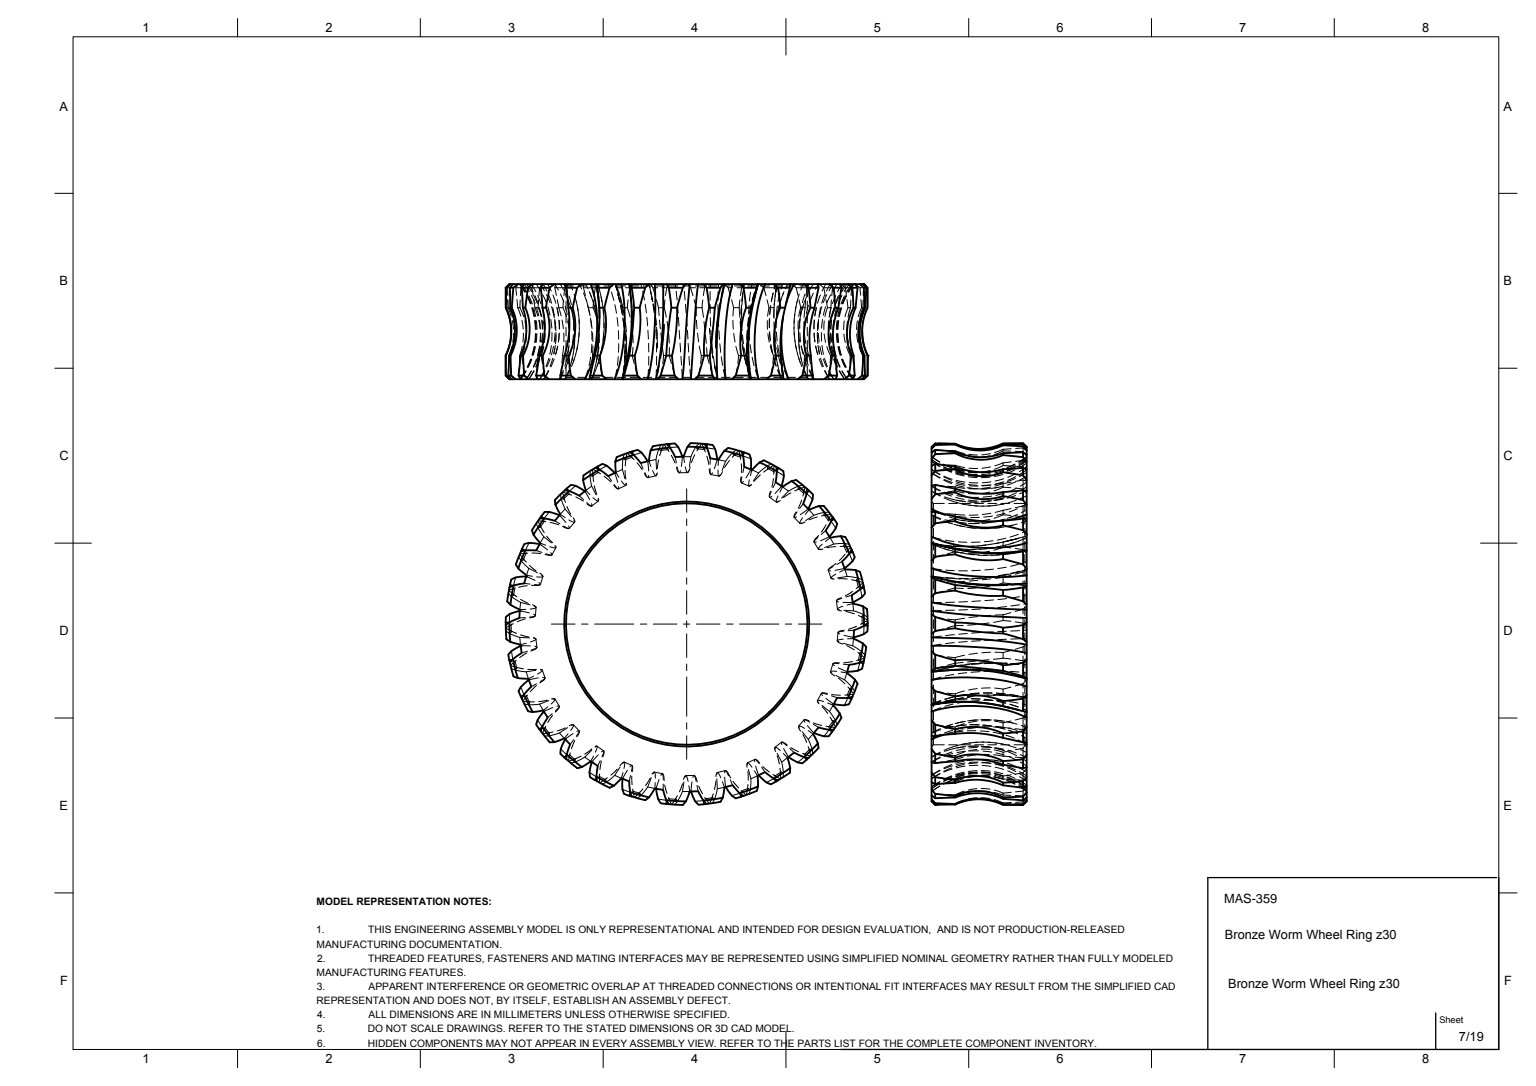
ISO-10303-21;
HEADER;
/* Generated by software containing ST-Developer
 * from STEP Tools, Inc. (www.steptools.com) 
 */

FILE_DESCRIPTION(
/* description */ (''),
/* implementation_level */ '2;1');

FILE_NAME(
/* name */ 'Bronze Worm Wheel Ring z30.step',
/* time_stamp */ '2026-10-15T14:25:16-07:00',
/* author */ (''),
/* organization */ (''),
/* preprocessor_version */ 'ST-DEVELOPER v20.2',
/* originating_system */ 'Autodesk Translation Framework v15.15.0.0',
/* authorisation */ '');

FILE_SCHEMA (('AUTOMOTIVE_DESIGN { 1 0 10303 214 3 1 1 }'));
ENDSEC;

DATA;
#10=MECHANICAL_DESIGN_GEOMETRIC_PRESENTATION_REPRESENTATION('',(#327),#86429);
#127=TOROIDAL_SURFACE('',#16553,6.3,1.5);
#128=TOROIDAL_SURFACE('',#16562,6.3,1.5);
#129=TOROIDAL_SURFACE('',#16571,6.3,1.5);
#130=TOROIDAL_SURFACE('',#16580,6.3,1.5);
#131=TOROIDAL_SURFACE('',#16589,6.3,1.5);
#132=TOROIDAL_SURFACE('',#16598,6.3,1.5);
#133=TOROIDAL_SURFACE('',#16607,6.3,1.5);
#134=TOROIDAL_SURFACE('',#16616,6.3,1.5);
#135=TOROIDAL_SURFACE('',#16625,6.3,1.5);
#136=TOROIDAL_SURFACE('',#16634,6.3,1.5);
#137=TOROIDAL_SURFACE('',#16643,6.3,1.5);
#138=TOROIDAL_SURFACE('',#16652,6.3,1.5);
#139=TOROIDAL_SURFACE('',#16661,6.3,1.5);
#140=TOROIDAL_SURFACE('',#16670,6.3,1.5);
#141=TOROIDAL_SURFACE('',#16679,6.3,1.5);
#142=TOROIDAL_SURFACE('',#16688,6.3,1.5);
#143=TOROIDAL_SURFACE('',#16697,6.3,1.5);
#144=TOROIDAL_SURFACE('',#16706,6.3,1.5);
#145=TOROIDAL_SURFACE('',#16715,6.3,1.5);
#146=TOROIDAL_SURFACE('',#16724,6.3,1.5);
#147=TOROIDAL_SURFACE('',#16733,6.3,1.5);
#148=TOROIDAL_SURFACE('',#16742,6.3,1.5);
#149=TOROIDAL_SURFACE('',#16751,6.3,1.5);
#150=TOROIDAL_SURFACE('',#16760,6.3,1.5);
#151=TOROIDAL_SURFACE('',#16769,6.3,1.5);
#152=TOROIDAL_SURFACE('',#16778,6.3,1.5);
#153=TOROIDAL_SURFACE('',#16787,6.3,1.5);
#154=TOROIDAL_SURFACE('',#16798,6.3,1.5);
#155=TOROIDAL_SURFACE('',#16811,6.3,1.5);
#156=TOROIDAL_SURFACE('',#16817,6.3,1.5);
#164=B_SPLINE_SURFACE_WITH_KNOTS('',3,3,((#29446,#29447,#29448,#29449,#29450,
#29451,#29452,#29453,#29454,#29455,#29456,#29457,#29458,#29459),(#29460,
#29461,#29462,#29463,#29464,#29465,#29466,#29467,#29468,#29469,#29470,#29471,
#29472,#29473),(#29474,#29475,#29476,#29477,#29478,#29479,#29480,#29481,
#29482,#29483,#29484,#29485,#29486,#29487),(#29488,#29489,#29490,#29491,
#29492,#29493,#29494,#29495,#29496,#29497,#29498,#29499,#29500,#29501),
(#29502,#29503,#29504,#29505,#29506,#29507,#29508,#29509,#29510,#29511,
#29512,#29513,#29514,#29515),(#29516,#29517,#29518,#29519,#29520,#29521,
#29522,#29523,#29524,#29525,#29526,#29527,#29528,#29529),(#29530,#29531,
#29532,#29533,#29534,#29535,#29536,#29537,#29538,#29539,#29540,#29541,#29542,
#29543),(#29544,#29545,#29546,#29547,#29548,#29549,#29550,#29551,#29552,
#29553,#29554,#29555,#29556,#29557),(#29558,#29559,#29560,#29561,#29562,
#29563,#29564,#29565,#29566,#29567,#29568,#29569,#29570,#29571),(#29572,
#29573,#29574,#29575,#29576,#29577,#29578,#29579,#29580,#29581,#29582,#29583,
#29584,#29585),(#29586,#29587,#29588,#29589,#29590,#29591,#29592,#29593,
#29594,#29595,#29596,#29597,#29598,#29599),(#29600,#29601,#29602,#29603,
#29604,#29605,#29606,#29607,#29608,#29609,#29610,#29611,#29612,#29613),
(#29614,#29615,#29616,#29617,#29618,#29619,#29620,#29621,#29622,#29623,
#29624,#29625,#29626,#29627),(#29628,#29629,#29630,#29631,#29632,#29633,
#29634,#29635,#29636,#29637,#29638,#29639,#29640,#29641),(#29642,#29643,
#29644,#29645,#29646,#29647,#29648,#29649,#29650,#29651,#29652,#29653,#29654,
#29655),(#29656,#29657,#29658,#29659,#29660,#29661,#29662,#29663,#29664,
#29665,#29666,#29667,#29668,#29669),(#29670,#29671,#29672,#29673,#29674,
#29675,#29676,#29677,#29678,#29679,#29680,#29681,#29682,#29683),(#29684,
#29685,#29686,#29687,#29688,#29689,#29690,#29691,#29692,#29693,#29694,#29695,
#29696,#29697),(#29698,#29699,#29700,#29701,#29702,#29703,#29704,#29705,
#29706,#29707,#29708,#29709,#29710,#29711),(#29712,#29713,#29714,#29715,
#29716,#29717,#29718,#29719,#29720,#29721,#29722,#29723,#29724,#29725),
(#29726,#29727,#29728,#29729,#29730,#29731,#29732,#29733,#29734,#29735,
#29736,#29737,#29738,#29739),(#29740,#29741,#29742,#29743,#29744,#29745,
#29746,#29747,#29748,#29749,#29750,#29751,#29752,#29753),(#29754,#29755,
#29756,#29757,#29758,#29759,#29760,#29761,#29762,#29763,#29764,#29765,#29766,
#29767),(#29768,#29769,#29770,#29771,#29772,#29773,#29774,#29775,#29776,
#29777,#29778,#29779,#29780,#29781),(#29782,#29783,#29784,#29785,#29786,
#29787,#29788,#29789,#29790,#29791,#29792,#29793,#29794,#29795),(#29796,
#29797,#29798,#29799,#29800,#29801,#29802,#29803,#29804,#29805,#29806,#29807,
#29808,#29809),(#29810,#29811,#29812,#29813,#29814,#29815,#29816,#29817,
#29818,#29819,#29820,#29821,#29822,#29823),(#29824,#29825,#29826,#29827,
#29828,#29829,#29830,#29831,#29832,#29833,#29834,#29835,#29836,#29837),
(#29838,#29839,#29840,#29841,#29842,#29843,#29844,#29845,#29846,#29847,
#29848,#29849,#29850,#29851),(#29852,#29853,#29854,#29855,#29856,#29857,
#29858,#29859,#29860,#29861,#29862,#29863,#29864,#29865),(#29866,#29867,
#29868,#29869,#29870,#29871,#29872,#29873,#29874,#29875,#29876,#29877,#29878,
#29879),(#29880,#29881,#29882,#29883,#29884,#29885,#29886,#29887,#29888,
#29889,#29890,#29891,#29892,#29893),(#29894,#29895,#29896,#29897,#29898,
#29899,#29900,#29901,#29902,#29903,#29904,#29905,#29906,#29907),(#29908,
#29909,#29910,#29911,#29912,#29913,#29914,#29915,#29916,#29917,#29918,#29919,
#29920,#29921)),.UNSPECIFIED.,.F.,.F.,.F.,(4,1,1,1,1,1,1,1,1,1,1,1,1,1,
1,1,1,1,1,1,1,1,1,1,1,1,1,1,1,1,1,4),(4,2,2,2,2,2,4),(0.0331549352864052,
0.102215297051662,0.171275658816919,0.172354726969501,0.173433795122083,
0.174512863274665,0.175591931427247,0.179908204037576,0.188540749258233,
0.19717329447889,0.205805839699547,0.223070930140861,0.240336020582176,
0.274866201464804,0.309396382347432,0.378456744112689,0.412986924995318,
0.447517105877946,0.482047286760574,0.516577467643203,0.551107648525831,
0.568372738967145,0.585637829408459,0.654698191173716,0.723758552938973,
0.79281891470423,0.827349095586858,0.861879276469487,0.896409457352115,
0.930939638234743,0.948204728676057,1.),(0.0377143719370964,0.167070624995476,
0.336553194126115,0.499999999999991,0.663446805873868,0.832929375004528,
0.962285628058762),.UNSPECIFIED.);
#165=B_SPLINE_SURFACE_WITH_KNOTS('',3,3,((#29982,#29983,#29984,#29985,#29986,
#29987,#29988,#29989,#29990,#29991,#29992,#29993,#29994,#29995),(#29996,
#29997,#29998,#29999,#30000,#30001,#30002,#30003,#30004,#30005,#30006,#30007,
#30008,#30009),(#30010,#30011,#30012,#30013,#30014,#30015,#30016,#30017,
#30018,#30019,#30020,#30021,#30022,#30023),(#30024,#30025,#30026,#30027,
#30028,#30029,#30030,#30031,#30032,#30033,#30034,#30035,#30036,#30037)),
 .UNSPECIFIED.,.F.,.F.,.F.,(4,4),(4,2,2,2,2,2,4),(0.,1.),(0.0377143719414207,
0.167070624995476,0.336553194126115,0.499999999999991,0.663446805873868,
0.832929375004528,0.962285628058582),.UNSPECIFIED.);
#166=B_SPLINE_SURFACE_WITH_KNOTS('',3,3,((#30052,#30053,#30054,#30055,#30056,
#30057,#30058,#30059,#30060,#30061,#30062,#30063,#30064,#30065),(#30066,
#30067,#30068,#30069,#30070,#30071,#30072,#30073,#30074,#30075,#30076,#30077,
#30078,#30079),(#30080,#30081,#30082,#30083,#30084,#30085,#30086,#30087,
#30088,#30089,#30090,#30091,#30092,#30093),(#30094,#30095,#30096,#30097,
#30098,#30099,#30100,#30101,#30102,#30103,#30104,#30105,#30106,#30107),
(#30108,#30109,#30110,#30111,#30112,#30113,#30114,#30115,#30116,#30117,
#30118,#30119,#30120,#30121),(#30122,#30123,#30124,#30125,#30126,#30127,
#30128,#30129,#30130,#30131,#30132,#30133,#30134,#30135),(#30136,#30137,
#30138,#30139,#30140,#30141,#30142,#30143,#30144,#30145,#30146,#30147,#30148,
#30149),(#30150,#30151,#30152,#30153,#30154,#30155,#30156,#30157,#30158,
#30159,#30160,#30161,#30162,#30163),(#30164,#30165,#30166,#30167,#30168,
#30169,#30170,#30171,#30172,#30173,#30174,#30175,#30176,#30177),(#30178,
#30179,#30180,#30181,#30182,#30183,#30184,#30185,#30186,#30187,#30188,#30189,
#30190,#30191),(#30192,#30193,#30194,#30195,#30196,#30197,#30198,#30199,
#30200,#30201,#30202,#30203,#30204,#30205),(#30206,#30207,#30208,#30209,
#30210,#30211,#30212,#30213,#30214,#30215,#30216,#30217,#30218,#30219),
(#30220,#30221,#30222,#30223,#30224,#30225,#30226,#30227,#30228,#30229,
#30230,#30231,#30232,#30233),(#30234,#30235,#30236,#30237,#30238,#30239,
#30240,#30241,#30242,#30243,#30244,#30245,#30246,#30247),(#30248,#30249,
#30250,#30251,#30252,#30253,#30254,#30255,#30256,#30257,#30258,#30259,#30260,
#30261),(#30262,#30263,#30264,#30265,#30266,#30267,#30268,#30269,#30270,
#30271,#30272,#30273,#30274,#30275),(#30276,#30277,#30278,#30279,#30280,
#30281,#30282,#30283,#30284,#30285,#30286,#30287,#30288,#30289),(#30290,
#30291,#30292,#30293,#30294,#30295,#30296,#30297,#30298,#30299,#30300,#30301,
#30302,#30303),(#30304,#30305,#30306,#30307,#30308,#30309,#30310,#30311,
#30312,#30313,#30314,#30315,#30316,#30317),(#30318,#30319,#30320,#30321,
#30322,#30323,#30324,#30325,#30326,#30327,#30328,#30329,#30330,#30331),
(#30332,#30333,#30334,#30335,#30336,#30337,#30338,#30339,#30340,#30341,
#30342,#30343,#30344,#30345),(#30346,#30347,#30348,#30349,#30350,#30351,
#30352,#30353,#30354,#30355,#30356,#30357,#30358,#30359),(#30360,#30361,
#30362,#30363,#30364,#30365,#30366,#30367,#30368,#30369,#30370,#30371,#30372,
#30373),(#30374,#30375,#30376,#30377,#30378,#30379,#30380,#30381,#30382,
#30383,#30384,#30385,#30386,#30387),(#30388,#30389,#30390,#30391,#30392,
#30393,#30394,#30395,#30396,#30397,#30398,#30399,#30400,#30401),(#30402,
#30403,#30404,#30405,#30406,#30407,#30408,#30409,#30410,#30411,#30412,#30413,
#30414,#30415),(#30416,#30417,#30418,#30419,#30420,#30421,#30422,#30423,
#30424,#30425,#30426,#30427,#30428,#30429),(#30430,#30431,#30432,#30433,
#30434,#30435,#30436,#30437,#30438,#30439,#30440,#30441,#30442,#30443),
(#30444,#30445,#30446,#30447,#30448,#30449,#30450,#30451,#30452,#30453,
#30454,#30455,#30456,#30457),(#30458,#30459,#30460,#30461,#30462,#30463,
#30464,#30465,#30466,#30467,#30468,#30469,#30470,#30471),(#30472,#30473,
#30474,#30475,#30476,#30477,#30478,#30479,#30480,#30481,#30482,#30483,#30484,
#30485),(#30486,#30487,#30488,#30489,#30490,#30491,#30492,#30493,#30494,
#30495,#30496,#30497,#30498,#30499),(#30500,#30501,#30502,#30503,#30504,
#30505,#30506,#30507,#30508,#30509,#30510,#30511,#30512,#30513),(#30514,
#30515,#30516,#30517,#30518,#30519,#30520,#30521,#30522,#30523,#30524,#30525,
#30526,#30527),(#30528,#30529,#30530,#30531,#30532,#30533,#30534,#30535,
#30536,#30537,#30538,#30539,#30540,#30541),(#30542,#30543,#30544,#30545,
#30546,#30547,#30548,#30549,#30550,#30551,#30552,#30553,#30554,#30555),
(#30556,#30557,#30558,#30559,#30560,#30561,#30562,#30563,#30564,#30565,
#30566,#30567,#30568,#30569)),.UNSPECIFIED.,.F.,.F.,.F.,(4,1,1,1,1,1,1,
1,1,1,1,1,1,1,1,1,1,1,1,1,1,1,1,1,1,1,1,1,1,1,1,1,1,1,4),(4,2,2,2,2,2,4),
(0.,0.0517952713240545,0.069060361765406,0.103590542648109,0.138120723530812,
0.146753268751488,0.155385813972164,0.189915994854866,0.276241447061624,
0.34530180882703,0.379831989709733,0.414362170592436,0.448892351475139,
0.46615744191649,0.483422532357842,0.552482894123248,0.587013075005951,
0.621543255888654,0.69060361765406,0.759663979419466,0.776929069860817,
0.794194160302169,0.802826705522845,0.81145925074352,0.815775523353858,
0.820091795964196,0.822249932269365,0.824408068574534,0.826566204879703,
0.827645273032287,0.82818480710858,0.828724341184872,0.897784702950278,
0.932314883832981,0.966845064715684),(0.037714371941,0.167070624995476,
0.336553194126115,0.499999999999991,0.663446805873868,0.832929375004528,
0.962285628058665),.UNSPECIFIED.);
#167=B_SPLINE_SURFACE_WITH_KNOTS('',3,3,((#30669,#30670,#30671,#30672,#30673,
#30674,#30675,#30676,#30677,#30678,#30679,#30680,#30681,#30682),(#30683,
#30684,#30685,#30686,#30687,#30688,#30689,#30690,#30691,#30692,#30693,#30694,
#30695,#30696),(#30697,#30698,#30699,#30700,#30701,#30702,#30703,#30704,
#30705,#30706,#30707,#30708,#30709,#30710),(#30711,#30712,#30713,#30714,
#30715,#30716,#30717,#30718,#30719,#30720,#30721,#30722,#30723,#30724),
(#30725,#30726,#30727,#30728,#30729,#30730,#30731,#30732,#30733,#30734,
#30735,#30736,#30737,#30738),(#30739,#30740,#30741,#30742,#30743,#30744,
#30745,#30746,#30747,#30748,#30749,#30750,#30751,#30752),(#30753,#30754,
#30755,#30756,#30757,#30758,#30759,#30760,#30761,#30762,#30763,#30764,#30765,
#30766),(#30767,#30768,#30769,#30770,#30771,#30772,#30773,#30774,#30775,
#30776,#30777,#30778,#30779,#30780),(#30781,#30782,#30783,#30784,#30785,
#30786,#30787,#30788,#30789,#30790,#30791,#30792,#30793,#30794),(#30795,
#30796,#30797,#30798,#30799,#30800,#30801,#30802,#30803,#30804,#30805,#30806,
#30807,#30808),(#30809,#30810,#30811,#30812,#30813,#30814,#30815,#30816,
#30817,#30818,#30819,#30820,#30821,#30822),(#30823,#30824,#30825,#30826,
#30827,#30828,#30829,#30830,#30831,#30832,#30833,#30834,#30835,#30836),
(#30837,#30838,#30839,#30840,#30841,#30842,#30843,#30844,#30845,#30846,
#30847,#30848,#30849,#30850),(#30851,#30852,#30853,#30854,#30855,#30856,
#30857,#30858,#30859,#30860,#30861,#30862,#30863,#30864),(#30865,#30866,
#30867,#30868,#30869,#30870,#30871,#30872,#30873,#30874,#30875,#30876,#30877,
#30878),(#30879,#30880,#30881,#30882,#30883,#30884,#30885,#30886,#30887,
#30888,#30889,#30890,#30891,#30892),(#30893,#30894,#30895,#30896,#30897,
#30898,#30899,#30900,#30901,#30902,#30903,#30904,#30905,#30906),(#30907,
#30908,#30909,#30910,#30911,#30912,#30913,#30914,#30915,#30916,#30917,#30918,
#30919,#30920),(#30921,#30922,#30923,#30924,#30925,#30926,#30927,#30928,
#30929,#30930,#30931,#30932,#30933,#30934),(#30935,#30936,#30937,#30938,
#30939,#30940,#30941,#30942,#30943,#30944,#30945,#30946,#30947,#30948),
(#30949,#30950,#30951,#30952,#30953,#30954,#30955,#30956,#30957,#30958,
#30959,#30960,#30961,#30962),(#30963,#30964,#30965,#30966,#30967,#30968,
#30969,#30970,#30971,#30972,#30973,#30974,#30975,#30976),(#30977,#30978,
#30979,#30980,#30981,#30982,#30983,#30984,#30985,#30986,#30987,#30988,#30989,
#30990),(#30991,#30992,#30993,#30994,#30995,#30996,#30997,#30998,#30999,
#31000,#31001,#31002,#31003,#31004),(#31005,#31006,#31007,#31008,#31009,
#31010,#31011,#31012,#31013,#31014,#31015,#31016,#31017,#31018),(#31019,
#31020,#31021,#31022,#31023,#31024,#31025,#31026,#31027,#31028,#31029,#31030,
#31031,#31032),(#31033,#31034,#31035,#31036,#31037,#31038,#31039,#31040,
#31041,#31042,#31043,#31044,#31045,#31046),(#31047,#31048,#31049,#31050,
#31051,#31052,#31053,#31054,#31055,#31056,#31057,#31058,#31059,#31060),
(#31061,#31062,#31063,#31064,#31065,#31066,#31067,#31068,#31069,#31070,
#31071,#31072,#31073,#31074),(#31075,#31076,#31077,#31078,#31079,#31080,
#31081,#31082,#31083,#31084,#31085,#31086,#31087,#31088),(#31089,#31090,
#31091,#31092,#31093,#31094,#31095,#31096,#31097,#31098,#31099,#31100,#31101,
#31102),(#31103,#31104,#31105,#31106,#31107,#31108,#31109,#31110,#31111,
#31112,#31113,#31114,#31115,#31116),(#31117,#31118,#31119,#31120,#31121,
#31122,#31123,#31124,#31125,#31126,#31127,#31128,#31129,#31130),(#31131,
#31132,#31133,#31134,#31135,#31136,#31137,#31138,#31139,#31140,#31141,#31142,
#31143,#31144),(#31145,#31146,#31147,#31148,#31149,#31150,#31151,#31152,
#31153,#31154,#31155,#31156,#31157,#31158),(#31159,#31160,#31161,#31162,
#31163,#31164,#31165,#31166,#31167,#31168,#31169,#31170,#31171,#31172)),
 .UNSPECIFIED.,.F.,.F.,.F.,(4,1,1,1,1,1,1,1,1,1,1,1,1,1,1,1,1,1,1,1,1,1,
1,1,1,1,1,1,1,1,1,1,1,4),(4,2,2,2,2,2,4),(0.033154935286399,0.0676851161690276,
0.102215297051656,0.171275658816913,0.172354726969496,0.173433795122078,
0.17451286327466,0.175591931427242,0.179908204037571,0.188540749258228,
0.197173294478885,0.205805839699542,0.223070930140856,0.240336020582171,
0.274866201464799,0.309396382347428,0.378456744112685,0.412986924995314,
0.447517105877942,0.482047286760571,0.5165774676432,0.551107648525828,0.568372738967142,
0.585637829408457,0.654698191173714,0.706493462497657,0.723758552938971,
0.792818914704228,0.827349095586857,0.861879276469486,0.896409457352114,
0.930939638234743,0.948204728676057,1.),(0.0377143719407808,0.167070624995476,
0.336553194126115,0.499999999999991,0.663446805873868,0.832929375004528,
0.962285628059334),.UNSPECIFIED.);
#168=B_SPLINE_SURFACE_WITH_KNOTS('',3,3,((#31237,#31238,#31239,#31240,#31241,
#31242,#31243,#31244,#31245,#31246,#31247,#31248,#31249,#31250),(#31251,
#31252,#31253,#31254,#31255,#31256,#31257,#31258,#31259,#31260,#31261,#31262,
#31263,#31264),(#31265,#31266,#31267,#31268,#31269,#31270,#31271,#31272,
#31273,#31274,#31275,#31276,#31277,#31278),(#31279,#31280,#31281,#31282,
#31283,#31284,#31285,#31286,#31287,#31288,#31289,#31290,#31291,#31292)),
 .UNSPECIFIED.,.F.,.F.,.F.,(4,4),(4,2,2,2,2,2,4),(0.,1.),(0.0377143719414207,
0.167070624995476,0.336553194126115,0.499999999999991,0.663446805873868,
0.832929375004528,0.962285628058582),.UNSPECIFIED.);
#169=B_SPLINE_SURFACE_WITH_KNOTS('',3,3,((#31307,#31308,#31309,#31310,#31311,
#31312,#31313,#31314,#31315,#31316,#31317,#31318,#31319,#31320),(#31321,
#31322,#31323,#31324,#31325,#31326,#31327,#31328,#31329,#31330,#31331,#31332,
#31333,#31334),(#31335,#31336,#31337,#31338,#31339,#31340,#31341,#31342,
#31343,#31344,#31345,#31346,#31347,#31348),(#31349,#31350,#31351,#31352,
#31353,#31354,#31355,#31356,#31357,#31358,#31359,#31360,#31361,#31362),
(#31363,#31364,#31365,#31366,#31367,#31368,#31369,#31370,#31371,#31372,
#31373,#31374,#31375,#31376),(#31377,#31378,#31379,#31380,#31381,#31382,
#31383,#31384,#31385,#31386,#31387,#31388,#31389,#31390),(#31391,#31392,
#31393,#31394,#31395,#31396,#31397,#31398,#31399,#31400,#31401,#31402,#31403,
#31404),(#31405,#31406,#31407,#31408,#31409,#31410,#31411,#31412,#31413,
#31414,#31415,#31416,#31417,#31418),(#31419,#31420,#31421,#31422,#31423,
#31424,#31425,#31426,#31427,#31428,#31429,#31430,#31431,#31432),(#31433,
#31434,#31435,#31436,#31437,#31438,#31439,#31440,#31441,#31442,#31443,#31444,
#31445,#31446),(#31447,#31448,#31449,#31450,#31451,#31452,#31453,#31454,
#31455,#31456,#31457,#31458,#31459,#31460),(#31461,#31462,#31463,#31464,
#31465,#31466,#31467,#31468,#31469,#31470,#31471,#31472,#31473,#31474),
(#31475,#31476,#31477,#31478,#31479,#31480,#31481,#31482,#31483,#31484,
#31485,#31486,#31487,#31488),(#31489,#31490,#31491,#31492,#31493,#31494,
#31495,#31496,#31497,#31498,#31499,#31500,#31501,#31502),(#31503,#31504,
#31505,#31506,#31507,#31508,#31509,#31510,#31511,#31512,#31513,#31514,#31515,
#31516),(#31517,#31518,#31519,#31520,#31521,#31522,#31523,#31524,#31525,
#31526,#31527,#31528,#31529,#31530),(#31531,#31532,#31533,#31534,#31535,
#31536,#31537,#31538,#31539,#31540,#31541,#31542,#31543,#31544),(#31545,
#31546,#31547,#31548,#31549,#31550,#31551,#31552,#31553,#31554,#31555,#31556,
#31557,#31558),(#31559,#31560,#31561,#31562,#31563,#31564,#31565,#31566,
#31567,#31568,#31569,#31570,#31571,#31572),(#31573,#31574,#31575,#31576,
#31577,#31578,#31579,#31580,#31581,#31582,#31583,#31584,#31585,#31586),
(#31587,#31588,#31589,#31590,#31591,#31592,#31593,#31594,#31595,#31596,
#31597,#31598,#31599,#31600),(#31601,#31602,#31603,#31604,#31605,#31606,
#31607,#31608,#31609,#31610,#31611,#31612,#31613,#31614),(#31615,#31616,
#31617,#31618,#31619,#31620,#31621,#31622,#31623,#31624,#31625,#31626,#31627,
#31628),(#31629,#31630,#31631,#31632,#31633,#31634,#31635,#31636,#31637,
#31638,#31639,#31640,#31641,#31642),(#31643,#31644,#31645,#31646,#31647,
#31648,#31649,#31650,#31651,#31652,#31653,#31654,#31655,#31656),(#31657,
#31658,#31659,#31660,#31661,#31662,#31663,#31664,#31665,#31666,#31667,#31668,
#31669,#31670),(#31671,#31672,#31673,#31674,#31675,#31676,#31677,#31678,
#31679,#31680,#31681,#31682,#31683,#31684),(#31685,#31686,#31687,#31688,
#31689,#31690,#31691,#31692,#31693,#31694,#31695,#31696,#31697,#31698),
(#31699,#31700,#31701,#31702,#31703,#31704,#31705,#31706,#31707,#31708,
#31709,#31710,#31711,#31712),(#31713,#31714,#31715,#31716,#31717,#31718,
#31719,#31720,#31721,#31722,#31723,#31724,#31725,#31726),(#31727,#31728,
#31729,#31730,#31731,#31732,#31733,#31734,#31735,#31736,#31737,#31738,#31739,
#31740),(#31741,#31742,#31743,#31744,#31745,#31746,#31747,#31748,#31749,
#31750,#31751,#31752,#31753,#31754),(#31755,#31756,#31757,#31758,#31759,
#31760,#31761,#31762,#31763,#31764,#31765,#31766,#31767,#31768),(#31769,
#31770,#31771,#31772,#31773,#31774,#31775,#31776,#31777,#31778,#31779,#31780,
#31781,#31782),(#31783,#31784,#31785,#31786,#31787,#31788,#31789,#31790,
#31791,#31792,#31793,#31794,#31795,#31796),(#31797,#31798,#31799,#31800,
#31801,#31802,#31803,#31804,#31805,#31806,#31807,#31808,#31809,#31810),
(#31811,#31812,#31813,#31814,#31815,#31816,#31817,#31818,#31819,#31820,
#31821,#31822,#31823,#31824),(#31825,#31826,#31827,#31828,#31829,#31830,
#31831,#31832,#31833,#31834,#31835,#31836,#31837,#31838),(#31839,#31840,
#31841,#31842,#31843,#31844,#31845,#31846,#31847,#31848,#31849,#31850,#31851,
#31852),(#31853,#31854,#31855,#31856,#31857,#31858,#31859,#31860,#31861,
#31862,#31863,#31864,#31865,#31866),(#31867,#31868,#31869,#31870,#31871,
#31872,#31873,#31874,#31875,#31876,#31877,#31878,#31879,#31880)),
 .UNSPECIFIED.,.F.,.F.,.F.,(4,1,1,1,1,1,1,1,1,1,1,1,1,1,1,1,1,1,1,1,1,1,
1,1,1,1,1,1,1,1,1,1,1,1,1,1,1,1,4),(4,2,2,2,2,2,4),(0.,0.0517952713240545,
0.069060361765406,0.103590542648109,0.138120723530812,0.155385813972164,
0.172650904413515,0.207181085296218,0.276241447061624,0.34530180882703,
0.379831989709733,0.414362170592436,0.448892351475139,0.483422532357842,
0.552482894123248,0.5697479845646,0.621543255888654,0.638808346330006,0.69060361765406,
0.707868708095412,0.716501253316088,0.725133798536763,0.759663979419467,
0.768296524640142,0.776929069860818,0.79419416030217,0.802826705522845,
0.811459250743521,0.820091795964197,0.824408068574535,0.825487136727119,
0.826566204879704,0.827645273032288,0.82818480710858,0.828454574146726,
0.828724341184873,0.897784702950279,0.932314883832982,0.966845064715685),
(0.0377143719412118,0.167070624995476,0.336553194126115,0.499999999999991,
0.663446805873868,0.832929375004528,0.962285628060063),.UNSPECIFIED.);
#170=B_SPLINE_SURFACE_WITH_KNOTS('',3,3,((#31940,#31941,#31942,#31943,#31944,
#31945,#31946,#31947,#31948,#31949,#31950,#31951,#31952,#31953),(#31954,
#31955,#31956,#31957,#31958,#31959,#31960,#31961,#31962,#31963,#31964,#31965,
#31966,#31967),(#31968,#31969,#31970,#31971,#31972,#31973,#31974,#31975,
#31976,#31977,#31978,#31979,#31980,#31981),(#31982,#31983,#31984,#31985,
#31986,#31987,#31988,#31989,#31990,#31991,#31992,#31993,#31994,#31995),
(#31996,#31997,#31998,#31999,#32000,#32001,#32002,#32003,#32004,#32005,
#32006,#32007,#32008,#32009),(#32010,#32011,#32012,#32013,#32014,#32015,
#32016,#32017,#32018,#32019,#32020,#32021,#32022,#32023),(#32024,#32025,
#32026,#32027,#32028,#32029,#32030,#32031,#32032,#32033,#32034,#32035,#32036,
#32037),(#32038,#32039,#32040,#32041,#32042,#32043,#32044,#32045,#32046,
#32047,#32048,#32049,#32050,#32051),(#32052,#32053,#32054,#32055,#32056,
#32057,#32058,#32059,#32060,#32061,#32062,#32063,#32064,#32065),(#32066,
#32067,#32068,#32069,#32070,#32071,#32072,#32073,#32074,#32075,#32076,#32077,
#32078,#32079),(#32080,#32081,#32082,#32083,#32084,#32085,#32086,#32087,
#32088,#32089,#32090,#32091,#32092,#32093),(#32094,#32095,#32096,#32097,
#32098,#32099,#32100,#32101,#32102,#32103,#32104,#32105,#32106,#32107),
(#32108,#32109,#32110,#32111,#32112,#32113,#32114,#32115,#32116,#32117,
#32118,#32119,#32120,#32121),(#32122,#32123,#32124,#32125,#32126,#32127,
#32128,#32129,#32130,#32131,#32132,#32133,#32134,#32135),(#32136,#32137,
#32138,#32139,#32140,#32141,#32142,#32143,#32144,#32145,#32146,#32147,#32148,
#32149),(#32150,#32151,#32152,#32153,#32154,#32155,#32156,#32157,#32158,
#32159,#32160,#32161,#32162,#32163),(#32164,#32165,#32166,#32167,#32168,
#32169,#32170,#32171,#32172,#32173,#32174,#32175,#32176,#32177),(#32178,
#32179,#32180,#32181,#32182,#32183,#32184,#32185,#32186,#32187,#32188,#32189,
#32190,#32191),(#32192,#32193,#32194,#32195,#32196,#32197,#32198,#32199,
#32200,#32201,#32202,#32203,#32204,#32205),(#32206,#32207,#32208,#32209,
#32210,#32211,#32212,#32213,#32214,#32215,#32216,#32217,#32218,#32219),
(#32220,#32221,#32222,#32223,#32224,#32225,#32226,#32227,#32228,#32229,
#32230,#32231,#32232,#32233),(#32234,#32235,#32236,#32237,#32238,#32239,
#32240,#32241,#32242,#32243,#32244,#32245,#32246,#32247),(#32248,#32249,
#32250,#32251,#32252,#32253,#32254,#32255,#32256,#32257,#32258,#32259,#32260,
#32261),(#32262,#32263,#32264,#32265,#32266,#32267,#32268,#32269,#32270,
#32271,#32272,#32273,#32274,#32275),(#32276,#32277,#32278,#32279,#32280,
#32281,#32282,#32283,#32284,#32285,#32286,#32287,#32288,#32289),(#32290,
#32291,#32292,#32293,#32294,#32295,#32296,#32297,#32298,#32299,#32300,#32301,
#32302,#32303),(#32304,#32305,#32306,#32307,#32308,#32309,#32310,#32311,
#32312,#32313,#32314,#32315,#32316,#32317),(#32318,#32319,#32320,#32321,
#32322,#32323,#32324,#32325,#32326,#32327,#32328,#32329,#32330,#32331),
(#32332,#32333,#32334,#32335,#32336,#32337,#32338,#32339,#32340,#32341,
#32342,#32343,#32344,#32345),(#32346,#32347,#32348,#32349,#32350,#32351,
#32352,#32353,#32354,#32355,#32356,#32357,#32358,#32359),(#32360,#32361,
#32362,#32363,#32364,#32365,#32366,#32367,#32368,#32369,#32370,#32371,#32372,
#32373),(#32374,#32375,#32376,#32377,#32378,#32379,#32380,#32381,#32382,
#32383,#32384,#32385,#32386,#32387),(#32388,#32389,#32390,#32391,#32392,
#32393,#32394,#32395,#32396,#32397,#32398,#32399,#32400,#32401),(#32402,
#32403,#32404,#32405,#32406,#32407,#32408,#32409,#32410,#32411,#32412,#32413,
#32414,#32415),(#32416,#32417,#32418,#32419,#32420,#32421,#32422,#32423,
#32424,#32425,#32426,#32427,#32428,#32429),(#32430,#32431,#32432,#32433,
#32434,#32435,#32436,#32437,#32438,#32439,#32440,#32441,#32442,#32443),
(#32444,#32445,#32446,#32447,#32448,#32449,#32450,#32451,#32452,#32453,
#32454,#32455,#32456,#32457)),.UNSPECIFIED.,.F.,.F.,.F.,(4,1,1,1,1,1,1,
1,1,1,1,1,1,1,1,1,1,1,1,1,1,1,1,1,1,1,1,1,1,1,1,1,1,1,4),(4,2,2,2,2,2,4),
(0.0331549352864065,0.0676851161690348,0.102215297051663,0.17127565881692,
0.171815192893211,0.172354726969502,0.172894261045793,0.173433795122084,
0.175591931427248,0.179908204037577,0.184224476647905,0.188540749258234,
0.205805839699548,0.223070930140862,0.240336020582177,0.274866201464805,
0.309396382347433,0.37845674411269,0.412986924995318,0.447517105877947,
0.482047286760575,0.516577467643203,0.551107648525831,0.568372738967146,
0.58563782940846,0.654698191173717,0.706493462497659,0.723758552938973,
0.79281891470423,0.827349095586858,0.861879276469487,0.896409457352115,
0.930939638234743,0.948204728676057,1.),(0.0377143719413302,0.167070624995476,
0.336553194126115,0.499999999999991,0.663446805873868,0.832929375004528,
0.962285628059334),.UNSPECIFIED.);
#171=B_SPLINE_SURFACE_WITH_KNOTS('',3,3,((#32522,#32523,#32524,#32525,#32526,
#32527,#32528,#32529,#32530,#32531,#32532,#32533,#32534,#32535),(#32536,
#32537,#32538,#32539,#32540,#32541,#32542,#32543,#32544,#32545,#32546,#32547,
#32548,#32549),(#32550,#32551,#32552,#32553,#32554,#32555,#32556,#32557,
#32558,#32559,#32560,#32561,#32562,#32563),(#32564,#32565,#32566,#32567,
#32568,#32569,#32570,#32571,#32572,#32573,#32574,#32575,#32576,#32577)),
 .UNSPECIFIED.,.F.,.F.,.F.,(4,4),(4,2,2,2,2,2,4),(0.,1.),(0.0377143719414212,
0.167070624995476,0.336553194126115,0.499999999999991,0.663446805873868,
0.832929375004528,0.962285628058582),.UNSPECIFIED.);
#172=B_SPLINE_SURFACE_WITH_KNOTS('',3,3,((#32592,#32593,#32594,#32595,#32596,
#32597,#32598,#32599,#32600,#32601,#32602,#32603,#32604,#32605),(#32606,
#32607,#32608,#32609,#32610,#32611,#32612,#32613,#32614,#32615,#32616,#32617,
#32618,#32619),(#32620,#32621,#32622,#32623,#32624,#32625,#32626,#32627,
#32628,#32629,#32630,#32631,#32632,#32633),(#32634,#32635,#32636,#32637,
#32638,#32639,#32640,#32641,#32642,#32643,#32644,#32645,#32646,#32647),
(#32648,#32649,#32650,#32651,#32652,#32653,#32654,#32655,#32656,#32657,
#32658,#32659,#32660,#32661),(#32662,#32663,#32664,#32665,#32666,#32667,
#32668,#32669,#32670,#32671,#32672,#32673,#32674,#32675),(#32676,#32677,
#32678,#32679,#32680,#32681,#32682,#32683,#32684,#32685,#32686,#32687,#32688,
#32689),(#32690,#32691,#32692,#32693,#32694,#32695,#32696,#32697,#32698,
#32699,#32700,#32701,#32702,#32703),(#32704,#32705,#32706,#32707,#32708,
#32709,#32710,#32711,#32712,#32713,#32714,#32715,#32716,#32717),(#32718,
#32719,#32720,#32721,#32722,#32723,#32724,#32725,#32726,#32727,#32728,#32729,
#32730,#32731),(#32732,#32733,#32734,#32735,#32736,#32737,#32738,#32739,
#32740,#32741,#32742,#32743,#32744,#32745),(#32746,#32747,#32748,#32749,
#32750,#32751,#32752,#32753,#32754,#32755,#32756,#32757,#32758,#32759),
(#32760,#32761,#32762,#32763,#32764,#32765,#32766,#32767,#32768,#32769,
#32770,#32771,#32772,#32773),(#32774,#32775,#32776,#32777,#32778,#32779,
#32780,#32781,#32782,#32783,#32784,#32785,#32786,#32787),(#32788,#32789,
#32790,#32791,#32792,#32793,#32794,#32795,#32796,#32797,#32798,#32799,#32800,
#32801),(#32802,#32803,#32804,#32805,#32806,#32807,#32808,#32809,#32810,
#32811,#32812,#32813,#32814,#32815),(#32816,#32817,#32818,#32819,#32820,
#32821,#32822,#32823,#32824,#32825,#32826,#32827,#32828,#32829),(#32830,
#32831,#32832,#32833,#32834,#32835,#32836,#32837,#32838,#32839,#32840,#32841,
#32842,#32843),(#32844,#32845,#32846,#32847,#32848,#32849,#32850,#32851,
#32852,#32853,#32854,#32855,#32856,#32857),(#32858,#32859,#32860,#32861,
#32862,#32863,#32864,#32865,#32866,#32867,#32868,#32869,#32870,#32871),
(#32872,#32873,#32874,#32875,#32876,#32877,#32878,#32879,#32880,#32881,
#32882,#32883,#32884,#32885),(#32886,#32887,#32888,#32889,#32890,#32891,
#32892,#32893,#32894,#32895,#32896,#32897,#32898,#32899),(#32900,#32901,
#32902,#32903,#32904,#32905,#32906,#32907,#32908,#32909,#32910,#32911,#32912,
#32913),(#32914,#32915,#32916,#32917,#32918,#32919,#32920,#32921,#32922,
#32923,#32924,#32925,#32926,#32927),(#32928,#32929,#32930,#32931,#32932,
#32933,#32934,#32935,#32936,#32937,#32938,#32939,#32940,#32941),(#32942,
#32943,#32944,#32945,#32946,#32947,#32948,#32949,#32950,#32951,#32952,#32953,
#32954,#32955),(#32956,#32957,#32958,#32959,#32960,#32961,#32962,#32963,
#32964,#32965,#32966,#32967,#32968,#32969),(#32970,#32971,#32972,#32973,
#32974,#32975,#32976,#32977,#32978,#32979,#32980,#32981,#32982,#32983),
(#32984,#32985,#32986,#32987,#32988,#32989,#32990,#32991,#32992,#32993,
#32994,#32995,#32996,#32997),(#32998,#32999,#33000,#33001,#33002,#33003,
#33004,#33005,#33006,#33007,#33008,#33009,#33010,#33011),(#33012,#33013,
#33014,#33015,#33016,#33017,#33018,#33019,#33020,#33021,#33022,#33023,#33024,
#33025),(#33026,#33027,#33028,#33029,#33030,#33031,#33032,#33033,#33034,
#33035,#33036,#33037,#33038,#33039),(#33040,#33041,#33042,#33043,#33044,
#33045,#33046,#33047,#33048,#33049,#33050,#33051,#33052,#33053),(#33054,
#33055,#33056,#33057,#33058,#33059,#33060,#33061,#33062,#33063,#33064,#33065,
#33066,#33067),(#33068,#33069,#33070,#33071,#33072,#33073,#33074,#33075,
#33076,#33077,#33078,#33079,#33080,#33081),(#33082,#33083,#33084,#33085,
#33086,#33087,#33088,#33089,#33090,#33091,#33092,#33093,#33094,#33095),
(#33096,#33097,#33098,#33099,#33100,#33101,#33102,#33103,#33104,#33105,
#33106,#33107,#33108,#33109),(#33110,#33111,#33112,#33113,#33114,#33115,
#33116,#33117,#33118,#33119,#33120,#33121,#33122,#33123),(#33124,#33125,
#33126,#33127,#33128,#33129,#33130,#33131,#33132,#33133,#33134,#33135,#33136,
#33137),(#33138,#33139,#33140,#33141,#33142,#33143,#33144,#33145,#33146,
#33147,#33148,#33149,#33150,#33151),(#33152,#33153,#33154,#33155,#33156,
#33157,#33158,#33159,#33160,#33161,#33162,#33163,#33164,#33165),(#33166,
#33167,#33168,#33169,#33170,#33171,#33172,#33173,#33174,#33175,#33176,#33177,
#33178,#33179),(#33180,#33181,#33182,#33183,#33184,#33185,#33186,#33187,
#33188,#33189,#33190,#33191,#33192,#33193),(#33194,#33195,#33196,#33197,
#33198,#33199,#33200,#33201,#33202,#33203,#33204,#33205,#33206,#33207),
(#33208,#33209,#33210,#33211,#33212,#33213,#33214,#33215,#33216,#33217,
#33218,#33219,#33220,#33221),(#33222,#33223,#33224,#33225,#33226,#33227,
#33228,#33229,#33230,#33231,#33232,#33233,#33234,#33235),(#33236,#33237,
#33238,#33239,#33240,#33241,#33242,#33243,#33244,#33245,#33246,#33247,#33248,
#33249)),.UNSPECIFIED.,.F.,.F.,.F.,(4,1,1,1,1,1,1,1,1,1,1,1,1,1,1,1,1,1,
1,1,1,1,1,1,1,1,1,1,1,1,1,1,1,1,1,1,1,1,1,1,1,1,1,1,4),(4,2,2,2,2,2,4),
(0.,0.0517952713240546,0.0690603617654062,0.103590542648109,0.138120723530812,
0.155385813972164,0.172650904413515,0.207181085296219,0.276241447061625,
0.345301808827031,0.379831989709734,0.414362170592437,0.422994715813113,
0.431627261033789,0.44889235147514,0.466157441916492,0.483422532357843,
0.552482894123249,0.621543255888656,0.656073436771359,0.690603617654062,
0.699236162874738,0.707868708095413,0.725133798536765,0.759663979419468,
0.77692906986082,0.785561615081495,0.789877887691833,0.794194160302171,
0.802826705522847,0.811459250743523,0.81577552335386,0.820091795964198,
0.824408068574536,0.826566204879705,0.827105738955997,0.82764527303229,
0.828184807108582,0.828454574146728,0.828589457665801,0.828724341184874,
0.880519612508929,0.89778470295028,0.932314883832983,0.966845064715687),
(0.0377143719413724,0.167070624995476,0.336553194126115,0.499999999999991,
0.663446805873868,0.832929375004528,0.96228562805881),.UNSPECIFIED.);
#173=B_SPLINE_SURFACE_WITH_KNOTS('',3,3,((#33305,#33306,#33307,#33308,#33309,
#33310,#33311,#33312,#33313,#33314,#33315,#33316,#33317,#33318),(#33319,
#33320,#33321,#33322,#33323,#33324,#33325,#33326,#33327,#33328,#33329,#33330,
#33331,#33332),(#33333,#33334,#33335,#33336,#33337,#33338,#33339,#33340,
#33341,#33342,#33343,#33344,#33345,#33346),(#33347,#33348,#33349,#33350,
#33351,#33352,#33353,#33354,#33355,#33356,#33357,#33358,#33359,#33360),
(#33361,#33362,#33363,#33364,#33365,#33366,#33367,#33368,#33369,#33370,
#33371,#33372,#33373,#33374),(#33375,#33376,#33377,#33378,#33379,#33380,
#33381,#33382,#33383,#33384,#33385,#33386,#33387,#33388),(#33389,#33390,
#33391,#33392,#33393,#33394,#33395,#33396,#33397,#33398,#33399,#33400,#33401,
#33402),(#33403,#33404,#33405,#33406,#33407,#33408,#33409,#33410,#33411,
#33412,#33413,#33414,#33415,#33416),(#33417,#33418,#33419,#33420,#33421,
#33422,#33423,#33424,#33425,#33426,#33427,#33428,#33429,#33430),(#33431,
#33432,#33433,#33434,#33435,#33436,#33437,#33438,#33439,#33440,#33441,#33442,
#33443,#33444),(#33445,#33446,#33447,#33448,#33449,#33450,#33451,#33452,
#33453,#33454,#33455,#33456,#33457,#33458),(#33459,#33460,#33461,#33462,
#33463,#33464,#33465,#33466,#33467,#33468,#33469,#33470,#33471,#33472),
(#33473,#33474,#33475,#33476,#33477,#33478,#33479,#33480,#33481,#33482,
#33483,#33484,#33485,#33486),(#33487,#33488,#33489,#33490,#33491,#33492,
#33493,#33494,#33495,#33496,#33497,#33498,#33499,#33500),(#33501,#33502,
#33503,#33504,#33505,#33506,#33507,#33508,#33509,#33510,#33511,#33512,#33513,
#33514),(#33515,#33516,#33517,#33518,#33519,#33520,#33521,#33522,#33523,
#33524,#33525,#33526,#33527,#33528),(#33529,#33530,#33531,#33532,#33533,
#33534,#33535,#33536,#33537,#33538,#33539,#33540,#33541,#33542),(#33543,
#33544,#33545,#33546,#33547,#33548,#33549,#33550,#33551,#33552,#33553,#33554,
#33555,#33556),(#33557,#33558,#33559,#33560,#33561,#33562,#33563,#33564,
#33565,#33566,#33567,#33568,#33569,#33570),(#33571,#33572,#33573,#33574,
#33575,#33576,#33577,#33578,#33579,#33580,#33581,#33582,#33583,#33584),
(#33585,#33586,#33587,#33588,#33589,#33590,#33591,#33592,#33593,#33594,
#33595,#33596,#33597,#33598),(#33599,#33600,#33601,#33602,#33603,#33604,
#33605,#33606,#33607,#33608,#33609,#33610,#33611,#33612),(#33613,#33614,
#33615,#33616,#33617,#33618,#33619,#33620,#33621,#33622,#33623,#33624,#33625,
#33626),(#33627,#33628,#33629,#33630,#33631,#33632,#33633,#33634,#33635,
#33636,#33637,#33638,#33639,#33640),(#33641,#33642,#33643,#33644,#33645,
#33646,#33647,#33648,#33649,#33650,#33651,#33652,#33653,#33654),(#33655,
#33656,#33657,#33658,#33659,#33660,#33661,#33662,#33663,#33664,#33665,#33666,
#33667,#33668),(#33669,#33670,#33671,#33672,#33673,#33674,#33675,#33676,
#33677,#33678,#33679,#33680,#33681,#33682),(#33683,#33684,#33685,#33686,
#33687,#33688,#33689,#33690,#33691,#33692,#33693,#33694,#33695,#33696),
(#33697,#33698,#33699,#33700,#33701,#33702,#33703,#33704,#33705,#33706,
#33707,#33708,#33709,#33710),(#33711,#33712,#33713,#33714,#33715,#33716,
#33717,#33718,#33719,#33720,#33721,#33722,#33723,#33724),(#33725,#33726,
#33727,#33728,#33729,#33730,#33731,#33732,#33733,#33734,#33735,#33736,#33737,
#33738),(#33739,#33740,#33741,#33742,#33743,#33744,#33745,#33746,#33747,
#33748,#33749,#33750,#33751,#33752),(#33753,#33754,#33755,#33756,#33757,
#33758,#33759,#33760,#33761,#33762,#33763,#33764,#33765,#33766),(#33767,
#33768,#33769,#33770,#33771,#33772,#33773,#33774,#33775,#33776,#33777,#33778,
#33779,#33780),(#33781,#33782,#33783,#33784,#33785,#33786,#33787,#33788,
#33789,#33790,#33791,#33792,#33793,#33794),(#33795,#33796,#33797,#33798,
#33799,#33800,#33801,#33802,#33803,#33804,#33805,#33806,#33807,#33808),
(#33809,#33810,#33811,#33812,#33813,#33814,#33815,#33816,#33817,#33818,
#33819,#33820,#33821,#33822),(#33823,#33824,#33825,#33826,#33827,#33828,
#33829,#33830,#33831,#33832,#33833,#33834,#33835,#33836),(#33837,#33838,
#33839,#33840,#33841,#33842,#33843,#33844,#33845,#33846,#33847,#33848,#33849,
#33850),(#33851,#33852,#33853,#33854,#33855,#33856,#33857,#33858,#33859,
#33860,#33861,#33862,#33863,#33864)),.UNSPECIFIED.,.F.,.F.,.F.,(4,1,1,1,
1,1,1,1,1,1,1,1,1,1,1,1,1,1,1,1,1,1,1,1,1,1,1,1,1,1,1,1,1,1,1,1,1,4),(4,
2,2,2,2,2,4),(0.0331549352864051,0.102215297051662,0.171275658816919,0.171545425855064,
0.17181519289321,0.172354726969501,0.173433795122083,0.174512863274665,
0.175591931427247,0.179908204037576,0.184224476647904,0.186382612953069,
0.188540749258233,0.19717329447889,0.205805839699547,0.214438384920204,
0.223070930140861,0.22738720275119,0.231703475361518,0.240336020582175,
0.309396382347432,0.343926563230061,0.378456744112689,0.447517105877946,
0.482047286760574,0.499312377201888,0.507944922422545,0.512261195032874,
0.516577467643203,0.585637829408459,0.723758552938973,0.79281891470423,
0.827349095586858,0.861879276469486,0.896409457352115,0.930939638234743,
0.948204728676057,1.),(0.0377143719413517,0.167070624995476,0.336553194126115,
0.499999999999991,0.663446805873868,0.832929375004528,0.96228562805941),
 .UNSPECIFIED.);
#174=B_SPLINE_SURFACE_WITH_KNOTS('',3,3,((#33923,#33924,#33925,#33926,#33927,
#33928,#33929,#33930,#33931,#33932,#33933,#33934,#33935,#33936),(#33937,
#33938,#33939,#33940,#33941,#33942,#33943,#33944,#33945,#33946,#33947,#33948,
#33949,#33950),(#33951,#33952,#33953,#33954,#33955,#33956,#33957,#33958,
#33959,#33960,#33961,#33962,#33963,#33964),(#33965,#33966,#33967,#33968,
#33969,#33970,#33971,#33972,#33973,#33974,#33975,#33976,#33977,#33978)),
 .UNSPECIFIED.,.F.,.F.,.F.,(4,4),(4,2,2,2,2,2,4),(0.,1.),(0.0377143719414209,
0.167070624995476,0.336553194126115,0.499999999999991,0.663446805873868,
0.832929375004528,0.962285628058582),.UNSPECIFIED.);
#175=B_SPLINE_SURFACE_WITH_KNOTS('',3,3,((#33993,#33994,#33995,#33996,#33997,
#33998,#33999,#34000,#34001,#34002,#34003,#34004,#34005,#34006),(#34007,
#34008,#34009,#34010,#34011,#34012,#34013,#34014,#34015,#34016,#34017,#34018,
#34019,#34020),(#34021,#34022,#34023,#34024,#34025,#34026,#34027,#34028,
#34029,#34030,#34031,#34032,#34033,#34034),(#34035,#34036,#34037,#34038,
#34039,#34040,#34041,#34042,#34043,#34044,#34045,#34046,#34047,#34048),
(#34049,#34050,#34051,#34052,#34053,#34054,#34055,#34056,#34057,#34058,
#34059,#34060,#34061,#34062),(#34063,#34064,#34065,#34066,#34067,#34068,
#34069,#34070,#34071,#34072,#34073,#34074,#34075,#34076),(#34077,#34078,
#34079,#34080,#34081,#34082,#34083,#34084,#34085,#34086,#34087,#34088,#34089,
#34090),(#34091,#34092,#34093,#34094,#34095,#34096,#34097,#34098,#34099,
#34100,#34101,#34102,#34103,#34104),(#34105,#34106,#34107,#34108,#34109,
#34110,#34111,#34112,#34113,#34114,#34115,#34116,#34117,#34118),(#34119,
#34120,#34121,#34122,#34123,#34124,#34125,#34126,#34127,#34128,#34129,#34130,
#34131,#34132),(#34133,#34134,#34135,#34136,#34137,#34138,#34139,#34140,
#34141,#34142,#34143,#34144,#34145,#34146),(#34147,#34148,#34149,#34150,
#34151,#34152,#34153,#34154,#34155,#34156,#34157,#34158,#34159,#34160),
(#34161,#34162,#34163,#34164,#34165,#34166,#34167,#34168,#34169,#34170,
#34171,#34172,#34173,#34174),(#34175,#34176,#34177,#34178,#34179,#34180,
#34181,#34182,#34183,#34184,#34185,#34186,#34187,#34188),(#34189,#34190,
#34191,#34192,#34193,#34194,#34195,#34196,#34197,#34198,#34199,#34200,#34201,
#34202),(#34203,#34204,#34205,#34206,#34207,#34208,#34209,#34210,#34211,
#34212,#34213,#34214,#34215,#34216),(#34217,#34218,#34219,#34220,#34221,
#34222,#34223,#34224,#34225,#34226,#34227,#34228,#34229,#34230),(#34231,
#34232,#34233,#34234,#34235,#34236,#34237,#34238,#34239,#34240,#34241,#34242,
#34243,#34244),(#34245,#34246,#34247,#34248,#34249,#34250,#34251,#34252,
#34253,#34254,#34255,#34256,#34257,#34258),(#34259,#34260,#34261,#34262,
#34263,#34264,#34265,#34266,#34267,#34268,#34269,#34270,#34271,#34272),
(#34273,#34274,#34275,#34276,#34277,#34278,#34279,#34280,#34281,#34282,
#34283,#34284,#34285,#34286),(#34287,#34288,#34289,#34290,#34291,#34292,
#34293,#34294,#34295,#34296,#34297,#34298,#34299,#34300),(#34301,#34302,
#34303,#34304,#34305,#34306,#34307,#34308,#34309,#34310,#34311,#34312,#34313,
#34314),(#34315,#34316,#34317,#34318,#34319,#34320,#34321,#34322,#34323,
#34324,#34325,#34326,#34327,#34328),(#34329,#34330,#34331,#34332,#34333,
#34334,#34335,#34336,#34337,#34338,#34339,#34340,#34341,#34342),(#34343,
#34344,#34345,#34346,#34347,#34348,#34349,#34350,#34351,#34352,#34353,#34354,
#34355,#34356),(#34357,#34358,#34359,#34360,#34361,#34362,#34363,#34364,
#34365,#34366,#34367,#34368,#34369,#34370),(#34371,#34372,#34373,#34374,
#34375,#34376,#34377,#34378,#34379,#34380,#34381,#34382,#34383,#34384),
(#34385,#34386,#34387,#34388,#34389,#34390,#34391,#34392,#34393,#34394,
#34395,#34396,#34397,#34398),(#34399,#34400,#34401,#34402,#34403,#34404,
#34405,#34406,#34407,#34408,#34409,#34410,#34411,#34412),(#34413,#34414,
#34415,#34416,#34417,#34418,#34419,#34420,#34421,#34422,#34423,#34424,#34425,
#34426),(#34427,#34428,#34429,#34430,#34431,#34432,#34433,#34434,#34435,
#34436,#34437,#34438,#34439,#34440)),.UNSPECIFIED.,.F.,.F.,.F.,(4,1,1,1,
1,1,1,1,1,1,1,1,1,1,1,1,1,1,1,1,1,1,1,1,1,1,1,1,1,4),(4,2,2,2,2,2,4),(0.,
0.0517952713240544,0.0690603617654059,0.103590542648109,0.138120723530812,
0.155385813972163,0.189915994854866,0.276241447061624,0.310771627944327,
0.345301808827029,0.379831989709732,0.397097080151084,0.40572962537176,
0.414362170592435,0.483422532357841,0.552482894123247,0.621543255888653,
0.64744089155068,0.690603617654059,0.725133798536762,0.759663979419465,
0.776929069860816,0.794194160302168,0.811459250743519,0.820091795964195,
0.824408068574533,0.826566204879702,0.828724341184871,0.897784702950277,
0.966845064715683),(0.0377143719413786,0.167070624995476,0.336553194126115,
0.499999999999991,0.663446805873868,0.832929375004528,0.96228562805878),
 .UNSPECIFIED.);
#176=B_SPLINE_SURFACE_WITH_KNOTS('',3,3,((#34496,#34497,#34498,#34499,#34500,
#34501,#34502,#34503,#34504,#34505,#34506,#34507,#34508,#34509),(#34510,
#34511,#34512,#34513,#34514,#34515,#34516,#34517,#34518,#34519,#34520,#34521,
#34522,#34523),(#34524,#34525,#34526,#34527,#34528,#34529,#34530,#34531,
#34532,#34533,#34534,#34535,#34536,#34537),(#34538,#34539,#34540,#34541,
#34542,#34543,#34544,#34545,#34546,#34547,#34548,#34549,#34550,#34551),
(#34552,#34553,#34554,#34555,#34556,#34557,#34558,#34559,#34560,#34561,
#34562,#34563,#34564,#34565),(#34566,#34567,#34568,#34569,#34570,#34571,
#34572,#34573,#34574,#34575,#34576,#34577,#34578,#34579),(#34580,#34581,
#34582,#34583,#34584,#34585,#34586,#34587,#34588,#34589,#34590,#34591,#34592,
#34593),(#34594,#34595,#34596,#34597,#34598,#34599,#34600,#34601,#34602,
#34603,#34604,#34605,#34606,#34607),(#34608,#34609,#34610,#34611,#34612,
#34613,#34614,#34615,#34616,#34617,#34618,#34619,#34620,#34621),(#34622,
#34623,#34624,#34625,#34626,#34627,#34628,#34629,#34630,#34631,#34632,#34633,
#34634,#34635),(#34636,#34637,#34638,#34639,#34640,#34641,#34642,#34643,
#34644,#34645,#34646,#34647,#34648,#34649),(#34650,#34651,#34652,#34653,
#34654,#34655,#34656,#34657,#34658,#34659,#34660,#34661,#34662,#34663),
(#34664,#34665,#34666,#34667,#34668,#34669,#34670,#34671,#34672,#34673,
#34674,#34675,#34676,#34677),(#34678,#34679,#34680,#34681,#34682,#34683,
#34684,#34685,#34686,#34687,#34688,#34689,#34690,#34691),(#34692,#34693,
#34694,#34695,#34696,#34697,#34698,#34699,#34700,#34701,#34702,#34703,#34704,
#34705),(#34706,#34707,#34708,#34709,#34710,#34711,#34712,#34713,#34714,
#34715,#34716,#34717,#34718,#34719),(#34720,#34721,#34722,#34723,#34724,
#34725,#34726,#34727,#34728,#34729,#34730,#34731,#34732,#34733),(#34734,
#34735,#34736,#34737,#34738,#34739,#34740,#34741,#34742,#34743,#34744,#34745,
#34746,#34747),(#34748,#34749,#34750,#34751,#34752,#34753,#34754,#34755,
#34756,#34757,#34758,#34759,#34760,#34761),(#34762,#34763,#34764,#34765,
#34766,#34767,#34768,#34769,#34770,#34771,#34772,#34773,#34774,#34775),
(#34776,#34777,#34778,#34779,#34780,#34781,#34782,#34783,#34784,#34785,
#34786,#34787,#34788,#34789),(#34790,#34791,#34792,#34793,#34794,#34795,
#34796,#34797,#34798,#34799,#34800,#34801,#34802,#34803),(#34804,#34805,
#34806,#34807,#34808,#34809,#34810,#34811,#34812,#34813,#34814,#34815,#34816,
#34817),(#34818,#34819,#34820,#34821,#34822,#34823,#34824,#34825,#34826,
#34827,#34828,#34829,#34830,#34831),(#34832,#34833,#34834,#34835,#34836,
#34837,#34838,#34839,#34840,#34841,#34842,#34843,#34844,#34845),(#34846,
#34847,#34848,#34849,#34850,#34851,#34852,#34853,#34854,#34855,#34856,#34857,
#34858,#34859),(#34860,#34861,#34862,#34863,#34864,#34865,#34866,#34867,
#34868,#34869,#34870,#34871,#34872,#34873),(#34874,#34875,#34876,#34877,
#34878,#34879,#34880,#34881,#34882,#34883,#34884,#34885,#34886,#34887),
(#34888,#34889,#34890,#34891,#34892,#34893,#34894,#34895,#34896,#34897,
#34898,#34899,#34900,#34901),(#34902,#34903,#34904,#34905,#34906,#34907,
#34908,#34909,#34910,#34911,#34912,#34913,#34914,#34915),(#34916,#34917,
#34918,#34919,#34920,#34921,#34922,#34923,#34924,#34925,#34926,#34927,#34928,
#34929),(#34930,#34931,#34932,#34933,#34934,#34935,#34936,#34937,#34938,
#34939,#34940,#34941,#34942,#34943),(#34944,#34945,#34946,#34947,#34948,
#34949,#34950,#34951,#34952,#34953,#34954,#34955,#34956,#34957),(#34958,
#34959,#34960,#34961,#34962,#34963,#34964,#34965,#34966,#34967,#34968,#34969,
#34970,#34971),(#34972,#34973,#34974,#34975,#34976,#34977,#34978,#34979,
#34980,#34981,#34982,#34983,#34984,#34985),(#34986,#34987,#34988,#34989,
#34990,#34991,#34992,#34993,#34994,#34995,#34996,#34997,#34998,#34999),
(#35000,#35001,#35002,#35003,#35004,#35005,#35006,#35007,#35008,#35009,
#35010,#35011,#35012,#35013),(#35014,#35015,#35016,#35017,#35018,#35019,
#35020,#35021,#35022,#35023,#35024,#35025,#35026,#35027),(#35028,#35029,
#35030,#35031,#35032,#35033,#35034,#35035,#35036,#35037,#35038,#35039,#35040,
#35041),(#35042,#35043,#35044,#35045,#35046,#35047,#35048,#35049,#35050,
#35051,#35052,#35053,#35054,#35055),(#35056,#35057,#35058,#35059,#35060,
#35061,#35062,#35063,#35064,#35065,#35066,#35067,#35068,#35069),(#35070,
#35071,#35072,#35073,#35074,#35075,#35076,#35077,#35078,#35079,#35080,#35081,
#35082,#35083),(#35084,#35085,#35086,#35087,#35088,#35089,#35090,#35091,
#35092,#35093,#35094,#35095,#35096,#35097),(#35098,#35099,#35100,#35101,
#35102,#35103,#35104,#35105,#35106,#35107,#35108,#35109,#35110,#35111),
(#35112,#35113,#35114,#35115,#35116,#35117,#35118,#35119,#35120,#35121,
#35122,#35123,#35124,#35125),(#35126,#35127,#35128,#35129,#35130,#35131,
#35132,#35133,#35134,#35135,#35136,#35137,#35138,#35139),(#35140,#35141,
#35142,#35143,#35144,#35145,#35146,#35147,#35148,#35149,#35150,#35151,#35152,
#35153)),.UNSPECIFIED.,.F.,.F.,.F.,(4,1,1,1,1,1,1,1,1,1,1,1,1,1,1,1,1,1,
1,1,1,1,1,1,1,1,1,1,1,1,1,1,1,1,1,1,1,1,1,1,1,1,1,1,4),(4,2,2,2,2,2,4),
(0.0331549352864063,0.0676851161690347,0.102215297051663,0.136745477934291,
0.17127565881692,0.171545425855065,0.171815192893211,0.172084959931356,
0.172354726969502,0.173433795122084,0.175591931427248,0.177750067732413,
0.179908204037577,0.184224476647905,0.188540749258234,0.205805839699548,
0.223070930140862,0.227387202751191,0.231703475361519,0.240336020582176,
0.274866201464805,0.292131291906119,0.309396382347433,0.343926563230061,
0.37845674411269,0.412986924995318,0.430252015436632,0.447517105877946,
0.516577467643203,0.551107648525831,0.58563782940846,0.620168010291088,
0.654698191173717,0.671963281615031,0.723758552938973,0.79281891470423,
0.827349095586858,0.844614186028172,0.853246731248829,0.861879276469487,
0.896409457352115,0.930939638234743,0.948204728676057,0.965469819117372,
1.),(0.0377143719413899,0.167070624995476,0.336553194126115,0.499999999999991,
0.663446805873868,0.832929375004528,0.96228562805941),.UNSPECIFIED.);
#177=B_SPLINE_SURFACE_WITH_KNOTS('',3,3,((#35212,#35213,#35214,#35215,#35216,
#35217,#35218,#35219,#35220,#35221,#35222,#35223,#35224,#35225),(#35226,
#35227,#35228,#35229,#35230,#35231,#35232,#35233,#35234,#35235,#35236,#35237,
#35238,#35239),(#35240,#35241,#35242,#35243,#35244,#35245,#35246,#35247,
#35248,#35249,#35250,#35251,#35252,#35253),(#35254,#35255,#35256,#35257,
#35258,#35259,#35260,#35261,#35262,#35263,#35264,#35265,#35266,#35267)),
 .UNSPECIFIED.,.F.,.F.,.F.,(4,4),(4,2,2,2,2,2,4),(0.,1.),(0.0377143719414212,
0.167070624995476,0.336553194126115,0.499999999999991,0.663446805873868,
0.832929375004528,0.962285628058582),.UNSPECIFIED.);
#178=B_SPLINE_SURFACE_WITH_KNOTS('',3,3,((#35282,#35283,#35284,#35285,#35286,
#35287,#35288,#35289,#35290,#35291,#35292,#35293,#35294,#35295),(#35296,
#35297,#35298,#35299,#35300,#35301,#35302,#35303,#35304,#35305,#35306,#35307,
#35308,#35309),(#35310,#35311,#35312,#35313,#35314,#35315,#35316,#35317,
#35318,#35319,#35320,#35321,#35322,#35323),(#35324,#35325,#35326,#35327,
#35328,#35329,#35330,#35331,#35332,#35333,#35334,#35335,#35336,#35337),
(#35338,#35339,#35340,#35341,#35342,#35343,#35344,#35345,#35346,#35347,
#35348,#35349,#35350,#35351),(#35352,#35353,#35354,#35355,#35356,#35357,
#35358,#35359,#35360,#35361,#35362,#35363,#35364,#35365),(#35366,#35367,
#35368,#35369,#35370,#35371,#35372,#35373,#35374,#35375,#35376,#35377,#35378,
#35379),(#35380,#35381,#35382,#35383,#35384,#35385,#35386,#35387,#35388,
#35389,#35390,#35391,#35392,#35393),(#35394,#35395,#35396,#35397,#35398,
#35399,#35400,#35401,#35402,#35403,#35404,#35405,#35406,#35407),(#35408,
#35409,#35410,#35411,#35412,#35413,#35414,#35415,#35416,#35417,#35418,#35419,
#35420,#35421),(#35422,#35423,#35424,#35425,#35426,#35427,#35428,#35429,
#35430,#35431,#35432,#35433,#35434,#35435),(#35436,#35437,#35438,#35439,
#35440,#35441,#35442,#35443,#35444,#35445,#35446,#35447,#35448,#35449),
(#35450,#35451,#35452,#35453,#35454,#35455,#35456,#35457,#35458,#35459,
#35460,#35461,#35462,#35463),(#35464,#35465,#35466,#35467,#35468,#35469,
#35470,#35471,#35472,#35473,#35474,#35475,#35476,#35477),(#35478,#35479,
#35480,#35481,#35482,#35483,#35484,#35485,#35486,#35487,#35488,#35489,#35490,
#35491),(#35492,#35493,#35494,#35495,#35496,#35497,#35498,#35499,#35500,
#35501,#35502,#35503,#35504,#35505),(#35506,#35507,#35508,#35509,#35510,
#35511,#35512,#35513,#35514,#35515,#35516,#35517,#35518,#35519),(#35520,
#35521,#35522,#35523,#35524,#35525,#35526,#35527,#35528,#35529,#35530,#35531,
#35532,#35533),(#35534,#35535,#35536,#35537,#35538,#35539,#35540,#35541,
#35542,#35543,#35544,#35545,#35546,#35547),(#35548,#35549,#35550,#35551,
#35552,#35553,#35554,#35555,#35556,#35557,#35558,#35559,#35560,#35561),
(#35562,#35563,#35564,#35565,#35566,#35567,#35568,#35569,#35570,#35571,
#35572,#35573,#35574,#35575),(#35576,#35577,#35578,#35579,#35580,#35581,
#35582,#35583,#35584,#35585,#35586,#35587,#35588,#35589),(#35590,#35591,
#35592,#35593,#35594,#35595,#35596,#35597,#35598,#35599,#35600,#35601,#35602,
#35603),(#35604,#35605,#35606,#35607,#35608,#35609,#35610,#35611,#35612,
#35613,#35614,#35615,#35616,#35617),(#35618,#35619,#35620,#35621,#35622,
#35623,#35624,#35625,#35626,#35627,#35628,#35629,#35630,#35631),(#35632,
#35633,#35634,#35635,#35636,#35637,#35638,#35639,#35640,#35641,#35642,#35643,
#35644,#35645),(#35646,#35647,#35648,#35649,#35650,#35651,#35652,#35653,
#35654,#35655,#35656,#35657,#35658,#35659),(#35660,#35661,#35662,#35663,
#35664,#35665,#35666,#35667,#35668,#35669,#35670,#35671,#35672,#35673),
(#35674,#35675,#35676,#35677,#35678,#35679,#35680,#35681,#35682,#35683,
#35684,#35685,#35686,#35687),(#35688,#35689,#35690,#35691,#35692,#35693,
#35694,#35695,#35696,#35697,#35698,#35699,#35700,#35701),(#35702,#35703,
#35704,#35705,#35706,#35707,#35708,#35709,#35710,#35711,#35712,#35713,#35714,
#35715),(#35716,#35717,#35718,#35719,#35720,#35721,#35722,#35723,#35724,
#35725,#35726,#35727,#35728,#35729)),.UNSPECIFIED.,.F.,.F.,.F.,(4,1,1,1,
1,1,1,1,1,1,1,1,1,1,1,1,1,1,1,1,1,1,1,1,1,1,1,1,1,4),(4,2,2,2,2,2,4),(0.,
0.0517952713240546,0.0690603617654061,0.103590542648109,0.138120723530812,
0.155385813972164,0.189915994854867,0.276241447061625,0.310771627944328,
0.345301808827031,0.379831989709734,0.397097080151085,0.405729625371761,
0.414362170592437,0.483422532357843,0.552482894123249,0.621543255888655,
0.647440891550682,0.690603617654061,0.725133798536764,0.759663979419467,
0.776929069860819,0.79419416030217,0.811459250743522,0.820091795964198,
0.824408068574536,0.826566204879705,0.828724341184873,0.89778470295028,
0.966845064715686),(0.0377143719408444,0.167070624995476,0.336553194126115,
0.499999999999991,0.663446805873868,0.832929375004528,0.962285628060942),
 .UNSPECIFIED.);
#179=B_SPLINE_SURFACE_WITH_KNOTS('',3,3,((#35785,#35786,#35787,#35788,#35789,
#35790,#35791,#35792,#35793,#35794,#35795,#35796,#35797,#35798),(#35799,
#35800,#35801,#35802,#35803,#35804,#35805,#35806,#35807,#35808,#35809,#35810,
#35811,#35812),(#35813,#35814,#35815,#35816,#35817,#35818,#35819,#35820,
#35821,#35822,#35823,#35824,#35825,#35826),(#35827,#35828,#35829,#35830,
#35831,#35832,#35833,#35834,#35835,#35836,#35837,#35838,#35839,#35840),
(#35841,#35842,#35843,#35844,#35845,#35846,#35847,#35848,#35849,#35850,
#35851,#35852,#35853,#35854),(#35855,#35856,#35857,#35858,#35859,#35860,
#35861,#35862,#35863,#35864,#35865,#35866,#35867,#35868),(#35869,#35870,
#35871,#35872,#35873,#35874,#35875,#35876,#35877,#35878,#35879,#35880,#35881,
#35882),(#35883,#35884,#35885,#35886,#35887,#35888,#35889,#35890,#35891,
#35892,#35893,#35894,#35895,#35896),(#35897,#35898,#35899,#35900,#35901,
#35902,#35903,#35904,#35905,#35906,#35907,#35908,#35909,#35910),(#35911,
#35912,#35913,#35914,#35915,#35916,#35917,#35918,#35919,#35920,#35921,#35922,
#35923,#35924),(#35925,#35926,#35927,#35928,#35929,#35930,#35931,#35932,
#35933,#35934,#35935,#35936,#35937,#35938),(#35939,#35940,#35941,#35942,
#35943,#35944,#35945,#35946,#35947,#35948,#35949,#35950,#35951,#35952),
(#35953,#35954,#35955,#35956,#35957,#35958,#35959,#35960,#35961,#35962,
#35963,#35964,#35965,#35966),(#35967,#35968,#35969,#35970,#35971,#35972,
#35973,#35974,#35975,#35976,#35977,#35978,#35979,#35980),(#35981,#35982,
#35983,#35984,#35985,#35986,#35987,#35988,#35989,#35990,#35991,#35992,#35993,
#35994),(#35995,#35996,#35997,#35998,#35999,#36000,#36001,#36002,#36003,
#36004,#36005,#36006,#36007,#36008),(#36009,#36010,#36011,#36012,#36013,
#36014,#36015,#36016,#36017,#36018,#36019,#36020,#36021,#36022),(#36023,
#36024,#36025,#36026,#36027,#36028,#36029,#36030,#36031,#36032,#36033,#36034,
#36035,#36036),(#36037,#36038,#36039,#36040,#36041,#36042,#36043,#36044,
#36045,#36046,#36047,#36048,#36049,#36050),(#36051,#36052,#36053,#36054,
#36055,#36056,#36057,#36058,#36059,#36060,#36061,#36062,#36063,#36064),
(#36065,#36066,#36067,#36068,#36069,#36070,#36071,#36072,#36073,#36074,
#36075,#36076,#36077,#36078),(#36079,#36080,#36081,#36082,#36083,#36084,
#36085,#36086,#36087,#36088,#36089,#36090,#36091,#36092),(#36093,#36094,
#36095,#36096,#36097,#36098,#36099,#36100,#36101,#36102,#36103,#36104,#36105,
#36106),(#36107,#36108,#36109,#36110,#36111,#36112,#36113,#36114,#36115,
#36116,#36117,#36118,#36119,#36120),(#36121,#36122,#36123,#36124,#36125,
#36126,#36127,#36128,#36129,#36130,#36131,#36132,#36133,#36134),(#36135,
#36136,#36137,#36138,#36139,#36140,#36141,#36142,#36143,#36144,#36145,#36146,
#36147,#36148),(#36149,#36150,#36151,#36152,#36153,#36154,#36155,#36156,
#36157,#36158,#36159,#36160,#36161,#36162),(#36163,#36164,#36165,#36166,
#36167,#36168,#36169,#36170,#36171,#36172,#36173,#36174,#36175,#36176),
(#36177,#36178,#36179,#36180,#36181,#36182,#36183,#36184,#36185,#36186,
#36187,#36188,#36189,#36190),(#36191,#36192,#36193,#36194,#36195,#36196,
#36197,#36198,#36199,#36200,#36201,#36202,#36203,#36204),(#36205,#36206,
#36207,#36208,#36209,#36210,#36211,#36212,#36213,#36214,#36215,#36216,#36217,
#36218),(#36219,#36220,#36221,#36222,#36223,#36224,#36225,#36226,#36227,
#36228,#36229,#36230,#36231,#36232),(#36233,#36234,#36235,#36236,#36237,
#36238,#36239,#36240,#36241,#36242,#36243,#36244,#36245,#36246),(#36247,
#36248,#36249,#36250,#36251,#36252,#36253,#36254,#36255,#36256,#36257,#36258,
#36259,#36260)),.UNSPECIFIED.,.F.,.F.,.F.,(4,1,1,1,1,1,1,1,1,1,1,1,1,1,
1,1,1,1,1,1,1,1,1,1,1,1,1,1,1,1,1,4),(4,2,2,2,2,2,4),(0.0331549352864075,
0.102215297051664,0.171275658816921,0.172354726969503,0.173433795122085,
0.174512863274667,0.175591931427249,0.179908204037578,0.188540749258235,
0.201489567089221,0.205805839699549,0.223070930140863,0.240336020582177,
0.274866201464806,0.309396382347434,0.378456744112691,0.412986924995319,
0.447517105877947,0.482047286760576,0.516577467643204,0.551107648525832,
0.568372738967146,0.58563782940846,0.654698191173717,0.723758552938974,
0.79281891470423,0.827349095586859,0.861879276469487,0.896409457352115,
0.930939638234743,0.948204728676058,1.),(0.0377143719407316,0.167070624995476,
0.336553194126115,0.499999999999991,0.663446805873868,0.832929375004528,
0.962285628058715),.UNSPECIFIED.);
#180=B_SPLINE_SURFACE_WITH_KNOTS('',3,3,((#36323,#36324,#36325,#36326,#36327,
#36328,#36329,#36330,#36331,#36332,#36333,#36334,#36335,#36336),(#36337,
#36338,#36339,#36340,#36341,#36342,#36343,#36344,#36345,#36346,#36347,#36348,
#36349,#36350),(#36351,#36352,#36353,#36354,#36355,#36356,#36357,#36358,
#36359,#36360,#36361,#36362,#36363,#36364),(#36365,#36366,#36367,#36368,
#36369,#36370,#36371,#36372,#36373,#36374,#36375,#36376,#36377,#36378)),
 .UNSPECIFIED.,.F.,.F.,.F.,(4,4),(4,2,2,2,2,2,4),(0.,1.),(0.0377143719414212,
0.167070624995476,0.336553194126115,0.499999999999991,0.663446805873868,
0.832929375004528,0.962285628058582),.UNSPECIFIED.);
#181=B_SPLINE_SURFACE_WITH_KNOTS('',3,3,((#36393,#36394,#36395,#36396,#36397,
#36398,#36399,#36400,#36401,#36402,#36403,#36404,#36405,#36406),(#36407,
#36408,#36409,#36410,#36411,#36412,#36413,#36414,#36415,#36416,#36417,#36418,
#36419,#36420),(#36421,#36422,#36423,#36424,#36425,#36426,#36427,#36428,
#36429,#36430,#36431,#36432,#36433,#36434),(#36435,#36436,#36437,#36438,
#36439,#36440,#36441,#36442,#36443,#36444,#36445,#36446,#36447,#36448),
(#36449,#36450,#36451,#36452,#36453,#36454,#36455,#36456,#36457,#36458,
#36459,#36460,#36461,#36462),(#36463,#36464,#36465,#36466,#36467,#36468,
#36469,#36470,#36471,#36472,#36473,#36474,#36475,#36476),(#36477,#36478,
#36479,#36480,#36481,#36482,#36483,#36484,#36485,#36486,#36487,#36488,#36489,
#36490),(#36491,#36492,#36493,#36494,#36495,#36496,#36497,#36498,#36499,
#36500,#36501,#36502,#36503,#36504),(#36505,#36506,#36507,#36508,#36509,
#36510,#36511,#36512,#36513,#36514,#36515,#36516,#36517,#36518),(#36519,
#36520,#36521,#36522,#36523,#36524,#36525,#36526,#36527,#36528,#36529,#36530,
#36531,#36532),(#36533,#36534,#36535,#36536,#36537,#36538,#36539,#36540,
#36541,#36542,#36543,#36544,#36545,#36546),(#36547,#36548,#36549,#36550,
#36551,#36552,#36553,#36554,#36555,#36556,#36557,#36558,#36559,#36560),
(#36561,#36562,#36563,#36564,#36565,#36566,#36567,#36568,#36569,#36570,
#36571,#36572,#36573,#36574),(#36575,#36576,#36577,#36578,#36579,#36580,
#36581,#36582,#36583,#36584,#36585,#36586,#36587,#36588),(#36589,#36590,
#36591,#36592,#36593,#36594,#36595,#36596,#36597,#36598,#36599,#36600,#36601,
#36602),(#36603,#36604,#36605,#36606,#36607,#36608,#36609,#36610,#36611,
#36612,#36613,#36614,#36615,#36616),(#36617,#36618,#36619,#36620,#36621,
#36622,#36623,#36624,#36625,#36626,#36627,#36628,#36629,#36630),(#36631,
#36632,#36633,#36634,#36635,#36636,#36637,#36638,#36639,#36640,#36641,#36642,
#36643,#36644),(#36645,#36646,#36647,#36648,#36649,#36650,#36651,#36652,
#36653,#36654,#36655,#36656,#36657,#36658),(#36659,#36660,#36661,#36662,
#36663,#36664,#36665,#36666,#36667,#36668,#36669,#36670,#36671,#36672),
(#36673,#36674,#36675,#36676,#36677,#36678,#36679,#36680,#36681,#36682,
#36683,#36684,#36685,#36686),(#36687,#36688,#36689,#36690,#36691,#36692,
#36693,#36694,#36695,#36696,#36697,#36698,#36699,#36700),(#36701,#36702,
#36703,#36704,#36705,#36706,#36707,#36708,#36709,#36710,#36711,#36712,#36713,
#36714),(#36715,#36716,#36717,#36718,#36719,#36720,#36721,#36722,#36723,
#36724,#36725,#36726,#36727,#36728),(#36729,#36730,#36731,#36732,#36733,
#36734,#36735,#36736,#36737,#36738,#36739,#36740,#36741,#36742),(#36743,
#36744,#36745,#36746,#36747,#36748,#36749,#36750,#36751,#36752,#36753,#36754,
#36755,#36756),(#36757,#36758,#36759,#36760,#36761,#36762,#36763,#36764,
#36765,#36766,#36767,#36768,#36769,#36770),(#36771,#36772,#36773,#36774,
#36775,#36776,#36777,#36778,#36779,#36780,#36781,#36782,#36783,#36784),
(#36785,#36786,#36787,#36788,#36789,#36790,#36791,#36792,#36793,#36794,
#36795,#36796,#36797,#36798),(#36799,#36800,#36801,#36802,#36803,#36804,
#36805,#36806,#36807,#36808,#36809,#36810,#36811,#36812),(#36813,#36814,
#36815,#36816,#36817,#36818,#36819,#36820,#36821,#36822,#36823,#36824,#36825,
#36826),(#36827,#36828,#36829,#36830,#36831,#36832,#36833,#36834,#36835,
#36836,#36837,#36838,#36839,#36840),(#36841,#36842,#36843,#36844,#36845,
#36846,#36847,#36848,#36849,#36850,#36851,#36852,#36853,#36854),(#36855,
#36856,#36857,#36858,#36859,#36860,#36861,#36862,#36863,#36864,#36865,#36866,
#36867,#36868),(#36869,#36870,#36871,#36872,#36873,#36874,#36875,#36876,
#36877,#36878,#36879,#36880,#36881,#36882),(#36883,#36884,#36885,#36886,
#36887,#36888,#36889,#36890,#36891,#36892,#36893,#36894,#36895,#36896),
(#36897,#36898,#36899,#36900,#36901,#36902,#36903,#36904,#36905,#36906,
#36907,#36908,#36909,#36910),(#36911,#36912,#36913,#36914,#36915,#36916,
#36917,#36918,#36919,#36920,#36921,#36922,#36923,#36924),(#36925,#36926,
#36927,#36928,#36929,#36930,#36931,#36932,#36933,#36934,#36935,#36936,#36937,
#36938),(#36939,#36940,#36941,#36942,#36943,#36944,#36945,#36946,#36947,
#36948,#36949,#36950,#36951,#36952),(#36953,#36954,#36955,#36956,#36957,
#36958,#36959,#36960,#36961,#36962,#36963,#36964,#36965,#36966),(#36967,
#36968,#36969,#36970,#36971,#36972,#36973,#36974,#36975,#36976,#36977,#36978,
#36979,#36980),(#36981,#36982,#36983,#36984,#36985,#36986,#36987,#36988,
#36989,#36990,#36991,#36992,#36993,#36994),(#36995,#36996,#36997,#36998,
#36999,#37000,#37001,#37002,#37003,#37004,#37005,#37006,#37007,#37008)),
 .UNSPECIFIED.,.F.,.F.,.F.,(4,1,1,1,1,1,1,1,1,1,1,1,1,1,1,1,1,1,1,1,1,1,
1,1,1,1,1,1,1,1,1,1,1,1,1,1,1,1,1,1,1,4),(4,2,2,2,2,2,4),(0.,0.0345301808827031,
0.0517952713240546,0.0690603617654061,0.103590542648109,0.138120723530812,
0.155385813972164,0.172650904413515,0.207181085296218,0.276241447061624,
0.345301808827031,0.379831989709734,0.414362170592437,0.44889235147514,
0.483422532357843,0.552482894123249,0.5697479845646,0.587013075005952,0.621543255888655,
0.656073436771358,0.690603617654061,0.725133798536764,0.759663979419467,
0.763980252029805,0.768296524640143,0.770454660945312,0.776929069860819,
0.79419416030217,0.811459250743522,0.813617387048691,0.815775523353859,
0.820091795964197,0.824408068574535,0.82548713672712,0.826566204879704,
0.827645273032289,0.828184807108581,0.828454574146727,0.828724341184873,
0.897784702950279,0.932314883832982,0.966845064715685),(0.0377143719397814,
0.167070624995476,0.336553194126115,0.499999999999991,0.663446805873868,
0.832929375004528,0.962285628059059),.UNSPECIFIED.);
#182=B_SPLINE_SURFACE_WITH_KNOTS('',3,3,((#37068,#37069,#37070,#37071,#37072,
#37073,#37074,#37075,#37076,#37077,#37078,#37079,#37080,#37081),(#37082,
#37083,#37084,#37085,#37086,#37087,#37088,#37089,#37090,#37091,#37092,#37093,
#37094,#37095),(#37096,#37097,#37098,#37099,#37100,#37101,#37102,#37103,
#37104,#37105,#37106,#37107,#37108,#37109),(#37110,#37111,#37112,#37113,
#37114,#37115,#37116,#37117,#37118,#37119,#37120,#37121,#37122,#37123),
(#37124,#37125,#37126,#37127,#37128,#37129,#37130,#37131,#37132,#37133,
#37134,#37135,#37136,#37137),(#37138,#37139,#37140,#37141,#37142,#37143,
#37144,#37145,#37146,#37147,#37148,#37149,#37150,#37151),(#37152,#37153,
#37154,#37155,#37156,#37157,#37158,#37159,#37160,#37161,#37162,#37163,#37164,
#37165),(#37166,#37167,#37168,#37169,#37170,#37171,#37172,#37173,#37174,
#37175,#37176,#37177,#37178,#37179),(#37180,#37181,#37182,#37183,#37184,
#37185,#37186,#37187,#37188,#37189,#37190,#37191,#37192,#37193),(#37194,
#37195,#37196,#37197,#37198,#37199,#37200,#37201,#37202,#37203,#37204,#37205,
#37206,#37207),(#37208,#37209,#37210,#37211,#37212,#37213,#37214,#37215,
#37216,#37217,#37218,#37219,#37220,#37221),(#37222,#37223,#37224,#37225,
#37226,#37227,#37228,#37229,#37230,#37231,#37232,#37233,#37234,#37235),
(#37236,#37237,#37238,#37239,#37240,#37241,#37242,#37243,#37244,#37245,
#37246,#37247,#37248,#37249),(#37250,#37251,#37252,#37253,#37254,#37255,
#37256,#37257,#37258,#37259,#37260,#37261,#37262,#37263),(#37264,#37265,
#37266,#37267,#37268,#37269,#37270,#37271,#37272,#37273,#37274,#37275,#37276,
#37277),(#37278,#37279,#37280,#37281,#37282,#37283,#37284,#37285,#37286,
#37287,#37288,#37289,#37290,#37291),(#37292,#37293,#37294,#37295,#37296,
#37297,#37298,#37299,#37300,#37301,#37302,#37303,#37304,#37305),(#37306,
#37307,#37308,#37309,#37310,#37311,#37312,#37313,#37314,#37315,#37316,#37317,
#37318,#37319),(#37320,#37321,#37322,#37323,#37324,#37325,#37326,#37327,
#37328,#37329,#37330,#37331,#37332,#37333),(#37334,#37335,#37336,#37337,
#37338,#37339,#37340,#37341,#37342,#37343,#37344,#37345,#37346,#37347),
(#37348,#37349,#37350,#37351,#37352,#37353,#37354,#37355,#37356,#37357,
#37358,#37359,#37360,#37361),(#37362,#37363,#37364,#37365,#37366,#37367,
#37368,#37369,#37370,#37371,#37372,#37373,#37374,#37375),(#37376,#37377,
#37378,#37379,#37380,#37381,#37382,#37383,#37384,#37385,#37386,#37387,#37388,
#37389),(#37390,#37391,#37392,#37393,#37394,#37395,#37396,#37397,#37398,
#37399,#37400,#37401,#37402,#37403),(#37404,#37405,#37406,#37407,#37408,
#37409,#37410,#37411,#37412,#37413,#37414,#37415,#37416,#37417),(#37418,
#37419,#37420,#37421,#37422,#37423,#37424,#37425,#37426,#37427,#37428,#37429,
#37430,#37431),(#37432,#37433,#37434,#37435,#37436,#37437,#37438,#37439,
#37440,#37441,#37442,#37443,#37444,#37445),(#37446,#37447,#37448,#37449,
#37450,#37451,#37452,#37453,#37454,#37455,#37456,#37457,#37458,#37459),
(#37460,#37461,#37462,#37463,#37464,#37465,#37466,#37467,#37468,#37469,
#37470,#37471,#37472,#37473),(#37474,#37475,#37476,#37477,#37478,#37479,
#37480,#37481,#37482,#37483,#37484,#37485,#37486,#37487),(#37488,#37489,
#37490,#37491,#37492,#37493,#37494,#37495,#37496,#37497,#37498,#37499,#37500,
#37501),(#37502,#37503,#37504,#37505,#37506,#37507,#37508,#37509,#37510,
#37511,#37512,#37513,#37514,#37515),(#37516,#37517,#37518,#37519,#37520,
#37521,#37522,#37523,#37524,#37525,#37526,#37527,#37528,#37529)),
 .UNSPECIFIED.,.F.,.F.,.F.,(4,1,1,1,1,1,1,1,1,1,1,1,1,1,1,1,1,1,1,1,1,1,
1,1,1,1,1,1,1,1,4),(4,2,2,2,2,2,4),(0.0331549352864083,0.102215297051665,
0.171275658816921,0.172354726969503,0.173433795122086,0.174512863274668,
0.17559193142725,0.179908204037578,0.188540749258235,0.20580583969955,0.223070930140864,
0.231703475361521,0.240336020582178,0.309396382347434,0.378456744112691,
0.412986924995319,0.447517105877948,0.482047286760576,0.516577467643204,
0.551107648525832,0.568372738967146,0.585637829408461,0.654698191173717,
0.723758552938974,0.79281891470423,0.827349095586859,0.861879276469487,
0.896409457352115,0.930939638234743,0.948204728676058,1.),(0.0377143719413654,
0.167070624995476,0.336553194126115,0.499999999999991,0.663446805873868,
0.832929375004528,0.962285628058767),.UNSPECIFIED.);
#183=B_SPLINE_SURFACE_WITH_KNOTS('',3,3,((#37588,#37589,#37590,#37591,#37592,
#37593,#37594,#37595,#37596,#37597,#37598,#37599,#37600,#37601),(#37602,
#37603,#37604,#37605,#37606,#37607,#37608,#37609,#37610,#37611,#37612,#37613,
#37614,#37615),(#37616,#37617,#37618,#37619,#37620,#37621,#37622,#37623,
#37624,#37625,#37626,#37627,#37628,#37629),(#37630,#37631,#37632,#37633,
#37634,#37635,#37636,#37637,#37638,#37639,#37640,#37641,#37642,#37643)),
 .UNSPECIFIED.,.F.,.F.,.F.,(4,4),(4,2,2,2,2,2,4),(0.,1.),(0.037714371941421,
0.167070624995476,0.336553194126115,0.499999999999991,0.663446805873868,
0.832929375004528,0.962285628058582),.UNSPECIFIED.);
#184=B_SPLINE_SURFACE_WITH_KNOTS('',3,3,((#37658,#37659,#37660,#37661,#37662,
#37663,#37664,#37665,#37666,#37667,#37668,#37669,#37670,#37671),(#37672,
#37673,#37674,#37675,#37676,#37677,#37678,#37679,#37680,#37681,#37682,#37683,
#37684,#37685),(#37686,#37687,#37688,#37689,#37690,#37691,#37692,#37693,
#37694,#37695,#37696,#37697,#37698,#37699),(#37700,#37701,#37702,#37703,
#37704,#37705,#37706,#37707,#37708,#37709,#37710,#37711,#37712,#37713),
(#37714,#37715,#37716,#37717,#37718,#37719,#37720,#37721,#37722,#37723,
#37724,#37725,#37726,#37727),(#37728,#37729,#37730,#37731,#37732,#37733,
#37734,#37735,#37736,#37737,#37738,#37739,#37740,#37741),(#37742,#37743,
#37744,#37745,#37746,#37747,#37748,#37749,#37750,#37751,#37752,#37753,#37754,
#37755),(#37756,#37757,#37758,#37759,#37760,#37761,#37762,#37763,#37764,
#37765,#37766,#37767,#37768,#37769),(#37770,#37771,#37772,#37773,#37774,
#37775,#37776,#37777,#37778,#37779,#37780,#37781,#37782,#37783),(#37784,
#37785,#37786,#37787,#37788,#37789,#37790,#37791,#37792,#37793,#37794,#37795,
#37796,#37797),(#37798,#37799,#37800,#37801,#37802,#37803,#37804,#37805,
#37806,#37807,#37808,#37809,#37810,#37811),(#37812,#37813,#37814,#37815,
#37816,#37817,#37818,#37819,#37820,#37821,#37822,#37823,#37824,#37825),
(#37826,#37827,#37828,#37829,#37830,#37831,#37832,#37833,#37834,#37835,
#37836,#37837,#37838,#37839),(#37840,#37841,#37842,#37843,#37844,#37845,
#37846,#37847,#37848,#37849,#37850,#37851,#37852,#37853),(#37854,#37855,
#37856,#37857,#37858,#37859,#37860,#37861,#37862,#37863,#37864,#37865,#37866,
#37867),(#37868,#37869,#37870,#37871,#37872,#37873,#37874,#37875,#37876,
#37877,#37878,#37879,#37880,#37881),(#37882,#37883,#37884,#37885,#37886,
#37887,#37888,#37889,#37890,#37891,#37892,#37893,#37894,#37895),(#37896,
#37897,#37898,#37899,#37900,#37901,#37902,#37903,#37904,#37905,#37906,#37907,
#37908,#37909),(#37910,#37911,#37912,#37913,#37914,#37915,#37916,#37917,
#37918,#37919,#37920,#37921,#37922,#37923),(#37924,#37925,#37926,#37927,
#37928,#37929,#37930,#37931,#37932,#37933,#37934,#37935,#37936,#37937),
(#37938,#37939,#37940,#37941,#37942,#37943,#37944,#37945,#37946,#37947,
#37948,#37949,#37950,#37951),(#37952,#37953,#37954,#37955,#37956,#37957,
#37958,#37959,#37960,#37961,#37962,#37963,#37964,#37965),(#37966,#37967,
#37968,#37969,#37970,#37971,#37972,#37973,#37974,#37975,#37976,#37977,#37978,
#37979),(#37980,#37981,#37982,#37983,#37984,#37985,#37986,#37987,#37988,
#37989,#37990,#37991,#37992,#37993),(#37994,#37995,#37996,#37997,#37998,
#37999,#38000,#38001,#38002,#38003,#38004,#38005,#38006,#38007),(#38008,
#38009,#38010,#38011,#38012,#38013,#38014,#38015,#38016,#38017,#38018,#38019,
#38020,#38021),(#38022,#38023,#38024,#38025,#38026,#38027,#38028,#38029,
#38030,#38031,#38032,#38033,#38034,#38035),(#38036,#38037,#38038,#38039,
#38040,#38041,#38042,#38043,#38044,#38045,#38046,#38047,#38048,#38049),
(#38050,#38051,#38052,#38053,#38054,#38055,#38056,#38057,#38058,#38059,
#38060,#38061,#38062,#38063),(#38064,#38065,#38066,#38067,#38068,#38069,
#38070,#38071,#38072,#38073,#38074,#38075,#38076,#38077),(#38078,#38079,
#38080,#38081,#38082,#38083,#38084,#38085,#38086,#38087,#38088,#38089,#38090,
#38091),(#38092,#38093,#38094,#38095,#38096,#38097,#38098,#38099,#38100,
#38101,#38102,#38103,#38104,#38105),(#38106,#38107,#38108,#38109,#38110,
#38111,#38112,#38113,#38114,#38115,#38116,#38117,#38118,#38119)),
 .UNSPECIFIED.,.F.,.F.,.F.,(4,1,1,1,1,1,1,1,1,1,1,1,1,1,1,1,1,1,1,1,1,1,
1,1,1,1,1,1,1,1,4),(4,2,2,2,2,2,4),(0.,0.0517952713240546,0.0690603617654061,
0.103590542648109,0.138120723530812,0.155385813972164,0.172650904413515,
0.207181085296218,0.276241447061625,0.414362170592437,0.422994715813113,
0.431627261033788,0.44889235147514,0.474789987137167,0.483422532357843,
0.552482894123249,0.604278165447304,0.621543255888655,0.690603617654061,
0.725133798536764,0.759663979419467,0.776929069860819,0.79419416030217,
0.811459250743522,0.820091795964198,0.824408068574536,0.826566204879705,
0.827645273032289,0.828724341184873,0.89778470295028,0.966845064715686),
(0.0377143719413095,0.167070624995476,0.336553194126115,0.499999999999991,
0.663446805873868,0.832929375004528,0.962285628059314),.UNSPECIFIED.);
#185=B_SPLINE_SURFACE_WITH_KNOTS('',3,3,((#38171,#38172,#38173,#38174,#38175,
#38176,#38177,#38178,#38179,#38180,#38181,#38182,#38183,#38184),(#38185,
#38186,#38187,#38188,#38189,#38190,#38191,#38192,#38193,#38194,#38195,#38196,
#38197,#38198),(#38199,#38200,#38201,#38202,#38203,#38204,#38205,#38206,
#38207,#38208,#38209,#38210,#38211,#38212),(#38213,#38214,#38215,#38216,
#38217,#38218,#38219,#38220,#38221,#38222,#38223,#38224,#38225,#38226),
(#38227,#38228,#38229,#38230,#38231,#38232,#38233,#38234,#38235,#38236,
#38237,#38238,#38239,#38240),(#38241,#38242,#38243,#38244,#38245,#38246,
#38247,#38248,#38249,#38250,#38251,#38252,#38253,#38254),(#38255,#38256,
#38257,#38258,#38259,#38260,#38261,#38262,#38263,#38264,#38265,#38266,#38267,
#38268),(#38269,#38270,#38271,#38272,#38273,#38274,#38275,#38276,#38277,
#38278,#38279,#38280,#38281,#38282),(#38283,#38284,#38285,#38286,#38287,
#38288,#38289,#38290,#38291,#38292,#38293,#38294,#38295,#38296),(#38297,
#38298,#38299,#38300,#38301,#38302,#38303,#38304,#38305,#38306,#38307,#38308,
#38309,#38310),(#38311,#38312,#38313,#38314,#38315,#38316,#38317,#38318,
#38319,#38320,#38321,#38322,#38323,#38324),(#38325,#38326,#38327,#38328,
#38329,#38330,#38331,#38332,#38333,#38334,#38335,#38336,#38337,#38338),
(#38339,#38340,#38341,#38342,#38343,#38344,#38345,#38346,#38347,#38348,
#38349,#38350,#38351,#38352),(#38353,#38354,#38355,#38356,#38357,#38358,
#38359,#38360,#38361,#38362,#38363,#38364,#38365,#38366),(#38367,#38368,
#38369,#38370,#38371,#38372,#38373,#38374,#38375,#38376,#38377,#38378,#38379,
#38380),(#38381,#38382,#38383,#38384,#38385,#38386,#38387,#38388,#38389,
#38390,#38391,#38392,#38393,#38394),(#38395,#38396,#38397,#38398,#38399,
#38400,#38401,#38402,#38403,#38404,#38405,#38406,#38407,#38408),(#38409,
#38410,#38411,#38412,#38413,#38414,#38415,#38416,#38417,#38418,#38419,#38420,
#38421,#38422),(#38423,#38424,#38425,#38426,#38427,#38428,#38429,#38430,
#38431,#38432,#38433,#38434,#38435,#38436),(#38437,#38438,#38439,#38440,
#38441,#38442,#38443,#38444,#38445,#38446,#38447,#38448,#38449,#38450),
(#38451,#38452,#38453,#38454,#38455,#38456,#38457,#38458,#38459,#38460,
#38461,#38462,#38463,#38464),(#38465,#38466,#38467,#38468,#38469,#38470,
#38471,#38472,#38473,#38474,#38475,#38476,#38477,#38478),(#38479,#38480,
#38481,#38482,#38483,#38484,#38485,#38486,#38487,#38488,#38489,#38490,#38491,
#38492),(#38493,#38494,#38495,#38496,#38497,#38498,#38499,#38500,#38501,
#38502,#38503,#38504,#38505,#38506),(#38507,#38508,#38509,#38510,#38511,
#38512,#38513,#38514,#38515,#38516,#38517,#38518,#38519,#38520),(#38521,
#38522,#38523,#38524,#38525,#38526,#38527,#38528,#38529,#38530,#38531,#38532,
#38533,#38534),(#38535,#38536,#38537,#38538,#38539,#38540,#38541,#38542,
#38543,#38544,#38545,#38546,#38547,#38548),(#38549,#38550,#38551,#38552,
#38553,#38554,#38555,#38556,#38557,#38558,#38559,#38560,#38561,#38562),
(#38563,#38564,#38565,#38566,#38567,#38568,#38569,#38570,#38571,#38572,
#38573,#38574,#38575,#38576)),.UNSPECIFIED.,.F.,.F.,.F.,(4,1,1,1,1,1,1,
1,1,1,1,1,1,1,1,1,1,1,1,1,1,1,1,1,1,1,4),(4,2,2,2,2,2,4),(0.0331549352864055,
0.102215297051662,0.171275658816919,0.173433795122083,0.175591931427247,
0.179908204037576,0.188540749258233,0.205805839699547,0.240336020582176,
0.274866201464804,0.309396382347432,0.378456744112689,0.412986924995318,
0.447517105877946,0.516577467643203,0.585637829408459,0.602902919849774,
0.620168010291088,0.654698191173716,0.689228372056345,0.723758552938973,
0.810084005145544,0.861879276469486,0.896409457352115,0.930939638234743,
0.948204728676057,1.),(0.0377143719413947,0.167070624995476,0.336553194126115,
0.499999999999991,0.663446805873868,0.832929375004528,0.962285628058718),
 .UNSPECIFIED.);
#186=B_SPLINE_SURFACE_WITH_KNOTS('',3,3,((#38633,#38634,#38635,#38636,#38637,
#38638,#38639,#38640,#38641,#38642,#38643,#38644,#38645,#38646),(#38647,
#38648,#38649,#38650,#38651,#38652,#38653,#38654,#38655,#38656,#38657,#38658,
#38659,#38660),(#38661,#38662,#38663,#38664,#38665,#38666,#38667,#38668,
#38669,#38670,#38671,#38672,#38673,#38674),(#38675,#38676,#38677,#38678,
#38679,#38680,#38681,#38682,#38683,#38684,#38685,#38686,#38687,#38688)),
 .UNSPECIFIED.,.F.,.F.,.F.,(4,4),(4,2,2,2,2,2,4),(0.,1.),(0.0377143719414212,
0.167070624995476,0.336553194126115,0.499999999999991,0.663446805873868,
0.832929375004528,0.962285628058582),.UNSPECIFIED.);
#187=B_SPLINE_SURFACE_WITH_KNOTS('',3,3,((#38703,#38704,#38705,#38706,#38707,
#38708,#38709,#38710,#38711,#38712,#38713,#38714,#38715,#38716),(#38717,
#38718,#38719,#38720,#38721,#38722,#38723,#38724,#38725,#38726,#38727,#38728,
#38729,#38730),(#38731,#38732,#38733,#38734,#38735,#38736,#38737,#38738,
#38739,#38740,#38741,#38742,#38743,#38744),(#38745,#38746,#38747,#38748,
#38749,#38750,#38751,#38752,#38753,#38754,#38755,#38756,#38757,#38758),
(#38759,#38760,#38761,#38762,#38763,#38764,#38765,#38766,#38767,#38768,
#38769,#38770,#38771,#38772),(#38773,#38774,#38775,#38776,#38777,#38778,
#38779,#38780,#38781,#38782,#38783,#38784,#38785,#38786),(#38787,#38788,
#38789,#38790,#38791,#38792,#38793,#38794,#38795,#38796,#38797,#38798,#38799,
#38800),(#38801,#38802,#38803,#38804,#38805,#38806,#38807,#38808,#38809,
#38810,#38811,#38812,#38813,#38814),(#38815,#38816,#38817,#38818,#38819,
#38820,#38821,#38822,#38823,#38824,#38825,#38826,#38827,#38828),(#38829,
#38830,#38831,#38832,#38833,#38834,#38835,#38836,#38837,#38838,#38839,#38840,
#38841,#38842),(#38843,#38844,#38845,#38846,#38847,#38848,#38849,#38850,
#38851,#38852,#38853,#38854,#38855,#38856),(#38857,#38858,#38859,#38860,
#38861,#38862,#38863,#38864,#38865,#38866,#38867,#38868,#38869,#38870),
(#38871,#38872,#38873,#38874,#38875,#38876,#38877,#38878,#38879,#38880,
#38881,#38882,#38883,#38884),(#38885,#38886,#38887,#38888,#38889,#38890,
#38891,#38892,#38893,#38894,#38895,#38896,#38897,#38898),(#38899,#38900,
#38901,#38902,#38903,#38904,#38905,#38906,#38907,#38908,#38909,#38910,#38911,
#38912),(#38913,#38914,#38915,#38916,#38917,#38918,#38919,#38920,#38921,
#38922,#38923,#38924,#38925,#38926),(#38927,#38928,#38929,#38930,#38931,
#38932,#38933,#38934,#38935,#38936,#38937,#38938,#38939,#38940),(#38941,
#38942,#38943,#38944,#38945,#38946,#38947,#38948,#38949,#38950,#38951,#38952,
#38953,#38954),(#38955,#38956,#38957,#38958,#38959,#38960,#38961,#38962,
#38963,#38964,#38965,#38966,#38967,#38968),(#38969,#38970,#38971,#38972,
#38973,#38974,#38975,#38976,#38977,#38978,#38979,#38980,#38981,#38982),
(#38983,#38984,#38985,#38986,#38987,#38988,#38989,#38990,#38991,#38992,
#38993,#38994,#38995,#38996),(#38997,#38998,#38999,#39000,#39001,#39002,
#39003,#39004,#39005,#39006,#39007,#39008,#39009,#39010),(#39011,#39012,
#39013,#39014,#39015,#39016,#39017,#39018,#39019,#39020,#39021,#39022,#39023,
#39024),(#39025,#39026,#39027,#39028,#39029,#39030,#39031,#39032,#39033,
#39034,#39035,#39036,#39037,#39038),(#39039,#39040,#39041,#39042,#39043,
#39044,#39045,#39046,#39047,#39048,#39049,#39050,#39051,#39052),(#39053,
#39054,#39055,#39056,#39057,#39058,#39059,#39060,#39061,#39062,#39063,#39064,
#39065,#39066),(#39067,#39068,#39069,#39070,#39071,#39072,#39073,#39074,
#39075,#39076,#39077,#39078,#39079,#39080),(#39081,#39082,#39083,#39084,
#39085,#39086,#39087,#39088,#39089,#39090,#39091,#39092,#39093,#39094),
(#39095,#39096,#39097,#39098,#39099,#39100,#39101,#39102,#39103,#39104,
#39105,#39106,#39107,#39108),(#39109,#39110,#39111,#39112,#39113,#39114,
#39115,#39116,#39117,#39118,#39119,#39120,#39121,#39122),(#39123,#39124,
#39125,#39126,#39127,#39128,#39129,#39130,#39131,#39132,#39133,#39134,#39135,
#39136),(#39137,#39138,#39139,#39140,#39141,#39142,#39143,#39144,#39145,
#39146,#39147,#39148,#39149,#39150),(#39151,#39152,#39153,#39154,#39155,
#39156,#39157,#39158,#39159,#39160,#39161,#39162,#39163,#39164),(#39165,
#39166,#39167,#39168,#39169,#39170,#39171,#39172,#39173,#39174,#39175,#39176,
#39177,#39178),(#39179,#39180,#39181,#39182,#39183,#39184,#39185,#39186,
#39187,#39188,#39189,#39190,#39191,#39192)),.UNSPECIFIED.,.F.,.F.,.F.,(4,
1,1,1,1,1,1,1,1,1,1,1,1,1,1,1,1,1,1,1,1,1,1,1,1,1,1,1,1,1,1,1,4),(4,2,2,
2,2,2,4),(0.,0.0517952713240544,0.0690603617654059,0.103590542648109,0.138120723530812,
0.155385813972163,0.172650904413515,0.207181085296218,0.276241447061624,
0.34530180882703,0.379831989709732,0.414362170592435,0.431627261033787,
0.448892351475138,0.46615744191649,0.483422532357841,0.552482894123247,
0.58701307500595,0.604278165447302,0.621543255888653,0.656073436771356,
0.690603617654059,0.759663979419465,0.776929069860816,0.794194160302168,
0.811459250743519,0.820091795964195,0.824408068574533,0.826566204879702,
0.827645273032286,0.828724341184871,0.897784702950277,0.966845064715683),
(0.0377143719406538,0.167070624995476,0.336553194126115,0.499999999999991,
0.663446805873868,0.832929375004528,0.96228562805863),.UNSPECIFIED.);
#188=B_SPLINE_SURFACE_WITH_KNOTS('',3,3,((#39248,#39249,#39250,#39251,#39252,
#39253,#39254,#39255,#39256,#39257,#39258,#39259,#39260,#39261),(#39262,
#39263,#39264,#39265,#39266,#39267,#39268,#39269,#39270,#39271,#39272,#39273,
#39274,#39275),(#39276,#39277,#39278,#39279,#39280,#39281,#39282,#39283,
#39284,#39285,#39286,#39287,#39288,#39289),(#39290,#39291,#39292,#39293,
#39294,#39295,#39296,#39297,#39298,#39299,#39300,#39301,#39302,#39303),
(#39304,#39305,#39306,#39307,#39308,#39309,#39310,#39311,#39312,#39313,
#39314,#39315,#39316,#39317),(#39318,#39319,#39320,#39321,#39322,#39323,
#39324,#39325,#39326,#39327,#39328,#39329,#39330,#39331),(#39332,#39333,
#39334,#39335,#39336,#39337,#39338,#39339,#39340,#39341,#39342,#39343,#39344,
#39345),(#39346,#39347,#39348,#39349,#39350,#39351,#39352,#39353,#39354,
#39355,#39356,#39357,#39358,#39359),(#39360,#39361,#39362,#39363,#39364,
#39365,#39366,#39367,#39368,#39369,#39370,#39371,#39372,#39373),(#39374,
#39375,#39376,#39377,#39378,#39379,#39380,#39381,#39382,#39383,#39384,#39385,
#39386,#39387),(#39388,#39389,#39390,#39391,#39392,#39393,#39394,#39395,
#39396,#39397,#39398,#39399,#39400,#39401),(#39402,#39403,#39404,#39405,
#39406,#39407,#39408,#39409,#39410,#39411,#39412,#39413,#39414,#39415),
(#39416,#39417,#39418,#39419,#39420,#39421,#39422,#39423,#39424,#39425,
#39426,#39427,#39428,#39429),(#39430,#39431,#39432,#39433,#39434,#39435,
#39436,#39437,#39438,#39439,#39440,#39441,#39442,#39443),(#39444,#39445,
#39446,#39447,#39448,#39449,#39450,#39451,#39452,#39453,#39454,#39455,#39456,
#39457),(#39458,#39459,#39460,#39461,#39462,#39463,#39464,#39465,#39466,
#39467,#39468,#39469,#39470,#39471),(#39472,#39473,#39474,#39475,#39476,
#39477,#39478,#39479,#39480,#39481,#39482,#39483,#39484,#39485),(#39486,
#39487,#39488,#39489,#39490,#39491,#39492,#39493,#39494,#39495,#39496,#39497,
#39498,#39499),(#39500,#39501,#39502,#39503,#39504,#39505,#39506,#39507,
#39508,#39509,#39510,#39511,#39512,#39513),(#39514,#39515,#39516,#39517,
#39518,#39519,#39520,#39521,#39522,#39523,#39524,#39525,#39526,#39527),
(#39528,#39529,#39530,#39531,#39532,#39533,#39534,#39535,#39536,#39537,
#39538,#39539,#39540,#39541),(#39542,#39543,#39544,#39545,#39546,#39547,
#39548,#39549,#39550,#39551,#39552,#39553,#39554,#39555),(#39556,#39557,
#39558,#39559,#39560,#39561,#39562,#39563,#39564,#39565,#39566,#39567,#39568,
#39569),(#39570,#39571,#39572,#39573,#39574,#39575,#39576,#39577,#39578,
#39579,#39580,#39581,#39582,#39583),(#39584,#39585,#39586,#39587,#39588,
#39589,#39590,#39591,#39592,#39593,#39594,#39595,#39596,#39597),(#39598,
#39599,#39600,#39601,#39602,#39603,#39604,#39605,#39606,#39607,#39608,#39609,
#39610,#39611),(#39612,#39613,#39614,#39615,#39616,#39617,#39618,#39619,
#39620,#39621,#39622,#39623,#39624,#39625),(#39626,#39627,#39628,#39629,
#39630,#39631,#39632,#39633,#39634,#39635,#39636,#39637,#39638,#39639),
(#39640,#39641,#39642,#39643,#39644,#39645,#39646,#39647,#39648,#39649,
#39650,#39651,#39652,#39653),(#39654,#39655,#39656,#39657,#39658,#39659,
#39660,#39661,#39662,#39663,#39664,#39665,#39666,#39667),(#39668,#39669,
#39670,#39671,#39672,#39673,#39674,#39675,#39676,#39677,#39678,#39679,#39680,
#39681),(#39682,#39683,#39684,#39685,#39686,#39687,#39688,#39689,#39690,
#39691,#39692,#39693,#39694,#39695),(#39696,#39697,#39698,#39699,#39700,
#39701,#39702,#39703,#39704,#39705,#39706,#39707,#39708,#39709),(#39710,
#39711,#39712,#39713,#39714,#39715,#39716,#39717,#39718,#39719,#39720,#39721,
#39722,#39723),(#39724,#39725,#39726,#39727,#39728,#39729,#39730,#39731,
#39732,#39733,#39734,#39735,#39736,#39737),(#39738,#39739,#39740,#39741,
#39742,#39743,#39744,#39745,#39746,#39747,#39748,#39749,#39750,#39751)),
 .UNSPECIFIED.,.F.,.F.,.F.,(4,1,1,1,1,1,1,1,1,1,1,1,1,1,1,1,1,1,1,1,1,1,
1,1,1,1,1,1,1,1,1,1,1,4),(4,2,2,2,2,2,4),(0.0331549352864097,0.102215297051666,
0.171275658816923,0.171815192893214,0.172354726969505,0.172894261045796,
0.173433795122087,0.175591931427251,0.177750067732415,0.178829135884997,
0.17990820403758,0.188540749258237,0.205805839699551,0.214438384920208,
0.223070930140865,0.231703475361522,0.240336020582179,0.274866201464807,
0.309396382347435,0.378456744112692,0.41298692499532,0.430252015436634,
0.447517105877948,0.516577467643205,0.585637829408461,0.671963281615032,
0.689228372056346,0.723758552938974,0.810084005145545,0.861879276469487,
0.896409457352115,0.930939638234744,0.948204728676058,1.),(0.0377143719409187,
0.167070624995476,0.336553194126115,0.499999999999991,0.663446805873868,
0.832929375004528,0.962285628058664),.UNSPECIFIED.);
#189=B_SPLINE_SURFACE_WITH_KNOTS('',3,3,((#39812,#39813,#39814,#39815,#39816,
#39817,#39818,#39819,#39820,#39821,#39822,#39823,#39824,#39825),(#39826,
#39827,#39828,#39829,#39830,#39831,#39832,#39833,#39834,#39835,#39836,#39837,
#39838,#39839),(#39840,#39841,#39842,#39843,#39844,#39845,#39846,#39847,
#39848,#39849,#39850,#39851,#39852,#39853),(#39854,#39855,#39856,#39857,
#39858,#39859,#39860,#39861,#39862,#39863,#39864,#39865,#39866,#39867)),
 .UNSPECIFIED.,.F.,.F.,.F.,(4,4),(4,2,2,2,2,2,4),(0.,1.),(0.0377143719414211,
0.167070624995476,0.336553194126115,0.499999999999991,0.663446805873868,
0.832929375004528,0.962285628058582),.UNSPECIFIED.);
#190=B_SPLINE_SURFACE_WITH_KNOTS('',3,3,((#39882,#39883,#39884,#39885,#39886,
#39887,#39888,#39889,#39890,#39891,#39892,#39893,#39894,#39895),(#39896,
#39897,#39898,#39899,#39900,#39901,#39902,#39903,#39904,#39905,#39906,#39907,
#39908,#39909),(#39910,#39911,#39912,#39913,#39914,#39915,#39916,#39917,
#39918,#39919,#39920,#39921,#39922,#39923),(#39924,#39925,#39926,#39927,
#39928,#39929,#39930,#39931,#39932,#39933,#39934,#39935,#39936,#39937),
(#39938,#39939,#39940,#39941,#39942,#39943,#39944,#39945,#39946,#39947,
#39948,#39949,#39950,#39951),(#39952,#39953,#39954,#39955,#39956,#39957,
#39958,#39959,#39960,#39961,#39962,#39963,#39964,#39965),(#39966,#39967,
#39968,#39969,#39970,#39971,#39972,#39973,#39974,#39975,#39976,#39977,#39978,
#39979),(#39980,#39981,#39982,#39983,#39984,#39985,#39986,#39987,#39988,
#39989,#39990,#39991,#39992,#39993),(#39994,#39995,#39996,#39997,#39998,
#39999,#40000,#40001,#40002,#40003,#40004,#40005,#40006,#40007),(#40008,
#40009,#40010,#40011,#40012,#40013,#40014,#40015,#40016,#40017,#40018,#40019,
#40020,#40021),(#40022,#40023,#40024,#40025,#40026,#40027,#40028,#40029,
#40030,#40031,#40032,#40033,#40034,#40035),(#40036,#40037,#40038,#40039,
#40040,#40041,#40042,#40043,#40044,#40045,#40046,#40047,#40048,#40049),
(#40050,#40051,#40052,#40053,#40054,#40055,#40056,#40057,#40058,#40059,
#40060,#40061,#40062,#40063),(#40064,#40065,#40066,#40067,#40068,#40069,
#40070,#40071,#40072,#40073,#40074,#40075,#40076,#40077),(#40078,#40079,
#40080,#40081,#40082,#40083,#40084,#40085,#40086,#40087,#40088,#40089,#40090,
#40091),(#40092,#40093,#40094,#40095,#40096,#40097,#40098,#40099,#40100,
#40101,#40102,#40103,#40104,#40105),(#40106,#40107,#40108,#40109,#40110,
#40111,#40112,#40113,#40114,#40115,#40116,#40117,#40118,#40119),(#40120,
#40121,#40122,#40123,#40124,#40125,#40126,#40127,#40128,#40129,#40130,#40131,
#40132,#40133),(#40134,#40135,#40136,#40137,#40138,#40139,#40140,#40141,
#40142,#40143,#40144,#40145,#40146,#40147),(#40148,#40149,#40150,#40151,
#40152,#40153,#40154,#40155,#40156,#40157,#40158,#40159,#40160,#40161),
(#40162,#40163,#40164,#40165,#40166,#40167,#40168,#40169,#40170,#40171,
#40172,#40173,#40174,#40175),(#40176,#40177,#40178,#40179,#40180,#40181,
#40182,#40183,#40184,#40185,#40186,#40187,#40188,#40189),(#40190,#40191,
#40192,#40193,#40194,#40195,#40196,#40197,#40198,#40199,#40200,#40201,#40202,
#40203),(#40204,#40205,#40206,#40207,#40208,#40209,#40210,#40211,#40212,
#40213,#40214,#40215,#40216,#40217),(#40218,#40219,#40220,#40221,#40222,
#40223,#40224,#40225,#40226,#40227,#40228,#40229,#40230,#40231),(#40232,
#40233,#40234,#40235,#40236,#40237,#40238,#40239,#40240,#40241,#40242,#40243,
#40244,#40245),(#40246,#40247,#40248,#40249,#40250,#40251,#40252,#40253,
#40254,#40255,#40256,#40257,#40258,#40259),(#40260,#40261,#40262,#40263,
#40264,#40265,#40266,#40267,#40268,#40269,#40270,#40271,#40272,#40273),
(#40274,#40275,#40276,#40277,#40278,#40279,#40280,#40281,#40282,#40283,
#40284,#40285,#40286,#40287),(#40288,#40289,#40290,#40291,#40292,#40293,
#40294,#40295,#40296,#40297,#40298,#40299,#40300,#40301),(#40302,#40303,
#40304,#40305,#40306,#40307,#40308,#40309,#40310,#40311,#40312,#40313,#40314,
#40315),(#40316,#40317,#40318,#40319,#40320,#40321,#40322,#40323,#40324,
#40325,#40326,#40327,#40328,#40329),(#40330,#40331,#40332,#40333,#40334,
#40335,#40336,#40337,#40338,#40339,#40340,#40341,#40342,#40343),(#40344,
#40345,#40346,#40347,#40348,#40349,#40350,#40351,#40352,#40353,#40354,#40355,
#40356,#40357),(#40358,#40359,#40360,#40361,#40362,#40363,#40364,#40365,
#40366,#40367,#40368,#40369,#40370,#40371),(#40372,#40373,#40374,#40375,
#40376,#40377,#40378,#40379,#40380,#40381,#40382,#40383,#40384,#40385),
(#40386,#40387,#40388,#40389,#40390,#40391,#40392,#40393,#40394,#40395,
#40396,#40397,#40398,#40399),(#40400,#40401,#40402,#40403,#40404,#40405,
#40406,#40407,#40408,#40409,#40410,#40411,#40412,#40413),(#40414,#40415,
#40416,#40417,#40418,#40419,#40420,#40421,#40422,#40423,#40424,#40425,#40426,
#40427),(#40428,#40429,#40430,#40431,#40432,#40433,#40434,#40435,#40436,
#40437,#40438,#40439,#40440,#40441)),.UNSPECIFIED.,.F.,.F.,.F.,(4,1,1,1,
1,1,1,1,1,1,1,1,1,1,1,1,1,1,1,1,1,1,1,1,1,1,1,1,1,1,1,1,1,1,1,1,1,4),(4,
2,2,2,2,2,4),(0.,0.0517952713240544,0.0690603617654059,0.0863254522067574,
0.103590542648109,0.138120723530812,0.155385813972163,0.189915994854866,
0.207181085296218,0.276241447061624,0.345301808827029,0.379831989709732,
0.414362170592435,0.448892351475138,0.500687622799193,0.552482894123247,
0.569747984564599,0.621543255888653,0.638808346330004,0.690603617654059,
0.725133798536762,0.742398888978113,0.759663979419465,0.776929069860816,
0.794194160302168,0.798510432912505,0.802826705522843,0.811459250743519,
0.820091795964195,0.822249932269364,0.824408068574533,0.826566204879702,
0.827645273032286,0.828184807108578,0.828724341184871,0.897784702950276,
0.932314883832979,0.966845064715682),(0.0377143719385139,0.167070624995476,
0.336553194126115,0.499999999999991,0.663446805873868,0.832929375004528,
0.962285628061),.UNSPECIFIED.);
#191=B_SPLINE_SURFACE_WITH_KNOTS('',3,3,((#40497,#40498,#40499,#40500,#40501,
#40502,#40503,#40504,#40505,#40506,#40507,#40508,#40509,#40510),(#40511,
#40512,#40513,#40514,#40515,#40516,#40517,#40518,#40519,#40520,#40521,#40522,
#40523,#40524),(#40525,#40526,#40527,#40528,#40529,#40530,#40531,#40532,
#40533,#40534,#40535,#40536,#40537,#40538),(#40539,#40540,#40541,#40542,
#40543,#40544,#40545,#40546,#40547,#40548,#40549,#40550,#40551,#40552),
(#40553,#40554,#40555,#40556,#40557,#40558,#40559,#40560,#40561,#40562,
#40563,#40564,#40565,#40566),(#40567,#40568,#40569,#40570,#40571,#40572,
#40573,#40574,#40575,#40576,#40577,#40578,#40579,#40580),(#40581,#40582,
#40583,#40584,#40585,#40586,#40587,#40588,#40589,#40590,#40591,#40592,#40593,
#40594),(#40595,#40596,#40597,#40598,#40599,#40600,#40601,#40602,#40603,
#40604,#40605,#40606,#40607,#40608),(#40609,#40610,#40611,#40612,#40613,
#40614,#40615,#40616,#40617,#40618,#40619,#40620,#40621,#40622),(#40623,
#40624,#40625,#40626,#40627,#40628,#40629,#40630,#40631,#40632,#40633,#40634,
#40635,#40636),(#40637,#40638,#40639,#40640,#40641,#40642,#40643,#40644,
#40645,#40646,#40647,#40648,#40649,#40650),(#40651,#40652,#40653,#40654,
#40655,#40656,#40657,#40658,#40659,#40660,#40661,#40662,#40663,#40664),
(#40665,#40666,#40667,#40668,#40669,#40670,#40671,#40672,#40673,#40674,
#40675,#40676,#40677,#40678),(#40679,#40680,#40681,#40682,#40683,#40684,
#40685,#40686,#40687,#40688,#40689,#40690,#40691,#40692),(#40693,#40694,
#40695,#40696,#40697,#40698,#40699,#40700,#40701,#40702,#40703,#40704,#40705,
#40706),(#40707,#40708,#40709,#40710,#40711,#40712,#40713,#40714,#40715,
#40716,#40717,#40718,#40719,#40720),(#40721,#40722,#40723,#40724,#40725,
#40726,#40727,#40728,#40729,#40730,#40731,#40732,#40733,#40734),(#40735,
#40736,#40737,#40738,#40739,#40740,#40741,#40742,#40743,#40744,#40745,#40746,
#40747,#40748),(#40749,#40750,#40751,#40752,#40753,#40754,#40755,#40756,
#40757,#40758,#40759,#40760,#40761,#40762),(#40763,#40764,#40765,#40766,
#40767,#40768,#40769,#40770,#40771,#40772,#40773,#40774,#40775,#40776),
(#40777,#40778,#40779,#40780,#40781,#40782,#40783,#40784,#40785,#40786,
#40787,#40788,#40789,#40790),(#40791,#40792,#40793,#40794,#40795,#40796,
#40797,#40798,#40799,#40800,#40801,#40802,#40803,#40804),(#40805,#40806,
#40807,#40808,#40809,#40810,#40811,#40812,#40813,#40814,#40815,#40816,#40817,
#40818),(#40819,#40820,#40821,#40822,#40823,#40824,#40825,#40826,#40827,
#40828,#40829,#40830,#40831,#40832),(#40833,#40834,#40835,#40836,#40837,
#40838,#40839,#40840,#40841,#40842,#40843,#40844,#40845,#40846),(#40847,
#40848,#40849,#40850,#40851,#40852,#40853,#40854,#40855,#40856,#40857,#40858,
#40859,#40860),(#40861,#40862,#40863,#40864,#40865,#40866,#40867,#40868,
#40869,#40870,#40871,#40872,#40873,#40874),(#40875,#40876,#40877,#40878,
#40879,#40880,#40881,#40882,#40883,#40884,#40885,#40886,#40887,#40888),
(#40889,#40890,#40891,#40892,#40893,#40894,#40895,#40896,#40897,#40898,
#40899,#40900,#40901,#40902)),.UNSPECIFIED.,.F.,.F.,.F.,(4,1,1,1,1,1,1,
1,1,1,1,1,1,1,1,1,1,1,1,1,1,1,1,1,1,1,4),(4,2,2,2,2,2,4),(0.0331549352864072,
0.102215297051664,0.17127565881692,0.173433795122085,0.175591931427249,
0.179908204037578,0.188540749258235,0.205805839699549,0.240336020582177,
0.274866201464805,0.309396382347434,0.37845674411269,0.412986924995319,
0.447517105877947,0.516577467643204,0.58563782940846,0.602902919849775,
0.620168010291089,0.654698191173717,0.689228372056345,0.723758552938974,
0.810084005145544,0.861879276469487,0.896409457352115,0.930939638234743,
0.948204728676058,1.),(0.0377143719409187,0.167070624995476,0.336553194126115,
0.499999999999991,0.663446805873868,0.832929375004528,0.962285628058774),
 .UNSPECIFIED.);
#192=B_SPLINE_SURFACE_WITH_KNOTS('',3,3,((#40959,#40960,#40961,#40962,#40963,
#40964,#40965,#40966,#40967,#40968,#40969,#40970,#40971,#40972),(#40973,
#40974,#40975,#40976,#40977,#40978,#40979,#40980,#40981,#40982,#40983,#40984,
#40985,#40986),(#40987,#40988,#40989,#40990,#40991,#40992,#40993,#40994,
#40995,#40996,#40997,#40998,#40999,#41000),(#41001,#41002,#41003,#41004,
#41005,#41006,#41007,#41008,#41009,#41010,#41011,#41012,#41013,#41014)),
 .UNSPECIFIED.,.F.,.F.,.F.,(4,4),(4,2,2,2,2,2,4),(0.,1.),(0.0377143719414211,
0.167070624995476,0.336553194126115,0.499999999999991,0.663446805873868,
0.832929375004528,0.962285628058582),.UNSPECIFIED.);
#193=B_SPLINE_SURFACE_WITH_KNOTS('',3,3,((#41029,#41030,#41031,#41032,#41033,
#41034,#41035,#41036,#41037,#41038,#41039,#41040,#41041,#41042),(#41043,
#41044,#41045,#41046,#41047,#41048,#41049,#41050,#41051,#41052,#41053,#41054,
#41055,#41056),(#41057,#41058,#41059,#41060,#41061,#41062,#41063,#41064,
#41065,#41066,#41067,#41068,#41069,#41070),(#41071,#41072,#41073,#41074,
#41075,#41076,#41077,#41078,#41079,#41080,#41081,#41082,#41083,#41084),
(#41085,#41086,#41087,#41088,#41089,#41090,#41091,#41092,#41093,#41094,
#41095,#41096,#41097,#41098),(#41099,#41100,#41101,#41102,#41103,#41104,
#41105,#41106,#41107,#41108,#41109,#41110,#41111,#41112),(#41113,#41114,
#41115,#41116,#41117,#41118,#41119,#41120,#41121,#41122,#41123,#41124,#41125,
#41126),(#41127,#41128,#41129,#41130,#41131,#41132,#41133,#41134,#41135,
#41136,#41137,#41138,#41139,#41140),(#41141,#41142,#41143,#41144,#41145,
#41146,#41147,#41148,#41149,#41150,#41151,#41152,#41153,#41154),(#41155,
#41156,#41157,#41158,#41159,#41160,#41161,#41162,#41163,#41164,#41165,#41166,
#41167,#41168),(#41169,#41170,#41171,#41172,#41173,#41174,#41175,#41176,
#41177,#41178,#41179,#41180,#41181,#41182),(#41183,#41184,#41185,#41186,
#41187,#41188,#41189,#41190,#41191,#41192,#41193,#41194,#41195,#41196),
(#41197,#41198,#41199,#41200,#41201,#41202,#41203,#41204,#41205,#41206,
#41207,#41208,#41209,#41210),(#41211,#41212,#41213,#41214,#41215,#41216,
#41217,#41218,#41219,#41220,#41221,#41222,#41223,#41224),(#41225,#41226,
#41227,#41228,#41229,#41230,#41231,#41232,#41233,#41234,#41235,#41236,#41237,
#41238),(#41239,#41240,#41241,#41242,#41243,#41244,#41245,#41246,#41247,
#41248,#41249,#41250,#41251,#41252),(#41253,#41254,#41255,#41256,#41257,
#41258,#41259,#41260,#41261,#41262,#41263,#41264,#41265,#41266),(#41267,
#41268,#41269,#41270,#41271,#41272,#41273,#41274,#41275,#41276,#41277,#41278,
#41279,#41280),(#41281,#41282,#41283,#41284,#41285,#41286,#41287,#41288,
#41289,#41290,#41291,#41292,#41293,#41294),(#41295,#41296,#41297,#41298,
#41299,#41300,#41301,#41302,#41303,#41304,#41305,#41306,#41307,#41308),
(#41309,#41310,#41311,#41312,#41313,#41314,#41315,#41316,#41317,#41318,
#41319,#41320,#41321,#41322),(#41323,#41324,#41325,#41326,#41327,#41328,
#41329,#41330,#41331,#41332,#41333,#41334,#41335,#41336),(#41337,#41338,
#41339,#41340,#41341,#41342,#41343,#41344,#41345,#41346,#41347,#41348,#41349,
#41350),(#41351,#41352,#41353,#41354,#41355,#41356,#41357,#41358,#41359,
#41360,#41361,#41362,#41363,#41364),(#41365,#41366,#41367,#41368,#41369,
#41370,#41371,#41372,#41373,#41374,#41375,#41376,#41377,#41378),(#41379,
#41380,#41381,#41382,#41383,#41384,#41385,#41386,#41387,#41388,#41389,#41390,
#41391,#41392),(#41393,#41394,#41395,#41396,#41397,#41398,#41399,#41400,
#41401,#41402,#41403,#41404,#41405,#41406),(#41407,#41408,#41409,#41410,
#41411,#41412,#41413,#41414,#41415,#41416,#41417,#41418,#41419,#41420),
(#41421,#41422,#41423,#41424,#41425,#41426,#41427,#41428,#41429,#41430,
#41431,#41432,#41433,#41434),(#41435,#41436,#41437,#41438,#41439,#41440,
#41441,#41442,#41443,#41444,#41445,#41446,#41447,#41448),(#41449,#41450,
#41451,#41452,#41453,#41454,#41455,#41456,#41457,#41458,#41459,#41460,#41461,
#41462),(#41463,#41464,#41465,#41466,#41467,#41468,#41469,#41470,#41471,
#41472,#41473,#41474,#41475,#41476),(#41477,#41478,#41479,#41480,#41481,
#41482,#41483,#41484,#41485,#41486,#41487,#41488,#41489,#41490),(#41491,
#41492,#41493,#41494,#41495,#41496,#41497,#41498,#41499,#41500,#41501,#41502,
#41503,#41504),(#41505,#41506,#41507,#41508,#41509,#41510,#41511,#41512,
#41513,#41514,#41515,#41516,#41517,#41518),(#41519,#41520,#41521,#41522,
#41523,#41524,#41525,#41526,#41527,#41528,#41529,#41530,#41531,#41532),
(#41533,#41534,#41535,#41536,#41537,#41538,#41539,#41540,#41541,#41542,
#41543,#41544,#41545,#41546)),.UNSPECIFIED.,.F.,.F.,.F.,(4,1,1,1,1,1,1,
1,1,1,1,1,1,1,1,1,1,1,1,1,1,1,1,1,1,1,1,1,1,1,1,1,1,1,4),(4,2,2,2,2,2,4),
(0.,0.034530180882703,0.0517952713240545,0.0690603617654059,0.103590542648109,
0.138120723530812,0.155385813972163,0.189915994854866,0.207181085296218,
0.276241447061624,0.34530180882703,0.379831989709733,0.414362170592436,
0.448892351475139,0.483422532357842,0.552482894123247,0.621543255888653,
0.656073436771356,0.690603617654059,0.725133798536762,0.759663979419465,
0.776929069860817,0.785561615081493,0.794194160302168,0.81145925074352,
0.815775523353858,0.820091795964196,0.824408068574533,0.826566204879702,
0.827645273032287,0.828724341184871,0.880519612508926,0.897784702950277,
0.93231488383298,0.966845064715683),(0.0377143719413868,0.167070624995476,
0.336553194126115,0.499999999999991,0.663446805873868,0.832929375004528,
0.962285628060268),.UNSPECIFIED.);
#194=B_SPLINE_SURFACE_WITH_KNOTS('',3,3,((#41598,#41599,#41600,#41601,#41602,
#41603,#41604,#41605,#41606,#41607,#41608,#41609,#41610,#41611),(#41612,
#41613,#41614,#41615,#41616,#41617,#41618,#41619,#41620,#41621,#41622,#41623,
#41624,#41625),(#41626,#41627,#41628,#41629,#41630,#41631,#41632,#41633,
#41634,#41635,#41636,#41637,#41638,#41639),(#41640,#41641,#41642,#41643,
#41644,#41645,#41646,#41647,#41648,#41649,#41650,#41651,#41652,#41653),
(#41654,#41655,#41656,#41657,#41658,#41659,#41660,#41661,#41662,#41663,
#41664,#41665,#41666,#41667),(#41668,#41669,#41670,#41671,#41672,#41673,
#41674,#41675,#41676,#41677,#41678,#41679,#41680,#41681),(#41682,#41683,
#41684,#41685,#41686,#41687,#41688,#41689,#41690,#41691,#41692,#41693,#41694,
#41695),(#41696,#41697,#41698,#41699,#41700,#41701,#41702,#41703,#41704,
#41705,#41706,#41707,#41708,#41709),(#41710,#41711,#41712,#41713,#41714,
#41715,#41716,#41717,#41718,#41719,#41720,#41721,#41722,#41723),(#41724,
#41725,#41726,#41727,#41728,#41729,#41730,#41731,#41732,#41733,#41734,#41735,
#41736,#41737),(#41738,#41739,#41740,#41741,#41742,#41743,#41744,#41745,
#41746,#41747,#41748,#41749,#41750,#41751),(#41752,#41753,#41754,#41755,
#41756,#41757,#41758,#41759,#41760,#41761,#41762,#41763,#41764,#41765),
(#41766,#41767,#41768,#41769,#41770,#41771,#41772,#41773,#41774,#41775,
#41776,#41777,#41778,#41779),(#41780,#41781,#41782,#41783,#41784,#41785,
#41786,#41787,#41788,#41789,#41790,#41791,#41792,#41793),(#41794,#41795,
#41796,#41797,#41798,#41799,#41800,#41801,#41802,#41803,#41804,#41805,#41806,
#41807),(#41808,#41809,#41810,#41811,#41812,#41813,#41814,#41815,#41816,
#41817,#41818,#41819,#41820,#41821),(#41822,#41823,#41824,#41825,#41826,
#41827,#41828,#41829,#41830,#41831,#41832,#41833,#41834,#41835),(#41836,
#41837,#41838,#41839,#41840,#41841,#41842,#41843,#41844,#41845,#41846,#41847,
#41848,#41849),(#41850,#41851,#41852,#41853,#41854,#41855,#41856,#41857,
#41858,#41859,#41860,#41861,#41862,#41863),(#41864,#41865,#41866,#41867,
#41868,#41869,#41870,#41871,#41872,#41873,#41874,#41875,#41876,#41877),
(#41878,#41879,#41880,#41881,#41882,#41883,#41884,#41885,#41886,#41887,
#41888,#41889,#41890,#41891),(#41892,#41893,#41894,#41895,#41896,#41897,
#41898,#41899,#41900,#41901,#41902,#41903,#41904,#41905),(#41906,#41907,
#41908,#41909,#41910,#41911,#41912,#41913,#41914,#41915,#41916,#41917,#41918,
#41919),(#41920,#41921,#41922,#41923,#41924,#41925,#41926,#41927,#41928,
#41929,#41930,#41931,#41932,#41933),(#41934,#41935,#41936,#41937,#41938,
#41939,#41940,#41941,#41942,#41943,#41944,#41945,#41946,#41947),(#41948,
#41949,#41950,#41951,#41952,#41953,#41954,#41955,#41956,#41957,#41958,#41959,
#41960,#41961),(#41962,#41963,#41964,#41965,#41966,#41967,#41968,#41969,
#41970,#41971,#41972,#41973,#41974,#41975),(#41976,#41977,#41978,#41979,
#41980,#41981,#41982,#41983,#41984,#41985,#41986,#41987,#41988,#41989),
(#41990,#41991,#41992,#41993,#41994,#41995,#41996,#41997,#41998,#41999,
#42000,#42001,#42002,#42003),(#42004,#42005,#42006,#42007,#42008,#42009,
#42010,#42011,#42012,#42013,#42014,#42015,#42016,#42017)),.UNSPECIFIED.,
 .F.,.F.,.F.,(4,1,1,1,1,1,1,1,1,1,1,1,1,1,1,1,1,1,1,1,1,1,1,1,1,1,1,4),
(4,2,2,2,2,2,4),(0.0331549352864093,0.102215297051666,0.171275658816922,
0.173433795122087,0.175591931427251,0.179908204037579,0.188540749258236,
0.20580583969955,0.214438384920208,0.223070930140865,0.240336020582179,
0.309396382347435,0.395721834554006,0.447517105877948,0.482047286760576,
0.49931237720189,0.516577467643205,0.551107648525833,0.585637829408461,
0.620168010291089,0.723758552938974,0.79281891470423,0.827349095586859,
0.861879276469487,0.896409457352115,0.930939638234743,0.948204728676058,
1.),(0.0377143719413723,0.167070624995476,0.336553194126115,0.499999999999991,
0.663446805873868,0.832929375004528,0.96228562805941),.UNSPECIFIED.);
#195=B_SPLINE_SURFACE_WITH_KNOTS('',3,3,((#42074,#42075,#42076,#42077,#42078,
#42079,#42080,#42081,#42082,#42083,#42084,#42085,#42086,#42087),(#42088,
#42089,#42090,#42091,#42092,#42093,#42094,#42095,#42096,#42097,#42098,#42099,
#42100,#42101),(#42102,#42103,#42104,#42105,#42106,#42107,#42108,#42109,
#42110,#42111,#42112,#42113,#42114,#42115),(#42116,#42117,#42118,#42119,
#42120,#42121,#42122,#42123,#42124,#42125,#42126,#42127,#42128,#42129)),
 .UNSPECIFIED.,.F.,.F.,.F.,(4,4),(4,2,2,2,2,2,4),(0.,1.),(0.0377143719414211,
0.167070624995476,0.336553194126115,0.499999999999991,0.663446805873868,
0.832929375004528,0.962285628058582),.UNSPECIFIED.);
#196=B_SPLINE_SURFACE_WITH_KNOTS('',3,3,((#42144,#42145,#42146,#42147,#42148,
#42149,#42150,#42151,#42152,#42153,#42154,#42155,#42156,#42157),(#42158,
#42159,#42160,#42161,#42162,#42163,#42164,#42165,#42166,#42167,#42168,#42169,
#42170,#42171),(#42172,#42173,#42174,#42175,#42176,#42177,#42178,#42179,
#42180,#42181,#42182,#42183,#42184,#42185),(#42186,#42187,#42188,#42189,
#42190,#42191,#42192,#42193,#42194,#42195,#42196,#42197,#42198,#42199),
(#42200,#42201,#42202,#42203,#42204,#42205,#42206,#42207,#42208,#42209,
#42210,#42211,#42212,#42213),(#42214,#42215,#42216,#42217,#42218,#42219,
#42220,#42221,#42222,#42223,#42224,#42225,#42226,#42227),(#42228,#42229,
#42230,#42231,#42232,#42233,#42234,#42235,#42236,#42237,#42238,#42239,#42240,
#42241),(#42242,#42243,#42244,#42245,#42246,#42247,#42248,#42249,#42250,
#42251,#42252,#42253,#42254,#42255),(#42256,#42257,#42258,#42259,#42260,
#42261,#42262,#42263,#42264,#42265,#42266,#42267,#42268,#42269),(#42270,
#42271,#42272,#42273,#42274,#42275,#42276,#42277,#42278,#42279,#42280,#42281,
#42282,#42283),(#42284,#42285,#42286,#42287,#42288,#42289,#42290,#42291,
#42292,#42293,#42294,#42295,#42296,#42297),(#42298,#42299,#42300,#42301,
#42302,#42303,#42304,#42305,#42306,#42307,#42308,#42309,#42310,#42311),
(#42312,#42313,#42314,#42315,#42316,#42317,#42318,#42319,#42320,#42321,
#42322,#42323,#42324,#42325),(#42326,#42327,#42328,#42329,#42330,#42331,
#42332,#42333,#42334,#42335,#42336,#42337,#42338,#42339),(#42340,#42341,
#42342,#42343,#42344,#42345,#42346,#42347,#42348,#42349,#42350,#42351,#42352,
#42353),(#42354,#42355,#42356,#42357,#42358,#42359,#42360,#42361,#42362,
#42363,#42364,#42365,#42366,#42367),(#42368,#42369,#42370,#42371,#42372,
#42373,#42374,#42375,#42376,#42377,#42378,#42379,#42380,#42381),(#42382,
#42383,#42384,#42385,#42386,#42387,#42388,#42389,#42390,#42391,#42392,#42393,
#42394,#42395),(#42396,#42397,#42398,#42399,#42400,#42401,#42402,#42403,
#42404,#42405,#42406,#42407,#42408,#42409),(#42410,#42411,#42412,#42413,
#42414,#42415,#42416,#42417,#42418,#42419,#42420,#42421,#42422,#42423),
(#42424,#42425,#42426,#42427,#42428,#42429,#42430,#42431,#42432,#42433,
#42434,#42435,#42436,#42437),(#42438,#42439,#42440,#42441,#42442,#42443,
#42444,#42445,#42446,#42447,#42448,#42449,#42450,#42451),(#42452,#42453,
#42454,#42455,#42456,#42457,#42458,#42459,#42460,#42461,#42462,#42463,#42464,
#42465),(#42466,#42467,#42468,#42469,#42470,#42471,#42472,#42473,#42474,
#42475,#42476,#42477,#42478,#42479),(#42480,#42481,#42482,#42483,#42484,
#42485,#42486,#42487,#42488,#42489,#42490,#42491,#42492,#42493),(#42494,
#42495,#42496,#42497,#42498,#42499,#42500,#42501,#42502,#42503,#42504,#42505,
#42506,#42507)),.UNSPECIFIED.,.F.,.F.,.F.,(4,1,1,1,1,1,1,1,1,1,1,1,1,1,
1,1,1,1,1,1,1,1,1,4),(4,2,2,2,2,2,4),(0.,0.0517952713240544,0.0690603617654059,
0.103590542648109,0.138120723530812,0.189915994854866,0.276241447061623,
0.310771627944326,0.414362170592435,0.431627261033787,0.483422532357841,
0.552482894123247,0.621543255888653,0.690603617654059,0.759663979419464,
0.776929069860816,0.794194160302167,0.811459250743519,0.820091795964194,
0.824408068574532,0.826566204879701,0.82872434118487,0.897784702950276,
0.966845064715682),(0.0377143719391271,0.167070624995476,0.336553194126115,
0.499999999999991,0.663446805873868,0.832929375004528,0.962285628058624),
 .UNSPECIFIED.);
#197=B_SPLINE_SURFACE_WITH_KNOTS('',3,3,((#42559,#42560,#42561,#42562,#42563,
#42564,#42565,#42566,#42567,#42568,#42569,#42570,#42571,#42572),(#42573,
#42574,#42575,#42576,#42577,#42578,#42579,#42580,#42581,#42582,#42583,#42584,
#42585,#42586),(#42587,#42588,#42589,#42590,#42591,#42592,#42593,#42594,
#42595,#42596,#42597,#42598,#42599,#42600),(#42601,#42602,#42603,#42604,
#42605,#42606,#42607,#42608,#42609,#42610,#42611,#42612,#42613,#42614),
(#42615,#42616,#42617,#42618,#42619,#42620,#42621,#42622,#42623,#42624,
#42625,#42626,#42627,#42628),(#42629,#42630,#42631,#42632,#42633,#42634,
#42635,#42636,#42637,#42638,#42639,#42640,#42641,#42642),(#42643,#42644,
#42645,#42646,#42647,#42648,#42649,#42650,#42651,#42652,#42653,#42654,#42655,
#42656),(#42657,#42658,#42659,#42660,#42661,#42662,#42663,#42664,#42665,
#42666,#42667,#42668,#42669,#42670),(#42671,#42672,#42673,#42674,#42675,
#42676,#42677,#42678,#42679,#42680,#42681,#42682,#42683,#42684),(#42685,
#42686,#42687,#42688,#42689,#42690,#42691,#42692,#42693,#42694,#42695,#42696,
#42697,#42698),(#42699,#42700,#42701,#42702,#42703,#42704,#42705,#42706,
#42707,#42708,#42709,#42710,#42711,#42712),(#42713,#42714,#42715,#42716,
#42717,#42718,#42719,#42720,#42721,#42722,#42723,#42724,#42725,#42726),
(#42727,#42728,#42729,#42730,#42731,#42732,#42733,#42734,#42735,#42736,
#42737,#42738,#42739,#42740),(#42741,#42742,#42743,#42744,#42745,#42746,
#42747,#42748,#42749,#42750,#42751,#42752,#42753,#42754),(#42755,#42756,
#42757,#42758,#42759,#42760,#42761,#42762,#42763,#42764,#42765,#42766,#42767,
#42768),(#42769,#42770,#42771,#42772,#42773,#42774,#42775,#42776,#42777,
#42778,#42779,#42780,#42781,#42782),(#42783,#42784,#42785,#42786,#42787,
#42788,#42789,#42790,#42791,#42792,#42793,#42794,#42795,#42796),(#42797,
#42798,#42799,#42800,#42801,#42802,#42803,#42804,#42805,#42806,#42807,#42808,
#42809,#42810),(#42811,#42812,#42813,#42814,#42815,#42816,#42817,#42818,
#42819,#42820,#42821,#42822,#42823,#42824),(#42825,#42826,#42827,#42828,
#42829,#42830,#42831,#42832,#42833,#42834,#42835,#42836,#42837,#42838),
(#42839,#42840,#42841,#42842,#42843,#42844,#42845,#42846,#42847,#42848,
#42849,#42850,#42851,#42852),(#42853,#42854,#42855,#42856,#42857,#42858,
#42859,#42860,#42861,#42862,#42863,#42864,#42865,#42866),(#42867,#42868,
#42869,#42870,#42871,#42872,#42873,#42874,#42875,#42876,#42877,#42878,#42879,
#42880),(#42881,#42882,#42883,#42884,#42885,#42886,#42887,#42888,#42889,
#42890,#42891,#42892,#42893,#42894),(#42895,#42896,#42897,#42898,#42899,
#42900,#42901,#42902,#42903,#42904,#42905,#42906,#42907,#42908),(#42909,
#42910,#42911,#42912,#42913,#42914,#42915,#42916,#42917,#42918,#42919,#42920,
#42921,#42922),(#42923,#42924,#42925,#42926,#42927,#42928,#42929,#42930,
#42931,#42932,#42933,#42934,#42935,#42936),(#42937,#42938,#42939,#42940,
#42941,#42942,#42943,#42944,#42945,#42946,#42947,#42948,#42949,#42950),
(#42951,#42952,#42953,#42954,#42955,#42956,#42957,#42958,#42959,#42960,
#42961,#42962,#42963,#42964),(#42965,#42966,#42967,#42968,#42969,#42970,
#42971,#42972,#42973,#42974,#42975,#42976,#42977,#42978)),.UNSPECIFIED.,
 .F.,.F.,.F.,(4,1,1,1,1,1,1,1,1,1,1,1,1,1,1,1,1,1,1,1,1,1,1,1,1,1,1,4),
(4,2,2,2,2,2,4),(0.0331549352864094,0.102215297051666,0.171275658816922,
0.173433795122087,0.175591931427251,0.179908204037579,0.188540749258236,
0.205805839699551,0.223070930140865,0.240336020582179,0.274866201464807,
0.309396382347435,0.378456744112692,0.41298692499532,0.447517105877948,
0.482047286760576,0.516577467643205,0.551107648525833,0.568372738967147,
0.585637829408461,0.689228372056346,0.723758552938974,0.810084005145545,
0.861879276469487,0.896409457352115,0.930939638234743,0.948204728676058,
1.),(0.0377143719413819,0.167070624995476,0.336553194126115,0.499999999999991,
0.663446805873868,0.832929375004528,0.962285628058676),.UNSPECIFIED.);
#198=B_SPLINE_SURFACE_WITH_KNOTS('',3,3,((#43039,#43040,#43041,#43042,#43043,
#43044,#43045,#43046,#43047,#43048,#43049,#43050,#43051,#43052),(#43053,
#43054,#43055,#43056,#43057,#43058,#43059,#43060,#43061,#43062,#43063,#43064,
#43065,#43066),(#43067,#43068,#43069,#43070,#43071,#43072,#43073,#43074,
#43075,#43076,#43077,#43078,#43079,#43080),(#43081,#43082,#43083,#43084,
#43085,#43086,#43087,#43088,#43089,#43090,#43091,#43092,#43093,#43094)),
 .UNSPECIFIED.,.F.,.F.,.F.,(4,4),(4,2,2,2,2,2,4),(0.,1.),(0.0377143719414212,
0.167070624995476,0.336553194126115,0.499999999999991,0.663446805873868,
0.832929375004528,0.962285628058582),.UNSPECIFIED.);
#199=B_SPLINE_SURFACE_WITH_KNOTS('',3,3,((#43109,#43110,#43111,#43112,#43113,
#43114,#43115,#43116,#43117,#43118,#43119,#43120,#43121,#43122),(#43123,
#43124,#43125,#43126,#43127,#43128,#43129,#43130,#43131,#43132,#43133,#43134,
#43135,#43136),(#43137,#43138,#43139,#43140,#43141,#43142,#43143,#43144,
#43145,#43146,#43147,#43148,#43149,#43150),(#43151,#43152,#43153,#43154,
#43155,#43156,#43157,#43158,#43159,#43160,#43161,#43162,#43163,#43164),
(#43165,#43166,#43167,#43168,#43169,#43170,#43171,#43172,#43173,#43174,
#43175,#43176,#43177,#43178),(#43179,#43180,#43181,#43182,#43183,#43184,
#43185,#43186,#43187,#43188,#43189,#43190,#43191,#43192),(#43193,#43194,
#43195,#43196,#43197,#43198,#43199,#43200,#43201,#43202,#43203,#43204,#43205,
#43206),(#43207,#43208,#43209,#43210,#43211,#43212,#43213,#43214,#43215,
#43216,#43217,#43218,#43219,#43220),(#43221,#43222,#43223,#43224,#43225,
#43226,#43227,#43228,#43229,#43230,#43231,#43232,#43233,#43234),(#43235,
#43236,#43237,#43238,#43239,#43240,#43241,#43242,#43243,#43244,#43245,#43246,
#43247,#43248),(#43249,#43250,#43251,#43252,#43253,#43254,#43255,#43256,
#43257,#43258,#43259,#43260,#43261,#43262),(#43263,#43264,#43265,#43266,
#43267,#43268,#43269,#43270,#43271,#43272,#43273,#43274,#43275,#43276),
(#43277,#43278,#43279,#43280,#43281,#43282,#43283,#43284,#43285,#43286,
#43287,#43288,#43289,#43290),(#43291,#43292,#43293,#43294,#43295,#43296,
#43297,#43298,#43299,#43300,#43301,#43302,#43303,#43304),(#43305,#43306,
#43307,#43308,#43309,#43310,#43311,#43312,#43313,#43314,#43315,#43316,#43317,
#43318),(#43319,#43320,#43321,#43322,#43323,#43324,#43325,#43326,#43327,
#43328,#43329,#43330,#43331,#43332),(#43333,#43334,#43335,#43336,#43337,
#43338,#43339,#43340,#43341,#43342,#43343,#43344,#43345,#43346),(#43347,
#43348,#43349,#43350,#43351,#43352,#43353,#43354,#43355,#43356,#43357,#43358,
#43359,#43360),(#43361,#43362,#43363,#43364,#43365,#43366,#43367,#43368,
#43369,#43370,#43371,#43372,#43373,#43374),(#43375,#43376,#43377,#43378,
#43379,#43380,#43381,#43382,#43383,#43384,#43385,#43386,#43387,#43388),
(#43389,#43390,#43391,#43392,#43393,#43394,#43395,#43396,#43397,#43398,
#43399,#43400,#43401,#43402),(#43403,#43404,#43405,#43406,#43407,#43408,
#43409,#43410,#43411,#43412,#43413,#43414,#43415,#43416),(#43417,#43418,
#43419,#43420,#43421,#43422,#43423,#43424,#43425,#43426,#43427,#43428,#43429,
#43430),(#43431,#43432,#43433,#43434,#43435,#43436,#43437,#43438,#43439,
#43440,#43441,#43442,#43443,#43444),(#43445,#43446,#43447,#43448,#43449,
#43450,#43451,#43452,#43453,#43454,#43455,#43456,#43457,#43458),(#43459,
#43460,#43461,#43462,#43463,#43464,#43465,#43466,#43467,#43468,#43469,#43470,
#43471,#43472),(#43473,#43474,#43475,#43476,#43477,#43478,#43479,#43480,
#43481,#43482,#43483,#43484,#43485,#43486),(#43487,#43488,#43489,#43490,
#43491,#43492,#43493,#43494,#43495,#43496,#43497,#43498,#43499,#43500),
(#43501,#43502,#43503,#43504,#43505,#43506,#43507,#43508,#43509,#43510,
#43511,#43512,#43513,#43514),(#43515,#43516,#43517,#43518,#43519,#43520,
#43521,#43522,#43523,#43524,#43525,#43526,#43527,#43528),(#43529,#43530,
#43531,#43532,#43533,#43534,#43535,#43536,#43537,#43538,#43539,#43540,#43541,
#43542)),.UNSPECIFIED.,.F.,.F.,.F.,(4,1,1,1,1,1,1,1,1,1,1,1,1,1,1,1,1,1,
1,1,1,1,1,1,1,1,1,1,4),(4,2,2,2,2,2,4),(0.,0.0517952713240544,0.0690603617654058,
0.103590542648109,0.138120723530812,0.155385813972163,0.189915994854866,
0.276241447061623,0.345301808827029,0.397097080151083,0.414362170592435,
0.448892351475138,0.552482894123247,0.621543255888652,0.690603617654058,
0.725133798536761,0.759663979419464,0.76829652464014,0.776929069860816,
0.794194160302167,0.811459250743518,0.815775523353856,0.820091795964194,
0.824408068574532,0.826566204879701,0.827645273032285,0.82872434118487,
0.897784702950276,0.966845064715681),(0.037714371940714,0.167070624995476,
0.336553194126115,0.499999999999991,0.663446805873868,0.832929375004528,
0.962285628059076),.UNSPECIFIED.);
#200=B_SPLINE_SURFACE_WITH_KNOTS('',3,3,((#43594,#43595,#43596,#43597,#43598,
#43599,#43600,#43601,#43602,#43603,#43604,#43605,#43606,#43607),(#43608,
#43609,#43610,#43611,#43612,#43613,#43614,#43615,#43616,#43617,#43618,#43619,
#43620,#43621),(#43622,#43623,#43624,#43625,#43626,#43627,#43628,#43629,
#43630,#43631,#43632,#43633,#43634,#43635),(#43636,#43637,#43638,#43639,
#43640,#43641,#43642,#43643,#43644,#43645,#43646,#43647,#43648,#43649),
(#43650,#43651,#43652,#43653,#43654,#43655,#43656,#43657,#43658,#43659,
#43660,#43661,#43662,#43663),(#43664,#43665,#43666,#43667,#43668,#43669,
#43670,#43671,#43672,#43673,#43674,#43675,#43676,#43677),(#43678,#43679,
#43680,#43681,#43682,#43683,#43684,#43685,#43686,#43687,#43688,#43689,#43690,
#43691),(#43692,#43693,#43694,#43695,#43696,#43697,#43698,#43699,#43700,
#43701,#43702,#43703,#43704,#43705),(#43706,#43707,#43708,#43709,#43710,
#43711,#43712,#43713,#43714,#43715,#43716,#43717,#43718,#43719),(#43720,
#43721,#43722,#43723,#43724,#43725,#43726,#43727,#43728,#43729,#43730,#43731,
#43732,#43733),(#43734,#43735,#43736,#43737,#43738,#43739,#43740,#43741,
#43742,#43743,#43744,#43745,#43746,#43747),(#43748,#43749,#43750,#43751,
#43752,#43753,#43754,#43755,#43756,#43757,#43758,#43759,#43760,#43761),
(#43762,#43763,#43764,#43765,#43766,#43767,#43768,#43769,#43770,#43771,
#43772,#43773,#43774,#43775),(#43776,#43777,#43778,#43779,#43780,#43781,
#43782,#43783,#43784,#43785,#43786,#43787,#43788,#43789),(#43790,#43791,
#43792,#43793,#43794,#43795,#43796,#43797,#43798,#43799,#43800,#43801,#43802,
#43803),(#43804,#43805,#43806,#43807,#43808,#43809,#43810,#43811,#43812,
#43813,#43814,#43815,#43816,#43817),(#43818,#43819,#43820,#43821,#43822,
#43823,#43824,#43825,#43826,#43827,#43828,#43829,#43830,#43831),(#43832,
#43833,#43834,#43835,#43836,#43837,#43838,#43839,#43840,#43841,#43842,#43843,
#43844,#43845),(#43846,#43847,#43848,#43849,#43850,#43851,#43852,#43853,
#43854,#43855,#43856,#43857,#43858,#43859),(#43860,#43861,#43862,#43863,
#43864,#43865,#43866,#43867,#43868,#43869,#43870,#43871,#43872,#43873),
(#43874,#43875,#43876,#43877,#43878,#43879,#43880,#43881,#43882,#43883,
#43884,#43885,#43886,#43887),(#43888,#43889,#43890,#43891,#43892,#43893,
#43894,#43895,#43896,#43897,#43898,#43899,#43900,#43901),(#43902,#43903,
#43904,#43905,#43906,#43907,#43908,#43909,#43910,#43911,#43912,#43913,#43914,
#43915),(#43916,#43917,#43918,#43919,#43920,#43921,#43922,#43923,#43924,
#43925,#43926,#43927,#43928,#43929),(#43930,#43931,#43932,#43933,#43934,
#43935,#43936,#43937,#43938,#43939,#43940,#43941,#43942,#43943),(#43944,
#43945,#43946,#43947,#43948,#43949,#43950,#43951,#43952,#43953,#43954,#43955,
#43956,#43957),(#43958,#43959,#43960,#43961,#43962,#43963,#43964,#43965,
#43966,#43967,#43968,#43969,#43970,#43971),(#43972,#43973,#43974,#43975,
#43976,#43977,#43978,#43979,#43980,#43981,#43982,#43983,#43984,#43985),
(#43986,#43987,#43988,#43989,#43990,#43991,#43992,#43993,#43994,#43995,
#43996,#43997,#43998,#43999),(#44000,#44001,#44002,#44003,#44004,#44005,
#44006,#44007,#44008,#44009,#44010,#44011,#44012,#44013),(#44014,#44015,
#44016,#44017,#44018,#44019,#44020,#44021,#44022,#44023,#44024,#44025,#44026,
#44027)),.UNSPECIFIED.,.F.,.F.,.F.,(4,1,1,1,1,1,1,1,1,1,1,1,1,1,1,1,1,1,
1,1,1,1,1,1,1,1,1,1,4),(4,2,2,2,2,2,4),(0.0331549352864062,0.102215297051663,
0.136745477934291,0.17127565881692,0.173433795122084,0.175591931427248,
0.179908204037577,0.188540749258234,0.197173294478891,0.205805839699548,
0.223070930140862,0.240336020582176,0.274866201464805,0.309396382347433,
0.37845674411269,0.412986924995318,0.430252015436632,0.447517105877946,
0.516577467643203,0.58563782940846,0.654698191173716,0.689228372056345,
0.723758552938973,0.827349095586858,0.861879276469486,0.896409457352115,
0.930939638234743,0.948204728676057,1.),(0.0377143719407421,0.167070624995476,
0.336553194126115,0.499999999999991,0.663446805873868,0.832929375004528,
0.962285628059324),.UNSPECIFIED.);
#201=B_SPLINE_SURFACE_WITH_KNOTS('',3,3,((#44088,#44089,#44090,#44091,#44092,
#44093,#44094,#44095,#44096,#44097,#44098,#44099,#44100,#44101),(#44102,
#44103,#44104,#44105,#44106,#44107,#44108,#44109,#44110,#44111,#44112,#44113,
#44114,#44115),(#44116,#44117,#44118,#44119,#44120,#44121,#44122,#44123,
#44124,#44125,#44126,#44127,#44128,#44129),(#44130,#44131,#44132,#44133,
#44134,#44135,#44136,#44137,#44138,#44139,#44140,#44141,#44142,#44143)),
 .UNSPECIFIED.,.F.,.F.,.F.,(4,4),(4,2,2,2,2,2,4),(0.,1.),(0.0377143719414212,
0.167070624995476,0.336553194126115,0.499999999999991,0.663446805873868,
0.832929375004528,0.962285628058582),.UNSPECIFIED.);
#202=B_SPLINE_SURFACE_WITH_KNOTS('',3,3,((#44158,#44159,#44160,#44161,#44162,
#44163,#44164,#44165,#44166,#44167,#44168,#44169,#44170,#44171),(#44172,
#44173,#44174,#44175,#44176,#44177,#44178,#44179,#44180,#44181,#44182,#44183,
#44184,#44185),(#44186,#44187,#44188,#44189,#44190,#44191,#44192,#44193,
#44194,#44195,#44196,#44197,#44198,#44199),(#44200,#44201,#44202,#44203,
#44204,#44205,#44206,#44207,#44208,#44209,#44210,#44211,#44212,#44213),
(#44214,#44215,#44216,#44217,#44218,#44219,#44220,#44221,#44222,#44223,
#44224,#44225,#44226,#44227),(#44228,#44229,#44230,#44231,#44232,#44233,
#44234,#44235,#44236,#44237,#44238,#44239,#44240,#44241),(#44242,#44243,
#44244,#44245,#44246,#44247,#44248,#44249,#44250,#44251,#44252,#44253,#44254,
#44255),(#44256,#44257,#44258,#44259,#44260,#44261,#44262,#44263,#44264,
#44265,#44266,#44267,#44268,#44269),(#44270,#44271,#44272,#44273,#44274,
#44275,#44276,#44277,#44278,#44279,#44280,#44281,#44282,#44283),(#44284,
#44285,#44286,#44287,#44288,#44289,#44290,#44291,#44292,#44293,#44294,#44295,
#44296,#44297),(#44298,#44299,#44300,#44301,#44302,#44303,#44304,#44305,
#44306,#44307,#44308,#44309,#44310,#44311),(#44312,#44313,#44314,#44315,
#44316,#44317,#44318,#44319,#44320,#44321,#44322,#44323,#44324,#44325),
(#44326,#44327,#44328,#44329,#44330,#44331,#44332,#44333,#44334,#44335,
#44336,#44337,#44338,#44339),(#44340,#44341,#44342,#44343,#44344,#44345,
#44346,#44347,#44348,#44349,#44350,#44351,#44352,#44353),(#44354,#44355,
#44356,#44357,#44358,#44359,#44360,#44361,#44362,#44363,#44364,#44365,#44366,
#44367),(#44368,#44369,#44370,#44371,#44372,#44373,#44374,#44375,#44376,
#44377,#44378,#44379,#44380,#44381),(#44382,#44383,#44384,#44385,#44386,
#44387,#44388,#44389,#44390,#44391,#44392,#44393,#44394,#44395),(#44396,
#44397,#44398,#44399,#44400,#44401,#44402,#44403,#44404,#44405,#44406,#44407,
#44408,#44409),(#44410,#44411,#44412,#44413,#44414,#44415,#44416,#44417,
#44418,#44419,#44420,#44421,#44422,#44423),(#44424,#44425,#44426,#44427,
#44428,#44429,#44430,#44431,#44432,#44433,#44434,#44435,#44436,#44437),
(#44438,#44439,#44440,#44441,#44442,#44443,#44444,#44445,#44446,#44447,
#44448,#44449,#44450,#44451),(#44452,#44453,#44454,#44455,#44456,#44457,
#44458,#44459,#44460,#44461,#44462,#44463,#44464,#44465),(#44466,#44467,
#44468,#44469,#44470,#44471,#44472,#44473,#44474,#44475,#44476,#44477,#44478,
#44479),(#44480,#44481,#44482,#44483,#44484,#44485,#44486,#44487,#44488,
#44489,#44490,#44491,#44492,#44493),(#44494,#44495,#44496,#44497,#44498,
#44499,#44500,#44501,#44502,#44503,#44504,#44505,#44506,#44507),(#44508,
#44509,#44510,#44511,#44512,#44513,#44514,#44515,#44516,#44517,#44518,#44519,
#44520,#44521),(#44522,#44523,#44524,#44525,#44526,#44527,#44528,#44529,
#44530,#44531,#44532,#44533,#44534,#44535),(#44536,#44537,#44538,#44539,
#44540,#44541,#44542,#44543,#44544,#44545,#44546,#44547,#44548,#44549),
(#44550,#44551,#44552,#44553,#44554,#44555,#44556,#44557,#44558,#44559,
#44560,#44561,#44562,#44563),(#44564,#44565,#44566,#44567,#44568,#44569,
#44570,#44571,#44572,#44573,#44574,#44575,#44576,#44577),(#44578,#44579,
#44580,#44581,#44582,#44583,#44584,#44585,#44586,#44587,#44588,#44589,#44590,
#44591),(#44592,#44593,#44594,#44595,#44596,#44597,#44598,#44599,#44600,
#44601,#44602,#44603,#44604,#44605),(#44606,#44607,#44608,#44609,#44610,
#44611,#44612,#44613,#44614,#44615,#44616,#44617,#44618,#44619),(#44620,
#44621,#44622,#44623,#44624,#44625,#44626,#44627,#44628,#44629,#44630,#44631,
#44632,#44633),(#44634,#44635,#44636,#44637,#44638,#44639,#44640,#44641,
#44642,#44643,#44644,#44645,#44646,#44647)),.UNSPECIFIED.,.F.,.F.,.F.,(4,
1,1,1,1,1,1,1,1,1,1,1,1,1,1,1,1,1,1,1,1,1,1,1,1,1,1,1,1,1,1,1,4),(4,2,2,
2,2,2,4),(0.,0.0517952713240545,0.069060361765406,0.0863254522067576,0.103590542648109,
0.138120723530812,0.155385813972164,0.189915994854867,0.207181085296218,
0.276241447061624,0.34530180882703,0.379831989709733,0.414362170592436,
0.448892351475139,0.483422532357842,0.517952713240545,0.552482894123248,
0.587013075005951,0.656073436771357,0.69060361765406,0.725133798536763,
0.759663979419467,0.785561615081494,0.79419416030217,0.811459250743521,
0.815775523353859,0.820091795964197,0.824408068574535,0.828724341184873,
0.880519612508927,0.897784702950279,0.932314883832982,0.966845064715685),
(0.0377143719406521,0.167070624995476,0.336553194126115,0.499999999999991,
0.663446805873868,0.832929375004528,0.962285628059093),.UNSPECIFIED.);
#203=B_SPLINE_SURFACE_WITH_KNOTS('',3,3,((#44699,#44700,#44701,#44702,#44703,
#44704,#44705,#44706,#44707,#44708,#44709,#44710,#44711,#44712),(#44713,
#44714,#44715,#44716,#44717,#44718,#44719,#44720,#44721,#44722,#44723,#44724,
#44725,#44726),(#44727,#44728,#44729,#44730,#44731,#44732,#44733,#44734,
#44735,#44736,#44737,#44738,#44739,#44740),(#44741,#44742,#44743,#44744,
#44745,#44746,#44747,#44748,#44749,#44750,#44751,#44752,#44753,#44754),
(#44755,#44756,#44757,#44758,#44759,#44760,#44761,#44762,#44763,#44764,
#44765,#44766,#44767,#44768),(#44769,#44770,#44771,#44772,#44773,#44774,
#44775,#44776,#44777,#44778,#44779,#44780,#44781,#44782),(#44783,#44784,
#44785,#44786,#44787,#44788,#44789,#44790,#44791,#44792,#44793,#44794,#44795,
#44796),(#44797,#44798,#44799,#44800,#44801,#44802,#44803,#44804,#44805,
#44806,#44807,#44808,#44809,#44810),(#44811,#44812,#44813,#44814,#44815,
#44816,#44817,#44818,#44819,#44820,#44821,#44822,#44823,#44824),(#44825,
#44826,#44827,#44828,#44829,#44830,#44831,#44832,#44833,#44834,#44835,#44836,
#44837,#44838),(#44839,#44840,#44841,#44842,#44843,#44844,#44845,#44846,
#44847,#44848,#44849,#44850,#44851,#44852),(#44853,#44854,#44855,#44856,
#44857,#44858,#44859,#44860,#44861,#44862,#44863,#44864,#44865,#44866),
(#44867,#44868,#44869,#44870,#44871,#44872,#44873,#44874,#44875,#44876,
#44877,#44878,#44879,#44880),(#44881,#44882,#44883,#44884,#44885,#44886,
#44887,#44888,#44889,#44890,#44891,#44892,#44893,#44894),(#44895,#44896,
#44897,#44898,#44899,#44900,#44901,#44902,#44903,#44904,#44905,#44906,#44907,
#44908),(#44909,#44910,#44911,#44912,#44913,#44914,#44915,#44916,#44917,
#44918,#44919,#44920,#44921,#44922),(#44923,#44924,#44925,#44926,#44927,
#44928,#44929,#44930,#44931,#44932,#44933,#44934,#44935,#44936),(#44937,
#44938,#44939,#44940,#44941,#44942,#44943,#44944,#44945,#44946,#44947,#44948,
#44949,#44950),(#44951,#44952,#44953,#44954,#44955,#44956,#44957,#44958,
#44959,#44960,#44961,#44962,#44963,#44964),(#44965,#44966,#44967,#44968,
#44969,#44970,#44971,#44972,#44973,#44974,#44975,#44976,#44977,#44978),
(#44979,#44980,#44981,#44982,#44983,#44984,#44985,#44986,#44987,#44988,
#44989,#44990,#44991,#44992),(#44993,#44994,#44995,#44996,#44997,#44998,
#44999,#45000,#45001,#45002,#45003,#45004,#45005,#45006),(#45007,#45008,
#45009,#45010,#45011,#45012,#45013,#45014,#45015,#45016,#45017,#45018,#45019,
#45020),(#45021,#45022,#45023,#45024,#45025,#45026,#45027,#45028,#45029,
#45030,#45031,#45032,#45033,#45034),(#45035,#45036,#45037,#45038,#45039,
#45040,#45041,#45042,#45043,#45044,#45045,#45046,#45047,#45048),(#45049,
#45050,#45051,#45052,#45053,#45054,#45055,#45056,#45057,#45058,#45059,#45060,
#45061,#45062),(#45063,#45064,#45065,#45066,#45067,#45068,#45069,#45070,
#45071,#45072,#45073,#45074,#45075,#45076),(#45077,#45078,#45079,#45080,
#45081,#45082,#45083,#45084,#45085,#45086,#45087,#45088,#45089,#45090)),
 .UNSPECIFIED.,.F.,.F.,.F.,(4,1,1,1,1,1,1,1,1,1,1,1,1,1,1,1,1,1,1,1,1,1,
1,1,1,4),(4,2,2,2,2,2,4),(0.0331549352864051,0.102215297051662,0.171275658816919,
0.175591931427247,0.179908204037576,0.188540749258233,0.205805839699547,
0.223070930140861,0.240336020582175,0.274866201464804,0.309396382347432,
0.378456744112689,0.412986924995317,0.430252015436631,0.447517105877946,
0.516577467643203,0.585637829408459,0.654698191173716,0.689228372056344,
0.723758552938973,0.827349095586858,0.861879276469486,0.896409457352115,
0.930939638234743,0.948204728676057,1.),(0.0377143719409181,0.167070624995476,
0.336553194126115,0.499999999999991,0.663446805873868,0.832929375004528,
0.962285628059611),.UNSPECIFIED.);
#204=B_SPLINE_SURFACE_WITH_KNOTS('',3,3,((#45149,#45150,#45151,#45152,#45153,
#45154,#45155,#45156,#45157,#45158,#45159,#45160,#45161,#45162),(#45163,
#45164,#45165,#45166,#45167,#45168,#45169,#45170,#45171,#45172,#45173,#45174,
#45175,#45176),(#45177,#45178,#45179,#45180,#45181,#45182,#45183,#45184,
#45185,#45186,#45187,#45188,#45189,#45190),(#45191,#45192,#45193,#45194,
#45195,#45196,#45197,#45198,#45199,#45200,#45201,#45202,#45203,#45204)),
 .UNSPECIFIED.,.F.,.F.,.F.,(4,4),(4,2,2,2,2,2,4),(0.,1.),(0.0377143719414212,
0.167070624995476,0.336553194126115,0.499999999999991,0.663446805873868,
0.832929375004528,0.962285628058582),.UNSPECIFIED.);
#205=B_SPLINE_SURFACE_WITH_KNOTS('',3,3,((#45219,#45220,#45221,#45222,#45223,
#45224,#45225,#45226,#45227,#45228,#45229,#45230,#45231,#45232),(#45233,
#45234,#45235,#45236,#45237,#45238,#45239,#45240,#45241,#45242,#45243,#45244,
#45245,#45246),(#45247,#45248,#45249,#45250,#45251,#45252,#45253,#45254,
#45255,#45256,#45257,#45258,#45259,#45260),(#45261,#45262,#45263,#45264,
#45265,#45266,#45267,#45268,#45269,#45270,#45271,#45272,#45273,#45274),
(#45275,#45276,#45277,#45278,#45279,#45280,#45281,#45282,#45283,#45284,
#45285,#45286,#45287,#45288),(#45289,#45290,#45291,#45292,#45293,#45294,
#45295,#45296,#45297,#45298,#45299,#45300,#45301,#45302),(#45303,#45304,
#45305,#45306,#45307,#45308,#45309,#45310,#45311,#45312,#45313,#45314,#45315,
#45316),(#45317,#45318,#45319,#45320,#45321,#45322,#45323,#45324,#45325,
#45326,#45327,#45328,#45329,#45330),(#45331,#45332,#45333,#45334,#45335,
#45336,#45337,#45338,#45339,#45340,#45341,#45342,#45343,#45344),(#45345,
#45346,#45347,#45348,#45349,#45350,#45351,#45352,#45353,#45354,#45355,#45356,
#45357,#45358),(#45359,#45360,#45361,#45362,#45363,#45364,#45365,#45366,
#45367,#45368,#45369,#45370,#45371,#45372),(#45373,#45374,#45375,#45376,
#45377,#45378,#45379,#45380,#45381,#45382,#45383,#45384,#45385,#45386),
(#45387,#45388,#45389,#45390,#45391,#45392,#45393,#45394,#45395,#45396,
#45397,#45398,#45399,#45400),(#45401,#45402,#45403,#45404,#45405,#45406,
#45407,#45408,#45409,#45410,#45411,#45412,#45413,#45414),(#45415,#45416,
#45417,#45418,#45419,#45420,#45421,#45422,#45423,#45424,#45425,#45426,#45427,
#45428),(#45429,#45430,#45431,#45432,#45433,#45434,#45435,#45436,#45437,
#45438,#45439,#45440,#45441,#45442),(#45443,#45444,#45445,#45446,#45447,
#45448,#45449,#45450,#45451,#45452,#45453,#45454,#45455,#45456),(#45457,
#45458,#45459,#45460,#45461,#45462,#45463,#45464,#45465,#45466,#45467,#45468,
#45469,#45470),(#45471,#45472,#45473,#45474,#45475,#45476,#45477,#45478,
#45479,#45480,#45481,#45482,#45483,#45484),(#45485,#45486,#45487,#45488,
#45489,#45490,#45491,#45492,#45493,#45494,#45495,#45496,#45497,#45498),
(#45499,#45500,#45501,#45502,#45503,#45504,#45505,#45506,#45507,#45508,
#45509,#45510,#45511,#45512),(#45513,#45514,#45515,#45516,#45517,#45518,
#45519,#45520,#45521,#45522,#45523,#45524,#45525,#45526),(#45527,#45528,
#45529,#45530,#45531,#45532,#45533,#45534,#45535,#45536,#45537,#45538,#45539,
#45540),(#45541,#45542,#45543,#45544,#45545,#45546,#45547,#45548,#45549,
#45550,#45551,#45552,#45553,#45554),(#45555,#45556,#45557,#45558,#45559,
#45560,#45561,#45562,#45563,#45564,#45565,#45566,#45567,#45568),(#45569,
#45570,#45571,#45572,#45573,#45574,#45575,#45576,#45577,#45578,#45579,#45580,
#45581,#45582)),.UNSPECIFIED.,.F.,.F.,.F.,(4,1,1,1,1,1,1,1,1,1,1,1,1,1,
1,1,1,1,1,1,1,1,1,4),(4,2,2,2,2,2,4),(0.,0.0517952713240545,0.0690603617654061,
0.103590542648109,0.138120723530812,0.155385813972164,0.276241447061624,
0.310771627944327,0.34530180882703,0.414362170592436,0.483422532357842,
0.535217803681897,0.552482894123248,0.621543255888655,0.656073436771358,
0.690603617654061,0.725133798536764,0.759663979419467,0.79419416030217,
0.811459250743521,0.820091795964197,0.828724341184873,0.897784702950279,
0.966845064715685),(0.037714371941385,0.167070624995476,0.336553194126115,
0.499999999999991,0.663446805873868,0.832929375004528,0.962285628060415),
 .UNSPECIFIED.);
#206=B_SPLINE_SURFACE_WITH_KNOTS('',3,3,((#45642,#45643,#45644,#45645,#45646,
#45647,#45648,#45649,#45650,#45651,#45652,#45653,#45654,#45655),(#45656,
#45657,#45658,#45659,#45660,#45661,#45662,#45663,#45664,#45665,#45666,#45667,
#45668,#45669),(#45670,#45671,#45672,#45673,#45674,#45675,#45676,#45677,
#45678,#45679,#45680,#45681,#45682,#45683),(#45684,#45685,#45686,#45687,
#45688,#45689,#45690,#45691,#45692,#45693,#45694,#45695,#45696,#45697),
(#45698,#45699,#45700,#45701,#45702,#45703,#45704,#45705,#45706,#45707,
#45708,#45709,#45710,#45711),(#45712,#45713,#45714,#45715,#45716,#45717,
#45718,#45719,#45720,#45721,#45722,#45723,#45724,#45725),(#45726,#45727,
#45728,#45729,#45730,#45731,#45732,#45733,#45734,#45735,#45736,#45737,#45738,
#45739),(#45740,#45741,#45742,#45743,#45744,#45745,#45746,#45747,#45748,
#45749,#45750,#45751,#45752,#45753),(#45754,#45755,#45756,#45757,#45758,
#45759,#45760,#45761,#45762,#45763,#45764,#45765,#45766,#45767),(#45768,
#45769,#45770,#45771,#45772,#45773,#45774,#45775,#45776,#45777,#45778,#45779,
#45780,#45781),(#45782,#45783,#45784,#45785,#45786,#45787,#45788,#45789,
#45790,#45791,#45792,#45793,#45794,#45795),(#45796,#45797,#45798,#45799,
#45800,#45801,#45802,#45803,#45804,#45805,#45806,#45807,#45808,#45809),
(#45810,#45811,#45812,#45813,#45814,#45815,#45816,#45817,#45818,#45819,
#45820,#45821,#45822,#45823),(#45824,#45825,#45826,#45827,#45828,#45829,
#45830,#45831,#45832,#45833,#45834,#45835,#45836,#45837),(#45838,#45839,
#45840,#45841,#45842,#45843,#45844,#45845,#45846,#45847,#45848,#45849,#45850,
#45851),(#45852,#45853,#45854,#45855,#45856,#45857,#45858,#45859,#45860,
#45861,#45862,#45863,#45864,#45865),(#45866,#45867,#45868,#45869,#45870,
#45871,#45872,#45873,#45874,#45875,#45876,#45877,#45878,#45879),(#45880,
#45881,#45882,#45883,#45884,#45885,#45886,#45887,#45888,#45889,#45890,#45891,
#45892,#45893),(#45894,#45895,#45896,#45897,#45898,#45899,#45900,#45901,
#45902,#45903,#45904,#45905,#45906,#45907),(#45908,#45909,#45910,#45911,
#45912,#45913,#45914,#45915,#45916,#45917,#45918,#45919,#45920,#45921),
(#45922,#45923,#45924,#45925,#45926,#45927,#45928,#45929,#45930,#45931,
#45932,#45933,#45934,#45935),(#45936,#45937,#45938,#45939,#45940,#45941,
#45942,#45943,#45944,#45945,#45946,#45947,#45948,#45949),(#45950,#45951,
#45952,#45953,#45954,#45955,#45956,#45957,#45958,#45959,#45960,#45961,#45962,
#45963),(#45964,#45965,#45966,#45967,#45968,#45969,#45970,#45971,#45972,
#45973,#45974,#45975,#45976,#45977),(#45978,#45979,#45980,#45981,#45982,
#45983,#45984,#45985,#45986,#45987,#45988,#45989,#45990,#45991),(#45992,
#45993,#45994,#45995,#45996,#45997,#45998,#45999,#46000,#46001,#46002,#46003,
#46004,#46005)),.UNSPECIFIED.,.F.,.F.,.F.,(4,1,1,1,1,1,1,1,1,1,1,1,1,1,
1,1,1,1,1,1,1,1,1,4),(4,2,2,2,2,2,4),(0.0331549352864075,0.102215297051664,
0.171275658816921,0.175591931427249,0.179908204037578,0.188540749258235,
0.205805839699549,0.223070930140863,0.240336020582177,0.309396382347434,
0.37845674411269,0.412986924995319,0.430252015436633,0.447517105877947,
0.58563782940846,0.620168010291089,0.671963281615031,0.723758552938974,
0.810084005145544,0.861879276469487,0.896409457352115,0.930939638234743,
0.948204728676058,1.),(0.0377143719412197,0.167070624995476,0.336553194126115,
0.499999999999991,0.663446805873868,0.832929375004528,0.962285628058676),
 .UNSPECIFIED.);
#207=B_SPLINE_SURFACE_WITH_KNOTS('',3,3,((#46064,#46065,#46066,#46067,#46068,
#46069,#46070,#46071,#46072,#46073,#46074,#46075,#46076,#46077),(#46078,
#46079,#46080,#46081,#46082,#46083,#46084,#46085,#46086,#46087,#46088,#46089,
#46090,#46091),(#46092,#46093,#46094,#46095,#46096,#46097,#46098,#46099,
#46100,#46101,#46102,#46103,#46104,#46105),(#46106,#46107,#46108,#46109,
#46110,#46111,#46112,#46113,#46114,#46115,#46116,#46117,#46118,#46119)),
 .UNSPECIFIED.,.F.,.F.,.F.,(4,4),(4,2,2,2,2,2,4),(0.,1.),(0.0377143719414212,
0.167070624995476,0.336553194126115,0.499999999999991,0.663446805873868,
0.832929375004528,0.962285628058582),.UNSPECIFIED.);
#208=B_SPLINE_SURFACE_WITH_KNOTS('',3,3,((#46134,#46135,#46136,#46137,#46138,
#46139,#46140,#46141,#46142,#46143,#46144,#46145,#46146,#46147),(#46148,
#46149,#46150,#46151,#46152,#46153,#46154,#46155,#46156,#46157,#46158,#46159,
#46160,#46161),(#46162,#46163,#46164,#46165,#46166,#46167,#46168,#46169,
#46170,#46171,#46172,#46173,#46174,#46175),(#46176,#46177,#46178,#46179,
#46180,#46181,#46182,#46183,#46184,#46185,#46186,#46187,#46188,#46189),
(#46190,#46191,#46192,#46193,#46194,#46195,#46196,#46197,#46198,#46199,
#46200,#46201,#46202,#46203),(#46204,#46205,#46206,#46207,#46208,#46209,
#46210,#46211,#46212,#46213,#46214,#46215,#46216,#46217),(#46218,#46219,
#46220,#46221,#46222,#46223,#46224,#46225,#46226,#46227,#46228,#46229,#46230,
#46231),(#46232,#46233,#46234,#46235,#46236,#46237,#46238,#46239,#46240,
#46241,#46242,#46243,#46244,#46245),(#46246,#46247,#46248,#46249,#46250,
#46251,#46252,#46253,#46254,#46255,#46256,#46257,#46258,#46259),(#46260,
#46261,#46262,#46263,#46264,#46265,#46266,#46267,#46268,#46269,#46270,#46271,
#46272,#46273),(#46274,#46275,#46276,#46277,#46278,#46279,#46280,#46281,
#46282,#46283,#46284,#46285,#46286,#46287),(#46288,#46289,#46290,#46291,
#46292,#46293,#46294,#46295,#46296,#46297,#46298,#46299,#46300,#46301),
(#46302,#46303,#46304,#46305,#46306,#46307,#46308,#46309,#46310,#46311,
#46312,#46313,#46314,#46315),(#46316,#46317,#46318,#46319,#46320,#46321,
#46322,#46323,#46324,#46325,#46326,#46327,#46328,#46329),(#46330,#46331,
#46332,#46333,#46334,#46335,#46336,#46337,#46338,#46339,#46340,#46341,#46342,
#46343),(#46344,#46345,#46346,#46347,#46348,#46349,#46350,#46351,#46352,
#46353,#46354,#46355,#46356,#46357),(#46358,#46359,#46360,#46361,#46362,
#46363,#46364,#46365,#46366,#46367,#46368,#46369,#46370,#46371),(#46372,
#46373,#46374,#46375,#46376,#46377,#46378,#46379,#46380,#46381,#46382,#46383,
#46384,#46385),(#46386,#46387,#46388,#46389,#46390,#46391,#46392,#46393,
#46394,#46395,#46396,#46397,#46398,#46399),(#46400,#46401,#46402,#46403,
#46404,#46405,#46406,#46407,#46408,#46409,#46410,#46411,#46412,#46413),
(#46414,#46415,#46416,#46417,#46418,#46419,#46420,#46421,#46422,#46423,
#46424,#46425,#46426,#46427),(#46428,#46429,#46430,#46431,#46432,#46433,
#46434,#46435,#46436,#46437,#46438,#46439,#46440,#46441),(#46442,#46443,
#46444,#46445,#46446,#46447,#46448,#46449,#46450,#46451,#46452,#46453,#46454,
#46455),(#46456,#46457,#46458,#46459,#46460,#46461,#46462,#46463,#46464,
#46465,#46466,#46467,#46468,#46469),(#46470,#46471,#46472,#46473,#46474,
#46475,#46476,#46477,#46478,#46479,#46480,#46481,#46482,#46483),(#46484,
#46485,#46486,#46487,#46488,#46489,#46490,#46491,#46492,#46493,#46494,#46495,
#46496,#46497),(#46498,#46499,#46500,#46501,#46502,#46503,#46504,#46505,
#46506,#46507,#46508,#46509,#46510,#46511)),.UNSPECIFIED.,.F.,.F.,.F.,(4,
1,1,1,1,1,1,1,1,1,1,1,1,1,1,1,1,1,1,1,1,1,1,1,4),(4,2,2,2,2,2,4),(0.,0.0517952713240545,
0.0690603617654059,0.103590542648109,0.138120723530812,0.155385813972163,
0.189915994854866,0.276241447061624,0.34530180882703,0.379831989709733,
0.414362170592436,0.448892351475139,0.552482894123247,0.621543255888653,
0.690603617654059,0.759663979419465,0.768296524640141,0.776929069860817,
0.794194160302168,0.81145925074352,0.820091795964196,0.828724341184871,
0.897784702950277,0.93231488383298,0.966845064715683),(0.0377143719404219,
0.167070624995476,0.336553194126115,0.499999999999991,0.663446805873868,
0.832929375004528,0.962285628059789),.UNSPECIFIED.);
#209=B_SPLINE_SURFACE_WITH_KNOTS('',3,3,((#46567,#46568,#46569,#46570,#46571,
#46572,#46573,#46574,#46575,#46576,#46577,#46578,#46579,#46580),(#46581,
#46582,#46583,#46584,#46585,#46586,#46587,#46588,#46589,#46590,#46591,#46592,
#46593,#46594),(#46595,#46596,#46597,#46598,#46599,#46600,#46601,#46602,
#46603,#46604,#46605,#46606,#46607,#46608),(#46609,#46610,#46611,#46612,
#46613,#46614,#46615,#46616,#46617,#46618,#46619,#46620,#46621,#46622),
(#46623,#46624,#46625,#46626,#46627,#46628,#46629,#46630,#46631,#46632,
#46633,#46634,#46635,#46636),(#46637,#46638,#46639,#46640,#46641,#46642,
#46643,#46644,#46645,#46646,#46647,#46648,#46649,#46650),(#46651,#46652,
#46653,#46654,#46655,#46656,#46657,#46658,#46659,#46660,#46661,#46662,#46663,
#46664),(#46665,#46666,#46667,#46668,#46669,#46670,#46671,#46672,#46673,
#46674,#46675,#46676,#46677,#46678),(#46679,#46680,#46681,#46682,#46683,
#46684,#46685,#46686,#46687,#46688,#46689,#46690,#46691,#46692),(#46693,
#46694,#46695,#46696,#46697,#46698,#46699,#46700,#46701,#46702,#46703,#46704,
#46705,#46706),(#46707,#46708,#46709,#46710,#46711,#46712,#46713,#46714,
#46715,#46716,#46717,#46718,#46719,#46720),(#46721,#46722,#46723,#46724,
#46725,#46726,#46727,#46728,#46729,#46730,#46731,#46732,#46733,#46734),
(#46735,#46736,#46737,#46738,#46739,#46740,#46741,#46742,#46743,#46744,
#46745,#46746,#46747,#46748),(#46749,#46750,#46751,#46752,#46753,#46754,
#46755,#46756,#46757,#46758,#46759,#46760,#46761,#46762),(#46763,#46764,
#46765,#46766,#46767,#46768,#46769,#46770,#46771,#46772,#46773,#46774,#46775,
#46776),(#46777,#46778,#46779,#46780,#46781,#46782,#46783,#46784,#46785,
#46786,#46787,#46788,#46789,#46790),(#46791,#46792,#46793,#46794,#46795,
#46796,#46797,#46798,#46799,#46800,#46801,#46802,#46803,#46804),(#46805,
#46806,#46807,#46808,#46809,#46810,#46811,#46812,#46813,#46814,#46815,#46816,
#46817,#46818),(#46819,#46820,#46821,#46822,#46823,#46824,#46825,#46826,
#46827,#46828,#46829,#46830,#46831,#46832),(#46833,#46834,#46835,#46836,
#46837,#46838,#46839,#46840,#46841,#46842,#46843,#46844,#46845,#46846),
(#46847,#46848,#46849,#46850,#46851,#46852,#46853,#46854,#46855,#46856,
#46857,#46858,#46859,#46860),(#46861,#46862,#46863,#46864,#46865,#46866,
#46867,#46868,#46869,#46870,#46871,#46872,#46873,#46874),(#46875,#46876,
#46877,#46878,#46879,#46880,#46881,#46882,#46883,#46884,#46885,#46886,#46887,
#46888),(#46889,#46890,#46891,#46892,#46893,#46894,#46895,#46896,#46897,
#46898,#46899,#46900,#46901,#46902),(#46903,#46904,#46905,#46906,#46907,
#46908,#46909,#46910,#46911,#46912,#46913,#46914,#46915,#46916),(#46917,
#46918,#46919,#46920,#46921,#46922,#46923,#46924,#46925,#46926,#46927,#46928,
#46929,#46930),(#46931,#46932,#46933,#46934,#46935,#46936,#46937,#46938,
#46939,#46940,#46941,#46942,#46943,#46944),(#46945,#46946,#46947,#46948,
#46949,#46950,#46951,#46952,#46953,#46954,#46955,#46956,#46957,#46958),
(#46959,#46960,#46961,#46962,#46963,#46964,#46965,#46966,#46967,#46968,
#46969,#46970,#46971,#46972),(#46973,#46974,#46975,#46976,#46977,#46978,
#46979,#46980,#46981,#46982,#46983,#46984,#46985,#46986),(#46987,#46988,
#46989,#46990,#46991,#46992,#46993,#46994,#46995,#46996,#46997,#46998,#46999,
#47000)),.UNSPECIFIED.,.F.,.F.,.F.,(4,1,1,1,1,1,1,1,1,1,1,1,1,1,1,1,1,1,
1,1,1,1,1,1,1,1,1,1,4),(4,2,2,2,2,2,4),(0.0331549352864085,0.0676851161690368,
0.102215297051665,0.119480387492979,0.171275658816922,0.179908204037579,
0.188540749258236,0.197173294478893,0.20580583969955,0.240336020582178,
0.274866201464806,0.309396382347435,0.378456744112691,0.412986924995319,
0.447517105877948,0.482047286760576,0.551107648525832,0.585637829408461,
0.620168010291089,0.654698191173717,0.723758552938974,0.810084005145544,
0.827349095586859,0.844614186028173,0.861879276469487,0.896409457352115,
0.930939638234743,0.948204728676058,1.),(0.0377143719401151,0.167070624995476,
0.336553194126115,0.499999999999991,0.663446805873868,0.832929375004528,
0.962285628058773),.UNSPECIFIED.);
#210=B_SPLINE_SURFACE_WITH_KNOTS('',3,3,((#47059,#47060,#47061,#47062,#47063,
#47064,#47065,#47066,#47067,#47068,#47069,#47070,#47071,#47072),(#47073,
#47074,#47075,#47076,#47077,#47078,#47079,#47080,#47081,#47082,#47083,#47084,
#47085,#47086),(#47087,#47088,#47089,#47090,#47091,#47092,#47093,#47094,
#47095,#47096,#47097,#47098,#47099,#47100),(#47101,#47102,#47103,#47104,
#47105,#47106,#47107,#47108,#47109,#47110,#47111,#47112,#47113,#47114)),
 .UNSPECIFIED.,.F.,.F.,.F.,(4,4),(4,2,2,2,2,2,4),(0.,1.),(0.0377143719414212,
0.167070624995476,0.336553194126115,0.499999999999991,0.663446805873868,
0.832929375004528,0.962285628058582),.UNSPECIFIED.);
#211=B_SPLINE_SURFACE_WITH_KNOTS('',3,3,((#47129,#47130,#47131,#47132,#47133,
#47134,#47135,#47136,#47137,#47138,#47139,#47140,#47141,#47142),(#47143,
#47144,#47145,#47146,#47147,#47148,#47149,#47150,#47151,#47152,#47153,#47154,
#47155,#47156),(#47157,#47158,#47159,#47160,#47161,#47162,#47163,#47164,
#47165,#47166,#47167,#47168,#47169,#47170),(#47171,#47172,#47173,#47174,
#47175,#47176,#47177,#47178,#47179,#47180,#47181,#47182,#47183,#47184),
(#47185,#47186,#47187,#47188,#47189,#47190,#47191,#47192,#47193,#47194,
#47195,#47196,#47197,#47198),(#47199,#47200,#47201,#47202,#47203,#47204,
#47205,#47206,#47207,#47208,#47209,#47210,#47211,#47212),(#47213,#47214,
#47215,#47216,#47217,#47218,#47219,#47220,#47221,#47222,#47223,#47224,#47225,
#47226),(#47227,#47228,#47229,#47230,#47231,#47232,#47233,#47234,#47235,
#47236,#47237,#47238,#47239,#47240),(#47241,#47242,#47243,#47244,#47245,
#47246,#47247,#47248,#47249,#47250,#47251,#47252,#47253,#47254),(#47255,
#47256,#47257,#47258,#47259,#47260,#47261,#47262,#47263,#47264,#47265,#47266,
#47267,#47268),(#47269,#47270,#47271,#47272,#47273,#47274,#47275,#47276,
#47277,#47278,#47279,#47280,#47281,#47282),(#47283,#47284,#47285,#47286,
#47287,#47288,#47289,#47290,#47291,#47292,#47293,#47294,#47295,#47296),
(#47297,#47298,#47299,#47300,#47301,#47302,#47303,#47304,#47305,#47306,
#47307,#47308,#47309,#47310),(#47311,#47312,#47313,#47314,#47315,#47316,
#47317,#47318,#47319,#47320,#47321,#47322,#47323,#47324),(#47325,#47326,
#47327,#47328,#47329,#47330,#47331,#47332,#47333,#47334,#47335,#47336,#47337,
#47338),(#47339,#47340,#47341,#47342,#47343,#47344,#47345,#47346,#47347,
#47348,#47349,#47350,#47351,#47352),(#47353,#47354,#47355,#47356,#47357,
#47358,#47359,#47360,#47361,#47362,#47363,#47364,#47365,#47366),(#47367,
#47368,#47369,#47370,#47371,#47372,#47373,#47374,#47375,#47376,#47377,#47378,
#47379,#47380),(#47381,#47382,#47383,#47384,#47385,#47386,#47387,#47388,
#47389,#47390,#47391,#47392,#47393,#47394),(#47395,#47396,#47397,#47398,
#47399,#47400,#47401,#47402,#47403,#47404,#47405,#47406,#47407,#47408),
(#47409,#47410,#47411,#47412,#47413,#47414,#47415,#47416,#47417,#47418,
#47419,#47420,#47421,#47422),(#47423,#47424,#47425,#47426,#47427,#47428,
#47429,#47430,#47431,#47432,#47433,#47434,#47435,#47436),(#47437,#47438,
#47439,#47440,#47441,#47442,#47443,#47444,#47445,#47446,#47447,#47448,#47449,
#47450),(#47451,#47452,#47453,#47454,#47455,#47456,#47457,#47458,#47459,
#47460,#47461,#47462,#47463,#47464),(#47465,#47466,#47467,#47468,#47469,
#47470,#47471,#47472,#47473,#47474,#47475,#47476,#47477,#47478),(#47479,
#47480,#47481,#47482,#47483,#47484,#47485,#47486,#47487,#47488,#47489,#47490,
#47491,#47492),(#47493,#47494,#47495,#47496,#47497,#47498,#47499,#47500,
#47501,#47502,#47503,#47504,#47505,#47506),(#47507,#47508,#47509,#47510,
#47511,#47512,#47513,#47514,#47515,#47516,#47517,#47518,#47519,#47520),
(#47521,#47522,#47523,#47524,#47525,#47526,#47527,#47528,#47529,#47530,
#47531,#47532,#47533,#47534)),.UNSPECIFIED.,.F.,.F.,.F.,(4,1,1,1,1,1,1,
1,1,1,1,1,1,1,1,1,1,1,1,1,1,1,1,1,1,1,4),(4,2,2,2,2,2,4),(0.,0.0517952713240544,
0.0690603617654059,0.103590542648109,0.138120723530812,0.172650904413515,
0.276241447061623,0.310771627944326,0.345301808827029,0.414362170592435,
0.483422532357841,0.552482894123247,0.569747984564598,0.58701307500595,
0.621543255888653,0.690603617654059,0.725133798536761,0.759663979419464,
0.776929069860816,0.794194160302167,0.811459250743519,0.820091795964194,
0.824408068574532,0.82872434118487,0.897784702950276,0.932314883832979,
0.966845064715682),(0.0377143719394609,0.167070624995476,0.336553194126115,
0.499999999999991,0.663446805873868,0.832929375004528,0.962285628058648),
 .UNSPECIFIED.);
#212=B_SPLINE_SURFACE_WITH_KNOTS('',3,3,((#47592,#47593,#47594,#47595,#47596,
#47597,#47598,#47599,#47600,#47601,#47602,#47603,#47604,#47605),(#47606,
#47607,#47608,#47609,#47610,#47611,#47612,#47613,#47614,#47615,#47616,#47617,
#47618,#47619),(#47620,#47621,#47622,#47623,#47624,#47625,#47626,#47627,
#47628,#47629,#47630,#47631,#47632,#47633),(#47634,#47635,#47636,#47637,
#47638,#47639,#47640,#47641,#47642,#47643,#47644,#47645,#47646,#47647),
(#47648,#47649,#47650,#47651,#47652,#47653,#47654,#47655,#47656,#47657,
#47658,#47659,#47660,#47661),(#47662,#47663,#47664,#47665,#47666,#47667,
#47668,#47669,#47670,#47671,#47672,#47673,#47674,#47675),(#47676,#47677,
#47678,#47679,#47680,#47681,#47682,#47683,#47684,#47685,#47686,#47687,#47688,
#47689),(#47690,#47691,#47692,#47693,#47694,#47695,#47696,#47697,#47698,
#47699,#47700,#47701,#47702,#47703),(#47704,#47705,#47706,#47707,#47708,
#47709,#47710,#47711,#47712,#47713,#47714,#47715,#47716,#47717),(#47718,
#47719,#47720,#47721,#47722,#47723,#47724,#47725,#47726,#47727,#47728,#47729,
#47730,#47731),(#47732,#47733,#47734,#47735,#47736,#47737,#47738,#47739,
#47740,#47741,#47742,#47743,#47744,#47745),(#47746,#47747,#47748,#47749,
#47750,#47751,#47752,#47753,#47754,#47755,#47756,#47757,#47758,#47759),
(#47760,#47761,#47762,#47763,#47764,#47765,#47766,#47767,#47768,#47769,
#47770,#47771,#47772,#47773),(#47774,#47775,#47776,#47777,#47778,#47779,
#47780,#47781,#47782,#47783,#47784,#47785,#47786,#47787),(#47788,#47789,
#47790,#47791,#47792,#47793,#47794,#47795,#47796,#47797,#47798,#47799,#47800,
#47801),(#47802,#47803,#47804,#47805,#47806,#47807,#47808,#47809,#47810,
#47811,#47812,#47813,#47814,#47815),(#47816,#47817,#47818,#47819,#47820,
#47821,#47822,#47823,#47824,#47825,#47826,#47827,#47828,#47829),(#47830,
#47831,#47832,#47833,#47834,#47835,#47836,#47837,#47838,#47839,#47840,#47841,
#47842,#47843),(#47844,#47845,#47846,#47847,#47848,#47849,#47850,#47851,
#47852,#47853,#47854,#47855,#47856,#47857),(#47858,#47859,#47860,#47861,
#47862,#47863,#47864,#47865,#47866,#47867,#47868,#47869,#47870,#47871),
(#47872,#47873,#47874,#47875,#47876,#47877,#47878,#47879,#47880,#47881,
#47882,#47883,#47884,#47885)),.UNSPECIFIED.,.F.,.F.,.F.,(4,1,1,1,1,1,1,
1,1,1,1,1,1,1,1,1,1,1,4),(4,2,2,2,2,2,4),(0.0331549352864064,0.102215297051663,
0.136745477934291,0.240336020582176,0.309396382347433,0.37845674411269,
0.447517105877946,0.551107648525831,0.58563782940846,0.620168010291088,
0.706493462497659,0.723758552938973,0.758288733821602,0.827349095586858,
0.861879276469487,0.896409457352115,0.930939638234743,0.948204728676057,
1.),(0.0377143719408274,0.167070624995476,0.336553194126115,0.499999999999991,
0.663446805873868,0.832929375004528,0.962285628058718),.UNSPECIFIED.);
#213=B_SPLINE_SURFACE_WITH_KNOTS('',3,3,((#47942,#47943,#47944,#47945,#47946,
#47947,#47948,#47949,#47950,#47951,#47952,#47953,#47954,#47955),(#47956,
#47957,#47958,#47959,#47960,#47961,#47962,#47963,#47964,#47965,#47966,#47967,
#47968,#47969),(#47970,#47971,#47972,#47973,#47974,#47975,#47976,#47977,
#47978,#47979,#47980,#47981,#47982,#47983),(#47984,#47985,#47986,#47987,
#47988,#47989,#47990,#47991,#47992,#47993,#47994,#47995,#47996,#47997)),
 .UNSPECIFIED.,.F.,.F.,.F.,(4,4),(4,2,2,2,2,2,4),(0.,1.),(0.0377143719414211,
0.167070624995476,0.336553194126115,0.499999999999991,0.663446805873868,
0.832929375004528,0.962285628058582),.UNSPECIFIED.);
#214=B_SPLINE_SURFACE_WITH_KNOTS('',3,3,((#48012,#48013,#48014,#48015,#48016,
#48017,#48018,#48019,#48020,#48021,#48022,#48023,#48024,#48025),(#48026,
#48027,#48028,#48029,#48030,#48031,#48032,#48033,#48034,#48035,#48036,#48037,
#48038,#48039),(#48040,#48041,#48042,#48043,#48044,#48045,#48046,#48047,
#48048,#48049,#48050,#48051,#48052,#48053),(#48054,#48055,#48056,#48057,
#48058,#48059,#48060,#48061,#48062,#48063,#48064,#48065,#48066,#48067),
(#48068,#48069,#48070,#48071,#48072,#48073,#48074,#48075,#48076,#48077,
#48078,#48079,#48080,#48081),(#48082,#48083,#48084,#48085,#48086,#48087,
#48088,#48089,#48090,#48091,#48092,#48093,#48094,#48095),(#48096,#48097,
#48098,#48099,#48100,#48101,#48102,#48103,#48104,#48105,#48106,#48107,#48108,
#48109),(#48110,#48111,#48112,#48113,#48114,#48115,#48116,#48117,#48118,
#48119,#48120,#48121,#48122,#48123),(#48124,#48125,#48126,#48127,#48128,
#48129,#48130,#48131,#48132,#48133,#48134,#48135,#48136,#48137),(#48138,
#48139,#48140,#48141,#48142,#48143,#48144,#48145,#48146,#48147,#48148,#48149,
#48150,#48151),(#48152,#48153,#48154,#48155,#48156,#48157,#48158,#48159,
#48160,#48161,#48162,#48163,#48164,#48165),(#48166,#48167,#48168,#48169,
#48170,#48171,#48172,#48173,#48174,#48175,#48176,#48177,#48178,#48179),
(#48180,#48181,#48182,#48183,#48184,#48185,#48186,#48187,#48188,#48189,
#48190,#48191,#48192,#48193),(#48194,#48195,#48196,#48197,#48198,#48199,
#48200,#48201,#48202,#48203,#48204,#48205,#48206,#48207),(#48208,#48209,
#48210,#48211,#48212,#48213,#48214,#48215,#48216,#48217,#48218,#48219,#48220,
#48221),(#48222,#48223,#48224,#48225,#48226,#48227,#48228,#48229,#48230,
#48231,#48232,#48233,#48234,#48235),(#48236,#48237,#48238,#48239,#48240,
#48241,#48242,#48243,#48244,#48245,#48246,#48247,#48248,#48249),(#48250,
#48251,#48252,#48253,#48254,#48255,#48256,#48257,#48258,#48259,#48260,#48261,
#48262,#48263),(#48264,#48265,#48266,#48267,#48268,#48269,#48270,#48271,
#48272,#48273,#48274,#48275,#48276,#48277),(#48278,#48279,#48280,#48281,
#48282,#48283,#48284,#48285,#48286,#48287,#48288,#48289,#48290,#48291),
(#48292,#48293,#48294,#48295,#48296,#48297,#48298,#48299,#48300,#48301,
#48302,#48303,#48304,#48305),(#48306,#48307,#48308,#48309,#48310,#48311,
#48312,#48313,#48314,#48315,#48316,#48317,#48318,#48319),(#48320,#48321,
#48322,#48323,#48324,#48325,#48326,#48327,#48328,#48329,#48330,#48331,#48332,
#48333),(#48334,#48335,#48336,#48337,#48338,#48339,#48340,#48341,#48342,
#48343,#48344,#48345,#48346,#48347),(#48348,#48349,#48350,#48351,#48352,
#48353,#48354,#48355,#48356,#48357,#48358,#48359,#48360,#48361),(#48362,
#48363,#48364,#48365,#48366,#48367,#48368,#48369,#48370,#48371,#48372,#48373,
#48374,#48375),(#48376,#48377,#48378,#48379,#48380,#48381,#48382,#48383,
#48384,#48385,#48386,#48387,#48388,#48389),(#48390,#48391,#48392,#48393,
#48394,#48395,#48396,#48397,#48398,#48399,#48400,#48401,#48402,#48403),
(#48404,#48405,#48406,#48407,#48408,#48409,#48410,#48411,#48412,#48413,
#48414,#48415,#48416,#48417),(#48418,#48419,#48420,#48421,#48422,#48423,
#48424,#48425,#48426,#48427,#48428,#48429,#48430,#48431),(#48432,#48433,
#48434,#48435,#48436,#48437,#48438,#48439,#48440,#48441,#48442,#48443,#48444,
#48445),(#48446,#48447,#48448,#48449,#48450,#48451,#48452,#48453,#48454,
#48455,#48456,#48457,#48458,#48459),(#48460,#48461,#48462,#48463,#48464,
#48465,#48466,#48467,#48468,#48469,#48470,#48471,#48472,#48473)),
 .UNSPECIFIED.,.F.,.F.,.F.,(4,1,1,1,1,1,1,1,1,1,1,1,1,1,1,1,1,1,1,1,1,1,
1,1,1,1,1,1,1,1,4),(4,2,2,2,2,2,4),(0.,0.0517952713240545,0.069060361765406,
0.103590542648109,0.138120723530812,0.172650904413515,0.207181085296218,
0.276241447061624,0.34530180882703,0.414362170592436,0.448892351475139,
0.517952713240545,0.552482894123248,0.587013075005951,0.621543255888654,
0.647440891550682,0.69060361765406,0.725133798536763,0.759663979419467,
0.776929069860818,0.79419416030217,0.811459250743521,0.815775523353859,
0.820091795964197,0.824408068574535,0.826566204879704,0.827645273032288,
0.828724341184873,0.897784702950279,0.932314883832982,0.966845064715685),
(0.0377143719414145,0.167070624995476,0.336553194126115,0.499999999999991,
0.663446805873868,0.832929375004528,0.962285628059096),.UNSPECIFIED.);
#215=B_SPLINE_SURFACE_WITH_KNOTS('',3,3,((#48533,#48534,#48535,#48536,#48537,
#48538,#48539,#48540,#48541,#48542,#48543,#48544,#48545,#48546),(#48547,
#48548,#48549,#48550,#48551,#48552,#48553,#48554,#48555,#48556,#48557,#48558,
#48559,#48560),(#48561,#48562,#48563,#48564,#48565,#48566,#48567,#48568,
#48569,#48570,#48571,#48572,#48573,#48574),(#48575,#48576,#48577,#48578,
#48579,#48580,#48581,#48582,#48583,#48584,#48585,#48586,#48587,#48588),
(#48589,#48590,#48591,#48592,#48593,#48594,#48595,#48596,#48597,#48598,
#48599,#48600,#48601,#48602),(#48603,#48604,#48605,#48606,#48607,#48608,
#48609,#48610,#48611,#48612,#48613,#48614,#48615,#48616),(#48617,#48618,
#48619,#48620,#48621,#48622,#48623,#48624,#48625,#48626,#48627,#48628,#48629,
#48630),(#48631,#48632,#48633,#48634,#48635,#48636,#48637,#48638,#48639,
#48640,#48641,#48642,#48643,#48644),(#48645,#48646,#48647,#48648,#48649,
#48650,#48651,#48652,#48653,#48654,#48655,#48656,#48657,#48658),(#48659,
#48660,#48661,#48662,#48663,#48664,#48665,#48666,#48667,#48668,#48669,#48670,
#48671,#48672),(#48673,#48674,#48675,#48676,#48677,#48678,#48679,#48680,
#48681,#48682,#48683,#48684,#48685,#48686),(#48687,#48688,#48689,#48690,
#48691,#48692,#48693,#48694,#48695,#48696,#48697,#48698,#48699,#48700),
(#48701,#48702,#48703,#48704,#48705,#48706,#48707,#48708,#48709,#48710,
#48711,#48712,#48713,#48714),(#48715,#48716,#48717,#48718,#48719,#48720,
#48721,#48722,#48723,#48724,#48725,#48726,#48727,#48728),(#48729,#48730,
#48731,#48732,#48733,#48734,#48735,#48736,#48737,#48738,#48739,#48740,#48741,
#48742),(#48743,#48744,#48745,#48746,#48747,#48748,#48749,#48750,#48751,
#48752,#48753,#48754,#48755,#48756),(#48757,#48758,#48759,#48760,#48761,
#48762,#48763,#48764,#48765,#48766,#48767,#48768,#48769,#48770),(#48771,
#48772,#48773,#48774,#48775,#48776,#48777,#48778,#48779,#48780,#48781,#48782,
#48783,#48784),(#48785,#48786,#48787,#48788,#48789,#48790,#48791,#48792,
#48793,#48794,#48795,#48796,#48797,#48798),(#48799,#48800,#48801,#48802,
#48803,#48804,#48805,#48806,#48807,#48808,#48809,#48810,#48811,#48812),
(#48813,#48814,#48815,#48816,#48817,#48818,#48819,#48820,#48821,#48822,
#48823,#48824,#48825,#48826),(#48827,#48828,#48829,#48830,#48831,#48832,
#48833,#48834,#48835,#48836,#48837,#48838,#48839,#48840),(#48841,#48842,
#48843,#48844,#48845,#48846,#48847,#48848,#48849,#48850,#48851,#48852,#48853,
#48854),(#48855,#48856,#48857,#48858,#48859,#48860,#48861,#48862,#48863,
#48864,#48865,#48866,#48867,#48868),(#48869,#48870,#48871,#48872,#48873,
#48874,#48875,#48876,#48877,#48878,#48879,#48880,#48881,#48882),(#48883,
#48884,#48885,#48886,#48887,#48888,#48889,#48890,#48891,#48892,#48893,#48894,
#48895,#48896),(#48897,#48898,#48899,#48900,#48901,#48902,#48903,#48904,
#48905,#48906,#48907,#48908,#48909,#48910),(#48911,#48912,#48913,#48914,
#48915,#48916,#48917,#48918,#48919,#48920,#48921,#48922,#48923,#48924),
(#48925,#48926,#48927,#48928,#48929,#48930,#48931,#48932,#48933,#48934,
#48935,#48936,#48937,#48938),(#48939,#48940,#48941,#48942,#48943,#48944,
#48945,#48946,#48947,#48948,#48949,#48950,#48951,#48952)),.UNSPECIFIED.,
 .F.,.F.,.F.,(4,1,1,1,1,1,1,1,1,1,1,1,1,1,1,1,1,1,1,1,1,1,1,1,1,1,1,4),
(4,2,2,2,2,2,4),(0.0331549352864089,0.102215297051665,0.171275658816922,
0.173433795122086,0.17559193142725,0.179908204037579,0.188540749258236,
0.20580583969955,0.223070930140864,0.240336020582178,0.274866201464807,
0.309396382347435,0.378456744112691,0.41298692499532,0.447517105877948,
0.482047286760576,0.516577467643204,0.551107648525833,0.568372738967147,
0.585637829408461,0.689228372056346,0.723758552938974,0.810084005145545,
0.861879276469487,0.896409457352115,0.930939638234743,0.948204728676058,
1.),(0.0377143719403939,0.167070624995476,0.336553194126115,0.499999999999991,
0.663446805873868,0.832929375004528,0.962285628059341),.UNSPECIFIED.);
#216=B_SPLINE_SURFACE_WITH_KNOTS('',3,3,((#49013,#49014,#49015,#49016,#49017,
#49018,#49019,#49020,#49021,#49022,#49023,#49024,#49025,#49026),(#49027,
#49028,#49029,#49030,#49031,#49032,#49033,#49034,#49035,#49036,#49037,#49038,
#49039,#49040),(#49041,#49042,#49043,#49044,#49045,#49046,#49047,#49048,
#49049,#49050,#49051,#49052,#49053,#49054),(#49055,#49056,#49057,#49058,
#49059,#49060,#49061,#49062,#49063,#49064,#49065,#49066,#49067,#49068)),
 .UNSPECIFIED.,.F.,.F.,.F.,(4,4),(4,2,2,2,2,2,4),(0.,1.),(0.0377143719414212,
0.167070624995476,0.336553194126115,0.499999999999991,0.663446805873868,
0.832929375004528,0.962285628058582),.UNSPECIFIED.);
#217=B_SPLINE_SURFACE_WITH_KNOTS('',3,3,((#49083,#49084,#49085,#49086,#49087,
#49088,#49089,#49090,#49091,#49092,#49093,#49094,#49095,#49096),(#49097,
#49098,#49099,#49100,#49101,#49102,#49103,#49104,#49105,#49106,#49107,#49108,
#49109,#49110),(#49111,#49112,#49113,#49114,#49115,#49116,#49117,#49118,
#49119,#49120,#49121,#49122,#49123,#49124),(#49125,#49126,#49127,#49128,
#49129,#49130,#49131,#49132,#49133,#49134,#49135,#49136,#49137,#49138),
(#49139,#49140,#49141,#49142,#49143,#49144,#49145,#49146,#49147,#49148,
#49149,#49150,#49151,#49152),(#49153,#49154,#49155,#49156,#49157,#49158,
#49159,#49160,#49161,#49162,#49163,#49164,#49165,#49166),(#49167,#49168,
#49169,#49170,#49171,#49172,#49173,#49174,#49175,#49176,#49177,#49178,#49179,
#49180),(#49181,#49182,#49183,#49184,#49185,#49186,#49187,#49188,#49189,
#49190,#49191,#49192,#49193,#49194),(#49195,#49196,#49197,#49198,#49199,
#49200,#49201,#49202,#49203,#49204,#49205,#49206,#49207,#49208),(#49209,
#49210,#49211,#49212,#49213,#49214,#49215,#49216,#49217,#49218,#49219,#49220,
#49221,#49222),(#49223,#49224,#49225,#49226,#49227,#49228,#49229,#49230,
#49231,#49232,#49233,#49234,#49235,#49236),(#49237,#49238,#49239,#49240,
#49241,#49242,#49243,#49244,#49245,#49246,#49247,#49248,#49249,#49250),
(#49251,#49252,#49253,#49254,#49255,#49256,#49257,#49258,#49259,#49260,
#49261,#49262,#49263,#49264),(#49265,#49266,#49267,#49268,#49269,#49270,
#49271,#49272,#49273,#49274,#49275,#49276,#49277,#49278),(#49279,#49280,
#49281,#49282,#49283,#49284,#49285,#49286,#49287,#49288,#49289,#49290,#49291,
#49292),(#49293,#49294,#49295,#49296,#49297,#49298,#49299,#49300,#49301,
#49302,#49303,#49304,#49305,#49306),(#49307,#49308,#49309,#49310,#49311,
#49312,#49313,#49314,#49315,#49316,#49317,#49318,#49319,#49320),(#49321,
#49322,#49323,#49324,#49325,#49326,#49327,#49328,#49329,#49330,#49331,#49332,
#49333,#49334),(#49335,#49336,#49337,#49338,#49339,#49340,#49341,#49342,
#49343,#49344,#49345,#49346,#49347,#49348),(#49349,#49350,#49351,#49352,
#49353,#49354,#49355,#49356,#49357,#49358,#49359,#49360,#49361,#49362),
(#49363,#49364,#49365,#49366,#49367,#49368,#49369,#49370,#49371,#49372,
#49373,#49374,#49375,#49376),(#49377,#49378,#49379,#49380,#49381,#49382,
#49383,#49384,#49385,#49386,#49387,#49388,#49389,#49390),(#49391,#49392,
#49393,#49394,#49395,#49396,#49397,#49398,#49399,#49400,#49401,#49402,#49403,
#49404),(#49405,#49406,#49407,#49408,#49409,#49410,#49411,#49412,#49413,
#49414,#49415,#49416,#49417,#49418),(#49419,#49420,#49421,#49422,#49423,
#49424,#49425,#49426,#49427,#49428,#49429,#49430,#49431,#49432),(#49433,
#49434,#49435,#49436,#49437,#49438,#49439,#49440,#49441,#49442,#49443,#49444,
#49445,#49446),(#49447,#49448,#49449,#49450,#49451,#49452,#49453,#49454,
#49455,#49456,#49457,#49458,#49459,#49460),(#49461,#49462,#49463,#49464,
#49465,#49466,#49467,#49468,#49469,#49470,#49471,#49472,#49473,#49474),
(#49475,#49476,#49477,#49478,#49479,#49480,#49481,#49482,#49483,#49484,
#49485,#49486,#49487,#49488),(#49489,#49490,#49491,#49492,#49493,#49494,
#49495,#49496,#49497,#49498,#49499,#49500,#49501,#49502),(#49503,#49504,
#49505,#49506,#49507,#49508,#49509,#49510,#49511,#49512,#49513,#49514,#49515,
#49516),(#49517,#49518,#49519,#49520,#49521,#49522,#49523,#49524,#49525,
#49526,#49527,#49528,#49529,#49530)),.UNSPECIFIED.,.F.,.F.,.F.,(4,1,1,1,
1,1,1,1,1,1,1,1,1,1,1,1,1,1,1,1,1,1,1,1,1,1,1,1,1,4),(4,2,2,2,2,2,4),(0.,
0.0517952713240545,0.069060361765406,0.103590542648109,0.138120723530812,
0.172650904413515,0.207181085296218,0.276241447061624,0.34530180882703,
0.414362170592436,0.483422532357842,0.552482894123248,0.561115439343924,
0.5697479845646,0.587013075005951,0.621543255888654,0.69060361765406,0.725133798536763,
0.759663979419466,0.776929069860818,0.794194160302169,0.811459250743521,
0.815775523353859,0.820091795964197,0.824408068574535,0.826566204879703,
0.827645273032288,0.828724341184872,0.897784702950278,0.966845064715684),
(0.037714371939343,0.167070624995476,0.336553194126115,0.499999999999991,
0.663446805873868,0.832929375004528,0.962285628058644),.UNSPECIFIED.);
#218=B_SPLINE_SURFACE_WITH_KNOTS('',3,3,((#49586,#49587,#49588,#49589,#49590,
#49591,#49592,#49593,#49594,#49595,#49596,#49597,#49598,#49599),(#49600,
#49601,#49602,#49603,#49604,#49605,#49606,#49607,#49608,#49609,#49610,#49611,
#49612,#49613),(#49614,#49615,#49616,#49617,#49618,#49619,#49620,#49621,
#49622,#49623,#49624,#49625,#49626,#49627),(#49628,#49629,#49630,#49631,
#49632,#49633,#49634,#49635,#49636,#49637,#49638,#49639,#49640,#49641),
(#49642,#49643,#49644,#49645,#49646,#49647,#49648,#49649,#49650,#49651,
#49652,#49653,#49654,#49655),(#49656,#49657,#49658,#49659,#49660,#49661,
#49662,#49663,#49664,#49665,#49666,#49667,#49668,#49669),(#49670,#49671,
#49672,#49673,#49674,#49675,#49676,#49677,#49678,#49679,#49680,#49681,#49682,
#49683),(#49684,#49685,#49686,#49687,#49688,#49689,#49690,#49691,#49692,
#49693,#49694,#49695,#49696,#49697),(#49698,#49699,#49700,#49701,#49702,
#49703,#49704,#49705,#49706,#49707,#49708,#49709,#49710,#49711),(#49712,
#49713,#49714,#49715,#49716,#49717,#49718,#49719,#49720,#49721,#49722,#49723,
#49724,#49725),(#49726,#49727,#49728,#49729,#49730,#49731,#49732,#49733,
#49734,#49735,#49736,#49737,#49738,#49739),(#49740,#49741,#49742,#49743,
#49744,#49745,#49746,#49747,#49748,#49749,#49750,#49751,#49752,#49753),
(#49754,#49755,#49756,#49757,#49758,#49759,#49760,#49761,#49762,#49763,
#49764,#49765,#49766,#49767),(#49768,#49769,#49770,#49771,#49772,#49773,
#49774,#49775,#49776,#49777,#49778,#49779,#49780,#49781),(#49782,#49783,
#49784,#49785,#49786,#49787,#49788,#49789,#49790,#49791,#49792,#49793,#49794,
#49795),(#49796,#49797,#49798,#49799,#49800,#49801,#49802,#49803,#49804,
#49805,#49806,#49807,#49808,#49809),(#49810,#49811,#49812,#49813,#49814,
#49815,#49816,#49817,#49818,#49819,#49820,#49821,#49822,#49823),(#49824,
#49825,#49826,#49827,#49828,#49829,#49830,#49831,#49832,#49833,#49834,#49835,
#49836,#49837),(#49838,#49839,#49840,#49841,#49842,#49843,#49844,#49845,
#49846,#49847,#49848,#49849,#49850,#49851),(#49852,#49853,#49854,#49855,
#49856,#49857,#49858,#49859,#49860,#49861,#49862,#49863,#49864,#49865),
(#49866,#49867,#49868,#49869,#49870,#49871,#49872,#49873,#49874,#49875,
#49876,#49877,#49878,#49879),(#49880,#49881,#49882,#49883,#49884,#49885,
#49886,#49887,#49888,#49889,#49890,#49891,#49892,#49893),(#49894,#49895,
#49896,#49897,#49898,#49899,#49900,#49901,#49902,#49903,#49904,#49905,#49906,
#49907),(#49908,#49909,#49910,#49911,#49912,#49913,#49914,#49915,#49916,
#49917,#49918,#49919,#49920,#49921),(#49922,#49923,#49924,#49925,#49926,
#49927,#49928,#49929,#49930,#49931,#49932,#49933,#49934,#49935),(#49936,
#49937,#49938,#49939,#49940,#49941,#49942,#49943,#49944,#49945,#49946,#49947,
#49948,#49949),(#49950,#49951,#49952,#49953,#49954,#49955,#49956,#49957,
#49958,#49959,#49960,#49961,#49962,#49963),(#49964,#49965,#49966,#49967,
#49968,#49969,#49970,#49971,#49972,#49973,#49974,#49975,#49976,#49977),
(#49978,#49979,#49980,#49981,#49982,#49983,#49984,#49985,#49986,#49987,
#49988,#49989,#49990,#49991),(#49992,#49993,#49994,#49995,#49996,#49997,
#49998,#49999,#50000,#50001,#50002,#50003,#50004,#50005)),.UNSPECIFIED.,
 .F.,.F.,.F.,(4,1,1,1,1,1,1,1,1,1,1,1,1,1,1,1,1,1,1,1,1,1,1,1,1,1,1,4),
(4,2,2,2,2,2,4),(0.0331549352864079,0.102215297051665,0.171275658816921,
0.173433795122085,0.17559193142725,0.179908204037578,0.188540749258235,
0.205805839699549,0.240336020582178,0.309396382347434,0.378456744112691,
0.412986924995319,0.430252015436633,0.43888456065729,0.443200833267619,
0.447517105877947,0.516577467643204,0.585637829408461,0.620168010291089,
0.723758552938974,0.79281891470423,0.827349095586858,0.861879276469487,
0.896409457352115,0.913674547793429,0.930939638234743,0.948204728676058,
1.00005376760518),(0.0377143719409181,0.167070624995476,0.336553194126115,
0.499999999999991,0.663446805873868,0.832929375004528,0.962339395663765),
 .UNSPECIFIED.);
#219=B_SPLINE_SURFACE_WITH_KNOTS('',3,3,((#50068,#50069,#50070,#50071,#50072,
#50073,#50074,#50075,#50076,#50077,#50078,#50079,#50080,#50081),(#50082,
#50083,#50084,#50085,#50086,#50087,#50088,#50089,#50090,#50091,#50092,#50093,
#50094,#50095),(#50096,#50097,#50098,#50099,#50100,#50101,#50102,#50103,
#50104,#50105,#50106,#50107,#50108,#50109),(#50110,#50111,#50112,#50113,
#50114,#50115,#50116,#50117,#50118,#50119,#50120,#50121,#50122,#50123)),
 .UNSPECIFIED.,.F.,.F.,.F.,(4,4),(4,2,2,2,2,2,4),(0.,1.),(0.0377143719414212,
0.167070624995476,0.336553194126115,0.499999999999991,0.663446805873868,
0.832929375004528,0.962285628058582),.UNSPECIFIED.);
#220=B_SPLINE_SURFACE_WITH_KNOTS('',3,3,((#50138,#50139,#50140,#50141,#50142,
#50143,#50144,#50145,#50146,#50147,#50148,#50149,#50150,#50151),(#50152,
#50153,#50154,#50155,#50156,#50157,#50158,#50159,#50160,#50161,#50162,#50163,
#50164,#50165),(#50166,#50167,#50168,#50169,#50170,#50171,#50172,#50173,
#50174,#50175,#50176,#50177,#50178,#50179),(#50180,#50181,#50182,#50183,
#50184,#50185,#50186,#50187,#50188,#50189,#50190,#50191,#50192,#50193),
(#50194,#50195,#50196,#50197,#50198,#50199,#50200,#50201,#50202,#50203,
#50204,#50205,#50206,#50207),(#50208,#50209,#50210,#50211,#50212,#50213,
#50214,#50215,#50216,#50217,#50218,#50219,#50220,#50221),(#50222,#50223,
#50224,#50225,#50226,#50227,#50228,#50229,#50230,#50231,#50232,#50233,#50234,
#50235),(#50236,#50237,#50238,#50239,#50240,#50241,#50242,#50243,#50244,
#50245,#50246,#50247,#50248,#50249),(#50250,#50251,#50252,#50253,#50254,
#50255,#50256,#50257,#50258,#50259,#50260,#50261,#50262,#50263),(#50264,
#50265,#50266,#50267,#50268,#50269,#50270,#50271,#50272,#50273,#50274,#50275,
#50276,#50277),(#50278,#50279,#50280,#50281,#50282,#50283,#50284,#50285,
#50286,#50287,#50288,#50289,#50290,#50291),(#50292,#50293,#50294,#50295,
#50296,#50297,#50298,#50299,#50300,#50301,#50302,#50303,#50304,#50305),
(#50306,#50307,#50308,#50309,#50310,#50311,#50312,#50313,#50314,#50315,
#50316,#50317,#50318,#50319),(#50320,#50321,#50322,#50323,#50324,#50325,
#50326,#50327,#50328,#50329,#50330,#50331,#50332,#50333),(#50334,#50335,
#50336,#50337,#50338,#50339,#50340,#50341,#50342,#50343,#50344,#50345,#50346,
#50347),(#50348,#50349,#50350,#50351,#50352,#50353,#50354,#50355,#50356,
#50357,#50358,#50359,#50360,#50361),(#50362,#50363,#50364,#50365,#50366,
#50367,#50368,#50369,#50370,#50371,#50372,#50373,#50374,#50375),(#50376,
#50377,#50378,#50379,#50380,#50381,#50382,#50383,#50384,#50385,#50386,#50387,
#50388,#50389),(#50390,#50391,#50392,#50393,#50394,#50395,#50396,#50397,
#50398,#50399,#50400,#50401,#50402,#50403),(#50404,#50405,#50406,#50407,
#50408,#50409,#50410,#50411,#50412,#50413,#50414,#50415,#50416,#50417),
(#50418,#50419,#50420,#50421,#50422,#50423,#50424,#50425,#50426,#50427,
#50428,#50429,#50430,#50431),(#50432,#50433,#50434,#50435,#50436,#50437,
#50438,#50439,#50440,#50441,#50442,#50443,#50444,#50445),(#50446,#50447,
#50448,#50449,#50450,#50451,#50452,#50453,#50454,#50455,#50456,#50457,#50458,
#50459),(#50460,#50461,#50462,#50463,#50464,#50465,#50466,#50467,#50468,
#50469,#50470,#50471,#50472,#50473),(#50474,#50475,#50476,#50477,#50478,
#50479,#50480,#50481,#50482,#50483,#50484,#50485,#50486,#50487),(#50488,
#50489,#50490,#50491,#50492,#50493,#50494,#50495,#50496,#50497,#50498,#50499,
#50500,#50501)),.UNSPECIFIED.,.F.,.F.,.F.,(4,1,1,1,1,1,1,1,1,1,1,1,1,1,
1,1,1,1,1,1,1,1,1,4),(4,2,2,2,2,2,4),(0.,0.0517952713240544,0.0690603617654059,
0.103590542648109,0.138120723530812,0.189915994854866,0.276241447061624,
0.310771627944327,0.414362170592435,0.431627261033787,0.483422532357841,
0.552482894123247,0.621543255888653,0.690603617654059,0.759663979419465,
0.776929069860816,0.794194160302168,0.811459250743519,0.820091795964195,
0.824408068574533,0.826566204879702,0.828724341184871,0.897784702950277,
0.966845064715683),(0.0377143719411898,0.167070624995476,0.336553194126115,
0.499999999999991,0.663446805873868,0.832929375004528,0.962285628059115),
 .UNSPECIFIED.);
#221=B_SPLINE_SURFACE_WITH_KNOTS('',3,3,((#50553,#50554,#50555,#50556,#50557,
#50558,#50559,#50560,#50561,#50562,#50563,#50564,#50565,#50566),(#50567,
#50568,#50569,#50570,#50571,#50572,#50573,#50574,#50575,#50576,#50577,#50578,
#50579,#50580),(#50581,#50582,#50583,#50584,#50585,#50586,#50587,#50588,
#50589,#50590,#50591,#50592,#50593,#50594),(#50595,#50596,#50597,#50598,
#50599,#50600,#50601,#50602,#50603,#50604,#50605,#50606,#50607,#50608),
(#50609,#50610,#50611,#50612,#50613,#50614,#50615,#50616,#50617,#50618,
#50619,#50620,#50621,#50622),(#50623,#50624,#50625,#50626,#50627,#50628,
#50629,#50630,#50631,#50632,#50633,#50634,#50635,#50636),(#50637,#50638,
#50639,#50640,#50641,#50642,#50643,#50644,#50645,#50646,#50647,#50648,#50649,
#50650),(#50651,#50652,#50653,#50654,#50655,#50656,#50657,#50658,#50659,
#50660,#50661,#50662,#50663,#50664),(#50665,#50666,#50667,#50668,#50669,
#50670,#50671,#50672,#50673,#50674,#50675,#50676,#50677,#50678),(#50679,
#50680,#50681,#50682,#50683,#50684,#50685,#50686,#50687,#50688,#50689,#50690,
#50691,#50692),(#50693,#50694,#50695,#50696,#50697,#50698,#50699,#50700,
#50701,#50702,#50703,#50704,#50705,#50706),(#50707,#50708,#50709,#50710,
#50711,#50712,#50713,#50714,#50715,#50716,#50717,#50718,#50719,#50720),
(#50721,#50722,#50723,#50724,#50725,#50726,#50727,#50728,#50729,#50730,
#50731,#50732,#50733,#50734),(#50735,#50736,#50737,#50738,#50739,#50740,
#50741,#50742,#50743,#50744,#50745,#50746,#50747,#50748),(#50749,#50750,
#50751,#50752,#50753,#50754,#50755,#50756,#50757,#50758,#50759,#50760,#50761,
#50762),(#50763,#50764,#50765,#50766,#50767,#50768,#50769,#50770,#50771,
#50772,#50773,#50774,#50775,#50776),(#50777,#50778,#50779,#50780,#50781,
#50782,#50783,#50784,#50785,#50786,#50787,#50788,#50789,#50790),(#50791,
#50792,#50793,#50794,#50795,#50796,#50797,#50798,#50799,#50800,#50801,#50802,
#50803,#50804),(#50805,#50806,#50807,#50808,#50809,#50810,#50811,#50812,
#50813,#50814,#50815,#50816,#50817,#50818),(#50819,#50820,#50821,#50822,
#50823,#50824,#50825,#50826,#50827,#50828,#50829,#50830,#50831,#50832),
(#50833,#50834,#50835,#50836,#50837,#50838,#50839,#50840,#50841,#50842,
#50843,#50844,#50845,#50846),(#50847,#50848,#50849,#50850,#50851,#50852,
#50853,#50854,#50855,#50856,#50857,#50858,#50859,#50860),(#50861,#50862,
#50863,#50864,#50865,#50866,#50867,#50868,#50869,#50870,#50871,#50872,#50873,
#50874),(#50875,#50876,#50877,#50878,#50879,#50880,#50881,#50882,#50883,
#50884,#50885,#50886,#50887,#50888),(#50889,#50890,#50891,#50892,#50893,
#50894,#50895,#50896,#50897,#50898,#50899,#50900,#50901,#50902),(#50903,
#50904,#50905,#50906,#50907,#50908,#50909,#50910,#50911,#50912,#50913,#50914,
#50915,#50916),(#50917,#50918,#50919,#50920,#50921,#50922,#50923,#50924,
#50925,#50926,#50927,#50928,#50929,#50930),(#50931,#50932,#50933,#50934,
#50935,#50936,#50937,#50938,#50939,#50940,#50941,#50942,#50943,#50944)),
 .UNSPECIFIED.,.F.,.F.,.F.,(4,1,1,1,1,1,1,1,1,1,1,1,1,1,1,1,1,1,1,1,1,1,
1,1,1,4),(4,2,2,2,2,2,4),(0.0331549352864085,0.102215297051665,0.171275658816922,
0.17559193142725,0.179908204037579,0.188540749258236,0.20580583969955,0.240336020582178,
0.274866201464806,0.309396382347435,0.378456744112691,0.412986924995319,
0.447517105877948,0.482047286760576,0.516577467643204,0.551107648525832,
0.585637829408461,0.654698191173717,0.723758552938974,0.810084005145544,
0.827349095586859,0.861879276469487,0.896409457352115,0.930939638234743,
0.948204728676058,1.),(0.0377143719408683,0.167070624995476,0.336553194126115,
0.499999999999991,0.663446805873868,0.832929375004528,0.962285628059217),
 .UNSPECIFIED.);
#222=B_SPLINE_SURFACE_WITH_KNOTS('',3,3,((#51003,#51004,#51005,#51006,#51007,
#51008,#51009,#51010,#51011,#51012,#51013,#51014,#51015,#51016),(#51017,
#51018,#51019,#51020,#51021,#51022,#51023,#51024,#51025,#51026,#51027,#51028,
#51029,#51030),(#51031,#51032,#51033,#51034,#51035,#51036,#51037,#51038,
#51039,#51040,#51041,#51042,#51043,#51044),(#51045,#51046,#51047,#51048,
#51049,#51050,#51051,#51052,#51053,#51054,#51055,#51056,#51057,#51058)),
 .UNSPECIFIED.,.F.,.F.,.F.,(4,4),(4,2,2,2,2,2,4),(0.,1.),(0.0377143719414212,
0.167070624995476,0.336553194126115,0.499999999999991,0.663446805873868,
0.832929375004528,0.962285628058582),.UNSPECIFIED.);
#223=B_SPLINE_SURFACE_WITH_KNOTS('',3,3,((#51073,#51074,#51075,#51076,#51077,
#51078,#51079,#51080,#51081,#51082,#51083,#51084,#51085,#51086),(#51087,
#51088,#51089,#51090,#51091,#51092,#51093,#51094,#51095,#51096,#51097,#51098,
#51099,#51100),(#51101,#51102,#51103,#51104,#51105,#51106,#51107,#51108,
#51109,#51110,#51111,#51112,#51113,#51114),(#51115,#51116,#51117,#51118,
#51119,#51120,#51121,#51122,#51123,#51124,#51125,#51126,#51127,#51128),
(#51129,#51130,#51131,#51132,#51133,#51134,#51135,#51136,#51137,#51138,
#51139,#51140,#51141,#51142),(#51143,#51144,#51145,#51146,#51147,#51148,
#51149,#51150,#51151,#51152,#51153,#51154,#51155,#51156),(#51157,#51158,
#51159,#51160,#51161,#51162,#51163,#51164,#51165,#51166,#51167,#51168,#51169,
#51170),(#51171,#51172,#51173,#51174,#51175,#51176,#51177,#51178,#51179,
#51180,#51181,#51182,#51183,#51184),(#51185,#51186,#51187,#51188,#51189,
#51190,#51191,#51192,#51193,#51194,#51195,#51196,#51197,#51198),(#51199,
#51200,#51201,#51202,#51203,#51204,#51205,#51206,#51207,#51208,#51209,#51210,
#51211,#51212),(#51213,#51214,#51215,#51216,#51217,#51218,#51219,#51220,
#51221,#51222,#51223,#51224,#51225,#51226),(#51227,#51228,#51229,#51230,
#51231,#51232,#51233,#51234,#51235,#51236,#51237,#51238,#51239,#51240),
(#51241,#51242,#51243,#51244,#51245,#51246,#51247,#51248,#51249,#51250,
#51251,#51252,#51253,#51254),(#51255,#51256,#51257,#51258,#51259,#51260,
#51261,#51262,#51263,#51264,#51265,#51266,#51267,#51268),(#51269,#51270,
#51271,#51272,#51273,#51274,#51275,#51276,#51277,#51278,#51279,#51280,#51281,
#51282),(#51283,#51284,#51285,#51286,#51287,#51288,#51289,#51290,#51291,
#51292,#51293,#51294,#51295,#51296),(#51297,#51298,#51299,#51300,#51301,
#51302,#51303,#51304,#51305,#51306,#51307,#51308,#51309,#51310),(#51311,
#51312,#51313,#51314,#51315,#51316,#51317,#51318,#51319,#51320,#51321,#51322,
#51323,#51324),(#51325,#51326,#51327,#51328,#51329,#51330,#51331,#51332,
#51333,#51334,#51335,#51336,#51337,#51338),(#51339,#51340,#51341,#51342,
#51343,#51344,#51345,#51346,#51347,#51348,#51349,#51350,#51351,#51352),
(#51353,#51354,#51355,#51356,#51357,#51358,#51359,#51360,#51361,#51362,
#51363,#51364,#51365,#51366),(#51367,#51368,#51369,#51370,#51371,#51372,
#51373,#51374,#51375,#51376,#51377,#51378,#51379,#51380),(#51381,#51382,
#51383,#51384,#51385,#51386,#51387,#51388,#51389,#51390,#51391,#51392,#51393,
#51394),(#51395,#51396,#51397,#51398,#51399,#51400,#51401,#51402,#51403,
#51404,#51405,#51406,#51407,#51408),(#51409,#51410,#51411,#51412,#51413,
#51414,#51415,#51416,#51417,#51418,#51419,#51420,#51421,#51422),(#51423,
#51424,#51425,#51426,#51427,#51428,#51429,#51430,#51431,#51432,#51433,#51434,
#51435,#51436),(#51437,#51438,#51439,#51440,#51441,#51442,#51443,#51444,
#51445,#51446,#51447,#51448,#51449,#51450)),.UNSPECIFIED.,.F.,.F.,.F.,(4,
1,1,1,1,1,1,1,1,1,1,1,1,1,1,1,1,1,1,1,1,1,1,1,4),(4,2,2,2,2,2,4),(0.,0.0517952713240545,
0.069060361765406,0.103590542648109,0.138120723530812,0.172650904413515,
0.207181085296218,0.276241447061624,0.414362170592436,0.431627261033787,
0.483422532357842,0.552482894123248,0.621543255888654,0.69060361765406,
0.759663979419466,0.776929069860817,0.785561615081493,0.794194160302168,
0.81145925074352,0.820091795964196,0.824408068574534,0.826566204879703,
0.828724341184871,0.897784702950277,0.966845064715684),(0.037714371941379,
0.167070624995476,0.336553194126115,0.499999999999991,0.663446805873868,
0.832929375004528,0.962285628059256),.UNSPECIFIED.);
#224=B_SPLINE_SURFACE_WITH_KNOTS('',3,3,((#51502,#51503,#51504,#51505,#51506,
#51507,#51508,#51509,#51510,#51511,#51512,#51513,#51514,#51515),(#51516,
#51517,#51518,#51519,#51520,#51521,#51522,#51523,#51524,#51525,#51526,#51527,
#51528,#51529),(#51530,#51531,#51532,#51533,#51534,#51535,#51536,#51537,
#51538,#51539,#51540,#51541,#51542,#51543),(#51544,#51545,#51546,#51547,
#51548,#51549,#51550,#51551,#51552,#51553,#51554,#51555,#51556,#51557),
(#51558,#51559,#51560,#51561,#51562,#51563,#51564,#51565,#51566,#51567,
#51568,#51569,#51570,#51571),(#51572,#51573,#51574,#51575,#51576,#51577,
#51578,#51579,#51580,#51581,#51582,#51583,#51584,#51585),(#51586,#51587,
#51588,#51589,#51590,#51591,#51592,#51593,#51594,#51595,#51596,#51597,#51598,
#51599),(#51600,#51601,#51602,#51603,#51604,#51605,#51606,#51607,#51608,
#51609,#51610,#51611,#51612,#51613),(#51614,#51615,#51616,#51617,#51618,
#51619,#51620,#51621,#51622,#51623,#51624,#51625,#51626,#51627),(#51628,
#51629,#51630,#51631,#51632,#51633,#51634,#51635,#51636,#51637,#51638,#51639,
#51640,#51641),(#51642,#51643,#51644,#51645,#51646,#51647,#51648,#51649,
#51650,#51651,#51652,#51653,#51654,#51655),(#51656,#51657,#51658,#51659,
#51660,#51661,#51662,#51663,#51664,#51665,#51666,#51667,#51668,#51669),
(#51670,#51671,#51672,#51673,#51674,#51675,#51676,#51677,#51678,#51679,
#51680,#51681,#51682,#51683),(#51684,#51685,#51686,#51687,#51688,#51689,
#51690,#51691,#51692,#51693,#51694,#51695,#51696,#51697),(#51698,#51699,
#51700,#51701,#51702,#51703,#51704,#51705,#51706,#51707,#51708,#51709,#51710,
#51711),(#51712,#51713,#51714,#51715,#51716,#51717,#51718,#51719,#51720,
#51721,#51722,#51723,#51724,#51725),(#51726,#51727,#51728,#51729,#51730,
#51731,#51732,#51733,#51734,#51735,#51736,#51737,#51738,#51739),(#51740,
#51741,#51742,#51743,#51744,#51745,#51746,#51747,#51748,#51749,#51750,#51751,
#51752,#51753),(#51754,#51755,#51756,#51757,#51758,#51759,#51760,#51761,
#51762,#51763,#51764,#51765,#51766,#51767),(#51768,#51769,#51770,#51771,
#51772,#51773,#51774,#51775,#51776,#51777,#51778,#51779,#51780,#51781),
(#51782,#51783,#51784,#51785,#51786,#51787,#51788,#51789,#51790,#51791,
#51792,#51793,#51794,#51795),(#51796,#51797,#51798,#51799,#51800,#51801,
#51802,#51803,#51804,#51805,#51806,#51807,#51808,#51809),(#51810,#51811,
#51812,#51813,#51814,#51815,#51816,#51817,#51818,#51819,#51820,#51821,#51822,
#51823),(#51824,#51825,#51826,#51827,#51828,#51829,#51830,#51831,#51832,
#51833,#51834,#51835,#51836,#51837),(#51838,#51839,#51840,#51841,#51842,
#51843,#51844,#51845,#51846,#51847,#51848,#51849,#51850,#51851),(#51852,
#51853,#51854,#51855,#51856,#51857,#51858,#51859,#51860,#51861,#51862,#51863,
#51864,#51865),(#51866,#51867,#51868,#51869,#51870,#51871,#51872,#51873,
#51874,#51875,#51876,#51877,#51878,#51879),(#51880,#51881,#51882,#51883,
#51884,#51885,#51886,#51887,#51888,#51889,#51890,#51891,#51892,#51893),
(#51894,#51895,#51896,#51897,#51898,#51899,#51900,#51901,#51902,#51903,
#51904,#51905,#51906,#51907),(#51908,#51909,#51910,#51911,#51912,#51913,
#51914,#51915,#51916,#51917,#51918,#51919,#51920,#51921),(#51922,#51923,
#51924,#51925,#51926,#51927,#51928,#51929,#51930,#51931,#51932,#51933,#51934,
#51935),(#51936,#51937,#51938,#51939,#51940,#51941,#51942,#51943,#51944,
#51945,#51946,#51947,#51948,#51949),(#51950,#51951,#51952,#51953,#51954,
#51955,#51956,#51957,#51958,#51959,#51960,#51961,#51962,#51963)),
 .UNSPECIFIED.,.F.,.F.,.F.,(4,1,1,1,1,1,1,1,1,1,1,1,1,1,1,1,1,1,1,1,1,1,
1,1,1,1,1,1,1,1,4),(4,2,2,2,2,2,4),(0.0331549352864046,0.102215297051661,
0.171275658816918,0.1723547269695,0.173433795122083,0.174512863274665,0.175591931427247,
0.179908204037575,0.188540749258232,0.19717329447889,0.201489567089218,
0.205805839699547,0.223070930140861,0.240336020582175,0.274866201464803,
0.309396382347432,0.378456744112689,0.412986924995317,0.430252015436631,
0.447517105877945,0.516577467643202,0.585637829408459,0.654698191173716,
0.689228372056344,0.723758552938973,0.810084005145544,0.861879276469486,
0.896409457352115,0.930939638234743,0.948204728676057,1.),(0.0377143719409187,
0.167070624995476,0.336553194126115,0.499999999999991,0.663446805873868,
0.832929375004528,0.962285628058616),.UNSPECIFIED.);
#225=B_SPLINE_SURFACE_WITH_KNOTS('',3,3,((#52024,#52025,#52026,#52027,#52028,
#52029,#52030,#52031,#52032,#52033,#52034,#52035,#52036,#52037),(#52038,
#52039,#52040,#52041,#52042,#52043,#52044,#52045,#52046,#52047,#52048,#52049,
#52050,#52051),(#52052,#52053,#52054,#52055,#52056,#52057,#52058,#52059,
#52060,#52061,#52062,#52063,#52064,#52065),(#52066,#52067,#52068,#52069,
#52070,#52071,#52072,#52073,#52074,#52075,#52076,#52077,#52078,#52079)),
 .UNSPECIFIED.,.F.,.F.,.F.,(4,4),(4,2,2,2,2,2,4),(0.,1.),(0.0377143719414211,
0.167070624995476,0.336553194126115,0.499999999999991,0.663446805873868,
0.832929375004528,0.962285628058582),.UNSPECIFIED.);
#226=B_SPLINE_SURFACE_WITH_KNOTS('',3,3,((#52094,#52095,#52096,#52097,#52098,
#52099,#52100,#52101,#52102,#52103,#52104,#52105,#52106,#52107),(#52108,
#52109,#52110,#52111,#52112,#52113,#52114,#52115,#52116,#52117,#52118,#52119,
#52120,#52121),(#52122,#52123,#52124,#52125,#52126,#52127,#52128,#52129,
#52130,#52131,#52132,#52133,#52134,#52135),(#52136,#52137,#52138,#52139,
#52140,#52141,#52142,#52143,#52144,#52145,#52146,#52147,#52148,#52149),
(#52150,#52151,#52152,#52153,#52154,#52155,#52156,#52157,#52158,#52159,
#52160,#52161,#52162,#52163),(#52164,#52165,#52166,#52167,#52168,#52169,
#52170,#52171,#52172,#52173,#52174,#52175,#52176,#52177),(#52178,#52179,
#52180,#52181,#52182,#52183,#52184,#52185,#52186,#52187,#52188,#52189,#52190,
#52191),(#52192,#52193,#52194,#52195,#52196,#52197,#52198,#52199,#52200,
#52201,#52202,#52203,#52204,#52205),(#52206,#52207,#52208,#52209,#52210,
#52211,#52212,#52213,#52214,#52215,#52216,#52217,#52218,#52219),(#52220,
#52221,#52222,#52223,#52224,#52225,#52226,#52227,#52228,#52229,#52230,#52231,
#52232,#52233),(#52234,#52235,#52236,#52237,#52238,#52239,#52240,#52241,
#52242,#52243,#52244,#52245,#52246,#52247),(#52248,#52249,#52250,#52251,
#52252,#52253,#52254,#52255,#52256,#52257,#52258,#52259,#52260,#52261),
(#52262,#52263,#52264,#52265,#52266,#52267,#52268,#52269,#52270,#52271,
#52272,#52273,#52274,#52275),(#52276,#52277,#52278,#52279,#52280,#52281,
#52282,#52283,#52284,#52285,#52286,#52287,#52288,#52289),(#52290,#52291,
#52292,#52293,#52294,#52295,#52296,#52297,#52298,#52299,#52300,#52301,#52302,
#52303),(#52304,#52305,#52306,#52307,#52308,#52309,#52310,#52311,#52312,
#52313,#52314,#52315,#52316,#52317),(#52318,#52319,#52320,#52321,#52322,
#52323,#52324,#52325,#52326,#52327,#52328,#52329,#52330,#52331),(#52332,
#52333,#52334,#52335,#52336,#52337,#52338,#52339,#52340,#52341,#52342,#52343,
#52344,#52345),(#52346,#52347,#52348,#52349,#52350,#52351,#52352,#52353,
#52354,#52355,#52356,#52357,#52358,#52359),(#52360,#52361,#52362,#52363,
#52364,#52365,#52366,#52367,#52368,#52369,#52370,#52371,#52372,#52373),
(#52374,#52375,#52376,#52377,#52378,#52379,#52380,#52381,#52382,#52383,
#52384,#52385,#52386,#52387),(#52388,#52389,#52390,#52391,#52392,#52393,
#52394,#52395,#52396,#52397,#52398,#52399,#52400,#52401),(#52402,#52403,
#52404,#52405,#52406,#52407,#52408,#52409,#52410,#52411,#52412,#52413,#52414,
#52415),(#52416,#52417,#52418,#52419,#52420,#52421,#52422,#52423,#52424,
#52425,#52426,#52427,#52428,#52429),(#52430,#52431,#52432,#52433,#52434,
#52435,#52436,#52437,#52438,#52439,#52440,#52441,#52442,#52443),(#52444,
#52445,#52446,#52447,#52448,#52449,#52450,#52451,#52452,#52453,#52454,#52455,
#52456,#52457),(#52458,#52459,#52460,#52461,#52462,#52463,#52464,#52465,
#52466,#52467,#52468,#52469,#52470,#52471),(#52472,#52473,#52474,#52475,
#52476,#52477,#52478,#52479,#52480,#52481,#52482,#52483,#52484,#52485),
(#52486,#52487,#52488,#52489,#52490,#52491,#52492,#52493,#52494,#52495,
#52496,#52497,#52498,#52499),(#52500,#52501,#52502,#52503,#52504,#52505,
#52506,#52507,#52508,#52509,#52510,#52511,#52512,#52513),(#52514,#52515,
#52516,#52517,#52518,#52519,#52520,#52521,#52522,#52523,#52524,#52525,#52526,
#52527),(#52528,#52529,#52530,#52531,#52532,#52533,#52534,#52535,#52536,
#52537,#52538,#52539,#52540,#52541),(#52542,#52543,#52544,#52545,#52546,
#52547,#52548,#52549,#52550,#52551,#52552,#52553,#52554,#52555),(#52556,
#52557,#52558,#52559,#52560,#52561,#52562,#52563,#52564,#52565,#52566,#52567,
#52568,#52569),(#52570,#52571,#52572,#52573,#52574,#52575,#52576,#52577,
#52578,#52579,#52580,#52581,#52582,#52583),(#52584,#52585,#52586,#52587,
#52588,#52589,#52590,#52591,#52592,#52593,#52594,#52595,#52596,#52597),
(#52598,#52599,#52600,#52601,#52602,#52603,#52604,#52605,#52606,#52607,
#52608,#52609,#52610,#52611),(#52612,#52613,#52614,#52615,#52616,#52617,
#52618,#52619,#52620,#52621,#52622,#52623,#52624,#52625),(#52626,#52627,
#52628,#52629,#52630,#52631,#52632,#52633,#52634,#52635,#52636,#52637,#52638,
#52639),(#52640,#52641,#52642,#52643,#52644,#52645,#52646,#52647,#52648,
#52649,#52650,#52651,#52652,#52653),(#52654,#52655,#52656,#52657,#52658,
#52659,#52660,#52661,#52662,#52663,#52664,#52665,#52666,#52667)),
 .UNSPECIFIED.,.F.,.F.,.F.,(4,1,1,1,1,1,1,1,1,1,1,1,1,1,1,1,1,1,1,1,1,1,
1,1,1,1,1,1,1,1,1,1,1,1,1,1,1,1,4),(4,2,2,2,2,2,4),(0.,0.0517952713240546,
0.0690603617654062,0.103590542648109,0.138120723530812,0.172650904413515,
0.207181085296219,0.276241447061625,0.310771627944328,0.345301808827031,
0.414362170592437,0.422994715813113,0.431627261033789,0.44889235147514,
0.483422532357843,0.552482894123249,0.587013075005953,0.595645620226628,
0.621543255888656,0.656073436771359,0.690603617654062,0.725133798536765,
0.759663979419468,0.763980252029806,0.768296524640144,0.77692906986082,
0.794194160302171,0.802826705522847,0.811459250743523,0.820091795964198,
0.824408068574536,0.825487136727121,0.826566204879705,0.82764527303229,
0.828184807108582,0.828454574146728,0.828724341184874,0.89778470295028,
0.966845064715687),(0.0377143719402601,0.167070624995476,0.336553194126115,
0.499999999999991,0.663446805873868,0.832929375004528,0.962285628059988),
 .UNSPECIFIED.);
#227=B_SPLINE_SURFACE_WITH_KNOTS('',3,3,((#52721,#52722,#52723,#52724,#52725,
#52726,#52727,#52728,#52729,#52730,#52731,#52732,#52733,#52734),(#52735,
#52736,#52737,#52738,#52739,#52740,#52741,#52742,#52743,#52744,#52745,#52746,
#52747,#52748),(#52749,#52750,#52751,#52752,#52753,#52754,#52755,#52756,
#52757,#52758,#52759,#52760,#52761,#52762),(#52763,#52764,#52765,#52766,
#52767,#52768,#52769,#52770,#52771,#52772,#52773,#52774,#52775,#52776),
(#52777,#52778,#52779,#52780,#52781,#52782,#52783,#52784,#52785,#52786,
#52787,#52788,#52789,#52790),(#52791,#52792,#52793,#52794,#52795,#52796,
#52797,#52798,#52799,#52800,#52801,#52802,#52803,#52804),(#52805,#52806,
#52807,#52808,#52809,#52810,#52811,#52812,#52813,#52814,#52815,#52816,#52817,
#52818),(#52819,#52820,#52821,#52822,#52823,#52824,#52825,#52826,#52827,
#52828,#52829,#52830,#52831,#52832),(#52833,#52834,#52835,#52836,#52837,
#52838,#52839,#52840,#52841,#52842,#52843,#52844,#52845,#52846),(#52847,
#52848,#52849,#52850,#52851,#52852,#52853,#52854,#52855,#52856,#52857,#52858,
#52859,#52860),(#52861,#52862,#52863,#52864,#52865,#52866,#52867,#52868,
#52869,#52870,#52871,#52872,#52873,#52874),(#52875,#52876,#52877,#52878,
#52879,#52880,#52881,#52882,#52883,#52884,#52885,#52886,#52887,#52888),
(#52889,#52890,#52891,#52892,#52893,#52894,#52895,#52896,#52897,#52898,
#52899,#52900,#52901,#52902),(#52903,#52904,#52905,#52906,#52907,#52908,
#52909,#52910,#52911,#52912,#52913,#52914,#52915,#52916),(#52917,#52918,
#52919,#52920,#52921,#52922,#52923,#52924,#52925,#52926,#52927,#52928,#52929,
#52930),(#52931,#52932,#52933,#52934,#52935,#52936,#52937,#52938,#52939,
#52940,#52941,#52942,#52943,#52944),(#52945,#52946,#52947,#52948,#52949,
#52950,#52951,#52952,#52953,#52954,#52955,#52956,#52957,#52958),(#52959,
#52960,#52961,#52962,#52963,#52964,#52965,#52966,#52967,#52968,#52969,#52970,
#52971,#52972),(#52973,#52974,#52975,#52976,#52977,#52978,#52979,#52980,
#52981,#52982,#52983,#52984,#52985,#52986),(#52987,#52988,#52989,#52990,
#52991,#52992,#52993,#52994,#52995,#52996,#52997,#52998,#52999,#53000),
(#53001,#53002,#53003,#53004,#53005,#53006,#53007,#53008,#53009,#53010,
#53011,#53012,#53013,#53014),(#53015,#53016,#53017,#53018,#53019,#53020,
#53021,#53022,#53023,#53024,#53025,#53026,#53027,#53028),(#53029,#53030,
#53031,#53032,#53033,#53034,#53035,#53036,#53037,#53038,#53039,#53040,#53041,
#53042),(#53043,#53044,#53045,#53046,#53047,#53048,#53049,#53050,#53051,
#53052,#53053,#53054,#53055,#53056),(#53057,#53058,#53059,#53060,#53061,
#53062,#53063,#53064,#53065,#53066,#53067,#53068,#53069,#53070),(#53071,
#53072,#53073,#53074,#53075,#53076,#53077,#53078,#53079,#53080,#53081,#53082,
#53083,#53084),(#53085,#53086,#53087,#53088,#53089,#53090,#53091,#53092,
#53093,#53094,#53095,#53096,#53097,#53098),(#53099,#53100,#53101,#53102,
#53103,#53104,#53105,#53106,#53107,#53108,#53109,#53110,#53111,#53112),
(#53113,#53114,#53115,#53116,#53117,#53118,#53119,#53120,#53121,#53122,
#53123,#53124,#53125,#53126)),.UNSPECIFIED.,.F.,.F.,.F.,(4,1,1,1,1,1,1,
1,1,1,1,1,1,1,1,1,1,1,1,1,1,1,1,1,1,1,4),(4,2,2,2,2,2,4),(0.0331549352864105,
0.102215297051667,0.171275658816923,0.173433795122088,0.175591931427252,
0.17990820403758,0.188540749258237,0.205805839699551,0.24033602058218,0.274866201464808,
0.309396382347436,0.378456744112692,0.412986924995321,0.447517105877949,
0.516577467643205,0.585637829408462,0.602902919849776,0.62016801029109,
0.654698191173718,0.689228372056346,0.723758552938975,0.810084005145545,
0.861879276469487,0.896409457352116,0.930939638234744,0.948204728676058,
1.),(0.0377143719413902,0.167070624995476,0.336553194126115,0.499999999999991,
0.663446805873868,0.832929375004528,0.962285628058762),.UNSPECIFIED.);
#228=B_SPLINE_SURFACE_WITH_KNOTS('',3,3,((#53183,#53184,#53185,#53186,#53187,
#53188,#53189,#53190,#53191,#53192,#53193,#53194,#53195,#53196),(#53197,
#53198,#53199,#53200,#53201,#53202,#53203,#53204,#53205,#53206,#53207,#53208,
#53209,#53210),(#53211,#53212,#53213,#53214,#53215,#53216,#53217,#53218,
#53219,#53220,#53221,#53222,#53223,#53224),(#53225,#53226,#53227,#53228,
#53229,#53230,#53231,#53232,#53233,#53234,#53235,#53236,#53237,#53238)),
 .UNSPECIFIED.,.F.,.F.,.F.,(4,4),(4,2,2,2,2,2,4),(0.,1.),(0.0377143719414212,
0.167070624995476,0.336553194126115,0.499999999999991,0.663446805873868,
0.832929375004528,0.962285628058582),.UNSPECIFIED.);
#229=B_SPLINE_SURFACE_WITH_KNOTS('',3,3,((#53253,#53254,#53255,#53256,#53257,
#53258,#53259,#53260,#53261,#53262,#53263,#53264,#53265,#53266),(#53267,
#53268,#53269,#53270,#53271,#53272,#53273,#53274,#53275,#53276,#53277,#53278,
#53279,#53280),(#53281,#53282,#53283,#53284,#53285,#53286,#53287,#53288,
#53289,#53290,#53291,#53292,#53293,#53294),(#53295,#53296,#53297,#53298,
#53299,#53300,#53301,#53302,#53303,#53304,#53305,#53306,#53307,#53308),
(#53309,#53310,#53311,#53312,#53313,#53314,#53315,#53316,#53317,#53318,
#53319,#53320,#53321,#53322),(#53323,#53324,#53325,#53326,#53327,#53328,
#53329,#53330,#53331,#53332,#53333,#53334,#53335,#53336),(#53337,#53338,
#53339,#53340,#53341,#53342,#53343,#53344,#53345,#53346,#53347,#53348,#53349,
#53350),(#53351,#53352,#53353,#53354,#53355,#53356,#53357,#53358,#53359,
#53360,#53361,#53362,#53363,#53364),(#53365,#53366,#53367,#53368,#53369,
#53370,#53371,#53372,#53373,#53374,#53375,#53376,#53377,#53378),(#53379,
#53380,#53381,#53382,#53383,#53384,#53385,#53386,#53387,#53388,#53389,#53390,
#53391,#53392),(#53393,#53394,#53395,#53396,#53397,#53398,#53399,#53400,
#53401,#53402,#53403,#53404,#53405,#53406),(#53407,#53408,#53409,#53410,
#53411,#53412,#53413,#53414,#53415,#53416,#53417,#53418,#53419,#53420),
(#53421,#53422,#53423,#53424,#53425,#53426,#53427,#53428,#53429,#53430,
#53431,#53432,#53433,#53434),(#53435,#53436,#53437,#53438,#53439,#53440,
#53441,#53442,#53443,#53444,#53445,#53446,#53447,#53448),(#53449,#53450,
#53451,#53452,#53453,#53454,#53455,#53456,#53457,#53458,#53459,#53460,#53461,
#53462),(#53463,#53464,#53465,#53466,#53467,#53468,#53469,#53470,#53471,
#53472,#53473,#53474,#53475,#53476),(#53477,#53478,#53479,#53480,#53481,
#53482,#53483,#53484,#53485,#53486,#53487,#53488,#53489,#53490),(#53491,
#53492,#53493,#53494,#53495,#53496,#53497,#53498,#53499,#53500,#53501,#53502,
#53503,#53504),(#53505,#53506,#53507,#53508,#53509,#53510,#53511,#53512,
#53513,#53514,#53515,#53516,#53517,#53518),(#53519,#53520,#53521,#53522,
#53523,#53524,#53525,#53526,#53527,#53528,#53529,#53530,#53531,#53532),
(#53533,#53534,#53535,#53536,#53537,#53538,#53539,#53540,#53541,#53542,
#53543,#53544,#53545,#53546),(#53547,#53548,#53549,#53550,#53551,#53552,
#53553,#53554,#53555,#53556,#53557,#53558,#53559,#53560),(#53561,#53562,
#53563,#53564,#53565,#53566,#53567,#53568,#53569,#53570,#53571,#53572,#53573,
#53574),(#53575,#53576,#53577,#53578,#53579,#53580,#53581,#53582,#53583,
#53584,#53585,#53586,#53587,#53588),(#53589,#53590,#53591,#53592,#53593,
#53594,#53595,#53596,#53597,#53598,#53599,#53600,#53601,#53602),(#53603,
#53604,#53605,#53606,#53607,#53608,#53609,#53610,#53611,#53612,#53613,#53614,
#53615,#53616),(#53617,#53618,#53619,#53620,#53621,#53622,#53623,#53624,
#53625,#53626,#53627,#53628,#53629,#53630),(#53631,#53632,#53633,#53634,
#53635,#53636,#53637,#53638,#53639,#53640,#53641,#53642,#53643,#53644),
(#53645,#53646,#53647,#53648,#53649,#53650,#53651,#53652,#53653,#53654,
#53655,#53656,#53657,#53658),(#53659,#53660,#53661,#53662,#53663,#53664,
#53665,#53666,#53667,#53668,#53669,#53670,#53671,#53672),(#53673,#53674,
#53675,#53676,#53677,#53678,#53679,#53680,#53681,#53682,#53683,#53684,#53685,
#53686),(#53687,#53688,#53689,#53690,#53691,#53692,#53693,#53694,#53695,
#53696,#53697,#53698,#53699,#53700),(#53701,#53702,#53703,#53704,#53705,
#53706,#53707,#53708,#53709,#53710,#53711,#53712,#53713,#53714)),
 .UNSPECIFIED.,.F.,.F.,.F.,(4,1,1,1,1,1,1,1,1,1,1,1,1,1,1,1,1,1,1,1,1,1,
1,1,1,1,1,1,1,1,4),(4,2,2,2,2,2,4),(0.,0.0517952713240545,0.069060361765406,
0.103590542648109,0.138120723530812,0.172650904413515,0.207181085296218,
0.276241447061624,0.310771627944327,0.414362170592436,0.483422532357842,
0.500687622799194,0.517952713240545,0.552482894123248,0.621543255888654,
0.69060361765406,0.759663979419466,0.776929069860818,0.785561615081493,
0.789877887691831,0.794194160302169,0.802826705522845,0.811459250743521,
0.820091795964196,0.824408068574534,0.826566204879703,0.827645273032288,
0.82818480710858,0.828724341184872,0.897784702950278,0.966845064715684),
(0.0377143719414203,0.167070624995476,0.336553194126115,0.499999999999991,
0.663446805873868,0.832929375004528,0.962285628060272),.UNSPECIFIED.);
#230=B_SPLINE_SURFACE_WITH_KNOTS('',3,3,((#53766,#53767,#53768,#53769,#53770,
#53771,#53772,#53773,#53774,#53775,#53776,#53777,#53778,#53779),(#53780,
#53781,#53782,#53783,#53784,#53785,#53786,#53787,#53788,#53789,#53790,#53791,
#53792,#53793),(#53794,#53795,#53796,#53797,#53798,#53799,#53800,#53801,
#53802,#53803,#53804,#53805,#53806,#53807),(#53808,#53809,#53810,#53811,
#53812,#53813,#53814,#53815,#53816,#53817,#53818,#53819,#53820,#53821),
(#53822,#53823,#53824,#53825,#53826,#53827,#53828,#53829,#53830,#53831,
#53832,#53833,#53834,#53835),(#53836,#53837,#53838,#53839,#53840,#53841,
#53842,#53843,#53844,#53845,#53846,#53847,#53848,#53849),(#53850,#53851,
#53852,#53853,#53854,#53855,#53856,#53857,#53858,#53859,#53860,#53861,#53862,
#53863),(#53864,#53865,#53866,#53867,#53868,#53869,#53870,#53871,#53872,
#53873,#53874,#53875,#53876,#53877),(#53878,#53879,#53880,#53881,#53882,
#53883,#53884,#53885,#53886,#53887,#53888,#53889,#53890,#53891),(#53892,
#53893,#53894,#53895,#53896,#53897,#53898,#53899,#53900,#53901,#53902,#53903,
#53904,#53905),(#53906,#53907,#53908,#53909,#53910,#53911,#53912,#53913,
#53914,#53915,#53916,#53917,#53918,#53919),(#53920,#53921,#53922,#53923,
#53924,#53925,#53926,#53927,#53928,#53929,#53930,#53931,#53932,#53933),
(#53934,#53935,#53936,#53937,#53938,#53939,#53940,#53941,#53942,#53943,
#53944,#53945,#53946,#53947),(#53948,#53949,#53950,#53951,#53952,#53953,
#53954,#53955,#53956,#53957,#53958,#53959,#53960,#53961),(#53962,#53963,
#53964,#53965,#53966,#53967,#53968,#53969,#53970,#53971,#53972,#53973,#53974,
#53975),(#53976,#53977,#53978,#53979,#53980,#53981,#53982,#53983,#53984,
#53985,#53986,#53987,#53988,#53989),(#53990,#53991,#53992,#53993,#53994,
#53995,#53996,#53997,#53998,#53999,#54000,#54001,#54002,#54003),(#54004,
#54005,#54006,#54007,#54008,#54009,#54010,#54011,#54012,#54013,#54014,#54015,
#54016,#54017),(#54018,#54019,#54020,#54021,#54022,#54023,#54024,#54025,
#54026,#54027,#54028,#54029,#54030,#54031),(#54032,#54033,#54034,#54035,
#54036,#54037,#54038,#54039,#54040,#54041,#54042,#54043,#54044,#54045),
(#54046,#54047,#54048,#54049,#54050,#54051,#54052,#54053,#54054,#54055,
#54056,#54057,#54058,#54059),(#54060,#54061,#54062,#54063,#54064,#54065,
#54066,#54067,#54068,#54069,#54070,#54071,#54072,#54073),(#54074,#54075,
#54076,#54077,#54078,#54079,#54080,#54081,#54082,#54083,#54084,#54085,#54086,
#54087),(#54088,#54089,#54090,#54091,#54092,#54093,#54094,#54095,#54096,
#54097,#54098,#54099,#54100,#54101),(#54102,#54103,#54104,#54105,#54106,
#54107,#54108,#54109,#54110,#54111,#54112,#54113,#54114,#54115),(#54116,
#54117,#54118,#54119,#54120,#54121,#54122,#54123,#54124,#54125,#54126,#54127,
#54128,#54129),(#54130,#54131,#54132,#54133,#54134,#54135,#54136,#54137,
#54138,#54139,#54140,#54141,#54142,#54143),(#54144,#54145,#54146,#54147,
#54148,#54149,#54150,#54151,#54152,#54153,#54154,#54155,#54156,#54157),
(#54158,#54159,#54160,#54161,#54162,#54163,#54164,#54165,#54166,#54167,
#54168,#54169,#54170,#54171),(#54172,#54173,#54174,#54175,#54176,#54177,
#54178,#54179,#54180,#54181,#54182,#54183,#54184,#54185),(#54186,#54187,
#54188,#54189,#54190,#54191,#54192,#54193,#54194,#54195,#54196,#54197,#54198,
#54199)),.UNSPECIFIED.,.F.,.F.,.F.,(4,1,1,1,1,1,1,1,1,1,1,1,1,1,1,1,1,1,
1,1,1,1,1,1,1,1,1,1,4),(4,2,2,2,2,2,4),(0.0331549352864077,0.102215297051664,
0.171275658816921,0.173433795122085,0.175591931427249,0.179908204037578,
0.188540749258235,0.205805839699549,0.223070930140863,0.240336020582177,
0.309396382347434,0.378456744112691,0.447517105877947,0.516577467643204,
0.551107648525832,0.58563782940846,0.594270374629118,0.602902919849775,
0.620168010291089,0.654698191173717,0.689228372056345,0.723758552938974,
0.810084005145544,0.844614186028173,0.861879276469487,0.896409457352115,
0.930939638234743,0.948204728676058,1.),(0.0377143719414061,0.167070624995476,
0.336553194126115,0.499999999999991,0.663446805873868,0.832929375004528,
0.962285628058718),.UNSPECIFIED.);
#231=B_SPLINE_SURFACE_WITH_KNOTS('',3,3,((#54256,#54257,#54258,#54259,#54260,
#54261,#54262,#54263,#54264,#54265,#54266,#54267,#54268,#54269),(#54270,
#54271,#54272,#54273,#54274,#54275,#54276,#54277,#54278,#54279,#54280,#54281,
#54282,#54283),(#54284,#54285,#54286,#54287,#54288,#54289,#54290,#54291,
#54292,#54293,#54294,#54295,#54296,#54297),(#54298,#54299,#54300,#54301,
#54302,#54303,#54304,#54305,#54306,#54307,#54308,#54309,#54310,#54311)),
 .UNSPECIFIED.,.F.,.F.,.F.,(4,4),(4,2,2,2,2,2,4),(0.,1.),(0.0377143719414212,
0.167070624995476,0.336553194126115,0.499999999999991,0.663446805873868,
0.832929375004528,0.962285628058582),.UNSPECIFIED.);
#232=B_SPLINE_SURFACE_WITH_KNOTS('',3,3,((#54326,#54327,#54328,#54329,#54330,
#54331,#54332,#54333,#54334,#54335,#54336,#54337,#54338,#54339),(#54340,
#54341,#54342,#54343,#54344,#54345,#54346,#54347,#54348,#54349,#54350,#54351,
#54352,#54353),(#54354,#54355,#54356,#54357,#54358,#54359,#54360,#54361,
#54362,#54363,#54364,#54365,#54366,#54367),(#54368,#54369,#54370,#54371,
#54372,#54373,#54374,#54375,#54376,#54377,#54378,#54379,#54380,#54381),
(#54382,#54383,#54384,#54385,#54386,#54387,#54388,#54389,#54390,#54391,
#54392,#54393,#54394,#54395),(#54396,#54397,#54398,#54399,#54400,#54401,
#54402,#54403,#54404,#54405,#54406,#54407,#54408,#54409),(#54410,#54411,
#54412,#54413,#54414,#54415,#54416,#54417,#54418,#54419,#54420,#54421,#54422,
#54423),(#54424,#54425,#54426,#54427,#54428,#54429,#54430,#54431,#54432,
#54433,#54434,#54435,#54436,#54437),(#54438,#54439,#54440,#54441,#54442,
#54443,#54444,#54445,#54446,#54447,#54448,#54449,#54450,#54451),(#54452,
#54453,#54454,#54455,#54456,#54457,#54458,#54459,#54460,#54461,#54462,#54463,
#54464,#54465),(#54466,#54467,#54468,#54469,#54470,#54471,#54472,#54473,
#54474,#54475,#54476,#54477,#54478,#54479),(#54480,#54481,#54482,#54483,
#54484,#54485,#54486,#54487,#54488,#54489,#54490,#54491,#54492,#54493),
(#54494,#54495,#54496,#54497,#54498,#54499,#54500,#54501,#54502,#54503,
#54504,#54505,#54506,#54507),(#54508,#54509,#54510,#54511,#54512,#54513,
#54514,#54515,#54516,#54517,#54518,#54519,#54520,#54521),(#54522,#54523,
#54524,#54525,#54526,#54527,#54528,#54529,#54530,#54531,#54532,#54533,#54534,
#54535),(#54536,#54537,#54538,#54539,#54540,#54541,#54542,#54543,#54544,
#54545,#54546,#54547,#54548,#54549),(#54550,#54551,#54552,#54553,#54554,
#54555,#54556,#54557,#54558,#54559,#54560,#54561,#54562,#54563),(#54564,
#54565,#54566,#54567,#54568,#54569,#54570,#54571,#54572,#54573,#54574,#54575,
#54576,#54577),(#54578,#54579,#54580,#54581,#54582,#54583,#54584,#54585,
#54586,#54587,#54588,#54589,#54590,#54591),(#54592,#54593,#54594,#54595,
#54596,#54597,#54598,#54599,#54600,#54601,#54602,#54603,#54604,#54605),
(#54606,#54607,#54608,#54609,#54610,#54611,#54612,#54613,#54614,#54615,
#54616,#54617,#54618,#54619),(#54620,#54621,#54622,#54623,#54624,#54625,
#54626,#54627,#54628,#54629,#54630,#54631,#54632,#54633),(#54634,#54635,
#54636,#54637,#54638,#54639,#54640,#54641,#54642,#54643,#54644,#54645,#54646,
#54647),(#54648,#54649,#54650,#54651,#54652,#54653,#54654,#54655,#54656,
#54657,#54658,#54659,#54660,#54661),(#54662,#54663,#54664,#54665,#54666,
#54667,#54668,#54669,#54670,#54671,#54672,#54673,#54674,#54675),(#54676,
#54677,#54678,#54679,#54680,#54681,#54682,#54683,#54684,#54685,#54686,#54687,
#54688,#54689),(#54690,#54691,#54692,#54693,#54694,#54695,#54696,#54697,
#54698,#54699,#54700,#54701,#54702,#54703),(#54704,#54705,#54706,#54707,
#54708,#54709,#54710,#54711,#54712,#54713,#54714,#54715,#54716,#54717),
(#54718,#54719,#54720,#54721,#54722,#54723,#54724,#54725,#54726,#54727,
#54728,#54729,#54730,#54731),(#54732,#54733,#54734,#54735,#54736,#54737,
#54738,#54739,#54740,#54741,#54742,#54743,#54744,#54745),(#54746,#54747,
#54748,#54749,#54750,#54751,#54752,#54753,#54754,#54755,#54756,#54757,#54758,
#54759)),.UNSPECIFIED.,.F.,.F.,.F.,(4,1,1,1,1,1,1,1,1,1,1,1,1,1,1,1,1,1,
1,1,1,1,1,1,1,1,1,1,4),(4,2,2,2,2,2,4),(0.,0.0517952713240543,0.0690603617654058,
0.103590542648109,0.138120723530812,0.155385813972163,0.189915994854866,
0.276241447061623,0.345301808827029,0.414362170592435,0.431627261033786,
0.448892351475138,0.48342253235784,0.517952713240543,0.552482894123246,
0.587013075005949,0.621543255888652,0.690603617654058,0.699236162874733,
0.725133798536761,0.759663979419464,0.794194160302166,0.811459250743518,
0.820091795964194,0.824408068574531,0.8265662048797,0.828724341184869,0.897784702950275,
0.966845064715681),(0.0377143719405064,0.167070624995476,0.336553194126115,
0.499999999999991,0.663446805873868,0.832929375004528,0.962285628058607),
 .UNSPECIFIED.);
#233=B_SPLINE_SURFACE_WITH_KNOTS('',3,3,((#54817,#54818,#54819,#54820,#54821,
#54822,#54823,#54824,#54825,#54826,#54827,#54828,#54829,#54830),(#54831,
#54832,#54833,#54834,#54835,#54836,#54837,#54838,#54839,#54840,#54841,#54842,
#54843,#54844),(#54845,#54846,#54847,#54848,#54849,#54850,#54851,#54852,
#54853,#54854,#54855,#54856,#54857,#54858),(#54859,#54860,#54861,#54862,
#54863,#54864,#54865,#54866,#54867,#54868,#54869,#54870,#54871,#54872),
(#54873,#54874,#54875,#54876,#54877,#54878,#54879,#54880,#54881,#54882,
#54883,#54884,#54885,#54886),(#54887,#54888,#54889,#54890,#54891,#54892,
#54893,#54894,#54895,#54896,#54897,#54898,#54899,#54900),(#54901,#54902,
#54903,#54904,#54905,#54906,#54907,#54908,#54909,#54910,#54911,#54912,#54913,
#54914),(#54915,#54916,#54917,#54918,#54919,#54920,#54921,#54922,#54923,
#54924,#54925,#54926,#54927,#54928),(#54929,#54930,#54931,#54932,#54933,
#54934,#54935,#54936,#54937,#54938,#54939,#54940,#54941,#54942),(#54943,
#54944,#54945,#54946,#54947,#54948,#54949,#54950,#54951,#54952,#54953,#54954,
#54955,#54956),(#54957,#54958,#54959,#54960,#54961,#54962,#54963,#54964,
#54965,#54966,#54967,#54968,#54969,#54970),(#54971,#54972,#54973,#54974,
#54975,#54976,#54977,#54978,#54979,#54980,#54981,#54982,#54983,#54984),
(#54985,#54986,#54987,#54988,#54989,#54990,#54991,#54992,#54993,#54994,
#54995,#54996,#54997,#54998),(#54999,#55000,#55001,#55002,#55003,#55004,
#55005,#55006,#55007,#55008,#55009,#55010,#55011,#55012),(#55013,#55014,
#55015,#55016,#55017,#55018,#55019,#55020,#55021,#55022,#55023,#55024,#55025,
#55026),(#55027,#55028,#55029,#55030,#55031,#55032,#55033,#55034,#55035,
#55036,#55037,#55038,#55039,#55040),(#55041,#55042,#55043,#55044,#55045,
#55046,#55047,#55048,#55049,#55050,#55051,#55052,#55053,#55054),(#55055,
#55056,#55057,#55058,#55059,#55060,#55061,#55062,#55063,#55064,#55065,#55066,
#55067,#55068),(#55069,#55070,#55071,#55072,#55073,#55074,#55075,#55076,
#55077,#55078,#55079,#55080,#55081,#55082),(#55083,#55084,#55085,#55086,
#55087,#55088,#55089,#55090,#55091,#55092,#55093,#55094,#55095,#55096),
(#55097,#55098,#55099,#55100,#55101,#55102,#55103,#55104,#55105,#55106,
#55107,#55108,#55109,#55110),(#55111,#55112,#55113,#55114,#55115,#55116,
#55117,#55118,#55119,#55120,#55121,#55122,#55123,#55124),(#55125,#55126,
#55127,#55128,#55129,#55130,#55131,#55132,#55133,#55134,#55135,#55136,#55137,
#55138),(#55139,#55140,#55141,#55142,#55143,#55144,#55145,#55146,#55147,
#55148,#55149,#55150,#55151,#55152),(#55153,#55154,#55155,#55156,#55157,
#55158,#55159,#55160,#55161,#55162,#55163,#55164,#55165,#55166),(#55167,
#55168,#55169,#55170,#55171,#55172,#55173,#55174,#55175,#55176,#55177,#55178,
#55179,#55180),(#55181,#55182,#55183,#55184,#55185,#55186,#55187,#55188,
#55189,#55190,#55191,#55192,#55193,#55194),(#55195,#55196,#55197,#55198,
#55199,#55200,#55201,#55202,#55203,#55204,#55205,#55206,#55207,#55208),
(#55209,#55210,#55211,#55212,#55213,#55214,#55215,#55216,#55217,#55218,
#55219,#55220,#55221,#55222),(#55223,#55224,#55225,#55226,#55227,#55228,
#55229,#55230,#55231,#55232,#55233,#55234,#55235,#55236),(#55237,#55238,
#55239,#55240,#55241,#55242,#55243,#55244,#55245,#55246,#55247,#55248,#55249,
#55250),(#55251,#55252,#55253,#55254,#55255,#55256,#55257,#55258,#55259,
#55260,#55261,#55262,#55263,#55264),(#55265,#55266,#55267,#55268,#55269,
#55270,#55271,#55272,#55273,#55274,#55275,#55276,#55277,#55278)),
 .UNSPECIFIED.,.F.,.F.,.F.,(4,1,1,1,1,1,1,1,1,1,1,1,1,1,1,1,1,1,1,1,1,1,
1,1,1,1,1,1,1,1,4),(4,2,2,2,2,2,4),(0.0331549352864095,0.102215297051666,
0.171275658816922,0.172354726969505,0.173433795122087,0.175591931427251,
0.179908204037579,0.188540749258237,0.205805839699551,0.223070930140865,
0.240336020582179,0.274866201464807,0.309396382347435,0.378456744112692,
0.395721834554006,0.447517105877948,0.516577467643205,0.525210012863862,
0.551107648525833,0.568372738967147,0.577005284187804,0.585637829408461,
0.723758552938974,0.79281891470423,0.827349095586859,0.844614186028173,
0.861879276469487,0.896409457352115,0.930939638234743,0.948204728676058,
1.),(0.0377143719411004,0.167070624995476,0.336553194126115,0.499999999999991,
0.663446805873868,0.832929375004528,0.962285628058762),.UNSPECIFIED.);
#234=B_SPLINE_SURFACE_WITH_KNOTS('',3,3,((#55335,#55336,#55337,#55338,#55339,
#55340,#55341,#55342,#55343,#55344,#55345,#55346,#55347,#55348),(#55349,
#55350,#55351,#55352,#55353,#55354,#55355,#55356,#55357,#55358,#55359,#55360,
#55361,#55362),(#55363,#55364,#55365,#55366,#55367,#55368,#55369,#55370,
#55371,#55372,#55373,#55374,#55375,#55376),(#55377,#55378,#55379,#55380,
#55381,#55382,#55383,#55384,#55385,#55386,#55387,#55388,#55389,#55390)),
 .UNSPECIFIED.,.F.,.F.,.F.,(4,4),(4,2,2,2,2,2,4),(0.,1.),(0.0377143719414212,
0.167070624995476,0.336553194126115,0.499999999999991,0.663446805873868,
0.832929375004528,0.962285628058582),.UNSPECIFIED.);
#235=B_SPLINE_SURFACE_WITH_KNOTS('',3,3,((#55405,#55406,#55407,#55408,#55409,
#55410,#55411,#55412,#55413,#55414,#55415,#55416,#55417,#55418),(#55419,
#55420,#55421,#55422,#55423,#55424,#55425,#55426,#55427,#55428,#55429,#55430,
#55431,#55432),(#55433,#55434,#55435,#55436,#55437,#55438,#55439,#55440,
#55441,#55442,#55443,#55444,#55445,#55446),(#55447,#55448,#55449,#55450,
#55451,#55452,#55453,#55454,#55455,#55456,#55457,#55458,#55459,#55460),
(#55461,#55462,#55463,#55464,#55465,#55466,#55467,#55468,#55469,#55470,
#55471,#55472,#55473,#55474),(#55475,#55476,#55477,#55478,#55479,#55480,
#55481,#55482,#55483,#55484,#55485,#55486,#55487,#55488),(#55489,#55490,
#55491,#55492,#55493,#55494,#55495,#55496,#55497,#55498,#55499,#55500,#55501,
#55502),(#55503,#55504,#55505,#55506,#55507,#55508,#55509,#55510,#55511,
#55512,#55513,#55514,#55515,#55516),(#55517,#55518,#55519,#55520,#55521,
#55522,#55523,#55524,#55525,#55526,#55527,#55528,#55529,#55530),(#55531,
#55532,#55533,#55534,#55535,#55536,#55537,#55538,#55539,#55540,#55541,#55542,
#55543,#55544),(#55545,#55546,#55547,#55548,#55549,#55550,#55551,#55552,
#55553,#55554,#55555,#55556,#55557,#55558),(#55559,#55560,#55561,#55562,
#55563,#55564,#55565,#55566,#55567,#55568,#55569,#55570,#55571,#55572),
(#55573,#55574,#55575,#55576,#55577,#55578,#55579,#55580,#55581,#55582,
#55583,#55584,#55585,#55586),(#55587,#55588,#55589,#55590,#55591,#55592,
#55593,#55594,#55595,#55596,#55597,#55598,#55599,#55600),(#55601,#55602,
#55603,#55604,#55605,#55606,#55607,#55608,#55609,#55610,#55611,#55612,#55613,
#55614),(#55615,#55616,#55617,#55618,#55619,#55620,#55621,#55622,#55623,
#55624,#55625,#55626,#55627,#55628),(#55629,#55630,#55631,#55632,#55633,
#55634,#55635,#55636,#55637,#55638,#55639,#55640,#55641,#55642),(#55643,
#55644,#55645,#55646,#55647,#55648,#55649,#55650,#55651,#55652,#55653,#55654,
#55655,#55656),(#55657,#55658,#55659,#55660,#55661,#55662,#55663,#55664,
#55665,#55666,#55667,#55668,#55669,#55670),(#55671,#55672,#55673,#55674,
#55675,#55676,#55677,#55678,#55679,#55680,#55681,#55682,#55683,#55684),
(#55685,#55686,#55687,#55688,#55689,#55690,#55691,#55692,#55693,#55694,
#55695,#55696,#55697,#55698),(#55699,#55700,#55701,#55702,#55703,#55704,
#55705,#55706,#55707,#55708,#55709,#55710,#55711,#55712),(#55713,#55714,
#55715,#55716,#55717,#55718,#55719,#55720,#55721,#55722,#55723,#55724,#55725,
#55726),(#55727,#55728,#55729,#55730,#55731,#55732,#55733,#55734,#55735,
#55736,#55737,#55738,#55739,#55740),(#55741,#55742,#55743,#55744,#55745,
#55746,#55747,#55748,#55749,#55750,#55751,#55752,#55753,#55754),(#55755,
#55756,#55757,#55758,#55759,#55760,#55761,#55762,#55763,#55764,#55765,#55766,
#55767,#55768),(#55769,#55770,#55771,#55772,#55773,#55774,#55775,#55776,
#55777,#55778,#55779,#55780,#55781,#55782),(#55783,#55784,#55785,#55786,
#55787,#55788,#55789,#55790,#55791,#55792,#55793,#55794,#55795,#55796),
(#55797,#55798,#55799,#55800,#55801,#55802,#55803,#55804,#55805,#55806,
#55807,#55808,#55809,#55810),(#55811,#55812,#55813,#55814,#55815,#55816,
#55817,#55818,#55819,#55820,#55821,#55822,#55823,#55824),(#55825,#55826,
#55827,#55828,#55829,#55830,#55831,#55832,#55833,#55834,#55835,#55836,#55837,
#55838)),.UNSPECIFIED.,.F.,.F.,.F.,(4,1,1,1,1,1,1,1,1,1,1,1,1,1,1,1,1,1,
1,1,1,1,1,1,1,1,1,1,4),(4,2,2,2,2,2,4),(0.,0.0517952713240543,0.0690603617654058,
0.103590542648109,0.138120723530812,0.155385813972163,0.189915994854866,
0.276241447061623,0.345301808827029,0.414362170592435,0.431627261033786,
0.448892351475138,0.48342253235784,0.517952713240543,0.552482894123246,
0.587013075005949,0.621543255888652,0.690603617654058,0.699236162874733,
0.725133798536761,0.759663979419464,0.794194160302166,0.811459250743518,
0.820091795964194,0.824408068574531,0.8265662048797,0.828724341184869,0.897784702950275,
0.966845064715681),(0.0377143719395592,0.167070624995476,0.336553194126115,
0.499999999999991,0.663446805873868,0.832929375004528,0.962285628060022),
 .UNSPECIFIED.);
#236=B_SPLINE_SURFACE_WITH_KNOTS('',3,3,((#55896,#55897,#55898,#55899,#55900,
#55901,#55902,#55903,#55904,#55905,#55906,#55907,#55908,#55909),(#55910,
#55911,#55912,#55913,#55914,#55915,#55916,#55917,#55918,#55919,#55920,#55921,
#55922,#55923),(#55924,#55925,#55926,#55927,#55928,#55929,#55930,#55931,
#55932,#55933,#55934,#55935,#55936,#55937),(#55938,#55939,#55940,#55941,
#55942,#55943,#55944,#55945,#55946,#55947,#55948,#55949,#55950,#55951),
(#55952,#55953,#55954,#55955,#55956,#55957,#55958,#55959,#55960,#55961,
#55962,#55963,#55964,#55965),(#55966,#55967,#55968,#55969,#55970,#55971,
#55972,#55973,#55974,#55975,#55976,#55977,#55978,#55979),(#55980,#55981,
#55982,#55983,#55984,#55985,#55986,#55987,#55988,#55989,#55990,#55991,#55992,
#55993),(#55994,#55995,#55996,#55997,#55998,#55999,#56000,#56001,#56002,
#56003,#56004,#56005,#56006,#56007),(#56008,#56009,#56010,#56011,#56012,
#56013,#56014,#56015,#56016,#56017,#56018,#56019,#56020,#56021),(#56022,
#56023,#56024,#56025,#56026,#56027,#56028,#56029,#56030,#56031,#56032,#56033,
#56034,#56035),(#56036,#56037,#56038,#56039,#56040,#56041,#56042,#56043,
#56044,#56045,#56046,#56047,#56048,#56049),(#56050,#56051,#56052,#56053,
#56054,#56055,#56056,#56057,#56058,#56059,#56060,#56061,#56062,#56063),
(#56064,#56065,#56066,#56067,#56068,#56069,#56070,#56071,#56072,#56073,
#56074,#56075,#56076,#56077),(#56078,#56079,#56080,#56081,#56082,#56083,
#56084,#56085,#56086,#56087,#56088,#56089,#56090,#56091),(#56092,#56093,
#56094,#56095,#56096,#56097,#56098,#56099,#56100,#56101,#56102,#56103,#56104,
#56105),(#56106,#56107,#56108,#56109,#56110,#56111,#56112,#56113,#56114,
#56115,#56116,#56117,#56118,#56119),(#56120,#56121,#56122,#56123,#56124,
#56125,#56126,#56127,#56128,#56129,#56130,#56131,#56132,#56133),(#56134,
#56135,#56136,#56137,#56138,#56139,#56140,#56141,#56142,#56143,#56144,#56145,
#56146,#56147),(#56148,#56149,#56150,#56151,#56152,#56153,#56154,#56155,
#56156,#56157,#56158,#56159,#56160,#56161),(#56162,#56163,#56164,#56165,
#56166,#56167,#56168,#56169,#56170,#56171,#56172,#56173,#56174,#56175),
(#56176,#56177,#56178,#56179,#56180,#56181,#56182,#56183,#56184,#56185,
#56186,#56187,#56188,#56189),(#56190,#56191,#56192,#56193,#56194,#56195,
#56196,#56197,#56198,#56199,#56200,#56201,#56202,#56203),(#56204,#56205,
#56206,#56207,#56208,#56209,#56210,#56211,#56212,#56213,#56214,#56215,#56216,
#56217),(#56218,#56219,#56220,#56221,#56222,#56223,#56224,#56225,#56226,
#56227,#56228,#56229,#56230,#56231),(#56232,#56233,#56234,#56235,#56236,
#56237,#56238,#56239,#56240,#56241,#56242,#56243,#56244,#56245),(#56246,
#56247,#56248,#56249,#56250,#56251,#56252,#56253,#56254,#56255,#56256,#56257,
#56258,#56259),(#56260,#56261,#56262,#56263,#56264,#56265,#56266,#56267,
#56268,#56269,#56270,#56271,#56272,#56273),(#56274,#56275,#56276,#56277,
#56278,#56279,#56280,#56281,#56282,#56283,#56284,#56285,#56286,#56287),
(#56288,#56289,#56290,#56291,#56292,#56293,#56294,#56295,#56296,#56297,
#56298,#56299,#56300,#56301),(#56302,#56303,#56304,#56305,#56306,#56307,
#56308,#56309,#56310,#56311,#56312,#56313,#56314,#56315),(#56316,#56317,
#56318,#56319,#56320,#56321,#56322,#56323,#56324,#56325,#56326,#56327,#56328,
#56329),(#56330,#56331,#56332,#56333,#56334,#56335,#56336,#56337,#56338,
#56339,#56340,#56341,#56342,#56343),(#56344,#56345,#56346,#56347,#56348,
#56349,#56350,#56351,#56352,#56353,#56354,#56355,#56356,#56357),(#56358,
#56359,#56360,#56361,#56362,#56363,#56364,#56365,#56366,#56367,#56368,#56369,
#56370,#56371),(#56372,#56373,#56374,#56375,#56376,#56377,#56378,#56379,
#56380,#56381,#56382,#56383,#56384,#56385),(#56386,#56387,#56388,#56389,
#56390,#56391,#56392,#56393,#56394,#56395,#56396,#56397,#56398,#56399),
(#56400,#56401,#56402,#56403,#56404,#56405,#56406,#56407,#56408,#56409,
#56410,#56411,#56412,#56413),(#56414,#56415,#56416,#56417,#56418,#56419,
#56420,#56421,#56422,#56423,#56424,#56425,#56426,#56427),(#56428,#56429,
#56430,#56431,#56432,#56433,#56434,#56435,#56436,#56437,#56438,#56439,#56440,
#56441),(#56442,#56443,#56444,#56445,#56446,#56447,#56448,#56449,#56450,
#56451,#56452,#56453,#56454,#56455),(#56456,#56457,#56458,#56459,#56460,
#56461,#56462,#56463,#56464,#56465,#56466,#56467,#56468,#56469),(#56470,
#56471,#56472,#56473,#56474,#56475,#56476,#56477,#56478,#56479,#56480,#56481,
#56482,#56483),(#56484,#56485,#56486,#56487,#56488,#56489,#56490,#56491,
#56492,#56493,#56494,#56495,#56496,#56497)),.UNSPECIFIED.,.F.,.F.,.F.,(4,
1,1,1,1,1,1,1,1,1,1,1,1,1,1,1,1,1,1,1,1,1,1,1,1,1,1,1,1,1,1,1,1,1,1,1,1,
1,1,1,4),(4,2,2,2,2,2,4),(0.0331549352864066,0.067685116169035,0.102215297051663,
0.136745477934292,0.17127565881692,0.171815192893211,0.172354726969502,
0.173433795122084,0.175591931427249,0.179908204037577,0.184224476647906,
0.188540749258234,0.205805839699548,0.214438384920205,0.240336020582177,
0.274866201464805,0.309396382347433,0.37845674411269,0.412986924995318,
0.430252015436632,0.43888456065729,0.443200833267618,0.445358969572782,
0.446438037725365,0.447517105877947,0.482047286760575,0.516577467643203,
0.551107648525832,0.58563782940846,0.620168010291088,0.654698191173717,
0.689228372056345,0.723758552938973,0.79281891470423,0.827349095586858,
0.844614186028173,0.861879276469487,0.896409457352115,0.930939638234743,
0.948204728676058,1.),(0.0377143719407316,0.167070624995476,0.336553194126115,
0.499999999999991,0.663446805873868,0.832929375004528,0.962285628060079),
 .UNSPECIFIED.);
#237=B_SPLINE_SURFACE_WITH_KNOTS('',3,3,((#56560,#56561,#56562,#56563,#56564,
#56565,#56566,#56567,#56568,#56569,#56570,#56571,#56572,#56573),(#56574,
#56575,#56576,#56577,#56578,#56579,#56580,#56581,#56582,#56583,#56584,#56585,
#56586,#56587),(#56588,#56589,#56590,#56591,#56592,#56593,#56594,#56595,
#56596,#56597,#56598,#56599,#56600,#56601),(#56602,#56603,#56604,#56605,
#56606,#56607,#56608,#56609,#56610,#56611,#56612,#56613,#56614,#56615)),
 .UNSPECIFIED.,.F.,.F.,.F.,(4,4),(4,2,2,2,2,2,4),(0.,1.),(0.0377143719414212,
0.167070624995476,0.336553194126115,0.499999999999991,0.663446805873868,
0.832929375004528,0.962285628058582),.UNSPECIFIED.);
#238=B_SPLINE_SURFACE_WITH_KNOTS('',3,3,((#56630,#56631,#56632,#56633,#56634,
#56635,#56636,#56637,#56638,#56639,#56640,#56641,#56642,#56643),(#56644,
#56645,#56646,#56647,#56648,#56649,#56650,#56651,#56652,#56653,#56654,#56655,
#56656,#56657),(#56658,#56659,#56660,#56661,#56662,#56663,#56664,#56665,
#56666,#56667,#56668,#56669,#56670,#56671),(#56672,#56673,#56674,#56675,
#56676,#56677,#56678,#56679,#56680,#56681,#56682,#56683,#56684,#56685),
(#56686,#56687,#56688,#56689,#56690,#56691,#56692,#56693,#56694,#56695,
#56696,#56697,#56698,#56699),(#56700,#56701,#56702,#56703,#56704,#56705,
#56706,#56707,#56708,#56709,#56710,#56711,#56712,#56713),(#56714,#56715,
#56716,#56717,#56718,#56719,#56720,#56721,#56722,#56723,#56724,#56725,#56726,
#56727),(#56728,#56729,#56730,#56731,#56732,#56733,#56734,#56735,#56736,
#56737,#56738,#56739,#56740,#56741),(#56742,#56743,#56744,#56745,#56746,
#56747,#56748,#56749,#56750,#56751,#56752,#56753,#56754,#56755),(#56756,
#56757,#56758,#56759,#56760,#56761,#56762,#56763,#56764,#56765,#56766,#56767,
#56768,#56769),(#56770,#56771,#56772,#56773,#56774,#56775,#56776,#56777,
#56778,#56779,#56780,#56781,#56782,#56783),(#56784,#56785,#56786,#56787,
#56788,#56789,#56790,#56791,#56792,#56793,#56794,#56795,#56796,#56797),
(#56798,#56799,#56800,#56801,#56802,#56803,#56804,#56805,#56806,#56807,
#56808,#56809,#56810,#56811),(#56812,#56813,#56814,#56815,#56816,#56817,
#56818,#56819,#56820,#56821,#56822,#56823,#56824,#56825),(#56826,#56827,
#56828,#56829,#56830,#56831,#56832,#56833,#56834,#56835,#56836,#56837,#56838,
#56839),(#56840,#56841,#56842,#56843,#56844,#56845,#56846,#56847,#56848,
#56849,#56850,#56851,#56852,#56853),(#56854,#56855,#56856,#56857,#56858,
#56859,#56860,#56861,#56862,#56863,#56864,#56865,#56866,#56867),(#56868,
#56869,#56870,#56871,#56872,#56873,#56874,#56875,#56876,#56877,#56878,#56879,
#56880,#56881),(#56882,#56883,#56884,#56885,#56886,#56887,#56888,#56889,
#56890,#56891,#56892,#56893,#56894,#56895),(#56896,#56897,#56898,#56899,
#56900,#56901,#56902,#56903,#56904,#56905,#56906,#56907,#56908,#56909),
(#56910,#56911,#56912,#56913,#56914,#56915,#56916,#56917,#56918,#56919,
#56920,#56921,#56922,#56923),(#56924,#56925,#56926,#56927,#56928,#56929,
#56930,#56931,#56932,#56933,#56934,#56935,#56936,#56937),(#56938,#56939,
#56940,#56941,#56942,#56943,#56944,#56945,#56946,#56947,#56948,#56949,#56950,
#56951),(#56952,#56953,#56954,#56955,#56956,#56957,#56958,#56959,#56960,
#56961,#56962,#56963,#56964,#56965),(#56966,#56967,#56968,#56969,#56970,
#56971,#56972,#56973,#56974,#56975,#56976,#56977,#56978,#56979),(#56980,
#56981,#56982,#56983,#56984,#56985,#56986,#56987,#56988,#56989,#56990,#56991,
#56992,#56993),(#56994,#56995,#56996,#56997,#56998,#56999,#57000,#57001,
#57002,#57003,#57004,#57005,#57006,#57007),(#57008,#57009,#57010,#57011,
#57012,#57013,#57014,#57015,#57016,#57017,#57018,#57019,#57020,#57021),
(#57022,#57023,#57024,#57025,#57026,#57027,#57028,#57029,#57030,#57031,
#57032,#57033,#57034,#57035),(#57036,#57037,#57038,#57039,#57040,#57041,
#57042,#57043,#57044,#57045,#57046,#57047,#57048,#57049),(#57050,#57051,
#57052,#57053,#57054,#57055,#57056,#57057,#57058,#57059,#57060,#57061,#57062,
#57063),(#57064,#57065,#57066,#57067,#57068,#57069,#57070,#57071,#57072,
#57073,#57074,#57075,#57076,#57077),(#57078,#57079,#57080,#57081,#57082,
#57083,#57084,#57085,#57086,#57087,#57088,#57089,#57090,#57091),(#57092,
#57093,#57094,#57095,#57096,#57097,#57098,#57099,#57100,#57101,#57102,#57103,
#57104,#57105),(#57106,#57107,#57108,#57109,#57110,#57111,#57112,#57113,
#57114,#57115,#57116,#57117,#57118,#57119),(#57120,#57121,#57122,#57123,
#57124,#57125,#57126,#57127,#57128,#57129,#57130,#57131,#57132,#57133),
(#57134,#57135,#57136,#57137,#57138,#57139,#57140,#57141,#57142,#57143,
#57144,#57145,#57146,#57147),(#57148,#57149,#57150,#57151,#57152,#57153,
#57154,#57155,#57156,#57157,#57158,#57159,#57160,#57161),(#57162,#57163,
#57164,#57165,#57166,#57167,#57168,#57169,#57170,#57171,#57172,#57173,#57174,
#57175),(#57176,#57177,#57178,#57179,#57180,#57181,#57182,#57183,#57184,
#57185,#57186,#57187,#57188,#57189)),.UNSPECIFIED.,.F.,.F.,.F.,(4,1,1,1,
1,1,1,1,1,1,1,1,1,1,1,1,1,1,1,1,1,1,1,1,1,1,1,1,1,1,1,1,1,1,1,1,1,4),(4,
2,2,2,2,2,4),(0.,0.0517952713240546,0.0690603617654061,0.103590542648109,
0.138120723530812,0.172650904413515,0.207181085296218,0.276241447061624,
0.414362170592437,0.483422532357843,0.48773880496818,0.492055077578518,
0.500687622799194,0.517952713240546,0.552482894123249,0.621543255888655,
0.638808346330006,0.690603617654061,0.759663979419467,0.768296524640143,
0.772612797250481,0.776929069860818,0.785561615081494,0.79419416030217,
0.802826705522846,0.811459250743522,0.81361738704869,0.815775523353859,
0.820091795964197,0.824408068574535,0.82548713672712,0.826566204879704,
0.827645273032289,0.828184807108581,0.828454574146727,0.828724341184873,
0.897784702950279,0.966845064715685),(0.0377143719407368,0.167070624995476,
0.336553194126115,0.499999999999991,0.663446805873868,0.832929375004528,
0.96228562805882),.UNSPECIFIED.);
#239=B_SPLINE_SURFACE_WITH_KNOTS('',3,3,((#57243,#57244,#57245,#57246,#57247,
#57248,#57249,#57250,#57251,#57252,#57253,#57254,#57255,#57256),(#57257,
#57258,#57259,#57260,#57261,#57262,#57263,#57264,#57265,#57266,#57267,#57268,
#57269,#57270),(#57271,#57272,#57273,#57274,#57275,#57276,#57277,#57278,
#57279,#57280,#57281,#57282,#57283,#57284),(#57285,#57286,#57287,#57288,
#57289,#57290,#57291,#57292,#57293,#57294,#57295,#57296,#57297,#57298),
(#57299,#57300,#57301,#57302,#57303,#57304,#57305,#57306,#57307,#57308,
#57309,#57310,#57311,#57312),(#57313,#57314,#57315,#57316,#57317,#57318,
#57319,#57320,#57321,#57322,#57323,#57324,#57325,#57326),(#57327,#57328,
#57329,#57330,#57331,#57332,#57333,#57334,#57335,#57336,#57337,#57338,#57339,
#57340),(#57341,#57342,#57343,#57344,#57345,#57346,#57347,#57348,#57349,
#57350,#57351,#57352,#57353,#57354),(#57355,#57356,#57357,#57358,#57359,
#57360,#57361,#57362,#57363,#57364,#57365,#57366,#57367,#57368),(#57369,
#57370,#57371,#57372,#57373,#57374,#57375,#57376,#57377,#57378,#57379,#57380,
#57381,#57382),(#57383,#57384,#57385,#57386,#57387,#57388,#57389,#57390,
#57391,#57392,#57393,#57394,#57395,#57396),(#57397,#57398,#57399,#57400,
#57401,#57402,#57403,#57404,#57405,#57406,#57407,#57408,#57409,#57410),
(#57411,#57412,#57413,#57414,#57415,#57416,#57417,#57418,#57419,#57420,
#57421,#57422,#57423,#57424),(#57425,#57426,#57427,#57428,#57429,#57430,
#57431,#57432,#57433,#57434,#57435,#57436,#57437,#57438),(#57439,#57440,
#57441,#57442,#57443,#57444,#57445,#57446,#57447,#57448,#57449,#57450,#57451,
#57452),(#57453,#57454,#57455,#57456,#57457,#57458,#57459,#57460,#57461,
#57462,#57463,#57464,#57465,#57466),(#57467,#57468,#57469,#57470,#57471,
#57472,#57473,#57474,#57475,#57476,#57477,#57478,#57479,#57480),(#57481,
#57482,#57483,#57484,#57485,#57486,#57487,#57488,#57489,#57490,#57491,#57492,
#57493,#57494),(#57495,#57496,#57497,#57498,#57499,#57500,#57501,#57502,
#57503,#57504,#57505,#57506,#57507,#57508),(#57509,#57510,#57511,#57512,
#57513,#57514,#57515,#57516,#57517,#57518,#57519,#57520,#57521,#57522),
(#57523,#57524,#57525,#57526,#57527,#57528,#57529,#57530,#57531,#57532,
#57533,#57534,#57535,#57536),(#57537,#57538,#57539,#57540,#57541,#57542,
#57543,#57544,#57545,#57546,#57547,#57548,#57549,#57550),(#57551,#57552,
#57553,#57554,#57555,#57556,#57557,#57558,#57559,#57560,#57561,#57562,#57563,
#57564),(#57565,#57566,#57567,#57568,#57569,#57570,#57571,#57572,#57573,
#57574,#57575,#57576,#57577,#57578),(#57579,#57580,#57581,#57582,#57583,
#57584,#57585,#57586,#57587,#57588,#57589,#57590,#57591,#57592),(#57593,
#57594,#57595,#57596,#57597,#57598,#57599,#57600,#57601,#57602,#57603,#57604,
#57605,#57606),(#57607,#57608,#57609,#57610,#57611,#57612,#57613,#57614,
#57615,#57616,#57617,#57618,#57619,#57620),(#57621,#57622,#57623,#57624,
#57625,#57626,#57627,#57628,#57629,#57630,#57631,#57632,#57633,#57634),
(#57635,#57636,#57637,#57638,#57639,#57640,#57641,#57642,#57643,#57644,
#57645,#57646,#57647,#57648),(#57649,#57650,#57651,#57652,#57653,#57654,
#57655,#57656,#57657,#57658,#57659,#57660,#57661,#57662),(#57663,#57664,
#57665,#57666,#57667,#57668,#57669,#57670,#57671,#57672,#57673,#57674,#57675,
#57676),(#57677,#57678,#57679,#57680,#57681,#57682,#57683,#57684,#57685,
#57686,#57687,#57688,#57689,#57690),(#57691,#57692,#57693,#57694,#57695,
#57696,#57697,#57698,#57699,#57700,#57701,#57702,#57703,#57704),(#57705,
#57706,#57707,#57708,#57709,#57710,#57711,#57712,#57713,#57714,#57715,#57716,
#57717,#57718),(#57719,#57720,#57721,#57722,#57723,#57724,#57725,#57726,
#57727,#57728,#57729,#57730,#57731,#57732),(#57733,#57734,#57735,#57736,
#57737,#57738,#57739,#57740,#57741,#57742,#57743,#57744,#57745,#57746)),
 .UNSPECIFIED.,.F.,.F.,.F.,(4,1,1,1,1,1,1,1,1,1,1,1,1,1,1,1,1,1,1,1,1,1,
1,1,1,1,1,1,1,1,1,1,1,4),(4,2,2,2,2,2,4),(0.0331549352864083,0.0676851161690366,
0.102215297051665,0.171275658816921,0.172354726969504,0.173433795122086,
0.174512863274668,0.17559193142725,0.179908204037579,0.188540749258236,
0.197173294478893,0.20580583969955,0.223070930140864,0.240336020582178,
0.274866201464806,0.309396382347435,0.378456744112691,0.412986924995319,
0.447517105877948,0.482047286760576,0.516577467643204,0.551107648525832,
0.568372738967147,0.585637829408461,0.654698191173717,0.70649346249766,
0.723758552938974,0.79281891470423,0.827349095586859,0.861879276469487,
0.896409457352115,0.930939638234743,0.948204728676058,1.),(0.037714371941404,
0.167070624995476,0.336553194126115,0.499999999999991,0.663446805873868,
0.832929375004528,0.962285628059334),.UNSPECIFIED.);
#240=B_SPLINE_SURFACE_WITH_KNOTS('',3,3,((#57811,#57812,#57813,#57814,#57815,
#57816,#57817,#57818,#57819,#57820,#57821,#57822,#57823,#57824),(#57825,
#57826,#57827,#57828,#57829,#57830,#57831,#57832,#57833,#57834,#57835,#57836,
#57837,#57838),(#57839,#57840,#57841,#57842,#57843,#57844,#57845,#57846,
#57847,#57848,#57849,#57850,#57851,#57852),(#57853,#57854,#57855,#57856,
#57857,#57858,#57859,#57860,#57861,#57862,#57863,#57864,#57865,#57866)),
 .UNSPECIFIED.,.F.,.F.,.F.,(4,4),(4,2,2,2,2,2,4),(0.,1.),(0.0377143719414212,
0.167070624995476,0.336553194126115,0.499999999999991,0.663446805873868,
0.832929375004528,0.962285628058582),.UNSPECIFIED.);
#241=B_SPLINE_SURFACE_WITH_KNOTS('',3,3,((#57881,#57882,#57883,#57884,#57885,
#57886,#57887,#57888,#57889,#57890,#57891,#57892,#57893,#57894),(#57895,
#57896,#57897,#57898,#57899,#57900,#57901,#57902,#57903,#57904,#57905,#57906,
#57907,#57908),(#57909,#57910,#57911,#57912,#57913,#57914,#57915,#57916,
#57917,#57918,#57919,#57920,#57921,#57922),(#57923,#57924,#57925,#57926,
#57927,#57928,#57929,#57930,#57931,#57932,#57933,#57934,#57935,#57936),
(#57937,#57938,#57939,#57940,#57941,#57942,#57943,#57944,#57945,#57946,
#57947,#57948,#57949,#57950),(#57951,#57952,#57953,#57954,#57955,#57956,
#57957,#57958,#57959,#57960,#57961,#57962,#57963,#57964),(#57965,#57966,
#57967,#57968,#57969,#57970,#57971,#57972,#57973,#57974,#57975,#57976,#57977,
#57978),(#57979,#57980,#57981,#57982,#57983,#57984,#57985,#57986,#57987,
#57988,#57989,#57990,#57991,#57992),(#57993,#57994,#57995,#57996,#57997,
#57998,#57999,#58000,#58001,#58002,#58003,#58004,#58005,#58006),(#58007,
#58008,#58009,#58010,#58011,#58012,#58013,#58014,#58015,#58016,#58017,#58018,
#58019,#58020),(#58021,#58022,#58023,#58024,#58025,#58026,#58027,#58028,
#58029,#58030,#58031,#58032,#58033,#58034),(#58035,#58036,#58037,#58038,
#58039,#58040,#58041,#58042,#58043,#58044,#58045,#58046,#58047,#58048),
(#58049,#58050,#58051,#58052,#58053,#58054,#58055,#58056,#58057,#58058,
#58059,#58060,#58061,#58062),(#58063,#58064,#58065,#58066,#58067,#58068,
#58069,#58070,#58071,#58072,#58073,#58074,#58075,#58076),(#58077,#58078,
#58079,#58080,#58081,#58082,#58083,#58084,#58085,#58086,#58087,#58088,#58089,
#58090),(#58091,#58092,#58093,#58094,#58095,#58096,#58097,#58098,#58099,
#58100,#58101,#58102,#58103,#58104),(#58105,#58106,#58107,#58108,#58109,
#58110,#58111,#58112,#58113,#58114,#58115,#58116,#58117,#58118),(#58119,
#58120,#58121,#58122,#58123,#58124,#58125,#58126,#58127,#58128,#58129,#58130,
#58131,#58132),(#58133,#58134,#58135,#58136,#58137,#58138,#58139,#58140,
#58141,#58142,#58143,#58144,#58145,#58146),(#58147,#58148,#58149,#58150,
#58151,#58152,#58153,#58154,#58155,#58156,#58157,#58158,#58159,#58160),
(#58161,#58162,#58163,#58164,#58165,#58166,#58167,#58168,#58169,#58170,
#58171,#58172,#58173,#58174),(#58175,#58176,#58177,#58178,#58179,#58180,
#58181,#58182,#58183,#58184,#58185,#58186,#58187,#58188),(#58189,#58190,
#58191,#58192,#58193,#58194,#58195,#58196,#58197,#58198,#58199,#58200,#58201,
#58202),(#58203,#58204,#58205,#58206,#58207,#58208,#58209,#58210,#58211,
#58212,#58213,#58214,#58215,#58216),(#58217,#58218,#58219,#58220,#58221,
#58222,#58223,#58224,#58225,#58226,#58227,#58228,#58229,#58230),(#58231,
#58232,#58233,#58234,#58235,#58236,#58237,#58238,#58239,#58240,#58241,#58242,
#58243,#58244)),.UNSPECIFIED.,.F.,.F.,.F.,(4,1,1,1,1,1,1,1,1,1,1,1,1,1,
1,1,1,1,1,1,1,1,1,4),(4,2,2,2,2,2,4),(0.,0.0517952713240544,0.0690603617654058,
0.103590542648109,0.138120723530812,0.189915994854866,0.24171126617892,
0.276241447061623,0.310771627944326,0.345301808827029,0.379831989709732,
0.414362170592435,0.448892351475138,0.483422532357841,0.552482894123247,
0.587013075005949,0.690603617654058,0.759663979419464,0.76829652464014,
0.776929069860816,0.794194160302167,0.863254522067573,0.897784702950276,
0.966845064715682),(0.0377143719413297,0.167070624995476,0.336553194126115,
0.499999999999991,0.663446805873868,0.832929375004528,0.962285628058621),
 .UNSPECIFIED.);
#242=B_SPLINE_SURFACE_WITH_KNOTS('',3,3,((#58300,#58301,#58302,#58303,#58304,
#58305,#58306,#58307,#58308,#58309,#58310,#58311,#58312,#58313),(#58314,
#58315,#58316,#58317,#58318,#58319,#58320,#58321,#58322,#58323,#58324,#58325,
#58326,#58327),(#58328,#58329,#58330,#58331,#58332,#58333,#58334,#58335,
#58336,#58337,#58338,#58339,#58340,#58341),(#58342,#58343,#58344,#58345,
#58346,#58347,#58348,#58349,#58350,#58351,#58352,#58353,#58354,#58355),
(#58356,#58357,#58358,#58359,#58360,#58361,#58362,#58363,#58364,#58365,
#58366,#58367,#58368,#58369),(#58370,#58371,#58372,#58373,#58374,#58375,
#58376,#58377,#58378,#58379,#58380,#58381,#58382,#58383),(#58384,#58385,
#58386,#58387,#58388,#58389,#58390,#58391,#58392,#58393,#58394,#58395,#58396,
#58397),(#58398,#58399,#58400,#58401,#58402,#58403,#58404,#58405,#58406,
#58407,#58408,#58409,#58410,#58411),(#58412,#58413,#58414,#58415,#58416,
#58417,#58418,#58419,#58420,#58421,#58422,#58423,#58424,#58425),(#58426,
#58427,#58428,#58429,#58430,#58431,#58432,#58433,#58434,#58435,#58436,#58437,
#58438,#58439),(#58440,#58441,#58442,#58443,#58444,#58445,#58446,#58447,
#58448,#58449,#58450,#58451,#58452,#58453),(#58454,#58455,#58456,#58457,
#58458,#58459,#58460,#58461,#58462,#58463,#58464,#58465,#58466,#58467),
(#58468,#58469,#58470,#58471,#58472,#58473,#58474,#58475,#58476,#58477,
#58478,#58479,#58480,#58481),(#58482,#58483,#58484,#58485,#58486,#58487,
#58488,#58489,#58490,#58491,#58492,#58493,#58494,#58495),(#58496,#58497,
#58498,#58499,#58500,#58501,#58502,#58503,#58504,#58505,#58506,#58507,#58508,
#58509),(#58510,#58511,#58512,#58513,#58514,#58515,#58516,#58517,#58518,
#58519,#58520,#58521,#58522,#58523),(#58524,#58525,#58526,#58527,#58528,
#58529,#58530,#58531,#58532,#58533,#58534,#58535,#58536,#58537),(#58538,
#58539,#58540,#58541,#58542,#58543,#58544,#58545,#58546,#58547,#58548,#58549,
#58550,#58551),(#58552,#58553,#58554,#58555,#58556,#58557,#58558,#58559,
#58560,#58561,#58562,#58563,#58564,#58565),(#58566,#58567,#58568,#58569,
#58570,#58571,#58572,#58573,#58574,#58575,#58576,#58577,#58578,#58579),
(#58580,#58581,#58582,#58583,#58584,#58585,#58586,#58587,#58588,#58589,
#58590,#58591,#58592,#58593),(#58594,#58595,#58596,#58597,#58598,#58599,
#58600,#58601,#58602,#58603,#58604,#58605,#58606,#58607),(#58608,#58609,
#58610,#58611,#58612,#58613,#58614,#58615,#58616,#58617,#58618,#58619,#58620,
#58621),(#58622,#58623,#58624,#58625,#58626,#58627,#58628,#58629,#58630,
#58631,#58632,#58633,#58634,#58635),(#58636,#58637,#58638,#58639,#58640,
#58641,#58642,#58643,#58644,#58645,#58646,#58647,#58648,#58649),(#58650,
#58651,#58652,#58653,#58654,#58655,#58656,#58657,#58658,#58659,#58660,#58661,
#58662,#58663),(#58664,#58665,#58666,#58667,#58668,#58669,#58670,#58671,
#58672,#58673,#58674,#58675,#58676,#58677),(#58678,#58679,#58680,#58681,
#58682,#58683,#58684,#58685,#58686,#58687,#58688,#58689,#58690,#58691),
(#58692,#58693,#58694,#58695,#58696,#58697,#58698,#58699,#58700,#58701,
#58702,#58703,#58704,#58705),(#58706,#58707,#58708,#58709,#58710,#58711,
#58712,#58713,#58714,#58715,#58716,#58717,#58718,#58719),(#58720,#58721,
#58722,#58723,#58724,#58725,#58726,#58727,#58728,#58729,#58730,#58731,#58732,
#58733),(#58734,#58735,#58736,#58737,#58738,#58739,#58740,#58741,#58742,
#58743,#58744,#58745,#58746,#58747),(#58748,#58749,#58750,#58751,#58752,
#58753,#58754,#58755,#58756,#58757,#58758,#58759,#58760,#58761),(#58762,
#58763,#58764,#58765,#58766,#58767,#58768,#58769,#58770,#58771,#58772,#58773,
#58774,#58775),(#58776,#58777,#58778,#58779,#58780,#58781,#58782,#58783,
#58784,#58785,#58786,#58787,#58788,#58789),(#58790,#58791,#58792,#58793,
#58794,#58795,#58796,#58797,#58798,#58799,#58800,#58801,#58802,#58803)),
 .UNSPECIFIED.,.F.,.F.,.F.,(4,1,1,1,1,1,1,1,1,1,1,1,1,1,1,1,1,1,1,1,1,1,
1,1,1,1,1,1,1,1,1,1,1,4),(4,2,2,2,2,2,4),(0.0331549352864083,0.0676851161690366,
0.102215297051665,0.171275658816921,0.172354726969504,0.173433795122086,
0.174512863274668,0.17559193142725,0.179908204037578,0.188540749258236,
0.197173294478893,0.20580583969955,0.223070930140864,0.240336020582178,
0.274866201464806,0.309396382347434,0.378456744112691,0.412986924995319,
0.447517105877948,0.482047286760576,0.516577467643204,0.551107648525832,
0.568372738967146,0.585637829408461,0.654698191173717,0.70649346249766,
0.723758552938974,0.79281891470423,0.827349095586859,0.861879276469487,
0.896409457352115,0.930939638234743,0.948204728676058,1.),(0.0377143719412435,
0.167070624995476,0.336553194126115,0.499999999999991,0.663446805873868,
0.832929375004528,0.962285628059578),.UNSPECIFIED.);
#243=B_SPLINE_SURFACE_WITH_KNOTS('',3,3,((#58868,#58869,#58870,#58871,#58872,
#58873,#58874,#58875,#58876,#58877,#58878,#58879,#58880,#58881),(#58882,
#58883,#58884,#58885,#58886,#58887,#58888,#58889,#58890,#58891,#58892,#58893,
#58894,#58895),(#58896,#58897,#58898,#58899,#58900,#58901,#58902,#58903,
#58904,#58905,#58906,#58907,#58908,#58909),(#58910,#58911,#58912,#58913,
#58914,#58915,#58916,#58917,#58918,#58919,#58920,#58921,#58922,#58923)),
 .UNSPECIFIED.,.F.,.F.,.F.,(4,4),(4,2,2,2,2,2,4),(0.,1.),(0.037714371941421,
0.167070624995476,0.336553194126115,0.499999999999991,0.663446805873868,
0.832929375004528,0.962285628058582),.UNSPECIFIED.);
#244=B_SPLINE_SURFACE_WITH_KNOTS('',3,3,((#58938,#58939,#58940,#58941,#58942,
#58943,#58944,#58945,#58946,#58947,#58948,#58949,#58950,#58951),(#58952,
#58953,#58954,#58955,#58956,#58957,#58958,#58959,#58960,#58961,#58962,#58963,
#58964,#58965),(#58966,#58967,#58968,#58969,#58970,#58971,#58972,#58973,
#58974,#58975,#58976,#58977,#58978,#58979),(#58980,#58981,#58982,#58983,
#58984,#58985,#58986,#58987,#58988,#58989,#58990,#58991,#58992,#58993),
(#58994,#58995,#58996,#58997,#58998,#58999,#59000,#59001,#59002,#59003,
#59004,#59005,#59006,#59007),(#59008,#59009,#59010,#59011,#59012,#59013,
#59014,#59015,#59016,#59017,#59018,#59019,#59020,#59021),(#59022,#59023,
#59024,#59025,#59026,#59027,#59028,#59029,#59030,#59031,#59032,#59033,#59034,
#59035),(#59036,#59037,#59038,#59039,#59040,#59041,#59042,#59043,#59044,
#59045,#59046,#59047,#59048,#59049),(#59050,#59051,#59052,#59053,#59054,
#59055,#59056,#59057,#59058,#59059,#59060,#59061,#59062,#59063),(#59064,
#59065,#59066,#59067,#59068,#59069,#59070,#59071,#59072,#59073,#59074,#59075,
#59076,#59077),(#59078,#59079,#59080,#59081,#59082,#59083,#59084,#59085,
#59086,#59087,#59088,#59089,#59090,#59091),(#59092,#59093,#59094,#59095,
#59096,#59097,#59098,#59099,#59100,#59101,#59102,#59103,#59104,#59105),
(#59106,#59107,#59108,#59109,#59110,#59111,#59112,#59113,#59114,#59115,
#59116,#59117,#59118,#59119),(#59120,#59121,#59122,#59123,#59124,#59125,
#59126,#59127,#59128,#59129,#59130,#59131,#59132,#59133),(#59134,#59135,
#59136,#59137,#59138,#59139,#59140,#59141,#59142,#59143,#59144,#59145,#59146,
#59147),(#59148,#59149,#59150,#59151,#59152,#59153,#59154,#59155,#59156,
#59157,#59158,#59159,#59160,#59161),(#59162,#59163,#59164,#59165,#59166,
#59167,#59168,#59169,#59170,#59171,#59172,#59173,#59174,#59175),(#59176,
#59177,#59178,#59179,#59180,#59181,#59182,#59183,#59184,#59185,#59186,#59187,
#59188,#59189),(#59190,#59191,#59192,#59193,#59194,#59195,#59196,#59197,
#59198,#59199,#59200,#59201,#59202,#59203),(#59204,#59205,#59206,#59207,
#59208,#59209,#59210,#59211,#59212,#59213,#59214,#59215,#59216,#59217),
(#59218,#59219,#59220,#59221,#59222,#59223,#59224,#59225,#59226,#59227,
#59228,#59229,#59230,#59231),(#59232,#59233,#59234,#59235,#59236,#59237,
#59238,#59239,#59240,#59241,#59242,#59243,#59244,#59245),(#59246,#59247,
#59248,#59249,#59250,#59251,#59252,#59253,#59254,#59255,#59256,#59257,#59258,
#59259),(#59260,#59261,#59262,#59263,#59264,#59265,#59266,#59267,#59268,
#59269,#59270,#59271,#59272,#59273),(#59274,#59275,#59276,#59277,#59278,
#59279,#59280,#59281,#59282,#59283,#59284,#59285,#59286,#59287),(#59288,
#59289,#59290,#59291,#59292,#59293,#59294,#59295,#59296,#59297,#59298,#59299,
#59300,#59301),(#59302,#59303,#59304,#59305,#59306,#59307,#59308,#59309,
#59310,#59311,#59312,#59313,#59314,#59315),(#59316,#59317,#59318,#59319,
#59320,#59321,#59322,#59323,#59324,#59325,#59326,#59327,#59328,#59329),
(#59330,#59331,#59332,#59333,#59334,#59335,#59336,#59337,#59338,#59339,
#59340,#59341,#59342,#59343),(#59344,#59345,#59346,#59347,#59348,#59349,
#59350,#59351,#59352,#59353,#59354,#59355,#59356,#59357),(#59358,#59359,
#59360,#59361,#59362,#59363,#59364,#59365,#59366,#59367,#59368,#59369,#59370,
#59371),(#59372,#59373,#59374,#59375,#59376,#59377,#59378,#59379,#59380,
#59381,#59382,#59383,#59384,#59385),(#59386,#59387,#59388,#59389,#59390,
#59391,#59392,#59393,#59394,#59395,#59396,#59397,#59398,#59399),(#59400,
#59401,#59402,#59403,#59404,#59405,#59406,#59407,#59408,#59409,#59410,#59411,
#59412,#59413),(#59414,#59415,#59416,#59417,#59418,#59419,#59420,#59421,
#59422,#59423,#59424,#59425,#59426,#59427),(#59428,#59429,#59430,#59431,
#59432,#59433,#59434,#59435,#59436,#59437,#59438,#59439,#59440,#59441),
(#59442,#59443,#59444,#59445,#59446,#59447,#59448,#59449,#59450,#59451,
#59452,#59453,#59454,#59455),(#59456,#59457,#59458,#59459,#59460,#59461,
#59462,#59463,#59464,#59465,#59466,#59467,#59468,#59469),(#59470,#59471,
#59472,#59473,#59474,#59475,#59476,#59477,#59478,#59479,#59480,#59481,#59482,
#59483),(#59484,#59485,#59486,#59487,#59488,#59489,#59490,#59491,#59492,
#59493,#59494,#59495,#59496,#59497),(#59498,#59499,#59500,#59501,#59502,
#59503,#59504,#59505,#59506,#59507,#59508,#59509,#59510,#59511),(#59512,
#59513,#59514,#59515,#59516,#59517,#59518,#59519,#59520,#59521,#59522,#59523,
#59524,#59525),(#59526,#59527,#59528,#59529,#59530,#59531,#59532,#59533,
#59534,#59535,#59536,#59537,#59538,#59539),(#59540,#59541,#59542,#59543,
#59544,#59545,#59546,#59547,#59548,#59549,#59550,#59551,#59552,#59553),
(#59554,#59555,#59556,#59557,#59558,#59559,#59560,#59561,#59562,#59563,
#59564,#59565,#59566,#59567),(#59568,#59569,#59570,#59571,#59572,#59573,
#59574,#59575,#59576,#59577,#59578,#59579,#59580,#59581),(#59582,#59583,
#59584,#59585,#59586,#59587,#59588,#59589,#59590,#59591,#59592,#59593,#59594,
#59595)),.UNSPECIFIED.,.F.,.F.,.F.,(4,1,1,1,1,1,1,1,1,1,1,1,1,1,1,1,1,1,
1,1,1,1,1,1,1,1,1,1,1,1,1,1,1,1,1,1,1,1,1,1,1,1,1,1,4),(4,2,2,2,2,2,4),
(0.,0.0517952713240546,0.0690603617654062,0.103590542648109,0.138120723530812,
0.155385813972164,0.172650904413515,0.207181085296219,0.276241447061625,
0.345301808827031,0.379831989709734,0.414362170592437,0.422994715813113,
0.431627261033789,0.44889235147514,0.466157441916492,0.483422532357843,
0.55248289412325,0.621543255888656,0.656073436771359,0.690603617654062,
0.699236162874738,0.707868708095414,0.725133798536765,0.759663979419468,
0.763980252029806,0.768296524640144,0.77692906986082,0.785561615081495,
0.794194160302171,0.802826705522847,0.811459250743523,0.820091795964199,
0.822249932269367,0.823329000421952,0.824408068574537,0.826566204879705,
0.82764527303229,0.827915040070436,0.828184807108582,0.828454574146728,
0.828724341184874,0.897784702950281,0.932314883832984,0.966845064715687),
(0.0377143719413837,0.167070624995476,0.336553194126115,0.499999999999991,
0.663446805873868,0.832929375004528,0.962285628058658),.UNSPECIFIED.);
#245=B_SPLINE_SURFACE_WITH_KNOTS('',3,3,((#59653,#59654,#59655,#59656,#59657,
#59658,#59659,#59660,#59661,#59662,#59663,#59664,#59665,#59666),(#59667,
#59668,#59669,#59670,#59671,#59672,#59673,#59674,#59675,#59676,#59677,#59678,
#59679,#59680),(#59681,#59682,#59683,#59684,#59685,#59686,#59687,#59688,
#59689,#59690,#59691,#59692,#59693,#59694),(#59695,#59696,#59697,#59698,
#59699,#59700,#59701,#59702,#59703,#59704,#59705,#59706,#59707,#59708),
(#59709,#59710,#59711,#59712,#59713,#59714,#59715,#59716,#59717,#59718,
#59719,#59720,#59721,#59722),(#59723,#59724,#59725,#59726,#59727,#59728,
#59729,#59730,#59731,#59732,#59733,#59734,#59735,#59736),(#59737,#59738,
#59739,#59740,#59741,#59742,#59743,#59744,#59745,#59746,#59747,#59748,#59749,
#59750),(#59751,#59752,#59753,#59754,#59755,#59756,#59757,#59758,#59759,
#59760,#59761,#59762,#59763,#59764),(#59765,#59766,#59767,#59768,#59769,
#59770,#59771,#59772,#59773,#59774,#59775,#59776,#59777,#59778),(#59779,
#59780,#59781,#59782,#59783,#59784,#59785,#59786,#59787,#59788,#59789,#59790,
#59791,#59792),(#59793,#59794,#59795,#59796,#59797,#59798,#59799,#59800,
#59801,#59802,#59803,#59804,#59805,#59806),(#59807,#59808,#59809,#59810,
#59811,#59812,#59813,#59814,#59815,#59816,#59817,#59818,#59819,#59820),
(#59821,#59822,#59823,#59824,#59825,#59826,#59827,#59828,#59829,#59830,
#59831,#59832,#59833,#59834),(#59835,#59836,#59837,#59838,#59839,#59840,
#59841,#59842,#59843,#59844,#59845,#59846,#59847,#59848),(#59849,#59850,
#59851,#59852,#59853,#59854,#59855,#59856,#59857,#59858,#59859,#59860,#59861,
#59862),(#59863,#59864,#59865,#59866,#59867,#59868,#59869,#59870,#59871,
#59872,#59873,#59874,#59875,#59876),(#59877,#59878,#59879,#59880,#59881,
#59882,#59883,#59884,#59885,#59886,#59887,#59888,#59889,#59890),(#59891,
#59892,#59893,#59894,#59895,#59896,#59897,#59898,#59899,#59900,#59901,#59902,
#59903,#59904),(#59905,#59906,#59907,#59908,#59909,#59910,#59911,#59912,
#59913,#59914,#59915,#59916,#59917,#59918),(#59919,#59920,#59921,#59922,
#59923,#59924,#59925,#59926,#59927,#59928,#59929,#59930,#59931,#59932),
(#59933,#59934,#59935,#59936,#59937,#59938,#59939,#59940,#59941,#59942,
#59943,#59944,#59945,#59946),(#59947,#59948,#59949,#59950,#59951,#59952,
#59953,#59954,#59955,#59956,#59957,#59958,#59959,#59960),(#59961,#59962,
#59963,#59964,#59965,#59966,#59967,#59968,#59969,#59970,#59971,#59972,#59973,
#59974),(#59975,#59976,#59977,#59978,#59979,#59980,#59981,#59982,#59983,
#59984,#59985,#59986,#59987,#59988),(#59989,#59990,#59991,#59992,#59993,
#59994,#59995,#59996,#59997,#59998,#59999,#60000,#60001,#60002),(#60003,
#60004,#60005,#60006,#60007,#60008,#60009,#60010,#60011,#60012,#60013,#60014,
#60015,#60016),(#60017,#60018,#60019,#60020,#60021,#60022,#60023,#60024,
#60025,#60026,#60027,#60028,#60029,#60030),(#60031,#60032,#60033,#60034,
#60035,#60036,#60037,#60038,#60039,#60040,#60041,#60042,#60043,#60044),
(#60045,#60046,#60047,#60048,#60049,#60050,#60051,#60052,#60053,#60054,
#60055,#60056,#60057,#60058),(#60059,#60060,#60061,#60062,#60063,#60064,
#60065,#60066,#60067,#60068,#60069,#60070,#60071,#60072),(#60073,#60074,
#60075,#60076,#60077,#60078,#60079,#60080,#60081,#60082,#60083,#60084,#60085,
#60086),(#60087,#60088,#60089,#60090,#60091,#60092,#60093,#60094,#60095,
#60096,#60097,#60098,#60099,#60100),(#60101,#60102,#60103,#60104,#60105,
#60106,#60107,#60108,#60109,#60110,#60111,#60112,#60113,#60114),(#60115,
#60116,#60117,#60118,#60119,#60120,#60121,#60122,#60123,#60124,#60125,#60126,
#60127,#60128),(#60129,#60130,#60131,#60132,#60133,#60134,#60135,#60136,
#60137,#60138,#60139,#60140,#60141,#60142),(#60143,#60144,#60145,#60146,
#60147,#60148,#60149,#60150,#60151,#60152,#60153,#60154,#60155,#60156),
(#60157,#60158,#60159,#60160,#60161,#60162,#60163,#60164,#60165,#60166,
#60167,#60168,#60169,#60170),(#60171,#60172,#60173,#60174,#60175,#60176,
#60177,#60178,#60179,#60180,#60181,#60182,#60183,#60184),(#60185,#60186,
#60187,#60188,#60189,#60190,#60191,#60192,#60193,#60194,#60195,#60196,#60197,
#60198),(#60199,#60200,#60201,#60202,#60203,#60204,#60205,#60206,#60207,
#60208,#60209,#60210,#60211,#60212)),.UNSPECIFIED.,.F.,.F.,.F.,(4,1,1,1,
1,1,1,1,1,1,1,1,1,1,1,1,1,1,1,1,1,1,1,1,1,1,1,1,1,1,1,1,1,1,1,1,1,4),(4,
2,2,2,2,2,4),(0.0331549352864082,0.102215297051665,0.171275658816921,0.171815192893212,
0.172354726969503,0.172894261045795,0.173433795122086,0.17559193142725,
0.179908204037578,0.182066340342743,0.184224476647907,0.188540749258235,
0.197173294478893,0.201489567089221,0.20580583969955,0.214438384920207,
0.223070930140864,0.227387202751192,0.231703475361521,0.240336020582178,
0.309396382347434,0.361191653671377,0.378456744112691,0.447517105877948,
0.482047286760576,0.49931237720189,0.507944922422547,0.512261195032876,
0.516577467643204,0.585637829408461,0.723758552938974,0.79281891470423,
0.827349095586859,0.861879276469487,0.896409457352115,0.930939638234743,
0.948204728676058,1.),(0.0377143719407819,0.167070624995476,0.336553194126115,
0.499999999999991,0.663446805873868,0.832929375004528,0.962285628058724),
 .UNSPECIFIED.);
#246=B_SPLINE_SURFACE_WITH_KNOTS('',3,3,((#60271,#60272,#60273,#60274,#60275,
#60276,#60277,#60278,#60279,#60280,#60281,#60282,#60283,#60284),(#60285,
#60286,#60287,#60288,#60289,#60290,#60291,#60292,#60293,#60294,#60295,#60296,
#60297,#60298),(#60299,#60300,#60301,#60302,#60303,#60304,#60305,#60306,
#60307,#60308,#60309,#60310,#60311,#60312),(#60313,#60314,#60315,#60316,
#60317,#60318,#60319,#60320,#60321,#60322,#60323,#60324,#60325,#60326)),
 .UNSPECIFIED.,.F.,.F.,.F.,(4,4),(4,2,2,2,2,2,4),(0.,1.),(0.0377143719414212,
0.167070624995476,0.336553194126115,0.499999999999991,0.663446805873868,
0.832929375004528,0.962285628058582),.UNSPECIFIED.);
#247=B_SPLINE_SURFACE_WITH_KNOTS('',3,3,((#60341,#60342,#60343,#60344,#60345,
#60346,#60347,#60348,#60349,#60350,#60351,#60352,#60353,#60354),(#60355,
#60356,#60357,#60358,#60359,#60360,#60361,#60362,#60363,#60364,#60365,#60366,
#60367,#60368),(#60369,#60370,#60371,#60372,#60373,#60374,#60375,#60376,
#60377,#60378,#60379,#60380,#60381,#60382),(#60383,#60384,#60385,#60386,
#60387,#60388,#60389,#60390,#60391,#60392,#60393,#60394,#60395,#60396),
(#60397,#60398,#60399,#60400,#60401,#60402,#60403,#60404,#60405,#60406,
#60407,#60408,#60409,#60410),(#60411,#60412,#60413,#60414,#60415,#60416,
#60417,#60418,#60419,#60420,#60421,#60422,#60423,#60424),(#60425,#60426,
#60427,#60428,#60429,#60430,#60431,#60432,#60433,#60434,#60435,#60436,#60437,
#60438),(#60439,#60440,#60441,#60442,#60443,#60444,#60445,#60446,#60447,
#60448,#60449,#60450,#60451,#60452),(#60453,#60454,#60455,#60456,#60457,
#60458,#60459,#60460,#60461,#60462,#60463,#60464,#60465,#60466),(#60467,
#60468,#60469,#60470,#60471,#60472,#60473,#60474,#60475,#60476,#60477,#60478,
#60479,#60480),(#60481,#60482,#60483,#60484,#60485,#60486,#60487,#60488,
#60489,#60490,#60491,#60492,#60493,#60494),(#60495,#60496,#60497,#60498,
#60499,#60500,#60501,#60502,#60503,#60504,#60505,#60506,#60507,#60508),
(#60509,#60510,#60511,#60512,#60513,#60514,#60515,#60516,#60517,#60518,
#60519,#60520,#60521,#60522),(#60523,#60524,#60525,#60526,#60527,#60528,
#60529,#60530,#60531,#60532,#60533,#60534,#60535,#60536),(#60537,#60538,
#60539,#60540,#60541,#60542,#60543,#60544,#60545,#60546,#60547,#60548,#60549,
#60550),(#60551,#60552,#60553,#60554,#60555,#60556,#60557,#60558,#60559,
#60560,#60561,#60562,#60563,#60564),(#60565,#60566,#60567,#60568,#60569,
#60570,#60571,#60572,#60573,#60574,#60575,#60576,#60577,#60578),(#60579,
#60580,#60581,#60582,#60583,#60584,#60585,#60586,#60587,#60588,#60589,#60590,
#60591,#60592),(#60593,#60594,#60595,#60596,#60597,#60598,#60599,#60600,
#60601,#60602,#60603,#60604,#60605,#60606),(#60607,#60608,#60609,#60610,
#60611,#60612,#60613,#60614,#60615,#60616,#60617,#60618,#60619,#60620),
(#60621,#60622,#60623,#60624,#60625,#60626,#60627,#60628,#60629,#60630,
#60631,#60632,#60633,#60634),(#60635,#60636,#60637,#60638,#60639,#60640,
#60641,#60642,#60643,#60644,#60645,#60646,#60647,#60648),(#60649,#60650,
#60651,#60652,#60653,#60654,#60655,#60656,#60657,#60658,#60659,#60660,#60661,
#60662),(#60663,#60664,#60665,#60666,#60667,#60668,#60669,#60670,#60671,
#60672,#60673,#60674,#60675,#60676),(#60677,#60678,#60679,#60680,#60681,
#60682,#60683,#60684,#60685,#60686,#60687,#60688,#60689,#60690),(#60691,
#60692,#60693,#60694,#60695,#60696,#60697,#60698,#60699,#60700,#60701,#60702,
#60703,#60704)),.UNSPECIFIED.,.F.,.F.,.F.,(4,1,1,1,1,1,1,1,1,1,1,1,1,1,
1,1,1,1,1,1,1,1,1,4),(4,2,2,2,2,2,4),(0.,0.0517952713240545,0.069060361765406,
0.103590542648109,0.138120723530812,0.189915994854866,0.241711266178921,
0.276241447061624,0.310771627944327,0.34530180882703,0.362566899268381,
0.379831989709733,0.414362170592436,0.552482894123248,0.587013075005951,
0.621543255888654,0.69060361765406,0.759663979419466,0.768296524640142,
0.776929069860817,0.794194160302169,0.863254522067575,0.897784702950278,
0.966845064715684),(0.0377143719414028,0.167070624995476,0.336553194126115,
0.499999999999991,0.663446805873868,0.832929375004528,0.962285628059076),
 .UNSPECIFIED.);
#248=B_SPLINE_SURFACE_WITH_KNOTS('',3,3,((#60773,#60774,#60775,#60776,#60777,
#60778,#60779,#60780,#60781,#60782,#60783,#60784,#60785,#60786),(#60787,
#60788,#60789,#60790,#60791,#60792,#60793,#60794,#60795,#60796,#60797,#60798,
#60799,#60800),(#60801,#60802,#60803,#60804,#60805,#60806,#60807,#60808,
#60809,#60810,#60811,#60812,#60813,#60814),(#60815,#60816,#60817,#60818,
#60819,#60820,#60821,#60822,#60823,#60824,#60825,#60826,#60827,#60828),
(#60829,#60830,#60831,#60832,#60833,#60834,#60835,#60836,#60837,#60838,
#60839,#60840,#60841,#60842),(#60843,#60844,#60845,#60846,#60847,#60848,
#60849,#60850,#60851,#60852,#60853,#60854,#60855,#60856),(#60857,#60858,
#60859,#60860,#60861,#60862,#60863,#60864,#60865,#60866,#60867,#60868,#60869,
#60870),(#60871,#60872,#60873,#60874,#60875,#60876,#60877,#60878,#60879,
#60880,#60881,#60882,#60883,#60884),(#60885,#60886,#60887,#60888,#60889,
#60890,#60891,#60892,#60893,#60894,#60895,#60896,#60897,#60898),(#60899,
#60900,#60901,#60902,#60903,#60904,#60905,#60906,#60907,#60908,#60909,#60910,
#60911,#60912),(#60913,#60914,#60915,#60916,#60917,#60918,#60919,#60920,
#60921,#60922,#60923,#60924,#60925,#60926),(#60927,#60928,#60929,#60930,
#60931,#60932,#60933,#60934,#60935,#60936,#60937,#60938,#60939,#60940),
(#60941,#60942,#60943,#60944,#60945,#60946,#60947,#60948,#60949,#60950,
#60951,#60952,#60953,#60954),(#60955,#60956,#60957,#60958,#60959,#60960,
#60961,#60962,#60963,#60964,#60965,#60966,#60967,#60968),(#60969,#60970,
#60971,#60972,#60973,#60974,#60975,#60976,#60977,#60978,#60979,#60980,#60981,
#60982),(#60983,#60984,#60985,#60986,#60987,#60988,#60989,#60990,#60991,
#60992,#60993,#60994,#60995,#60996),(#60997,#60998,#60999,#61000,#61001,
#61002,#61003,#61004,#61005,#61006,#61007,#61008,#61009,#61010),(#61011,
#61012,#61013,#61014,#61015,#61016,#61017,#61018,#61019,#61020,#61021,#61022,
#61023,#61024),(#61025,#61026,#61027,#61028,#61029,#61030,#61031,#61032,
#61033,#61034,#61035,#61036,#61037,#61038),(#61039,#61040,#61041,#61042,
#61043,#61044,#61045,#61046,#61047,#61048,#61049,#61050,#61051,#61052),
(#61053,#61054,#61055,#61056,#61057,#61058,#61059,#61060,#61061,#61062,
#61063,#61064,#61065,#61066),(#61067,#61068,#61069,#61070,#61071,#61072,
#61073,#61074,#61075,#61076,#61077,#61078,#61079,#61080),(#61081,#61082,
#61083,#61084,#61085,#61086,#61087,#61088,#61089,#61090,#61091,#61092,#61093,
#61094),(#61095,#61096,#61097,#61098,#61099,#61100,#61101,#61102,#61103,
#61104,#61105,#61106,#61107,#61108),(#61109,#61110,#61111,#61112,#61113,
#61114,#61115,#61116,#61117,#61118,#61119,#61120,#61121,#61122),(#61123,
#61124,#61125,#61126,#61127,#61128,#61129,#61130,#61131,#61132,#61133,#61134,
#61135,#61136),(#61137,#61138,#61139,#61140,#61141,#61142,#61143,#61144,
#61145,#61146,#61147,#61148,#61149,#61150),(#61151,#61152,#61153,#61154,
#61155,#61156,#61157,#61158,#61159,#61160,#61161,#61162,#61163,#61164),
(#61165,#61166,#61167,#61168,#61169,#61170,#61171,#61172,#61173,#61174,
#61175,#61176,#61177,#61178),(#61179,#61180,#61181,#61182,#61183,#61184,
#61185,#61186,#61187,#61188,#61189,#61190,#61191,#61192),(#61193,#61194,
#61195,#61196,#61197,#61198,#61199,#61200,#61201,#61202,#61203,#61204,#61205,
#61206),(#61207,#61208,#61209,#61210,#61211,#61212,#61213,#61214,#61215,
#61216,#61217,#61218,#61219,#61220),(#61221,#61222,#61223,#61224,#61225,
#61226,#61227,#61228,#61229,#61230,#61231,#61232,#61233,#61234),(#61235,
#61236,#61237,#61238,#61239,#61240,#61241,#61242,#61243,#61244,#61245,#61246,
#61247,#61248),(#61249,#61250,#61251,#61252,#61253,#61254,#61255,#61256,
#61257,#61258,#61259,#61260,#61261,#61262),(#61263,#61264,#61265,#61266,
#61267,#61268,#61269,#61270,#61271,#61272,#61273,#61274,#61275,#61276)),
 .UNSPECIFIED.,.F.,.F.,.F.,(4,1,1,1,1,1,1,1,1,1,1,1,1,1,1,1,1,1,1,1,1,1,
1,1,1,1,1,1,1,1,1,1,1,4),(4,2,2,2,2,2,4),(0.0331549352864088,0.102215297051665,
0.171275658816922,0.171815192893213,0.172354726969504,0.172894261045795,
0.173433795122086,0.17559193142725,0.179908204037579,0.182066340342743,
0.188540749258236,0.197173294478893,0.20580583969955,0.214438384920207,
0.223070930140864,0.240336020582178,0.274866201464807,0.292131291906121,
0.309396382347435,0.378456744112691,0.41298692499532,0.430252015436634,
0.447517105877948,0.516577467643204,0.585637829408461,0.654698191173717,
0.689228372056346,0.723758552938974,0.810084005145544,0.861879276469487,
0.896409457352115,0.930939638234743,0.948204728676058,1.),(0.0377143719413782,
0.167070624995476,0.336553194126115,0.499999999999991,0.663446805873868,
0.832929375004528,0.962285628059578),.UNSPECIFIED.);
#249=B_SPLINE_SURFACE_WITH_KNOTS('',3,3,((#61328,#61329,#61330,#61331,#61332,
#61333,#61334,#61335,#61336,#61337,#61338,#61339,#61340,#61341),(#61342,
#61343,#61344,#61345,#61346,#61347,#61348,#61349,#61350,#61351,#61352,#61353,
#61354,#61355),(#61356,#61357,#61358,#61359,#61360,#61361,#61362,#61363,
#61364,#61365,#61366,#61367,#61368,#61369),(#61370,#61371,#61372,#61373,
#61374,#61375,#61376,#61377,#61378,#61379,#61380,#61381,#61382,#61383)),
 .UNSPECIFIED.,.F.,.F.,.F.,(4,4),(4,2,2,2,2,2,4),(0.,1.),(0.037714371941421,
0.167070624995476,0.336553194126115,0.499999999999991,0.663446805873868,
0.832929375004528,0.962285628058582),.UNSPECIFIED.);
#250=B_SPLINE_SURFACE_WITH_KNOTS('',3,3,((#61398,#61399,#61400,#61401,#61402,
#61403,#61404,#61405,#61406,#61407,#61408,#61409,#61410,#61411),(#61412,
#61413,#61414,#61415,#61416,#61417,#61418,#61419,#61420,#61421,#61422,#61423,
#61424,#61425),(#61426,#61427,#61428,#61429,#61430,#61431,#61432,#61433,
#61434,#61435,#61436,#61437,#61438,#61439),(#61440,#61441,#61442,#61443,
#61444,#61445,#61446,#61447,#61448,#61449,#61450,#61451,#61452,#61453),
(#61454,#61455,#61456,#61457,#61458,#61459,#61460,#61461,#61462,#61463,
#61464,#61465,#61466,#61467),(#61468,#61469,#61470,#61471,#61472,#61473,
#61474,#61475,#61476,#61477,#61478,#61479,#61480,#61481),(#61482,#61483,
#61484,#61485,#61486,#61487,#61488,#61489,#61490,#61491,#61492,#61493,#61494,
#61495),(#61496,#61497,#61498,#61499,#61500,#61501,#61502,#61503,#61504,
#61505,#61506,#61507,#61508,#61509),(#61510,#61511,#61512,#61513,#61514,
#61515,#61516,#61517,#61518,#61519,#61520,#61521,#61522,#61523),(#61524,
#61525,#61526,#61527,#61528,#61529,#61530,#61531,#61532,#61533,#61534,#61535,
#61536,#61537),(#61538,#61539,#61540,#61541,#61542,#61543,#61544,#61545,
#61546,#61547,#61548,#61549,#61550,#61551),(#61552,#61553,#61554,#61555,
#61556,#61557,#61558,#61559,#61560,#61561,#61562,#61563,#61564,#61565),
(#61566,#61567,#61568,#61569,#61570,#61571,#61572,#61573,#61574,#61575,
#61576,#61577,#61578,#61579),(#61580,#61581,#61582,#61583,#61584,#61585,
#61586,#61587,#61588,#61589,#61590,#61591,#61592,#61593),(#61594,#61595,
#61596,#61597,#61598,#61599,#61600,#61601,#61602,#61603,#61604,#61605,#61606,
#61607),(#61608,#61609,#61610,#61611,#61612,#61613,#61614,#61615,#61616,
#61617,#61618,#61619,#61620,#61621),(#61622,#61623,#61624,#61625,#61626,
#61627,#61628,#61629,#61630,#61631,#61632,#61633,#61634,#61635),(#61636,
#61637,#61638,#61639,#61640,#61641,#61642,#61643,#61644,#61645,#61646,#61647,
#61648,#61649),(#61650,#61651,#61652,#61653,#61654,#61655,#61656,#61657,
#61658,#61659,#61660,#61661,#61662,#61663),(#61664,#61665,#61666,#61667,
#61668,#61669,#61670,#61671,#61672,#61673,#61674,#61675,#61676,#61677),
(#61678,#61679,#61680,#61681,#61682,#61683,#61684,#61685,#61686,#61687,
#61688,#61689,#61690,#61691),(#61692,#61693,#61694,#61695,#61696,#61697,
#61698,#61699,#61700,#61701,#61702,#61703,#61704,#61705),(#61706,#61707,
#61708,#61709,#61710,#61711,#61712,#61713,#61714,#61715,#61716,#61717,#61718,
#61719),(#61720,#61721,#61722,#61723,#61724,#61725,#61726,#61727,#61728,
#61729,#61730,#61731,#61732,#61733),(#61734,#61735,#61736,#61737,#61738,
#61739,#61740,#61741,#61742,#61743,#61744,#61745,#61746,#61747),(#61748,
#61749,#61750,#61751,#61752,#61753,#61754,#61755,#61756,#61757,#61758,#61759,
#61760,#61761),(#61762,#61763,#61764,#61765,#61766,#61767,#61768,#61769,
#61770,#61771,#61772,#61773,#61774,#61775),(#61776,#61777,#61778,#61779,
#61780,#61781,#61782,#61783,#61784,#61785,#61786,#61787,#61788,#61789),
(#61790,#61791,#61792,#61793,#61794,#61795,#61796,#61797,#61798,#61799,
#61800,#61801,#61802,#61803),(#61804,#61805,#61806,#61807,#61808,#61809,
#61810,#61811,#61812,#61813,#61814,#61815,#61816,#61817),(#61818,#61819,
#61820,#61821,#61822,#61823,#61824,#61825,#61826,#61827,#61828,#61829,#61830,
#61831),(#61832,#61833,#61834,#61835,#61836,#61837,#61838,#61839,#61840,
#61841,#61842,#61843,#61844,#61845),(#61846,#61847,#61848,#61849,#61850,
#61851,#61852,#61853,#61854,#61855,#61856,#61857,#61858,#61859),(#61860,
#61861,#61862,#61863,#61864,#61865,#61866,#61867,#61868,#61869,#61870,#61871,
#61872,#61873),(#61874,#61875,#61876,#61877,#61878,#61879,#61880,#61881,
#61882,#61883,#61884,#61885,#61886,#61887),(#61888,#61889,#61890,#61891,
#61892,#61893,#61894,#61895,#61896,#61897,#61898,#61899,#61900,#61901),
(#61902,#61903,#61904,#61905,#61906,#61907,#61908,#61909,#61910,#61911,
#61912,#61913,#61914,#61915),(#61916,#61917,#61918,#61919,#61920,#61921,
#61922,#61923,#61924,#61925,#61926,#61927,#61928,#61929),(#61930,#61931,
#61932,#61933,#61934,#61935,#61936,#61937,#61938,#61939,#61940,#61941,#61942,
#61943),(#61944,#61945,#61946,#61947,#61948,#61949,#61950,#61951,#61952,
#61953,#61954,#61955,#61956,#61957),(#61958,#61959,#61960,#61961,#61962,
#61963,#61964,#61965,#61966,#61967,#61968,#61969,#61970,#61971),(#61972,
#61973,#61974,#61975,#61976,#61977,#61978,#61979,#61980,#61981,#61982,#61983,
#61984,#61985),(#61986,#61987,#61988,#61989,#61990,#61991,#61992,#61993,
#61994,#61995,#61996,#61997,#61998,#61999),(#62000,#62001,#62002,#62003,
#62004,#62005,#62006,#62007,#62008,#62009,#62010,#62011,#62012,#62013),
(#62014,#62015,#62016,#62017,#62018,#62019,#62020,#62021,#62022,#62023,
#62024,#62025,#62026,#62027),(#62028,#62029,#62030,#62031,#62032,#62033,
#62034,#62035,#62036,#62037,#62038,#62039,#62040,#62041)),.UNSPECIFIED.,
 .F.,.F.,.F.,(4,1,1,1,1,1,1,1,1,1,1,1,1,1,1,1,1,1,1,1,1,1,1,1,1,1,1,1,1,
1,1,1,1,1,1,1,1,1,1,1,1,1,1,4),(4,2,2,2,2,2,4),(0.,0.034530180882703,0.0517952713240545,
0.069060361765406,0.103590542648109,0.138120723530812,0.146753268751488,
0.155385813972164,0.172650904413515,0.207181085296218,0.276241447061624,
0.310771627944327,0.34530180882703,0.379831989709733,0.414362170592436,
0.448892351475139,0.483422532357842,0.500687622799194,0.552482894123248,
0.5697479845646,0.621543255888654,0.656073436771357,0.69060361765406,0.707868708095412,
0.716501253316088,0.725133798536763,0.759663979419467,0.776929069860818,
0.785561615081494,0.79419416030217,0.802826705522845,0.811459250743521,
0.820091795964197,0.824408068574535,0.825487136727119,0.826566204879704,
0.827645273032288,0.82818480710858,0.828454574146726,0.828724341184873,
0.863254522067576,0.897784702950279,0.932314883832982,0.966845064715685),
(0.0377143719413179,0.167070624995476,0.336553194126115,0.499999999999991,
0.663446805873868,0.832929375004528,0.962285628060395),.UNSPECIFIED.);
#251=B_SPLINE_SURFACE_WITH_KNOTS('',3,3,((#62109,#62110,#62111,#62112,#62113,
#62114,#62115,#62116,#62117,#62118,#62119,#62120,#62121,#62122),(#62123,
#62124,#62125,#62126,#62127,#62128,#62129,#62130,#62131,#62132,#62133,#62134,
#62135,#62136),(#62137,#62138,#62139,#62140,#62141,#62142,#62143,#62144,
#62145,#62146,#62147,#62148,#62149,#62150),(#62151,#62152,#62153,#62154,
#62155,#62156,#62157,#62158,#62159,#62160,#62161,#62162,#62163,#62164),
(#62165,#62166,#62167,#62168,#62169,#62170,#62171,#62172,#62173,#62174,
#62175,#62176,#62177,#62178),(#62179,#62180,#62181,#62182,#62183,#62184,
#62185,#62186,#62187,#62188,#62189,#62190,#62191,#62192),(#62193,#62194,
#62195,#62196,#62197,#62198,#62199,#62200,#62201,#62202,#62203,#62204,#62205,
#62206),(#62207,#62208,#62209,#62210,#62211,#62212,#62213,#62214,#62215,
#62216,#62217,#62218,#62219,#62220),(#62221,#62222,#62223,#62224,#62225,
#62226,#62227,#62228,#62229,#62230,#62231,#62232,#62233,#62234),(#62235,
#62236,#62237,#62238,#62239,#62240,#62241,#62242,#62243,#62244,#62245,#62246,
#62247,#62248),(#62249,#62250,#62251,#62252,#62253,#62254,#62255,#62256,
#62257,#62258,#62259,#62260,#62261,#62262),(#62263,#62264,#62265,#62266,
#62267,#62268,#62269,#62270,#62271,#62272,#62273,#62274,#62275,#62276),
(#62277,#62278,#62279,#62280,#62281,#62282,#62283,#62284,#62285,#62286,
#62287,#62288,#62289,#62290),(#62291,#62292,#62293,#62294,#62295,#62296,
#62297,#62298,#62299,#62300,#62301,#62302,#62303,#62304),(#62305,#62306,
#62307,#62308,#62309,#62310,#62311,#62312,#62313,#62314,#62315,#62316,#62317,
#62318),(#62319,#62320,#62321,#62322,#62323,#62324,#62325,#62326,#62327,
#62328,#62329,#62330,#62331,#62332),(#62333,#62334,#62335,#62336,#62337,
#62338,#62339,#62340,#62341,#62342,#62343,#62344,#62345,#62346),(#62347,
#62348,#62349,#62350,#62351,#62352,#62353,#62354,#62355,#62356,#62357,#62358,
#62359,#62360),(#62361,#62362,#62363,#62364,#62365,#62366,#62367,#62368,
#62369,#62370,#62371,#62372,#62373,#62374),(#62375,#62376,#62377,#62378,
#62379,#62380,#62381,#62382,#62383,#62384,#62385,#62386,#62387,#62388),
(#62389,#62390,#62391,#62392,#62393,#62394,#62395,#62396,#62397,#62398,
#62399,#62400,#62401,#62402),(#62403,#62404,#62405,#62406,#62407,#62408,
#62409,#62410,#62411,#62412,#62413,#62414,#62415,#62416),(#62417,#62418,
#62419,#62420,#62421,#62422,#62423,#62424,#62425,#62426,#62427,#62428,#62429,
#62430),(#62431,#62432,#62433,#62434,#62435,#62436,#62437,#62438,#62439,
#62440,#62441,#62442,#62443,#62444),(#62445,#62446,#62447,#62448,#62449,
#62450,#62451,#62452,#62453,#62454,#62455,#62456,#62457,#62458),(#62459,
#62460,#62461,#62462,#62463,#62464,#62465,#62466,#62467,#62468,#62469,#62470,
#62471,#62472),(#62473,#62474,#62475,#62476,#62477,#62478,#62479,#62480,
#62481,#62482,#62483,#62484,#62485,#62486),(#62487,#62488,#62489,#62490,
#62491,#62492,#62493,#62494,#62495,#62496,#62497,#62498,#62499,#62500),
(#62501,#62502,#62503,#62504,#62505,#62506,#62507,#62508,#62509,#62510,
#62511,#62512,#62513,#62514),(#62515,#62516,#62517,#62518,#62519,#62520,
#62521,#62522,#62523,#62524,#62525,#62526,#62527,#62528)),.UNSPECIFIED.,
 .F.,.F.,.F.,(4,1,1,1,1,1,1,1,1,1,1,1,1,1,1,1,1,1,1,1,1,1,1,1,1,1,1,4),
(4,2,2,2,2,2,4),(0.0331549352864031,0.10221529705166,0.171275658816917,
0.173433795122081,0.175591931427245,0.179908204037574,0.188540749258231,
0.205805839699545,0.214438384920203,0.22307093014086,0.240336020582174,
0.309396382347431,0.395721834554002,0.447517105877945,0.482047286760573,
0.499312377201887,0.516577467643202,0.55110764852583,0.585637829408458,
0.620168010291087,0.723758552938972,0.792818914704229,0.827349095586858,
0.861879276469486,0.896409457352115,0.930939638234743,0.948204728676057,
1.),(0.0377143719413312,0.167070624995476,0.336553194126115,0.499999999999991,
0.663446805873868,0.832929375004528,0.962285628058676),.UNSPECIFIED.);
#252=B_SPLINE_SURFACE_WITH_KNOTS('',3,3,((#62573,#62574,#62575,#62576,#62577,
#62578,#62579,#62580,#62581,#62582,#62583,#62584,#62585,#62586),(#62587,
#62588,#62589,#62590,#62591,#62592,#62593,#62594,#62595,#62596,#62597,#62598,
#62599,#62600),(#62601,#62602,#62603,#62604,#62605,#62606,#62607,#62608,
#62609,#62610,#62611,#62612,#62613,#62614),(#62615,#62616,#62617,#62618,
#62619,#62620,#62621,#62622,#62623,#62624,#62625,#62626,#62627,#62628)),
 .UNSPECIFIED.,.F.,.F.,.F.,(4,4),(4,2,2,2,2,2,4),(0.,1.),(0.037714371941421,
0.167070624995476,0.336553194126115,0.499999999999991,0.663446805873868,
0.832929375004528,0.962285628058582),.UNSPECIFIED.);
#253=B_SPLINE_SURFACE_WITH_KNOTS('',3,3,((#62643,#62644,#62645,#62646,#62647,
#62648,#62649,#62650,#62651,#62652,#62653,#62654,#62655,#62656),(#62657,
#62658,#62659,#62660,#62661,#62662,#62663,#62664,#62665,#62666,#62667,#62668,
#62669,#62670),(#62671,#62672,#62673,#62674,#62675,#62676,#62677,#62678,
#62679,#62680,#62681,#62682,#62683,#62684),(#62685,#62686,#62687,#62688,
#62689,#62690,#62691,#62692,#62693,#62694,#62695,#62696,#62697,#62698),
(#62699,#62700,#62701,#62702,#62703,#62704,#62705,#62706,#62707,#62708,
#62709,#62710,#62711,#62712),(#62713,#62714,#62715,#62716,#62717,#62718,
#62719,#62720,#62721,#62722,#62723,#62724,#62725,#62726),(#62727,#62728,
#62729,#62730,#62731,#62732,#62733,#62734,#62735,#62736,#62737,#62738,#62739,
#62740),(#62741,#62742,#62743,#62744,#62745,#62746,#62747,#62748,#62749,
#62750,#62751,#62752,#62753,#62754),(#62755,#62756,#62757,#62758,#62759,
#62760,#62761,#62762,#62763,#62764,#62765,#62766,#62767,#62768),(#62769,
#62770,#62771,#62772,#62773,#62774,#62775,#62776,#62777,#62778,#62779,#62780,
#62781,#62782),(#62783,#62784,#62785,#62786,#62787,#62788,#62789,#62790,
#62791,#62792,#62793,#62794,#62795,#62796),(#62797,#62798,#62799,#62800,
#62801,#62802,#62803,#62804,#62805,#62806,#62807,#62808,#62809,#62810),
(#62811,#62812,#62813,#62814,#62815,#62816,#62817,#62818,#62819,#62820,
#62821,#62822,#62823,#62824),(#62825,#62826,#62827,#62828,#62829,#62830,
#62831,#62832,#62833,#62834,#62835,#62836,#62837,#62838),(#62839,#62840,
#62841,#62842,#62843,#62844,#62845,#62846,#62847,#62848,#62849,#62850,#62851,
#62852),(#62853,#62854,#62855,#62856,#62857,#62858,#62859,#62860,#62861,
#62862,#62863,#62864,#62865,#62866),(#62867,#62868,#62869,#62870,#62871,
#62872,#62873,#62874,#62875,#62876,#62877,#62878,#62879,#62880),(#62881,
#62882,#62883,#62884,#62885,#62886,#62887,#62888,#62889,#62890,#62891,#62892,
#62893,#62894),(#62895,#62896,#62897,#62898,#62899,#62900,#62901,#62902,
#62903,#62904,#62905,#62906,#62907,#62908),(#62909,#62910,#62911,#62912,
#62913,#62914,#62915,#62916,#62917,#62918,#62919,#62920,#62921,#62922),
(#62923,#62924,#62925,#62926,#62927,#62928,#62929,#62930,#62931,#62932,
#62933,#62934,#62935,#62936),(#62937,#62938,#62939,#62940,#62941,#62942,
#62943,#62944,#62945,#62946,#62947,#62948,#62949,#62950),(#62951,#62952,
#62953,#62954,#62955,#62956,#62957,#62958,#62959,#62960,#62961,#62962,#62963,
#62964),(#62965,#62966,#62967,#62968,#62969,#62970,#62971,#62972,#62973,
#62974,#62975,#62976,#62977,#62978),(#62979,#62980,#62981,#62982,#62983,
#62984,#62985,#62986,#62987,#62988,#62989,#62990,#62991,#62992),(#62993,
#62994,#62995,#62996,#62997,#62998,#62999,#63000,#63001,#63002,#63003,#63004,
#63005,#63006),(#63007,#63008,#63009,#63010,#63011,#63012,#63013,#63014,
#63015,#63016,#63017,#63018,#63019,#63020),(#63021,#63022,#63023,#63024,
#63025,#63026,#63027,#63028,#63029,#63030,#63031,#63032,#63033,#63034),
(#63035,#63036,#63037,#63038,#63039,#63040,#63041,#63042,#63043,#63044,
#63045,#63046,#63047,#63048),(#63049,#63050,#63051,#63052,#63053,#63054,
#63055,#63056,#63057,#63058,#63059,#63060,#63061,#63062),(#63063,#63064,
#63065,#63066,#63067,#63068,#63069,#63070,#63071,#63072,#63073,#63074,#63075,
#63076)),.UNSPECIFIED.,.F.,.F.,.F.,(4,1,1,1,1,1,1,1,1,1,1,1,1,1,1,1,1,1,
1,1,1,1,1,1,1,1,1,1,4),(4,2,2,2,2,2,4),(0.,0.0517952713240546,0.0690603617654061,
0.103590542648109,0.138120723530812,0.155385813972164,0.189915994854867,
0.276241447061624,0.34530180882703,0.414362170592436,0.431627261033788,
0.448892351475139,0.483422532357842,0.517952713240545,0.552482894123249,
0.587013075005952,0.621543255888655,0.690603617654061,0.699236162874737,
0.725133798536764,0.759663979419467,0.79419416030217,0.811459250743521,
0.820091795964197,0.824408068574535,0.826566204879704,0.828724341184873,
0.897784702950279,0.966845064715685),(0.0377143719404219,0.167070624995476,
0.336553194126115,0.499999999999991,0.663446805873868,0.832929375004528,
0.962285628061492),.UNSPECIFIED.);
#291=SHAPE_REPRESENTATION_RELATIONSHIP('SRR','None',#86506,#309);
#309=ADVANCED_BREP_SHAPE_REPRESENTATION('',(#345),#86415);
#327=STYLED_ITEM('',(#86605),#345);
#345=MANIFOLD_SOLID_BREP('Body1',#15617);
#418=B_SPLINE_CURVE_WITH_KNOTS('',3,(#26828,#26829,#26830,#26831,#26832,
#26833,#26834,#26835,#26836,#26837,#26838,#26839,#26840,#26841,#26842,#26843,
#26844,#26845,#26846),.UNSPECIFIED.,.F.,.F.,(4,1,1,1,1,1,1,1,1,1,1,1,1,
1,1,1,4),(0.,0.0325793930090435,0.0434391906787246,0.0651587860180869,0.0868783813574492,
0.0923082801922898,0.0977381790271304,0.119457774366493,0.173756762714898,
0.217195953393623,0.238915548732985,0.260635144072348,0.28235473941171,
0.293214537081391,0.304074334751072,0.347513525429797,0.350797960844041),
 .UNSPECIFIED.);
#419=B_SPLINE_CURVE_WITH_KNOTS('',3,(#26850,#26851,#26852,#26853,#26854,
#26855,#26856,#26857,#26858,#26859,#26860,#26861,#26862,#26863,#26864,#26865,
#26866,#26867,#26868),.UNSPECIFIED.,.F.,.F.,(4,1,1,1,1,1,1,1,1,1,1,1,1,
1,1,1,4),(0.351264129075342,0.354255847547048,0.372150346521233,0.390044845495419,
0.407939344469604,0.416886593956697,0.42583384344379,0.46162284139216,0.488464589853438,
0.497411839340531,0.533200837288902,0.551095336263087,0.568989835237273,
0.586884334211458,0.604778833185643,0.613726082672736,0.640567831134014),
 .UNSPECIFIED.);
#420=B_SPLINE_CURVE_WITH_KNOTS('',3,(#26872,#26873,#26874,#26875,#26876,
#26877,#26878,#26879,#26880,#26881,#26882,#26883,#26884,#26885,#26886,#26887,
#26888,#26889),.UNSPECIFIED.,.F.,.F.,(4,1,1,1,1,1,1,1,1,1,1,1,1,1,1,4),
(0.,0.0325793930343183,0.0434391907124244,0.0651587860686366,0.0868783814248488,
0.0977381791029549,0.108597976781061,0.130317572137273,0.173756762849698,
0.217195953562122,0.238915548918334,0.260635144274546,0.282354739630759,
0.304074334986971,0.347513525699395,0.350847233099761),.UNSPECIFIED.);
#421=B_SPLINE_CURVE_WITH_KNOTS('',3,(#26893,#26894,#26895,#26896,#26897,
#26898,#26899,#26900,#26901,#26902,#26903,#26904,#26905,#26906,#26907,#26908,
#26909,#26910,#26911),.UNSPECIFIED.,.F.,.F.,(4,1,1,1,1,1,1,1,1,1,1,1,1,
1,1,1,4),(0.351264249492161,0.354255847579901,0.372150346750411,0.39004484592092,
0.40793934509143,0.416886594676685,0.42583384426194,0.46162284260296,0.488464591358724,
0.497411840943979,0.533200839284999,0.551095338455509,0.568989837626019,
0.586884336796529,0.604778835967039,0.613726085552294,0.640567834308058),
 .UNSPECIFIED.);
#422=B_SPLINE_CURVE_WITH_KNOTS('',3,(#26915,#26916,#26917,#26918,#26919,
#26920,#26921,#26922,#26923,#26924,#26925,#26926,#26927,#26928,#26929,#26930,
#26931,#26932,#26933,#26934,#26935),.UNSPECIFIED.,.F.,.F.,(4,1,1,1,1,1,
1,1,1,1,1,1,1,1,1,1,1,1,4),(0.,0.0325793930168542,0.0434391906891389,0.0651587860337083,
0.0868783813782778,0.0977381790505625,0.108597976722847,0.130317572067417,
0.173756762756556,0.217195953445694,0.238915548790264,0.260635144134833,
0.266065042970976,0.271494941807118,0.282354739479403,0.293214537151688,
0.304074334823972,0.347513525513111,0.350819403961439),.UNSPECIFIED.);
#423=B_SPLINE_CURVE_WITH_KNOTS('',3,(#26939,#26940,#26941,#26942,#26943,
#26944,#26945,#26946,#26947,#26948,#26949,#26950,#26951,#26952,#26953,#26954,
#26955,#26956),.UNSPECIFIED.,.F.,.F.,(4,1,1,1,1,1,1,1,1,1,1,1,1,1,1,4),
(0.351261425313741,0.35425584743808,0.372150345761052,0.381097594922539,
0.385571219503282,0.387808031793653,0.390044844084025,0.425833840729969,
0.497411834021859,0.533200830667804,0.551095328990776,0.568989827313749,
0.586884325636721,0.604778823959693,0.61372607312118,0.640567820605638),
 .UNSPECIFIED.);
#424=B_SPLINE_CURVE_WITH_KNOTS('',3,(#26960,#26961,#26962,#26963,#26964,
#26965,#26966,#26967,#26968,#26969,#26970,#26971,#26972,#26973,#26974,#26975,
#26976,#26977,#26978),.UNSPECIFIED.,.F.,.F.,(4,1,1,1,1,1,1,1,1,1,1,1,1,
1,1,1,4),(0.,0.0325793930229512,0.0434391906972683,0.0651587860459025,0.0868783813945366,
0.0977381790688537,0.119457774417488,0.173756762789073,0.195476358137707,
0.217195953486341,0.238915548834976,0.249775346509293,0.255205245346451,
0.26063514418361,0.304074334880878,0.347513525578146,0.350819878802366),
 .UNSPECIFIED.);
#425=B_SPLINE_CURVE_WITH_KNOTS('',3,(#26982,#26983,#26984,#26985,#26986,
#26987,#26988,#26989,#26990,#26991,#26992,#26993,#26994,#26995,#26996,#26997,
#26998,#26999,#27000,#27001,#27002),.UNSPECIFIED.,.F.,.F.,(4,1,1,1,1,1,
1,1,1,1,1,1,1,1,1,1,1,1,4),(0.351261425313739,0.354255847492041,0.390044844782951,
0.407939343428406,0.42583384207386,0.443728340719315,0.46162283936477,0.470570088687497,
0.497411836655679,0.533200833946589,0.551095332592044,0.560042581914771,
0.564516206576135,0.568989831237498,0.586884329882953,0.604778828528408,
0.613726077851135,0.622673327173863,0.640567825819317),.UNSPECIFIED.);
#426=B_SPLINE_CURVE_WITH_KNOTS('',3,(#27006,#27007,#27008,#27009,#27010,
#27011,#27012,#27013,#27014,#27015,#27016,#27017,#27018,#27019,#27020,#27021,
#27022,#27023,#27024),.UNSPECIFIED.,.F.,.F.,(4,1,1,1,1,1,1,1,1,1,1,1,1,
1,1,1,4),(0.,0.032579393007947,0.0434391906772627,0.065158786015894,0.0868783813545254,
0.0977381790238411,0.119457774362472,0.173756762709051,0.195476358047682,
0.217195953386313,0.238915548724945,0.24977534639426,0.255205245228918,
0.260635144063576,0.304074334740839,0.347513525418102,0.350819155150611),
 .UNSPECIFIED.);
#427=B_SPLINE_CURVE_WITH_KNOTS('',3,(#27028,#27029,#27030,#27031,#27032,
#27033,#27034,#27035,#27036,#27037,#27038,#27039,#27040,#27041,#27042,#27043,
#27044,#27045),.UNSPECIFIED.,.F.,.F.,(4,1,1,1,1,1,1,1,1,1,1,1,1,1,1,4),
(0.351261425313739,0.35425584787858,0.372150348833954,0.390044849789328,
0.407939350744702,0.416886601222389,0.425833851700076,0.461622853610824,
0.497411855521572,0.53320085743232,0.551095358387694,0.568989859343068,
0.586884360298442,0.604778861253817,0.613726111731503,0.640567863164564),
 .UNSPECIFIED.);
#428=B_SPLINE_CURVE_WITH_KNOTS('',3,(#27049,#27050,#27051,#27052,#27053,
#27054,#27055,#27056,#27057,#27058,#27059,#27060,#27061,#27062,#27063,#27064,
#27065,#27066,#27067),.UNSPECIFIED.,.F.,.F.,(4,1,1,1,1,1,1,1,1,1,1,1,1,
1,1,1,4),(0.,0.0218558225633788,0.0327837338450682,0.0437116451267576,0.0655674676901365,
0.0874232902535153,0.0983512015352047,0.109279112816894,0.131134935380273,
0.174846580507031,0.218558225633788,0.240414048197167,0.262269870760546,
0.284125693323925,0.305981515887303,0.349693161014061,0.353045062814117),
 .UNSPECIFIED.);
#429=B_SPLINE_CURVE_WITH_KNOTS('',3,(#27071,#27072,#27073,#27074,#27075,
#27076,#27077,#27078,#27079,#27080,#27081,#27082,#27083,#27084,#27085,#27086,
#27087,#27088),.UNSPECIFIED.,.F.,.F.,(4,1,1,1,1,1,1,1,1,1,1,1,1,1,1,4),
(0.134726986384039,0.138033894591262,0.157795792183236,0.177557689775211,
0.197319587367185,0.207200536163172,0.21708148495916,0.256605280143108,
0.296129075327057,0.335652870511006,0.35541476810298,0.375176665694955,
0.394938563286929,0.414700460878903,0.424581409674891,0.454224256062852),
 .UNSPECIFIED.);
#430=B_SPLINE_CURVE_WITH_KNOTS('',3,(#27092,#27093,#27094,#27095,#27096,
#27097,#27098,#27099,#27100,#27101,#27102,#27103,#27104,#27105,#27106,#27107,
#27108,#27109,#27110),.UNSPECIFIED.,.F.,.F.,(4,1,1,1,1,1,1,1,1,1,1,1,1,
1,1,1,4),(0.,0.032572548443813,0.0434300645917507,0.065145096887626,0.0868601291835013,
0.097717645331439,0.108575161479377,0.130290193775252,0.173720258367003,
0.260580387550504,0.266009145624473,0.271437903698442,0.282295419846379,
0.298581694068286,0.304010452142255,0.347440516734005,0.350748646683325),
 .UNSPECIFIED.);
#431=B_SPLINE_CURVE_WITH_KNOTS('',3,(#27114,#27115,#27116,#27117,#27118,
#27119,#27120,#27121,#27122,#27123,#27124,#27125,#27126,#27127,#27128,#27129,
#27130),.UNSPECIFIED.,.F.,.F.,(4,1,1,1,1,1,1,1,1,1,1,1,1,1,4),(0.0574324344854207,
0.0593504322920632,0.0822759013466683,0.105201370401273,0.110932737664925,
0.116664104928576,0.128126839455878,0.139589573983181,0.151052308510483,
0.17970914482874,0.196903246619694,0.208365981146996,0.219828715674299,
0.22556008293795,0.242754184728904),.UNSPECIFIED.);
#432=B_SPLINE_CURVE_WITH_KNOTS('',3,(#27134,#27135,#27136,#27137,#27138,
#27139,#27140,#27141,#27142,#27143,#27144,#27145,#27146,#27147,#27148,#27149,
#27150,#27151,#27152,#27153),.UNSPECIFIED.,.F.,.F.,(4,1,1,1,1,1,1,1,1,1,
1,1,1,1,1,1,1,4),(0.,0.0325789546137133,0.0434386061516177,0.0651579092274265,
0.0868772123032354,0.0977368638411398,0.108596515379044,0.130315818454853,
0.173754424606471,0.217193030758089,0.238912333833897,0.260631636909706,
0.271491288447611,0.282350939985515,0.29321059152342,0.304070243061324,
0.347508849212942,0.350821898751245),.UNSPECIFIED.);
#433=B_SPLINE_CURVE_WITH_KNOTS('',3,(#27157,#27158,#27159,#27160,#27161,
#27162,#27163,#27164,#27165,#27166,#27167,#27168,#27169,#27170,#27171),
 .UNSPECIFIED.,.F.,.F.,(4,1,1,1,1,1,1,1,1,1,1,1,4),(0.351261425313739,0.354255847717629,
0.390044847704719,0.425833847691809,0.470570097675672,0.479517347672445,
0.49741184766599,0.542148097649853,0.568989847640171,0.586884347633716,
0.604778847627261,0.613726097624034,0.640567847614352),.UNSPECIFIED.);
#434=B_SPLINE_CURVE_WITH_KNOTS('',3,(#27175,#27176,#27177,#27178,#27179,
#27180,#27181,#27182,#27183,#27184,#27185,#27186,#27187,#27188,#27189,#27190,
#27191,#27192,#27193),.UNSPECIFIED.,.F.,.F.,(4,1,1,1,1,1,1,1,1,1,1,1,1,
1,1,1,4),(0.,0.0325793930141872,0.043439190685583,0.0542989883569787,0.0651587860283745,
0.086878381371166,0.0977381790425617,0.119457774385353,0.130317572056749,
0.173756762742332,0.217195953427915,0.238915548770706,0.260635144113498,
0.282354739456289,0.314934132470477,0.347513525484664,0.350848293700851),
 .UNSPECIFIED.);
#435=B_SPLINE_CURVE_WITH_KNOTS('',3,(#27197,#27198,#27199,#27200,#27201,
#27202,#27203,#27204,#27205,#27206,#27207,#27208,#27209,#27210,#27211,#27212,
#27213),.UNSPECIFIED.,.F.,.F.,(4,1,1,1,1,1,1,1,1,1,1,1,1,1,4),(0.351261530740907,
0.354255847382348,0.390044843362201,0.425833839342054,0.434781088337017,
0.44372833733198,0.461622835321907,0.479517333311833,0.49741183130176,0.542148076276576,
0.568989823261466,0.586884321251392,0.604778819241319,0.613726068236282,
0.640567815221172),.UNSPECIFIED.);
#436=B_SPLINE_CURVE_WITH_KNOTS('',3,(#27217,#27218,#27219,#27220,#27221,
#27222,#27223,#27224,#27225,#27226,#27227,#27228,#27229,#27230,#27231,#27232,
#27233,#27234,#27235),.UNSPECIFIED.,.F.,.F.,(4,1,1,1,1,1,1,1,1,1,1,1,1,
1,1,1,4),(0.,0.021719595347394,0.032579393021091,0.043439190694788,0.065158786042182,
0.0868783813895759,0.0977381790632729,0.119457774410667,0.130317572084364,
0.173756762779152,0.21719595347394,0.238915548821334,0.260635144168728,
0.282354739516122,0.304074334863516,0.347513525558304,0.350824050932044),
 .UNSPECIFIED.);
#437=B_SPLINE_CURVE_WITH_KNOTS('',3,(#27239,#27240,#27241,#27242,#27243,
#27244,#27245,#27246,#27247,#27248,#27249,#27250,#27251,#27252,#27253,#27254,
#27255,#27256),.UNSPECIFIED.,.F.,.F.,(4,1,1,1,1,1,1,1,1,1,1,1,1,1,1,4),
(0.351271479446867,0.354255847276431,0.3721503446334,0.381097593311884,
0.390044841990369,0.407939339347338,0.425833836704307,0.443728334061276,
0.497411826132183,0.533200820846121,0.55109531820309,0.568989815560059,
0.586884312917028,0.604778810273997,0.613726058952482,0.640567804987935),
 .UNSPECIFIED.);
#438=B_SPLINE_CURVE_WITH_KNOTS('',3,(#27260,#27261,#27262,#27263,#27264,
#27265,#27266,#27267,#27268,#27269,#27270,#27271,#27272,#27273,#27274),
 .UNSPECIFIED.,.F.,.F.,(4,1,1,1,1,1,1,1,1,1,1,1,4),(0.,0.0325793930123882,
0.0434391906831843,0.0651587860247764,0.0868783813663685,0.119457774378757,
0.173756762732737,0.195476358074329,0.260635144099105,0.271494941769902,
0.30407433478229,0.347513525465474,0.350791036601536),.UNSPECIFIED.);
#439=B_SPLINE_CURVE_WITH_KNOTS('',3,(#27278,#27279,#27280,#27281,#27282,
#27283,#27284,#27285,#27286,#27287,#27288,#27289,#27290,#27291,#27292,#27293,
#27294),.UNSPECIFIED.,.F.,.F.,(4,1,1,1,1,1,1,1,1,1,1,1,1,1,4),(0.351261728605554,
0.354255847725072,0.37215034776309,0.390044847801108,0.407939347839126,
0.416886597858135,0.425833847877144,0.479517347991197,0.497411848029215,
0.542148098124259,0.568989848181286,0.586884348219304,0.604778848257322,
0.613726098276331,0.640567848333357),.UNSPECIFIED.);
#440=B_SPLINE_CURVE_WITH_KNOTS('',3,(#27298,#27299,#27300,#27301,#27302,
#27303,#27304,#27305,#27306,#27307,#27308,#27309,#27310,#27311,#27312,#27313),
 .UNSPECIFIED.,.F.,.F.,(4,1,1,1,1,1,1,1,1,1,1,1,1,4),(0.,0.0325793930249551,
0.0434391906999401,0.0651587860499102,0.0868783813998803,0.0977381790748653,
0.119457774424835,0.173756762799761,0.217195953499701,0.249775346524656,
0.260635144199641,0.282354739549611,0.347513525599521,0.350789741290272),
 .UNSPECIFIED.);
#441=B_SPLINE_CURVE_WITH_KNOTS('',3,(#27317,#27318,#27319,#27320,#27321,
#27322,#27323,#27324,#27325,#27326,#27327,#27328,#27329,#27330,#27331),
 .UNSPECIFIED.,.F.,.F.,(4,1,1,1,1,1,1,1,1,1,1,1,4),(0.351261425313738,0.35425584759651,
0.390044846136022,0.425833844675534,0.461622843215046,0.479517342484802,
0.497411841754558,0.551095339563825,0.568989838833581,0.586884338103337,
0.604778837373093,0.613726087007971,0.640567835912605),.UNSPECIFIED.);
#442=B_SPLINE_CURVE_WITH_KNOTS('',3,(#27335,#27336,#27337,#27338,#27339,
#27340,#27341,#27342,#27343,#27344,#27345,#27346,#27347,#27348,#27349,#27350,
#27351,#27352,#27353,#27354),.UNSPECIFIED.,.F.,.F.,(4,1,1,1,1,1,1,1,1,1,
1,1,1,1,1,1,1,4),(0.,0.0325793930116233,0.0434391906821644,0.0542989883527054,
0.0651587860232465,0.0868783813643287,0.0977381790348698,0.119457774375952,
0.130317572046493,0.173756762728657,0.217195953410822,0.238915548751904,
0.260635144092986,0.282354739434068,0.30407433477515,0.325793930116233,
0.347513525457315,0.350813372103892),.UNSPECIFIED.);
#443=B_SPLINE_CURVE_WITH_KNOTS('',3,(#27358,#27359,#27360,#27361,#27362,
#27363,#27364,#27365,#27366,#27367,#27368,#27369,#27370,#27371,#27372),
 .UNSPECIFIED.,.F.,.F.,(4,1,1,1,1,1,1,1,1,1,1,1,4),(0.351261425313738,0.354255847421228,
0.390044843865796,0.425833840310363,0.461622836754931,0.479517334977215,
0.497411833199498,0.55109532786635,0.568989826088633,0.586884324310917,
0.604778822533201,0.613726071644343,0.640567818977768),.UNSPECIFIED.);
#444=B_SPLINE_CURVE_WITH_KNOTS('',3,(#27376,#27377,#27378,#27379,#27380,
#27381,#27382,#27383,#27384,#27385,#27386,#27387,#27388,#27389,#27390,#27391),
 .UNSPECIFIED.,.F.,.F.,(4,1,1,1,1,1,1,1,1,1,1,1,1,4),(0.,0.0325793097402814,
0.0434390796537085,0.0651586194805627,0.086878159307417,0.0977379292208441,
0.173756318614834,0.195475858441688,0.217195398268542,0.260634477922251,
0.304073557575959,0.336652867316241,0.347512637229668,0.350798526118062),
 .UNSPECIFIED.);
#445=B_SPLINE_CURVE_WITH_KNOTS('',3,(#27395,#27396,#27397,#27398,#27399,
#27400,#27401,#27402,#27403,#27404,#27405,#27406,#27407,#27408),
 .UNSPECIFIED.,.F.,.F.,(4,1,1,1,1,1,1,1,1,1,1,4),(0.0931972916890651,0.0981391683195413,
0.216268676323884,0.24580105332497,0.290099618826599,0.334398184328228,
0.408229126830942,0.452527692332571,0.482060069333657,0.511592446334743,
0.526358634835285,0.570657200336914),.UNSPECIFIED.);
#446=B_SPLINE_CURVE_WITH_KNOTS('',3,(#27412,#27413,#27414,#27415,#27416,
#27417,#27418,#27419,#27420,#27421,#27422,#27423,#27424,#27425,#27426,#27427),
 .UNSPECIFIED.,.F.,.F.,(4,1,1,1,1,1,1,1,1,1,1,1,1,4),(0.,0.0368941921573239,
0.0491922562097653,0.0737883843146479,0.0983845124195305,0.110682576471972,
0.135278704576854,0.196769024839061,0.245961281048826,0.270557409153709,
0.295153537258592,0.319749665363474,0.393538049678122,0.397251142174947),
 .UNSPECIFIED.);
#447=B_SPLINE_CURVE_WITH_KNOTS('',3,(#27431,#27432,#27433,#27434,#27435,
#27436,#27437,#27438,#27439,#27440,#27441,#27442,#27443,#27444,#27445,#27446,
#27447,#27448),.UNSPECIFIED.,.F.,.F.,(4,1,1,1,1,1,1,1,1,1,1,1,1,1,1,4),
(0.136741791121389,0.139904182663315,0.158819432388561,0.196649931839055,
0.215565181564302,0.234480431289549,0.253395681014796,0.291226180465289,
0.338514304778406,0.34797192964103,0.357429554503653,0.366887179366277,
0.385802429091524,0.404717678816771,0.414175303679394,0.442548178267264),
 .UNSPECIFIED.);
#448=B_SPLINE_CURVE_WITH_KNOTS('',3,(#27452,#27453,#27454,#27455,#27456,
#27457,#27458,#27459,#27460,#27461,#27462,#27463,#27464,#27465,#27466),
 .UNSPECIFIED.,.F.,.F.,(4,1,1,1,1,1,1,1,1,1,1,1,4),(0.,0.0325793930125535,
0.0434391906834047,0.0651587860251071,0.0868783813668094,0.108597976708512,
0.173756762733619,0.195476358075321,0.217195953417024,0.260635144100428,
0.304074334783833,0.347513525467238,0.350846174826461),.UNSPECIFIED.);
#449=B_SPLINE_CURVE_WITH_KNOTS('',3,(#27470,#27471,#27472,#27473,#27474,
#27475,#27476,#27477,#27478,#27479,#27480,#27481,#27482,#27483,#27484,#27485),
 .UNSPECIFIED.,.F.,.F.,(4,1,1,1,1,1,1,1,1,1,1,1,1,4),(0.351271301501517,
0.354255847707038,0.407939347497804,0.425833847428059,0.443728347358315,
0.488464597183953,0.497411847149081,0.515306347079336,0.551095346939847,
0.568989846870102,0.586884346800358,0.604778846730613,0.613726096695741,
0.640567846591124),.UNSPECIFIED.);
#450=B_SPLINE_CURVE_WITH_KNOTS('',3,(#27489,#27490,#27491,#27492,#27493,
#27494,#27495,#27496,#27497,#27498,#27499,#27500,#27501,#27502,#27503,#27504),
 .UNSPECIFIED.,.F.,.F.,(4,1,1,1,1,1,1,1,1,1,1,1,1,4),(0.,0.0325793930317906,
0.0434391907090541,0.0651587860635812,0.0868783814181082,0.108597976772635,
0.130317572127162,0.173756762836216,0.217195953545271,0.260635144254325,
0.282354739608852,0.325793930317906,0.347513525672433,0.350848293890421),
 .UNSPECIFIED.);
#451=B_SPLINE_CURVE_WITH_KNOTS('',3,(#27508,#27509,#27510,#27511,#27512,
#27513,#27514,#27515,#27516,#27517,#27518,#27519,#27520,#27521,#27522,#27523,
#27524),.UNSPECIFIED.,.F.,.F.,(4,1,1,1,1,1,1,1,1,1,1,1,1,1,4),(0.351261678797134,
0.35425584762492,0.372150347064446,0.390044846503972,0.407939345943498,
0.416886595663261,0.425833845383024,0.479517343701602,0.497411843141128,
0.542148091739942,0.568989840899231,0.586884340338757,0.604778839778283,
0.613726089498046,0.640567838657335),.UNSPECIFIED.);
#452=B_SPLINE_CURVE_WITH_KNOTS('',3,(#27528,#27529,#27530,#27531,#27532,
#27533,#27534,#27535,#27536,#27537,#27538,#27539,#27540,#27541,#27542),
 .UNSPECIFIED.,.F.,.F.,(4,1,1,1,1,1,1,1,1,1,1,1,4),(0.,0.0325793930157896,
0.0434391906877195,0.0651587860315793,0.086878381375439,0.108597976719299,
0.130317572063159,0.173756762750878,0.217195953438598,0.260635144126317,
0.304074334814037,0.347513525501756,0.350842474191291),.UNSPECIFIED.);
#453=B_SPLINE_CURVE_WITH_KNOTS('',3,(#27546,#27547,#27548,#27549,#27550,
#27551,#27552,#27553,#27554,#27555,#27556,#27557,#27558,#27559,#27560,#27561,
#27562,#27563,#27564,#27565,#27566,#27567,#27568,#27569,#27570,#27571,#27572,
#27573,#27574,#27575,#27576,#27577,#27578,#27579,#27580,#27581,#27582,#27583,
#27584,#27585),.UNSPECIFIED.,.F.,.F.,(4,3,3,3,3,3,3,3,3,3,3,3,3,4),(0.000100343318888589,
0.00211700710578998,0.0116301296248504,0.0176438447776065,0.0203218262442056,
0.0279911126768708,0.0341353720887311,0.0378914478697084,0.0416646752176139,
0.045727158280587,0.0481343714586611,0.0509000843805532,0.0542503351447326,
0.0813895718295443),.UNSPECIFIED.);
#454=B_SPLINE_CURVE_WITH_KNOTS('',3,(#27589,#27590,#27591,#27592,#27593,
#27594,#27595,#27596,#27597,#27598,#27599,#27600,#27601,#27602,#27603),
 .UNSPECIFIED.,.F.,.F.,(4,1,1,1,1,1,1,1,1,1,1,1,4),(0.,0.0325793930236318,
0.0434391906981757,0.0651587860472636,0.0868783813963514,0.119457774419983,
0.173756762792703,0.195476358141791,0.260635144189054,0.271494941863598,
0.30407433488723,0.347513525585406,0.350787783602951),.UNSPECIFIED.);
#455=B_SPLINE_CURVE_WITH_KNOTS('',3,(#27607,#27608,#27609,#27610,#27611,
#27612,#27613,#27614,#27615,#27616,#27617,#27618,#27619,#27620,#27621,#27622,
#27623),.UNSPECIFIED.,.F.,.F.,(4,1,1,1,1,1,1,1,1,1,1,1,1,1,4),(0.351273472241782,
0.354255847802748,0.372150348304963,0.390044848807178,0.407939349309393,
0.425833849811608,0.461622850816039,0.497411851820469,0.542148103076006,
0.551095353327114,0.568989853829329,0.586884354331544,0.604778854833759,
0.613726105084867,0.64056785583819),.UNSPECIFIED.);
#456=B_SPLINE_CURVE_WITH_KNOTS('',3,(#27627,#27628,#27629,#27630,#27631,
#27632,#27633,#27634,#27635,#27636,#27637,#27638,#27639,#27640,#27641),
 .UNSPECIFIED.,.F.,.F.,(4,1,1,1,1,1,1,1,1,1,1,1,4),(0.,0.032579393022239,
0.0434391906963187,0.065158786044478,0.0868783813926374,0.108597976740797,
0.130317572088956,0.173756762785275,0.260635144177912,0.271494941851992,
0.304074334874231,0.347513525570549,0.350823140362429),.UNSPECIFIED.);
#457=B_SPLINE_CURVE_WITH_KNOTS('',3,(#27645,#27646,#27647,#27648,#27649,
#27650,#27651,#27652,#27653,#27654,#27655,#27656,#27657,#27658,#27659),
 .UNSPECIFIED.,.F.,.F.,(4,1,1,1,1,1,1,1,1,1,1,1,4),(0.351261425313741,0.35425584764769,
0.390044846798899,0.425833845950108,0.461622845101317,0.479517344676922,
0.497411844252526,0.542148093191537,0.568989842554944,0.586884342130548,
0.604778841706153,0.613726091493955,0.640567840857362),.UNSPECIFIED.);
#458=B_SPLINE_CURVE_WITH_KNOTS('',3,(#27663,#27664,#27665,#27666,#27667,
#27668,#27669,#27670,#27671,#27672,#27673,#27674,#27675,#27676,#27677,#27678,
#27679,#27680,#27681),.UNSPECIFIED.,.F.,.F.,(4,1,1,1,1,1,1,1,1,1,1,1,1,
1,1,1,4),(0.,0.0327837338451708,0.0437116451268944,0.0655674676903416,0.0874232902537888,
0.109279112817236,0.131134935380683,0.174846580507578,0.196702403071025,
0.218558225634472,0.262269870761366,0.267733826402228,0.27319778204309,
0.284125693324814,0.305981515888261,0.349693161015155,0.35304098170316),
 .UNSPECIFIED.);
#459=B_SPLINE_CURVE_WITH_KNOTS('',3,(#27685,#27686,#27687,#27688,#27689,
#27690,#27691,#27692,#27693,#27694,#27695,#27696,#27697,#27698,#27699,#27700,
#27701),.UNSPECIFIED.,.F.,.F.,(4,1,1,1,1,1,1,1,1,1,1,1,1,1,4),(0.134727030764327,
0.138033894591211,0.177557689775802,0.217081484960394,0.226962433756542,
0.23684338255269,0.256605280144986,0.276367177737282,0.296129075329578,
0.345533819310318,0.375176665698762,0.394938563291058,0.414700460883354,
0.424581409679502,0.454224256067946),.UNSPECIFIED.);
#460=B_SPLINE_CURVE_WITH_KNOTS('',3,(#27705,#27706,#27707,#27708,#27709,
#27710,#27711,#27712),.UNSPECIFIED.,.F.,.F.,(4,2,2,4),(0.,0.0512135387342888,
0.087237825725378,0.157821777158906),.UNSPECIFIED.);
#461=B_SPLINE_CURVE_WITH_KNOTS('',3,(#27716,#27717,#27718,#27719,#27720,
#27721,#27722,#27723,#27724,#27725,#27726,#27727,#27728,#27729,#27730,#27731,
#27732,#27733,#27734,#27735),.UNSPECIFIED.,.F.,.F.,(4,1,1,1,1,1,1,1,1,1,
1,1,1,1,1,1,1,4),(0.0574322859850518,0.0593504322657392,0.0822759010057599,
0.0937386353757703,0.105201369745781,0.108067053338283,0.110932736930786,
0.116664104115791,0.128126838485801,0.139589572855812,0.151052307225822,
0.179709143150848,0.191171877520858,0.196903244705864,0.208365979075874,
0.219828713445884,0.22556008063089,0.242754182185905),.UNSPECIFIED.);
#462=B_SPLINE_CURVE_WITH_KNOTS('',3,(#27739,#27740,#27741,#27742,#27743,
#27744,#27745,#27746,#27747,#27748,#27749,#27750,#27751,#27752,#27753,#27754,
#27755,#27756),.UNSPECIFIED.,.F.,.F.,(4,1,1,1,1,1,1,1,1,1,1,1,1,1,1,4),
(0.,0.0325789545997274,0.0434386061329699,0.0651579091994548,0.0868772122659398,
0.0977368637991822,0.119456166865667,0.17375442453188,0.217193030664849,
0.260631636797819,0.271491288331062,0.282350939864304,0.304070242930789,
0.325789545997274,0.347508849063759,0.350802705344221),.UNSPECIFIED.);
#463=B_SPLINE_CURVE_WITH_KNOTS('',3,(#27760,#27761,#27762,#27763,#27764,
#27765,#27766,#27767,#27768,#27769,#27770,#27771,#27772,#27773,#27774,#27775,
#27776,#27777,#27778),.UNSPECIFIED.,.F.,.F.,(4,1,1,1,1,1,1,1,1,1,1,1,1,
1,1,1,4),(0.351274828846267,0.354255848623625,0.39004485943905,0.394518485790978,
0.407939364846763,0.416886617550619,0.421360243902547,0.425833870254475,
0.497411891885325,0.53320090270075,0.551095408108462,0.560042660812319,
0.568989913516175,0.586884418923887,0.6047789243316,0.613726177035456,0.640567935147025),
 .UNSPECIFIED.);
#464=B_SPLINE_CURVE_WITH_KNOTS('',3,(#27782,#27783,#27784,#27785,#27786,
#27787,#27788,#27789,#27790,#27791,#27792,#27793,#27794,#27795,#27796,#27797,
#27798,#27799),.UNSPECIFIED.,.F.,.F.,(4,1,1,1,1,1,1,1,1,1,1,1,1,1,1,4),
(0.,0.0325793930123313,0.0434391906831083,0.0651587860246625,0.0868783813662167,
0.0977381790369938,0.119457774378548,0.173756762732433,0.217195953415542,
0.26063514409865,0.271494941769427,0.282354739440204,0.304074334781758,
0.325793930123313,0.347513525464867,0.350806496344244),.UNSPECIFIED.);
#465=B_SPLINE_CURVE_WITH_KNOTS('',3,(#27803,#27804,#27805,#27806,#27807,
#27808,#27809,#27810,#27811,#27812,#27813,#27814,#27815,#27816,#27817,#27818,
#27819,#27820,#27821,#27822,#27823,#27824,#27825),.UNSPECIFIED.,.F.,.F.,
(4,2,2,1,1,1,1,1,1,1,1,1,1,1,1,1,1,1,4),(0.351271261271763,0.353137441377921,
0.354255847573797,0.372150346707808,0.390044845841819,0.407939344975829,
0.42583384410984,0.443728343243851,0.461622842377862,0.479517341511873,
0.497411840645883,0.533200838913905,0.551095338047916,0.560042587614921,
0.568989837181927,0.586884336315937,0.604778835449948,0.613726085016954,
0.64056783371797),.UNSPECIFIED.);
#466=B_SPLINE_CURVE_WITH_KNOTS('',3,(#27829,#27830,#27831,#27832,#27833,
#27834,#27835,#27836,#27837,#27838,#27839,#27840,#27841,#27842,#27843,#27844,
#27845,#27846),.UNSPECIFIED.,.F.,.F.,(4,1,1,1,1,1,1,1,1,1,1,1,1,1,1,4),
(0.,0.0325793930260695,0.0434391907014261,0.0651587860521391,0.0868783814028521,
0.108597976753565,0.130317572104278,0.173756762805704,0.260635144208556,
0.304074334909982,0.306789284328822,0.309504233747661,0.314934132585339,
0.325793930260696,0.347513525611409,0.350836093641256),.UNSPECIFIED.);
#467=B_SPLINE_CURVE_WITH_KNOTS('',3,(#27850,#27851,#27852,#27853,#27854,
#27855,#27856,#27857,#27858,#27859,#27860,#27861,#27862,#27863,#27864,#27865,
#27866,#27867,#27868),.UNSPECIFIED.,.F.,.F.,(4,1,1,1,1,1,1,1,1,1,1,1,1,
1,1,1,4),(0.351264100247147,0.354255847560549,0.372150346615404,0.390044845670259,
0.407939344725115,0.416886594252542,0.42583384377997,0.461622841889681,
0.488464590471964,0.497411839999392,0.533200838109102,0.551095337163958,
0.568989836218813,0.586884335273668,0.604778834328524,0.613726083855951,
0.640567832438234),.UNSPECIFIED.);
#468=B_SPLINE_CURVE_WITH_KNOTS('',3,(#27872,#27873,#27874,#27875,#27876,
#27877,#27878,#27879,#27880,#27881,#27882,#27883,#27884,#27885,#27886,#27887,
#27888,#27889),.UNSPECIFIED.,.F.,.F.,(4,1,1,1,1,1,1,1,1,1,1,1,1,1,1,4),
(0.,0.0325793930079354,0.0434391906772472,0.0651587860158707,0.0868783813544943,
0.11945777436243,0.152037167370365,0.173756762708989,0.195476358047612,
0.217195953386236,0.238915548724859,0.260635144063483,0.282354739402107,
0.30407433474073,0.347513525417977,0.350816322009827),.UNSPECIFIED.);
#469=B_SPLINE_CURVE_WITH_KNOTS('',3,(#27893,#27894,#27895,#27896,#27897,
#27898,#27899,#27900,#27901,#27902,#27903,#27904,#27905,#27906,#27907,#27908,
#27909,#27910,#27911),.UNSPECIFIED.,.F.,.F.,(4,1,1,1,1,1,1,1,1,1,1,1,1,
1,1,1,4),(0.351263876883672,0.354255847479606,0.372150346050742,0.390044844621878,
0.407939343193014,0.416886592478582,0.42583384176415,0.461622838906422,
0.488464586763126,0.497411836048694,0.533200833190966,0.551095331762102,
0.568989830333238,0.586884328904374,0.60477882747551,0.613726076761078,
0.640567824617782),.UNSPECIFIED.);
#470=B_SPLINE_CURVE_WITH_KNOTS('',3,(#27915,#27916,#27917,#27918,#27919,
#27920,#27921,#27922,#27923,#27924,#27925,#27926,#27927,#27928,#27929,#27930,
#27931,#27932,#27933,#27934,#27935),.UNSPECIFIED.,.F.,.F.,(4,1,1,1,1,1,
1,1,1,1,1,1,1,1,1,1,1,1,4),(0.,0.0325793930226444,0.0434391906968592,0.0651587860452888,
0.0868783813937184,0.0977381790679332,0.108597976742148,0.130317572090578,
0.173756762787437,0.217195953484296,0.238915548832726,0.260635144181155,
0.266065043018263,0.27149494185537,0.282354739529585,0.2932145372038,0.304074334878014,
0.347513525574874,0.350818340766546),.UNSPECIFIED.);
#471=B_SPLINE_CURVE_WITH_KNOTS('',3,(#27939,#27940,#27941,#27942,#27943,
#27944,#27945,#27946,#27947,#27948,#27949,#27950,#27951,#27952,#27953,#27954,
#27955,#27956),.UNSPECIFIED.,.F.,.F.,(4,1,1,1,1,1,1,1,1,1,1,1,1,1,1,4),
(0.351261425313741,0.354255848056333,0.372150350073952,0.381097601082762,
0.385571226587167,0.38780803933937,0.390044852091572,0.425833856126811,
0.49741186419729,0.533200868232529,0.551095370250149,0.568989872267768,
0.586884374285388,0.604778876303007,0.613726127311817,0.640567880338247),
 .UNSPECIFIED.);
#472=B_SPLINE_CURVE_WITH_KNOTS('',3,(#27960,#27961,#27962,#27963,#27964,
#27965,#27966,#27967,#27968,#27969,#27970,#27971,#27972,#27973,#27974,#27975,
#27976),.UNSPECIFIED.,.F.,.F.,(4,1,1,1,1,1,1,1,1,1,1,1,1,1,4),(0.,0.0325793930148059,
0.0434391906864078,0.0651587860296118,0.0868783813728157,0.119457774387622,
0.152037167402427,0.173756762745631,0.195476358088835,0.217195953432039,
0.228055751103641,0.238915548775243,0.260635144118447,0.347513525491263,
0.35080304454135),.UNSPECIFIED.);
#473=B_SPLINE_CURVE_WITH_KNOTS('',3,(#27980,#27981,#27982,#27983,#27984,
#27985,#27986,#27987,#27988,#27989,#27990,#27991,#27992,#27993,#27994),
 .UNSPECIFIED.,.F.,.F.,(4,1,1,1,1,1,1,1,1,1,1,1,4),(0.35126142531374,0.354255847892618,
0.390044849971179,0.42583385204974,0.4616228541283,0.479517355167581,0.497411856206861,
0.542148108805062,0.568989860363982,0.586884361403262,0.604778862442543,
0.613726112962183,0.640567864521103),.UNSPECIFIED.);
#474=B_SPLINE_CURVE_WITH_KNOTS('',3,(#27998,#27999,#28000,#28001,#28002,
#28003,#28004,#28005,#28006,#28007,#28008,#28009,#28010,#28011,#28012,#28013,
#28014,#28015,#28016,#28017,#28018,#28019),.UNSPECIFIED.,.F.,.F.,(4,1,1,
1,1,1,1,1,1,1,1,1,1,1,1,1,1,1,1,4),(0.,0.0217195398190078,0.0325793097285116,
0.0434390796380155,0.0651586194570233,0.086878159276031,0.092308044230783,
0.0977379291855349,0.108597699095039,0.130317238914047,0.173756318552062,
0.19547585837107,0.217195398190078,0.238914938009085,0.260634477828093,
0.282354017647101,0.304073557466109,0.314933327375612,0.347512637104124,
0.350829886386395),.UNSPECIFIED.);
#475=B_SPLINE_CURVE_WITH_KNOTS('',3,(#28023,#28024,#28025,#28026,#28027,
#28028,#28029,#28030,#28031,#28032,#28033,#28034,#28035,#28036,#28037,#28038,
#28039,#28040),.UNSPECIFIED.,.F.,.F.,(4,1,1,1,1,1,1,1,1,1,1,1,1,1,1,4),
(0.0932056818412186,0.0981391682442792,0.127671545353425,0.142437733907998,
0.15720392246257,0.186736299571716,0.216268676680861,0.245801053790007,
0.334398185117444,0.393462939335735,0.42299531644488,0.452527693554026,
0.482060070663172,0.511592447772317,0.52635863632689,0.570657201990608),
 .UNSPECIFIED.);
#476=B_SPLINE_CURVE_WITH_KNOTS('',3,(#28044,#28045,#28046,#28047,#28048,
#28049),.UNSPECIFIED.,.F.,.F.,(4,2,4),(0.,0.0601601681445252,0.0880292330372518),
 .UNSPECIFIED.);
#477=B_SPLINE_CURVE_WITH_KNOTS('',3,(#28053,#28054,#28055,#28056,#28057,
#28058,#28059,#28060,#28061,#28062,#28063,#28064,#28065,#28066,#28067,#28068,
#28069,#28070,#28071,#28072,#28073,#28074,#28075,#28076,#28077,#28078,#28079,
#28080,#28081,#28082,#28083,#28084,#28085,#28086,#28087,#28088,#28089,#28090,
#28091,#28092,#28093,#28094,#28095,#28096,#28097,#28098,#28099,#28100,#28101,
#28102,#28103,#28104,#28105,#28106,#28107,#28108,#28109,#28110),
 .UNSPECIFIED.,.F.,.F.,(4,3,3,3,3,3,3,3,3,3,3,3,3,3,3,3,3,3,3,4),(6.08712730435348E-5,
0.00275844945283138,0.0137381870738885,0.0225620476034396,0.0312714732191953,
0.0362576288629832,0.0423533777643801,0.0549063154363092,0.0674592531082383,
0.0925651284520965,0.142776879139813,0.255475301627304,0.367738092144255,
0.372730032656669,0.391490074030401,0.400744250952332,0.409965101196975,
0.421939848038402,0.429790402970525,0.485968151358161),.UNSPECIFIED.);
#478=B_SPLINE_CURVE_WITH_KNOTS('',3,(#28119,#28120,#28121,#28122,#28123,
#28124,#28125,#28126),.UNSPECIFIED.,.F.,.F.,(4,2,2,4),(6.11743783436508E-5,
0.191849769363527,0.239938446755784,0.283419085994991),.UNSPECIFIED.);
#479=B_SPLINE_CURVE_WITH_KNOTS('',3,(#28130,#28131,#28132,#28133,#28134,
#28135,#28136,#28137,#28138,#28139,#28140,#28141,#28142,#28143,#28144,#28145,
#28146,#28147),.UNSPECIFIED.,.F.,.F.,(4,1,1,1,1,1,1,1,1,1,1,1,1,1,1,4),
(0.,0.0325750462990963,0.0434333950654617,0.0651500925981926,0.0868667901309233,
0.108583487663654,0.130300185196385,0.173733580261847,0.217166975327308,
0.26060037039277,0.271458719159135,0.282317067925501,0.304033765458232,
0.325750462990963,0.347467160523693,0.350763145419038),.UNSPECIFIED.);
#480=B_SPLINE_CURVE_WITH_KNOTS('',3,(#28151,#28152,#28153,#28154,#28155,
#28156,#28157,#28158,#28159,#28160,#28161,#28162,#28163,#28164,#28165,#28166,
#28167,#28168),.UNSPECIFIED.,.F.,.F.,(4,1,1,1,1,1,1,1,1,1,1,1,1,1,1,4),
(0.0932058072533814,0.096518162942361,0.116363502645051,0.136208842347741,
0.156054182050431,0.165976851901776,0.175899521753121,0.215590201158501,
0.255280880563881,0.304894229820606,0.324739569523297,0.334662239374642,
0.354507579077332,0.374352918780022,0.384275588631367,0.414043598185402),
 .UNSPECIFIED.);
#481=B_SPLINE_CURVE_WITH_KNOTS('',3,(#28172,#28173,#28174,#28175,#28176,
#28177,#28178,#28179,#28180,#28181,#28182,#28183,#28184,#28185,#28186,#28187,
#28188,#28189),.UNSPECIFIED.,.F.,.F.,(4,1,1,1,1,1,1,1,1,1,1,1,1,1,1,4),
(0.,0.0325788513745152,0.0434384684993537,0.0651577027490305,0.0868769369987073,
0.108596171248384,0.130315405498061,0.173753873997415,0.238911576746445,
0.260630810996122,0.282350045245799,0.304069279495476,0.314928896620314,
0.325788513745152,0.347507747994829,0.350794257840603),.UNSPECIFIED.);
#482=B_SPLINE_CURVE_WITH_KNOTS('',3,(#28193,#28194,#28195,#28196,#28197,
#28198,#28199,#28200,#28201,#28202,#28203,#28204,#28205,#28206,#28207,#28208,
#28209,#28210,#28211,#28212,#28213,#28214,#28215,#28216,#28217,#28218,#28219,
#28220,#28221,#28222,#28223,#28224,#28225,#28226,#28227,#28228,#28229,#28230,
#28231,#28232,#28233,#28234,#28235,#28236,#28237,#28238,#28239,#28240,#28241,
#28242,#28243,#28244,#28245,#28246,#28247,#28248,#28249,#28250),
 .UNSPECIFIED.,.F.,.F.,(4,3,3,3,3,3,3,3,3,3,3,3,3,3,3,3,3,3,3,4),(2.64881849881361E-5,
0.00307223750536735,0.028642489643384,0.0367669288755048,0.0524286784203567,
0.0679644484217536,0.0833030784739446,0.0990034397740617,0.115012342116765,
0.132014384921338,0.171542385361576,0.19885726229201,0.214932531301613,
0.22333513626821,0.232015923980944,0.270309223346912,0.31550125331855,0.341731569313757,
0.371362864081148,0.439678803039698),.UNSPECIFIED.);
#483=B_SPLINE_CURVE_WITH_KNOTS('',3,(#28254,#28255,#28256,#28257,#28258,
#28259,#28260,#28261,#28262,#28263,#28264,#28265,#28266,#28267,#28268),
 .UNSPECIFIED.,.F.,.F.,(4,1,1,1,1,1,1,1,1,1,1,1,4),(0.,0.0325813112900846,
0.0434417483867794,0.0651626225801691,0.0868834967735589,0.119464808063643,
0.173766993547118,0.195487867740507,0.217208741933897,0.260650490320676,
0.304092238707456,0.347533987094235,0.350847240140668),.UNSPECIFIED.);
#484=B_SPLINE_CURVE_WITH_KNOTS('',3,(#28272,#28273,#28274,#28275,#28276,
#28277),.UNSPECIFIED.,.F.,.F.,(4,2,4),(8.14301014391022E-5,0.196579653373709,
0.311490292475107),.UNSPECIFIED.);
#485=B_SPLINE_CURVE_WITH_KNOTS('',3,(#28281,#28282,#28283,#28284,#28285,
#28286,#28287,#28288,#28289,#28290,#28291,#28292,#28293,#28294,#28295,#28296,
#28297,#28298),.UNSPECIFIED.,.F.,.F.,(4,1,1,1,1,1,1,1,1,1,1,1,1,1,1,4),
(0.,0.0325813113329355,0.0434417484439139,0.0651626226658709,0.0868834968878278,
0.108604371109785,0.130325245331742,0.173766993775656,0.260650490663484,
0.304092239107397,0.306807348385142,0.309522457662887,0.314952676218376,
0.325813113329354,0.347533987551311,0.350857049542678),.UNSPECIFIED.);
#486=B_SPLINE_CURVE_WITH_KNOTS('',3,(#28302,#28303,#28304,#28305,#28306,
#28307,#28308,#28309,#28310,#28311,#28312,#28313,#28314,#28315,#28316,#28317,
#28318,#28319,#28320,#28321,#28322,#28323,#28324,#28325,#28326,#28327,#28328,
#28329,#28330,#28331,#28332,#28333,#28334,#28335,#28336,#28337,#28338,#28339,
#28340,#28341,#28342,#28343,#28344,#28345,#28346,#28347,#28348,#28349,#28350,
#28351,#28352,#28353,#28354,#28355,#28356),.UNSPECIFIED.,.F.,.F.,(4,3,3,
3,3,3,3,3,3,3,3,3,3,3,3,3,3,3,4),(2.11964464360651E-5,0.00307933761122651,
0.0395949433846797,0.0486546450384591,0.0576974609832352,0.0668894095700696,
0.071471610540102,0.0760053733416042,0.0940997687264147,0.112217019766355,
0.148197822286634,0.184121554894769,0.202078226650051,0.211018420941679,
0.219896800832225,0.23983820976113,0.2677172728698,0.278184634008653,0.312492015504387),
 .UNSPECIFIED.);
#487=B_SPLINE_CURVE_WITH_KNOTS('',3,(#28360,#28361,#28362,#28363,#28364,
#28365,#28366,#28367,#28368,#28369,#28370,#28371,#28372,#28373,#28374,#28375,
#28376,#28377,#28378),.UNSPECIFIED.,.F.,.F.,(4,1,1,1,1,1,1,1,1,1,1,1,1,
1,1,1,4),(0.,0.0325813112891162,0.0434417483854882,0.0651626225782322,0.0868834967709763,
0.10860437096372,0.130325245156464,0.173766993541953,0.184627430638325,
0.217208741927441,0.260650490312929,0.271510927409301,0.282371364505673,
0.304092238698417,0.325813112891161,0.347533987083905,0.35082133726808),
 .UNSPECIFIED.);
#488=B_SPLINE_CURVE_WITH_KNOTS('',3,(#28382,#28383,#28384,#28385,#28386,
#28387),.UNSPECIFIED.,.F.,.F.,(4,2,4),(0.000173516420610335,0.167723093051734,
0.254522511958816),.UNSPECIFIED.);
#489=B_SPLINE_CURVE_WITH_KNOTS('',3,(#28391,#28392,#28393,#28394,#28395,
#28396,#28397,#28398,#28399,#28400,#28401,#28402,#28403,#28404,#28405,#28406,
#28407,#28408,#28409),.UNSPECIFIED.,.F.,.F.,(4,1,1,1,1,1,1,1,1,1,1,1,1,
1,1,1,4),(0.,0.0325813113093916,0.0434417484125221,0.0651626226187831,0.0868834968250442,
0.108604371031305,0.130325245237566,0.173766993650088,0.184627430753219,
0.21720874206261,0.260650490475133,0.271510927578263,0.282371364681394,
0.304092238887655,0.325813113093916,0.347533987300177,0.350820075515927),
 .UNSPECIFIED.);
#490=B_SPLINE_CURVE_WITH_KNOTS('',3,(#28413,#28414,#28415,#28416,#28417,
#28418),.UNSPECIFIED.,.F.,.F.,(4,2,4),(0.,0.264764622084999,0.482894632601792),
 .UNSPECIFIED.);
#491=B_SPLINE_CURVE_WITH_KNOTS('',3,(#28422,#28423,#28424,#28425,#28426,
#28427,#28428,#28429,#28430,#28431,#28432,#28433,#28434,#28435,#28436,#28437,
#28438,#28439,#28440,#28441,#28442,#28443,#28444),.UNSPECIFIED.,.F.,.F.,
(4,1,1,1,1,1,1,1,1,1,1,1,1,1,1,1,1,1,1,1,4),(0.,0.0325813113021046,0.0434417484028061,
0.0651626226042092,0.0868834968056123,0.0977439339063137,0.108604371007015,
0.130325245208418,0.173766993611225,0.195487867812628,0.217208742014031,
0.238929616215434,0.260650490416837,0.28237136461824,0.304092238819643,
0.325813113021046,0.347533987222449,0.348212764541243,0.348891541860037,
0.350249096497625,0.35080830738772),.UNSPECIFIED.);
#492=B_SPLINE_CURVE_WITH_KNOTS('',3,(#28448,#28449,#28450,#28451,#28452,
#28453,#28454,#28455,#28456,#28457,#28458,#28459,#28460,#28461,#28462,#28463,
#28464,#28465,#28466,#28467,#28468,#28469,#28470,#28471,#28472,#28473,#28474,
#28475,#28476,#28477,#28478,#28479,#28480,#28481,#28482,#28483,#28484,#28485,
#28486,#28487,#28488,#28489,#28490,#28491,#28492,#28493),.UNSPECIFIED.,
 .F.,.F.,(4,3,3,3,3,3,3,3,3,3,3,3,3,3,3,4),(2.29325682757538E-5,0.00307497248475355,
0.0214432536953726,0.0402954758924377,0.0593096938468517,0.0691626711428028,
0.0790635228724472,0.120294907072033,0.165515885024277,0.233611439622154,
0.268825942121262,0.290245409680214,0.354810754057985,0.445312525809899,
0.479839949490667,0.594280619733159),.UNSPECIFIED.);
#493=B_SPLINE_CURVE_WITH_KNOTS('',3,(#28497,#28498,#28499,#28500,#28501,
#28502,#28503,#28504,#28505,#28506,#28507,#28508,#28509,#28510,#28511,#28512,
#28513,#28514,#28515),.UNSPECIFIED.,.F.,.F.,(4,1,1,1,1,1,1,1,1,1,1,1,1,
1,1,1,4),(0.,0.0325811093290978,0.0434414791054637,0.0651622186581956,0.0868829582109275,
0.0977433279872934,0.108603697763659,0.130324437316391,0.173765916421855,
0.260648874632782,0.266079059520965,0.271509244409148,0.282369614185514,
0.298660168850063,0.304090353738246,0.34753183284371,0.35083845041488),
 .UNSPECIFIED.);
#494=B_SPLINE_CURVE_WITH_KNOTS('',3,(#28519,#28520,#28521,#28522,#28523,
#28524,#28525,#28526,#28527,#28528,#28529,#28530,#28531,#28532,#28533,#28534,
#28535,#28536),.UNSPECIFIED.,.F.,.F.,(4,1,1,1,1,1,1,1,1,1,1,1,1,1,1,4),
(0.134735529536501,0.138033894591027,0.157795792185277,0.177557689779527,
0.197319587373778,0.207200536170903,0.217081484968028,0.256605280156529,
0.29612907534503,0.345533819330656,0.365295716924906,0.375176665722032,
0.394938563316282,0.414700460910532,0.424581409707658,0.454224256099033),
 .UNSPECIFIED.);
#495=B_SPLINE_CURVE_WITH_KNOTS('',3,(#28540,#28541,#28542,#28543,#28544,
#28545,#28546,#28547,#28548,#28549,#28550,#28551,#28552,#28553,#28554,#28555,
#28556,#28557,#28558,#28559),.UNSPECIFIED.,.F.,.F.,(4,1,1,1,1,1,1,1,1,1,
1,1,1,1,1,1,1,4),(0.,0.0325779980296814,0.0434373307062418,0.0651559960593628,
0.0868746614124837,0.0977339940890442,0.119452659442165,0.173749322824967,
0.195467988178088,0.217186653531209,0.23890531888433,0.249764651560891,
0.255194317899171,0.260623984237451,0.282342649590572,0.304061314943693,
0.347498645649935,0.350792283140098),.UNSPECIFIED.);
#496=B_SPLINE_CURVE_WITH_KNOTS('',3,(#28563,#28564,#28565,#28566,#28567,
#28568,#28569,#28570,#28571,#28572,#28573,#28574,#28575,#28576,#28577,#28578,
#28579),.UNSPECIFIED.,.F.,.F.,(4,1,1,1,1,1,1,1,1,1,1,1,1,1,4),(0.0574322859849621,
0.0593504322721664,0.0708131666834375,0.0765445338890731,0.0822759010947087,
0.105201369917251,0.139589573151064,0.151052307562335,0.173977776384878,
0.185440510796149,0.19690324520742,0.208365979618691,0.219828714029962,
0.225560081235598,0.242754182852504),.UNSPECIFIED.);
#497=B_SPLINE_CURVE_WITH_KNOTS('',3,(#28583,#28584,#28585,#28586,#28587,
#28588,#28589,#28590,#28591,#28592,#28593,#28594,#28595,#28596,#28597,#28598,
#28599),.UNSPECIFIED.,.F.,.F.,(4,1,1,1,1,1,1,1,1,1,1,1,1,1,4),(0.,0.0325780266935636,
0.0434373689247514,0.0651560533871272,0.086874737849503,0.119452764543067,
0.173749475699006,0.195468160161382,0.217186844623757,0.238905529086133,
0.249764871317321,0.260624213548509,0.30406158247326,0.347498951398012,
0.35078480449443),.UNSPECIFIED.);
#498=B_SPLINE_CURVE_WITH_KNOTS('',3,(#28603,#28604,#28605,#28606,#28607,
#28608,#28609,#28610),.UNSPECIFIED.,.F.,.F.,(4,2,2,4),(0.000125698572975419,
0.227792182462144,0.286179225344766,0.357965061381181),.UNSPECIFIED.);
#499=B_SPLINE_CURVE_WITH_KNOTS('',3,(#28614,#28615,#28616,#28617,#28618,
#28619,#28620,#28621,#28622,#28623,#28624,#28625,#28626,#28627,#28628),
 .UNSPECIFIED.,.F.,.F.,(4,1,1,1,1,1,1,1,1,1,1,1,4),(0.,0.032581311307726,
0.0434417484103013,0.065162622615452,0.0868834968206025,0.119464808128328,
0.173766993641205,0.195487867846356,0.217208742051506,0.260650490461807,
0.304092238872109,0.34753398728241,0.350846347076693),.UNSPECIFIED.);
#500=B_SPLINE_CURVE_WITH_KNOTS('',3,(#28632,#28633,#28634,#28635,#28636,
#28637),.UNSPECIFIED.,.F.,.F.,(4,2,4),(6.30123959129944E-5,0.28662538597019,
0.558744736279564),.UNSPECIFIED.);
#501=B_SPLINE_CURVE_WITH_KNOTS('',3,(#28641,#28642,#28643,#28644,#28645,
#28646,#28647,#28648,#28649,#28650,#28651,#28652,#28653,#28654,#28655,#28656,
#28657),.UNSPECIFIED.,.F.,.F.,(4,1,1,1,1,1,1,1,1,1,1,1,1,1,4),(0.,0.0325813112990995,
0.0434417483987993,0.065162622598199,0.0868834967975986,0.108604370996998,
0.119464808096698,0.173766993595197,0.217208741993997,0.260650490392796,
0.282371364592195,0.304092238791595,0.325813112990995,0.347533987190394,
0.350818585035077),.UNSPECIFIED.);
#502=B_SPLINE_CURVE_WITH_KNOTS('',3,(#28661,#28662,#28663,#28664,#28665,
#28666),.UNSPECIFIED.,.F.,.F.,(4,2,4),(8.10097431310763E-5,0.0939376681945024,
0.135055213019345),.UNSPECIFIED.);
#503=B_SPLINE_CURVE_WITH_KNOTS('',3,(#28670,#28671,#28672,#28673,#28674,
#28675,#28676,#28677,#28678,#28679,#28680,#28681,#28682,#28683,#28684,#28685,
#28686),.UNSPECIFIED.,.F.,.F.,(4,1,1,1,1,1,1,1,1,1,1,1,2,4),(0.,0.0325813113113254,
0.0434417484151006,0.0543021855188758,0.0651626226226509,0.0868834968302012,
0.108604371037751,0.130325245245302,0.173766993660402,0.238929616283053,
0.260650490490603,0.304092238905704,0.347533987320804,0.350868951891457),
 .UNSPECIFIED.);
#504=B_SPLINE_CURVE_WITH_KNOTS('',3,(#28690,#28691,#28692,#28693,#28694,
#28695),.UNSPECIFIED.,.F.,.F.,(4,2,4),(9.94409432394449E-5,0.227746038346159,
0.389493151962301),.UNSPECIFIED.);
#505=B_SPLINE_CURVE_WITH_KNOTS('',3,(#28699,#28700,#28701,#28702,#28703,
#28704,#28705,#28706,#28707,#28708,#28709,#28710,#28711,#28712,#28713,#28714,
#28715),.UNSPECIFIED.,.F.,.F.,(4,1,1,1,1,1,1,1,1,1,1,1,1,1,4),(0.,0.0325813113011869,
0.0434417484015825,0.0651626226023737,0.0868834968031649,0.119464808104352,
0.17376699360633,0.195487867807121,0.260650490409495,0.27151092750989,0.282371364610286,
0.304092238811077,0.325813113011869,0.34753398721266,0.350822431972601),
 .UNSPECIFIED.);
#506=B_SPLINE_CURVE_WITH_KNOTS('',3,(#28719,#28720,#28721,#28722,#28723,
#28724),.UNSPECIFIED.,.F.,.F.,(4,2,4),(5.13423395914222E-5,0.227662696235558,
0.386226851134491),.UNSPECIFIED.);
#507=B_SPLINE_CURVE_WITH_KNOTS('',3,(#28728,#28729,#28730,#28731,#28732,
#28733,#28734,#28735,#28736,#28737,#28738,#28739,#28740,#28741,#28742,#28743),
 .UNSPECIFIED.,.F.,.F.,(4,1,1,1,1,1,1,1,1,1,1,1,1,4),(0.,0.0325813113000667,
0.0434417484000888,0.0651626226001333,0.0868834968001777,0.108604371000222,
0.152046119400311,0.173766993600355,0.184627430700377,0.238929616200488,
0.260650490400533,0.282371364600577,0.347533987200711,0.35081085871336),
 .UNSPECIFIED.);
#508=B_SPLINE_CURVE_WITH_KNOTS('',3,(#28747,#28748,#28749,#28750,#28751,
#28752,#28753,#28754,#28755,#28756,#28757,#28758,#28759,#28760,#28761,#28762,
#28763,#28764,#28765,#28766,#28767,#28768,#28769,#28770,#28771,#28772,#28773,
#28774,#28775,#28776,#28777,#28778,#28779,#28780,#28781,#28782,#28783),
 .UNSPECIFIED.,.F.,.F.,(4,3,3,3,3,3,3,3,3,3,3,3,4),(0.000120425573379091,
0.00317624209811181,0.034923100327543,0.0622117780158951,0.0875829757712474,
0.0998257630783663,0.112050473037524,0.149386931156097,0.162459268273195,
0.176536957109724,0.194439588055033,0.206018741387147,0.264230255678867),
 .UNSPECIFIED.);
#509=B_SPLINE_CURVE_WITH_KNOTS('',3,(#28787,#28788,#28789,#28790,#28791,
#28792,#28793,#28794,#28795,#28796,#28797,#28798,#28799,#28800,#28801,#28802,
#28803,#28804),.UNSPECIFIED.,.F.,.F.,(4,1,1,1,1,1,1,1,1,1,1,1,1,1,1,4),
(0.,0.0325751931318221,0.0434335908424294,0.0651503862636442,0.0868671816848588,
0.0977255793954661,0.108583977106074,0.119442374816681,0.173734363369718,
0.217167954212147,0.238884749633362,0.260601545054576,0.282318340475791,
0.325751931318221,0.347468726739435,0.350792906271863),.UNSPECIFIED.);
#510=B_SPLINE_CURVE_WITH_KNOTS('',3,(#28808,#28809,#28810,#28811,#28812,
#28813,#28814,#28815,#28816,#28817),.UNSPECIFIED.,.F.,.F.,(4,2,2,2,4),(2.68015753038539E-5,
0.146332244518046,0.219070648592723,0.270822325009499,0.340813208551893),
 .UNSPECIFIED.);
#511=B_SPLINE_CURVE_WITH_KNOTS('',3,(#28821,#28822,#28823,#28824,#28825,
#28826,#28827,#28828,#28829,#28830,#28831,#28832,#28833,#28834),
 .UNSPECIFIED.,.F.,.F.,(4,1,1,1,1,1,1,1,1,1,1,4),(0.,0.0325788513687624,
0.0434384684916831,0.0651577027375248,0.0868769369833663,0.119455788352129,
0.173753873966733,0.206332725335495,0.238911576704257,0.260630810950099,
0.347507747933465,0.35083610433132),.UNSPECIFIED.);
#512=B_SPLINE_CURVE_WITH_KNOTS('',3,(#28838,#28839,#28840,#28841,#28842,
#28843),.UNSPECIFIED.,.F.,.F.,(4,2,4),(4.81243928056727E-5,0.094951878313684,
0.175392450319733),.UNSPECIFIED.);
#513=B_SPLINE_CURVE_WITH_KNOTS('',3,(#28847,#28848,#28849,#28850,#28851,
#28852,#28853,#28854,#28855,#28856,#28857,#28858,#28859,#28860,#28861),
 .UNSPECIFIED.,.F.,.F.,(4,1,1,1,1,1,1,1,1,1,1,1,4),(0.,0.0325813112935661,
0.0434417483914214,0.0651626225871322,0.0868834967828429,0.108604370978554,
0.173766993565686,0.195487867761397,0.217208741957107,0.260650490348529,
0.30409223873995,0.347533987131372,0.350868951700208),.UNSPECIFIED.);
#514=B_SPLINE_CURVE_WITH_KNOTS('',3,(#28865,#28866,#28867,#28868,#28869,
#28870,#28871,#28872,#28873,#28874,#28875,#28876,#28877,#28878,#28879,#28880,
#28881,#28882,#28883,#28884,#28885,#28886,#28887,#28888,#28889,#28890,#28891,
#28892,#28893,#28894,#28895,#28896,#28897,#28898,#28899,#28900,#28901,#28902,
#28903,#28904,#28905,#28906,#28907,#28908,#28909,#28910,#28911,#28912,#28913,
#28914,#28915,#28916),.UNSPECIFIED.,.F.,.F.,(4,3,3,3,3,3,3,3,3,3,3,3,3,
3,3,3,3,4),(2.08975011247579E-5,0.00308607105095766,0.0215396517126696,
0.0405802381433016,0.0599061205553268,0.0800477842295079,0.100708814480148,
0.122385505337789,0.169065775168934,0.2240388208304,0.240016854106345,0.276817460735969,
0.299181834597421,0.36391927474236,0.406482599347405,0.447325093929158,
0.482679027142275,0.593863693098499),.UNSPECIFIED.);
#515=B_SPLINE_CURVE_WITH_KNOTS('',3,(#28920,#28921,#28922,#28923,#28924,
#28925,#28926,#28927,#28928,#28929,#28930,#28931,#28932,#28933,#28934),
 .UNSPECIFIED.,.F.,.F.,(4,1,1,1,1,1,1,1,1,1,1,1,4),(0.,0.0325813113014245,
0.0434417484018993,0.065162622602849,0.0868834968037986,0.108604371004748,
0.173766993607597,0.195487867808547,0.217208742009496,0.260650490411396,
0.304092238813295,0.347533987215194,0.350868415382151),.UNSPECIFIED.);
#516=B_SPLINE_CURVE_WITH_KNOTS('',3,(#28938,#28939,#28940,#28941,#28942,
#28943,#28944,#28945,#28946,#28947,#28948,#28949,#28950,#28951,#28952,#28953,
#28954,#28955,#28956,#28957,#28958,#28959,#28960,#28961,#28962,#28963,#28964,
#28965,#28966,#28967,#28968,#28969,#28970,#28971,#28972,#28973,#28974,#28975,
#28976,#28977),.UNSPECIFIED.,.F.,.F.,(4,3,3,3,3,3,3,3,3,3,3,3,3,4),(1.8132500310452E-5,
0.00304106400815239,0.0495323610481579,0.0633408111336385,0.0700209626369159,
0.0898911299380531,0.116220295863278,0.151110195365111,0.166467059445078,
0.17462226984871,0.194444744111124,0.224081832239665,0.235151757120569,
0.271406539154298),.UNSPECIFIED.);
#517=B_SPLINE_CURVE_WITH_KNOTS('',3,(#28981,#28982,#28983,#28984,#28985,
#28986,#28987,#28988,#28989,#28990,#28991,#28992,#28993,#28994,#28995,#28996,
#28997),.UNSPECIFIED.,.F.,.F.,(4,1,1,1,1,1,1,1,1,1,1,1,1,1,4),(0.,0.0325813113088777,
0.0434417484118369,0.0651626226177552,0.0868834968236736,0.119464808132551,
0.173766993647347,0.195487867853266,0.260650490471021,0.27151092757398,
0.282371364676939,0.304092238882858,0.325813113088776,0.347533987294695,
0.350822723223362),.UNSPECIFIED.);
#518=B_SPLINE_CURVE_WITH_KNOTS('',3,(#29001,#29002,#29003,#29004,#29005,
#29006),.UNSPECIFIED.,.F.,.F.,(4,2,4),(7.69577465685739E-5,0.0940098568691888,
0.135160714322205),.UNSPECIFIED.);
#519=B_SPLINE_CURVE_WITH_KNOTS('',3,(#29010,#29011,#29012,#29013,#29014,
#29015,#29016,#29017,#29018,#29019,#29020,#29021,#29022,#29023,#29024,#29025,
#29026,#29027),.UNSPECIFIED.,.F.,.F.,(4,1,1,1,1,1,1,1,1,1,1,1,1,1,1,4),
(0.,0.0325813113041659,0.0434417484055545,0.0651626226083318,0.086883496811109,
0.108604371013886,0.130325245216663,0.173766993622218,0.23892961623055,
0.260650490433327,0.282371364636104,0.304092238838881,0.31495267594027,
0.325813113041659,0.347533987244436,0.350814109544273),.UNSPECIFIED.);
#520=B_SPLINE_CURVE_WITH_KNOTS('',3,(#29031,#29032,#29033,#29034,#29035,
#29036,#29037,#29038),.UNSPECIFIED.,.F.,.F.,(4,2,2,4),(3.31139120221695E-5,
0.227629525449843,0.255364348773956,0.28456350304073),.UNSPECIFIED.);
#521=B_SPLINE_CURVE_WITH_KNOTS('',3,(#29042,#29043,#29044,#29045,#29046,
#29047,#29048,#29049,#29050,#29051,#29052,#29053,#29054,#29055,#29056,#29057,
#29058),.UNSPECIFIED.,.F.,.F.,(4,1,1,1,1,1,1,1,1,1,1,1,1,1,4),(0.,0.0325813112927442,
0.0434417483903256,0.0651626225854883,0.0868834967806511,0.119464808073395,
0.173766993561302,0.195487867756465,0.217208741951628,0.23892961614679,
0.249790053244372,0.260650490341953,0.304092238732279,0.347533987122604,
0.350819280994235),.UNSPECIFIED.);
#522=B_SPLINE_CURVE_WITH_KNOTS('',3,(#29062,#29063,#29064,#29065,#29066,
#29067,#29068,#29069),.UNSPECIFIED.,.F.,.F.,(4,2,2,4),(8.75783588774737E-5,
0.227723333688707,0.267086083002731,0.303951261502786),.UNSPECIFIED.);
#523=B_SPLINE_CURVE_WITH_KNOTS('',3,(#29073,#29074,#29075,#29076,#29077,
#29078,#29079,#29080,#29081,#29082,#29083,#29084,#29085,#29086,#29087),
 .UNSPECIFIED.,.F.,.F.,(4,1,1,1,1,1,1,1,1,1,1,1,4),(0.,0.0325811092953062,
0.0434414790604082,0.0651622185906124,0.0868829581208164,0.119464067416123,
0.173765916241633,0.195486655771837,0.206347025536939,0.260648874362449,
0.304090353422858,0.347531832483266,0.350844600598755),.UNSPECIFIED.);
#524=B_SPLINE_CURVE_WITH_KNOTS('',3,(#29091,#29092,#29093,#29094,#29095,
#29096,#29097,#29098),.UNSPECIFIED.,.F.,.F.,(4,2,2,4),(2.27200726371039E-5,
0.231955136446205,0.488819014410125,1.2898502229429),.UNSPECIFIED.);
#525=B_SPLINE_CURVE_WITH_KNOTS('',3,(#29102,#29103,#29104,#29105,#29106,
#29107,#29108,#29109,#29110,#29111,#29112,#29113,#29114,#29115,#29116,#29117,
#29118),.UNSPECIFIED.,.F.,.F.,(4,1,1,1,1,1,1,1,1,1,1,1,1,1,4),(0.,0.0325779980334532,
0.043437330711271,0.0651559960669065,0.0868746614225421,0.119452659455995,
0.173749322845084,0.19546798820072,0.217186653556355,0.238905318911991,
0.249764651589808,0.260623984267626,0.304061314978897,0.347498645690168,
0.350781901481053),.UNSPECIFIED.);
#526=B_SPLINE_CURVE_WITH_KNOTS('',3,(#29122,#29123,#29124,#29125,#29126,
#29127,#29128,#29129,#29130,#29131,#29132,#29133,#29134,#29135,#29136,#29137,
#29138,#29139,#29140,#29141,#29142,#29143,#29144,#29145,#29146,#29147,#29148,
#29149,#29150,#29151,#29152,#29153,#29154,#29155,#29156,#29157,#29158,#29159,
#29160,#29161,#29162,#29163,#29164,#29165,#29166,#29167,#29168,#29169,#29170),
 .UNSPECIFIED.,.F.,.F.,(4,3,3,3,3,3,3,3,3,3,3,3,3,3,3,3,4),(1.37553095906785E-6,
0.00304386864164244,0.0381582824207633,0.0424078913534377,0.0550000496558162,
0.0634874491076403,0.0677090991850859,0.0718883344512816,0.139202166901755,
0.175799272796621,0.200576190294692,0.220626076332347,0.243429823456619,
0.289644318509875,0.337908382119408,0.363805344557365,0.456456048950493),
 .UNSPECIFIED.);
#527=B_SPLINE_CURVE_WITH_KNOTS('',3,(#29174,#29175,#29176,#29177,#29178,
#29179,#29180,#29181,#29182,#29183,#29184,#29185,#29186,#29187,#29188,#29189,
#29190,#29191),.UNSPECIFIED.,.F.,.F.,(4,1,1,1,1,1,1,1,1,1,1,1,1,1,1,4),
(0.,0.0325780266754328,0.043437368900577,0.0651560533508656,0.0868747378011541,
0.108593422251443,0.130312106701731,0.173749475602308,0.217186844502885,
0.260624213403462,0.271483555628607,0.282342897853751,0.304061582304039,
0.325780266754328,0.347498951204616,0.350807062835108),.UNSPECIFIED.);
#528=B_SPLINE_CURVE_WITH_KNOTS('',3,(#29195,#29196,#29197,#29198,#29199,
#29200,#29201,#29202,#29203,#29204,#29205,#29206,#29207,#29208,#29209,#29210,
#29211,#29212,#29213,#29214,#29215,#29216,#29217,#29218,#29219,#29220,#29221,
#29222,#29223,#29224,#29225,#29226,#29227,#29228,#29229,#29230,#29231,#29232,
#29233,#29234,#29235,#29236,#29237,#29238,#29239,#29240,#29241,#29242,#29243),
 .UNSPECIFIED.,.F.,.F.,(4,3,3,3,3,3,3,3,3,3,3,3,3,3,3,3,4),(0.,0.00302406508941641,
0.0395522621603711,0.057705333245643,0.0759815108224394,0.0940426303547463,
0.112199213405293,0.148158415042036,0.184110455163659,0.202070811707743,
0.211010109764078,0.219889141985247,0.237220260655798,0.25240704224699,
0.259630849810946,0.267667276481433,0.284994839229281),.UNSPECIFIED.);
#529=B_SPLINE_CURVE_WITH_KNOTS('',3,(#29247,#29248,#29249,#29250,#29251,
#29252,#29253,#29254,#29255,#29256,#29257,#29258,#29259,#29260,#29261,#29262,
#29263,#29264),.UNSPECIFIED.,.F.,.F.,(4,1,1,1,1,1,1,1,1,1,1,1,1,1,1,4),
(0.,0.0325813113104041,0.0434417484138721,0.0651626226208082,0.0868834968277442,
0.10860437103468,0.130325245241616,0.173766993655489,0.217208742069361,
0.260650490483233,0.271510927586701,0.282371364690169,0.304092238897105,
0.325813113104041,0.347533987310977,0.350830458492577),.UNSPECIFIED.);
#530=B_SPLINE_CURVE_WITH_KNOTS('',3,(#29268,#29269,#29270,#29271,#29272,
#29273,#29274,#29275),.UNSPECIFIED.,.F.,.F.,(4,2,2,4),(5.39325034638232E-5,
0.227672425891551,0.267374517425262,0.303028644711899),.UNSPECIFIED.);
#531=B_SPLINE_CURVE_WITH_KNOTS('',3,(#29279,#29280,#29281,#29282,#29283,
#29284,#29285,#29286,#29287,#29288,#29289,#29290,#29291,#29292,#29293,#29294,
#29295,#29296,#29297,#29298,#29299),.UNSPECIFIED.,.F.,.F.,(4,1,1,1,1,1,
1,1,1,1,1,1,1,1,1,1,1,1,4),(0.,0.0217208741937073,0.0325813112905609,0.0434417483874145,
0.0651626225811218,0.086883496774829,0.0923137153232559,0.0977439338716826,
0.108604370968536,0.130325245162244,0.173766993549658,0.206348304840219,
0.217208741937072,0.23892961613078,0.260650490324487,0.282371364518194,
0.304092238711901,0.347533987099316,0.350868951667842),.UNSPECIFIED.);
#532=B_SPLINE_CURVE_WITH_KNOTS('',3,(#29303,#29304,#29305,#29306,#29307,
#29308,#29309,#29310),.UNSPECIFIED.,.F.,.F.,(4,2,2,4),(5.31032778941324E-5,
0.227671003125575,0.267370133098792,0.303019957630964),.UNSPECIFIED.);
#533=B_SPLINE_CURVE_WITH_KNOTS('',3,(#29314,#29315,#29316,#29317,#29318,
#29319,#29320,#29321,#29322,#29323,#29324,#29325,#29326,#29327,#29328,#29329,
#29330,#29331),.UNSPECIFIED.,.F.,.F.,(4,1,1,1,1,1,1,1,1,1,1,1,1,1,1,4),
(0.,0.0325813112956053,0.0434417483941404,0.0651626225912106,0.0868834967882808,
0.108604370985351,0.130325245182421,0.173766993576562,0.260650490364843,
0.304092238758983,0.306807348033617,0.309522457308251,0.314952675857518,
0.325813112956053,0.347533987153123,0.350847650043364),.UNSPECIFIED.);
#534=B_SPLINE_CURVE_WITH_KNOTS('',3,(#29335,#29336,#29337,#29338,#29339,
#29340,#29341,#29342,#29343,#29344,#29345,#29346,#29347,#29348,#29349,#29350,
#29351,#29352,#29353,#29354,#29355,#29356,#29357,#29358,#29359,#29360,#29361,
#29362,#29363,#29364,#29365,#29366,#29367,#29368,#29369,#29370,#29371,#29372,
#29373,#29374,#29375,#29376,#29377,#29378,#29379,#29380,#29381,#29382,#29383,
#29384,#29385,#29386,#29387,#29388,#29389),.UNSPECIFIED.,.F.,.F.,(4,3,3,
3,3,3,3,3,3,3,3,3,3,3,3,3,3,3,4),(1.69664194135058E-5,0.00307114277356412,
0.039585456561102,0.0486449755101495,0.0576877261582512,0.066879541498318,
0.0714617073426762,0.0759954470654279,0.0940893974202715,0.112206315525557,
0.148186601031976,0.184109848624511,0.20206634187012,0.211006462456386,
0.219884740867183,0.239823962825612,0.267679208993222,0.27814146155332,
0.312441926852791),.UNSPECIFIED.);
#535=B_SPLINE_CURVE_WITH_KNOTS('',3,(#29393,#29394,#29395,#29396,#29397,
#29398,#29399,#29400,#29401,#29402,#29403,#29404,#29405,#29406,#29407,#29408,
#29409,#29410,#29411),.UNSPECIFIED.,.F.,.F.,(4,1,1,1,1,1,1,1,1,1,1,1,1,
1,1,1,4),(0.,0.0325813112998826,0.0434417483998435,0.0651626225997652,0.0868834967996869,
0.108604370999609,0.13032524519953,0.173766993599374,0.184627430699335,
0.217208741999217,0.260650490399061,0.271510927499021,0.282371364598982,
0.304092238798904,0.325813112998826,0.347533987198747,0.350820570359218),
 .UNSPECIFIED.);
#536=B_SPLINE_CURVE_WITH_KNOTS('',3,(#29415,#29416,#29417,#29418,#29419,
#29420,#29421,#29422),.UNSPECIFIED.,.F.,.F.,(4,2,2,4),(0.,0.227561771076043,
0.271281179207273,0.310769966142806),.UNSPECIFIED.);
#537=B_SPLINE_CURVE_WITH_KNOTS('',3,(#29426,#29427,#29428,#29429,#29430,
#29431,#29432,#29433,#29434,#29435,#29436,#29437,#29438,#29439,#29440,#29441,
#29442,#29443,#29444),.UNSPECIFIED.,.F.,.F.,(4,1,1,1,1,1,1,1,1,1,1,1,1,
1,1,1,4),(0.,0.0325813112989154,0.0434417483985538,0.0651626225978307,0.0868834967971076,
0.108604370996385,0.130325245195661,0.173766993594215,0.184627430693854,
0.217208741992769,0.260650490391323,0.271510927490961,0.2823713645906,0.304092238789877,
0.325813112989153,0.34753398718843,0.350819913879885),.UNSPECIFIED.);
#538=B_SPLINE_CURVE_WITH_KNOTS('',3,(#29922,#29923,#29924,#29925,#29926,
#29927,#29928,#29929,#29930,#29931,#29932,#29933,#29934,#29935),
 .UNSPECIFIED.,.F.,.F.,(4,2,2,2,2,2,4),(0.0377143719414213,0.167070624995476,
0.336553194126115,0.499999999999991,0.663446805873868,0.832929375004528,
0.962285628058582),.UNSPECIFIED.);
#539=B_SPLINE_CURVE_WITH_KNOTS('',3,(#29937,#29938,#29939,#29940,#29941,
#29942,#29943,#29944,#29945,#29946),.UNSPECIFIED.,.F.,.F.,(4,2,2,2,4),(6.02998356774229E-5,
0.0827092794731852,0.124915109661161,0.159012423184403,0.16290738863864),
 .UNSPECIFIED.);
#540=B_SPLINE_CURVE_WITH_KNOTS('',3,(#29948,#29949,#29950,#29951,#29952,
#29953),.UNSPECIFIED.,.F.,.F.,(4,2,4),(1.00681757910309E-6,0.198376055662081,
0.616164391347873),.UNSPECIFIED.);
#541=B_SPLINE_CURVE_WITH_KNOTS('',3,(#29955,#29956,#29957,#29958,#29959,
#29960,#29961,#29962,#29963,#29964,#29965,#29966,#29967,#29968),
 .UNSPECIFIED.,.F.,.F.,(4,2,2,2,2,2,4),(-1.3697495952833,-1.10023259323731,
-0.875123171455467,-0.683367626235548,-0.492293828139748,-0.265579528785075,
-1.00032822303378E-6),.UNSPECIFIED.);
#542=B_SPLINE_CURVE_WITH_KNOTS('',3,(#29970,#29971,#29972,#29973,#29974,
#29975),.UNSPECIFIED.,.F.,.F.,(4,2,4),(2.07957879669281E-5,0.198544173877694,
0.338081838894613),.UNSPECIFIED.);
#543=B_SPLINE_CURVE_WITH_KNOTS('',3,(#29976,#29977,#29978,#29979,#29980,
#29981),.UNSPECIFIED.,.F.,.F.,(4,2,4),(7.3985770635887E-13,0.0834659910448719,
0.124630945443496),.UNSPECIFIED.);
#544=B_SPLINE_CURVE_WITH_KNOTS('',3,(#30038,#30039,#30040,#30041,#30042,
#30043,#30044,#30045,#30046,#30047,#30048,#30049,#30050,#30051),
 .UNSPECIFIED.,.F.,.F.,(4,2,2,2,2,2,4),(0.0377143719414213,0.167070624995476,
0.336553194126115,0.499999999999991,0.663446805873868,0.832929375004528,
0.962285628058582),.UNSPECIFIED.);
#545=B_SPLINE_CURVE_WITH_KNOTS('',3,(#30571,#30572,#30573,#30574,#30575,
#30576),.UNSPECIFIED.,.F.,.F.,(4,2,4),(2.29474227301907E-5,0.0820321645242487,
0.127086402594844),.UNSPECIFIED.);
#546=B_SPLINE_CURVE_WITH_KNOTS('',3,(#30578,#30579,#30580,#30581,#30582,
#30583,#30584,#30585,#30586,#30587),.UNSPECIFIED.,.F.,.F.,(4,2,2,2,4),(1.0015711071698E-6,
0.191278795792421,0.38757373555012,0.491221092732434,0.551410070798975),
 .UNSPECIFIED.);
#547=B_SPLINE_CURVE_WITH_KNOTS('',3,(#30589,#30590,#30591,#30592,#30593,
#30594,#30595,#30596,#30597,#30598,#30599,#30600,#30601,#30602),
 .UNSPECIFIED.,.F.,.F.,(4,2,2,2,2,2,4),(-1.35492578021256,-1.08827021184037,
-0.865791397536503,-0.676241847501408,-0.487357773086443,-0.263174151541431,
-1.00020091572966E-6),.UNSPECIFIED.);
#548=B_SPLINE_CURVE_WITH_KNOTS('',3,(#30604,#30605,#30606,#30607,#30608,
#30609),.UNSPECIFIED.,.F.,.F.,(4,2,4),(0.000114833391804824,0.165073300431955,
0.25614615827788),.UNSPECIFIED.);
#549=B_SPLINE_CURVE_WITH_KNOTS('',3,(#30610,#30611,#30612,#30613,#30614,
#30615),.UNSPECIFIED.,.F.,.F.,(4,2,4),(2.21353696645175E-12,0.0812321189495927,
0.187083951430582),.UNSPECIFIED.);
#550=B_SPLINE_CURVE_WITH_KNOTS('',3,(#30619,#30620,#30621,#30622,#30623,
#30624),.UNSPECIFIED.,.F.,.F.,(4,2,4),(2.9238385461313E-5,0.103447066749674,
0.163628142816379),.UNSPECIFIED.);
#551=B_SPLINE_CURVE_WITH_KNOTS('',3,(#30628,#30629,#30630,#30631,#30632,
#30633,#30634,#30635),.UNSPECIFIED.,.F.,.F.,(4,2,2,4),(1.0058637232954E-6,
0.195653995077043,0.273235261095345,0.534959287266804),.UNSPECIFIED.);
#552=B_SPLINE_CURVE_WITH_KNOTS('',3,(#30639,#30640,#30641,#30642,#30643,
#30644,#30645,#30646,#30647,#30648,#30649,#30650,#30651,#30652),
 .UNSPECIFIED.,.F.,.F.,(4,2,2,2,2,2,4),(-1.36676454451703,-1.09824091081614,
-0.873519748019839,-0.682131120567347,-0.491400640516798,-0.264972088549723,
-1.00035032482767E-6),.UNSPECIFIED.);
#553=B_SPLINE_CURVE_WITH_KNOTS('',3,(#30656,#30657,#30658,#30659,#30660,
#30661),.UNSPECIFIED.,.F.,.F.,(4,2,4),(0.000130181004474716,0.209368508323579,
0.347593165933443),.UNSPECIFIED.);
#554=B_SPLINE_CURVE_WITH_KNOTS('',3,(#30663,#30664,#30665,#30666,#30667,
#30668),.UNSPECIFIED.,.F.,.F.,(4,2,4),(4.22281107869509E-12,0.0949552245569479,
0.178548392329359),.UNSPECIFIED.);
#555=B_SPLINE_CURVE_WITH_KNOTS('',3,(#31173,#31174,#31175,#31176,#31177,
#31178,#31179,#31180,#31181,#31182,#31183,#31184,#31185,#31186),
 .UNSPECIFIED.,.F.,.F.,(4,2,2,2,2,2,4),(0.0377143719414213,0.167070624995476,
0.336553194126115,0.499999999999991,0.663446805873868,0.832929375004528,
0.962285628058582),.UNSPECIFIED.);
#556=B_SPLINE_CURVE_WITH_KNOTS('',3,(#31188,#31189,#31190,#31191,#31192,
#31193,#31194,#31195,#31196,#31197),.UNSPECIFIED.,.F.,.F.,(4,2,2,2,4),(6.27818039135639E-5,
0.082188319328403,0.124361031846954,0.160510990515046,0.165279378877141),
 .UNSPECIFIED.);
#557=B_SPLINE_CURVE_WITH_KNOTS('',3,(#31199,#31200,#31201,#31202,#31203,
#31204,#31205,#31206,#31207,#31208),.UNSPECIFIED.,.F.,.F.,(4,2,2,2,4),(1.00120787235036E-6,
0.178106589831891,0.361003049087605,0.458246244320469,0.518090207569899),
 .UNSPECIFIED.);
#558=B_SPLINE_CURVE_WITH_KNOTS('',3,(#31210,#31211,#31212,#31213,#31214,
#31215,#31216,#31217,#31218,#31219,#31220,#31221,#31222,#31223),
 .UNSPECIFIED.,.F.,.F.,(4,2,2,2,2,2,4),(-1.35451776762616,-1.08791731812649,
-0.865511022534625,-0.676038029847498,-0.48722621698279,-0.263105347394021,
-1.00024492573328E-6),.UNSPECIFIED.);
#559=B_SPLINE_CURVE_WITH_KNOTS('',3,(#31225,#31226,#31227,#31228,#31229,
#31230),.UNSPECIFIED.,.F.,.F.,(4,2,4),(5.14867016416543E-5,0.195132654327356,
0.330523874257241),.UNSPECIFIED.);
#560=B_SPLINE_CURVE_WITH_KNOTS('',3,(#31231,#31232,#31233,#31234,#31235,
#31236),.UNSPECIFIED.,.F.,.F.,(4,2,4),(2.74483044490136E-12,0.0801886121002409,
0.134391643166566),.UNSPECIFIED.);
#561=B_SPLINE_CURVE_WITH_KNOTS('',3,(#31293,#31294,#31295,#31296,#31297,
#31298,#31299,#31300,#31301,#31302,#31303,#31304,#31305,#31306),
 .UNSPECIFIED.,.F.,.F.,(4,2,2,2,2,2,4),(0.0377143719414213,0.167070624995476,
0.336553194126115,0.499999999999991,0.663446805873868,0.832929375004528,
0.962285628058582),.UNSPECIFIED.);
#562=B_SPLINE_CURVE_WITH_KNOTS('',3,(#31882,#31883,#31884,#31885,#31886,
#31887),.UNSPECIFIED.,.F.,.F.,(4,2,4),(3.83144405905161E-5,0.0820775777658897,
0.163588942869382),.UNSPECIFIED.);
#563=B_SPLINE_CURVE_WITH_KNOTS('',3,(#31889,#31890,#31891,#31892,#31893,
#31894,#31895,#31896,#31897,#31898),.UNSPECIFIED.,.F.,.F.,(4,2,2,2,4),(1.00111834067745E-6,
0.176745823297941,0.356256554433591,0.450695302353019,0.510467153062589),
 .UNSPECIFIED.);
#564=B_SPLINE_CURVE_WITH_KNOTS('',3,(#31900,#31901,#31902,#31903,#31904,
#31905,#31906,#31907,#31908,#31909,#31910,#31911,#31912,#31913),
 .UNSPECIFIED.,.F.,.F.,(4,2,2,2,2,2,4),(-1.35467512487212,-1.08805555198913,
-0.865672785184554,-0.676085696250677,-0.487155925003567,-0.26302937099976,
-1.00022677660484E-6),.UNSPECIFIED.);
#565=B_SPLINE_CURVE_WITH_KNOTS('',3,(#31915,#31916,#31917,#31918,#31919,
#31920),.UNSPECIFIED.,.F.,.F.,(4,2,4),(7.5428832328408E-5,0.105663039185365,
0.180626596448931),.UNSPECIFIED.);
#566=B_SPLINE_CURVE_WITH_KNOTS('',3,(#31921,#31922,#31923,#31924,#31925,
#31926,#31927,#31928,#31929,#31930),.UNSPECIFIED.,.F.,.F.,(4,2,2,2,4),(0.,
0.0810373126568711,0.0959717664713932,0.101312246402759,0.103448648415402),
 .UNSPECIFIED.);
#567=B_SPLINE_CURVE_WITH_KNOTS('',3,(#32458,#32459,#32460,#32461,#32462,
#32463,#32464,#32465,#32466,#32467,#32468,#32469,#32470,#32471),
 .UNSPECIFIED.,.F.,.F.,(4,2,2,2,2,2,4),(0.0377143719414213,0.167070624995476,
0.336553194126115,0.499999999999991,0.663446805873868,0.832929375004528,
0.962285628058582),.UNSPECIFIED.);
#568=B_SPLINE_CURVE_WITH_KNOTS('',3,(#32473,#32474,#32475,#32476,#32477,
#32478,#32479,#32480,#32481,#32482),.UNSPECIFIED.,.F.,.F.,(4,2,2,2,4),(6.00642358182352E-5,
0.0821817544261252,0.124362812830404,0.160530644634858,0.165303570917889),
 .UNSPECIFIED.);
#569=B_SPLINE_CURVE_WITH_KNOTS('',3,(#32484,#32485,#32486,#32487,#32488,
#32489,#32490,#32491,#32492,#32493),.UNSPECIFIED.,.F.,.F.,(4,2,2,2,4),(1.0012084904056E-6,
0.178254736450577,0.361162889837382,0.457988221849768,0.519343329924884),
 .UNSPECIFIED.);
#570=B_SPLINE_CURVE_WITH_KNOTS('',3,(#32495,#32496,#32497,#32498,#32499,
#32500,#32501,#32502,#32503,#32504,#32505,#32506,#32507,#32508),
 .UNSPECIFIED.,.F.,.F.,(4,2,2,2,2,2,4),(-1.35452989588837,-1.08792747113547,
-0.865519548823138,-0.676043361721358,-0.487228090638011,-0.263104534485106,
-1.00024503859763E-6),.UNSPECIFIED.);
#571=B_SPLINE_CURVE_WITH_KNOTS('',3,(#32510,#32511,#32512,#32513,#32514,
#32515),.UNSPECIFIED.,.F.,.F.,(4,2,4),(4.84470832014495E-5,0.182163199855647,
0.304984269132144),.UNSPECIFIED.);
#572=B_SPLINE_CURVE_WITH_KNOTS('',3,(#32516,#32517,#32518,#32519,#32520,
#32521),.UNSPECIFIED.,.F.,.F.,(4,2,4),(3.76146522406052E-12,0.0801875735797784,
0.135807623237589),.UNSPECIFIED.);
#573=B_SPLINE_CURVE_WITH_KNOTS('',3,(#32578,#32579,#32580,#32581,#32582,
#32583,#32584,#32585,#32586,#32587,#32588,#32589,#32590,#32591),
 .UNSPECIFIED.,.F.,.F.,(4,2,2,2,2,2,4),(0.0377143719414213,0.167070624995476,
0.336553194126115,0.499999999999991,0.663446805873868,0.832929375004528,
0.962285628058582),.UNSPECIFIED.);
#574=B_SPLINE_CURVE_WITH_KNOTS('',3,(#33251,#33252,#33253,#33254,#33255,
#33256),.UNSPECIFIED.,.F.,.F.,(4,2,4),(5.09831611999352E-6,0.0820253557161963,
0.163612440508287),.UNSPECIFIED.);
#575=B_SPLINE_CURVE_WITH_KNOTS('',3,(#33258,#33259,#33260,#33261,#33262,
#33263),.UNSPECIFIED.,.F.,.F.,(4,2,4),(1.00115786546793E-6,0.203270398076333,
0.655123139928109),.UNSPECIFIED.);
#576=B_SPLINE_CURVE_WITH_KNOTS('',3,(#33265,#33266,#33267,#33268,#33269,
#33270,#33271,#33272,#33273,#33274,#33275,#33276,#33277,#33278),
 .UNSPECIFIED.,.F.,.F.,(4,2,2,2,2,2,4),(-1.35341451706435,-1.08670028936229,
-0.86441625397775,-0.675525209241787,-0.487228648686942,-0.263116926873662,
-1.00023452885085E-6),.UNSPECIFIED.);
#577=B_SPLINE_CURVE_WITH_KNOTS('',3,(#33280,#33281,#33282,#33283,#33284,
#33285),.UNSPECIFIED.,.F.,.F.,(4,2,4),(8.06566033118487E-5,0.235791800547026,
0.430083034163372),.UNSPECIFIED.);
#578=B_SPLINE_CURVE_WITH_KNOTS('',3,(#33286,#33287,#33288,#33289,#33290,
#33291,#33292,#33293,#33294,#33295),.UNSPECIFIED.,.F.,.F.,(4,2,2,2,4),(0.,
0.0811226560809443,0.105916017129699,0.119512712641936,0.124075141076686),
 .UNSPECIFIED.);
#579=B_SPLINE_CURVE_WITH_KNOTS('',3,(#33865,#33866,#33867,#33868,#33869,
#33870,#33871,#33872,#33873,#33874,#33875,#33876,#33877,#33878),
 .UNSPECIFIED.,.F.,.F.,(4,2,2,2,2,2,4),(0.0377143719414213,0.167070624995476,
0.336553194126115,0.499999999999991,0.663446805873868,0.832929375004528,
0.962285628058582),.UNSPECIFIED.);
#580=B_SPLINE_CURVE_WITH_KNOTS('',3,(#33880,#33881,#33882,#33883,#33884,
#33885,#33886,#33887),.UNSPECIFIED.,.F.,.F.,(4,2,2,4),(3.90292133962738E-5,
0.0821103706390817,0.159792128481933,0.163589006475625),.UNSPECIFIED.);
#581=B_SPLINE_CURVE_WITH_KNOTS('',3,(#33889,#33890,#33891,#33892,#33893,
#33894),.UNSPECIFIED.,.F.,.F.,(4,2,4),(1.00679590137882E-6,0.198428655308229,
0.616220686425556),.UNSPECIFIED.);
#582=B_SPLINE_CURVE_WITH_KNOTS('',3,(#33896,#33897,#33898,#33899,#33900,
#33901,#33902,#33903,#33904,#33905,#33906,#33907,#33908,#33909),
 .UNSPECIFIED.,.F.,.F.,(4,2,2,2,2,2,4),(-1.36946436726572,-1.09993796007104,
-0.87483524085704,-0.683080422126019,-0.492004958736434,-0.265277755647832,
-1.00032716612113E-6),.UNSPECIFIED.);
#583=B_SPLINE_CURVE_WITH_KNOTS('',3,(#33911,#33912,#33913,#33914,#33915,
#33916),.UNSPECIFIED.,.F.,.F.,(4,2,4),(5.26674620364727E-6,0.201391218966152,
0.343250429838191),.UNSPECIFIED.);
#584=B_SPLINE_CURVE_WITH_KNOTS('',3,(#33917,#33918,#33919,#33920,#33921,
#33922),.UNSPECIFIED.,.F.,.F.,(4,2,4),(5.79777279590719E-12,0.0800737732076016,
0.153868907149876),.UNSPECIFIED.);
#585=B_SPLINE_CURVE_WITH_KNOTS('',3,(#33979,#33980,#33981,#33982,#33983,
#33984,#33985,#33986,#33987,#33988,#33989,#33990,#33991,#33992),
 .UNSPECIFIED.,.F.,.F.,(4,2,2,2,2,2,4),(0.0377143719414213,0.167070624995476,
0.336553194126115,0.499999999999991,0.663446805873868,0.832929375004528,
0.962285628058582),.UNSPECIFIED.);
#586=B_SPLINE_CURVE_WITH_KNOTS('',3,(#34442,#34443,#34444,#34445,#34446,
#34447,#34448,#34449),.UNSPECIFIED.,.F.,.F.,(4,2,2,4),(6.73894020493833E-6,
0.0820391933763412,0.122258941274579,0.165103583903822),.UNSPECIFIED.);
#587=B_SPLINE_CURVE_WITH_KNOTS('',3,(#34451,#34452,#34453,#34454,#34455,
#34456),.UNSPECIFIED.,.F.,.F.,(4,2,4),(1.00575280131252E-6,0.196998295881173,
0.611676358684534),.UNSPECIFIED.);
#588=B_SPLINE_CURVE_WITH_KNOTS('',3,(#34458,#34459,#34460,#34461,#34462,
#34463,#34464,#34465,#34466,#34467,#34468,#34469,#34470,#34471),
 .UNSPECIFIED.,.F.,.F.,(4,2,2,2,2,2,4),(-1.36653537100014,-1.09810186112548,
-0.873434408555324,-0.682043594538526,-0.49131851038635,-0.264945371797465,
-1.00034356989698E-6),.UNSPECIFIED.);
#589=B_SPLINE_CURVE_WITH_KNOTS('',3,(#34473,#34474,#34475,#34476,#34477,
#34478),.UNSPECIFIED.,.F.,.F.,(4,2,4),(8.77479325007996E-5,0.221380284319995,
0.382793527514749),.UNSPECIFIED.);
#590=B_SPLINE_CURVE_WITH_KNOTS('',3,(#34479,#34480,#34481,#34482,#34483,
#34484,#34485,#34486),.UNSPECIFIED.,.F.,.F.,(4,2,2,4),(2.39130355285181E-13,
0.0351374765588485,0.0713576360411048,0.114209460841156),.UNSPECIFIED.);
#591=B_SPLINE_CURVE_WITH_KNOTS('',3,(#35154,#35155,#35156,#35157,#35158,
#35159,#35160,#35161,#35162,#35163,#35164,#35165,#35166,#35167),
 .UNSPECIFIED.,.F.,.F.,(4,2,2,2,2,2,4),(0.0377143719414213,0.167070624995476,
0.336553194126115,0.499999999999991,0.663446805873868,0.832929375004528,
0.962285628058582),.UNSPECIFIED.);
#592=B_SPLINE_CURVE_WITH_KNOTS('',3,(#35169,#35170,#35171,#35172,#35173,
#35174),.UNSPECIFIED.,.F.,.F.,(4,2,4),(1.24525365641064E-5,0.0820262168893432,
0.163512197605749),.UNSPECIFIED.);
#593=B_SPLINE_CURVE_WITH_KNOTS('',3,(#35176,#35177,#35178,#35179,#35180,
#35181),.UNSPECIFIED.,.F.,.F.,(4,2,4),(1.00040793070525E-6,0.173262947876778,
0.559558397335178),.UNSPECIFIED.);
#594=B_SPLINE_CURVE_WITH_KNOTS('',3,(#35183,#35184,#35185,#35186,#35187,
#35188,#35189,#35190,#35191,#35192,#35193,#35194,#35195,#35196),
 .UNSPECIFIED.,.F.,.F.,(4,2,2,2,2,2,4),(-1.35063028345454,-1.08468537305046,
-0.862939535319615,-0.674245622212526,-0.486174128017263,-0.262647316233601,
-1.00009146822194E-6),.UNSPECIFIED.);
#595=B_SPLINE_CURVE_WITH_KNOTS('',3,(#35198,#35199,#35200,#35201,#35202,
#35203),.UNSPECIFIED.,.F.,.F.,(4,2,4),(1.936890280024E-5,0.202772428402345,
0.388563110243199),.UNSPECIFIED.);
#596=B_SPLINE_CURVE_WITH_KNOTS('',3,(#35204,#35205,#35206,#35207,#35208,
#35209,#35210,#35211),.UNSPECIFIED.,.F.,.F.,(4,2,2,4),(0.,0.00386300464665212,
0.0800231995509174,0.130453162506101),.UNSPECIFIED.);
#597=B_SPLINE_CURVE_WITH_KNOTS('',3,(#35268,#35269,#35270,#35271,#35272,
#35273,#35274,#35275,#35276,#35277,#35278,#35279,#35280,#35281),
 .UNSPECIFIED.,.F.,.F.,(4,2,2,2,2,2,4),(0.0377143719414213,0.167070624995476,
0.336553194126115,0.499999999999991,0.663446805873868,0.832929375004528,
0.962285628058582),.UNSPECIFIED.);
#598=B_SPLINE_CURVE_WITH_KNOTS('',3,(#35731,#35732,#35733,#35734,#35735,
#35736,#35737,#35738),.UNSPECIFIED.,.F.,.F.,(4,2,2,4),(6.90400899849116E-6,
0.0820395128145215,0.122259153116005,0.165101582267905),.UNSPECIFIED.);
#599=B_SPLINE_CURVE_WITH_KNOTS('',3,(#35740,#35741,#35742,#35743,#35744,
#35745),.UNSPECIFIED.,.F.,.F.,(4,2,4),(1.00575513369814E-6,0.196994699755262,
0.611609770297254),.UNSPECIFIED.);
#600=B_SPLINE_CURVE_WITH_KNOTS('',3,(#35747,#35748,#35749,#35750,#35751,
#35752,#35753,#35754,#35755,#35756,#35757,#35758,#35759,#35760),
 .UNSPECIFIED.,.F.,.F.,(4,2,2,2,2,2,4),(-1.36653731681659,-1.09810214381664,
-0.873434196730641,-0.682044304096007,-0.49132017893128,-0.264946970986512,
-1.00034369628633E-6),.UNSPECIFIED.);
#601=B_SPLINE_CURVE_WITH_KNOTS('',3,(#35762,#35763,#35764,#35765,#35766,
#35767),.UNSPECIFIED.,.F.,.F.,(4,2,4),(8.89329850189062E-5,0.221868589758904,
0.38383585754025),.UNSPECIFIED.);
#602=B_SPLINE_CURVE_WITH_KNOTS('',3,(#35768,#35769,#35770,#35771,#35772,
#35773,#35774,#35775),.UNSPECIFIED.,.F.,.F.,(4,2,2,4),(2.40826726029524E-12,
0.0351391314154969,0.0713608565247239,0.114146477814614),.UNSPECIFIED.);
#603=B_SPLINE_CURVE_WITH_KNOTS('',3,(#36261,#36262,#36263,#36264,#36265,
#36266,#36267,#36268,#36269,#36270,#36271,#36272,#36273,#36274),
 .UNSPECIFIED.,.F.,.F.,(4,2,2,2,2,2,4),(0.0377143719414213,0.167070624995476,
0.336553194126115,0.499999999999991,0.663446805873868,0.832929375004528,
0.962285628058582),.UNSPECIFIED.);
#604=B_SPLINE_CURVE_WITH_KNOTS('',3,(#36276,#36277,#36278,#36279,#36280,
#36281,#36282,#36283,#36284,#36285,#36286,#36287),.UNSPECIFIED.,.F.,.F.,
(4,2,2,2,2,4),(6.06953724766298E-5,0.0723177934624636,0.142586707446175,
0.189383971247134,0.229663834041465,0.234960972274723),.UNSPECIFIED.);
#605=B_SPLINE_CURVE_WITH_KNOTS('',3,(#36289,#36290,#36291,#36292,#36293,
#36294),.UNSPECIFIED.,.F.,.F.,(4,2,4),(1.00681844603221E-6,0.198376306856705,
0.616167083390173),.UNSPECIFIED.);
#606=B_SPLINE_CURVE_WITH_KNOTS('',3,(#36296,#36297,#36298,#36299,#36300,
#36301,#36302,#36303,#36304,#36305,#36306,#36307,#36308,#36309),
 .UNSPECIFIED.,.F.,.F.,(4,2,2,2,2,2,4),(-1.36975063911396,-1.10023328664463,
-0.875123658513123,-0.683368107151748,-0.492294313860235,-0.26558001556176,
-1.0003282794275E-6),.UNSPECIFIED.);
#607=B_SPLINE_CURVE_WITH_KNOTS('',3,(#36311,#36312,#36313,#36314,#36315,
#36316),.UNSPECIFIED.,.F.,.F.,(4,2,4),(2.03029926476926E-5,0.199101046105406,
0.339123960645439),.UNSPECIFIED.);
#608=B_SPLINE_CURVE_WITH_KNOTS('',3,(#36317,#36318,#36319,#36320,#36321,
#36322),.UNSPECIFIED.,.F.,.F.,(4,2,4),(0.,0.0801741784244009,0.133244087202315),
 .UNSPECIFIED.);
#609=B_SPLINE_CURVE_WITH_KNOTS('',3,(#36379,#36380,#36381,#36382,#36383,
#36384,#36385,#36386,#36387,#36388,#36389,#36390,#36391,#36392),
 .UNSPECIFIED.,.F.,.F.,(4,2,2,2,2,2,4),(0.0377143719414213,0.167070624995476,
0.336553194126115,0.499999999999991,0.663446805873868,0.832929375004528,
0.962285628058582),.UNSPECIFIED.);
#610=B_SPLINE_CURVE_WITH_KNOTS('',3,(#37010,#37011,#37012,#37013,#37014,
#37015,#37016,#37017),.UNSPECIFIED.,.F.,.F.,(4,2,2,4),(2.12328689868991E-5,
0.0820465025813729,0.0975804088568552,0.0980854119622017),.UNSPECIFIED.);
#611=B_SPLINE_CURVE_WITH_KNOTS('',3,(#37019,#37020,#37021,#37022,#37023,
#37024,#37025,#37026,#37027,#37028),.UNSPECIFIED.,.F.,.F.,(4,2,2,2,4),(1.00120754304711E-6,
0.180563424164471,0.364157287903267,0.442097033926019,0.497873685697995),
 .UNSPECIFIED.);
#612=B_SPLINE_CURVE_WITH_KNOTS('',3,(#37030,#37031,#37032,#37033,#37034,
#37035,#37036,#37037,#37038,#37039,#37040,#37041,#37042,#37043),
 .UNSPECIFIED.,.F.,.F.,(4,2,2,2,2,2,4),(-1.35482880152986,-1.08819875332802,
-0.865789686987352,-0.676162724939522,-0.487193738484184,-0.263042222431825,
-1.00024482310964E-6),.UNSPECIFIED.);
#613=B_SPLINE_CURVE_WITH_KNOTS('',3,(#37045,#37046,#37047,#37048,#37049,
#37050),.UNSPECIFIED.,.F.,.F.,(4,2,4),(4.92544827602823E-5,0.177705442380597,
0.325738385748943),.UNSPECIFIED.);
#614=B_SPLINE_CURVE_WITH_KNOTS('',3,(#37051,#37052,#37053,#37054,#37055,
#37056,#37057,#37058),.UNSPECIFIED.,.F.,.F.,(4,2,2,4),(0.,0.00483273455720385,
0.0810988666945897,0.131043136461057),.UNSPECIFIED.);
#615=B_SPLINE_CURVE_WITH_KNOTS('',3,(#37530,#37531,#37532,#37533,#37534,
#37535,#37536,#37537,#37538,#37539,#37540,#37541,#37542,#37543),
 .UNSPECIFIED.,.F.,.F.,(4,2,2,2,2,2,4),(0.0377143719414213,0.167070624995476,
0.336553194126115,0.499999999999991,0.663446805873868,0.832929375004528,
0.962285628058582),.UNSPECIFIED.);
#616=B_SPLINE_CURVE_WITH_KNOTS('',3,(#37545,#37546,#37547,#37548,#37549,
#37550,#37551,#37552),.UNSPECIFIED.,.F.,.F.,(4,2,2,4),(5.42376165162044E-5,
0.0821643460301592,0.213267550478571,0.227565828155254),.UNSPECIFIED.);
#617=B_SPLINE_CURVE_WITH_KNOTS('',3,(#37554,#37555,#37556,#37557,#37558,
#37559),.UNSPECIFIED.,.F.,.F.,(4,2,4),(1.00681606646651E-6,0.198408681306464,
0.616468624198531),.UNSPECIFIED.);
#618=B_SPLINE_CURVE_WITH_KNOTS('',3,(#37561,#37562,#37563,#37564,#37565,
#37566,#37567,#37568,#37569,#37570,#37571,#37572,#37573,#37574),
 .UNSPECIFIED.,.F.,.F.,(4,2,2,2,2,2,4),(-1.36977192354957,-1.10024954678324,
-0.875138273537566,-0.68337946038512,-0.492301827559948,-0.265581063709854,
-1.00032816558492E-6),.UNSPECIFIED.);
#619=B_SPLINE_CURVE_WITH_KNOTS('',3,(#37576,#37577,#37578,#37579,#37580,
#37581),.UNSPECIFIED.,.F.,.F.,(4,2,4),(5.21624935227409E-6,0.197869989680169,
0.3367373897978),.UNSPECIFIED.);
#620=B_SPLINE_CURVE_WITH_KNOTS('',3,(#37582,#37583,#37584,#37585,#37586,
#37587),.UNSPECIFIED.,.F.,.F.,(4,2,4),(1.02764932528255E-12,0.0801413076023557,
0.194331925601292),.UNSPECIFIED.);
#621=B_SPLINE_CURVE_WITH_KNOTS('',3,(#37644,#37645,#37646,#37647,#37648,
#37649,#37650,#37651,#37652,#37653,#37654,#37655,#37656,#37657),
 .UNSPECIFIED.,.F.,.F.,(4,2,2,2,2,2,4),(0.0377143719414213,0.167070624995476,
0.336553194126115,0.499999999999991,0.663446805873868,0.832929375004528,
0.962285628058582),.UNSPECIFIED.);
#622=B_SPLINE_CURVE_WITH_KNOTS('',3,(#38121,#38122,#38123,#38124,#38125,
#38126),.UNSPECIFIED.,.F.,.F.,(4,2,4),(1.3375296468513E-5,0.118849802950364,
0.770735236720951),.UNSPECIFIED.);
#623=B_SPLINE_CURVE_WITH_KNOTS('',3,(#38128,#38129,#38130,#38131,#38132,
#38133),.UNSPECIFIED.,.F.,.F.,(4,2,4),(1.00583908498562E-6,0.197083724989951,
0.612585872513722),.UNSPECIFIED.);
#624=B_SPLINE_CURVE_WITH_KNOTS('',3,(#38135,#38136,#38137,#38138,#38139,
#38140,#38141,#38142,#38143,#38144,#38145,#38146,#38147,#38148),
 .UNSPECIFIED.,.F.,.F.,(4,2,2,2,2,2,4),(-1.36677954016887,-1.09825974558988,
-0.873545667521562,-0.682153185342683,-0.491418884621818,-0.264981806425049,
-1.00034871381864E-6),.UNSPECIFIED.);
#625=B_SPLINE_CURVE_WITH_KNOTS('',3,(#38150,#38151,#38152,#38153,#38154,
#38155),.UNSPECIFIED.,.F.,.F.,(4,2,4),(2.0131697178417E-5,0.188528940513233,
0.322027145962636),.UNSPECIFIED.);
#626=B_SPLINE_CURVE_WITH_KNOTS('',3,(#38156,#38157,#38158,#38159,#38160,
#38161),.UNSPECIFIED.,.F.,.F.,(4,2,4),(5.18698018589852E-13,0.0829527696225184,
0.126881817845898),.UNSPECIFIED.);
#627=B_SPLINE_CURVE_WITH_KNOTS('',3,(#38577,#38578,#38579,#38580,#38581,
#38582,#38583,#38584,#38585,#38586,#38587,#38588,#38589,#38590),
 .UNSPECIFIED.,.F.,.F.,(4,2,2,2,2,2,4),(0.0377143719414213,0.167070624995476,
0.336553194126115,0.499999999999991,0.663446805873868,0.832929375004528,
0.962285628058582),.UNSPECIFIED.);
#628=B_SPLINE_CURVE_WITH_KNOTS('',3,(#38592,#38593,#38594,#38595,#38596,
#38597),.UNSPECIFIED.,.F.,.F.,(4,2,4),(3.25283738680958E-5,0.0575600610182617,
0.119710480217137),.UNSPECIFIED.);
#629=B_SPLINE_CURVE_WITH_KNOTS('',3,(#38599,#38600,#38601,#38602,#38603,
#38604),.UNSPECIFIED.,.F.,.F.,(4,2,4),(1.00574980111111E-6,0.196438860777099,
0.615936660954388),.UNSPECIFIED.);
#630=B_SPLINE_CURVE_WITH_KNOTS('',3,(#38606,#38607,#38608,#38609,#38610,
#38611,#38612,#38613,#38614,#38615,#38616,#38617,#38618,#38619),
 .UNSPECIFIED.,.F.,.F.,(4,2,2,2,2,2,4),(-1.36646497173156,-1.09803036534575,
-0.873371570921259,-0.682007908066334,-0.491310112387284,-0.264951815991902,
-1.00034338197123E-6),.UNSPECIFIED.);
#631=B_SPLINE_CURVE_WITH_KNOTS('',3,(#38621,#38622,#38623,#38624,#38625,
#38626),.UNSPECIFIED.,.F.,.F.,(4,2,4),(8.95077426275264E-5,0.213418487477568,
0.347676401385313),.UNSPECIFIED.);
#632=B_SPLINE_CURVE_WITH_KNOTS('',3,(#38627,#38628,#38629,#38630,#38631,
#38632),.UNSPECIFIED.,.F.,.F.,(4,2,4),(5.71589455049436E-13,0.0829410743851074,
0.160131049736526),.UNSPECIFIED.);
#633=B_SPLINE_CURVE_WITH_KNOTS('',3,(#38689,#38690,#38691,#38692,#38693,
#38694,#38695,#38696,#38697,#38698,#38699,#38700,#38701,#38702),
 .UNSPECIFIED.,.F.,.F.,(4,2,2,2,2,2,4),(0.0377143719414213,0.167070624995476,
0.336553194126115,0.499999999999991,0.663446805873868,0.832929375004528,
0.962285628058582),.UNSPECIFIED.);
#634=B_SPLINE_CURVE_WITH_KNOTS('',3,(#39194,#39195,#39196,#39197,#39198,
#39199,#39200,#39201),.UNSPECIFIED.,.F.,.F.,(4,2,2,4),(5.63653703654061E-6,
0.0819976592555741,0.0994840943119498,0.110621668417563),.UNSPECIFIED.);
#635=B_SPLINE_CURVE_WITH_KNOTS('',3,(#39203,#39204,#39205,#39206,#39207,
#39208),.UNSPECIFIED.,.F.,.F.,(4,2,4),(1.00578674459647E-6,0.196744693440733,
0.608070001195422),.UNSPECIFIED.);
#636=B_SPLINE_CURVE_WITH_KNOTS('',3,(#39210,#39211,#39212,#39213,#39214,
#39215,#39216,#39217,#39218,#39219,#39220,#39221,#39222,#39223),
 .UNSPECIFIED.,.F.,.F.,(4,2,2,2,2,2,4),(-1.36654018190171,-1.09811194514787,
-0.873433001188821,-0.682044964262726,-0.491323861095133,-0.264952627419438,
-1.00034558310118E-6),.UNSPECIFIED.);
#637=B_SPLINE_CURVE_WITH_KNOTS('',3,(#39225,#39226,#39227,#39228,#39229,
#39230),.UNSPECIFIED.,.F.,.F.,(4,2,4),(7.36982883605742E-6,0.21182056227566,
0.362967551660399),.UNSPECIFIED.);
#638=B_SPLINE_CURVE_WITH_KNOTS('',3,(#39231,#39232,#39233,#39234,#39235,
#39236,#39237,#39238),.UNSPECIFIED.,.F.,.F.,(4,2,2,4),(3.36762946852576E-12,
0.0811207756408513,0.121444988164551,0.192000399014979),.UNSPECIFIED.);
#639=B_SPLINE_CURVE_WITH_KNOTS('',3,(#39752,#39753,#39754,#39755,#39756,
#39757,#39758,#39759,#39760,#39761,#39762,#39763,#39764,#39765),
 .UNSPECIFIED.,.F.,.F.,(4,2,2,2,2,2,4),(0.0377143719414213,0.167070624995476,
0.336553194126115,0.499999999999991,0.663446805873868,0.832929375004528,
0.962285628058582),.UNSPECIFIED.);
#640=B_SPLINE_CURVE_WITH_KNOTS('',3,(#39767,#39768,#39769,#39770,#39771,
#39772,#39773,#39774),.UNSPECIFIED.,.F.,.F.,(4,2,2,4),(6.08478568690021E-5,
0.0749500177471191,0.137874692765321,0.214092945323678),.UNSPECIFIED.);
#641=B_SPLINE_CURVE_WITH_KNOTS('',3,(#39776,#39777,#39778,#39779,#39780,
#39781),.UNSPECIFIED.,.F.,.F.,(4,2,4),(1.00674948340903E-6,0.19860241559806,
0.616969018247203),.UNSPECIFIED.);
#642=B_SPLINE_CURVE_WITH_KNOTS('',3,(#39783,#39784,#39785,#39786,#39787,
#39788,#39789,#39790,#39791,#39792,#39793,#39794,#39795,#39796),
 .UNSPECIFIED.,.F.,.F.,(4,2,2,2,2,2,4),(-1.36942885849635,-1.09990630423119,
-0.874813906835148,-0.683066677551954,-0.491998067801788,-0.265271812378102,
-1.00032494267263E-6),.UNSPECIFIED.);
#643=B_SPLINE_CURVE_WITH_KNOTS('',3,(#39798,#39799,#39800,#39801,#39802,
#39803),.UNSPECIFIED.,.F.,.F.,(4,2,4),(2.26430690219157E-5,0.201402499858342,
0.343296266574079),.UNSPECIFIED.);
#644=B_SPLINE_CURVE_WITH_KNOTS('',3,(#39804,#39805,#39806,#39807,#39808,
#39809,#39810,#39811),.UNSPECIFIED.,.F.,.F.,(4,2,2,4),(1.74684428518018E-12,
0.0522340767156272,0.136645058339451,0.231738878590132),.UNSPECIFIED.);
#645=B_SPLINE_CURVE_WITH_KNOTS('',3,(#39868,#39869,#39870,#39871,#39872,
#39873,#39874,#39875,#39876,#39877,#39878,#39879,#39880,#39881),
 .UNSPECIFIED.,.F.,.F.,(4,2,2,2,2,2,4),(0.0377143719414213,0.167070624995476,
0.336553194126115,0.499999999999991,0.663446805873868,0.832929375004528,
0.962285628058582),.UNSPECIFIED.);
#646=B_SPLINE_CURVE_WITH_KNOTS('',3,(#40443,#40444,#40445,#40446,#40447,
#40448),.UNSPECIFIED.,.F.,.F.,(4,2,4),(3.99306793426499E-5,0.0820843888608893,
0.163582789889144),.UNSPECIFIED.);
#647=B_SPLINE_CURVE_WITH_KNOTS('',3,(#40450,#40451,#40452,#40453,#40454,
#40455,#40456,#40457,#40458,#40459),.UNSPECIFIED.,.F.,.F.,(4,2,2,2,4),(1.001144715258E-6,
0.176544129782838,0.356948476219595,0.452196137824933,0.511488742402409),
 .UNSPECIFIED.);
#648=B_SPLINE_CURVE_WITH_KNOTS('',3,(#40461,#40462,#40463,#40464,#40465,
#40466,#40467,#40468,#40469,#40470,#40471,#40472,#40473,#40474),
 .UNSPECIFIED.,.F.,.F.,(4,2,2,2,2,2,4),(-1.35478963372027,-1.08811184962075,
-0.865669720728692,-0.676143977124964,-0.487271283253805,-0.263087029256964,
-1.00023212990909E-6),.UNSPECIFIED.);
#649=B_SPLINE_CURVE_WITH_KNOTS('',3,(#40476,#40477,#40478,#40479,#40480,
#40481),.UNSPECIFIED.,.F.,.F.,(4,2,4),(6.51111114373825E-5,0.197951050690941,
0.363934107919122),.UNSPECIFIED.);
#650=B_SPLINE_CURVE_WITH_KNOTS('',3,(#40482,#40483,#40484,#40485,#40486,
#40487),.UNSPECIFIED.,.F.,.F.,(4,2,4),(0.,0.0810433266429397,0.145890417857538),
 .UNSPECIFIED.);
#651=B_SPLINE_CURVE_WITH_KNOTS('',3,(#40903,#40904,#40905,#40906,#40907,
#40908,#40909,#40910,#40911,#40912,#40913,#40914,#40915,#40916),
 .UNSPECIFIED.,.F.,.F.,(4,2,2,2,2,2,4),(0.0377143719414213,0.167070624995476,
0.336553194126115,0.499999999999991,0.663446805873868,0.832929375004528,
0.962285628058582),.UNSPECIFIED.);
#652=B_SPLINE_CURVE_WITH_KNOTS('',3,(#40918,#40919,#40920,#40921,#40922,
#40923),.UNSPECIFIED.,.F.,.F.,(4,2,4),(3.20283895616613E-5,0.0586306467901465,
0.121642806585947),.UNSPECIFIED.);
#653=B_SPLINE_CURVE_WITH_KNOTS('',3,(#40925,#40926,#40927,#40928,#40929,
#40930),.UNSPECIFIED.,.F.,.F.,(4,2,4),(1.00574695584138E-6,0.196441563595188,
0.616027525838472),.UNSPECIFIED.);
#654=B_SPLINE_CURVE_WITH_KNOTS('',3,(#40932,#40933,#40934,#40935,#40936,
#40937,#40938,#40939,#40940,#40941,#40942,#40943,#40944,#40945),
 .UNSPECIFIED.,.F.,.F.,(4,2,2,2,2,2,4),(-1.36646292126098,-1.09803107097949,
-0.873372841577203,-0.682007267078294,-0.491307511055257,-0.264949168082375,
-1.00034321282837E-6),.UNSPECIFIED.);
#655=B_SPLINE_CURVE_WITH_KNOTS('',3,(#40947,#40948,#40949,#40950,#40951,
#40952),.UNSPECIFIED.,.F.,.F.,(4,2,4),(8.66234192869361E-5,0.213329487663992,
0.347531973651816),.UNSPECIFIED.);
#656=B_SPLINE_CURVE_WITH_KNOTS('',3,(#40953,#40954,#40955,#40956,#40957,
#40958),.UNSPECIFIED.,.F.,.F.,(4,2,4),(8.38585718100273E-13,0.0801874437919323,
0.160125031278999),.UNSPECIFIED.);
#657=B_SPLINE_CURVE_WITH_KNOTS('',3,(#41015,#41016,#41017,#41018,#41019,
#41020,#41021,#41022,#41023,#41024,#41025,#41026,#41027,#41028),
 .UNSPECIFIED.,.F.,.F.,(4,2,2,2,2,2,4),(0.0377143719414213,0.167070624995476,
0.336553194126115,0.499999999999991,0.663446805873868,0.832929375004528,
0.962285628058582),.UNSPECIFIED.);
#658=B_SPLINE_CURVE_WITH_KNOTS('',3,(#41548,#41549,#41550,#41551,#41552,
#41553),.UNSPECIFIED.,.F.,.F.,(4,2,4),(5.78796480941106E-6,0.0820241632572779,
0.0983326513668803),.UNSPECIFIED.);
#659=B_SPLINE_CURVE_WITH_KNOTS('',3,(#41555,#41556,#41557,#41558,#41559,
#41560),.UNSPECIFIED.,.F.,.F.,(4,2,4),(1.00111011279019E-6,0.20056691109568,
0.646408027829995),.UNSPECIFIED.);
#660=B_SPLINE_CURVE_WITH_KNOTS('',3,(#41562,#41563,#41564,#41565,#41566,
#41567,#41568,#41569,#41570,#41571,#41572,#41573,#41574,#41575),
 .UNSPECIFIED.,.F.,.F.,(4,2,2,2,2,2,4),(-1.35329688927434,-1.08662400245728,
-0.864362407604642,-0.675470253341474,-0.487172784036078,-0.263083584774088,
-1.0002248669823E-6),.UNSPECIFIED.);
#661=B_SPLINE_CURVE_WITH_KNOTS('',3,(#41577,#41578,#41579,#41580,#41581,
#41582),.UNSPECIFIED.,.F.,.F.,(4,2,4),(7.6238807513628E-5,0.428958911085021,
0.98234564450394),.UNSPECIFIED.);
#662=B_SPLINE_CURVE_WITH_KNOTS('',3,(#41583,#41584,#41585,#41586,#41587,
#41588),.UNSPECIFIED.,.F.,.F.,(4,2,4),(2.36314343156334E-13,0.0811159727681617,
0.112753130003149),.UNSPECIFIED.);
#663=B_SPLINE_CURVE_WITH_KNOTS('',3,(#42018,#42019,#42020,#42021,#42022,
#42023,#42024,#42025,#42026,#42027,#42028,#42029,#42030,#42031),
 .UNSPECIFIED.,.F.,.F.,(4,2,2,2,2,2,4),(0.0377143719414213,0.167070624995476,
0.336553194126115,0.499999999999991,0.663446805873868,0.832929375004528,
0.962285628058582),.UNSPECIFIED.);
#664=B_SPLINE_CURVE_WITH_KNOTS('',3,(#42033,#42034,#42035,#42036,#42037,
#42038),.UNSPECIFIED.,.F.,.F.,(4,2,4),(3.17996200538999E-5,0.0821085150301028,
0.156371486023489),.UNSPECIFIED.);
#665=B_SPLINE_CURVE_WITH_KNOTS('',3,(#42040,#42041,#42042,#42043,#42044,
#42045),.UNSPECIFIED.,.F.,.F.,(4,2,4),(1.00587720305493E-6,0.195537009167673,
0.606860770741171),.UNSPECIFIED.);
#666=B_SPLINE_CURVE_WITH_KNOTS('',3,(#42047,#42048,#42049,#42050,#42051,
#42052,#42053,#42054,#42055,#42056,#42057,#42058,#42059,#42060),
 .UNSPECIFIED.,.F.,.F.,(4,2,2,2,2,2,4),(-1.36641479922188,-1.09801466418853,
-0.87334685635933,-0.681977540546231,-0.491275627793233,-0.264940661371275,
-1.00035098939736E-6),.UNSPECIFIED.);
#667=B_SPLINE_CURVE_WITH_KNOTS('',3,(#42062,#42063,#42064,#42065,#42066,
#42067),.UNSPECIFIED.,.F.,.F.,(4,2,4),(8.49732544616001E-5,0.171599040272099,
0.274221646995865),.UNSPECIFIED.);
#668=B_SPLINE_CURVE_WITH_KNOTS('',3,(#42068,#42069,#42070,#42071,#42072,
#42073),.UNSPECIFIED.,.F.,.F.,(4,2,4),(0.,0.0802786247734464,0.181190612654646),
 .UNSPECIFIED.);
#669=B_SPLINE_CURVE_WITH_KNOTS('',3,(#42130,#42131,#42132,#42133,#42134,
#42135,#42136,#42137,#42138,#42139,#42140,#42141,#42142,#42143),
 .UNSPECIFIED.,.F.,.F.,(4,2,2,2,2,2,4),(0.0377143719414213,0.167070624995476,
0.336553194126115,0.499999999999991,0.663446805873868,0.832929375004528,
0.962285628058582),.UNSPECIFIED.);
#670=B_SPLINE_CURVE_WITH_KNOTS('',3,(#42509,#42510,#42511,#42512,#42513,
#42514),.UNSPECIFIED.,.F.,.F.,(4,2,4),(2.77418896662162E-5,0.0821040997741305,
0.185637111823654),.UNSPECIFIED.);
#671=B_SPLINE_CURVE_WITH_KNOTS('',3,(#42516,#42517,#42518,#42519,#42520,
#42521),.UNSPECIFIED.,.F.,.F.,(4,2,4),(1.00575954346815E-6,0.196733751213732,
0.608207148250796),.UNSPECIFIED.);
#672=B_SPLINE_CURVE_WITH_KNOTS('',3,(#42523,#42524,#42525,#42526,#42527,
#42528,#42529,#42530,#42531,#42532,#42533,#42534,#42535,#42536),
 .UNSPECIFIED.,.F.,.F.,(4,2,2,2,2,2,4),(-1.36645102810747,-1.09803162874758,
-0.873371647969155,-0.681999637833079,-0.491294686089601,-0.264941085845053,
-1.00034395944326E-6),.UNSPECIFIED.);
#673=B_SPLINE_CURVE_WITH_KNOTS('',3,(#42538,#42539,#42540,#42541,#42542,
#42543),.UNSPECIFIED.,.F.,.F.,(4,2,4),(4.6534746752922E-5,0.221801216668018,
0.383393535508176),.UNSPECIFIED.);
#674=B_SPLINE_CURVE_WITH_KNOTS('',3,(#42544,#42545,#42546,#42547,#42548,
#42549),.UNSPECIFIED.,.F.,.F.,(4,2,4),(9.75142074189076E-12,0.0812508942657999,
0.181132066940532),.UNSPECIFIED.);
#675=B_SPLINE_CURVE_WITH_KNOTS('',3,(#42979,#42980,#42981,#42982,#42983,
#42984,#42985,#42986,#42987,#42988,#42989,#42990,#42991,#42992),
 .UNSPECIFIED.,.F.,.F.,(4,2,2,2,2,2,4),(0.0377143719414213,0.167070624995476,
0.336553194126115,0.499999999999991,0.663446805873868,0.832929375004528,
0.962285628058582),.UNSPECIFIED.);
#676=B_SPLINE_CURVE_WITH_KNOTS('',3,(#42994,#42995,#42996,#42997,#42998,
#42999,#43000,#43001,#43002,#43003),.UNSPECIFIED.,.F.,.F.,(4,2,2,2,4),(5.42770356477153E-5,
0.082170276446433,0.124430513201584,0.160833130319759,0.165642154100829),
 .UNSPECIFIED.);
#677=B_SPLINE_CURVE_WITH_KNOTS('',3,(#43005,#43006,#43007,#43008,#43009,
#43010),.UNSPECIFIED.,.F.,.F.,(4,2,4),(1.00682002279841E-6,0.198152813321902,
0.615513442370215),.UNSPECIFIED.);
#678=B_SPLINE_CURVE_WITH_KNOTS('',3,(#43012,#43013,#43014,#43015,#43016,
#43017,#43018,#43019,#43020,#43021,#43022,#43023,#43024,#43025),
 .UNSPECIFIED.,.F.,.F.,(4,2,2,2,2,2,4),(-1.36965848181598,-1.10016097342675,
-0.875066628972613,-0.683316003615392,-0.492247655326726,-0.265550093286376,
-1.00032835407965E-6),.UNSPECIFIED.);
#679=B_SPLINE_CURVE_WITH_KNOTS('',3,(#43027,#43028,#43029,#43030,#43031,
#43032),.UNSPECIFIED.,.F.,.F.,(4,2,4),(2.80984943197878E-5,0.207705089179129,
0.35709509524869),.UNSPECIFIED.);
#680=B_SPLINE_CURVE_WITH_KNOTS('',3,(#43033,#43034,#43035,#43036,#43037,
#43038),.UNSPECIFIED.,.F.,.F.,(4,2,4),(2.92897079760619E-13,0.0802239228803233,
0.139498602952362),.UNSPECIFIED.);
#681=B_SPLINE_CURVE_WITH_KNOTS('',3,(#43095,#43096,#43097,#43098,#43099,
#43100,#43101,#43102,#43103,#43104,#43105,#43106,#43107,#43108),
 .UNSPECIFIED.,.F.,.F.,(4,2,2,2,2,2,4),(0.0377143719414213,0.167070624995476,
0.336553194126115,0.499999999999991,0.663446805873868,0.832929375004528,
0.962285628058582),.UNSPECIFIED.);
#682=B_SPLINE_CURVE_WITH_KNOTS('',3,(#43544,#43545,#43546,#43547,#43548,
#43549),.UNSPECIFIED.,.F.,.F.,(4,2,4),(3.61744708263467E-5,0.0820903485190886,
0.151462981409793),.UNSPECIFIED.);
#683=B_SPLINE_CURVE_WITH_KNOTS('',3,(#43551,#43552,#43553,#43554,#43555,
#43556),.UNSPECIFIED.,.F.,.F.,(4,2,4),(1.00682037581877E-6,0.198591576030872,
0.612057308716193),.UNSPECIFIED.);
#684=B_SPLINE_CURVE_WITH_KNOTS('',3,(#43558,#43559,#43560,#43561,#43562,
#43563,#43564,#43565,#43566,#43567,#43568,#43569,#43570,#43571),
 .UNSPECIFIED.,.F.,.F.,(4,2,2,2,2,2,4),(-1.36969550267109,-1.10017893246134,
-0.875088347365155,-0.683338633894847,-0.492266819638581,-0.265550398905338,
-1.00032836821468E-6),.UNSPECIFIED.);
#685=B_SPLINE_CURVE_WITH_KNOTS('',3,(#43573,#43574,#43575,#43576,#43577,
#43578),.UNSPECIFIED.,.F.,.F.,(4,2,4),(3.32639783591171E-5,0.197339009355241,
0.335420963807672),.UNSPECIFIED.);
#686=B_SPLINE_CURVE_WITH_KNOTS('',3,(#43579,#43580,#43581,#43582,#43583,
#43584),.UNSPECIFIED.,.F.,.F.,(4,2,4),(3.15044624714952E-12,0.0812340423540164,
0.130576380927272),.UNSPECIFIED.);
#687=B_SPLINE_CURVE_WITH_KNOTS('',3,(#44028,#44029,#44030,#44031,#44032,
#44033,#44034,#44035,#44036,#44037,#44038,#44039,#44040,#44041),
 .UNSPECIFIED.,.F.,.F.,(4,2,2,2,2,2,4),(0.0377143719414213,0.167070624995476,
0.336553194126115,0.499999999999991,0.663446805873868,0.832929375004528,
0.962285628058582),.UNSPECIFIED.);
#688=B_SPLINE_CURVE_WITH_KNOTS('',3,(#44043,#44044,#44045,#44046,#44047,
#44048,#44049,#44050),.UNSPECIFIED.,.F.,.F.,(4,2,2,4),(7.66815118875742E-6,
0.0719725088285606,0.133933240585685,0.207132823723994),.UNSPECIFIED.);
#689=B_SPLINE_CURVE_WITH_KNOTS('',3,(#44052,#44053,#44054,#44055,#44056,
#44057),.UNSPECIFIED.,.F.,.F.,(4,2,4),(1.00645408089785E-6,0.202058735386919,
0.625169506815927),.UNSPECIFIED.);
#690=B_SPLINE_CURVE_WITH_KNOTS('',3,(#44059,#44060,#44061,#44062,#44063,
#44064,#44065,#44066,#44067,#44068,#44069,#44070,#44071,#44072),
 .UNSPECIFIED.,.F.,.F.,(4,2,2,2,2,2,4),(-1.36982770647676,-1.10026801869593,
-0.875089073772716,-0.683242477348657,-0.492101062955115,-0.265280784052238,
-1.00031248059293E-6),.UNSPECIFIED.);
#691=B_SPLINE_CURVE_WITH_KNOTS('',3,(#44074,#44075,#44076,#44077,#44078,
#44079),.UNSPECIFIED.,.F.,.F.,(4,2,4),(7.21374248179772E-5,0.145937889148844,
0.224935975704918),.UNSPECIFIED.);
#692=B_SPLINE_CURVE_WITH_KNOTS('',3,(#44080,#44081,#44082,#44083,#44084,
#44085,#44086,#44087),.UNSPECIFIED.,.F.,.F.,(4,2,2,4),(0.,0.00388201731530571,
0.0800806715946951,0.130377783514938),.UNSPECIFIED.);
#693=B_SPLINE_CURVE_WITH_KNOTS('',3,(#44144,#44145,#44146,#44147,#44148,
#44149,#44150,#44151,#44152,#44153,#44154,#44155,#44156,#44157),
 .UNSPECIFIED.,.F.,.F.,(4,2,2,2,2,2,4),(0.0377143719414213,0.167070624995476,
0.336553194126115,0.499999999999991,0.663446805873868,0.832929375004528,
0.962285628058582),.UNSPECIFIED.);
#694=B_SPLINE_CURVE_WITH_KNOTS('',3,(#44649,#44650,#44651,#44652,#44653,
#44654),.UNSPECIFIED.,.F.,.F.,(4,2,4),(2.46231051897258E-5,0.0821382968673538,
0.159729243346244),.UNSPECIFIED.);
#695=B_SPLINE_CURVE_WITH_KNOTS('',3,(#44656,#44657,#44658,#44659,#44660,
#44661),.UNSPECIFIED.,.F.,.F.,(4,2,4),(1.00103827732456E-6,0.198279414012427,
0.639031973469237),.UNSPECIFIED.);
#696=B_SPLINE_CURVE_WITH_KNOTS('',3,(#44663,#44664,#44665,#44666,#44667,
#44668,#44669,#44670,#44671,#44672,#44673,#44674,#44675,#44676),
 .UNSPECIFIED.,.F.,.F.,(4,2,2,2,2,2,4),(-1.3530882309929,-1.08643200781697,
-0.864215538893404,-0.67536646667284,-0.487108134126014,-0.263052051794661,
-1.00022350183771E-6),.UNSPECIFIED.);
#697=B_SPLINE_CURVE_WITH_KNOTS('',3,(#44678,#44679,#44680,#44681,#44682,
#44683),.UNSPECIFIED.,.F.,.F.,(4,2,4),(7.89412222038307E-5,0.167932169494167,
0.297563614930367),.UNSPECIFIED.);
#698=B_SPLINE_CURVE_WITH_KNOTS('',3,(#44684,#44685,#44686,#44687,#44688,
#44689),.UNSPECIFIED.,.F.,.F.,(4,2,4),(3.26720990769784E-12,0.110549333290049,
0.163767498068542),.UNSPECIFIED.);
#699=B_SPLINE_CURVE_WITH_KNOTS('',3,(#45091,#45092,#45093,#45094,#45095,
#45096,#45097,#45098,#45099,#45100,#45101,#45102,#45103,#45104),
 .UNSPECIFIED.,.F.,.F.,(4,2,2,2,2,2,4),(0.0377143719414213,0.167070624995476,
0.336553194126115,0.499999999999991,0.663446805873868,0.832929375004528,
0.962285628058582),.UNSPECIFIED.);
#700=B_SPLINE_CURVE_WITH_KNOTS('',3,(#45106,#45107,#45108,#45109,#45110,
#45111),.UNSPECIFIED.,.F.,.F.,(4,2,4),(6.726102877353E-5,0.116989061547652,
0.697184527165448),.UNSPECIFIED.);
#701=B_SPLINE_CURVE_WITH_KNOTS('',3,(#45113,#45114,#45115,#45116,#45117,
#45118),.UNSPECIFIED.,.F.,.F.,(4,2,4),(1.00666090718109E-6,0.198552744294137,
0.618327596429947),.UNSPECIFIED.);
#702=B_SPLINE_CURVE_WITH_KNOTS('',3,(#45120,#45121,#45122,#45123,#45124,
#45125,#45126,#45127,#45128,#45129,#45130,#45131,#45132,#45133),
 .UNSPECIFIED.,.F.,.F.,(4,2,2,2,2,2,4),(-1.36853366463682,-1.09981790730256,
-0.874751340081577,-0.683009325808431,-0.491945339785637,-0.26523823904143,
-1.00032068147704E-6),.UNSPECIFIED.);
#703=B_SPLINE_CURVE_WITH_KNOTS('',3,(#45135,#45136,#45137,#45138,#45139,
#45140),.UNSPECIFIED.,.F.,.F.,(4,2,4),(3.71680310896038E-5,0.188969719403689,
0.318357862923346),.UNSPECIFIED.);
#704=B_SPLINE_CURVE_WITH_KNOTS('',3,(#45141,#45142,#45143,#45144,#45145,
#45146,#45147,#45148),.UNSPECIFIED.,.F.,.F.,(4,2,2,4),(0.,0.00387868763366687,
0.0800762215668998,0.137711267059276),.UNSPECIFIED.);
#705=B_SPLINE_CURVE_WITH_KNOTS('',3,(#45205,#45206,#45207,#45208,#45209,
#45210,#45211,#45212,#45213,#45214,#45215,#45216,#45217,#45218),
 .UNSPECIFIED.,.F.,.F.,(4,2,2,2,2,2,4),(0.0377143719414213,0.167070624995476,
0.336553194126115,0.499999999999991,0.663446805873868,0.832929375004528,
0.962285628058582),.UNSPECIFIED.);
#706=B_SPLINE_CURVE_WITH_KNOTS('',3,(#45584,#45585,#45586,#45587,#45588,
#45589,#45590,#45591),.UNSPECIFIED.,.F.,.F.,(4,2,2,4),(3.86068946090691E-5,
0.0477481584382911,0.113775363683532,0.296176984369277),.UNSPECIFIED.);
#707=B_SPLINE_CURVE_WITH_KNOTS('',3,(#45593,#45594,#45595,#45596,#45597,
#45598,#45599,#45600,#45601,#45602),.UNSPECIFIED.,.F.,.F.,(4,2,2,2,4),(1.00675013885361E-6,
0.198280154256163,0.401801682357639,0.519968319797222,0.606410947309042),
 .UNSPECIFIED.);
#708=B_SPLINE_CURVE_WITH_KNOTS('',3,(#45604,#45605,#45606,#45607,#45608,
#45609,#45610,#45611,#45612,#45613,#45614,#45615,#45616,#45617),
 .UNSPECIFIED.,.F.,.F.,(4,2,2,2,2,2,4),(-1.36923063553463,-1.09976128371409,
-0.874703857588768,-0.68297060694838,-0.49191596635355,-0.265236424101605,
-1.00032497786205E-6),.UNSPECIFIED.);
#709=B_SPLINE_CURVE_WITH_KNOTS('',3,(#45619,#45620,#45621,#45622,#45623,
#45624),.UNSPECIFIED.,.F.,.F.,(4,2,4),(5.24545898662702E-5,0.182499654277947,
0.288993661227474),.UNSPECIFIED.);
#710=B_SPLINE_CURVE_WITH_KNOTS('',3,(#45625,#45626,#45627,#45628,#45629,
#45630,#45631,#45632),.UNSPECIFIED.,.F.,.F.,(4,2,2,4),(1.58568685059277E-13,
0.035377553448089,0.0719723147421016,0.13036658253743),.UNSPECIFIED.);
#711=B_SPLINE_CURVE_WITH_KNOTS('',3,(#46006,#46007,#46008,#46009,#46010,
#46011,#46012,#46013,#46014,#46015,#46016,#46017,#46018,#46019),
 .UNSPECIFIED.,.F.,.F.,(4,2,2,2,2,2,4),(0.0377143719414213,0.167070624995476,
0.336553194126115,0.499999999999991,0.663446805873868,0.832929375004528,
0.962285628058582),.UNSPECIFIED.);
#712=B_SPLINE_CURVE_WITH_KNOTS('',3,(#46021,#46022,#46023,#46024,#46025,
#46026,#46027,#46028),.UNSPECIFIED.,.F.,.F.,(4,2,2,4),(3.69697143127623E-5,
0.053751719227584,0.103579138587863,0.175747470358817),.UNSPECIFIED.);
#713=B_SPLINE_CURVE_WITH_KNOTS('',3,(#46030,#46031,#46032,#46033,#46034,
#46035),.UNSPECIFIED.,.F.,.F.,(4,2,4),(1.0067260897438E-6,0.198302453808835,
0.617617266278844),.UNSPECIFIED.);
#714=B_SPLINE_CURVE_WITH_KNOTS('',3,(#46037,#46038,#46039,#46040,#46041,
#46042,#46043,#46044,#46045,#46046,#46047,#46048,#46049,#46050),
 .UNSPECIFIED.,.F.,.F.,(4,2,2,2,2,2,4),(-1.36856131602685,-1.09983747446031,
-0.874764567364842,-0.683019106044176,-0.491951477912598,-0.265243600779506,
-1.00032381763926E-6),.UNSPECIFIED.);
#715=B_SPLINE_CURVE_WITH_KNOTS('',3,(#46052,#46053,#46054,#46055,#46056,
#46057),.UNSPECIFIED.,.F.,.F.,(4,2,4),(1.01102908296581E-5,0.229050332432197,
0.401317557299931),.UNSPECIFIED.);
#716=B_SPLINE_CURVE_WITH_KNOTS('',3,(#46058,#46059,#46060,#46061,#46062,
#46063),.UNSPECIFIED.,.F.,.F.,(4,2,4),(4.00958579207454E-13,0.0448362547412082,
0.0753294109411124),.UNSPECIFIED.);
#717=B_SPLINE_CURVE_WITH_KNOTS('',3,(#46120,#46121,#46122,#46123,#46124,
#46125,#46126,#46127,#46128,#46129,#46130,#46131,#46132,#46133),
 .UNSPECIFIED.,.F.,.F.,(4,2,2,2,2,2,4),(0.0377143719414213,0.167070624995476,
0.336553194126115,0.499999999999991,0.663446805873868,0.832929375004528,
0.962285628058582),.UNSPECIFIED.);
#718=B_SPLINE_CURVE_WITH_KNOTS('',3,(#46513,#46514,#46515,#46516,#46517,
#46518),.UNSPECIFIED.,.F.,.F.,(4,2,4),(4.34887184794296E-5,0.103480982422226,
0.149574548200566),.UNSPECIFIED.);
#719=B_SPLINE_CURVE_WITH_KNOTS('',3,(#46520,#46521,#46522,#46523,#46524,
#46525,#46526,#46527,#46528,#46529),.UNSPECIFIED.,.F.,.F.,(4,2,2,2,4),(1.00143118243601E-6,
0.180608739286493,0.368729050760223,0.465285214132863,0.552599028244089),
 .UNSPECIFIED.);
#720=B_SPLINE_CURVE_WITH_KNOTS('',3,(#46531,#46532,#46533,#46534,#46535,
#46536,#46537,#46538,#46539,#46540,#46541,#46542,#46543,#46544),
 .UNSPECIFIED.,.F.,.F.,(4,2,2,2,2,2,4),(-1.35524591239,-1.08845925117483,
-0.865940013333757,-0.676355299140697,-0.487422236949836,-0.263156882106951,
-1.00018709657936E-6),.UNSPECIFIED.);
#721=B_SPLINE_CURVE_WITH_KNOTS('',3,(#46546,#46547,#46548,#46549,#46550,
#46551),.UNSPECIFIED.,.F.,.F.,(4,2,4),(2.96547197040926E-5,0.217520565424474,
0.410447896098608),.UNSPECIFIED.);
#722=B_SPLINE_CURVE_WITH_KNOTS('',3,(#46552,#46553,#46554,#46555,#46556,
#46557),.UNSPECIFIED.,.F.,.F.,(4,2,4),(4.22886337875709E-12,0.0851568103986181,
0.190922300311632),.UNSPECIFIED.);
#723=B_SPLINE_CURVE_WITH_KNOTS('',3,(#47001,#47002,#47003,#47004,#47005,
#47006,#47007,#47008,#47009,#47010,#47011,#47012,#47013,#47014),
 .UNSPECIFIED.,.F.,.F.,(4,2,2,2,2,2,4),(0.0377143719414213,0.167070624995476,
0.336553194126115,0.499999999999991,0.663446805873868,0.832929375004528,
0.962285628058582),.UNSPECIFIED.);
#724=B_SPLINE_CURVE_WITH_KNOTS('',3,(#47016,#47017,#47018,#47019,#47020,
#47021),.UNSPECIFIED.,.F.,.F.,(4,2,4),(2.21311227024518E-5,0.059746661158349,
0.130829664938975),.UNSPECIFIED.);
#725=B_SPLINE_CURVE_WITH_KNOTS('',3,(#47023,#47024,#47025,#47026,#47027,
#47028),.UNSPECIFIED.,.F.,.F.,(4,2,4),(1.00115827109886E-6,0.204260590716849,
0.65966839194673),.UNSPECIFIED.);
#726=B_SPLINE_CURVE_WITH_KNOTS('',3,(#47030,#47031,#47032,#47033,#47034,
#47035,#47036,#47037,#47038,#47039,#47040,#47041,#47042,#47043),
 .UNSPECIFIED.,.F.,.F.,(4,2,2,2,2,2,4),(-1.35292348708793,-1.08632729712736,
-0.864134156802677,-0.675300660556552,-0.487063391819361,-0.263053608006327,
-1.00023460417283E-6),.UNSPECIFIED.);
#727=B_SPLINE_CURVE_WITH_KNOTS('',3,(#47045,#47046,#47047,#47048,#47049,
#47050),.UNSPECIFIED.,.F.,.F.,(4,2,4),(0.000113907795243102,0.308169653858189,
0.697441169951114),.UNSPECIFIED.);
#728=B_SPLINE_CURVE_WITH_KNOTS('',3,(#47051,#47052,#47053,#47054,#47055,
#47056,#47057,#47058),.UNSPECIFIED.,.F.,.F.,(4,2,2,4),(8.12439686031872E-13,
0.0801092010493702,0.132357556624391,0.174836143722638),.UNSPECIFIED.);
#729=B_SPLINE_CURVE_WITH_KNOTS('',3,(#47115,#47116,#47117,#47118,#47119,
#47120,#47121,#47122,#47123,#47124,#47125,#47126,#47127,#47128),
 .UNSPECIFIED.,.F.,.F.,(4,2,2,2,2,2,4),(0.0377143719414213,0.167070624995476,
0.336553194126115,0.499999999999991,0.663446805873868,0.832929375004528,
0.962285628058582),.UNSPECIFIED.);
#730=B_SPLINE_CURVE_WITH_KNOTS('',3,(#47536,#47537,#47538,#47539,#47540,
#47541),.UNSPECIFIED.,.F.,.F.,(4,2,4),(6.85948530913353E-5,0.117689713160168,
0.701425347858688),.UNSPECIFIED.);
#731=B_SPLINE_CURVE_WITH_KNOTS('',3,(#47543,#47544,#47545,#47546,#47547,
#47548,#47549,#47550,#47551,#47552),.UNSPECIFIED.,.F.,.F.,(4,2,2,2,4),(1.00112175382184E-6,
0.175138486721777,0.354266046028186,0.450458287458295,0.512798132480794),
 .UNSPECIFIED.);
#732=B_SPLINE_CURVE_WITH_KNOTS('',3,(#47554,#47555,#47556,#47557,#47558,
#47559,#47560,#47561,#47562,#47563,#47564,#47565,#47566,#47567),
 .UNSPECIFIED.,.F.,.F.,(4,2,2,2,2,2,4),(-1.35460666568921,-1.08802411036352,
-0.865653674945032,-0.67605696728004,-0.487118571463883,-0.263006191372635,
-1.00022748703302E-6),.UNSPECIFIED.);
#733=B_SPLINE_CURVE_WITH_KNOTS('',3,(#47569,#47570,#47571,#47572,#47573,
#47574),.UNSPECIFIED.,.F.,.F.,(4,2,4),(2.20616210062517E-5,0.193313035420533,
0.359805614049465),.UNSPECIFIED.);
#734=B_SPLINE_CURVE_WITH_KNOTS('',3,(#47575,#47576,#47577,#47578,#47579,
#47580,#47581,#47582),.UNSPECIFIED.,.F.,.F.,(4,2,2,4),(0.,0.00481423729226705,
0.0811672210679098,0.136469477695337),.UNSPECIFIED.);
#735=B_SPLINE_CURVE_WITH_KNOTS('',3,(#47886,#47887,#47888,#47889,#47890,
#47891,#47892,#47893,#47894,#47895,#47896,#47897,#47898,#47899),
 .UNSPECIFIED.,.F.,.F.,(4,2,2,2,2,2,4),(0.0377143719414213,0.167070624995476,
0.336553194126115,0.499999999999991,0.663446805873868,0.832929375004528,
0.962285628058582),.UNSPECIFIED.);
#736=B_SPLINE_CURVE_WITH_KNOTS('',3,(#47901,#47902,#47903,#47904,#47905,
#47906),.UNSPECIFIED.,.F.,.F.,(4,2,4),(4.33372062421294E-5,0.0872462844676235,
0.169929347173722),.UNSPECIFIED.);
#737=B_SPLINE_CURVE_WITH_KNOTS('',3,(#47908,#47909,#47910,#47911,#47912,
#47913),.UNSPECIFIED.,.F.,.F.,(4,2,4),(1.00509826735353E-6,0.230891419553613,
0.673928064810453),.UNSPECIFIED.);
#738=B_SPLINE_CURVE_WITH_KNOTS('',3,(#47915,#47916,#47917,#47918,#47919,
#47920,#47921,#47922,#47923,#47924,#47925,#47926,#47927,#47928),
 .UNSPECIFIED.,.F.,.F.,(4,2,2,2,2,2,4),(-1.36612196099995,-1.09794402529119,
-0.873297935175745,-0.681853284681958,-0.491110055755908,-0.264840632478997,
-1.00030635918908E-6),.UNSPECIFIED.);
#739=B_SPLINE_CURVE_WITH_KNOTS('',3,(#47930,#47931,#47932,#47933,#47934,
#47935),.UNSPECIFIED.,.F.,.F.,(4,2,4),(5.23876301957788E-5,0.312841131349345,
0.562209482106279),.UNSPECIFIED.);
#740=B_SPLINE_CURVE_WITH_KNOTS('',3,(#47936,#47937,#47938,#47939,#47940,
#47941),.UNSPECIFIED.,.F.,.F.,(4,2,4),(5.79986291934581E-13,0.0801909208299588,
0.203417498476444),.UNSPECIFIED.);
#741=B_SPLINE_CURVE_WITH_KNOTS('',3,(#47998,#47999,#48000,#48001,#48002,
#48003,#48004,#48005,#48006,#48007,#48008,#48009,#48010,#48011),
 .UNSPECIFIED.,.F.,.F.,(4,2,2,2,2,2,4),(0.0377143719414213,0.167070624995476,
0.336553194126115,0.499999999999991,0.663446805873868,0.832929375004528,
0.962285628058582),.UNSPECIFIED.);
#742=B_SPLINE_CURVE_WITH_KNOTS('',3,(#48475,#48476,#48477,#48478,#48479,
#48480,#48481,#48482),.UNSPECIFIED.,.F.,.F.,(4,2,2,4),(1.93377698411972E-5,
0.0820712727478993,0.122296786666274,0.170369462240826),.UNSPECIFIED.);
#743=B_SPLINE_CURVE_WITH_KNOTS('',3,(#48484,#48485,#48486,#48487,#48488,
#48489,#48490,#48491,#48492,#48493),.UNSPECIFIED.,.F.,.F.,(4,2,2,2,4),(1.00118992452698E-6,
0.179077885748985,0.36144549077746,0.457726266756894,0.517260714194413),
 .UNSPECIFIED.);
#744=B_SPLINE_CURVE_WITH_KNOTS('',3,(#48495,#48496,#48497,#48498,#48499,
#48500,#48501,#48502,#48503,#48504,#48505,#48506,#48507,#48508),
 .UNSPECIFIED.,.F.,.F.,(4,2,2,2,2,2,4),(-1.35490487101256,-1.0882371122648,
-0.865819079989883,-0.676189142194246,-0.487214042398886,-0.263045157964749,
-1.00024126735575E-6),.UNSPECIFIED.);
#745=B_SPLINE_CURVE_WITH_KNOTS('',3,(#48510,#48511,#48512,#48513,#48514,
#48515),.UNSPECIFIED.,.F.,.F.,(4,2,4),(8.91007845760208E-5,0.191315852305385,
0.359031481093143),.UNSPECIFIED.);
#746=B_SPLINE_CURVE_WITH_KNOTS('',3,(#48516,#48517,#48518,#48519,#48520,
#48521,#48522,#48523),.UNSPECIFIED.,.F.,.F.,(4,2,2,4),(0.,0.05072995219315,
0.0893288312911254,0.132513385708746),.UNSPECIFIED.);
#747=B_SPLINE_CURVE_WITH_KNOTS('',3,(#48953,#48954,#48955,#48956,#48957,
#48958,#48959,#48960,#48961,#48962,#48963,#48964,#48965,#48966),
 .UNSPECIFIED.,.F.,.F.,(4,2,2,2,2,2,4),(0.0377143719414213,0.167070624995476,
0.336553194126115,0.499999999999991,0.663446805873868,0.832929375004528,
0.962285628058582),.UNSPECIFIED.);
#748=B_SPLINE_CURVE_WITH_KNOTS('',3,(#48968,#48969,#48970,#48971,#48972,
#48973,#48974,#48975,#48976,#48977),.UNSPECIFIED.,.F.,.F.,(4,2,2,2,4),(5.46118981870342E-5,
0.082170984774354,0.124431208907008,0.160831785884752,0.165639953609767),
 .UNSPECIFIED.);
#749=B_SPLINE_CURVE_WITH_KNOTS('',3,(#48979,#48980,#48981,#48982,#48983,
#48984),.UNSPECIFIED.,.F.,.F.,(4,2,4),(1.00682141930218E-6,0.198151473936767,
0.615501668196838),.UNSPECIFIED.);
#750=B_SPLINE_CURVE_WITH_KNOTS('',3,(#48986,#48987,#48988,#48989,#48990,
#48991,#48992,#48993,#48994,#48995,#48996,#48997,#48998,#48999),
 .UNSPECIFIED.,.F.,.F.,(4,2,2,2,2,2,4),(-1.36965940615866,-1.10016160366861,
-0.875066962492997,-0.683316335775481,-0.4922480420488,-0.265550631343516,
-1.00032842355209E-6),.UNSPECIFIED.);
#751=B_SPLINE_CURVE_WITH_KNOTS('',3,(#49001,#49002,#49003,#49004,#49005,
#49006),.UNSPECIFIED.,.F.,.F.,(4,2,4),(2.8517522314608E-5,0.207870471119106,
0.357440650988324),.UNSPECIFIED.);
#752=B_SPLINE_CURVE_WITH_KNOTS('',3,(#49007,#49008,#49009,#49010,#49011,
#49012),.UNSPECIFIED.,.F.,.F.,(4,2,4),(3.11253900974665E-12,0.0802245432637982,
0.139502091510436),.UNSPECIFIED.);
#753=B_SPLINE_CURVE_WITH_KNOTS('',3,(#49069,#49070,#49071,#49072,#49073,
#49074,#49075,#49076,#49077,#49078,#49079,#49080,#49081,#49082),
 .UNSPECIFIED.,.F.,.F.,(4,2,2,2,2,2,4),(0.0377143719414213,0.167070624995476,
0.336553194126115,0.499999999999991,0.663446805873868,0.832929375004528,
0.962285628058582),.UNSPECIFIED.);
#754=B_SPLINE_CURVE_WITH_KNOTS('',3,(#49532,#49533,#49534,#49535,#49536,
#49537,#49538,#49539),.UNSPECIFIED.,.F.,.F.,(4,2,2,4),(5.42863886920242E-5,
0.115927289482269,0.403180122557581,0.690436409009198),.UNSPECIFIED.);
#755=B_SPLINE_CURVE_WITH_KNOTS('',3,(#49541,#49542,#49543,#49544,#49545,
#49546),.UNSPECIFIED.,.F.,.F.,(4,2,4),(1.0067111711105E-6,0.19906795124752,
0.614262232114511),.UNSPECIFIED.);
#756=B_SPLINE_CURVE_WITH_KNOTS('',3,(#49548,#49549,#49550,#49551,#49552,
#49553,#49554,#49555,#49556,#49557,#49558,#49559,#49560,#49561),
 .UNSPECIFIED.,.F.,.F.,(4,2,2,2,2,2,4),(-1.36941174610337,-1.09990067907437,
-0.87481431262687,-0.683060659900653,-0.491984873694128,-0.265259069617268,
-1.00032309670381E-6),.UNSPECIFIED.);
#757=B_SPLINE_CURVE_WITH_KNOTS('',3,(#49563,#49564,#49565,#49566,#49567,
#49568),.UNSPECIFIED.,.F.,.F.,(4,2,4),(6.11026370320298E-5,0.197154855683272,
0.335212309964277),.UNSPECIFIED.);
#758=B_SPLINE_CURVE_WITH_KNOTS('',3,(#49569,#49570,#49571,#49572,#49573,
#49574,#49575,#49576),.UNSPECIFIED.,.F.,.F.,(4,2,2,4),(0.,0.00480921378375552,
0.0810921310518215,0.12941952313067),.UNSPECIFIED.);
#759=B_SPLINE_CURVE_WITH_KNOTS('',3,(#50006,#50007,#50008,#50009,#50010,
#50011,#50012,#50013,#50014,#50015,#50016,#50017,#50018,#50019),
 .UNSPECIFIED.,.F.,.F.,(4,2,2,2,2,2,4),(0.0377143719414213,0.167070624995476,
0.336553194126115,0.499999999999991,0.663446805873868,0.832929375004528,
0.962285628058582),.UNSPECIFIED.);
#760=B_SPLINE_CURVE_WITH_KNOTS('',3,(#50021,#50022,#50023,#50024,#50025,
#50026,#50027,#50028,#50029,#50030),.UNSPECIFIED.,.F.,.F.,(4,2,2,2,4),(4.40252338115954E-5,
0.0593320969994734,0.077891435154,0.0947902856199741,0.0969876170690407),
 .UNSPECIFIED.);
#761=B_SPLINE_CURVE_WITH_KNOTS('',3,(#50032,#50033,#50034,#50035,#50036,
#50037),.UNSPECIFIED.,.F.,.F.,(4,2,4),(1.00575192677772E-6,0.196465123063792,
0.617668689286788),.UNSPECIFIED.);
#762=B_SPLINE_CURVE_WITH_KNOTS('',3,(#50039,#50040,#50041,#50042,#50043,
#50044,#50045,#50046,#50047,#50048,#50049,#50050,#50051,#50052),
 .UNSPECIFIED.,.F.,.F.,(4,2,2,2,2,2,4),(-1.36650845342114,-1.09810261018534,
-0.873436258570306,-0.682032732525366,-0.491294664691022,-0.264928244974586,
-1.00034351039345E-6),.UNSPECIFIED.);
#763=B_SPLINE_CURVE_WITH_KNOTS('',3,(#50054,#50055,#50056,#50057,#50058,
#50059),.UNSPECIFIED.,.F.,.F.,(4,2,4),(1.56372366413953E-5,0.223813981237213,
0.38728646607154),.UNSPECIFIED.);
#764=B_SPLINE_CURVE_WITH_KNOTS('',3,(#50060,#50061,#50062,#50063,#50064,
#50065,#50066,#50067),.UNSPECIFIED.,.F.,.F.,(4,2,2,4),(0.,0.0799523739475497,
0.120850709803476,0.158334330677306),.UNSPECIFIED.);
#765=B_SPLINE_CURVE_WITH_KNOTS('',3,(#50124,#50125,#50126,#50127,#50128,
#50129,#50130,#50131,#50132,#50133,#50134,#50135,#50136,#50137),
 .UNSPECIFIED.,.F.,.F.,(4,2,2,2,2,2,4),(0.0377143719414213,0.167070624995476,
0.336553194126115,0.499999999999991,0.663446805873868,0.832929375004528,
0.962285628058582),.UNSPECIFIED.);
#766=B_SPLINE_CURVE_WITH_KNOTS('',3,(#50503,#50504,#50505,#50506,#50507,
#50508),.UNSPECIFIED.,.F.,.F.,(4,2,4),(2.90735538954063E-5,0.0821068334164978,
0.185641730304597),.UNSPECIFIED.);
#767=B_SPLINE_CURVE_WITH_KNOTS('',3,(#50510,#50511,#50512,#50513,#50514,
#50515),.UNSPECIFIED.,.F.,.F.,(4,2,4),(1.00576589928379E-6,0.196720798610431,
0.607958009277496),.UNSPECIFIED.);
#768=B_SPLINE_CURVE_WITH_KNOTS('',3,(#50517,#50518,#50519,#50520,#50521,
#50522,#50523,#50524,#50525,#50526,#50527,#50528,#50529,#50530),
 .UNSPECIFIED.,.F.,.F.,(4,2,2,2,2,2,4),(-1.36645387087117,-1.09803009009587,
-0.873368980499991,-0.682000111522624,-0.491298508345502,-0.26494563806227,
-1.00034434035875E-6),.UNSPECIFIED.);
#769=B_SPLINE_CURVE_WITH_KNOTS('',3,(#50532,#50533,#50534,#50535,#50536,
#50537),.UNSPECIFIED.,.F.,.F.,(4,2,4),(5.04888740588569E-5,0.222104264584732,
0.384046823394325),.UNSPECIFIED.);
#770=B_SPLINE_CURVE_WITH_KNOTS('',3,(#50538,#50539,#50540,#50541,#50542,
#50543),.UNSPECIFIED.,.F.,.F.,(4,2,4),(0.,0.0812570486202188,0.181154925817027),
 .UNSPECIFIED.);
#771=B_SPLINE_CURVE_WITH_KNOTS('',3,(#50945,#50946,#50947,#50948,#50949,
#50950,#50951,#50952,#50953,#50954,#50955,#50956,#50957,#50958),
 .UNSPECIFIED.,.F.,.F.,(4,2,2,2,2,2,4),(0.0377143719414213,0.167070624995476,
0.336553194126115,0.499999999999991,0.663446805873868,0.832929375004528,
0.962285628058582),.UNSPECIFIED.);
#772=B_SPLINE_CURVE_WITH_KNOTS('',3,(#50960,#50961,#50962,#50963,#50964,
#50965,#50966,#50967),.UNSPECIFIED.,.F.,.F.,(4,2,2,4),(3.17122319223456E-5,
0.0452758658318462,0.104387964404602,0.163687991775634),.UNSPECIFIED.);
#773=B_SPLINE_CURVE_WITH_KNOTS('',3,(#50969,#50970,#50971,#50972,#50973,
#50974),.UNSPECIFIED.,.F.,.F.,(4,2,4),(1.00585128027205E-6,0.196560733785392,
0.622029044934339),.UNSPECIFIED.);
#774=B_SPLINE_CURVE_WITH_KNOTS('',3,(#50976,#50977,#50978,#50979,#50980,
#50981,#50982,#50983,#50984,#50985,#50986,#50987,#50988,#50989),
 .UNSPECIFIED.,.F.,.F.,(4,2,2,2,2,2,4),(-1.36674172606792,-1.09823421639304,
-0.873527156968718,-0.682129646363664,-0.49139025098167,-0.264967864874043,
-1.00034944706873E-6),.UNSPECIFIED.);
#775=B_SPLINE_CURVE_WITH_KNOTS('',3,(#50991,#50992,#50993,#50994,#50995,
#50996),.UNSPECIFIED.,.F.,.F.,(4,2,4),(6.32656345427143E-5,0.163040125320008,
0.265078073811059),.UNSPECIFIED.);
#776=B_SPLINE_CURVE_WITH_KNOTS('',3,(#50997,#50998,#50999,#51000,#51001,
#51002),.UNSPECIFIED.,.F.,.F.,(4,2,4),(2.68743761055743E-12,0.0899508604032875,
0.179627225923839),.UNSPECIFIED.);
#777=B_SPLINE_CURVE_WITH_KNOTS('',3,(#51059,#51060,#51061,#51062,#51063,
#51064,#51065,#51066,#51067,#51068,#51069,#51070,#51071,#51072),
 .UNSPECIFIED.,.F.,.F.,(4,2,2,2,2,2,4),(0.0377143719414213,0.167070624995476,
0.336553194126115,0.499999999999991,0.663446805873868,0.832929375004528,
0.962285628058582),.UNSPECIFIED.);
#778=B_SPLINE_CURVE_WITH_KNOTS('',3,(#51452,#51453,#51454,#51455,#51456,
#51457),.UNSPECIFIED.,.F.,.F.,(4,2,4),(2.02724939215941E-5,0.0820778995171911,
0.183608432352108),.UNSPECIFIED.);
#779=B_SPLINE_CURVE_WITH_KNOTS('',3,(#51459,#51460,#51461,#51462,#51463,
#51464),.UNSPECIFIED.,.F.,.F.,(4,2,4),(1.00573485054331E-6,0.196992912849433,
0.611376509494975),.UNSPECIFIED.);
#780=B_SPLINE_CURVE_WITH_KNOTS('',3,(#51466,#51467,#51468,#51469,#51470,
#51471,#51472,#51473,#51474,#51475,#51476,#51477,#51478,#51479),
 .UNSPECIFIED.,.F.,.F.,(4,2,2,2,2,2,4),(-1.36651508911559,-1.09808854337808,
-0.873419265282326,-0.682038625392179,-0.491323399854143,-0.264952793979431,
-1.00034248505535E-6),.UNSPECIFIED.);
#781=B_SPLINE_CURVE_WITH_KNOTS('',3,(#51481,#51482,#51483,#51484,#51485,
#51486),.UNSPECIFIED.,.F.,.F.,(4,2,4),(1.03339269301046E-5,0.176278240887036,
0.282118520392689),.UNSPECIFIED.);
#782=B_SPLINE_CURVE_WITH_KNOTS('',3,(#51487,#51488,#51489,#51490,#51491,
#51492),.UNSPECIFIED.,.F.,.F.,(4,2,4),(1.94846466985946E-13,0.0811435839467738,
0.185199096592569),.UNSPECIFIED.);
#783=B_SPLINE_CURVE_WITH_KNOTS('',3,(#51964,#51965,#51966,#51967,#51968,
#51969,#51970,#51971,#51972,#51973,#51974,#51975,#51976,#51977),
 .UNSPECIFIED.,.F.,.F.,(4,2,2,2,2,2,4),(0.0377143719414213,0.167070624995476,
0.336553194126115,0.499999999999991,0.663446805873868,0.832929375004528,
0.962285628058582),.UNSPECIFIED.);
#784=B_SPLINE_CURVE_WITH_KNOTS('',3,(#51979,#51980,#51981,#51982,#51983,
#51984,#51985,#51986),.UNSPECIFIED.,.F.,.F.,(4,2,2,4),(7.66048904690143E-5,
0.0724751619057042,0.135157008985432,0.209683518789831),.UNSPECIFIED.);
#785=B_SPLINE_CURVE_WITH_KNOTS('',3,(#51988,#51989,#51990,#51991,#51992,
#51993),.UNSPECIFIED.,.F.,.F.,(4,2,4),(1.00671823419874E-6,0.198656747545274,
0.617231925244798),.UNSPECIFIED.);
#786=B_SPLINE_CURVE_WITH_KNOTS('',3,(#51995,#51996,#51997,#51998,#51999,
#52000,#52001,#52002,#52003,#52004,#52005,#52006,#52007,#52008),
 .UNSPECIFIED.,.F.,.F.,(4,2,2,2,2,2,4),(-1.36939616200995,-1.09987950875221,
-0.874793162387835,-0.683050721286367,-0.491987088351277,-0.265266499330064,
-1.00032344033588E-6),.UNSPECIFIED.);
#787=B_SPLINE_CURVE_WITH_KNOTS('',3,(#52010,#52011,#52012,#52013,#52014,
#52015),.UNSPECIFIED.,.F.,.F.,(4,2,4),(3.08789861800714E-5,0.198559217559626,
0.337824153970451),.UNSPECIFIED.);
#788=B_SPLINE_CURVE_WITH_KNOTS('',3,(#52016,#52017,#52018,#52019,#52020,
#52021,#52022,#52023),.UNSPECIFIED.,.F.,.F.,(4,2,2,4),(4.33668191395318E-13,
0.0554692068429926,0.26010462373677,0.513538194310567),.UNSPECIFIED.);
#789=B_SPLINE_CURVE_WITH_KNOTS('',3,(#52080,#52081,#52082,#52083,#52084,
#52085,#52086,#52087,#52088,#52089,#52090,#52091,#52092,#52093),
 .UNSPECIFIED.,.F.,.F.,(4,2,2,2,2,2,4),(0.0377143719414213,0.167070624995476,
0.336553194126115,0.499999999999991,0.663446805873868,0.832929375004528,
0.962285628058582),.UNSPECIFIED.);
#790=B_SPLINE_CURVE_WITH_KNOTS('',3,(#52669,#52670,#52671,#52672,#52673,
#52674,#52675,#52676),.UNSPECIFIED.,.F.,.F.,(4,2,2,4),(4.0720543721802E-5,
0.082048395609366,0.10384153561188,0.165696528972352),.UNSPECIFIED.);
#791=B_SPLINE_CURVE_WITH_KNOTS('',3,(#52678,#52679,#52680,#52681,#52682,
#52683),.UNSPECIFIED.,.F.,.F.,(4,2,4),(1.00674327113181E-6,0.198975068155899,
0.613393100807198),.UNSPECIFIED.);
#792=B_SPLINE_CURVE_WITH_KNOTS('',3,(#52685,#52686,#52687,#52688,#52689,
#52690,#52691,#52692,#52693,#52694,#52695,#52696,#52697,#52698),
 .UNSPECIFIED.,.F.,.F.,(4,2,2,2,2,2,4),(-1.36945586316978,-1.09992910347376,
-0.874829785599427,-0.683077785823512,-0.492005087217108,-0.265273394907698,
-1.00032464471707E-6),.UNSPECIFIED.);
#793=B_SPLINE_CURVE_WITH_KNOTS('',3,(#52700,#52701,#52702,#52703,#52704,
#52705),.UNSPECIFIED.,.F.,.F.,(4,2,4),(3.77093093284653E-5,0.199023405936395,
0.338855740163895),.UNSPECIFIED.);
#794=B_SPLINE_CURVE_WITH_KNOTS('',3,(#52706,#52707,#52708,#52709,#52710,
#52711),.UNSPECIFIED.,.F.,.F.,(4,2,4),(0.,0.0811055819570389,0.134676521572393),
 .UNSPECIFIED.);
#795=B_SPLINE_CURVE_WITH_KNOTS('',3,(#53127,#53128,#53129,#53130,#53131,
#53132,#53133,#53134,#53135,#53136,#53137,#53138,#53139,#53140),
 .UNSPECIFIED.,.F.,.F.,(4,2,2,2,2,2,4),(0.0377143719414213,0.167070624995476,
0.336553194126115,0.499999999999991,0.663446805873868,0.832929375004528,
0.962285628058582),.UNSPECIFIED.);
#796=B_SPLINE_CURVE_WITH_KNOTS('',3,(#53142,#53143,#53144,#53145,#53146,
#53147),.UNSPECIFIED.,.F.,.F.,(4,2,4),(3.17663181462393E-5,0.0586300965114554,
0.12163893952438),.UNSPECIFIED.);
#797=B_SPLINE_CURVE_WITH_KNOTS('',3,(#53149,#53150,#53151,#53152,#53153,
#53154),.UNSPECIFIED.,.F.,.F.,(4,2,4),(1.00574544958261E-6,0.196442953126253,
0.616075190837725),.UNSPECIFIED.);
#798=B_SPLINE_CURVE_WITH_KNOTS('',3,(#53156,#53157,#53158,#53159,#53160,
#53161,#53162,#53163,#53164,#53165,#53166,#53167,#53168,#53169),
 .UNSPECIFIED.,.F.,.F.,(4,2,2,2,2,2,4),(-1.36646180861503,-1.09803139080332,
-0.873373464214575,-0.682006913510101,-0.491306155279075,-0.26494779063171,
-1.00034312451653E-6),.UNSPECIFIED.);
#799=B_SPLINE_CURVE_WITH_KNOTS('',3,(#53171,#53172,#53173,#53174,#53175,
#53176),.UNSPECIFIED.,.F.,.F.,(4,2,4),(8.51202734725518E-5,0.213282211024296,
0.347455197118523),.UNSPECIFIED.);
#800=B_SPLINE_CURVE_WITH_KNOTS('',3,(#53177,#53178,#53179,#53180,#53181,
#53182),.UNSPECIFIED.,.F.,.F.,(4,2,4),(8.22519357859456E-13,0.0801856487952568,
0.160124211305378),.UNSPECIFIED.);
#801=B_SPLINE_CURVE_WITH_KNOTS('',3,(#53239,#53240,#53241,#53242,#53243,
#53244,#53245,#53246,#53247,#53248,#53249,#53250,#53251,#53252),
 .UNSPECIFIED.,.F.,.F.,(4,2,2,2,2,2,4),(0.0377143719414213,0.167070624995476,
0.336553194126115,0.499999999999991,0.663446805873868,0.832929375004528,
0.962285628058582),.UNSPECIFIED.);
#802=B_SPLINE_CURVE_WITH_KNOTS('',3,(#53716,#53717,#53718,#53719,#53720,
#53721),.UNSPECIFIED.,.F.,.F.,(4,2,4),(2.85042569573143E-5,0.0779704082414512,
0.146157984837617),.UNSPECIFIED.);
#803=B_SPLINE_CURVE_WITH_KNOTS('',3,(#53723,#53724,#53725,#53726,#53727,
#53728),.UNSPECIFIED.,.F.,.F.,(4,2,4),(1.00575001969219E-6,0.196811902994003,
0.607209604097769),.UNSPECIFIED.);
#804=B_SPLINE_CURVE_WITH_KNOTS('',3,(#53730,#53731,#53732,#53733,#53734,
#53735,#53736,#53737,#53738,#53739,#53740,#53741,#53742,#53743),
 .UNSPECIFIED.,.F.,.F.,(4,2,2,2,2,2,4),(-1.36646927232899,-1.09805347703677,
-0.87339045221244,-0.682015194511553,-0.49130486745357,-0.264941327695831,
-1.00034339038765E-6),.UNSPECIFIED.);
#805=B_SPLINE_CURVE_WITH_KNOTS('',3,(#53745,#53746,#53747,#53748,#53749,
#53750),.UNSPECIFIED.,.F.,.F.,(4,2,4),(3.18944872613953E-5,0.201689934389403,
0.342722617046712),.UNSPECIFIED.);
#806=B_SPLINE_CURVE_WITH_KNOTS('',3,(#53751,#53752,#53753,#53754,#53755,
#53756),.UNSPECIFIED.,.F.,.F.,(4,2,4),(7.41583121241415E-13,0.0919471405631882,
0.218813839045918),.UNSPECIFIED.);
#807=B_SPLINE_CURVE_WITH_KNOTS('',3,(#54200,#54201,#54202,#54203,#54204,
#54205,#54206,#54207,#54208,#54209,#54210,#54211,#54212,#54213),
 .UNSPECIFIED.,.F.,.F.,(4,2,2,2,2,2,4),(0.0377143719414213,0.167070624995476,
0.336553194126115,0.499999999999991,0.663446805873868,0.832929375004528,
0.962285628058582),.UNSPECIFIED.);
#808=B_SPLINE_CURVE_WITH_KNOTS('',3,(#54215,#54216,#54217,#54218,#54219,
#54220),.UNSPECIFIED.,.F.,.F.,(4,2,4),(8.27853671649851E-6,0.117348681204103,
0.81803028591539),.UNSPECIFIED.);
#809=B_SPLINE_CURVE_WITH_KNOTS('',3,(#54222,#54223,#54224,#54225,#54226,
#54227),.UNSPECIFIED.,.F.,.F.,(4,2,4),(1.00584838939465E-6,0.196105737182075,
0.613752572300065),.UNSPECIFIED.);
#810=B_SPLINE_CURVE_WITH_KNOTS('',3,(#54229,#54230,#54231,#54232,#54233,
#54234,#54235,#54236,#54237,#54238,#54239,#54240,#54241,#54242),
 .UNSPECIFIED.,.F.,.F.,(4,2,2,2,2,2,4),(-1.36657598676591,-1.09814330805353,
-0.873456182939785,-0.682053794892946,-0.49131998381188,-0.264952672836963,
-1.00034927255395E-6),.UNSPECIFIED.);
#811=B_SPLINE_CURVE_WITH_KNOTS('',3,(#54244,#54245,#54246,#54247,#54248,
#54249),.UNSPECIFIED.,.F.,.F.,(4,2,4),(8.19755470884497E-5,0.23524102296215,
0.412699034637965),.UNSPECIFIED.);
#812=B_SPLINE_CURVE_WITH_KNOTS('',3,(#54250,#54251,#54252,#54253,#54254,
#54255),.UNSPECIFIED.,.F.,.F.,(4,2,4),(5.98025872820168E-13,0.0829465259271522,
0.178737241653031),.UNSPECIFIED.);
#813=B_SPLINE_CURVE_WITH_KNOTS('',3,(#54312,#54313,#54314,#54315,#54316,
#54317,#54318,#54319,#54320,#54321,#54322,#54323,#54324,#54325),
 .UNSPECIFIED.,.F.,.F.,(4,2,2,2,2,2,4),(0.0377143719414213,0.167070624995476,
0.336553194126115,0.499999999999991,0.663446805873868,0.832929375004528,
0.962285628058582),.UNSPECIFIED.);
#814=B_SPLINE_CURVE_WITH_KNOTS('',3,(#54761,#54762,#54763,#54764,#54765,
#54766,#54767,#54768,#54769,#54770),.UNSPECIFIED.,.F.,.F.,(4,2,2,2,4),(2.91083665470649E-5,
0.0448810650389932,0.10235865502192,0.143363070345125,0.176052267827766),
 .UNSPECIFIED.);
#815=B_SPLINE_CURVE_WITH_KNOTS('',3,(#54772,#54773,#54774,#54775,#54776,
#54777),.UNSPECIFIED.,.F.,.F.,(4,2,4),(1.00586691344213E-6,0.197039335069742,
0.614437201408451),.UNSPECIFIED.);
#816=B_SPLINE_CURVE_WITH_KNOTS('',3,(#54779,#54780,#54781,#54782,#54783,
#54784,#54785,#54786,#54787,#54788,#54789,#54790,#54791,#54792),
 .UNSPECIFIED.,.F.,.F.,(4,2,2,2,2,2,4),(-1.36676533760477,-1.09824478324466,
-0.873535367034155,-0.682138570180602,-0.491399555548606,-0.264972297603895,
-1.00035037616401E-6),.UNSPECIFIED.);
#817=B_SPLINE_CURVE_WITH_KNOTS('',3,(#54794,#54795,#54796,#54797,#54798,
#54799),.UNSPECIFIED.,.F.,.F.,(4,2,4),(0.00013096404143776,0.152963582320661,
0.248940965083308),.UNSPECIFIED.);
#818=B_SPLINE_CURVE_WITH_KNOTS('',3,(#54800,#54801,#54802,#54803,#54804,
#54805,#54806,#54807),.UNSPECIFIED.,.F.,.F.,(4,2,2,4),(3.81584992072495E-12,
0.0811754769524944,0.11370948911483,0.136181238711659),.UNSPECIFIED.);
#819=B_SPLINE_CURVE_WITH_KNOTS('',3,(#55279,#55280,#55281,#55282,#55283,
#55284,#55285,#55286,#55287,#55288,#55289,#55290,#55291,#55292),
 .UNSPECIFIED.,.F.,.F.,(4,2,2,2,2,2,4),(0.0377143719414213,0.167070624995476,
0.336553194126115,0.499999999999991,0.663446805873868,0.832929375004528,
0.962285628058582),.UNSPECIFIED.);
#820=B_SPLINE_CURVE_WITH_KNOTS('',3,(#55294,#55295,#55296,#55297,#55298,
#55299),.UNSPECIFIED.,.F.,.F.,(4,2,4),(1.31240404424589E-5,0.118148896618705,
0.705933282625893),.UNSPECIFIED.);
#821=B_SPLINE_CURVE_WITH_KNOTS('',3,(#55301,#55302,#55303,#55304,#55305,
#55306),.UNSPECIFIED.,.F.,.F.,(4,2,4),(1.00584283955035E-6,0.196654732302861,
0.618684486486058),.UNSPECIFIED.);
#822=B_SPLINE_CURVE_WITH_KNOTS('',3,(#55308,#55309,#55310,#55311,#55312,
#55313,#55314,#55315,#55316,#55317,#55318,#55319,#55320,#55321),
 .UNSPECIFIED.,.F.,.F.,(4,2,2,2,2,2,4),(-1.36678617495215,-1.09826185815999,
-0.873545812350535,-0.682155092083844,-0.491422802142017,-0.264985880565712,
-1.00034894152623E-6),.UNSPECIFIED.);
#823=B_SPLINE_CURVE_WITH_KNOTS('',3,(#55323,#55324,#55325,#55326,#55327,
#55328),.UNSPECIFIED.,.F.,.F.,(4,2,4),(1.56558672178928E-5,0.190788483130578,
0.32659926592214),.UNSPECIFIED.);
#824=B_SPLINE_CURVE_WITH_KNOTS('',3,(#55329,#55330,#55331,#55332,#55333,
#55334),.UNSPECIFIED.,.F.,.F.,(4,2,4),(1.03020526869841E-12,0.0800803859593916,
0.135679047359458),.UNSPECIFIED.);
#825=B_SPLINE_CURVE_WITH_KNOTS('',3,(#55391,#55392,#55393,#55394,#55395,
#55396,#55397,#55398,#55399,#55400,#55401,#55402,#55403,#55404),
 .UNSPECIFIED.,.F.,.F.,(4,2,2,2,2,2,4),(0.0377143719414213,0.167070624995476,
0.336553194126115,0.499999999999991,0.663446805873868,0.832929375004528,
0.962285628058582),.UNSPECIFIED.);
#826=B_SPLINE_CURVE_WITH_KNOTS('',3,(#55840,#55841,#55842,#55843,#55844,
#55845,#55846,#55847,#55848,#55849),.UNSPECIFIED.,.F.,.F.,(4,2,2,2,4),(2.95331200204396E-5,
0.0448823812946117,0.10236199038552,0.143361158366412,0.176043615886501),
 .UNSPECIFIED.);
#827=B_SPLINE_CURVE_WITH_KNOTS('',3,(#55851,#55852,#55853,#55854,#55855,
#55856),.UNSPECIFIED.,.F.,.F.,(4,2,4),(1.00586876398164E-6,0.197038889607744,
0.614451442266876),.UNSPECIFIED.);
#828=B_SPLINE_CURVE_WITH_KNOTS('',3,(#55858,#55859,#55860,#55861,#55862,
#55863,#55864,#55865,#55866,#55867,#55868,#55869,#55870,#55871),
 .UNSPECIFIED.,.F.,.F.,(4,2,2,2,2,2,4),(-1.36676752401463,-1.09824522385243,
-0.873535205630291,-0.682139122541776,-0.49140088307381,-0.264973665093558,
-1.00035048783346E-6),.UNSPECIFIED.);
#829=B_SPLINE_CURVE_WITH_KNOTS('',3,(#55873,#55874,#55875,#55876,#55877,
#55878),.UNSPECIFIED.,.F.,.F.,(4,2,4),(0.000132963294187387,0.153060747720903,
0.249120285259133),.UNSPECIFIED.);
#830=B_SPLINE_CURVE_WITH_KNOTS('',3,(#55879,#55880,#55881,#55882,#55883,
#55884,#55885,#55886),.UNSPECIFIED.,.F.,.F.,(4,2,2,4),(7.85771554400852E-12,
0.0811766790944722,0.113710097814863,0.136178725750842),.UNSPECIFIED.);
#831=B_SPLINE_CURVE_WITH_KNOTS('',3,(#56498,#56499,#56500,#56501,#56502,
#56503,#56504,#56505,#56506,#56507,#56508,#56509,#56510,#56511),
 .UNSPECIFIED.,.F.,.F.,(4,2,2,2,2,2,4),(0.0377143719414213,0.167070624995476,
0.336553194126115,0.499999999999991,0.663446805873868,0.832929375004528,
0.962285628058582),.UNSPECIFIED.);
#832=B_SPLINE_CURVE_WITH_KNOTS('',3,(#56513,#56514,#56515,#56516,#56517,
#56518,#56519,#56520,#56521,#56522),.UNSPECIFIED.,.F.,.F.,(4,2,2,2,4),(2.90874908040396E-5,
0.0695369396976002,0.127685025171556,0.192550047820966,0.193204673416467),
 .UNSPECIFIED.);
#833=B_SPLINE_CURVE_WITH_KNOTS('',3,(#56524,#56525,#56526,#56527,#56528,
#56529),.UNSPECIFIED.,.F.,.F.,(4,2,4),(1.00063186540735E-6,0.183871198323765,
0.593831676218595),.UNSPECIFIED.);
#834=B_SPLINE_CURVE_WITH_KNOTS('',3,(#56531,#56532,#56533,#56534,#56535,
#56536,#56537,#56538,#56539,#56540,#56541,#56542,#56543,#56544),
 .UNSPECIFIED.,.F.,.F.,(4,2,2,2,2,2,4),(-1.35138145767626,-1.08533623797411,
-0.863457932782986,-0.67461579591868,-0.48640715531557,-0.262769633851996,
-1.00013603251387E-6),.UNSPECIFIED.);
#835=B_SPLINE_CURVE_WITH_KNOTS('',3,(#56546,#56547,#56548,#56549,#56550,
#56551),.UNSPECIFIED.,.F.,.F.,(4,2,4),(7.67987202833742E-5,0.135045540153931,
0.23216672789008),.UNSPECIFIED.);
#836=B_SPLINE_CURVE_WITH_KNOTS('',3,(#56552,#56553,#56554,#56555,#56556,
#56557,#56558,#56559),.UNSPECIFIED.,.F.,.F.,(4,2,2,4),(5.70631864960257E-12,
0.0385065493161646,0.101661114347598,0.190748080830985),.UNSPECIFIED.);
#837=B_SPLINE_CURVE_WITH_KNOTS('',3,(#56616,#56617,#56618,#56619,#56620,
#56621,#56622,#56623,#56624,#56625,#56626,#56627,#56628,#56629),
 .UNSPECIFIED.,.F.,.F.,(4,2,2,2,2,2,4),(0.0377143719414213,0.167070624995476,
0.336553194126115,0.499999999999991,0.663446805873868,0.832929375004528,
0.962285628058582),.UNSPECIFIED.);
#838=B_SPLINE_CURVE_WITH_KNOTS('',3,(#57191,#57192,#57193,#57194,#57195,
#57196,#57197,#57198),.UNSPECIFIED.,.F.,.F.,(4,2,2,4),(3.73720623976683E-5,
0.0820934034488392,0.159780549935175,0.163589055589674),.UNSPECIFIED.);
#839=B_SPLINE_CURVE_WITH_KNOTS('',3,(#57200,#57201,#57202,#57203,#57204,
#57205),.UNSPECIFIED.,.F.,.F.,(4,2,4),(1.00680487095348E-6,0.198775773316189,
0.612602414802361),.UNSPECIFIED.);
#840=B_SPLINE_CURVE_WITH_KNOTS('',3,(#57207,#57208,#57209,#57210,#57211,
#57212,#57213,#57214,#57215,#57216,#57217,#57218,#57219,#57220),
 .UNSPECIFIED.,.F.,.F.,(4,2,2,2,2,2,4),(-1.36947028433637,-1.09994697149041,
-0.874841168477541,-0.68308329902947,-0.492005354543596,-0.265278186460551,
-1.00032760913201E-6),.UNSPECIFIED.);
#841=B_SPLINE_CURVE_WITH_KNOTS('',3,(#57222,#57223,#57224,#57225,#57226,
#57227),.UNSPECIFIED.,.F.,.F.,(4,2,4),(9.95249900306014E-6,0.201659078077706,
0.343960579336747),.UNSPECIFIED.);
#842=B_SPLINE_CURVE_WITH_KNOTS('',3,(#57228,#57229,#57230,#57231,#57232,
#57233),.UNSPECIFIED.,.F.,.F.,(4,2,4),(0.,0.0810866766827009,0.130143252265822),
 .UNSPECIFIED.);
#843=B_SPLINE_CURVE_WITH_KNOTS('',3,(#57747,#57748,#57749,#57750,#57751,
#57752,#57753,#57754,#57755,#57756,#57757,#57758,#57759,#57760),
 .UNSPECIFIED.,.F.,.F.,(4,2,2,2,2,2,4),(0.0377143719414213,0.167070624995476,
0.336553194126115,0.499999999999991,0.663446805873868,0.832929375004528,
0.962285628058582),.UNSPECIFIED.);
#844=B_SPLINE_CURVE_WITH_KNOTS('',3,(#57762,#57763,#57764,#57765,#57766,
#57767,#57768,#57769,#57770,#57771),.UNSPECIFIED.,.F.,.F.,(4,2,2,2,4),(6.26026778345803E-5,
0.0821879366532444,0.124360696633958,0.160511740289931,0.165280462627525),
 .UNSPECIFIED.);
#845=B_SPLINE_CURVE_WITH_KNOTS('',3,(#57773,#57774,#57775,#57776,#57777,
#57778,#57779,#57780,#57781,#57782),.UNSPECIFIED.,.F.,.F.,(4,2,2,2,4),(1.00120887031484E-6,
0.178144277374141,0.361084123405984,0.458351091752043,0.518212486842599),
 .UNSPECIFIED.);
#846=B_SPLINE_CURVE_WITH_KNOTS('',3,(#57784,#57785,#57786,#57787,#57788,
#57789,#57790,#57791,#57792,#57793,#57794,#57795,#57796,#57797),
 .UNSPECIFIED.,.F.,.F.,(4,2,2,2,2,2,4),(-1.35452120523838,-1.08792026996376,
-0.865513415712065,-0.676039627480199,-0.487227006474019,-0.263105526553072,
-1.00024511471768E-6),.UNSPECIFIED.);
#847=B_SPLINE_CURVE_WITH_KNOTS('',3,(#57799,#57800,#57801,#57802,#57803,
#57804),.UNSPECIFIED.,.F.,.F.,(4,2,4),(5.13023327127914E-5,0.195133577906603,
0.330520359442512),.UNSPECIFIED.);
#848=B_SPLINE_CURVE_WITH_KNOTS('',3,(#57805,#57806,#57807,#57808,#57809,
#57810),.UNSPECIFIED.,.F.,.F.,(4,2,4),(2.7857164981918E-12,0.0801884474066829,
0.134390902567056),.UNSPECIFIED.);
#849=B_SPLINE_CURVE_WITH_KNOTS('',3,(#57867,#57868,#57869,#57870,#57871,
#57872,#57873,#57874,#57875,#57876,#57877,#57878,#57879,#57880),
 .UNSPECIFIED.,.F.,.F.,(4,2,2,2,2,2,4),(0.0377143719414213,0.167070624995476,
0.336553194126115,0.499999999999991,0.663446805873868,0.832929375004528,
0.962285628058582),.UNSPECIFIED.);
#850=B_SPLINE_CURVE_WITH_KNOTS('',3,(#58246,#58247,#58248,#58249,#58250,
#58251,#58252,#58253),.UNSPECIFIED.,.F.,.F.,(4,2,2,4),(4.73120833335754E-5,
0.0422670695525102,0.0810849470856931,0.127252781970067),.UNSPECIFIED.);
#851=B_SPLINE_CURVE_WITH_KNOTS('',3,(#58255,#58256,#58257,#58258,#58259,
#58260),.UNSPECIFIED.,.F.,.F.,(4,2,4),(1.00647499030429E-6,0.200113073863495,
0.595429491994324),.UNSPECIFIED.);
#852=B_SPLINE_CURVE_WITH_KNOTS('',3,(#58262,#58263,#58264,#58265,#58266,
#58267,#58268,#58269,#58270,#58271,#58272,#58273,#58274,#58275),
 .UNSPECIFIED.,.F.,.F.,(4,2,2,2,2,2,4),(-1.36849439771666,-1.09954066052859,
-0.874510163535254,-0.682956346820273,-0.492067229987142,-0.265320521461021,
-1.00031346793631E-6),.UNSPECIFIED.);
#853=B_SPLINE_CURVE_WITH_KNOTS('',3,(#58277,#58278,#58279,#58280,#58281,
#58282),.UNSPECIFIED.,.F.,.F.,(4,2,4),(7.71756783525451E-5,0.307508164573013,
0.565378873758567),.UNSPECIFIED.);
#854=B_SPLINE_CURVE_WITH_KNOTS('',3,(#58283,#58284,#58285,#58286,#58287,
#58288,#58289,#58290),.UNSPECIFIED.,.F.,.F.,(4,2,2,4),(3.89766384540504E-13,
0.0811658080415485,0.130795260681648,0.217612754456687),.UNSPECIFIED.);
#855=B_SPLINE_CURVE_WITH_KNOTS('',3,(#58804,#58805,#58806,#58807,#58808,
#58809,#58810,#58811,#58812,#58813,#58814,#58815,#58816,#58817),
 .UNSPECIFIED.,.F.,.F.,(4,2,2,2,2,2,4),(0.0377143719414213,0.167070624995476,
0.336553194126115,0.499999999999991,0.663446805873868,0.832929375004528,
0.962285628058582),.UNSPECIFIED.);
#856=B_SPLINE_CURVE_WITH_KNOTS('',3,(#58819,#58820,#58821,#58822,#58823,
#58824,#58825,#58826,#58827,#58828),.UNSPECIFIED.,.F.,.F.,(4,2,2,2,4),(6.1190446859549E-5,
0.0821849189214334,0.124358056634849,0.160517624190395,0.165288966829186),
 .UNSPECIFIED.);
#857=B_SPLINE_CURVE_WITH_KNOTS('',3,(#58830,#58831,#58832,#58833,#58834,
#58835,#58836,#58837,#58838,#58839),.UNSPECIFIED.,.F.,.F.,(4,2,2,2,4),(1.00121666513906E-6,
0.178436610588235,0.361713510187113,0.459165212991689,0.519162438061592),
 .UNSPECIFIED.);
#858=B_SPLINE_CURVE_WITH_KNOTS('',3,(#58841,#58842,#58843,#58844,#58845,
#58846,#58847,#58848,#58849,#58850,#58851,#58852,#58853,#58854),
 .UNSPECIFIED.,.F.,.F.,(4,2,2,2,2,2,4),(-1.35454818634146,-1.08794337470072,
-0.865532135918778,-0.676052154638076,-0.487233237434815,-0.26310695574337,
-1.00024670269493E-6),.UNSPECIFIED.);
#859=B_SPLINE_CURVE_WITH_KNOTS('',3,(#58856,#58857,#58858,#58859,#58860,
#58861),.UNSPECIFIED.,.F.,.F.,(4,2,4),(4.98634138348218E-5,0.195141037972379,
0.330493201196748),.UNSPECIFIED.);
#860=B_SPLINE_CURVE_WITH_KNOTS('',3,(#58862,#58863,#58864,#58865,#58866,
#58867),.UNSPECIFIED.,.F.,.F.,(4,2,4),(4.57542679217533E-12,0.0801871578090029,
0.134385019693337),.UNSPECIFIED.);
#861=B_SPLINE_CURVE_WITH_KNOTS('',3,(#58924,#58925,#58926,#58927,#58928,
#58929,#58930,#58931,#58932,#58933,#58934,#58935,#58936,#58937),
 .UNSPECIFIED.,.F.,.F.,(4,2,2,2,2,2,4),(0.0377143719414213,0.167070624995476,
0.336553194126115,0.499999999999991,0.663446805873868,0.832929375004528,
0.962285628058582),.UNSPECIFIED.);
#862=B_SPLINE_CURVE_WITH_KNOTS('',3,(#59597,#59598,#59599,#59600,#59601,
#59602,#59603,#59604),.UNSPECIFIED.,.F.,.F.,(4,2,2,4),(1.07065022399325E-5,
0.0820415500405752,0.124395055584087,0.162715337467435),.UNSPECIFIED.);
#863=B_SPLINE_CURVE_WITH_KNOTS('',3,(#59606,#59607,#59608,#59609,#59610,
#59611,#59612,#59613,#59614,#59615),.UNSPECIFIED.,.F.,.F.,(4,2,2,2,4),(1.00134536322123E-6,
0.18222044597792,0.367842106932836,0.465703496956847,0.525884883424001),
 .UNSPECIFIED.);
#864=B_SPLINE_CURVE_WITH_KNOTS('',3,(#59617,#59618,#59619,#59620,#59621,
#59622,#59623,#59624,#59625,#59626,#59627,#59628,#59629,#59630),
 .UNSPECIFIED.,.F.,.F.,(4,2,2,2,2,2,4),(-1.35506345253935,-1.08840531341759,
-0.865944635772675,-0.676279073046853,-0.487277090549597,-0.263087864621955,
-1.00017583849435E-6),.UNSPECIFIED.);
#865=B_SPLINE_CURVE_WITH_KNOTS('',3,(#59632,#59633,#59634,#59635,#59636,
#59637),.UNSPECIFIED.,.F.,.F.,(4,2,4),(5.3962766046209E-5,0.108969967890436,
0.182584633205874),.UNSPECIFIED.);
#866=B_SPLINE_CURVE_WITH_KNOTS('',3,(#59638,#59639,#59640,#59641,#59642,
#59643),.UNSPECIFIED.,.F.,.F.,(4,2,4),(5.22653476197789E-12,0.0811239424511172,
0.11375725969146),.UNSPECIFIED.);
#867=B_SPLINE_CURVE_WITH_KNOTS('',3,(#60213,#60214,#60215,#60216,#60217,
#60218,#60219,#60220,#60221,#60222,#60223,#60224,#60225,#60226),
 .UNSPECIFIED.,.F.,.F.,(4,2,2,2,2,2,4),(0.0377143719414213,0.167070624995476,
0.336553194126115,0.499999999999991,0.663446805873868,0.832929375004528,
0.962285628058582),.UNSPECIFIED.);
#868=B_SPLINE_CURVE_WITH_KNOTS('',3,(#60228,#60229,#60230,#60231,#60232,
#60233,#60234,#60235),.UNSPECIFIED.,.F.,.F.,(4,2,2,4),(3.79993615621598E-5,
0.0820948071540982,0.159782168454658,0.163590605624764),.UNSPECIFIED.);
#869=B_SPLINE_CURVE_WITH_KNOTS('',3,(#60237,#60238,#60239,#60240,#60241,
#60242),.UNSPECIFIED.,.F.,.F.,(4,2,4),(1.00680304406573E-6,0.198371116469636,
0.616016616729024),.UNSPECIFIED.);
#870=B_SPLINE_CURVE_WITH_KNOTS('',3,(#60244,#60245,#60246,#60247,#60248,
#60249,#60250,#60251,#60252,#60253,#60254,#60255,#60256,#60257),
 .UNSPECIFIED.,.F.,.F.,(4,2,2,2,2,2,4),(-1.36946791051543,-1.09994504179602,
-0.874839555222837,-0.68308307358568,-0.492006341135471,-0.26527826440027,
-1.0003275292482E-6),.UNSPECIFIED.);
#871=B_SPLINE_CURVE_WITH_KNOTS('',3,(#60259,#60260,#60261,#60262,#60263,
#60264),.UNSPECIFIED.,.F.,.F.,(4,2,4),(9.21025416984816E-6,0.201412302234187,
0.34337647011839),.UNSPECIFIED.);
#872=B_SPLINE_CURVE_WITH_KNOTS('',3,(#60265,#60266,#60267,#60268,#60269,
#60270),.UNSPECIFIED.,.F.,.F.,(4,2,4),(1.74012010253697E-12,0.0799694236906792,
0.14961823093418),.UNSPECIFIED.);
#873=B_SPLINE_CURVE_WITH_KNOTS('',3,(#60327,#60328,#60329,#60330,#60331,
#60332,#60333,#60334,#60335,#60336,#60337,#60338,#60339,#60340),
 .UNSPECIFIED.,.F.,.F.,(4,2,2,2,2,2,4),(0.0377143719414213,0.167070624995476,
0.336553194126115,0.499999999999991,0.663446805873868,0.832929375004528,
0.962285628058582),.UNSPECIFIED.);
#874=B_SPLINE_CURVE_WITH_KNOTS('',3,(#60706,#60707,#60708,#60709,#60710,
#60711,#60712,#60713),.UNSPECIFIED.,.F.,.F.,(4,2,2,4),(0.000198665912013773,
0.0423192231855041,0.0819962999928345,0.222796246729331),.UNSPECIFIED.);
#875=B_SPLINE_CURVE_WITH_KNOTS('',3,(#60715,#60716,#60717,#60718,#60719,
#60720),.UNSPECIFIED.,.F.,.F.,(4,2,4),(1.00678242509254E-6,0.199083168651477,
0.591904491004669),.UNSPECIFIED.);
#876=B_SPLINE_CURVE_WITH_KNOTS('',3,(#60722,#60723,#60724,#60725,#60726,
#60727,#60728,#60729,#60730,#60731,#60732,#60733,#60734,#60735),
 .UNSPECIFIED.,.F.,.F.,(4,2,2,2,2,2,4),(-1.36893350864692,-1.09997929470732,
-0.87490648981194,-0.683305966268589,-0.4923773938272,-0.265638162538616,
-1.00032653094444E-6),.UNSPECIFIED.);
#877=B_SPLINE_CURVE_WITH_KNOTS('',3,(#60737,#60738,#60739,#60740,#60741,
#60742),.UNSPECIFIED.,.F.,.F.,(4,2,4),(6.74092780132926E-5,0.30785071191309,
0.598735524338827),.UNSPECIFIED.);
#878=B_SPLINE_CURVE_WITH_KNOTS('',3,(#60743,#60744,#60745,#60746,#60747,
#60748,#60749,#60750),.UNSPECIFIED.,.F.,.F.,(4,2,2,4),(6.87557743431209E-14,
0.0811979885087478,0.125523813671698,0.201873086677692),.UNSPECIFIED.);
#879=B_SPLINE_CURVE_WITH_KNOTS('',3,(#60755,#60756,#60757,#60758,#60759,
#60760,#60761,#60762,#60763,#60764),.UNSPECIFIED.,.F.,.F.,(4,2,2,2,4),(0.,
0.0285072227353245,0.0532892290060001,0.0661103821512685,0.0936902631120297),
 .UNSPECIFIED.);
#880=B_SPLINE_CURVE_WITH_KNOTS('',3,(#61277,#61278,#61279,#61280,#61281,
#61282,#61283,#61284,#61285,#61286,#61287,#61288,#61289,#61290),
 .UNSPECIFIED.,.F.,.F.,(4,2,2,2,2,2,4),(0.0377143719414213,0.167070624995476,
0.336553194126115,0.499999999999991,0.663446805873868,0.832929375004528,
0.962285628058582),.UNSPECIFIED.);
#881=B_SPLINE_CURVE_WITH_KNOTS('',3,(#61292,#61293,#61294,#61295,#61296,
#61297,#61298,#61299),.UNSPECIFIED.,.F.,.F.,(4,2,2,4),(8.2068747900806E-5,
0.0736236603178404,0.133996054723513,0.219980728701435),.UNSPECIFIED.);
#882=B_SPLINE_CURVE_WITH_KNOTS('',3,(#61301,#61302,#61303,#61304,#61305,
#61306),.UNSPECIFIED.,.F.,.F.,(4,2,4),(1.00672590815621E-6,0.199031231385238,
0.613338043951791),.UNSPECIFIED.);
#883=B_SPLINE_CURVE_WITH_KNOTS('',3,(#61308,#61309,#61310,#61311,#61312,
#61313,#61314,#61315,#61316,#61317,#61318,#61319,#61320,#61321),
 .UNSPECIFIED.,.F.,.F.,(4,2,2,2,2,2,4),(-1.36940170500402,-1.09988295614753,
-0.874791882030613,-0.683052425013262,-0.491992883634759,-0.265273198644392,
-1.00032379802467E-6),.UNSPECIFIED.);
#884=B_SPLINE_CURVE_WITH_KNOTS('',3,(#61322,#61323,#61324,#61325,#61326,
#61327),.UNSPECIFIED.,.F.,.F.,(4,2,4),(2.55717115154207E-6,0.198998134710777,
0.338859911257635),.UNSPECIFIED.);
#885=B_SPLINE_CURVE_WITH_KNOTS('',3,(#61384,#61385,#61386,#61387,#61388,
#61389,#61390,#61391,#61392,#61393,#61394,#61395,#61396,#61397),
 .UNSPECIFIED.,.F.,.F.,(4,2,2,2,2,2,4),(0.0377143719414213,0.167070624995476,
0.336553194126115,0.499999999999991,0.663446805873868,0.832929375004528,
0.962285628058582),.UNSPECIFIED.);
#886=B_SPLINE_CURVE_WITH_KNOTS('',3,(#62043,#62044,#62045,#62046,#62047,
#62048),.UNSPECIFIED.,.F.,.F.,(4,2,4),(2.35124835048059E-5,0.0896951576367538,
0.182831089214791),.UNSPECIFIED.);
#887=B_SPLINE_CURVE_WITH_KNOTS('',3,(#62050,#62051,#62052,#62053,#62054,
#62055),.UNSPECIFIED.,.F.,.F.,(4,2,4),(1.00039620620053E-6,0.178978044961171,
0.576833929771009),.UNSPECIFIED.);
#888=B_SPLINE_CURVE_WITH_KNOTS('',3,(#62057,#62058,#62059,#62060,#62061,
#62062,#62063,#62064,#62065,#62066,#62067,#62068,#62069,#62070),
 .UNSPECIFIED.,.F.,.F.,(4,2,2,2,2,2,4),(-1.35020638398027,-1.08443693237292,
-0.862819012108596,-0.674058735997087,-0.48593035055054,-0.262536029678697,
-1.00008876609848E-6),.UNSPECIFIED.);
#889=B_SPLINE_CURVE_WITH_KNOTS('',3,(#62072,#62073,#62074,#62075,#62076,
#62077),.UNSPECIFIED.,.F.,.F.,(4,2,4),(4.60565042976658E-5,0.201020831894536,
0.382076214067163),.UNSPECIFIED.);
#890=B_SPLINE_CURVE_WITH_KNOTS('',3,(#62078,#62079,#62080,#62081,#62082,
#62083),.UNSPECIFIED.,.F.,.F.,(4,2,4),(0.,0.0817717936353896,0.122657946516836),
 .UNSPECIFIED.);
#891=B_SPLINE_CURVE_WITH_KNOTS('',3,(#62086,#62087,#62088,#62089,#62090,
#62091),.UNSPECIFIED.,.F.,.F.,(4,2,4),(4.16219211490419E-13,0.0801522498243031,
0.181100777626267),.UNSPECIFIED.);
#892=B_SPLINE_CURVE_WITH_KNOTS('',3,(#62097,#62098,#62099,#62100,#62101,
#62102),.UNSPECIFIED.,.F.,.F.,(4,2,4),(9.76525933546162E-5,0.171030074764551,
0.274312857421989),.UNSPECIFIED.);
#893=B_SPLINE_CURVE_WITH_KNOTS('',3,(#62529,#62530,#62531,#62532,#62533,
#62534,#62535,#62536,#62537,#62538,#62539,#62540,#62541,#62542),
 .UNSPECIFIED.,.F.,.F.,(4,2,2,2,2,2,4),(0.0377143719414213,0.167070624995476,
0.336553194126115,0.499999999999991,0.663446805873868,0.832929375004528,
0.962285628058582),.UNSPECIFIED.);
#894=B_SPLINE_CURVE_WITH_KNOTS('',3,(#62544,#62545,#62546,#62547,#62548,
#62549),.UNSPECIFIED.,.F.,.F.,(4,2,4),(3.73183726292144E-5,0.103357039408085,
0.159897599535642),.UNSPECIFIED.);
#895=B_SPLINE_CURVE_WITH_KNOTS('',3,(#62551,#62552,#62553,#62554,#62555,
#62556,#62557,#62558),.UNSPECIFIED.,.F.,.F.,(4,2,2,4),(1.00587379666966E-6,
0.192203020379571,0.269152108519518,0.528949682547937),.UNSPECIFIED.);
#896=B_SPLINE_CURVE_WITH_KNOTS('',3,(#62559,#62560,#62561,#62562,#62563,
#62564,#62565,#62566,#62567,#62568,#62569,#62570,#62571,#62572),
 .UNSPECIFIED.,.F.,.F.,(4,2,2,2,2,2,4),(-1.36643940243578,-1.09802651843964,
-0.87334041482261,-0.68198104582902,-0.491290408247465,-0.264952115802241,
-1.00035096156786E-6),.UNSPECIFIED.);
#897=B_SPLINE_CURVE_WITH_KNOTS('',3,(#62629,#62630,#62631,#62632,#62633,
#62634,#62635,#62636,#62637,#62638,#62639,#62640,#62641,#62642),
 .UNSPECIFIED.,.F.,.F.,(4,2,2,2,2,2,4),(0.0377143719414213,0.167070624995476,
0.336553194126115,0.499999999999991,0.663446805873868,0.832929375004528,
0.962285628058582),.UNSPECIFIED.);
#1235=CONICAL_SURFACE('',#16478,3.325,0.785398163397446);
#1236=CONICAL_SURFACE('',#16516,3.325,0.785398163397448);
#1237=CONICAL_SURFACE('',#16549,4.9,0.785398163397446);
#1238=CONICAL_SURFACE('',#16557,4.9,0.785398163397446);
#1239=CONICAL_SURFACE('',#16558,4.9,0.785398163397446);
#1240=CONICAL_SURFACE('',#16566,4.9,0.785398163397446);
#1241=CONICAL_SURFACE('',#16567,4.9,0.785398163397446);
#1242=CONICAL_SURFACE('',#16575,4.9,0.785398163397446);
#1243=CONICAL_SURFACE('',#16576,4.9,0.785398163397446);
#1244=CONICAL_SURFACE('',#16584,4.9,0.785398163397446);
#1245=CONICAL_SURFACE('',#16585,4.9,0.785398163397446);
#1246=CONICAL_SURFACE('',#16593,4.9,0.785398163397446);
#1247=CONICAL_SURFACE('',#16594,4.9,0.785398163397446);
#1248=CONICAL_SURFACE('',#16602,4.9,0.785398163397446);
#1249=CONICAL_SURFACE('',#16603,4.9,0.785398163397446);
#1250=CONICAL_SURFACE('',#16611,4.9,0.785398163397446);
#1251=CONICAL_SURFACE('',#16612,4.9,0.785398163397446);
#1252=CONICAL_SURFACE('',#16620,4.9,0.785398163397446);
#1253=CONICAL_SURFACE('',#16621,4.9,0.785398163397446);
#1254=CONICAL_SURFACE('',#16629,4.9,0.785398163397446);
#1255=CONICAL_SURFACE('',#16630,4.9,0.785398163397446);
#1256=CONICAL_SURFACE('',#16638,4.9,0.785398163397446);
#1257=CONICAL_SURFACE('',#16639,4.9,0.785398163397446);
#1258=CONICAL_SURFACE('',#16647,4.9,0.785398163397446);
#1259=CONICAL_SURFACE('',#16648,4.9,0.785398163397446);
#1260=CONICAL_SURFACE('',#16656,4.9,0.785398163397446);
#1261=CONICAL_SURFACE('',#16657,4.9,0.785398163397446);
#1262=CONICAL_SURFACE('',#16665,4.9,0.785398163397446);
#1263=CONICAL_SURFACE('',#16666,4.9,0.785398163397446);
#1264=CONICAL_SURFACE('',#16674,4.9,0.785398163397446);
#1265=CONICAL_SURFACE('',#16675,4.9,0.785398163397446);
#1266=CONICAL_SURFACE('',#16683,4.9,0.785398163397446);
#1267=CONICAL_SURFACE('',#16684,4.9,0.785398163397446);
#1268=CONICAL_SURFACE('',#16692,4.9,0.785398163397446);
#1269=CONICAL_SURFACE('',#16693,4.9,0.785398163397446);
#1270=CONICAL_SURFACE('',#16701,4.9,0.785398163397446);
#1271=CONICAL_SURFACE('',#16702,4.9,0.785398163397446);
#1272=CONICAL_SURFACE('',#16710,4.9,0.785398163397446);
#1273=CONICAL_SURFACE('',#16711,4.9,0.785398163397446);
#1274=CONICAL_SURFACE('',#16719,4.9,0.785398163397446);
#1275=CONICAL_SURFACE('',#16720,4.9,0.785398163397446);
#1276=CONICAL_SURFACE('',#16728,4.9,0.785398163397446);
#1277=CONICAL_SURFACE('',#16729,4.9,0.785398163397446);
#1278=CONICAL_SURFACE('',#16737,4.9,0.785398163397446);
#1279=CONICAL_SURFACE('',#16738,4.9,0.785398163397446);
#1280=CONICAL_SURFACE('',#16746,4.9,0.785398163397446);
#1281=CONICAL_SURFACE('',#16747,4.9,0.785398163397446);
#1282=CONICAL_SURFACE('',#16755,4.9,0.785398163397446);
#1283=CONICAL_SURFACE('',#16756,4.9,0.785398163397446);
#1284=CONICAL_SURFACE('',#16764,4.9,0.785398163397446);
#1285=CONICAL_SURFACE('',#16765,4.9,0.785398163397446);
#1286=CONICAL_SURFACE('',#16773,4.9,0.785398163397446);
#1287=CONICAL_SURFACE('',#16774,4.9,0.785398163397446);
#1288=CONICAL_SURFACE('',#16782,4.9,0.785398163397446);
#1289=CONICAL_SURFACE('',#16783,4.9,0.785398163397446);
#1290=CONICAL_SURFACE('',#16791,4.9,0.785398163397446);
#1291=CONICAL_SURFACE('',#16792,4.9,0.785398163397446);
#1292=CONICAL_SURFACE('',#16794,4.9,0.785398163397446);
#1293=CONICAL_SURFACE('',#16802,4.9,0.785398163397446);
#1294=CONICAL_SURFACE('',#16803,4.9,0.785398163397446);
#1295=CONICAL_SURFACE('',#16809,4.9,0.785398163397446);
#1296=CONICAL_SURFACE('',#16818,4.9,0.785398163397446);
#1446=CYLINDRICAL_SURFACE('',#16482,3.3);
#1447=CYLINDRICAL_SURFACE('',#16551,4.95);
#1448=CYLINDRICAL_SURFACE('',#16555,4.95);
#1449=CYLINDRICAL_SURFACE('',#16560,4.95);
#1450=CYLINDRICAL_SURFACE('',#16564,4.95);
#1451=CYLINDRICAL_SURFACE('',#16569,4.95);
#1452=CYLINDRICAL_SURFACE('',#16573,4.95);
#1453=CYLINDRICAL_SURFACE('',#16578,4.95);
#1454=CYLINDRICAL_SURFACE('',#16582,4.95);
#1455=CYLINDRICAL_SURFACE('',#16587,4.95);
#1456=CYLINDRICAL_SURFACE('',#16591,4.95);
#1457=CYLINDRICAL_SURFACE('',#16596,4.95);
#1458=CYLINDRICAL_SURFACE('',#16600,4.95);
#1459=CYLINDRICAL_SURFACE('',#16605,4.95);
#1460=CYLINDRICAL_SURFACE('',#16609,4.95);
#1461=CYLINDRICAL_SURFACE('',#16614,4.95);
#1462=CYLINDRICAL_SURFACE('',#16618,4.95);
#1463=CYLINDRICAL_SURFACE('',#16623,4.95);
#1464=CYLINDRICAL_SURFACE('',#16627,4.95);
#1465=CYLINDRICAL_SURFACE('',#16632,4.95);
#1466=CYLINDRICAL_SURFACE('',#16636,4.95);
#1467=CYLINDRICAL_SURFACE('',#16641,4.95);
#1468=CYLINDRICAL_SURFACE('',#16645,4.95);
#1469=CYLINDRICAL_SURFACE('',#16650,4.95);
#1470=CYLINDRICAL_SURFACE('',#16654,4.95);
#1471=CYLINDRICAL_SURFACE('',#16659,4.95);
#1472=CYLINDRICAL_SURFACE('',#16663,4.95);
#1473=CYLINDRICAL_SURFACE('',#16668,4.95);
#1474=CYLINDRICAL_SURFACE('',#16672,4.95);
#1475=CYLINDRICAL_SURFACE('',#16677,4.95);
#1476=CYLINDRICAL_SURFACE('',#16681,4.95);
#1477=CYLINDRICAL_SURFACE('',#16686,4.95);
#1478=CYLINDRICAL_SURFACE('',#16690,4.95);
#1479=CYLINDRICAL_SURFACE('',#16695,4.95);
#1480=CYLINDRICAL_SURFACE('',#16699,4.95);
#1481=CYLINDRICAL_SURFACE('',#16704,4.95);
#1482=CYLINDRICAL_SURFACE('',#16708,4.95);
#1483=CYLINDRICAL_SURFACE('',#16713,4.95);
#1484=CYLINDRICAL_SURFACE('',#16717,4.95);
#1485=CYLINDRICAL_SURFACE('',#16722,4.95);
#1486=CYLINDRICAL_SURFACE('',#16726,4.95);
#1487=CYLINDRICAL_SURFACE('',#16731,4.95);
#1488=CYLINDRICAL_SURFACE('',#16735,4.95);
#1489=CYLINDRICAL_SURFACE('',#16740,4.95);
#1490=CYLINDRICAL_SURFACE('',#16744,4.95);
#1491=CYLINDRICAL_SURFACE('',#16749,4.95);
#1492=CYLINDRICAL_SURFACE('',#16753,4.95);
#1493=CYLINDRICAL_SURFACE('',#16758,4.95);
#1494=CYLINDRICAL_SURFACE('',#16762,4.95);
#1495=CYLINDRICAL_SURFACE('',#16767,4.95);
#1496=CYLINDRICAL_SURFACE('',#16771,4.95);
#1497=CYLINDRICAL_SURFACE('',#16776,4.95);
#1498=CYLINDRICAL_SURFACE('',#16780,4.95);
#1499=CYLINDRICAL_SURFACE('',#16785,4.95);
#1500=CYLINDRICAL_SURFACE('',#16789,4.95);
#1501=CYLINDRICAL_SURFACE('',#16796,4.95);
#1502=CYLINDRICAL_SURFACE('',#16800,4.95);
#1503=CYLINDRICAL_SURFACE('',#16805,4.95);
#1504=CYLINDRICAL_SURFACE('',#16807,4.95);
#1505=CYLINDRICAL_SURFACE('',#16813,4.95);
#1506=CYLINDRICAL_SURFACE('',#16814,4.95);
#1704=FACE_BOUND('',#3745,.T.);
#1705=FACE_BOUND('',#3748,.T.);
#2012=CIRCLE('',#16479,3.3);
#2013=CIRCLE('',#16480,3.35);
#2014=CIRCLE('',#16481,3.3);
#2015=CIRCLE('',#16483,3.3);
#2016=CIRCLE('',#16484,3.3);
#2017=CIRCLE('',#16486,4.85);
#2018=CIRCLE('',#16487,4.85);
#2019=CIRCLE('',#16488,4.85);
#2020=CIRCLE('',#16489,4.85);
#2021=CIRCLE('',#16490,4.85);
#2022=CIRCLE('',#16491,4.85);
#2023=CIRCLE('',#16492,4.85);
#2024=CIRCLE('',#16493,4.85);
#2025=CIRCLE('',#16494,4.85);
#2026=CIRCLE('',#16495,4.85);
#2027=CIRCLE('',#16496,4.85);
#2028=CIRCLE('',#16497,4.85);
#2029=CIRCLE('',#16498,4.85);
#2030=CIRCLE('',#16499,4.85);
#2031=CIRCLE('',#16500,4.85);
#2032=CIRCLE('',#16501,4.85);
#2033=CIRCLE('',#16502,4.85);
#2034=CIRCLE('',#16503,4.85);
#2035=CIRCLE('',#16504,4.85);
#2036=CIRCLE('',#16505,4.85);
#2037=CIRCLE('',#16506,4.85);
#2038=CIRCLE('',#16507,4.85);
#2039=CIRCLE('',#16508,4.85);
#2040=CIRCLE('',#16509,4.85);
#2041=CIRCLE('',#16510,4.85);
#2042=CIRCLE('',#16511,4.85);
#2043=CIRCLE('',#16512,4.85);
#2044=CIRCLE('',#16513,4.85);
#2045=CIRCLE('',#16514,4.85);
#2046=CIRCLE('',#16515,4.85);
#2047=CIRCLE('',#16517,3.35);
#2048=CIRCLE('',#16519,4.85);
#2049=CIRCLE('',#16520,4.85);
#2050=CIRCLE('',#16521,4.85);
#2051=CIRCLE('',#16522,4.85);
#2052=CIRCLE('',#16523,4.85);
#2053=CIRCLE('',#16524,4.85);
#2054=CIRCLE('',#16525,4.85);
#2055=CIRCLE('',#16526,4.85);
#2056=CIRCLE('',#16527,4.85);
#2057=CIRCLE('',#16528,4.85);
#2058=CIRCLE('',#16529,4.85);
#2059=CIRCLE('',#16530,4.85);
#2060=CIRCLE('',#16531,4.85);
#2061=CIRCLE('',#16532,4.85);
#2062=CIRCLE('',#16533,4.85);
#2063=CIRCLE('',#16534,4.85);
#2064=CIRCLE('',#16535,4.85);
#2065=CIRCLE('',#16536,4.85);
#2066=CIRCLE('',#16537,4.85);
#2067=CIRCLE('',#16538,4.85);
#2068=CIRCLE('',#16539,4.85);
#2069=CIRCLE('',#16540,4.85);
#2070=CIRCLE('',#16541,4.85);
#2071=CIRCLE('',#16542,4.85);
#2072=CIRCLE('',#16543,4.85);
#2073=CIRCLE('',#16544,4.85);
#2074=CIRCLE('',#16545,4.85);
#2075=CIRCLE('',#16546,4.85);
#2076=CIRCLE('',#16547,4.85);
#2077=CIRCLE('',#16548,4.85);
#2078=CIRCLE('',#16550,4.95);
#2079=CIRCLE('',#16552,4.95);
#2080=CIRCLE('',#16554,4.95);
#2081=CIRCLE('',#16556,4.95);
#2082=CIRCLE('',#16559,4.95);
#2083=CIRCLE('',#16561,4.95);
#2084=CIRCLE('',#16563,4.95);
#2085=CIRCLE('',#16565,4.95);
#2086=CIRCLE('',#16568,4.95);
#2087=CIRCLE('',#16570,4.95);
#2088=CIRCLE('',#16572,4.95);
#2089=CIRCLE('',#16574,4.95);
#2090=CIRCLE('',#16577,4.95);
#2091=CIRCLE('',#16579,4.95);
#2092=CIRCLE('',#16581,4.95);
#2093=CIRCLE('',#16583,4.95);
#2094=CIRCLE('',#16586,4.95);
#2095=CIRCLE('',#16588,4.95);
#2096=CIRCLE('',#16590,4.95);
#2097=CIRCLE('',#16592,4.95);
#2098=CIRCLE('',#16595,4.95);
#2099=CIRCLE('',#16597,4.95);
#2100=CIRCLE('',#16599,4.95);
#2101=CIRCLE('',#16601,4.95);
#2102=CIRCLE('',#16604,4.95);
#2103=CIRCLE('',#16606,4.95);
#2104=CIRCLE('',#16608,4.95);
#2105=CIRCLE('',#16610,4.95);
#2106=CIRCLE('',#16613,4.95);
#2107=CIRCLE('',#16615,4.95);
#2108=CIRCLE('',#16617,4.95);
#2109=CIRCLE('',#16619,4.95);
#2110=CIRCLE('',#16622,4.95);
#2111=CIRCLE('',#16624,4.95);
#2112=CIRCLE('',#16626,4.95);
#2113=CIRCLE('',#16628,4.95);
#2114=CIRCLE('',#16631,4.95);
#2115=CIRCLE('',#16633,4.95);
#2116=CIRCLE('',#16635,4.95);
#2117=CIRCLE('',#16637,4.95);
#2118=CIRCLE('',#16640,4.95);
#2119=CIRCLE('',#16642,4.95);
#2120=CIRCLE('',#16644,4.95);
#2121=CIRCLE('',#16646,4.95);
#2122=CIRCLE('',#16649,4.95);
#2123=CIRCLE('',#16651,4.95);
#2124=CIRCLE('',#16653,4.95);
#2125=CIRCLE('',#16655,4.95);
#2126=CIRCLE('',#16658,4.95);
#2127=CIRCLE('',#16660,4.95);
#2128=CIRCLE('',#16662,4.95);
#2129=CIRCLE('',#16664,4.95);
#2130=CIRCLE('',#16667,4.95);
#2131=CIRCLE('',#16669,4.95);
#2132=CIRCLE('',#16671,4.95);
#2133=CIRCLE('',#16673,4.95);
#2134=CIRCLE('',#16676,4.95);
#2135=CIRCLE('',#16678,4.95);
#2136=CIRCLE('',#16680,4.95);
#2137=CIRCLE('',#16682,4.95);
#2138=CIRCLE('',#16685,4.95);
#2139=CIRCLE('',#16687,4.95);
#2140=CIRCLE('',#16689,4.95);
#2141=CIRCLE('',#16691,4.95);
#2142=CIRCLE('',#16694,4.95);
#2143=CIRCLE('',#16696,4.95);
#2144=CIRCLE('',#16698,4.95);
#2145=CIRCLE('',#16700,4.95);
#2146=CIRCLE('',#16703,4.95);
#2147=CIRCLE('',#16705,4.95);
#2148=CIRCLE('',#16707,4.95);
#2149=CIRCLE('',#16709,4.95);
#2150=CIRCLE('',#16712,4.95);
#2151=CIRCLE('',#16714,4.95);
#2152=CIRCLE('',#16716,4.95);
#2153=CIRCLE('',#16718,4.95);
#2154=CIRCLE('',#16721,4.95);
#2155=CIRCLE('',#16723,4.95);
#2156=CIRCLE('',#16725,4.95);
#2157=CIRCLE('',#16727,4.95);
#2158=CIRCLE('',#16730,4.95);
#2159=CIRCLE('',#16732,4.95);
#2160=CIRCLE('',#16734,4.95);
#2161=CIRCLE('',#16736,4.95);
#2162=CIRCLE('',#16739,4.95);
#2163=CIRCLE('',#16741,4.95);
#2164=CIRCLE('',#16743,4.95);
#2165=CIRCLE('',#16745,4.95);
#2166=CIRCLE('',#16748,4.95);
#2167=CIRCLE('',#16750,4.95);
#2168=CIRCLE('',#16752,4.95);
#2169=CIRCLE('',#16754,4.95);
#2170=CIRCLE('',#16757,4.95);
#2171=CIRCLE('',#16759,4.95);
#2172=CIRCLE('',#16761,4.95);
#2173=CIRCLE('',#16763,4.95);
#2174=CIRCLE('',#16766,4.95);
#2175=CIRCLE('',#16768,4.95);
#2176=CIRCLE('',#16770,4.95);
#2177=CIRCLE('',#16772,4.95);
#2178=CIRCLE('',#16775,4.95);
#2179=CIRCLE('',#16777,4.95);
#2180=CIRCLE('',#16779,4.95);
#2181=CIRCLE('',#16781,4.95);
#2182=CIRCLE('',#16784,4.95);
#2183=CIRCLE('',#16786,4.95);
#2184=CIRCLE('',#16788,4.95);
#2185=CIRCLE('',#16790,4.95);
#2186=CIRCLE('',#16793,4.95);
#2187=CIRCLE('',#16795,4.95);
#2188=CIRCLE('',#16797,4.95);
#2189=CIRCLE('',#16799,4.95);
#2190=CIRCLE('',#16801,4.95);
#2191=CIRCLE('',#16804,4.95);
#2192=CIRCLE('',#16806,4.95);
#2193=CIRCLE('',#16808,4.95);
#2194=CIRCLE('',#16810,4.95);
#2195=CIRCLE('',#16812,4.95);
#2196=CIRCLE('',#16815,4.95);
#2197=CIRCLE('',#16816,4.95);
#2768=FACE_OUTER_BOUND('',#3742,.T.);
#2769=FACE_OUTER_BOUND('',#3743,.T.);
#2770=FACE_OUTER_BOUND('',#3744,.T.);
#2771=FACE_OUTER_BOUND('',#3746,.T.);
#2772=FACE_OUTER_BOUND('',#3747,.T.);
#2773=FACE_OUTER_BOUND('',#3749,.T.);
#2774=FACE_OUTER_BOUND('',#3750,.T.);
#2775=FACE_OUTER_BOUND('',#3751,.T.);
#2776=FACE_OUTER_BOUND('',#3752,.T.);
#2777=FACE_OUTER_BOUND('',#3753,.T.);
#2778=FACE_OUTER_BOUND('',#3754,.T.);
#2779=FACE_OUTER_BOUND('',#3755,.T.);
#2780=FACE_OUTER_BOUND('',#3756,.T.);
#2781=FACE_OUTER_BOUND('',#3757,.T.);
#2782=FACE_OUTER_BOUND('',#3758,.T.);
#2783=FACE_OUTER_BOUND('',#3759,.T.);
#2784=FACE_OUTER_BOUND('',#3760,.T.);
#2785=FACE_OUTER_BOUND('',#3761,.T.);
#2786=FACE_OUTER_BOUND('',#3762,.T.);
#2787=FACE_OUTER_BOUND('',#3763,.T.);
#2788=FACE_OUTER_BOUND('',#3764,.T.);
#2789=FACE_OUTER_BOUND('',#3765,.T.);
#2790=FACE_OUTER_BOUND('',#3766,.T.);
#2791=FACE_OUTER_BOUND('',#3767,.T.);
#2792=FACE_OUTER_BOUND('',#3768,.T.);
#2793=FACE_OUTER_BOUND('',#3769,.T.);
#2794=FACE_OUTER_BOUND('',#3770,.T.);
#2795=FACE_OUTER_BOUND('',#3771,.T.);
#2796=FACE_OUTER_BOUND('',#3772,.T.);
#2797=FACE_OUTER_BOUND('',#3773,.T.);
#2798=FACE_OUTER_BOUND('',#3774,.T.);
#2799=FACE_OUTER_BOUND('',#3775,.T.);
#2800=FACE_OUTER_BOUND('',#3776,.T.);
#2801=FACE_OUTER_BOUND('',#3777,.T.);
#2802=FACE_OUTER_BOUND('',#3778,.T.);
#2803=FACE_OUTER_BOUND('',#3779,.T.);
#2804=FACE_OUTER_BOUND('',#3780,.T.);
#2805=FACE_OUTER_BOUND('',#3781,.T.);
#2806=FACE_OUTER_BOUND('',#3782,.T.);
#2807=FACE_OUTER_BOUND('',#3783,.T.);
#2808=FACE_OUTER_BOUND('',#3784,.T.);
#2809=FACE_OUTER_BOUND('',#3785,.T.);
#2810=FACE_OUTER_BOUND('',#3786,.T.);
#2811=FACE_OUTER_BOUND('',#3787,.T.);
#2812=FACE_OUTER_BOUND('',#3788,.T.);
#2813=FACE_OUTER_BOUND('',#3789,.T.);
#2814=FACE_OUTER_BOUND('',#3790,.T.);
#2815=FACE_OUTER_BOUND('',#3791,.T.);
#2816=FACE_OUTER_BOUND('',#3792,.T.);
#2817=FACE_OUTER_BOUND('',#3793,.T.);
#2818=FACE_OUTER_BOUND('',#3794,.T.);
#2819=FACE_OUTER_BOUND('',#3795,.T.);
#2820=FACE_OUTER_BOUND('',#3796,.T.);
#2821=FACE_OUTER_BOUND('',#3797,.T.);
#2822=FACE_OUTER_BOUND('',#3798,.T.);
#2823=FACE_OUTER_BOUND('',#3799,.T.);
#2824=FACE_OUTER_BOUND('',#3800,.T.);
#2825=FACE_OUTER_BOUND('',#3801,.T.);
#2826=FACE_OUTER_BOUND('',#3802,.T.);
#2827=FACE_OUTER_BOUND('',#3803,.T.);
#2828=FACE_OUTER_BOUND('',#3804,.T.);
#2829=FACE_OUTER_BOUND('',#3805,.T.);
#2830=FACE_OUTER_BOUND('',#3806,.T.);
#2831=FACE_OUTER_BOUND('',#3807,.T.);
#2832=FACE_OUTER_BOUND('',#3808,.T.);
#2833=FACE_OUTER_BOUND('',#3809,.T.);
#2834=FACE_OUTER_BOUND('',#3810,.T.);
#2835=FACE_OUTER_BOUND('',#3811,.T.);
#2836=FACE_OUTER_BOUND('',#3812,.T.);
#2837=FACE_OUTER_BOUND('',#3813,.T.);
#2838=FACE_OUTER_BOUND('',#3814,.T.);
#2839=FACE_OUTER_BOUND('',#3815,.T.);
#2840=FACE_OUTER_BOUND('',#3816,.T.);
#2841=FACE_OUTER_BOUND('',#3817,.T.);
#2842=FACE_OUTER_BOUND('',#3818,.T.);
#2843=FACE_OUTER_BOUND('',#3819,.T.);
#2844=FACE_OUTER_BOUND('',#3820,.T.);
#2845=FACE_OUTER_BOUND('',#3821,.T.);
#2846=FACE_OUTER_BOUND('',#3822,.T.);
#2847=FACE_OUTER_BOUND('',#3823,.T.);
#2848=FACE_OUTER_BOUND('',#3824,.T.);
#2849=FACE_OUTER_BOUND('',#3825,.T.);
#2850=FACE_OUTER_BOUND('',#3826,.T.);
#2851=FACE_OUTER_BOUND('',#3827,.T.);
#2852=FACE_OUTER_BOUND('',#3828,.T.);
#2853=FACE_OUTER_BOUND('',#3829,.T.);
#2854=FACE_OUTER_BOUND('',#3830,.T.);
#2855=FACE_OUTER_BOUND('',#3831,.T.);
#2856=FACE_OUTER_BOUND('',#3832,.T.);
#2857=FACE_OUTER_BOUND('',#3833,.T.);
#2858=FACE_OUTER_BOUND('',#3834,.T.);
#2859=FACE_OUTER_BOUND('',#3835,.T.);
#2860=FACE_OUTER_BOUND('',#3836,.T.);
#2861=FACE_OUTER_BOUND('',#3837,.T.);
#2862=FACE_OUTER_BOUND('',#3838,.T.);
#2863=FACE_OUTER_BOUND('',#3839,.T.);
#2864=FACE_OUTER_BOUND('',#3840,.T.);
#2865=FACE_OUTER_BOUND('',#3841,.T.);
#2866=FACE_OUTER_BOUND('',#3842,.T.);
#2867=FACE_OUTER_BOUND('',#3843,.T.);
#2868=FACE_OUTER_BOUND('',#3844,.T.);
#2869=FACE_OUTER_BOUND('',#3845,.T.);
#2870=FACE_OUTER_BOUND('',#3846,.T.);
#2871=FACE_OUTER_BOUND('',#3847,.T.);
#2872=FACE_OUTER_BOUND('',#3848,.T.);
#2873=FACE_OUTER_BOUND('',#3849,.T.);
#2874=FACE_OUTER_BOUND('',#3850,.T.);
#2875=FACE_OUTER_BOUND('',#3851,.T.);
#2876=FACE_OUTER_BOUND('',#3852,.T.);
#2877=FACE_OUTER_BOUND('',#3853,.T.);
#2878=FACE_OUTER_BOUND('',#3854,.T.);
#2879=FACE_OUTER_BOUND('',#3855,.T.);
#2880=FACE_OUTER_BOUND('',#3856,.T.);
#2881=FACE_OUTER_BOUND('',#3857,.T.);
#2882=FACE_OUTER_BOUND('',#3858,.T.);
#2883=FACE_OUTER_BOUND('',#3859,.T.);
#2884=FACE_OUTER_BOUND('',#3860,.T.);
#2885=FACE_OUTER_BOUND('',#3861,.T.);
#2886=FACE_OUTER_BOUND('',#3862,.T.);
#2887=FACE_OUTER_BOUND('',#3863,.T.);
#2888=FACE_OUTER_BOUND('',#3864,.T.);
#2889=FACE_OUTER_BOUND('',#3865,.T.);
#2890=FACE_OUTER_BOUND('',#3866,.T.);
#2891=FACE_OUTER_BOUND('',#3867,.T.);
#2892=FACE_OUTER_BOUND('',#3868,.T.);
#2893=FACE_OUTER_BOUND('',#3869,.T.);
#2894=FACE_OUTER_BOUND('',#3870,.T.);
#2895=FACE_OUTER_BOUND('',#3871,.T.);
#2896=FACE_OUTER_BOUND('',#3872,.T.);
#2897=FACE_OUTER_BOUND('',#3873,.T.);
#2898=FACE_OUTER_BOUND('',#3874,.T.);
#2899=FACE_OUTER_BOUND('',#3875,.T.);
#2900=FACE_OUTER_BOUND('',#3876,.T.);
#2901=FACE_OUTER_BOUND('',#3877,.T.);
#2902=FACE_OUTER_BOUND('',#3878,.T.);
#2903=FACE_OUTER_BOUND('',#3879,.T.);
#2904=FACE_OUTER_BOUND('',#3880,.T.);
#2905=FACE_OUTER_BOUND('',#3881,.T.);
#2906=FACE_OUTER_BOUND('',#3882,.T.);
#2907=FACE_OUTER_BOUND('',#3883,.T.);
#2908=FACE_OUTER_BOUND('',#3884,.T.);
#2909=FACE_OUTER_BOUND('',#3885,.T.);
#2910=FACE_OUTER_BOUND('',#3886,.T.);
#2911=FACE_OUTER_BOUND('',#3887,.T.);
#2912=FACE_OUTER_BOUND('',#3888,.T.);
#2913=FACE_OUTER_BOUND('',#3889,.T.);
#2914=FACE_OUTER_BOUND('',#3890,.T.);
#2915=FACE_OUTER_BOUND('',#3891,.T.);
#2916=FACE_OUTER_BOUND('',#3892,.T.);
#2917=FACE_OUTER_BOUND('',#3893,.T.);
#2918=FACE_OUTER_BOUND('',#3894,.T.);
#2919=FACE_OUTER_BOUND('',#3895,.T.);
#2920=FACE_OUTER_BOUND('',#3896,.T.);
#2921=FACE_OUTER_BOUND('',#3897,.T.);
#2922=FACE_OUTER_BOUND('',#3898,.T.);
#2923=FACE_OUTER_BOUND('',#3899,.T.);
#2924=FACE_OUTER_BOUND('',#3900,.T.);
#2925=FACE_OUTER_BOUND('',#3901,.T.);
#2926=FACE_OUTER_BOUND('',#3902,.T.);
#2927=FACE_OUTER_BOUND('',#3903,.T.);
#2928=FACE_OUTER_BOUND('',#3904,.T.);
#2929=FACE_OUTER_BOUND('',#3905,.T.);
#2930=FACE_OUTER_BOUND('',#3906,.T.);
#2931=FACE_OUTER_BOUND('',#3907,.T.);
#2932=FACE_OUTER_BOUND('',#3908,.T.);
#2933=FACE_OUTER_BOUND('',#3909,.T.);
#2934=FACE_OUTER_BOUND('',#3910,.T.);
#2935=FACE_OUTER_BOUND('',#3911,.T.);
#2936=FACE_OUTER_BOUND('',#3912,.T.);
#2937=FACE_OUTER_BOUND('',#3913,.T.);
#2938=FACE_OUTER_BOUND('',#3914,.T.);
#2939=FACE_OUTER_BOUND('',#3915,.T.);
#2940=FACE_OUTER_BOUND('',#3916,.T.);
#2941=FACE_OUTER_BOUND('',#3917,.T.);
#2942=FACE_OUTER_BOUND('',#3918,.T.);
#2943=FACE_OUTER_BOUND('',#3919,.T.);
#2944=FACE_OUTER_BOUND('',#3920,.T.);
#2945=FACE_OUTER_BOUND('',#3921,.T.);
#2946=FACE_OUTER_BOUND('',#3922,.T.);
#2947=FACE_OUTER_BOUND('',#3923,.T.);
#2948=FACE_OUTER_BOUND('',#3924,.T.);
#2949=FACE_OUTER_BOUND('',#3925,.T.);
#2950=FACE_OUTER_BOUND('',#3926,.T.);
#2951=FACE_OUTER_BOUND('',#3927,.T.);
#2952=FACE_OUTER_BOUND('',#3928,.T.);
#2953=FACE_OUTER_BOUND('',#3929,.T.);
#2954=FACE_OUTER_BOUND('',#3930,.T.);
#2955=FACE_OUTER_BOUND('',#3931,.T.);
#2956=FACE_OUTER_BOUND('',#3932,.T.);
#2957=FACE_OUTER_BOUND('',#3933,.T.);
#2958=FACE_OUTER_BOUND('',#3934,.T.);
#2959=FACE_OUTER_BOUND('',#3935,.T.);
#2960=FACE_OUTER_BOUND('',#3936,.T.);
#2961=FACE_OUTER_BOUND('',#3937,.T.);
#2962=FACE_OUTER_BOUND('',#3938,.T.);
#2963=FACE_OUTER_BOUND('',#3939,.T.);
#2964=FACE_OUTER_BOUND('',#3940,.T.);
#2965=FACE_OUTER_BOUND('',#3941,.T.);
#2966=FACE_OUTER_BOUND('',#3942,.T.);
#2967=FACE_OUTER_BOUND('',#3943,.T.);
#2968=FACE_OUTER_BOUND('',#3944,.T.);
#2969=FACE_OUTER_BOUND('',#3945,.T.);
#2970=FACE_OUTER_BOUND('',#3946,.T.);
#2971=FACE_OUTER_BOUND('',#3947,.T.);
#2972=FACE_OUTER_BOUND('',#3948,.T.);
#2973=FACE_OUTER_BOUND('',#3949,.T.);
#2974=FACE_OUTER_BOUND('',#3950,.T.);
#2975=FACE_OUTER_BOUND('',#3951,.T.);
#2976=FACE_OUTER_BOUND('',#3952,.T.);
#2977=FACE_OUTER_BOUND('',#3953,.T.);
#2978=FACE_OUTER_BOUND('',#3954,.T.);
#2979=FACE_OUTER_BOUND('',#3955,.T.);
#2980=FACE_OUTER_BOUND('',#3956,.T.);
#2981=FACE_OUTER_BOUND('',#3957,.T.);
#2982=FACE_OUTER_BOUND('',#3958,.T.);
#2983=FACE_OUTER_BOUND('',#3959,.T.);
#2984=FACE_OUTER_BOUND('',#3960,.T.);
#2985=FACE_OUTER_BOUND('',#3961,.T.);
#2986=FACE_OUTER_BOUND('',#3962,.T.);
#2987=FACE_OUTER_BOUND('',#3963,.T.);
#2988=FACE_OUTER_BOUND('',#3964,.T.);
#2989=FACE_OUTER_BOUND('',#3965,.T.);
#2990=FACE_OUTER_BOUND('',#3966,.T.);
#2991=FACE_OUTER_BOUND('',#3967,.T.);
#2992=FACE_OUTER_BOUND('',#3968,.T.);
#2993=FACE_OUTER_BOUND('',#3969,.T.);
#2994=FACE_OUTER_BOUND('',#3970,.T.);
#2995=FACE_OUTER_BOUND('',#3971,.T.);
#2996=FACE_OUTER_BOUND('',#3972,.T.);
#2997=FACE_OUTER_BOUND('',#3973,.T.);
#2998=FACE_OUTER_BOUND('',#3974,.T.);
#2999=FACE_OUTER_BOUND('',#3975,.T.);
#3000=FACE_OUTER_BOUND('',#3976,.T.);
#3001=FACE_OUTER_BOUND('',#3977,.T.);
#3002=FACE_OUTER_BOUND('',#3978,.T.);
#3003=FACE_OUTER_BOUND('',#3979,.T.);
#3004=FACE_OUTER_BOUND('',#3980,.T.);
#3005=FACE_OUTER_BOUND('',#3981,.T.);
#3006=FACE_OUTER_BOUND('',#3982,.T.);
#3007=FACE_OUTER_BOUND('',#3983,.T.);
#3008=FACE_OUTER_BOUND('',#3984,.T.);
#3009=FACE_OUTER_BOUND('',#3985,.T.);
#3010=FACE_OUTER_BOUND('',#3986,.T.);
#3011=FACE_OUTER_BOUND('',#3987,.T.);
#3012=FACE_OUTER_BOUND('',#3988,.T.);
#3742=EDGE_LOOP('',(#11699,#11700,#11701,#11702,#11703));
#3743=EDGE_LOOP('',(#11704,#11705,#11706,#11707,#11708,#11709));
#3744=EDGE_LOOP('',(#11710,#11711,#11712,#11713,#11714,#11715,#11716,#11717,
#11718,#11719,#11720,#11721,#11722,#11723,#11724,#11725,#11726,#11727,#11728,
#11729,#11730,#11731,#11732,#11733,#11734,#11735,#11736,#11737,#11738,#11739,
#11740,#11741,#11742,#11743,#11744,#11745,#11746,#11747,#11748,#11749,#11750,
#11751,#11752,#11753,#11754,#11755,#11756,#11757,#11758,#11759,#11760,#11761,
#11762,#11763,#11764,#11765,#11766,#11767,#11768,#11769,#11770,#11771,#11772,
#11773,#11774,#11775,#11776,#11777,#11778,#11779,#11780,#11781,#11782,#11783,
#11784,#11785,#11786,#11787,#11788,#11789,#11790,#11791,#11792,#11793,#11794,
#11795,#11796,#11797,#11798,#11799,#11800,#11801,#11802,#11803,#11804,#11805,
#11806,#11807,#11808,#11809,#11810,#11811,#11812,#11813,#11814,#11815,#11816,
#11817,#11818,#11819,#11820,#11821,#11822,#11823,#11824,#11825,#11826,#11827,
#11828,#11829));
#3745=EDGE_LOOP('',(#11830));
#3746=EDGE_LOOP('',(#11831,#11832,#11833,#11834,#11835));
#3747=EDGE_LOOP('',(#11836,#11837,#11838,#11839,#11840,#11841,#11842,#11843,
#11844,#11845,#11846,#11847,#11848,#11849,#11850,#11851,#11852,#11853,#11854,
#11855,#11856,#11857,#11858,#11859,#11860,#11861,#11862,#11863,#11864,#11865,
#11866,#11867,#11868,#11869,#11870,#11871,#11872,#11873,#11874,#11875,#11876,
#11877,#11878,#11879,#11880,#11881,#11882,#11883,#11884,#11885,#11886,#11887,
#11888,#11889,#11890,#11891,#11892,#11893,#11894,#11895,#11896,#11897,#11898,
#11899,#11900,#11901,#11902,#11903,#11904,#11905,#11906,#11907,#11908,#11909,
#11910,#11911,#11912,#11913,#11914,#11915,#11916,#11917,#11918,#11919,#11920,
#11921,#11922,#11923,#11924,#11925,#11926,#11927,#11928,#11929,#11930,#11931,
#11932,#11933,#11934,#11935,#11936,#11937,#11938,#11939,#11940,#11941,#11942,
#11943,#11944,#11945,#11946,#11947,#11948,#11949,#11950,#11951,#11952,#11953,
#11954,#11955));
#3748=EDGE_LOOP('',(#11956));
#3749=EDGE_LOOP('',(#11957,#11958,#11959,#11960,#11961,#11962,#11963,#11964));
#3750=EDGE_LOOP('',(#11965,#11966,#11967,#11968));
#3751=EDGE_LOOP('',(#11969,#11970,#11971,#11972,#11973,#11974,#11975,#11976));
#3752=EDGE_LOOP('',(#11977,#11978,#11979,#11980));
#3753=EDGE_LOOP('',(#11981,#11982,#11983,#11984));
#3754=EDGE_LOOP('',(#11985,#11986,#11987,#11988));
#3755=EDGE_LOOP('',(#11989,#11990,#11991,#11992));
#3756=EDGE_LOOP('',(#11993,#11994,#11995,#11996));
#3757=EDGE_LOOP('',(#11997,#11998,#11999,#12000,#12001,#12002,#12003,#12004));
#3758=EDGE_LOOP('',(#12005,#12006,#12007,#12008));
#3759=EDGE_LOOP('',(#12009,#12010,#12011,#12012,#12013,#12014,#12015,#12016));
#3760=EDGE_LOOP('',(#12017,#12018,#12019,#12020));
#3761=EDGE_LOOP('',(#12021,#12022,#12023,#12024));
#3762=EDGE_LOOP('',(#12025,#12026,#12027,#12028));
#3763=EDGE_LOOP('',(#12029,#12030,#12031,#12032));
#3764=EDGE_LOOP('',(#12033,#12034,#12035,#12036));
#3765=EDGE_LOOP('',(#12037,#12038,#12039,#12040,#12041,#12042,#12043,#12044));
#3766=EDGE_LOOP('',(#12045,#12046,#12047,#12048));
#3767=EDGE_LOOP('',(#12049,#12050,#12051,#12052,#12053,#12054,#12055,#12056));
#3768=EDGE_LOOP('',(#12057,#12058,#12059,#12060));
#3769=EDGE_LOOP('',(#12061,#12062,#12063,#12064));
#3770=EDGE_LOOP('',(#12065,#12066,#12067,#12068));
#3771=EDGE_LOOP('',(#12069,#12070,#12071,#12072));
#3772=EDGE_LOOP('',(#12073,#12074,#12075,#12076));
#3773=EDGE_LOOP('',(#12077,#12078,#12079,#12080,#12081,#12082,#12083,#12084));
#3774=EDGE_LOOP('',(#12085,#12086,#12087,#12088));
#3775=EDGE_LOOP('',(#12089,#12090,#12091,#12092,#12093,#12094,#12095,#12096));
#3776=EDGE_LOOP('',(#12097,#12098,#12099,#12100));
#3777=EDGE_LOOP('',(#12101,#12102,#12103,#12104));
#3778=EDGE_LOOP('',(#12105,#12106,#12107,#12108));
#3779=EDGE_LOOP('',(#12109,#12110,#12111,#12112));
#3780=EDGE_LOOP('',(#12113,#12114,#12115,#12116));
#3781=EDGE_LOOP('',(#12117,#12118,#12119,#12120,#12121,#12122,#12123,#12124));
#3782=EDGE_LOOP('',(#12125,#12126,#12127,#12128));
#3783=EDGE_LOOP('',(#12129,#12130,#12131,#12132,#12133,#12134,#12135,#12136));
#3784=EDGE_LOOP('',(#12137,#12138,#12139,#12140));
#3785=EDGE_LOOP('',(#12141,#12142,#12143,#12144));
#3786=EDGE_LOOP('',(#12145,#12146,#12147,#12148));
#3787=EDGE_LOOP('',(#12149,#12150,#12151,#12152));
#3788=EDGE_LOOP('',(#12153,#12154,#12155,#12156));
#3789=EDGE_LOOP('',(#12157,#12158,#12159,#12160,#12161,#12162,#12163,#12164));
#3790=EDGE_LOOP('',(#12165,#12166,#12167,#12168));
#3791=EDGE_LOOP('',(#12169,#12170,#12171,#12172,#12173,#12174,#12175,#12176));
#3792=EDGE_LOOP('',(#12177,#12178,#12179,#12180));
#3793=EDGE_LOOP('',(#12181,#12182,#12183,#12184));
#3794=EDGE_LOOP('',(#12185,#12186,#12187,#12188));
#3795=EDGE_LOOP('',(#12189,#12190,#12191,#12192));
#3796=EDGE_LOOP('',(#12193,#12194,#12195,#12196));
#3797=EDGE_LOOP('',(#12197,#12198,#12199,#12200,#12201,#12202,#12203,#12204));
#3798=EDGE_LOOP('',(#12205,#12206,#12207,#12208));
#3799=EDGE_LOOP('',(#12209,#12210,#12211,#12212,#12213,#12214,#12215,#12216));
#3800=EDGE_LOOP('',(#12217,#12218,#12219,#12220));
#3801=EDGE_LOOP('',(#12221,#12222,#12223,#12224));
#3802=EDGE_LOOP('',(#12225,#12226,#12227,#12228));
#3803=EDGE_LOOP('',(#12229,#12230,#12231,#12232));
#3804=EDGE_LOOP('',(#12233,#12234,#12235,#12236));
#3805=EDGE_LOOP('',(#12237,#12238,#12239,#12240,#12241,#12242,#12243,#12244));
#3806=EDGE_LOOP('',(#12245,#12246,#12247,#12248));
#3807=EDGE_LOOP('',(#12249,#12250,#12251,#12252,#12253,#12254,#12255,#12256));
#3808=EDGE_LOOP('',(#12257,#12258,#12259,#12260));
#3809=EDGE_LOOP('',(#12261,#12262,#12263,#12264));
#3810=EDGE_LOOP('',(#12265,#12266,#12267,#12268));
#3811=EDGE_LOOP('',(#12269,#12270,#12271,#12272));
#3812=EDGE_LOOP('',(#12273,#12274,#12275,#12276));
#3813=EDGE_LOOP('',(#12277,#12278,#12279,#12280,#12281,#12282,#12283,#12284));
#3814=EDGE_LOOP('',(#12285,#12286,#12287,#12288));
#3815=EDGE_LOOP('',(#12289,#12290,#12291,#12292,#12293,#12294,#12295,#12296));
#3816=EDGE_LOOP('',(#12297,#12298,#12299,#12300));
#3817=EDGE_LOOP('',(#12301,#12302,#12303,#12304));
#3818=EDGE_LOOP('',(#12305,#12306,#12307,#12308));
#3819=EDGE_LOOP('',(#12309,#12310,#12311,#12312));
#3820=EDGE_LOOP('',(#12313,#12314,#12315,#12316));
#3821=EDGE_LOOP('',(#12317,#12318,#12319,#12320,#12321,#12322,#12323,#12324));
#3822=EDGE_LOOP('',(#12325,#12326,#12327,#12328));
#3823=EDGE_LOOP('',(#12329,#12330,#12331,#12332,#12333,#12334,#12335,#12336));
#3824=EDGE_LOOP('',(#12337,#12338,#12339,#12340));
#3825=EDGE_LOOP('',(#12341,#12342,#12343,#12344));
#3826=EDGE_LOOP('',(#12345,#12346,#12347,#12348));
#3827=EDGE_LOOP('',(#12349,#12350,#12351,#12352));
#3828=EDGE_LOOP('',(#12353,#12354,#12355,#12356));
#3829=EDGE_LOOP('',(#12357,#12358,#12359,#12360,#12361,#12362,#12363,#12364));
#3830=EDGE_LOOP('',(#12365,#12366,#12367,#12368));
#3831=EDGE_LOOP('',(#12369,#12370,#12371,#12372,#12373,#12374,#12375,#12376));
#3832=EDGE_LOOP('',(#12377,#12378,#12379,#12380));
#3833=EDGE_LOOP('',(#12381,#12382,#12383,#12384));
#3834=EDGE_LOOP('',(#12385,#12386,#12387,#12388));
#3835=EDGE_LOOP('',(#12389,#12390,#12391,#12392));
#3836=EDGE_LOOP('',(#12393,#12394,#12395,#12396));
#3837=EDGE_LOOP('',(#12397,#12398,#12399,#12400,#12401,#12402,#12403,#12404));
#3838=EDGE_LOOP('',(#12405,#12406,#12407,#12408));
#3839=EDGE_LOOP('',(#12409,#12410,#12411,#12412,#12413,#12414,#12415,#12416));
#3840=EDGE_LOOP('',(#12417,#12418,#12419,#12420));
#3841=EDGE_LOOP('',(#12421,#12422,#12423,#12424));
#3842=EDGE_LOOP('',(#12425,#12426,#12427,#12428));
#3843=EDGE_LOOP('',(#12429,#12430,#12431,#12432));
#3844=EDGE_LOOP('',(#12433,#12434,#12435,#12436));
#3845=EDGE_LOOP('',(#12437,#12438,#12439,#12440,#12441,#12442,#12443,#12444));
#3846=EDGE_LOOP('',(#12445,#12446,#12447,#12448));
#3847=EDGE_LOOP('',(#12449,#12450,#12451,#12452,#12453,#12454,#12455,#12456));
#3848=EDGE_LOOP('',(#12457,#12458,#12459,#12460));
#3849=EDGE_LOOP('',(#12461,#12462,#12463,#12464));
#3850=EDGE_LOOP('',(#12465,#12466,#12467,#12468));
#3851=EDGE_LOOP('',(#12469,#12470,#12471,#12472));
#3852=EDGE_LOOP('',(#12473,#12474,#12475,#12476));
#3853=EDGE_LOOP('',(#12477,#12478,#12479,#12480,#12481,#12482,#12483,#12484));
#3854=EDGE_LOOP('',(#12485,#12486,#12487,#12488));
#3855=EDGE_LOOP('',(#12489,#12490,#12491,#12492,#12493,#12494,#12495,#12496));
#3856=EDGE_LOOP('',(#12497,#12498,#12499,#12500));
#3857=EDGE_LOOP('',(#12501,#12502,#12503,#12504));
#3858=EDGE_LOOP('',(#12505,#12506,#12507,#12508));
#3859=EDGE_LOOP('',(#12509,#12510,#12511,#12512));
#3860=EDGE_LOOP('',(#12513,#12514,#12515,#12516));
#3861=EDGE_LOOP('',(#12517,#12518,#12519,#12520,#12521,#12522,#12523,#12524));
#3862=EDGE_LOOP('',(#12525,#12526,#12527,#12528));
#3863=EDGE_LOOP('',(#12529,#12530,#12531,#12532,#12533,#12534,#12535,#12536));
#3864=EDGE_LOOP('',(#12537,#12538,#12539,#12540));
#3865=EDGE_LOOP('',(#12541,#12542,#12543,#12544));
#3866=EDGE_LOOP('',(#12545,#12546,#12547,#12548));
#3867=EDGE_LOOP('',(#12549,#12550,#12551,#12552));
#3868=EDGE_LOOP('',(#12553,#12554,#12555,#12556));
#3869=EDGE_LOOP('',(#12557,#12558,#12559,#12560,#12561,#12562,#12563,#12564));
#3870=EDGE_LOOP('',(#12565,#12566,#12567,#12568));
#3871=EDGE_LOOP('',(#12569,#12570,#12571,#12572,#12573,#12574,#12575,#12576));
#3872=EDGE_LOOP('',(#12577,#12578,#12579,#12580));
#3873=EDGE_LOOP('',(#12581,#12582,#12583,#12584));
#3874=EDGE_LOOP('',(#12585,#12586,#12587,#12588));
#3875=EDGE_LOOP('',(#12589,#12590,#12591,#12592));
#3876=EDGE_LOOP('',(#12593,#12594,#12595,#12596));
#3877=EDGE_LOOP('',(#12597,#12598,#12599,#12600,#12601,#12602,#12603,#12604));
#3878=EDGE_LOOP('',(#12605,#12606,#12607,#12608));
#3879=EDGE_LOOP('',(#12609,#12610,#12611,#12612,#12613,#12614,#12615,#12616));
#3880=EDGE_LOOP('',(#12617,#12618,#12619,#12620));
#3881=EDGE_LOOP('',(#12621,#12622,#12623,#12624));
#3882=EDGE_LOOP('',(#12625,#12626,#12627,#12628));
#3883=EDGE_LOOP('',(#12629,#12630,#12631,#12632));
#3884=EDGE_LOOP('',(#12633,#12634,#12635,#12636));
#3885=EDGE_LOOP('',(#12637,#12638,#12639,#12640,#12641,#12642,#12643,#12644));
#3886=EDGE_LOOP('',(#12645,#12646,#12647,#12648));
#3887=EDGE_LOOP('',(#12649,#12650,#12651,#12652,#12653,#12654,#12655,#12656));
#3888=EDGE_LOOP('',(#12657,#12658,#12659,#12660));
#3889=EDGE_LOOP('',(#12661,#12662,#12663,#12664));
#3890=EDGE_LOOP('',(#12665,#12666,#12667,#12668));
#3891=EDGE_LOOP('',(#12669,#12670,#12671,#12672));
#3892=EDGE_LOOP('',(#12673,#12674,#12675,#12676));
#3893=EDGE_LOOP('',(#12677,#12678,#12679,#12680,#12681,#12682,#12683,#12684));
#3894=EDGE_LOOP('',(#12685,#12686,#12687,#12688));
#3895=EDGE_LOOP('',(#12689,#12690,#12691,#12692,#12693,#12694,#12695,#12696));
#3896=EDGE_LOOP('',(#12697,#12698,#12699,#12700));
#3897=EDGE_LOOP('',(#12701,#12702,#12703,#12704));
#3898=EDGE_LOOP('',(#12705,#12706,#12707,#12708));
#3899=EDGE_LOOP('',(#12709,#12710,#12711,#12712));
#3900=EDGE_LOOP('',(#12713,#12714,#12715,#12716));
#3901=EDGE_LOOP('',(#12717,#12718,#12719,#12720,#12721,#12722,#12723,#12724));
#3902=EDGE_LOOP('',(#12725,#12726,#12727,#12728));
#3903=EDGE_LOOP('',(#12729,#12730,#12731,#12732,#12733,#12734,#12735,#12736));
#3904=EDGE_LOOP('',(#12737,#12738,#12739,#12740));
#3905=EDGE_LOOP('',(#12741,#12742,#12743,#12744));
#3906=EDGE_LOOP('',(#12745,#12746,#12747,#12748));
#3907=EDGE_LOOP('',(#12749,#12750,#12751,#12752));
#3908=EDGE_LOOP('',(#12753,#12754,#12755,#12756));
#3909=EDGE_LOOP('',(#12757,#12758,#12759,#12760,#12761,#12762,#12763,#12764));
#3910=EDGE_LOOP('',(#12765,#12766,#12767,#12768));
#3911=EDGE_LOOP('',(#12769,#12770,#12771,#12772,#12773,#12774,#12775,#12776));
#3912=EDGE_LOOP('',(#12777,#12778,#12779,#12780));
#3913=EDGE_LOOP('',(#12781,#12782,#12783,#12784));
#3914=EDGE_LOOP('',(#12785,#12786,#12787,#12788));
#3915=EDGE_LOOP('',(#12789,#12790,#12791,#12792));
#3916=EDGE_LOOP('',(#12793,#12794,#12795,#12796));
#3917=EDGE_LOOP('',(#12797,#12798,#12799,#12800,#12801,#12802,#12803,#12804));
#3918=EDGE_LOOP('',(#12805,#12806,#12807,#12808));
#3919=EDGE_LOOP('',(#12809,#12810,#12811,#12812,#12813,#12814,#12815,#12816));
#3920=EDGE_LOOP('',(#12817,#12818,#12819,#12820));
#3921=EDGE_LOOP('',(#12821,#12822,#12823,#12824));
#3922=EDGE_LOOP('',(#12825,#12826,#12827,#12828));
#3923=EDGE_LOOP('',(#12829,#12830,#12831,#12832));
#3924=EDGE_LOOP('',(#12833,#12834,#12835,#12836));
#3925=EDGE_LOOP('',(#12837,#12838,#12839,#12840,#12841,#12842,#12843,#12844));
#3926=EDGE_LOOP('',(#12845,#12846,#12847,#12848));
#3927=EDGE_LOOP('',(#12849,#12850,#12851,#12852,#12853,#12854,#12855,#12856));
#3928=EDGE_LOOP('',(#12857,#12858,#12859,#12860));
#3929=EDGE_LOOP('',(#12861,#12862,#12863,#12864));
#3930=EDGE_LOOP('',(#12865,#12866,#12867,#12868));
#3931=EDGE_LOOP('',(#12869,#12870,#12871,#12872));
#3932=EDGE_LOOP('',(#12873,#12874,#12875,#12876));
#3933=EDGE_LOOP('',(#12877,#12878,#12879,#12880,#12881,#12882,#12883,#12884));
#3934=EDGE_LOOP('',(#12885,#12886,#12887,#12888));
#3935=EDGE_LOOP('',(#12889,#12890,#12891,#12892,#12893,#12894,#12895,#12896));
#3936=EDGE_LOOP('',(#12897,#12898,#12899,#12900));
#3937=EDGE_LOOP('',(#12901,#12902,#12903,#12904));
#3938=EDGE_LOOP('',(#12905,#12906,#12907,#12908));
#3939=EDGE_LOOP('',(#12909,#12910,#12911,#12912));
#3940=EDGE_LOOP('',(#12913,#12914,#12915,#12916));
#3941=EDGE_LOOP('',(#12917,#12918,#12919,#12920,#12921,#12922,#12923,#12924));
#3942=EDGE_LOOP('',(#12925,#12926,#12927,#12928));
#3943=EDGE_LOOP('',(#12929,#12930,#12931,#12932,#12933,#12934,#12935,#12936));
#3944=EDGE_LOOP('',(#12937,#12938,#12939,#12940));
#3945=EDGE_LOOP('',(#12941,#12942,#12943,#12944));
#3946=EDGE_LOOP('',(#12945,#12946,#12947,#12948));
#3947=EDGE_LOOP('',(#12949,#12950,#12951,#12952));
#3948=EDGE_LOOP('',(#12953,#12954,#12955,#12956));
#3949=EDGE_LOOP('',(#12957,#12958,#12959,#12960,#12961,#12962,#12963,#12964));
#3950=EDGE_LOOP('',(#12965,#12966,#12967,#12968));
#3951=EDGE_LOOP('',(#12969,#12970,#12971,#12972,#12973,#12974,#12975,#12976));
#3952=EDGE_LOOP('',(#12977,#12978,#12979,#12980));
#3953=EDGE_LOOP('',(#12981,#12982,#12983,#12984));
#3954=EDGE_LOOP('',(#12985,#12986,#12987,#12988));
#3955=EDGE_LOOP('',(#12989,#12990,#12991,#12992));
#3956=EDGE_LOOP('',(#12993,#12994,#12995,#12996));
#3957=EDGE_LOOP('',(#12997,#12998,#12999,#13000,#13001,#13002,#13003,#13004));
#3958=EDGE_LOOP('',(#13005,#13006,#13007,#13008));
#3959=EDGE_LOOP('',(#13009,#13010,#13011,#13012,#13013,#13014,#13015,#13016));
#3960=EDGE_LOOP('',(#13017,#13018,#13019,#13020));
#3961=EDGE_LOOP('',(#13021,#13022,#13023,#13024));
#3962=EDGE_LOOP('',(#13025,#13026,#13027,#13028));
#3963=EDGE_LOOP('',(#13029,#13030,#13031,#13032));
#3964=EDGE_LOOP('',(#13033,#13034,#13035,#13036));
#3965=EDGE_LOOP('',(#13037,#13038,#13039,#13040,#13041,#13042,#13043,#13044));
#3966=EDGE_LOOP('',(#13045,#13046,#13047,#13048));
#3967=EDGE_LOOP('',(#13049,#13050,#13051,#13052,#13053,#13054,#13055,#13056));
#3968=EDGE_LOOP('',(#13057,#13058,#13059,#13060));
#3969=EDGE_LOOP('',(#13061,#13062,#13063,#13064));
#3970=EDGE_LOOP('',(#13065,#13066,#13067,#13068));
#3971=EDGE_LOOP('',(#13069,#13070,#13071,#13072));
#3972=EDGE_LOOP('',(#13073,#13074,#13075,#13076));
#3973=EDGE_LOOP('',(#13077,#13078,#13079,#13080));
#3974=EDGE_LOOP('',(#13081,#13082,#13083,#13084,#13085,#13086,#13087,#13088));
#3975=EDGE_LOOP('',(#13089,#13090,#13091,#13092));
#3976=EDGE_LOOP('',(#13093,#13094,#13095,#13096,#13097,#13098,#13099,#13100));
#3977=EDGE_LOOP('',(#13101,#13102,#13103,#13104));
#3978=EDGE_LOOP('',(#13105,#13106,#13107,#13108));
#3979=EDGE_LOOP('',(#13109,#13110,#13111,#13112));
#3980=EDGE_LOOP('',(#13113,#13114,#13115,#13116));
#3981=EDGE_LOOP('',(#13117,#13118,#13119,#13120));
#3982=EDGE_LOOP('',(#13121,#13122,#13123,#13124));
#3983=EDGE_LOOP('',(#13125,#13126,#13127,#13128,#13129,#13130,#13131,#13132));
#3984=EDGE_LOOP('',(#13133,#13134,#13135,#13136));
#3985=EDGE_LOOP('',(#13137,#13138,#13139,#13140,#13141,#13142,#13143,#13144));
#3986=EDGE_LOOP('',(#13145,#13146,#13147,#13148));
#3987=EDGE_LOOP('',(#13149,#13150,#13151,#13152));
#3988=EDGE_LOOP('',(#13153,#13154,#13155,#13156));
#4886=LINE('',#26816,#5746);
#4887=LINE('',#26821,#5747);
#4888=LINE('',#26870,#5748);
#4889=LINE('',#26913,#5749);
#4890=LINE('',#26958,#5750);
#4891=LINE('',#27004,#5751);
#4892=LINE('',#27047,#5752);
#4893=LINE('',#27090,#5753);
#4894=LINE('',#27132,#5754);
#4895=LINE('',#27173,#5755);
#4896=LINE('',#27215,#5756);
#4897=LINE('',#27258,#5757);
#4898=LINE('',#27296,#5758);
#4899=LINE('',#27333,#5759);
#4900=LINE('',#27374,#5760);
#4901=LINE('',#27410,#5761);
#4902=LINE('',#27450,#5762);
#4903=LINE('',#27487,#5763);
#4904=LINE('',#27526,#5764);
#4905=LINE('',#27587,#5765);
#4906=LINE('',#27625,#5766);
#4907=LINE('',#27661,#5767);
#4908=LINE('',#27703,#5768);
#4909=LINE('',#27737,#5769);
#4910=LINE('',#27780,#5770);
#4911=LINE('',#27827,#5771);
#4912=LINE('',#27870,#5772);
#4913=LINE('',#27913,#5773);
#4914=LINE('',#27958,#5774);
#4915=LINE('',#27996,#5775);
#4916=LINE('',#28042,#5776);
#4917=LINE('',#28111,#5777);
#4918=LINE('',#28114,#5778);
#4919=LINE('',#28128,#5779);
#4920=LINE('',#28170,#5780);
#4921=LINE('',#28252,#5781);
#4922=LINE('',#28279,#5782);
#4923=LINE('',#28358,#5783);
#4924=LINE('',#28389,#5784);
#4925=LINE('',#28420,#5785);
#4926=LINE('',#28495,#5786);
#4927=LINE('',#28538,#5787);
#4928=LINE('',#28581,#5788);
#4929=LINE('',#28612,#5789);
#4930=LINE('',#28639,#5790);
#4931=LINE('',#28668,#5791);
#4932=LINE('',#28697,#5792);
#4933=LINE('',#28726,#5793);
#4934=LINE('',#28785,#5794);
#4935=LINE('',#28819,#5795);
#4936=LINE('',#28845,#5796);
#4937=LINE('',#28918,#5797);
#4938=LINE('',#28979,#5798);
#4939=LINE('',#29008,#5799);
#4940=LINE('',#29040,#5800);
#4941=LINE('',#29071,#5801);
#4942=LINE('',#29100,#5802);
#4943=LINE('',#29172,#5803);
#4944=LINE('',#29245,#5804);
#4945=LINE('',#29277,#5805);
#4946=LINE('',#29312,#5806);
#4947=LINE('',#29391,#5807);
#4948=LINE('',#29424,#5808);
#5746=VECTOR('',#19191,3.325);
#5747=VECTOR('',#19198,3.3);
#5748=VECTOR('',#19207,1.);
#5749=VECTOR('',#19210,1.);
#5750=VECTOR('',#19213,1.);
#5751=VECTOR('',#19216,1.);
#5752=VECTOR('',#19219,1.);
#5753=VECTOR('',#19222,1.);
#5754=VECTOR('',#19225,1.);
#5755=VECTOR('',#19228,1.);
#5756=VECTOR('',#19231,1.);
#5757=VECTOR('',#19234,1.);
#5758=VECTOR('',#19237,1.);
#5759=VECTOR('',#19240,1.);
#5760=VECTOR('',#19243,1.);
#5761=VECTOR('',#19246,1.);
#5762=VECTOR('',#19249,1.);
#5763=VECTOR('',#19252,1.);
#5764=VECTOR('',#19255,1.);
#5765=VECTOR('',#19258,1.);
#5766=VECTOR('',#19261,1.);
#5767=VECTOR('',#19264,1.);
#5768=VECTOR('',#19267,1.);
#5769=VECTOR('',#19270,1.);
#5770=VECTOR('',#19273,1.);
#5771=VECTOR('',#19276,1.);
#5772=VECTOR('',#19279,1.);
#5773=VECTOR('',#19282,1.);
#5774=VECTOR('',#19285,1.);
#5775=VECTOR('',#19288,1.);
#5776=VECTOR('',#19291,1.);
#5777=VECTOR('',#19294,1.);
#5778=VECTOR('',#19297,3.325);
#5779=VECTOR('',#19302,1.);
#5780=VECTOR('',#19305,1.);
#5781=VECTOR('',#19308,1.);
#5782=VECTOR('',#19311,1.);
#5783=VECTOR('',#19314,1.);
#5784=VECTOR('',#19317,1.);
#5785=VECTOR('',#19320,1.);
#5786=VECTOR('',#19323,1.);
#5787=VECTOR('',#19326,1.);
#5788=VECTOR('',#19329,1.);
#5789=VECTOR('',#19332,1.);
#5790=VECTOR('',#19335,1.);
#5791=VECTOR('',#19338,1.);
#5792=VECTOR('',#19341,1.);
#5793=VECTOR('',#19344,1.);
#5794=VECTOR('',#19347,1.);
#5795=VECTOR('',#19350,1.);
#5796=VECTOR('',#19353,1.);
#5797=VECTOR('',#19356,1.);
#5798=VECTOR('',#19359,1.);
#5799=VECTOR('',#19362,1.);
#5800=VECTOR('',#19365,1.);
#5801=VECTOR('',#19368,1.);
#5802=VECTOR('',#19371,1.);
#5803=VECTOR('',#19374,1.);
#5804=VECTOR('',#19377,1.);
#5805=VECTOR('',#19380,1.);
#5806=VECTOR('',#19383,1.);
#5807=VECTOR('',#19386,1.);
#5808=VECTOR('',#19389,1.);
#6596=VERTEX_POINT('',#26812);
#6597=VERTEX_POINT('',#26813);
#6598=VERTEX_POINT('',#26815);
#6599=VERTEX_POINT('',#26820);
#6600=VERTEX_POINT('',#26822);
#6601=VERTEX_POINT('',#26826);
#6602=VERTEX_POINT('',#26827);
#6603=VERTEX_POINT('',#26847);
#6604=VERTEX_POINT('',#26849);
#6605=VERTEX_POINT('',#26869);
#6606=VERTEX_POINT('',#26871);
#6607=VERTEX_POINT('',#26890);
#6608=VERTEX_POINT('',#26892);
#6609=VERTEX_POINT('',#26912);
#6610=VERTEX_POINT('',#26914);
#6611=VERTEX_POINT('',#26936);
#6612=VERTEX_POINT('',#26938);
#6613=VERTEX_POINT('',#26957);
#6614=VERTEX_POINT('',#26959);
#6615=VERTEX_POINT('',#26979);
#6616=VERTEX_POINT('',#26981);
#6617=VERTEX_POINT('',#27003);
#6618=VERTEX_POINT('',#27005);
#6619=VERTEX_POINT('',#27025);
#6620=VERTEX_POINT('',#27027);
#6621=VERTEX_POINT('',#27046);
#6622=VERTEX_POINT('',#27048);
#6623=VERTEX_POINT('',#27068);
#6624=VERTEX_POINT('',#27070);
#6625=VERTEX_POINT('',#27089);
#6626=VERTEX_POINT('',#27091);
#6627=VERTEX_POINT('',#27111);
#6628=VERTEX_POINT('',#27113);
#6629=VERTEX_POINT('',#27131);
#6630=VERTEX_POINT('',#27133);
#6631=VERTEX_POINT('',#27154);
#6632=VERTEX_POINT('',#27156);
#6633=VERTEX_POINT('',#27172);
#6634=VERTEX_POINT('',#27174);
#6635=VERTEX_POINT('',#27194);
#6636=VERTEX_POINT('',#27196);
#6637=VERTEX_POINT('',#27214);
#6638=VERTEX_POINT('',#27216);
#6639=VERTEX_POINT('',#27236);
#6640=VERTEX_POINT('',#27238);
#6641=VERTEX_POINT('',#27257);
#6642=VERTEX_POINT('',#27259);
#6643=VERTEX_POINT('',#27275);
#6644=VERTEX_POINT('',#27277);
#6645=VERTEX_POINT('',#27295);
#6646=VERTEX_POINT('',#27297);
#6647=VERTEX_POINT('',#27314);
#6648=VERTEX_POINT('',#27316);
#6649=VERTEX_POINT('',#27332);
#6650=VERTEX_POINT('',#27334);
#6651=VERTEX_POINT('',#27355);
#6652=VERTEX_POINT('',#27357);
#6653=VERTEX_POINT('',#27373);
#6654=VERTEX_POINT('',#27375);
#6655=VERTEX_POINT('',#27392);
#6656=VERTEX_POINT('',#27394);
#6657=VERTEX_POINT('',#27409);
#6658=VERTEX_POINT('',#27411);
#6659=VERTEX_POINT('',#27428);
#6660=VERTEX_POINT('',#27430);
#6661=VERTEX_POINT('',#27449);
#6662=VERTEX_POINT('',#27451);
#6663=VERTEX_POINT('',#27467);
#6664=VERTEX_POINT('',#27469);
#6665=VERTEX_POINT('',#27486);
#6666=VERTEX_POINT('',#27488);
#6667=VERTEX_POINT('',#27505);
#6668=VERTEX_POINT('',#27507);
#6669=VERTEX_POINT('',#27525);
#6670=VERTEX_POINT('',#27527);
#6671=VERTEX_POINT('',#27543);
#6672=VERTEX_POINT('',#27545);
#6673=VERTEX_POINT('',#27586);
#6674=VERTEX_POINT('',#27588);
#6675=VERTEX_POINT('',#27604);
#6676=VERTEX_POINT('',#27606);
#6677=VERTEX_POINT('',#27624);
#6678=VERTEX_POINT('',#27626);
#6679=VERTEX_POINT('',#27642);
#6680=VERTEX_POINT('',#27644);
#6681=VERTEX_POINT('',#27660);
#6682=VERTEX_POINT('',#27662);
#6683=VERTEX_POINT('',#27682);
#6684=VERTEX_POINT('',#27684);
#6685=VERTEX_POINT('',#27702);
#6686=VERTEX_POINT('',#27704);
#6687=VERTEX_POINT('',#27713);
#6688=VERTEX_POINT('',#27715);
#6689=VERTEX_POINT('',#27736);
#6690=VERTEX_POINT('',#27738);
#6691=VERTEX_POINT('',#27757);
#6692=VERTEX_POINT('',#27759);
#6693=VERTEX_POINT('',#27779);
#6694=VERTEX_POINT('',#27781);
#6695=VERTEX_POINT('',#27800);
#6696=VERTEX_POINT('',#27802);
#6697=VERTEX_POINT('',#27826);
#6698=VERTEX_POINT('',#27828);
#6699=VERTEX_POINT('',#27847);
#6700=VERTEX_POINT('',#27849);
#6701=VERTEX_POINT('',#27869);
#6702=VERTEX_POINT('',#27871);
#6703=VERTEX_POINT('',#27890);
#6704=VERTEX_POINT('',#27892);
#6705=VERTEX_POINT('',#27912);
#6706=VERTEX_POINT('',#27914);
#6707=VERTEX_POINT('',#27936);
#6708=VERTEX_POINT('',#27938);
#6709=VERTEX_POINT('',#27957);
#6710=VERTEX_POINT('',#27959);
#6711=VERTEX_POINT('',#27977);
#6712=VERTEX_POINT('',#27979);
#6713=VERTEX_POINT('',#27995);
#6714=VERTEX_POINT('',#27997);
#6715=VERTEX_POINT('',#28020);
#6716=VERTEX_POINT('',#28022);
#6717=VERTEX_POINT('',#28041);
#6718=VERTEX_POINT('',#28043);
#6719=VERTEX_POINT('',#28050);
#6720=VERTEX_POINT('',#28052);
#6721=VERTEX_POINT('',#28113);
#6722=VERTEX_POINT('',#28117);
#6723=VERTEX_POINT('',#28118);
#6724=VERTEX_POINT('',#28127);
#6725=VERTEX_POINT('',#28129);
#6726=VERTEX_POINT('',#28148);
#6727=VERTEX_POINT('',#28150);
#6728=VERTEX_POINT('',#28169);
#6729=VERTEX_POINT('',#28171);
#6730=VERTEX_POINT('',#28190);
#6731=VERTEX_POINT('',#28192);
#6732=VERTEX_POINT('',#28251);
#6733=VERTEX_POINT('',#28253);
#6734=VERTEX_POINT('',#28269);
#6735=VERTEX_POINT('',#28271);
#6736=VERTEX_POINT('',#28278);
#6737=VERTEX_POINT('',#28280);
#6738=VERTEX_POINT('',#28299);
#6739=VERTEX_POINT('',#28301);
#6740=VERTEX_POINT('',#28357);
#6741=VERTEX_POINT('',#28359);
#6742=VERTEX_POINT('',#28379);
#6743=VERTEX_POINT('',#28381);
#6744=VERTEX_POINT('',#28388);
#6745=VERTEX_POINT('',#28390);
#6746=VERTEX_POINT('',#28410);
#6747=VERTEX_POINT('',#28412);
#6748=VERTEX_POINT('',#28419);
#6749=VERTEX_POINT('',#28421);
#6750=VERTEX_POINT('',#28445);
#6751=VERTEX_POINT('',#28447);
#6752=VERTEX_POINT('',#28494);
#6753=VERTEX_POINT('',#28496);
#6754=VERTEX_POINT('',#28516);
#6755=VERTEX_POINT('',#28518);
#6756=VERTEX_POINT('',#28537);
#6757=VERTEX_POINT('',#28539);
#6758=VERTEX_POINT('',#28560);
#6759=VERTEX_POINT('',#28562);
#6760=VERTEX_POINT('',#28580);
#6761=VERTEX_POINT('',#28582);
#6762=VERTEX_POINT('',#28600);
#6763=VERTEX_POINT('',#28602);
#6764=VERTEX_POINT('',#28611);
#6765=VERTEX_POINT('',#28613);
#6766=VERTEX_POINT('',#28629);
#6767=VERTEX_POINT('',#28631);
#6768=VERTEX_POINT('',#28638);
#6769=VERTEX_POINT('',#28640);
#6770=VERTEX_POINT('',#28658);
#6771=VERTEX_POINT('',#28660);
#6772=VERTEX_POINT('',#28667);
#6773=VERTEX_POINT('',#28669);
#6774=VERTEX_POINT('',#28687);
#6775=VERTEX_POINT('',#28689);
#6776=VERTEX_POINT('',#28696);
#6777=VERTEX_POINT('',#28698);
#6778=VERTEX_POINT('',#28716);
#6779=VERTEX_POINT('',#28718);
#6780=VERTEX_POINT('',#28725);
#6781=VERTEX_POINT('',#28727);
#6782=VERTEX_POINT('',#28744);
#6783=VERTEX_POINT('',#28746);
#6784=VERTEX_POINT('',#28784);
#6785=VERTEX_POINT('',#28786);
#6786=VERTEX_POINT('',#28805);
#6787=VERTEX_POINT('',#28807);
#6788=VERTEX_POINT('',#28818);
#6789=VERTEX_POINT('',#28820);
#6790=VERTEX_POINT('',#28835);
#6791=VERTEX_POINT('',#28837);
#6792=VERTEX_POINT('',#28844);
#6793=VERTEX_POINT('',#28846);
#6794=VERTEX_POINT('',#28862);
#6795=VERTEX_POINT('',#28864);
#6796=VERTEX_POINT('',#28917);
#6797=VERTEX_POINT('',#28919);
#6798=VERTEX_POINT('',#28935);
#6799=VERTEX_POINT('',#28937);
#6800=VERTEX_POINT('',#28978);
#6801=VERTEX_POINT('',#28980);
#6802=VERTEX_POINT('',#28998);
#6803=VERTEX_POINT('',#29000);
#6804=VERTEX_POINT('',#29007);
#6805=VERTEX_POINT('',#29009);
#6806=VERTEX_POINT('',#29028);
#6807=VERTEX_POINT('',#29030);
#6808=VERTEX_POINT('',#29039);
#6809=VERTEX_POINT('',#29041);
#6810=VERTEX_POINT('',#29059);
#6811=VERTEX_POINT('',#29061);
#6812=VERTEX_POINT('',#29070);
#6813=VERTEX_POINT('',#29072);
#6814=VERTEX_POINT('',#29088);
#6815=VERTEX_POINT('',#29090);
#6816=VERTEX_POINT('',#29099);
#6817=VERTEX_POINT('',#29101);
#6818=VERTEX_POINT('',#29119);
#6819=VERTEX_POINT('',#29121);
#6820=VERTEX_POINT('',#29171);
#6821=VERTEX_POINT('',#29173);
#6822=VERTEX_POINT('',#29192);
#6823=VERTEX_POINT('',#29194);
#6824=VERTEX_POINT('',#29244);
#6825=VERTEX_POINT('',#29246);
#6826=VERTEX_POINT('',#29265);
#6827=VERTEX_POINT('',#29267);
#6828=VERTEX_POINT('',#29276);
#6829=VERTEX_POINT('',#29278);
#6830=VERTEX_POINT('',#29300);
#6831=VERTEX_POINT('',#29302);
#6832=VERTEX_POINT('',#29311);
#6833=VERTEX_POINT('',#29313);
#6834=VERTEX_POINT('',#29332);
#6835=VERTEX_POINT('',#29334);
#6836=VERTEX_POINT('',#29390);
#6837=VERTEX_POINT('',#29392);
#6838=VERTEX_POINT('',#29412);
#6839=VERTEX_POINT('',#29414);
#6840=VERTEX_POINT('',#29423);
#6841=VERTEX_POINT('',#29425);
#6842=VERTEX_POINT('',#29936);
#6843=VERTEX_POINT('',#29947);
#6844=VERTEX_POINT('',#29954);
#6845=VERTEX_POINT('',#29969);
#6846=VERTEX_POINT('',#30570);
#6847=VERTEX_POINT('',#30577);
#6848=VERTEX_POINT('',#30588);
#6849=VERTEX_POINT('',#30603);
#6850=VERTEX_POINT('',#30617);
#6851=VERTEX_POINT('',#30626);
#6852=VERTEX_POINT('',#30637);
#6853=VERTEX_POINT('',#30654);
#6854=VERTEX_POINT('',#31187);
#6855=VERTEX_POINT('',#31198);
#6856=VERTEX_POINT('',#31209);
#6857=VERTEX_POINT('',#31224);
#6858=VERTEX_POINT('',#31881);
#6859=VERTEX_POINT('',#31888);
#6860=VERTEX_POINT('',#31899);
#6861=VERTEX_POINT('',#31914);
#6862=VERTEX_POINT('',#32472);
#6863=VERTEX_POINT('',#32483);
#6864=VERTEX_POINT('',#32494);
#6865=VERTEX_POINT('',#32509);
#6866=VERTEX_POINT('',#33250);
#6867=VERTEX_POINT('',#33257);
#6868=VERTEX_POINT('',#33264);
#6869=VERTEX_POINT('',#33279);
#6870=VERTEX_POINT('',#33879);
#6871=VERTEX_POINT('',#33888);
#6872=VERTEX_POINT('',#33895);
#6873=VERTEX_POINT('',#33910);
#6874=VERTEX_POINT('',#34441);
#6875=VERTEX_POINT('',#34450);
#6876=VERTEX_POINT('',#34457);
#6877=VERTEX_POINT('',#34472);
#6878=VERTEX_POINT('',#35168);
#6879=VERTEX_POINT('',#35175);
#6880=VERTEX_POINT('',#35182);
#6881=VERTEX_POINT('',#35197);
#6882=VERTEX_POINT('',#35730);
#6883=VERTEX_POINT('',#35739);
#6884=VERTEX_POINT('',#35746);
#6885=VERTEX_POINT('',#35761);
#6886=VERTEX_POINT('',#36275);
#6887=VERTEX_POINT('',#36288);
#6888=VERTEX_POINT('',#36295);
#6889=VERTEX_POINT('',#36310);
#6890=VERTEX_POINT('',#37009);
#6891=VERTEX_POINT('',#37018);
#6892=VERTEX_POINT('',#37029);
#6893=VERTEX_POINT('',#37044);
#6894=VERTEX_POINT('',#37544);
#6895=VERTEX_POINT('',#37553);
#6896=VERTEX_POINT('',#37560);
#6897=VERTEX_POINT('',#37575);
#6898=VERTEX_POINT('',#38120);
#6899=VERTEX_POINT('',#38127);
#6900=VERTEX_POINT('',#38134);
#6901=VERTEX_POINT('',#38149);
#6902=VERTEX_POINT('',#38591);
#6903=VERTEX_POINT('',#38598);
#6904=VERTEX_POINT('',#38605);
#6905=VERTEX_POINT('',#38620);
#6906=VERTEX_POINT('',#39193);
#6907=VERTEX_POINT('',#39202);
#6908=VERTEX_POINT('',#39209);
#6909=VERTEX_POINT('',#39224);
#6910=VERTEX_POINT('',#39766);
#6911=VERTEX_POINT('',#39775);
#6912=VERTEX_POINT('',#39782);
#6913=VERTEX_POINT('',#39797);
#6914=VERTEX_POINT('',#40442);
#6915=VERTEX_POINT('',#40449);
#6916=VERTEX_POINT('',#40460);
#6917=VERTEX_POINT('',#40475);
#6918=VERTEX_POINT('',#40917);
#6919=VERTEX_POINT('',#40924);
#6920=VERTEX_POINT('',#40931);
#6921=VERTEX_POINT('',#40946);
#6922=VERTEX_POINT('',#41547);
#6923=VERTEX_POINT('',#41554);
#6924=VERTEX_POINT('',#41561);
#6925=VERTEX_POINT('',#41576);
#6926=VERTEX_POINT('',#42032);
#6927=VERTEX_POINT('',#42039);
#6928=VERTEX_POINT('',#42046);
#6929=VERTEX_POINT('',#42061);
#6930=VERTEX_POINT('',#42508);
#6931=VERTEX_POINT('',#42515);
#6932=VERTEX_POINT('',#42522);
#6933=VERTEX_POINT('',#42537);
#6934=VERTEX_POINT('',#42993);
#6935=VERTEX_POINT('',#43004);
#6936=VERTEX_POINT('',#43011);
#6937=VERTEX_POINT('',#43026);
#6938=VERTEX_POINT('',#43543);
#6939=VERTEX_POINT('',#43550);
#6940=VERTEX_POINT('',#43557);
#6941=VERTEX_POINT('',#43572);
#6942=VERTEX_POINT('',#44042);
#6943=VERTEX_POINT('',#44051);
#6944=VERTEX_POINT('',#44058);
#6945=VERTEX_POINT('',#44073);
#6946=VERTEX_POINT('',#44648);
#6947=VERTEX_POINT('',#44655);
#6948=VERTEX_POINT('',#44662);
#6949=VERTEX_POINT('',#44677);
#6950=VERTEX_POINT('',#45105);
#6951=VERTEX_POINT('',#45112);
#6952=VERTEX_POINT('',#45119);
#6953=VERTEX_POINT('',#45134);
#6954=VERTEX_POINT('',#45583);
#6955=VERTEX_POINT('',#45592);
#6956=VERTEX_POINT('',#45603);
#6957=VERTEX_POINT('',#45618);
#6958=VERTEX_POINT('',#46020);
#6959=VERTEX_POINT('',#46029);
#6960=VERTEX_POINT('',#46036);
#6961=VERTEX_POINT('',#46051);
#6962=VERTEX_POINT('',#46512);
#6963=VERTEX_POINT('',#46519);
#6964=VERTEX_POINT('',#46530);
#6965=VERTEX_POINT('',#46545);
#6966=VERTEX_POINT('',#47015);
#6967=VERTEX_POINT('',#47022);
#6968=VERTEX_POINT('',#47029);
#6969=VERTEX_POINT('',#47044);
#6970=VERTEX_POINT('',#47535);
#6971=VERTEX_POINT('',#47542);
#6972=VERTEX_POINT('',#47553);
#6973=VERTEX_POINT('',#47568);
#6974=VERTEX_POINT('',#47900);
#6975=VERTEX_POINT('',#47907);
#6976=VERTEX_POINT('',#47914);
#6977=VERTEX_POINT('',#47929);
#6978=VERTEX_POINT('',#48474);
#6979=VERTEX_POINT('',#48483);
#6980=VERTEX_POINT('',#48494);
#6981=VERTEX_POINT('',#48509);
#6982=VERTEX_POINT('',#48967);
#6983=VERTEX_POINT('',#48978);
#6984=VERTEX_POINT('',#48985);
#6985=VERTEX_POINT('',#49000);
#6986=VERTEX_POINT('',#49531);
#6987=VERTEX_POINT('',#49540);
#6988=VERTEX_POINT('',#49547);
#6989=VERTEX_POINT('',#49562);
#6990=VERTEX_POINT('',#50020);
#6991=VERTEX_POINT('',#50031);
#6992=VERTEX_POINT('',#50038);
#6993=VERTEX_POINT('',#50053);
#6994=VERTEX_POINT('',#50502);
#6995=VERTEX_POINT('',#50509);
#6996=VERTEX_POINT('',#50516);
#6997=VERTEX_POINT('',#50531);
#6998=VERTEX_POINT('',#50959);
#6999=VERTEX_POINT('',#50968);
#7000=VERTEX_POINT('',#50975);
#7001=VERTEX_POINT('',#50990);
#7002=VERTEX_POINT('',#51451);
#7003=VERTEX_POINT('',#51458);
#7004=VERTEX_POINT('',#51465);
#7005=VERTEX_POINT('',#51480);
#7006=VERTEX_POINT('',#51978);
#7007=VERTEX_POINT('',#51987);
#7008=VERTEX_POINT('',#51994);
#7009=VERTEX_POINT('',#52009);
#7010=VERTEX_POINT('',#52668);
#7011=VERTEX_POINT('',#52677);
#7012=VERTEX_POINT('',#52684);
#7013=VERTEX_POINT('',#52699);
#7014=VERTEX_POINT('',#53141);
#7015=VERTEX_POINT('',#53148);
#7016=VERTEX_POINT('',#53155);
#7017=VERTEX_POINT('',#53170);
#7018=VERTEX_POINT('',#53715);
#7019=VERTEX_POINT('',#53722);
#7020=VERTEX_POINT('',#53729);
#7021=VERTEX_POINT('',#53744);
#7022=VERTEX_POINT('',#54214);
#7023=VERTEX_POINT('',#54221);
#7024=VERTEX_POINT('',#54228);
#7025=VERTEX_POINT('',#54243);
#7026=VERTEX_POINT('',#54760);
#7027=VERTEX_POINT('',#54771);
#7028=VERTEX_POINT('',#54778);
#7029=VERTEX_POINT('',#54793);
#7030=VERTEX_POINT('',#55293);
#7031=VERTEX_POINT('',#55300);
#7032=VERTEX_POINT('',#55307);
#7033=VERTEX_POINT('',#55322);
#7034=VERTEX_POINT('',#55839);
#7035=VERTEX_POINT('',#55850);
#7036=VERTEX_POINT('',#55857);
#7037=VERTEX_POINT('',#55872);
#7038=VERTEX_POINT('',#56512);
#7039=VERTEX_POINT('',#56523);
#7040=VERTEX_POINT('',#56530);
#7041=VERTEX_POINT('',#56545);
#7042=VERTEX_POINT('',#57190);
#7043=VERTEX_POINT('',#57199);
#7044=VERTEX_POINT('',#57206);
#7045=VERTEX_POINT('',#57221);
#7046=VERTEX_POINT('',#57761);
#7047=VERTEX_POINT('',#57772);
#7048=VERTEX_POINT('',#57783);
#7049=VERTEX_POINT('',#57798);
#7050=VERTEX_POINT('',#58245);
#7051=VERTEX_POINT('',#58254);
#7052=VERTEX_POINT('',#58261);
#7053=VERTEX_POINT('',#58276);
#7054=VERTEX_POINT('',#58818);
#7055=VERTEX_POINT('',#58829);
#7056=VERTEX_POINT('',#58840);
#7057=VERTEX_POINT('',#58855);
#7058=VERTEX_POINT('',#59596);
#7059=VERTEX_POINT('',#59605);
#7060=VERTEX_POINT('',#59616);
#7061=VERTEX_POINT('',#59631);
#7062=VERTEX_POINT('',#60227);
#7063=VERTEX_POINT('',#60236);
#7064=VERTEX_POINT('',#60243);
#7065=VERTEX_POINT('',#60258);
#7066=VERTEX_POINT('',#60705);
#7067=VERTEX_POINT('',#60714);
#7068=VERTEX_POINT('',#60721);
#7069=VERTEX_POINT('',#60736);
#7070=VERTEX_POINT('',#60754);
#7071=VERTEX_POINT('',#61291);
#7072=VERTEX_POINT('',#61300);
#7073=VERTEX_POINT('',#61307);
#7074=VERTEX_POINT('',#62042);
#7075=VERTEX_POINT('',#62049);
#7076=VERTEX_POINT('',#62056);
#7077=VERTEX_POINT('',#62071);
#7078=VERTEX_POINT('',#62085);
#7079=VERTEX_POINT('',#62096);
#7080=VERTEX_POINT('',#62543);
#7081=VERTEX_POINT('',#62550);
#8471=EDGE_CURVE('',#6596,#6597,#2012,.T.);
#8472=EDGE_CURVE('',#6597,#6598,#4886,.T.);
#8473=EDGE_CURVE('',#6598,#6598,#2013,.T.);
#8474=EDGE_CURVE('',#6597,#6596,#2014,.T.);
#8475=EDGE_CURVE('',#6596,#6599,#4887,.T.);
#8476=EDGE_CURVE('',#6600,#6599,#2015,.T.);
#8477=EDGE_CURVE('',#6599,#6600,#2016,.T.);
#8478=EDGE_CURVE('',#6601,#6602,#418,.T.);
#8479=EDGE_CURVE('',#6603,#6602,#2017,.T.);
#8480=EDGE_CURVE('',#6603,#6604,#419,.T.);
#8481=EDGE_CURVE('',#6604,#6605,#4888,.T.);
#8482=EDGE_CURVE('',#6605,#6606,#420,.T.);
#8483=EDGE_CURVE('',#6607,#6606,#2018,.T.);
#8484=EDGE_CURVE('',#6607,#6608,#421,.T.);
#8485=EDGE_CURVE('',#6608,#6609,#4889,.T.);
#8486=EDGE_CURVE('',#6609,#6610,#422,.T.);
#8487=EDGE_CURVE('',#6611,#6610,#2019,.T.);
#8488=EDGE_CURVE('',#6611,#6612,#423,.T.);
#8489=EDGE_CURVE('',#6612,#6613,#4890,.T.);
#8490=EDGE_CURVE('',#6613,#6614,#424,.T.);
#8491=EDGE_CURVE('',#6615,#6614,#2020,.T.);
#8492=EDGE_CURVE('',#6615,#6616,#425,.T.);
#8493=EDGE_CURVE('',#6616,#6617,#4891,.T.);
#8494=EDGE_CURVE('',#6617,#6618,#426,.T.);
#8495=EDGE_CURVE('',#6619,#6618,#2021,.T.);
#8496=EDGE_CURVE('',#6619,#6620,#427,.T.);
#8497=EDGE_CURVE('',#6620,#6621,#4892,.T.);
#8498=EDGE_CURVE('',#6621,#6622,#428,.T.);
#8499=EDGE_CURVE('',#6623,#6622,#2022,.T.);
#8500=EDGE_CURVE('',#6623,#6624,#429,.T.);
#8501=EDGE_CURVE('',#6624,#6625,#4893,.T.);
#8502=EDGE_CURVE('',#6625,#6626,#430,.T.);
#8503=EDGE_CURVE('',#6627,#6626,#2023,.T.);
#8504=EDGE_CURVE('',#6627,#6628,#431,.T.);
#8505=EDGE_CURVE('',#6628,#6629,#4894,.T.);
#8506=EDGE_CURVE('',#6629,#6630,#432,.T.);
#8507=EDGE_CURVE('',#6631,#6630,#2024,.T.);
#8508=EDGE_CURVE('',#6631,#6632,#433,.T.);
#8509=EDGE_CURVE('',#6632,#6633,#4895,.T.);
#8510=EDGE_CURVE('',#6633,#6634,#434,.T.);
#8511=EDGE_CURVE('',#6635,#6634,#2025,.T.);
#8512=EDGE_CURVE('',#6635,#6636,#435,.T.);
#8513=EDGE_CURVE('',#6636,#6637,#4896,.T.);
#8514=EDGE_CURVE('',#6637,#6638,#436,.T.);
#8515=EDGE_CURVE('',#6639,#6638,#2026,.T.);
#8516=EDGE_CURVE('',#6639,#6640,#437,.T.);
#8517=EDGE_CURVE('',#6640,#6641,#4897,.T.);
#8518=EDGE_CURVE('',#6641,#6642,#438,.T.);
#8519=EDGE_CURVE('',#6643,#6642,#2027,.T.);
#8520=EDGE_CURVE('',#6643,#6644,#439,.T.);
#8521=EDGE_CURVE('',#6644,#6645,#4898,.T.);
#8522=EDGE_CURVE('',#6645,#6646,#440,.T.);
#8523=EDGE_CURVE('',#6647,#6646,#2028,.T.);
#8524=EDGE_CURVE('',#6647,#6648,#441,.T.);
#8525=EDGE_CURVE('',#6648,#6649,#4899,.T.);
#8526=EDGE_CURVE('',#6649,#6650,#442,.T.);
#8527=EDGE_CURVE('',#6651,#6650,#2029,.T.);
#8528=EDGE_CURVE('',#6651,#6652,#443,.T.);
#8529=EDGE_CURVE('',#6652,#6653,#4900,.T.);
#8530=EDGE_CURVE('',#6653,#6654,#444,.T.);
#8531=EDGE_CURVE('',#6655,#6654,#2030,.T.);
#8532=EDGE_CURVE('',#6655,#6656,#445,.T.);
#8533=EDGE_CURVE('',#6656,#6657,#4901,.T.);
#8534=EDGE_CURVE('',#6657,#6658,#446,.T.);
#8535=EDGE_CURVE('',#6659,#6658,#2031,.T.);
#8536=EDGE_CURVE('',#6659,#6660,#447,.T.);
#8537=EDGE_CURVE('',#6660,#6661,#4902,.T.);
#8538=EDGE_CURVE('',#6661,#6662,#448,.T.);
#8539=EDGE_CURVE('',#6663,#6662,#2032,.T.);
#8540=EDGE_CURVE('',#6663,#6664,#449,.T.);
#8541=EDGE_CURVE('',#6664,#6665,#4903,.T.);
#8542=EDGE_CURVE('',#6665,#6666,#450,.T.);
#8543=EDGE_CURVE('',#6667,#6666,#2033,.T.);
#8544=EDGE_CURVE('',#6667,#6668,#451,.T.);
#8545=EDGE_CURVE('',#6668,#6669,#4904,.T.);
#8546=EDGE_CURVE('',#6669,#6670,#452,.T.);
#8547=EDGE_CURVE('',#6671,#6670,#2034,.T.);
#8548=EDGE_CURVE('',#6671,#6672,#453,.T.);
#8549=EDGE_CURVE('',#6672,#6673,#4905,.T.);
#8550=EDGE_CURVE('',#6673,#6674,#454,.T.);
#8551=EDGE_CURVE('',#6675,#6674,#2035,.T.);
#8552=EDGE_CURVE('',#6675,#6676,#455,.T.);
#8553=EDGE_CURVE('',#6676,#6677,#4906,.T.);
#8554=EDGE_CURVE('',#6677,#6678,#456,.T.);
#8555=EDGE_CURVE('',#6679,#6678,#2036,.T.);
#8556=EDGE_CURVE('',#6679,#6680,#457,.T.);
#8557=EDGE_CURVE('',#6680,#6681,#4907,.T.);
#8558=EDGE_CURVE('',#6681,#6682,#458,.T.);
#8559=EDGE_CURVE('',#6683,#6682,#2037,.T.);
#8560=EDGE_CURVE('',#6683,#6684,#459,.T.);
#8561=EDGE_CURVE('',#6684,#6685,#4908,.T.);
#8562=EDGE_CURVE('',#6685,#6686,#460,.T.);
#8563=EDGE_CURVE('',#6687,#6686,#2038,.T.);
#8564=EDGE_CURVE('',#6687,#6688,#461,.T.);
#8565=EDGE_CURVE('',#6688,#6689,#4909,.T.);
#8566=EDGE_CURVE('',#6689,#6690,#462,.T.);
#8567=EDGE_CURVE('',#6691,#6690,#2039,.T.);
#8568=EDGE_CURVE('',#6691,#6692,#463,.T.);
#8569=EDGE_CURVE('',#6692,#6693,#4910,.T.);
#8570=EDGE_CURVE('',#6693,#6694,#464,.T.);
#8571=EDGE_CURVE('',#6695,#6694,#2040,.T.);
#8572=EDGE_CURVE('',#6695,#6696,#465,.T.);
#8573=EDGE_CURVE('',#6696,#6697,#4911,.T.);
#8574=EDGE_CURVE('',#6697,#6698,#466,.T.);
#8575=EDGE_CURVE('',#6699,#6698,#2041,.T.);
#8576=EDGE_CURVE('',#6699,#6700,#467,.T.);
#8577=EDGE_CURVE('',#6700,#6701,#4912,.T.);
#8578=EDGE_CURVE('',#6701,#6702,#468,.T.);
#8579=EDGE_CURVE('',#6703,#6702,#2042,.T.);
#8580=EDGE_CURVE('',#6703,#6704,#469,.T.);
#8581=EDGE_CURVE('',#6704,#6705,#4913,.T.);
#8582=EDGE_CURVE('',#6705,#6706,#470,.T.);
#8583=EDGE_CURVE('',#6707,#6706,#2043,.T.);
#8584=EDGE_CURVE('',#6707,#6708,#471,.T.);
#8585=EDGE_CURVE('',#6708,#6709,#4914,.T.);
#8586=EDGE_CURVE('',#6709,#6710,#472,.T.);
#8587=EDGE_CURVE('',#6711,#6710,#2044,.T.);
#8588=EDGE_CURVE('',#6711,#6712,#473,.T.);
#8589=EDGE_CURVE('',#6712,#6713,#4915,.T.);
#8590=EDGE_CURVE('',#6713,#6714,#474,.T.);
#8591=EDGE_CURVE('',#6715,#6714,#2045,.T.);
#8592=EDGE_CURVE('',#6715,#6716,#475,.T.);
#8593=EDGE_CURVE('',#6716,#6717,#4916,.T.);
#8594=EDGE_CURVE('',#6717,#6718,#476,.T.);
#8595=EDGE_CURVE('',#6719,#6718,#2046,.T.);
#8596=EDGE_CURVE('',#6719,#6720,#477,.T.);
#8597=EDGE_CURVE('',#6720,#6601,#4917,.T.);
#8598=EDGE_CURVE('',#6600,#6721,#4918,.T.);
#8599=EDGE_CURVE('',#6721,#6721,#2047,.T.);
#8600=EDGE_CURVE('',#6722,#6723,#478,.T.);
#8601=EDGE_CURVE('',#6723,#6724,#4919,.T.);
#8602=EDGE_CURVE('',#6724,#6725,#479,.T.);
#8603=EDGE_CURVE('',#6725,#6726,#2048,.T.);
#8604=EDGE_CURVE('',#6726,#6727,#480,.T.);
#8605=EDGE_CURVE('',#6727,#6728,#4920,.T.);
#8606=EDGE_CURVE('',#6728,#6729,#481,.T.);
#8607=EDGE_CURVE('',#6729,#6730,#2049,.T.);
#8608=EDGE_CURVE('',#6730,#6731,#482,.T.);
#8609=EDGE_CURVE('',#6731,#6732,#4921,.T.);
#8610=EDGE_CURVE('',#6732,#6733,#483,.T.);
#8611=EDGE_CURVE('',#6733,#6734,#2050,.T.);
#8612=EDGE_CURVE('',#6734,#6735,#484,.T.);
#8613=EDGE_CURVE('',#6735,#6736,#4922,.T.);
#8614=EDGE_CURVE('',#6736,#6737,#485,.T.);
#8615=EDGE_CURVE('',#6737,#6738,#2051,.T.);
#8616=EDGE_CURVE('',#6738,#6739,#486,.T.);
#8617=EDGE_CURVE('',#6739,#6740,#4923,.T.);
#8618=EDGE_CURVE('',#6740,#6741,#487,.T.);
#8619=EDGE_CURVE('',#6741,#6742,#2052,.T.);
#8620=EDGE_CURVE('',#6742,#6743,#488,.T.);
#8621=EDGE_CURVE('',#6743,#6744,#4924,.T.);
#8622=EDGE_CURVE('',#6744,#6745,#489,.T.);
#8623=EDGE_CURVE('',#6745,#6746,#2053,.T.);
#8624=EDGE_CURVE('',#6746,#6747,#490,.T.);
#8625=EDGE_CURVE('',#6747,#6748,#4925,.T.);
#8626=EDGE_CURVE('',#6748,#6749,#491,.T.);
#8627=EDGE_CURVE('',#6749,#6750,#2054,.T.);
#8628=EDGE_CURVE('',#6750,#6751,#492,.T.);
#8629=EDGE_CURVE('',#6751,#6752,#4926,.T.);
#8630=EDGE_CURVE('',#6752,#6753,#493,.T.);
#8631=EDGE_CURVE('',#6753,#6754,#2055,.T.);
#8632=EDGE_CURVE('',#6754,#6755,#494,.T.);
#8633=EDGE_CURVE('',#6755,#6756,#4927,.T.);
#8634=EDGE_CURVE('',#6756,#6757,#495,.T.);
#8635=EDGE_CURVE('',#6757,#6758,#2056,.T.);
#8636=EDGE_CURVE('',#6758,#6759,#496,.T.);
#8637=EDGE_CURVE('',#6759,#6760,#4928,.T.);
#8638=EDGE_CURVE('',#6760,#6761,#497,.T.);
#8639=EDGE_CURVE('',#6761,#6762,#2057,.T.);
#8640=EDGE_CURVE('',#6762,#6763,#498,.T.);
#8641=EDGE_CURVE('',#6763,#6764,#4929,.T.);
#8642=EDGE_CURVE('',#6764,#6765,#499,.T.);
#8643=EDGE_CURVE('',#6765,#6766,#2058,.T.);
#8644=EDGE_CURVE('',#6766,#6767,#500,.T.);
#8645=EDGE_CURVE('',#6767,#6768,#4930,.T.);
#8646=EDGE_CURVE('',#6768,#6769,#501,.T.);
#8647=EDGE_CURVE('',#6769,#6770,#2059,.T.);
#8648=EDGE_CURVE('',#6770,#6771,#502,.T.);
#8649=EDGE_CURVE('',#6771,#6772,#4931,.T.);
#8650=EDGE_CURVE('',#6772,#6773,#503,.T.);
#8651=EDGE_CURVE('',#6773,#6774,#2060,.T.);
#8652=EDGE_CURVE('',#6774,#6775,#504,.T.);
#8653=EDGE_CURVE('',#6775,#6776,#4932,.T.);
#8654=EDGE_CURVE('',#6776,#6777,#505,.T.);
#8655=EDGE_CURVE('',#6777,#6778,#2061,.T.);
#8656=EDGE_CURVE('',#6778,#6779,#506,.T.);
#8657=EDGE_CURVE('',#6779,#6780,#4933,.T.);
#8658=EDGE_CURVE('',#6780,#6781,#507,.T.);
#8659=EDGE_CURVE('',#6781,#6782,#2062,.T.);
#8660=EDGE_CURVE('',#6782,#6783,#508,.T.);
#8661=EDGE_CURVE('',#6783,#6784,#4934,.T.);
#8662=EDGE_CURVE('',#6784,#6785,#509,.T.);
#8663=EDGE_CURVE('',#6785,#6786,#2063,.T.);
#8664=EDGE_CURVE('',#6786,#6787,#510,.T.);
#8665=EDGE_CURVE('',#6787,#6788,#4935,.T.);
#8666=EDGE_CURVE('',#6788,#6789,#511,.T.);
#8667=EDGE_CURVE('',#6789,#6790,#2064,.T.);
#8668=EDGE_CURVE('',#6790,#6791,#512,.T.);
#8669=EDGE_CURVE('',#6791,#6792,#4936,.T.);
#8670=EDGE_CURVE('',#6792,#6793,#513,.T.);
#8671=EDGE_CURVE('',#6793,#6794,#2065,.T.);
#8672=EDGE_CURVE('',#6794,#6795,#514,.T.);
#8673=EDGE_CURVE('',#6795,#6796,#4937,.T.);
#8674=EDGE_CURVE('',#6796,#6797,#515,.T.);
#8675=EDGE_CURVE('',#6797,#6798,#2066,.T.);
#8676=EDGE_CURVE('',#6798,#6799,#516,.T.);
#8677=EDGE_CURVE('',#6799,#6800,#4938,.T.);
#8678=EDGE_CURVE('',#6800,#6801,#517,.T.);
#8679=EDGE_CURVE('',#6801,#6802,#2067,.T.);
#8680=EDGE_CURVE('',#6802,#6803,#518,.T.);
#8681=EDGE_CURVE('',#6803,#6804,#4939,.T.);
#8682=EDGE_CURVE('',#6804,#6805,#519,.T.);
#8683=EDGE_CURVE('',#6805,#6806,#2068,.T.);
#8684=EDGE_CURVE('',#6806,#6807,#520,.T.);
#8685=EDGE_CURVE('',#6807,#6808,#4940,.T.);
#8686=EDGE_CURVE('',#6808,#6809,#521,.T.);
#8687=EDGE_CURVE('',#6809,#6810,#2069,.T.);
#8688=EDGE_CURVE('',#6810,#6811,#522,.T.);
#8689=EDGE_CURVE('',#6811,#6812,#4941,.T.);
#8690=EDGE_CURVE('',#6812,#6813,#523,.T.);
#8691=EDGE_CURVE('',#6813,#6814,#2070,.T.);
#8692=EDGE_CURVE('',#6814,#6815,#524,.T.);
#8693=EDGE_CURVE('',#6815,#6816,#4942,.T.);
#8694=EDGE_CURVE('',#6816,#6817,#525,.T.);
#8695=EDGE_CURVE('',#6817,#6818,#2071,.T.);
#8696=EDGE_CURVE('',#6818,#6819,#526,.T.);
#8697=EDGE_CURVE('',#6819,#6820,#4943,.T.);
#8698=EDGE_CURVE('',#6820,#6821,#527,.T.);
#8699=EDGE_CURVE('',#6821,#6822,#2072,.T.);
#8700=EDGE_CURVE('',#6822,#6823,#528,.T.);
#8701=EDGE_CURVE('',#6823,#6824,#4944,.T.);
#8702=EDGE_CURVE('',#6824,#6825,#529,.T.);
#8703=EDGE_CURVE('',#6825,#6826,#2073,.T.);
#8704=EDGE_CURVE('',#6826,#6827,#530,.T.);
#8705=EDGE_CURVE('',#6827,#6828,#4945,.T.);
#8706=EDGE_CURVE('',#6828,#6829,#531,.T.);
#8707=EDGE_CURVE('',#6829,#6830,#2074,.T.);
#8708=EDGE_CURVE('',#6830,#6831,#532,.T.);
#8709=EDGE_CURVE('',#6831,#6832,#4946,.T.);
#8710=EDGE_CURVE('',#6832,#6833,#533,.T.);
#8711=EDGE_CURVE('',#6833,#6834,#2075,.T.);
#8712=EDGE_CURVE('',#6834,#6835,#534,.T.);
#8713=EDGE_CURVE('',#6835,#6836,#4947,.T.);
#8714=EDGE_CURVE('',#6836,#6837,#535,.T.);
#8715=EDGE_CURVE('',#6837,#6838,#2076,.T.);
#8716=EDGE_CURVE('',#6838,#6839,#536,.T.);
#8717=EDGE_CURVE('',#6839,#6840,#4948,.T.);
#8718=EDGE_CURVE('',#6840,#6841,#537,.T.);
#8719=EDGE_CURVE('',#6841,#6722,#2077,.T.);
#8720=EDGE_CURVE('',#6720,#6724,#538,.T.);
#8721=EDGE_CURVE('',#6842,#6719,#539,.T.);
#8722=EDGE_CURVE('',#6843,#6842,#540,.T.);
#8723=EDGE_CURVE('',#6844,#6843,#541,.T.);
#8724=EDGE_CURVE('',#6845,#6844,#542,.T.);
#8725=EDGE_CURVE('',#6725,#6845,#543,.T.);
#8726=EDGE_CURVE('',#6601,#6723,#544,.T.);
#8727=EDGE_CURVE('',#6846,#6722,#545,.T.);
#8728=EDGE_CURVE('',#6847,#6846,#546,.T.);
#8729=EDGE_CURVE('',#6848,#6847,#547,.T.);
#8730=EDGE_CURVE('',#6849,#6848,#548,.T.);
#8731=EDGE_CURVE('',#6602,#6849,#549,.T.);
#8732=EDGE_CURVE('',#6845,#6850,#2078,.T.);
#8733=EDGE_CURVE('',#6850,#6726,#550,.T.);
#8734=EDGE_CURVE('',#6844,#6851,#2079,.T.);
#8735=EDGE_CURVE('',#6851,#6850,#551,.T.);
#8736=EDGE_CURVE('',#6843,#6852,#2080,.T.);
#8737=EDGE_CURVE('',#6852,#6851,#552,.T.);
#8738=EDGE_CURVE('',#6842,#6853,#2081,.T.);
#8739=EDGE_CURVE('',#6853,#6852,#553,.T.);
#8740=EDGE_CURVE('',#6718,#6853,#554,.T.);
#8741=EDGE_CURVE('',#6604,#6840,#555,.T.);
#8742=EDGE_CURVE('',#6854,#6603,#556,.T.);
#8743=EDGE_CURVE('',#6855,#6854,#557,.T.);
#8744=EDGE_CURVE('',#6856,#6855,#558,.T.);
#8745=EDGE_CURVE('',#6857,#6856,#559,.T.);
#8746=EDGE_CURVE('',#6841,#6857,#560,.T.);
#8747=EDGE_CURVE('',#6605,#6839,#561,.T.);
#8748=EDGE_CURVE('',#6858,#6838,#562,.T.);
#8749=EDGE_CURVE('',#6859,#6858,#563,.T.);
#8750=EDGE_CURVE('',#6860,#6859,#564,.T.);
#8751=EDGE_CURVE('',#6861,#6860,#565,.T.);
#8752=EDGE_CURVE('',#6606,#6861,#566,.T.);
#8753=EDGE_CURVE('',#6857,#6846,#2082,.T.);
#8754=EDGE_CURVE('',#6856,#6847,#2083,.T.);
#8755=EDGE_CURVE('',#6855,#6848,#2084,.T.);
#8756=EDGE_CURVE('',#6854,#6849,#2085,.T.);
#8757=EDGE_CURVE('',#6608,#6836,#567,.T.);
#8758=EDGE_CURVE('',#6862,#6607,#568,.T.);
#8759=EDGE_CURVE('',#6863,#6862,#569,.T.);
#8760=EDGE_CURVE('',#6864,#6863,#570,.T.);
#8761=EDGE_CURVE('',#6865,#6864,#571,.T.);
#8762=EDGE_CURVE('',#6837,#6865,#572,.T.);
#8763=EDGE_CURVE('',#6609,#6835,#573,.T.);
#8764=EDGE_CURVE('',#6866,#6834,#574,.T.);
#8765=EDGE_CURVE('',#6867,#6866,#575,.T.);
#8766=EDGE_CURVE('',#6868,#6867,#576,.T.);
#8767=EDGE_CURVE('',#6869,#6868,#577,.T.);
#8768=EDGE_CURVE('',#6610,#6869,#578,.T.);
#8769=EDGE_CURVE('',#6865,#6858,#2086,.T.);
#8770=EDGE_CURVE('',#6864,#6859,#2087,.T.);
#8771=EDGE_CURVE('',#6863,#6860,#2088,.T.);
#8772=EDGE_CURVE('',#6862,#6861,#2089,.T.);
#8773=EDGE_CURVE('',#6612,#6832,#579,.T.);
#8774=EDGE_CURVE('',#6870,#6611,#580,.T.);
#8775=EDGE_CURVE('',#6871,#6870,#581,.T.);
#8776=EDGE_CURVE('',#6872,#6871,#582,.T.);
#8777=EDGE_CURVE('',#6873,#6872,#583,.T.);
#8778=EDGE_CURVE('',#6833,#6873,#584,.T.);
#8779=EDGE_CURVE('',#6613,#6831,#585,.T.);
#8780=EDGE_CURVE('',#6874,#6830,#586,.T.);
#8781=EDGE_CURVE('',#6875,#6874,#587,.T.);
#8782=EDGE_CURVE('',#6876,#6875,#588,.T.);
#8783=EDGE_CURVE('',#6877,#6876,#589,.T.);
#8784=EDGE_CURVE('',#6614,#6877,#590,.T.);
#8785=EDGE_CURVE('',#6873,#6866,#2090,.T.);
#8786=EDGE_CURVE('',#6872,#6867,#2091,.T.);
#8787=EDGE_CURVE('',#6871,#6868,#2092,.T.);
#8788=EDGE_CURVE('',#6870,#6869,#2093,.T.);
#8789=EDGE_CURVE('',#6616,#6828,#591,.T.);
#8790=EDGE_CURVE('',#6878,#6615,#592,.T.);
#8791=EDGE_CURVE('',#6879,#6878,#593,.T.);
#8792=EDGE_CURVE('',#6880,#6879,#594,.T.);
#8793=EDGE_CURVE('',#6881,#6880,#595,.T.);
#8794=EDGE_CURVE('',#6829,#6881,#596,.T.);
#8795=EDGE_CURVE('',#6617,#6827,#597,.T.);
#8796=EDGE_CURVE('',#6882,#6826,#598,.T.);
#8797=EDGE_CURVE('',#6883,#6882,#599,.T.);
#8798=EDGE_CURVE('',#6884,#6883,#600,.T.);
#8799=EDGE_CURVE('',#6885,#6884,#601,.T.);
#8800=EDGE_CURVE('',#6618,#6885,#602,.T.);
#8801=EDGE_CURVE('',#6881,#6874,#2094,.T.);
#8802=EDGE_CURVE('',#6880,#6875,#2095,.T.);
#8803=EDGE_CURVE('',#6879,#6876,#2096,.T.);
#8804=EDGE_CURVE('',#6878,#6877,#2097,.T.);
#8805=EDGE_CURVE('',#6620,#6824,#603,.T.);
#8806=EDGE_CURVE('',#6886,#6619,#604,.T.);
#8807=EDGE_CURVE('',#6887,#6886,#605,.T.);
#8808=EDGE_CURVE('',#6888,#6887,#606,.T.);
#8809=EDGE_CURVE('',#6889,#6888,#607,.T.);
#8810=EDGE_CURVE('',#6825,#6889,#608,.T.);
#8811=EDGE_CURVE('',#6621,#6823,#609,.T.);
#8812=EDGE_CURVE('',#6890,#6822,#610,.T.);
#8813=EDGE_CURVE('',#6891,#6890,#611,.T.);
#8814=EDGE_CURVE('',#6892,#6891,#612,.T.);
#8815=EDGE_CURVE('',#6893,#6892,#613,.T.);
#8816=EDGE_CURVE('',#6622,#6893,#614,.T.);
#8817=EDGE_CURVE('',#6889,#6882,#2098,.T.);
#8818=EDGE_CURVE('',#6888,#6883,#2099,.T.);
#8819=EDGE_CURVE('',#6887,#6884,#2100,.T.);
#8820=EDGE_CURVE('',#6886,#6885,#2101,.T.);
#8821=EDGE_CURVE('',#6624,#6820,#615,.T.);
#8822=EDGE_CURVE('',#6894,#6623,#616,.T.);
#8823=EDGE_CURVE('',#6895,#6894,#617,.T.);
#8824=EDGE_CURVE('',#6896,#6895,#618,.T.);
#8825=EDGE_CURVE('',#6897,#6896,#619,.T.);
#8826=EDGE_CURVE('',#6821,#6897,#620,.T.);
#8827=EDGE_CURVE('',#6625,#6819,#621,.T.);
#8828=EDGE_CURVE('',#6898,#6818,#622,.T.);
#8829=EDGE_CURVE('',#6899,#6898,#623,.T.);
#8830=EDGE_CURVE('',#6900,#6899,#624,.T.);
#8831=EDGE_CURVE('',#6901,#6900,#625,.T.);
#8832=EDGE_CURVE('',#6626,#6901,#626,.T.);
#8833=EDGE_CURVE('',#6897,#6890,#2102,.T.);
#8834=EDGE_CURVE('',#6896,#6891,#2103,.T.);
#8835=EDGE_CURVE('',#6895,#6892,#2104,.T.);
#8836=EDGE_CURVE('',#6894,#6893,#2105,.T.);
#8837=EDGE_CURVE('',#6628,#6816,#627,.T.);
#8838=EDGE_CURVE('',#6902,#6627,#628,.T.);
#8839=EDGE_CURVE('',#6903,#6902,#629,.T.);
#8840=EDGE_CURVE('',#6904,#6903,#630,.T.);
#8841=EDGE_CURVE('',#6905,#6904,#631,.T.);
#8842=EDGE_CURVE('',#6817,#6905,#632,.T.);
#8843=EDGE_CURVE('',#6629,#6815,#633,.T.);
#8844=EDGE_CURVE('',#6906,#6814,#634,.T.);
#8845=EDGE_CURVE('',#6907,#6906,#635,.T.);
#8846=EDGE_CURVE('',#6908,#6907,#636,.T.);
#8847=EDGE_CURVE('',#6909,#6908,#637,.T.);
#8848=EDGE_CURVE('',#6630,#6909,#638,.T.);
#8849=EDGE_CURVE('',#6905,#6898,#2106,.T.);
#8850=EDGE_CURVE('',#6904,#6899,#2107,.T.);
#8851=EDGE_CURVE('',#6903,#6900,#2108,.T.);
#8852=EDGE_CURVE('',#6902,#6901,#2109,.T.);
#8853=EDGE_CURVE('',#6632,#6812,#639,.T.);
#8854=EDGE_CURVE('',#6910,#6631,#640,.T.);
#8855=EDGE_CURVE('',#6911,#6910,#641,.T.);
#8856=EDGE_CURVE('',#6912,#6911,#642,.T.);
#8857=EDGE_CURVE('',#6913,#6912,#643,.T.);
#8858=EDGE_CURVE('',#6813,#6913,#644,.T.);
#8859=EDGE_CURVE('',#6633,#6811,#645,.T.);
#8860=EDGE_CURVE('',#6914,#6810,#646,.T.);
#8861=EDGE_CURVE('',#6915,#6914,#647,.T.);
#8862=EDGE_CURVE('',#6916,#6915,#648,.T.);
#8863=EDGE_CURVE('',#6917,#6916,#649,.T.);
#8864=EDGE_CURVE('',#6634,#6917,#650,.T.);
#8865=EDGE_CURVE('',#6913,#6906,#2110,.T.);
#8866=EDGE_CURVE('',#6912,#6907,#2111,.T.);
#8867=EDGE_CURVE('',#6911,#6908,#2112,.T.);
#8868=EDGE_CURVE('',#6910,#6909,#2113,.T.);
#8869=EDGE_CURVE('',#6636,#6808,#651,.T.);
#8870=EDGE_CURVE('',#6918,#6635,#652,.T.);
#8871=EDGE_CURVE('',#6919,#6918,#653,.T.);
#8872=EDGE_CURVE('',#6920,#6919,#654,.T.);
#8873=EDGE_CURVE('',#6921,#6920,#655,.T.);
#8874=EDGE_CURVE('',#6809,#6921,#656,.T.);
#8875=EDGE_CURVE('',#6637,#6807,#657,.T.);
#8876=EDGE_CURVE('',#6922,#6806,#658,.T.);
#8877=EDGE_CURVE('',#6923,#6922,#659,.T.);
#8878=EDGE_CURVE('',#6924,#6923,#660,.T.);
#8879=EDGE_CURVE('',#6925,#6924,#661,.T.);
#8880=EDGE_CURVE('',#6638,#6925,#662,.T.);
#8881=EDGE_CURVE('',#6921,#6914,#2114,.T.);
#8882=EDGE_CURVE('',#6920,#6915,#2115,.T.);
#8883=EDGE_CURVE('',#6919,#6916,#2116,.T.);
#8884=EDGE_CURVE('',#6918,#6917,#2117,.T.);
#8885=EDGE_CURVE('',#6640,#6804,#663,.T.);
#8886=EDGE_CURVE('',#6926,#6639,#664,.T.);
#8887=EDGE_CURVE('',#6927,#6926,#665,.T.);
#8888=EDGE_CURVE('',#6928,#6927,#666,.T.);
#8889=EDGE_CURVE('',#6929,#6928,#667,.T.);
#8890=EDGE_CURVE('',#6805,#6929,#668,.T.);
#8891=EDGE_CURVE('',#6641,#6803,#669,.T.);
#8892=EDGE_CURVE('',#6930,#6802,#670,.T.);
#8893=EDGE_CURVE('',#6931,#6930,#671,.T.);
#8894=EDGE_CURVE('',#6932,#6931,#672,.T.);
#8895=EDGE_CURVE('',#6933,#6932,#673,.T.);
#8896=EDGE_CURVE('',#6642,#6933,#674,.T.);
#8897=EDGE_CURVE('',#6929,#6922,#2118,.T.);
#8898=EDGE_CURVE('',#6928,#6923,#2119,.T.);
#8899=EDGE_CURVE('',#6927,#6924,#2120,.T.);
#8900=EDGE_CURVE('',#6926,#6925,#2121,.T.);
#8901=EDGE_CURVE('',#6644,#6800,#675,.T.);
#8902=EDGE_CURVE('',#6934,#6643,#676,.T.);
#8903=EDGE_CURVE('',#6935,#6934,#677,.T.);
#8904=EDGE_CURVE('',#6936,#6935,#678,.T.);
#8905=EDGE_CURVE('',#6937,#6936,#679,.T.);
#8906=EDGE_CURVE('',#6801,#6937,#680,.T.);
#8907=EDGE_CURVE('',#6645,#6799,#681,.T.);
#8908=EDGE_CURVE('',#6938,#6798,#682,.T.);
#8909=EDGE_CURVE('',#6939,#6938,#683,.T.);
#8910=EDGE_CURVE('',#6940,#6939,#684,.T.);
#8911=EDGE_CURVE('',#6941,#6940,#685,.T.);
#8912=EDGE_CURVE('',#6646,#6941,#686,.T.);
#8913=EDGE_CURVE('',#6937,#6930,#2122,.T.);
#8914=EDGE_CURVE('',#6936,#6931,#2123,.T.);
#8915=EDGE_CURVE('',#6935,#6932,#2124,.T.);
#8916=EDGE_CURVE('',#6934,#6933,#2125,.T.);
#8917=EDGE_CURVE('',#6648,#6796,#687,.T.);
#8918=EDGE_CURVE('',#6942,#6647,#688,.T.);
#8919=EDGE_CURVE('',#6943,#6942,#689,.T.);
#8920=EDGE_CURVE('',#6944,#6943,#690,.T.);
#8921=EDGE_CURVE('',#6945,#6944,#691,.T.);
#8922=EDGE_CURVE('',#6797,#6945,#692,.T.);
#8923=EDGE_CURVE('',#6649,#6795,#693,.T.);
#8924=EDGE_CURVE('',#6946,#6794,#694,.T.);
#8925=EDGE_CURVE('',#6947,#6946,#695,.T.);
#8926=EDGE_CURVE('',#6948,#6947,#696,.T.);
#8927=EDGE_CURVE('',#6949,#6948,#697,.T.);
#8928=EDGE_CURVE('',#6650,#6949,#698,.T.);
#8929=EDGE_CURVE('',#6945,#6938,#2126,.T.);
#8930=EDGE_CURVE('',#6944,#6939,#2127,.T.);
#8931=EDGE_CURVE('',#6943,#6940,#2128,.T.);
#8932=EDGE_CURVE('',#6942,#6941,#2129,.T.);
#8933=EDGE_CURVE('',#6652,#6792,#699,.T.);
#8934=EDGE_CURVE('',#6950,#6651,#700,.T.);
#8935=EDGE_CURVE('',#6951,#6950,#701,.T.);
#8936=EDGE_CURVE('',#6952,#6951,#702,.T.);
#8937=EDGE_CURVE('',#6953,#6952,#703,.T.);
#8938=EDGE_CURVE('',#6793,#6953,#704,.T.);
#8939=EDGE_CURVE('',#6653,#6791,#705,.T.);
#8940=EDGE_CURVE('',#6954,#6790,#706,.T.);
#8941=EDGE_CURVE('',#6955,#6954,#707,.T.);
#8942=EDGE_CURVE('',#6956,#6955,#708,.T.);
#8943=EDGE_CURVE('',#6957,#6956,#709,.T.);
#8944=EDGE_CURVE('',#6654,#6957,#710,.T.);
#8945=EDGE_CURVE('',#6953,#6946,#2130,.T.);
#8946=EDGE_CURVE('',#6952,#6947,#2131,.T.);
#8947=EDGE_CURVE('',#6951,#6948,#2132,.T.);
#8948=EDGE_CURVE('',#6950,#6949,#2133,.T.);
#8949=EDGE_CURVE('',#6656,#6788,#711,.T.);
#8950=EDGE_CURVE('',#6958,#6655,#712,.T.);
#8951=EDGE_CURVE('',#6959,#6958,#713,.T.);
#8952=EDGE_CURVE('',#6960,#6959,#714,.T.);
#8953=EDGE_CURVE('',#6961,#6960,#715,.T.);
#8954=EDGE_CURVE('',#6789,#6961,#716,.T.);
#8955=EDGE_CURVE('',#6657,#6787,#717,.T.);
#8956=EDGE_CURVE('',#6962,#6786,#718,.T.);
#8957=EDGE_CURVE('',#6963,#6962,#719,.T.);
#8958=EDGE_CURVE('',#6964,#6963,#720,.T.);
#8959=EDGE_CURVE('',#6965,#6964,#721,.T.);
#8960=EDGE_CURVE('',#6658,#6965,#722,.T.);
#8961=EDGE_CURVE('',#6961,#6954,#2134,.T.);
#8962=EDGE_CURVE('',#6960,#6955,#2135,.T.);
#8963=EDGE_CURVE('',#6959,#6956,#2136,.T.);
#8964=EDGE_CURVE('',#6958,#6957,#2137,.T.);
#8965=EDGE_CURVE('',#6660,#6784,#723,.T.);
#8966=EDGE_CURVE('',#6966,#6659,#724,.T.);
#8967=EDGE_CURVE('',#6967,#6966,#725,.T.);
#8968=EDGE_CURVE('',#6968,#6967,#726,.T.);
#8969=EDGE_CURVE('',#6969,#6968,#727,.T.);
#8970=EDGE_CURVE('',#6785,#6969,#728,.T.);
#8971=EDGE_CURVE('',#6661,#6783,#729,.T.);
#8972=EDGE_CURVE('',#6970,#6782,#730,.T.);
#8973=EDGE_CURVE('',#6971,#6970,#731,.T.);
#8974=EDGE_CURVE('',#6972,#6971,#732,.T.);
#8975=EDGE_CURVE('',#6973,#6972,#733,.T.);
#8976=EDGE_CURVE('',#6662,#6973,#734,.T.);
#8977=EDGE_CURVE('',#6969,#6962,#2138,.T.);
#8978=EDGE_CURVE('',#6968,#6963,#2139,.T.);
#8979=EDGE_CURVE('',#6967,#6964,#2140,.T.);
#8980=EDGE_CURVE('',#6966,#6965,#2141,.T.);
#8981=EDGE_CURVE('',#6664,#6780,#735,.T.);
#8982=EDGE_CURVE('',#6974,#6663,#736,.T.);
#8983=EDGE_CURVE('',#6975,#6974,#737,.T.);
#8984=EDGE_CURVE('',#6976,#6975,#738,.T.);
#8985=EDGE_CURVE('',#6977,#6976,#739,.T.);
#8986=EDGE_CURVE('',#6781,#6977,#740,.T.);
#8987=EDGE_CURVE('',#6665,#6779,#741,.T.);
#8988=EDGE_CURVE('',#6978,#6778,#742,.T.);
#8989=EDGE_CURVE('',#6979,#6978,#743,.T.);
#8990=EDGE_CURVE('',#6980,#6979,#744,.T.);
#8991=EDGE_CURVE('',#6981,#6980,#745,.T.);
#8992=EDGE_CURVE('',#6666,#6981,#746,.T.);
#8993=EDGE_CURVE('',#6977,#6970,#2142,.T.);
#8994=EDGE_CURVE('',#6976,#6971,#2143,.T.);
#8995=EDGE_CURVE('',#6975,#6972,#2144,.T.);
#8996=EDGE_CURVE('',#6974,#6973,#2145,.T.);
#8997=EDGE_CURVE('',#6668,#6776,#747,.T.);
#8998=EDGE_CURVE('',#6982,#6667,#748,.T.);
#8999=EDGE_CURVE('',#6983,#6982,#749,.T.);
#9000=EDGE_CURVE('',#6984,#6983,#750,.T.);
#9001=EDGE_CURVE('',#6985,#6984,#751,.T.);
#9002=EDGE_CURVE('',#6777,#6985,#752,.T.);
#9003=EDGE_CURVE('',#6669,#6775,#753,.T.);
#9004=EDGE_CURVE('',#6986,#6774,#754,.T.);
#9005=EDGE_CURVE('',#6987,#6986,#755,.T.);
#9006=EDGE_CURVE('',#6988,#6987,#756,.T.);
#9007=EDGE_CURVE('',#6989,#6988,#757,.T.);
#9008=EDGE_CURVE('',#6670,#6989,#758,.T.);
#9009=EDGE_CURVE('',#6985,#6978,#2146,.T.);
#9010=EDGE_CURVE('',#6984,#6979,#2147,.T.);
#9011=EDGE_CURVE('',#6983,#6980,#2148,.T.);
#9012=EDGE_CURVE('',#6982,#6981,#2149,.T.);
#9013=EDGE_CURVE('',#6672,#6772,#759,.T.);
#9014=EDGE_CURVE('',#6990,#6671,#760,.T.);
#9015=EDGE_CURVE('',#6991,#6990,#761,.T.);
#9016=EDGE_CURVE('',#6992,#6991,#762,.T.);
#9017=EDGE_CURVE('',#6993,#6992,#763,.T.);
#9018=EDGE_CURVE('',#6773,#6993,#764,.T.);
#9019=EDGE_CURVE('',#6673,#6771,#765,.T.);
#9020=EDGE_CURVE('',#6994,#6770,#766,.T.);
#9021=EDGE_CURVE('',#6995,#6994,#767,.T.);
#9022=EDGE_CURVE('',#6996,#6995,#768,.T.);
#9023=EDGE_CURVE('',#6997,#6996,#769,.T.);
#9024=EDGE_CURVE('',#6674,#6997,#770,.T.);
#9025=EDGE_CURVE('',#6993,#6986,#2150,.T.);
#9026=EDGE_CURVE('',#6992,#6987,#2151,.T.);
#9027=EDGE_CURVE('',#6991,#6988,#2152,.T.);
#9028=EDGE_CURVE('',#6990,#6989,#2153,.T.);
#9029=EDGE_CURVE('',#6676,#6768,#771,.T.);
#9030=EDGE_CURVE('',#6998,#6675,#772,.T.);
#9031=EDGE_CURVE('',#6999,#6998,#773,.T.);
#9032=EDGE_CURVE('',#7000,#6999,#774,.T.);
#9033=EDGE_CURVE('',#7001,#7000,#775,.T.);
#9034=EDGE_CURVE('',#6769,#7001,#776,.T.);
#9035=EDGE_CURVE('',#6677,#6767,#777,.T.);
#9036=EDGE_CURVE('',#7002,#6766,#778,.T.);
#9037=EDGE_CURVE('',#7003,#7002,#779,.T.);
#9038=EDGE_CURVE('',#7004,#7003,#780,.T.);
#9039=EDGE_CURVE('',#7005,#7004,#781,.T.);
#9040=EDGE_CURVE('',#6678,#7005,#782,.T.);
#9041=EDGE_CURVE('',#7001,#6994,#2154,.T.);
#9042=EDGE_CURVE('',#7000,#6995,#2155,.T.);
#9043=EDGE_CURVE('',#6999,#6996,#2156,.T.);
#9044=EDGE_CURVE('',#6998,#6997,#2157,.T.);
#9045=EDGE_CURVE('',#6680,#6764,#783,.T.);
#9046=EDGE_CURVE('',#7006,#6679,#784,.T.);
#9047=EDGE_CURVE('',#7007,#7006,#785,.T.);
#9048=EDGE_CURVE('',#7008,#7007,#786,.T.);
#9049=EDGE_CURVE('',#7009,#7008,#787,.T.);
#9050=EDGE_CURVE('',#6765,#7009,#788,.T.);
#9051=EDGE_CURVE('',#6681,#6763,#789,.T.);
#9052=EDGE_CURVE('',#7010,#6762,#790,.T.);
#9053=EDGE_CURVE('',#7011,#7010,#791,.T.);
#9054=EDGE_CURVE('',#7012,#7011,#792,.T.);
#9055=EDGE_CURVE('',#7013,#7012,#793,.T.);
#9056=EDGE_CURVE('',#6682,#7013,#794,.T.);
#9057=EDGE_CURVE('',#7009,#7002,#2158,.T.);
#9058=EDGE_CURVE('',#7008,#7003,#2159,.T.);
#9059=EDGE_CURVE('',#7007,#7004,#2160,.T.);
#9060=EDGE_CURVE('',#7006,#7005,#2161,.T.);
#9061=EDGE_CURVE('',#6684,#6760,#795,.T.);
#9062=EDGE_CURVE('',#7014,#6683,#796,.T.);
#9063=EDGE_CURVE('',#7015,#7014,#797,.T.);
#9064=EDGE_CURVE('',#7016,#7015,#798,.T.);
#9065=EDGE_CURVE('',#7017,#7016,#799,.T.);
#9066=EDGE_CURVE('',#6761,#7017,#800,.T.);
#9067=EDGE_CURVE('',#6685,#6759,#801,.T.);
#9068=EDGE_CURVE('',#7018,#6758,#802,.T.);
#9069=EDGE_CURVE('',#7019,#7018,#803,.T.);
#9070=EDGE_CURVE('',#7020,#7019,#804,.T.);
#9071=EDGE_CURVE('',#7021,#7020,#805,.T.);
#9072=EDGE_CURVE('',#6686,#7021,#806,.T.);
#9073=EDGE_CURVE('',#7017,#7010,#2162,.T.);
#9074=EDGE_CURVE('',#7016,#7011,#2163,.T.);
#9075=EDGE_CURVE('',#7015,#7012,#2164,.T.);
#9076=EDGE_CURVE('',#7014,#7013,#2165,.T.);
#9077=EDGE_CURVE('',#6688,#6756,#807,.T.);
#9078=EDGE_CURVE('',#7022,#6687,#808,.T.);
#9079=EDGE_CURVE('',#7023,#7022,#809,.T.);
#9080=EDGE_CURVE('',#7024,#7023,#810,.T.);
#9081=EDGE_CURVE('',#7025,#7024,#811,.T.);
#9082=EDGE_CURVE('',#6757,#7025,#812,.T.);
#9083=EDGE_CURVE('',#6689,#6755,#813,.T.);
#9084=EDGE_CURVE('',#7026,#6754,#814,.T.);
#9085=EDGE_CURVE('',#7027,#7026,#815,.T.);
#9086=EDGE_CURVE('',#7028,#7027,#816,.T.);
#9087=EDGE_CURVE('',#7029,#7028,#817,.T.);
#9088=EDGE_CURVE('',#6690,#7029,#818,.T.);
#9089=EDGE_CURVE('',#7025,#7018,#2166,.T.);
#9090=EDGE_CURVE('',#7024,#7019,#2167,.T.);
#9091=EDGE_CURVE('',#7023,#7020,#2168,.T.);
#9092=EDGE_CURVE('',#7022,#7021,#2169,.T.);
#9093=EDGE_CURVE('',#6692,#6752,#819,.T.);
#9094=EDGE_CURVE('',#7030,#6691,#820,.T.);
#9095=EDGE_CURVE('',#7031,#7030,#821,.T.);
#9096=EDGE_CURVE('',#7032,#7031,#822,.T.);
#9097=EDGE_CURVE('',#7033,#7032,#823,.T.);
#9098=EDGE_CURVE('',#6753,#7033,#824,.T.);
#9099=EDGE_CURVE('',#6693,#6751,#825,.T.);
#9100=EDGE_CURVE('',#7034,#6750,#826,.T.);
#9101=EDGE_CURVE('',#7035,#7034,#827,.T.);
#9102=EDGE_CURVE('',#7036,#7035,#828,.T.);
#9103=EDGE_CURVE('',#7037,#7036,#829,.T.);
#9104=EDGE_CURVE('',#6694,#7037,#830,.T.);
#9105=EDGE_CURVE('',#7033,#7026,#2170,.T.);
#9106=EDGE_CURVE('',#7032,#7027,#2171,.T.);
#9107=EDGE_CURVE('',#7031,#7028,#2172,.T.);
#9108=EDGE_CURVE('',#7030,#7029,#2173,.T.);
#9109=EDGE_CURVE('',#6696,#6748,#831,.T.);
#9110=EDGE_CURVE('',#7038,#6695,#832,.T.);
#9111=EDGE_CURVE('',#7039,#7038,#833,.T.);
#9112=EDGE_CURVE('',#7040,#7039,#834,.T.);
#9113=EDGE_CURVE('',#7041,#7040,#835,.T.);
#9114=EDGE_CURVE('',#6749,#7041,#836,.T.);
#9115=EDGE_CURVE('',#6697,#6747,#837,.T.);
#9116=EDGE_CURVE('',#7042,#6746,#838,.T.);
#9117=EDGE_CURVE('',#7043,#7042,#839,.T.);
#9118=EDGE_CURVE('',#7044,#7043,#840,.T.);
#9119=EDGE_CURVE('',#7045,#7044,#841,.T.);
#9120=EDGE_CURVE('',#6698,#7045,#842,.T.);
#9121=EDGE_CURVE('',#7041,#7034,#2174,.T.);
#9122=EDGE_CURVE('',#7040,#7035,#2175,.T.);
#9123=EDGE_CURVE('',#7039,#7036,#2176,.T.);
#9124=EDGE_CURVE('',#7038,#7037,#2177,.T.);
#9125=EDGE_CURVE('',#6700,#6744,#843,.T.);
#9126=EDGE_CURVE('',#7046,#6699,#844,.T.);
#9127=EDGE_CURVE('',#7047,#7046,#845,.T.);
#9128=EDGE_CURVE('',#7048,#7047,#846,.T.);
#9129=EDGE_CURVE('',#7049,#7048,#847,.T.);
#9130=EDGE_CURVE('',#6745,#7049,#848,.T.);
#9131=EDGE_CURVE('',#6701,#6743,#849,.T.);
#9132=EDGE_CURVE('',#7050,#6742,#850,.T.);
#9133=EDGE_CURVE('',#7051,#7050,#851,.T.);
#9134=EDGE_CURVE('',#7052,#7051,#852,.T.);
#9135=EDGE_CURVE('',#7053,#7052,#853,.T.);
#9136=EDGE_CURVE('',#6702,#7053,#854,.T.);
#9137=EDGE_CURVE('',#7049,#7042,#2178,.T.);
#9138=EDGE_CURVE('',#7048,#7043,#2179,.T.);
#9139=EDGE_CURVE('',#7047,#7044,#2180,.T.);
#9140=EDGE_CURVE('',#7046,#7045,#2181,.T.);
#9141=EDGE_CURVE('',#6704,#6740,#855,.T.);
#9142=EDGE_CURVE('',#7054,#6703,#856,.T.);
#9143=EDGE_CURVE('',#7055,#7054,#857,.T.);
#9144=EDGE_CURVE('',#7056,#7055,#858,.T.);
#9145=EDGE_CURVE('',#7057,#7056,#859,.T.);
#9146=EDGE_CURVE('',#6741,#7057,#860,.T.);
#9147=EDGE_CURVE('',#6705,#6739,#861,.T.);
#9148=EDGE_CURVE('',#7058,#6738,#862,.T.);
#9149=EDGE_CURVE('',#7059,#7058,#863,.T.);
#9150=EDGE_CURVE('',#7060,#7059,#864,.T.);
#9151=EDGE_CURVE('',#7061,#7060,#865,.T.);
#9152=EDGE_CURVE('',#6706,#7061,#866,.T.);
#9153=EDGE_CURVE('',#7057,#7050,#2182,.T.);
#9154=EDGE_CURVE('',#7056,#7051,#2183,.T.);
#9155=EDGE_CURVE('',#7055,#7052,#2184,.T.);
#9156=EDGE_CURVE('',#7054,#7053,#2185,.T.);
#9157=EDGE_CURVE('',#6708,#6736,#867,.T.);
#9158=EDGE_CURVE('',#7062,#6707,#868,.T.);
#9159=EDGE_CURVE('',#7063,#7062,#869,.T.);
#9160=EDGE_CURVE('',#7064,#7063,#870,.T.);
#9161=EDGE_CURVE('',#7065,#7064,#871,.T.);
#9162=EDGE_CURVE('',#6737,#7065,#872,.T.);
#9163=EDGE_CURVE('',#6709,#6735,#873,.T.);
#9164=EDGE_CURVE('',#7066,#6734,#874,.T.);
#9165=EDGE_CURVE('',#7067,#7066,#875,.T.);
#9166=EDGE_CURVE('',#7068,#7067,#876,.T.);
#9167=EDGE_CURVE('',#7069,#7068,#877,.T.);
#9168=EDGE_CURVE('',#6710,#7069,#878,.T.);
#9169=EDGE_CURVE('',#7065,#7058,#2186,.T.);
#9170=EDGE_CURVE('',#6733,#7070,#879,.T.);
#9171=EDGE_CURVE('',#7070,#7066,#2187,.T.);
#9172=EDGE_CURVE('',#7064,#7059,#2188,.T.);
#9173=EDGE_CURVE('',#7063,#7060,#2189,.T.);
#9174=EDGE_CURVE('',#7062,#7061,#2190,.T.);
#9175=EDGE_CURVE('',#6712,#6732,#880,.T.);
#9176=EDGE_CURVE('',#7071,#6711,#881,.T.);
#9177=EDGE_CURVE('',#7072,#7071,#882,.T.);
#9178=EDGE_CURVE('',#7073,#7072,#883,.T.);
#9179=EDGE_CURVE('',#7070,#7073,#884,.T.);
#9180=EDGE_CURVE('',#6713,#6731,#885,.T.);
#9181=EDGE_CURVE('',#7074,#6730,#886,.T.);
#9182=EDGE_CURVE('',#7075,#7074,#887,.T.);
#9183=EDGE_CURVE('',#7076,#7075,#888,.T.);
#9184=EDGE_CURVE('',#7077,#7076,#889,.T.);
#9185=EDGE_CURVE('',#6714,#7077,#890,.T.);
#9186=EDGE_CURVE('',#6729,#7078,#891,.T.);
#9187=EDGE_CURVE('',#7078,#7074,#2191,.T.);
#9188=EDGE_CURVE('',#7073,#7067,#2192,.T.);
#9189=EDGE_CURVE('',#7078,#7079,#892,.T.);
#9190=EDGE_CURVE('',#7079,#7075,#2193,.T.);
#9191=EDGE_CURVE('',#7071,#7069,#2194,.T.);
#9192=EDGE_CURVE('',#7072,#7068,#2195,.T.);
#9193=EDGE_CURVE('',#6716,#6728,#893,.T.);
#9194=EDGE_CURVE('',#7080,#6715,#894,.T.);
#9195=EDGE_CURVE('',#7081,#7080,#895,.T.);
#9196=EDGE_CURVE('',#7079,#7081,#896,.T.);
#9197=EDGE_CURVE('',#6717,#6727,#897,.T.);
#9198=EDGE_CURVE('',#7081,#7076,#2196,.T.);
#9199=EDGE_CURVE('',#7080,#7077,#2197,.T.);
#11699=ORIENTED_EDGE('',*,*,#8471,.T.);
#11700=ORIENTED_EDGE('',*,*,#8472,.T.);
#11701=ORIENTED_EDGE('',*,*,#8473,.T.);
#11702=ORIENTED_EDGE('',*,*,#8472,.F.);
#11703=ORIENTED_EDGE('',*,*,#8474,.T.);
#11704=ORIENTED_EDGE('',*,*,#8471,.F.);
#11705=ORIENTED_EDGE('',*,*,#8475,.T.);
#11706=ORIENTED_EDGE('',*,*,#8476,.F.);
#11707=ORIENTED_EDGE('',*,*,#8477,.F.);
#11708=ORIENTED_EDGE('',*,*,#8475,.F.);
#11709=ORIENTED_EDGE('',*,*,#8474,.F.);
#11710=ORIENTED_EDGE('',*,*,#8478,.T.);
#11711=ORIENTED_EDGE('',*,*,#8479,.F.);
#11712=ORIENTED_EDGE('',*,*,#8480,.T.);
#11713=ORIENTED_EDGE('',*,*,#8481,.T.);
#11714=ORIENTED_EDGE('',*,*,#8482,.T.);
#11715=ORIENTED_EDGE('',*,*,#8483,.F.);
#11716=ORIENTED_EDGE('',*,*,#8484,.T.);
#11717=ORIENTED_EDGE('',*,*,#8485,.T.);
#11718=ORIENTED_EDGE('',*,*,#8486,.T.);
#11719=ORIENTED_EDGE('',*,*,#8487,.F.);
#11720=ORIENTED_EDGE('',*,*,#8488,.T.);
#11721=ORIENTED_EDGE('',*,*,#8489,.T.);
#11722=ORIENTED_EDGE('',*,*,#8490,.T.);
#11723=ORIENTED_EDGE('',*,*,#8491,.F.);
#11724=ORIENTED_EDGE('',*,*,#8492,.T.);
#11725=ORIENTED_EDGE('',*,*,#8493,.T.);
#11726=ORIENTED_EDGE('',*,*,#8494,.T.);
#11727=ORIENTED_EDGE('',*,*,#8495,.F.);
#11728=ORIENTED_EDGE('',*,*,#8496,.T.);
#11729=ORIENTED_EDGE('',*,*,#8497,.T.);
#11730=ORIENTED_EDGE('',*,*,#8498,.T.);
#11731=ORIENTED_EDGE('',*,*,#8499,.F.);
#11732=ORIENTED_EDGE('',*,*,#8500,.T.);
#11733=ORIENTED_EDGE('',*,*,#8501,.T.);
#11734=ORIENTED_EDGE('',*,*,#8502,.T.);
#11735=ORIENTED_EDGE('',*,*,#8503,.F.);
#11736=ORIENTED_EDGE('',*,*,#8504,.T.);
#11737=ORIENTED_EDGE('',*,*,#8505,.T.);
#11738=ORIENTED_EDGE('',*,*,#8506,.T.);
#11739=ORIENTED_EDGE('',*,*,#8507,.F.);
#11740=ORIENTED_EDGE('',*,*,#8508,.T.);
#11741=ORIENTED_EDGE('',*,*,#8509,.T.);
#11742=ORIENTED_EDGE('',*,*,#8510,.T.);
#11743=ORIENTED_EDGE('',*,*,#8511,.F.);
#11744=ORIENTED_EDGE('',*,*,#8512,.T.);
#11745=ORIENTED_EDGE('',*,*,#8513,.T.);
#11746=ORIENTED_EDGE('',*,*,#8514,.T.);
#11747=ORIENTED_EDGE('',*,*,#8515,.F.);
#11748=ORIENTED_EDGE('',*,*,#8516,.T.);
#11749=ORIENTED_EDGE('',*,*,#8517,.T.);
#11750=ORIENTED_EDGE('',*,*,#8518,.T.);
#11751=ORIENTED_EDGE('',*,*,#8519,.F.);
#11752=ORIENTED_EDGE('',*,*,#8520,.T.);
#11753=ORIENTED_EDGE('',*,*,#8521,.T.);
#11754=ORIENTED_EDGE('',*,*,#8522,.T.);
#11755=ORIENTED_EDGE('',*,*,#8523,.F.);
#11756=ORIENTED_EDGE('',*,*,#8524,.T.);
#11757=ORIENTED_EDGE('',*,*,#8525,.T.);
#11758=ORIENTED_EDGE('',*,*,#8526,.T.);
#11759=ORIENTED_EDGE('',*,*,#8527,.F.);
#11760=ORIENTED_EDGE('',*,*,#8528,.T.);
#11761=ORIENTED_EDGE('',*,*,#8529,.T.);
#11762=ORIENTED_EDGE('',*,*,#8530,.T.);
#11763=ORIENTED_EDGE('',*,*,#8531,.F.);
#11764=ORIENTED_EDGE('',*,*,#8532,.T.);
#11765=ORIENTED_EDGE('',*,*,#8533,.T.);
#11766=ORIENTED_EDGE('',*,*,#8534,.T.);
#11767=ORIENTED_EDGE('',*,*,#8535,.F.);
#11768=ORIENTED_EDGE('',*,*,#8536,.T.);
#11769=ORIENTED_EDGE('',*,*,#8537,.T.);
#11770=ORIENTED_EDGE('',*,*,#8538,.T.);
#11771=ORIENTED_EDGE('',*,*,#8539,.F.);
#11772=ORIENTED_EDGE('',*,*,#8540,.T.);
#11773=ORIENTED_EDGE('',*,*,#8541,.T.);
#11774=ORIENTED_EDGE('',*,*,#8542,.T.);
#11775=ORIENTED_EDGE('',*,*,#8543,.F.);
#11776=ORIENTED_EDGE('',*,*,#8544,.T.);
#11777=ORIENTED_EDGE('',*,*,#8545,.T.);
#11778=ORIENTED_EDGE('',*,*,#8546,.T.);
#11779=ORIENTED_EDGE('',*,*,#8547,.F.);
#11780=ORIENTED_EDGE('',*,*,#8548,.T.);
#11781=ORIENTED_EDGE('',*,*,#8549,.T.);
#11782=ORIENTED_EDGE('',*,*,#8550,.T.);
#11783=ORIENTED_EDGE('',*,*,#8551,.F.);
#11784=ORIENTED_EDGE('',*,*,#8552,.T.);
#11785=ORIENTED_EDGE('',*,*,#8553,.T.);
#11786=ORIENTED_EDGE('',*,*,#8554,.T.);
#11787=ORIENTED_EDGE('',*,*,#8555,.F.);
#11788=ORIENTED_EDGE('',*,*,#8556,.T.);
#11789=ORIENTED_EDGE('',*,*,#8557,.T.);
#11790=ORIENTED_EDGE('',*,*,#8558,.T.);
#11791=ORIENTED_EDGE('',*,*,#8559,.F.);
#11792=ORIENTED_EDGE('',*,*,#8560,.T.);
#11793=ORIENTED_EDGE('',*,*,#8561,.T.);
#11794=ORIENTED_EDGE('',*,*,#8562,.T.);
#11795=ORIENTED_EDGE('',*,*,#8563,.F.);
#11796=ORIENTED_EDGE('',*,*,#8564,.T.);
#11797=ORIENTED_EDGE('',*,*,#8565,.T.);
#11798=ORIENTED_EDGE('',*,*,#8566,.T.);
#11799=ORIENTED_EDGE('',*,*,#8567,.F.);
#11800=ORIENTED_EDGE('',*,*,#8568,.T.);
#11801=ORIENTED_EDGE('',*,*,#8569,.T.);
#11802=ORIENTED_EDGE('',*,*,#8570,.T.);
#11803=ORIENTED_EDGE('',*,*,#8571,.F.);
#11804=ORIENTED_EDGE('',*,*,#8572,.T.);
#11805=ORIENTED_EDGE('',*,*,#8573,.T.);
#11806=ORIENTED_EDGE('',*,*,#8574,.T.);
#11807=ORIENTED_EDGE('',*,*,#8575,.F.);
#11808=ORIENTED_EDGE('',*,*,#8576,.T.);
#11809=ORIENTED_EDGE('',*,*,#8577,.T.);
#11810=ORIENTED_EDGE('',*,*,#8578,.T.);
#11811=ORIENTED_EDGE('',*,*,#8579,.F.);
#11812=ORIENTED_EDGE('',*,*,#8580,.T.);
#11813=ORIENTED_EDGE('',*,*,#8581,.T.);
#11814=ORIENTED_EDGE('',*,*,#8582,.T.);
#11815=ORIENTED_EDGE('',*,*,#8583,.F.);
#11816=ORIENTED_EDGE('',*,*,#8584,.T.);
#11817=ORIENTED_EDGE('',*,*,#8585,.T.);
#11818=ORIENTED_EDGE('',*,*,#8586,.T.);
#11819=ORIENTED_EDGE('',*,*,#8587,.F.);
#11820=ORIENTED_EDGE('',*,*,#8588,.T.);
#11821=ORIENTED_EDGE('',*,*,#8589,.T.);
#11822=ORIENTED_EDGE('',*,*,#8590,.T.);
#11823=ORIENTED_EDGE('',*,*,#8591,.F.);
#11824=ORIENTED_EDGE('',*,*,#8592,.T.);
#11825=ORIENTED_EDGE('',*,*,#8593,.T.);
#11826=ORIENTED_EDGE('',*,*,#8594,.T.);
#11827=ORIENTED_EDGE('',*,*,#8595,.F.);
#11828=ORIENTED_EDGE('',*,*,#8596,.T.);
#11829=ORIENTED_EDGE('',*,*,#8597,.T.);
#11830=ORIENTED_EDGE('',*,*,#8473,.F.);
#11831=ORIENTED_EDGE('',*,*,#8476,.T.);
#11832=ORIENTED_EDGE('',*,*,#8477,.T.);
#11833=ORIENTED_EDGE('',*,*,#8598,.T.);
#11834=ORIENTED_EDGE('',*,*,#8599,.T.);
#11835=ORIENTED_EDGE('',*,*,#8598,.F.);
#11836=ORIENTED_EDGE('',*,*,#8600,.T.);
#11837=ORIENTED_EDGE('',*,*,#8601,.T.);
#11838=ORIENTED_EDGE('',*,*,#8602,.T.);
#11839=ORIENTED_EDGE('',*,*,#8603,.T.);
#11840=ORIENTED_EDGE('',*,*,#8604,.T.);
#11841=ORIENTED_EDGE('',*,*,#8605,.T.);
#11842=ORIENTED_EDGE('',*,*,#8606,.T.);
#11843=ORIENTED_EDGE('',*,*,#8607,.T.);
#11844=ORIENTED_EDGE('',*,*,#8608,.T.);
#11845=ORIENTED_EDGE('',*,*,#8609,.T.);
#11846=ORIENTED_EDGE('',*,*,#8610,.T.);
#11847=ORIENTED_EDGE('',*,*,#8611,.T.);
#11848=ORIENTED_EDGE('',*,*,#8612,.T.);
#11849=ORIENTED_EDGE('',*,*,#8613,.T.);
#11850=ORIENTED_EDGE('',*,*,#8614,.T.);
#11851=ORIENTED_EDGE('',*,*,#8615,.T.);
#11852=ORIENTED_EDGE('',*,*,#8616,.T.);
#11853=ORIENTED_EDGE('',*,*,#8617,.T.);
#11854=ORIENTED_EDGE('',*,*,#8618,.T.);
#11855=ORIENTED_EDGE('',*,*,#8619,.T.);
#11856=ORIENTED_EDGE('',*,*,#8620,.T.);
#11857=ORIENTED_EDGE('',*,*,#8621,.T.);
#11858=ORIENTED_EDGE('',*,*,#8622,.T.);
#11859=ORIENTED_EDGE('',*,*,#8623,.T.);
#11860=ORIENTED_EDGE('',*,*,#8624,.T.);
#11861=ORIENTED_EDGE('',*,*,#8625,.T.);
#11862=ORIENTED_EDGE('',*,*,#8626,.T.);
#11863=ORIENTED_EDGE('',*,*,#8627,.T.);
#11864=ORIENTED_EDGE('',*,*,#8628,.T.);
#11865=ORIENTED_EDGE('',*,*,#8629,.T.);
#11866=ORIENTED_EDGE('',*,*,#8630,.T.);
#11867=ORIENTED_EDGE('',*,*,#8631,.T.);
#11868=ORIENTED_EDGE('',*,*,#8632,.T.);
#11869=ORIENTED_EDGE('',*,*,#8633,.T.);
#11870=ORIENTED_EDGE('',*,*,#8634,.T.);
#11871=ORIENTED_EDGE('',*,*,#8635,.T.);
#11872=ORIENTED_EDGE('',*,*,#8636,.T.);
#11873=ORIENTED_EDGE('',*,*,#8637,.T.);
#11874=ORIENTED_EDGE('',*,*,#8638,.T.);
#11875=ORIENTED_EDGE('',*,*,#8639,.T.);
#11876=ORIENTED_EDGE('',*,*,#8640,.T.);
#11877=ORIENTED_EDGE('',*,*,#8641,.T.);
#11878=ORIENTED_EDGE('',*,*,#8642,.T.);
#11879=ORIENTED_EDGE('',*,*,#8643,.T.);
#11880=ORIENTED_EDGE('',*,*,#8644,.T.);
#11881=ORIENTED_EDGE('',*,*,#8645,.T.);
#11882=ORIENTED_EDGE('',*,*,#8646,.T.);
#11883=ORIENTED_EDGE('',*,*,#8647,.T.);
#11884=ORIENTED_EDGE('',*,*,#8648,.T.);
#11885=ORIENTED_EDGE('',*,*,#8649,.T.);
#11886=ORIENTED_EDGE('',*,*,#8650,.T.);
#11887=ORIENTED_EDGE('',*,*,#8651,.T.);
#11888=ORIENTED_EDGE('',*,*,#8652,.T.);
#11889=ORIENTED_EDGE('',*,*,#8653,.T.);
#11890=ORIENTED_EDGE('',*,*,#8654,.T.);
#11891=ORIENTED_EDGE('',*,*,#8655,.T.);
#11892=ORIENTED_EDGE('',*,*,#8656,.T.);
#11893=ORIENTED_EDGE('',*,*,#8657,.T.);
#11894=ORIENTED_EDGE('',*,*,#8658,.T.);
#11895=ORIENTED_EDGE('',*,*,#8659,.T.);
#11896=ORIENTED_EDGE('',*,*,#8660,.T.);
#11897=ORIENTED_EDGE('',*,*,#8661,.T.);
#11898=ORIENTED_EDGE('',*,*,#8662,.T.);
#11899=ORIENTED_EDGE('',*,*,#8663,.T.);
#11900=ORIENTED_EDGE('',*,*,#8664,.T.);
#11901=ORIENTED_EDGE('',*,*,#8665,.T.);
#11902=ORIENTED_EDGE('',*,*,#8666,.T.);
#11903=ORIENTED_EDGE('',*,*,#8667,.T.);
#11904=ORIENTED_EDGE('',*,*,#8668,.T.);
#11905=ORIENTED_EDGE('',*,*,#8669,.T.);
#11906=ORIENTED_EDGE('',*,*,#8670,.T.);
#11907=ORIENTED_EDGE('',*,*,#8671,.T.);
#11908=ORIENTED_EDGE('',*,*,#8672,.T.);
#11909=ORIENTED_EDGE('',*,*,#8673,.T.);
#11910=ORIENTED_EDGE('',*,*,#8674,.T.);
#11911=ORIENTED_EDGE('',*,*,#8675,.T.);
#11912=ORIENTED_EDGE('',*,*,#8676,.T.);
#11913=ORIENTED_EDGE('',*,*,#8677,.T.);
#11914=ORIENTED_EDGE('',*,*,#8678,.T.);
#11915=ORIENTED_EDGE('',*,*,#8679,.T.);
#11916=ORIENTED_EDGE('',*,*,#8680,.T.);
#11917=ORIENTED_EDGE('',*,*,#8681,.T.);
#11918=ORIENTED_EDGE('',*,*,#8682,.T.);
#11919=ORIENTED_EDGE('',*,*,#8683,.T.);
#11920=ORIENTED_EDGE('',*,*,#8684,.T.);
#11921=ORIENTED_EDGE('',*,*,#8685,.T.);
#11922=ORIENTED_EDGE('',*,*,#8686,.T.);
#11923=ORIENTED_EDGE('',*,*,#8687,.T.);
#11924=ORIENTED_EDGE('',*,*,#8688,.T.);
#11925=ORIENTED_EDGE('',*,*,#8689,.T.);
#11926=ORIENTED_EDGE('',*,*,#8690,.T.);
#11927=ORIENTED_EDGE('',*,*,#8691,.T.);
#11928=ORIENTED_EDGE('',*,*,#8692,.T.);
#11929=ORIENTED_EDGE('',*,*,#8693,.T.);
#11930=ORIENTED_EDGE('',*,*,#8694,.T.);
#11931=ORIENTED_EDGE('',*,*,#8695,.T.);
#11932=ORIENTED_EDGE('',*,*,#8696,.T.);
#11933=ORIENTED_EDGE('',*,*,#8697,.T.);
#11934=ORIENTED_EDGE('',*,*,#8698,.T.);
#11935=ORIENTED_EDGE('',*,*,#8699,.T.);
#11936=ORIENTED_EDGE('',*,*,#8700,.T.);
#11937=ORIENTED_EDGE('',*,*,#8701,.T.);
#11938=ORIENTED_EDGE('',*,*,#8702,.T.);
#11939=ORIENTED_EDGE('',*,*,#8703,.T.);
#11940=ORIENTED_EDGE('',*,*,#8704,.T.);
#11941=ORIENTED_EDGE('',*,*,#8705,.T.);
#11942=ORIENTED_EDGE('',*,*,#8706,.T.);
#11943=ORIENTED_EDGE('',*,*,#8707,.T.);
#11944=ORIENTED_EDGE('',*,*,#8708,.T.);
#11945=ORIENTED_EDGE('',*,*,#8709,.T.);
#11946=ORIENTED_EDGE('',*,*,#8710,.T.);
#11947=ORIENTED_EDGE('',*,*,#8711,.T.);
#11948=ORIENTED_EDGE('',*,*,#8712,.T.);
#11949=ORIENTED_EDGE('',*,*,#8713,.T.);
#11950=ORIENTED_EDGE('',*,*,#8714,.T.);
#11951=ORIENTED_EDGE('',*,*,#8715,.T.);
#11952=ORIENTED_EDGE('',*,*,#8716,.T.);
#11953=ORIENTED_EDGE('',*,*,#8717,.T.);
#11954=ORIENTED_EDGE('',*,*,#8718,.T.);
#11955=ORIENTED_EDGE('',*,*,#8719,.T.);
#11956=ORIENTED_EDGE('',*,*,#8599,.F.);
#11957=ORIENTED_EDGE('',*,*,#8602,.F.);
#11958=ORIENTED_EDGE('',*,*,#8720,.F.);
#11959=ORIENTED_EDGE('',*,*,#8596,.F.);
#11960=ORIENTED_EDGE('',*,*,#8721,.F.);
#11961=ORIENTED_EDGE('',*,*,#8722,.F.);
#11962=ORIENTED_EDGE('',*,*,#8723,.F.);
#11963=ORIENTED_EDGE('',*,*,#8724,.F.);
#11964=ORIENTED_EDGE('',*,*,#8725,.F.);
#11965=ORIENTED_EDGE('',*,*,#8601,.F.);
#11966=ORIENTED_EDGE('',*,*,#8726,.F.);
#11967=ORIENTED_EDGE('',*,*,#8597,.F.);
#11968=ORIENTED_EDGE('',*,*,#8720,.T.);
#11969=ORIENTED_EDGE('',*,*,#8600,.F.);
#11970=ORIENTED_EDGE('',*,*,#8727,.F.);
#11971=ORIENTED_EDGE('',*,*,#8728,.F.);
#11972=ORIENTED_EDGE('',*,*,#8729,.F.);
#11973=ORIENTED_EDGE('',*,*,#8730,.F.);
#11974=ORIENTED_EDGE('',*,*,#8731,.F.);
#11975=ORIENTED_EDGE('',*,*,#8478,.F.);
#11976=ORIENTED_EDGE('',*,*,#8726,.T.);
#11977=ORIENTED_EDGE('',*,*,#8725,.T.);
#11978=ORIENTED_EDGE('',*,*,#8732,.T.);
#11979=ORIENTED_EDGE('',*,*,#8733,.T.);
#11980=ORIENTED_EDGE('',*,*,#8603,.F.);
#11981=ORIENTED_EDGE('',*,*,#8724,.T.);
#11982=ORIENTED_EDGE('',*,*,#8734,.T.);
#11983=ORIENTED_EDGE('',*,*,#8735,.T.);
#11984=ORIENTED_EDGE('',*,*,#8732,.F.);
#11985=ORIENTED_EDGE('',*,*,#8723,.T.);
#11986=ORIENTED_EDGE('',*,*,#8736,.T.);
#11987=ORIENTED_EDGE('',*,*,#8737,.T.);
#11988=ORIENTED_EDGE('',*,*,#8734,.F.);
#11989=ORIENTED_EDGE('',*,*,#8722,.T.);
#11990=ORIENTED_EDGE('',*,*,#8738,.T.);
#11991=ORIENTED_EDGE('',*,*,#8739,.T.);
#11992=ORIENTED_EDGE('',*,*,#8736,.F.);
#11993=ORIENTED_EDGE('',*,*,#8721,.T.);
#11994=ORIENTED_EDGE('',*,*,#8595,.T.);
#11995=ORIENTED_EDGE('',*,*,#8740,.T.);
#11996=ORIENTED_EDGE('',*,*,#8738,.F.);
#11997=ORIENTED_EDGE('',*,*,#8718,.F.);
#11998=ORIENTED_EDGE('',*,*,#8741,.F.);
#11999=ORIENTED_EDGE('',*,*,#8480,.F.);
#12000=ORIENTED_EDGE('',*,*,#8742,.F.);
#12001=ORIENTED_EDGE('',*,*,#8743,.F.);
#12002=ORIENTED_EDGE('',*,*,#8744,.F.);
#12003=ORIENTED_EDGE('',*,*,#8745,.F.);
#12004=ORIENTED_EDGE('',*,*,#8746,.F.);
#12005=ORIENTED_EDGE('',*,*,#8717,.F.);
#12006=ORIENTED_EDGE('',*,*,#8747,.F.);
#12007=ORIENTED_EDGE('',*,*,#8481,.F.);
#12008=ORIENTED_EDGE('',*,*,#8741,.T.);
#12009=ORIENTED_EDGE('',*,*,#8716,.F.);
#12010=ORIENTED_EDGE('',*,*,#8748,.F.);
#12011=ORIENTED_EDGE('',*,*,#8749,.F.);
#12012=ORIENTED_EDGE('',*,*,#8750,.F.);
#12013=ORIENTED_EDGE('',*,*,#8751,.F.);
#12014=ORIENTED_EDGE('',*,*,#8752,.F.);
#12015=ORIENTED_EDGE('',*,*,#8482,.F.);
#12016=ORIENTED_EDGE('',*,*,#8747,.T.);
#12017=ORIENTED_EDGE('',*,*,#8727,.T.);
#12018=ORIENTED_EDGE('',*,*,#8719,.F.);
#12019=ORIENTED_EDGE('',*,*,#8746,.T.);
#12020=ORIENTED_EDGE('',*,*,#8753,.T.);
#12021=ORIENTED_EDGE('',*,*,#8728,.T.);
#12022=ORIENTED_EDGE('',*,*,#8753,.F.);
#12023=ORIENTED_EDGE('',*,*,#8745,.T.);
#12024=ORIENTED_EDGE('',*,*,#8754,.T.);
#12025=ORIENTED_EDGE('',*,*,#8729,.T.);
#12026=ORIENTED_EDGE('',*,*,#8754,.F.);
#12027=ORIENTED_EDGE('',*,*,#8744,.T.);
#12028=ORIENTED_EDGE('',*,*,#8755,.T.);
#12029=ORIENTED_EDGE('',*,*,#8730,.T.);
#12030=ORIENTED_EDGE('',*,*,#8755,.F.);
#12031=ORIENTED_EDGE('',*,*,#8743,.T.);
#12032=ORIENTED_EDGE('',*,*,#8756,.T.);
#12033=ORIENTED_EDGE('',*,*,#8731,.T.);
#12034=ORIENTED_EDGE('',*,*,#8756,.F.);
#12035=ORIENTED_EDGE('',*,*,#8742,.T.);
#12036=ORIENTED_EDGE('',*,*,#8479,.T.);
#12037=ORIENTED_EDGE('',*,*,#8714,.F.);
#12038=ORIENTED_EDGE('',*,*,#8757,.F.);
#12039=ORIENTED_EDGE('',*,*,#8484,.F.);
#12040=ORIENTED_EDGE('',*,*,#8758,.F.);
#12041=ORIENTED_EDGE('',*,*,#8759,.F.);
#12042=ORIENTED_EDGE('',*,*,#8760,.F.);
#12043=ORIENTED_EDGE('',*,*,#8761,.F.);
#12044=ORIENTED_EDGE('',*,*,#8762,.F.);
#12045=ORIENTED_EDGE('',*,*,#8713,.F.);
#12046=ORIENTED_EDGE('',*,*,#8763,.F.);
#12047=ORIENTED_EDGE('',*,*,#8485,.F.);
#12048=ORIENTED_EDGE('',*,*,#8757,.T.);
#12049=ORIENTED_EDGE('',*,*,#8712,.F.);
#12050=ORIENTED_EDGE('',*,*,#8764,.F.);
#12051=ORIENTED_EDGE('',*,*,#8765,.F.);
#12052=ORIENTED_EDGE('',*,*,#8766,.F.);
#12053=ORIENTED_EDGE('',*,*,#8767,.F.);
#12054=ORIENTED_EDGE('',*,*,#8768,.F.);
#12055=ORIENTED_EDGE('',*,*,#8486,.F.);
#12056=ORIENTED_EDGE('',*,*,#8763,.T.);
#12057=ORIENTED_EDGE('',*,*,#8748,.T.);
#12058=ORIENTED_EDGE('',*,*,#8715,.F.);
#12059=ORIENTED_EDGE('',*,*,#8762,.T.);
#12060=ORIENTED_EDGE('',*,*,#8769,.T.);
#12061=ORIENTED_EDGE('',*,*,#8749,.T.);
#12062=ORIENTED_EDGE('',*,*,#8769,.F.);
#12063=ORIENTED_EDGE('',*,*,#8761,.T.);
#12064=ORIENTED_EDGE('',*,*,#8770,.T.);
#12065=ORIENTED_EDGE('',*,*,#8750,.T.);
#12066=ORIENTED_EDGE('',*,*,#8770,.F.);
#12067=ORIENTED_EDGE('',*,*,#8760,.T.);
#12068=ORIENTED_EDGE('',*,*,#8771,.T.);
#12069=ORIENTED_EDGE('',*,*,#8751,.T.);
#12070=ORIENTED_EDGE('',*,*,#8771,.F.);
#12071=ORIENTED_EDGE('',*,*,#8759,.T.);
#12072=ORIENTED_EDGE('',*,*,#8772,.T.);
#12073=ORIENTED_EDGE('',*,*,#8752,.T.);
#12074=ORIENTED_EDGE('',*,*,#8772,.F.);
#12075=ORIENTED_EDGE('',*,*,#8758,.T.);
#12076=ORIENTED_EDGE('',*,*,#8483,.T.);
#12077=ORIENTED_EDGE('',*,*,#8710,.F.);
#12078=ORIENTED_EDGE('',*,*,#8773,.F.);
#12079=ORIENTED_EDGE('',*,*,#8488,.F.);
#12080=ORIENTED_EDGE('',*,*,#8774,.F.);
#12081=ORIENTED_EDGE('',*,*,#8775,.F.);
#12082=ORIENTED_EDGE('',*,*,#8776,.F.);
#12083=ORIENTED_EDGE('',*,*,#8777,.F.);
#12084=ORIENTED_EDGE('',*,*,#8778,.F.);
#12085=ORIENTED_EDGE('',*,*,#8709,.F.);
#12086=ORIENTED_EDGE('',*,*,#8779,.F.);
#12087=ORIENTED_EDGE('',*,*,#8489,.F.);
#12088=ORIENTED_EDGE('',*,*,#8773,.T.);
#12089=ORIENTED_EDGE('',*,*,#8708,.F.);
#12090=ORIENTED_EDGE('',*,*,#8780,.F.);
#12091=ORIENTED_EDGE('',*,*,#8781,.F.);
#12092=ORIENTED_EDGE('',*,*,#8782,.F.);
#12093=ORIENTED_EDGE('',*,*,#8783,.F.);
#12094=ORIENTED_EDGE('',*,*,#8784,.F.);
#12095=ORIENTED_EDGE('',*,*,#8490,.F.);
#12096=ORIENTED_EDGE('',*,*,#8779,.T.);
#12097=ORIENTED_EDGE('',*,*,#8764,.T.);
#12098=ORIENTED_EDGE('',*,*,#8711,.F.);
#12099=ORIENTED_EDGE('',*,*,#8778,.T.);
#12100=ORIENTED_EDGE('',*,*,#8785,.T.);
#12101=ORIENTED_EDGE('',*,*,#8765,.T.);
#12102=ORIENTED_EDGE('',*,*,#8785,.F.);
#12103=ORIENTED_EDGE('',*,*,#8777,.T.);
#12104=ORIENTED_EDGE('',*,*,#8786,.T.);
#12105=ORIENTED_EDGE('',*,*,#8766,.T.);
#12106=ORIENTED_EDGE('',*,*,#8786,.F.);
#12107=ORIENTED_EDGE('',*,*,#8776,.T.);
#12108=ORIENTED_EDGE('',*,*,#8787,.T.);
#12109=ORIENTED_EDGE('',*,*,#8767,.T.);
#12110=ORIENTED_EDGE('',*,*,#8787,.F.);
#12111=ORIENTED_EDGE('',*,*,#8775,.T.);
#12112=ORIENTED_EDGE('',*,*,#8788,.T.);
#12113=ORIENTED_EDGE('',*,*,#8768,.T.);
#12114=ORIENTED_EDGE('',*,*,#8788,.F.);
#12115=ORIENTED_EDGE('',*,*,#8774,.T.);
#12116=ORIENTED_EDGE('',*,*,#8487,.T.);
#12117=ORIENTED_EDGE('',*,*,#8706,.F.);
#12118=ORIENTED_EDGE('',*,*,#8789,.F.);
#12119=ORIENTED_EDGE('',*,*,#8492,.F.);
#12120=ORIENTED_EDGE('',*,*,#8790,.F.);
#12121=ORIENTED_EDGE('',*,*,#8791,.F.);
#12122=ORIENTED_EDGE('',*,*,#8792,.F.);
#12123=ORIENTED_EDGE('',*,*,#8793,.F.);
#12124=ORIENTED_EDGE('',*,*,#8794,.F.);
#12125=ORIENTED_EDGE('',*,*,#8705,.F.);
#12126=ORIENTED_EDGE('',*,*,#8795,.F.);
#12127=ORIENTED_EDGE('',*,*,#8493,.F.);
#12128=ORIENTED_EDGE('',*,*,#8789,.T.);
#12129=ORIENTED_EDGE('',*,*,#8704,.F.);
#12130=ORIENTED_EDGE('',*,*,#8796,.F.);
#12131=ORIENTED_EDGE('',*,*,#8797,.F.);
#12132=ORIENTED_EDGE('',*,*,#8798,.F.);
#12133=ORIENTED_EDGE('',*,*,#8799,.F.);
#12134=ORIENTED_EDGE('',*,*,#8800,.F.);
#12135=ORIENTED_EDGE('',*,*,#8494,.F.);
#12136=ORIENTED_EDGE('',*,*,#8795,.T.);
#12137=ORIENTED_EDGE('',*,*,#8780,.T.);
#12138=ORIENTED_EDGE('',*,*,#8707,.F.);
#12139=ORIENTED_EDGE('',*,*,#8794,.T.);
#12140=ORIENTED_EDGE('',*,*,#8801,.T.);
#12141=ORIENTED_EDGE('',*,*,#8781,.T.);
#12142=ORIENTED_EDGE('',*,*,#8801,.F.);
#12143=ORIENTED_EDGE('',*,*,#8793,.T.);
#12144=ORIENTED_EDGE('',*,*,#8802,.T.);
#12145=ORIENTED_EDGE('',*,*,#8782,.T.);
#12146=ORIENTED_EDGE('',*,*,#8802,.F.);
#12147=ORIENTED_EDGE('',*,*,#8792,.T.);
#12148=ORIENTED_EDGE('',*,*,#8803,.T.);
#12149=ORIENTED_EDGE('',*,*,#8783,.T.);
#12150=ORIENTED_EDGE('',*,*,#8803,.F.);
#12151=ORIENTED_EDGE('',*,*,#8791,.T.);
#12152=ORIENTED_EDGE('',*,*,#8804,.T.);
#12153=ORIENTED_EDGE('',*,*,#8784,.T.);
#12154=ORIENTED_EDGE('',*,*,#8804,.F.);
#12155=ORIENTED_EDGE('',*,*,#8790,.T.);
#12156=ORIENTED_EDGE('',*,*,#8491,.T.);
#12157=ORIENTED_EDGE('',*,*,#8702,.F.);
#12158=ORIENTED_EDGE('',*,*,#8805,.F.);
#12159=ORIENTED_EDGE('',*,*,#8496,.F.);
#12160=ORIENTED_EDGE('',*,*,#8806,.F.);
#12161=ORIENTED_EDGE('',*,*,#8807,.F.);
#12162=ORIENTED_EDGE('',*,*,#8808,.F.);
#12163=ORIENTED_EDGE('',*,*,#8809,.F.);
#12164=ORIENTED_EDGE('',*,*,#8810,.F.);
#12165=ORIENTED_EDGE('',*,*,#8701,.F.);
#12166=ORIENTED_EDGE('',*,*,#8811,.F.);
#12167=ORIENTED_EDGE('',*,*,#8497,.F.);
#12168=ORIENTED_EDGE('',*,*,#8805,.T.);
#12169=ORIENTED_EDGE('',*,*,#8700,.F.);
#12170=ORIENTED_EDGE('',*,*,#8812,.F.);
#12171=ORIENTED_EDGE('',*,*,#8813,.F.);
#12172=ORIENTED_EDGE('',*,*,#8814,.F.);
#12173=ORIENTED_EDGE('',*,*,#8815,.F.);
#12174=ORIENTED_EDGE('',*,*,#8816,.F.);
#12175=ORIENTED_EDGE('',*,*,#8498,.F.);
#12176=ORIENTED_EDGE('',*,*,#8811,.T.);
#12177=ORIENTED_EDGE('',*,*,#8796,.T.);
#12178=ORIENTED_EDGE('',*,*,#8703,.F.);
#12179=ORIENTED_EDGE('',*,*,#8810,.T.);
#12180=ORIENTED_EDGE('',*,*,#8817,.T.);
#12181=ORIENTED_EDGE('',*,*,#8797,.T.);
#12182=ORIENTED_EDGE('',*,*,#8817,.F.);
#12183=ORIENTED_EDGE('',*,*,#8809,.T.);
#12184=ORIENTED_EDGE('',*,*,#8818,.T.);
#12185=ORIENTED_EDGE('',*,*,#8798,.T.);
#12186=ORIENTED_EDGE('',*,*,#8818,.F.);
#12187=ORIENTED_EDGE('',*,*,#8808,.T.);
#12188=ORIENTED_EDGE('',*,*,#8819,.T.);
#12189=ORIENTED_EDGE('',*,*,#8799,.T.);
#12190=ORIENTED_EDGE('',*,*,#8819,.F.);
#12191=ORIENTED_EDGE('',*,*,#8807,.T.);
#12192=ORIENTED_EDGE('',*,*,#8820,.T.);
#12193=ORIENTED_EDGE('',*,*,#8800,.T.);
#12194=ORIENTED_EDGE('',*,*,#8820,.F.);
#12195=ORIENTED_EDGE('',*,*,#8806,.T.);
#12196=ORIENTED_EDGE('',*,*,#8495,.T.);
#12197=ORIENTED_EDGE('',*,*,#8698,.F.);
#12198=ORIENTED_EDGE('',*,*,#8821,.F.);
#12199=ORIENTED_EDGE('',*,*,#8500,.F.);
#12200=ORIENTED_EDGE('',*,*,#8822,.F.);
#12201=ORIENTED_EDGE('',*,*,#8823,.F.);
#12202=ORIENTED_EDGE('',*,*,#8824,.F.);
#12203=ORIENTED_EDGE('',*,*,#8825,.F.);
#12204=ORIENTED_EDGE('',*,*,#8826,.F.);
#12205=ORIENTED_EDGE('',*,*,#8697,.F.);
#12206=ORIENTED_EDGE('',*,*,#8827,.F.);
#12207=ORIENTED_EDGE('',*,*,#8501,.F.);
#12208=ORIENTED_EDGE('',*,*,#8821,.T.);
#12209=ORIENTED_EDGE('',*,*,#8696,.F.);
#12210=ORIENTED_EDGE('',*,*,#8828,.F.);
#12211=ORIENTED_EDGE('',*,*,#8829,.F.);
#12212=ORIENTED_EDGE('',*,*,#8830,.F.);
#12213=ORIENTED_EDGE('',*,*,#8831,.F.);
#12214=ORIENTED_EDGE('',*,*,#8832,.F.);
#12215=ORIENTED_EDGE('',*,*,#8502,.F.);
#12216=ORIENTED_EDGE('',*,*,#8827,.T.);
#12217=ORIENTED_EDGE('',*,*,#8812,.T.);
#12218=ORIENTED_EDGE('',*,*,#8699,.F.);
#12219=ORIENTED_EDGE('',*,*,#8826,.T.);
#12220=ORIENTED_EDGE('',*,*,#8833,.T.);
#12221=ORIENTED_EDGE('',*,*,#8813,.T.);
#12222=ORIENTED_EDGE('',*,*,#8833,.F.);
#12223=ORIENTED_EDGE('',*,*,#8825,.T.);
#12224=ORIENTED_EDGE('',*,*,#8834,.T.);
#12225=ORIENTED_EDGE('',*,*,#8814,.T.);
#12226=ORIENTED_EDGE('',*,*,#8834,.F.);
#12227=ORIENTED_EDGE('',*,*,#8824,.T.);
#12228=ORIENTED_EDGE('',*,*,#8835,.T.);
#12229=ORIENTED_EDGE('',*,*,#8815,.T.);
#12230=ORIENTED_EDGE('',*,*,#8835,.F.);
#12231=ORIENTED_EDGE('',*,*,#8823,.T.);
#12232=ORIENTED_EDGE('',*,*,#8836,.T.);
#12233=ORIENTED_EDGE('',*,*,#8816,.T.);
#12234=ORIENTED_EDGE('',*,*,#8836,.F.);
#12235=ORIENTED_EDGE('',*,*,#8822,.T.);
#12236=ORIENTED_EDGE('',*,*,#8499,.T.);
#12237=ORIENTED_EDGE('',*,*,#8694,.F.);
#12238=ORIENTED_EDGE('',*,*,#8837,.F.);
#12239=ORIENTED_EDGE('',*,*,#8504,.F.);
#12240=ORIENTED_EDGE('',*,*,#8838,.F.);
#12241=ORIENTED_EDGE('',*,*,#8839,.F.);
#12242=ORIENTED_EDGE('',*,*,#8840,.F.);
#12243=ORIENTED_EDGE('',*,*,#8841,.F.);
#12244=ORIENTED_EDGE('',*,*,#8842,.F.);
#12245=ORIENTED_EDGE('',*,*,#8693,.F.);
#12246=ORIENTED_EDGE('',*,*,#8843,.F.);
#12247=ORIENTED_EDGE('',*,*,#8505,.F.);
#12248=ORIENTED_EDGE('',*,*,#8837,.T.);
#12249=ORIENTED_EDGE('',*,*,#8692,.F.);
#12250=ORIENTED_EDGE('',*,*,#8844,.F.);
#12251=ORIENTED_EDGE('',*,*,#8845,.F.);
#12252=ORIENTED_EDGE('',*,*,#8846,.F.);
#12253=ORIENTED_EDGE('',*,*,#8847,.F.);
#12254=ORIENTED_EDGE('',*,*,#8848,.F.);
#12255=ORIENTED_EDGE('',*,*,#8506,.F.);
#12256=ORIENTED_EDGE('',*,*,#8843,.T.);
#12257=ORIENTED_EDGE('',*,*,#8828,.T.);
#12258=ORIENTED_EDGE('',*,*,#8695,.F.);
#12259=ORIENTED_EDGE('',*,*,#8842,.T.);
#12260=ORIENTED_EDGE('',*,*,#8849,.T.);
#12261=ORIENTED_EDGE('',*,*,#8829,.T.);
#12262=ORIENTED_EDGE('',*,*,#8849,.F.);
#12263=ORIENTED_EDGE('',*,*,#8841,.T.);
#12264=ORIENTED_EDGE('',*,*,#8850,.T.);
#12265=ORIENTED_EDGE('',*,*,#8830,.T.);
#12266=ORIENTED_EDGE('',*,*,#8850,.F.);
#12267=ORIENTED_EDGE('',*,*,#8840,.T.);
#12268=ORIENTED_EDGE('',*,*,#8851,.T.);
#12269=ORIENTED_EDGE('',*,*,#8831,.T.);
#12270=ORIENTED_EDGE('',*,*,#8851,.F.);
#12271=ORIENTED_EDGE('',*,*,#8839,.T.);
#12272=ORIENTED_EDGE('',*,*,#8852,.T.);
#12273=ORIENTED_EDGE('',*,*,#8832,.T.);
#12274=ORIENTED_EDGE('',*,*,#8852,.F.);
#12275=ORIENTED_EDGE('',*,*,#8838,.T.);
#12276=ORIENTED_EDGE('',*,*,#8503,.T.);
#12277=ORIENTED_EDGE('',*,*,#8690,.F.);
#12278=ORIENTED_EDGE('',*,*,#8853,.F.);
#12279=ORIENTED_EDGE('',*,*,#8508,.F.);
#12280=ORIENTED_EDGE('',*,*,#8854,.F.);
#12281=ORIENTED_EDGE('',*,*,#8855,.F.);
#12282=ORIENTED_EDGE('',*,*,#8856,.F.);
#12283=ORIENTED_EDGE('',*,*,#8857,.F.);
#12284=ORIENTED_EDGE('',*,*,#8858,.F.);
#12285=ORIENTED_EDGE('',*,*,#8689,.F.);
#12286=ORIENTED_EDGE('',*,*,#8859,.F.);
#12287=ORIENTED_EDGE('',*,*,#8509,.F.);
#12288=ORIENTED_EDGE('',*,*,#8853,.T.);
#12289=ORIENTED_EDGE('',*,*,#8688,.F.);
#12290=ORIENTED_EDGE('',*,*,#8860,.F.);
#12291=ORIENTED_EDGE('',*,*,#8861,.F.);
#12292=ORIENTED_EDGE('',*,*,#8862,.F.);
#12293=ORIENTED_EDGE('',*,*,#8863,.F.);
#12294=ORIENTED_EDGE('',*,*,#8864,.F.);
#12295=ORIENTED_EDGE('',*,*,#8510,.F.);
#12296=ORIENTED_EDGE('',*,*,#8859,.T.);
#12297=ORIENTED_EDGE('',*,*,#8844,.T.);
#12298=ORIENTED_EDGE('',*,*,#8691,.F.);
#12299=ORIENTED_EDGE('',*,*,#8858,.T.);
#12300=ORIENTED_EDGE('',*,*,#8865,.T.);
#12301=ORIENTED_EDGE('',*,*,#8845,.T.);
#12302=ORIENTED_EDGE('',*,*,#8865,.F.);
#12303=ORIENTED_EDGE('',*,*,#8857,.T.);
#12304=ORIENTED_EDGE('',*,*,#8866,.T.);
#12305=ORIENTED_EDGE('',*,*,#8846,.T.);
#12306=ORIENTED_EDGE('',*,*,#8866,.F.);
#12307=ORIENTED_EDGE('',*,*,#8856,.T.);
#12308=ORIENTED_EDGE('',*,*,#8867,.T.);
#12309=ORIENTED_EDGE('',*,*,#8847,.T.);
#12310=ORIENTED_EDGE('',*,*,#8867,.F.);
#12311=ORIENTED_EDGE('',*,*,#8855,.T.);
#12312=ORIENTED_EDGE('',*,*,#8868,.T.);
#12313=ORIENTED_EDGE('',*,*,#8848,.T.);
#12314=ORIENTED_EDGE('',*,*,#8868,.F.);
#12315=ORIENTED_EDGE('',*,*,#8854,.T.);
#12316=ORIENTED_EDGE('',*,*,#8507,.T.);
#12317=ORIENTED_EDGE('',*,*,#8686,.F.);
#12318=ORIENTED_EDGE('',*,*,#8869,.F.);
#12319=ORIENTED_EDGE('',*,*,#8512,.F.);
#12320=ORIENTED_EDGE('',*,*,#8870,.F.);
#12321=ORIENTED_EDGE('',*,*,#8871,.F.);
#12322=ORIENTED_EDGE('',*,*,#8872,.F.);
#12323=ORIENTED_EDGE('',*,*,#8873,.F.);
#12324=ORIENTED_EDGE('',*,*,#8874,.F.);
#12325=ORIENTED_EDGE('',*,*,#8685,.F.);
#12326=ORIENTED_EDGE('',*,*,#8875,.F.);
#12327=ORIENTED_EDGE('',*,*,#8513,.F.);
#12328=ORIENTED_EDGE('',*,*,#8869,.T.);
#12329=ORIENTED_EDGE('',*,*,#8684,.F.);
#12330=ORIENTED_EDGE('',*,*,#8876,.F.);
#12331=ORIENTED_EDGE('',*,*,#8877,.F.);
#12332=ORIENTED_EDGE('',*,*,#8878,.F.);
#12333=ORIENTED_EDGE('',*,*,#8879,.F.);
#12334=ORIENTED_EDGE('',*,*,#8880,.F.);
#12335=ORIENTED_EDGE('',*,*,#8514,.F.);
#12336=ORIENTED_EDGE('',*,*,#8875,.T.);
#12337=ORIENTED_EDGE('',*,*,#8860,.T.);
#12338=ORIENTED_EDGE('',*,*,#8687,.F.);
#12339=ORIENTED_EDGE('',*,*,#8874,.T.);
#12340=ORIENTED_EDGE('',*,*,#8881,.T.);
#12341=ORIENTED_EDGE('',*,*,#8861,.T.);
#12342=ORIENTED_EDGE('',*,*,#8881,.F.);
#12343=ORIENTED_EDGE('',*,*,#8873,.T.);
#12344=ORIENTED_EDGE('',*,*,#8882,.T.);
#12345=ORIENTED_EDGE('',*,*,#8862,.T.);
#12346=ORIENTED_EDGE('',*,*,#8882,.F.);
#12347=ORIENTED_EDGE('',*,*,#8872,.T.);
#12348=ORIENTED_EDGE('',*,*,#8883,.T.);
#12349=ORIENTED_EDGE('',*,*,#8863,.T.);
#12350=ORIENTED_EDGE('',*,*,#8883,.F.);
#12351=ORIENTED_EDGE('',*,*,#8871,.T.);
#12352=ORIENTED_EDGE('',*,*,#8884,.T.);
#12353=ORIENTED_EDGE('',*,*,#8864,.T.);
#12354=ORIENTED_EDGE('',*,*,#8884,.F.);
#12355=ORIENTED_EDGE('',*,*,#8870,.T.);
#12356=ORIENTED_EDGE('',*,*,#8511,.T.);
#12357=ORIENTED_EDGE('',*,*,#8682,.F.);
#12358=ORIENTED_EDGE('',*,*,#8885,.F.);
#12359=ORIENTED_EDGE('',*,*,#8516,.F.);
#12360=ORIENTED_EDGE('',*,*,#8886,.F.);
#12361=ORIENTED_EDGE('',*,*,#8887,.F.);
#12362=ORIENTED_EDGE('',*,*,#8888,.F.);
#12363=ORIENTED_EDGE('',*,*,#8889,.F.);
#12364=ORIENTED_EDGE('',*,*,#8890,.F.);
#12365=ORIENTED_EDGE('',*,*,#8681,.F.);
#12366=ORIENTED_EDGE('',*,*,#8891,.F.);
#12367=ORIENTED_EDGE('',*,*,#8517,.F.);
#12368=ORIENTED_EDGE('',*,*,#8885,.T.);
#12369=ORIENTED_EDGE('',*,*,#8680,.F.);
#12370=ORIENTED_EDGE('',*,*,#8892,.F.);
#12371=ORIENTED_EDGE('',*,*,#8893,.F.);
#12372=ORIENTED_EDGE('',*,*,#8894,.F.);
#12373=ORIENTED_EDGE('',*,*,#8895,.F.);
#12374=ORIENTED_EDGE('',*,*,#8896,.F.);
#12375=ORIENTED_EDGE('',*,*,#8518,.F.);
#12376=ORIENTED_EDGE('',*,*,#8891,.T.);
#12377=ORIENTED_EDGE('',*,*,#8876,.T.);
#12378=ORIENTED_EDGE('',*,*,#8683,.F.);
#12379=ORIENTED_EDGE('',*,*,#8890,.T.);
#12380=ORIENTED_EDGE('',*,*,#8897,.T.);
#12381=ORIENTED_EDGE('',*,*,#8877,.T.);
#12382=ORIENTED_EDGE('',*,*,#8897,.F.);
#12383=ORIENTED_EDGE('',*,*,#8889,.T.);
#12384=ORIENTED_EDGE('',*,*,#8898,.T.);
#12385=ORIENTED_EDGE('',*,*,#8878,.T.);
#12386=ORIENTED_EDGE('',*,*,#8898,.F.);
#12387=ORIENTED_EDGE('',*,*,#8888,.T.);
#12388=ORIENTED_EDGE('',*,*,#8899,.T.);
#12389=ORIENTED_EDGE('',*,*,#8879,.T.);
#12390=ORIENTED_EDGE('',*,*,#8899,.F.);
#12391=ORIENTED_EDGE('',*,*,#8887,.T.);
#12392=ORIENTED_EDGE('',*,*,#8900,.T.);
#12393=ORIENTED_EDGE('',*,*,#8880,.T.);
#12394=ORIENTED_EDGE('',*,*,#8900,.F.);
#12395=ORIENTED_EDGE('',*,*,#8886,.T.);
#12396=ORIENTED_EDGE('',*,*,#8515,.T.);
#12397=ORIENTED_EDGE('',*,*,#8678,.F.);
#12398=ORIENTED_EDGE('',*,*,#8901,.F.);
#12399=ORIENTED_EDGE('',*,*,#8520,.F.);
#12400=ORIENTED_EDGE('',*,*,#8902,.F.);
#12401=ORIENTED_EDGE('',*,*,#8903,.F.);
#12402=ORIENTED_EDGE('',*,*,#8904,.F.);
#12403=ORIENTED_EDGE('',*,*,#8905,.F.);
#12404=ORIENTED_EDGE('',*,*,#8906,.F.);
#12405=ORIENTED_EDGE('',*,*,#8677,.F.);
#12406=ORIENTED_EDGE('',*,*,#8907,.F.);
#12407=ORIENTED_EDGE('',*,*,#8521,.F.);
#12408=ORIENTED_EDGE('',*,*,#8901,.T.);
#12409=ORIENTED_EDGE('',*,*,#8676,.F.);
#12410=ORIENTED_EDGE('',*,*,#8908,.F.);
#12411=ORIENTED_EDGE('',*,*,#8909,.F.);
#12412=ORIENTED_EDGE('',*,*,#8910,.F.);
#12413=ORIENTED_EDGE('',*,*,#8911,.F.);
#12414=ORIENTED_EDGE('',*,*,#8912,.F.);
#12415=ORIENTED_EDGE('',*,*,#8522,.F.);
#12416=ORIENTED_EDGE('',*,*,#8907,.T.);
#12417=ORIENTED_EDGE('',*,*,#8892,.T.);
#12418=ORIENTED_EDGE('',*,*,#8679,.F.);
#12419=ORIENTED_EDGE('',*,*,#8906,.T.);
#12420=ORIENTED_EDGE('',*,*,#8913,.T.);
#12421=ORIENTED_EDGE('',*,*,#8893,.T.);
#12422=ORIENTED_EDGE('',*,*,#8913,.F.);
#12423=ORIENTED_EDGE('',*,*,#8905,.T.);
#12424=ORIENTED_EDGE('',*,*,#8914,.T.);
#12425=ORIENTED_EDGE('',*,*,#8894,.T.);
#12426=ORIENTED_EDGE('',*,*,#8914,.F.);
#12427=ORIENTED_EDGE('',*,*,#8904,.T.);
#12428=ORIENTED_EDGE('',*,*,#8915,.T.);
#12429=ORIENTED_EDGE('',*,*,#8895,.T.);
#12430=ORIENTED_EDGE('',*,*,#8915,.F.);
#12431=ORIENTED_EDGE('',*,*,#8903,.T.);
#12432=ORIENTED_EDGE('',*,*,#8916,.T.);
#12433=ORIENTED_EDGE('',*,*,#8896,.T.);
#12434=ORIENTED_EDGE('',*,*,#8916,.F.);
#12435=ORIENTED_EDGE('',*,*,#8902,.T.);
#12436=ORIENTED_EDGE('',*,*,#8519,.T.);
#12437=ORIENTED_EDGE('',*,*,#8674,.F.);
#12438=ORIENTED_EDGE('',*,*,#8917,.F.);
#12439=ORIENTED_EDGE('',*,*,#8524,.F.);
#12440=ORIENTED_EDGE('',*,*,#8918,.F.);
#12441=ORIENTED_EDGE('',*,*,#8919,.F.);
#12442=ORIENTED_EDGE('',*,*,#8920,.F.);
#12443=ORIENTED_EDGE('',*,*,#8921,.F.);
#12444=ORIENTED_EDGE('',*,*,#8922,.F.);
#12445=ORIENTED_EDGE('',*,*,#8673,.F.);
#12446=ORIENTED_EDGE('',*,*,#8923,.F.);
#12447=ORIENTED_EDGE('',*,*,#8525,.F.);
#12448=ORIENTED_EDGE('',*,*,#8917,.T.);
#12449=ORIENTED_EDGE('',*,*,#8672,.F.);
#12450=ORIENTED_EDGE('',*,*,#8924,.F.);
#12451=ORIENTED_EDGE('',*,*,#8925,.F.);
#12452=ORIENTED_EDGE('',*,*,#8926,.F.);
#12453=ORIENTED_EDGE('',*,*,#8927,.F.);
#12454=ORIENTED_EDGE('',*,*,#8928,.F.);
#12455=ORIENTED_EDGE('',*,*,#8526,.F.);
#12456=ORIENTED_EDGE('',*,*,#8923,.T.);
#12457=ORIENTED_EDGE('',*,*,#8908,.T.);
#12458=ORIENTED_EDGE('',*,*,#8675,.F.);
#12459=ORIENTED_EDGE('',*,*,#8922,.T.);
#12460=ORIENTED_EDGE('',*,*,#8929,.T.);
#12461=ORIENTED_EDGE('',*,*,#8909,.T.);
#12462=ORIENTED_EDGE('',*,*,#8929,.F.);
#12463=ORIENTED_EDGE('',*,*,#8921,.T.);
#12464=ORIENTED_EDGE('',*,*,#8930,.T.);
#12465=ORIENTED_EDGE('',*,*,#8910,.T.);
#12466=ORIENTED_EDGE('',*,*,#8930,.F.);
#12467=ORIENTED_EDGE('',*,*,#8920,.T.);
#12468=ORIENTED_EDGE('',*,*,#8931,.T.);
#12469=ORIENTED_EDGE('',*,*,#8911,.T.);
#12470=ORIENTED_EDGE('',*,*,#8931,.F.);
#12471=ORIENTED_EDGE('',*,*,#8919,.T.);
#12472=ORIENTED_EDGE('',*,*,#8932,.T.);
#12473=ORIENTED_EDGE('',*,*,#8912,.T.);
#12474=ORIENTED_EDGE('',*,*,#8932,.F.);
#12475=ORIENTED_EDGE('',*,*,#8918,.T.);
#12476=ORIENTED_EDGE('',*,*,#8523,.T.);
#12477=ORIENTED_EDGE('',*,*,#8670,.F.);
#12478=ORIENTED_EDGE('',*,*,#8933,.F.);
#12479=ORIENTED_EDGE('',*,*,#8528,.F.);
#12480=ORIENTED_EDGE('',*,*,#8934,.F.);
#12481=ORIENTED_EDGE('',*,*,#8935,.F.);
#12482=ORIENTED_EDGE('',*,*,#8936,.F.);
#12483=ORIENTED_EDGE('',*,*,#8937,.F.);
#12484=ORIENTED_EDGE('',*,*,#8938,.F.);
#12485=ORIENTED_EDGE('',*,*,#8669,.F.);
#12486=ORIENTED_EDGE('',*,*,#8939,.F.);
#12487=ORIENTED_EDGE('',*,*,#8529,.F.);
#12488=ORIENTED_EDGE('',*,*,#8933,.T.);
#12489=ORIENTED_EDGE('',*,*,#8668,.F.);
#12490=ORIENTED_EDGE('',*,*,#8940,.F.);
#12491=ORIENTED_EDGE('',*,*,#8941,.F.);
#12492=ORIENTED_EDGE('',*,*,#8942,.F.);
#12493=ORIENTED_EDGE('',*,*,#8943,.F.);
#12494=ORIENTED_EDGE('',*,*,#8944,.F.);
#12495=ORIENTED_EDGE('',*,*,#8530,.F.);
#12496=ORIENTED_EDGE('',*,*,#8939,.T.);
#12497=ORIENTED_EDGE('',*,*,#8924,.T.);
#12498=ORIENTED_EDGE('',*,*,#8671,.F.);
#12499=ORIENTED_EDGE('',*,*,#8938,.T.);
#12500=ORIENTED_EDGE('',*,*,#8945,.T.);
#12501=ORIENTED_EDGE('',*,*,#8925,.T.);
#12502=ORIENTED_EDGE('',*,*,#8945,.F.);
#12503=ORIENTED_EDGE('',*,*,#8937,.T.);
#12504=ORIENTED_EDGE('',*,*,#8946,.T.);
#12505=ORIENTED_EDGE('',*,*,#8926,.T.);
#12506=ORIENTED_EDGE('',*,*,#8946,.F.);
#12507=ORIENTED_EDGE('',*,*,#8936,.T.);
#12508=ORIENTED_EDGE('',*,*,#8947,.T.);
#12509=ORIENTED_EDGE('',*,*,#8927,.T.);
#12510=ORIENTED_EDGE('',*,*,#8947,.F.);
#12511=ORIENTED_EDGE('',*,*,#8935,.T.);
#12512=ORIENTED_EDGE('',*,*,#8948,.T.);
#12513=ORIENTED_EDGE('',*,*,#8928,.T.);
#12514=ORIENTED_EDGE('',*,*,#8948,.F.);
#12515=ORIENTED_EDGE('',*,*,#8934,.T.);
#12516=ORIENTED_EDGE('',*,*,#8527,.T.);
#12517=ORIENTED_EDGE('',*,*,#8666,.F.);
#12518=ORIENTED_EDGE('',*,*,#8949,.F.);
#12519=ORIENTED_EDGE('',*,*,#8532,.F.);
#12520=ORIENTED_EDGE('',*,*,#8950,.F.);
#12521=ORIENTED_EDGE('',*,*,#8951,.F.);
#12522=ORIENTED_EDGE('',*,*,#8952,.F.);
#12523=ORIENTED_EDGE('',*,*,#8953,.F.);
#12524=ORIENTED_EDGE('',*,*,#8954,.F.);
#12525=ORIENTED_EDGE('',*,*,#8665,.F.);
#12526=ORIENTED_EDGE('',*,*,#8955,.F.);
#12527=ORIENTED_EDGE('',*,*,#8533,.F.);
#12528=ORIENTED_EDGE('',*,*,#8949,.T.);
#12529=ORIENTED_EDGE('',*,*,#8664,.F.);
#12530=ORIENTED_EDGE('',*,*,#8956,.F.);
#12531=ORIENTED_EDGE('',*,*,#8957,.F.);
#12532=ORIENTED_EDGE('',*,*,#8958,.F.);
#12533=ORIENTED_EDGE('',*,*,#8959,.F.);
#12534=ORIENTED_EDGE('',*,*,#8960,.F.);
#12535=ORIENTED_EDGE('',*,*,#8534,.F.);
#12536=ORIENTED_EDGE('',*,*,#8955,.T.);
#12537=ORIENTED_EDGE('',*,*,#8940,.T.);
#12538=ORIENTED_EDGE('',*,*,#8667,.F.);
#12539=ORIENTED_EDGE('',*,*,#8954,.T.);
#12540=ORIENTED_EDGE('',*,*,#8961,.T.);
#12541=ORIENTED_EDGE('',*,*,#8941,.T.);
#12542=ORIENTED_EDGE('',*,*,#8961,.F.);
#12543=ORIENTED_EDGE('',*,*,#8953,.T.);
#12544=ORIENTED_EDGE('',*,*,#8962,.T.);
#12545=ORIENTED_EDGE('',*,*,#8942,.T.);
#12546=ORIENTED_EDGE('',*,*,#8962,.F.);
#12547=ORIENTED_EDGE('',*,*,#8952,.T.);
#12548=ORIENTED_EDGE('',*,*,#8963,.T.);
#12549=ORIENTED_EDGE('',*,*,#8943,.T.);
#12550=ORIENTED_EDGE('',*,*,#8963,.F.);
#12551=ORIENTED_EDGE('',*,*,#8951,.T.);
#12552=ORIENTED_EDGE('',*,*,#8964,.T.);
#12553=ORIENTED_EDGE('',*,*,#8944,.T.);
#12554=ORIENTED_EDGE('',*,*,#8964,.F.);
#12555=ORIENTED_EDGE('',*,*,#8950,.T.);
#12556=ORIENTED_EDGE('',*,*,#8531,.T.);
#12557=ORIENTED_EDGE('',*,*,#8662,.F.);
#12558=ORIENTED_EDGE('',*,*,#8965,.F.);
#12559=ORIENTED_EDGE('',*,*,#8536,.F.);
#12560=ORIENTED_EDGE('',*,*,#8966,.F.);
#12561=ORIENTED_EDGE('',*,*,#8967,.F.);
#12562=ORIENTED_EDGE('',*,*,#8968,.F.);
#12563=ORIENTED_EDGE('',*,*,#8969,.F.);
#12564=ORIENTED_EDGE('',*,*,#8970,.F.);
#12565=ORIENTED_EDGE('',*,*,#8661,.F.);
#12566=ORIENTED_EDGE('',*,*,#8971,.F.);
#12567=ORIENTED_EDGE('',*,*,#8537,.F.);
#12568=ORIENTED_EDGE('',*,*,#8965,.T.);
#12569=ORIENTED_EDGE('',*,*,#8660,.F.);
#12570=ORIENTED_EDGE('',*,*,#8972,.F.);
#12571=ORIENTED_EDGE('',*,*,#8973,.F.);
#12572=ORIENTED_EDGE('',*,*,#8974,.F.);
#12573=ORIENTED_EDGE('',*,*,#8975,.F.);
#12574=ORIENTED_EDGE('',*,*,#8976,.F.);
#12575=ORIENTED_EDGE('',*,*,#8538,.F.);
#12576=ORIENTED_EDGE('',*,*,#8971,.T.);
#12577=ORIENTED_EDGE('',*,*,#8956,.T.);
#12578=ORIENTED_EDGE('',*,*,#8663,.F.);
#12579=ORIENTED_EDGE('',*,*,#8970,.T.);
#12580=ORIENTED_EDGE('',*,*,#8977,.T.);
#12581=ORIENTED_EDGE('',*,*,#8957,.T.);
#12582=ORIENTED_EDGE('',*,*,#8977,.F.);
#12583=ORIENTED_EDGE('',*,*,#8969,.T.);
#12584=ORIENTED_EDGE('',*,*,#8978,.T.);
#12585=ORIENTED_EDGE('',*,*,#8958,.T.);
#12586=ORIENTED_EDGE('',*,*,#8978,.F.);
#12587=ORIENTED_EDGE('',*,*,#8968,.T.);
#12588=ORIENTED_EDGE('',*,*,#8979,.T.);
#12589=ORIENTED_EDGE('',*,*,#8959,.T.);
#12590=ORIENTED_EDGE('',*,*,#8979,.F.);
#12591=ORIENTED_EDGE('',*,*,#8967,.T.);
#12592=ORIENTED_EDGE('',*,*,#8980,.T.);
#12593=ORIENTED_EDGE('',*,*,#8960,.T.);
#12594=ORIENTED_EDGE('',*,*,#8980,.F.);
#12595=ORIENTED_EDGE('',*,*,#8966,.T.);
#12596=ORIENTED_EDGE('',*,*,#8535,.T.);
#12597=ORIENTED_EDGE('',*,*,#8658,.F.);
#12598=ORIENTED_EDGE('',*,*,#8981,.F.);
#12599=ORIENTED_EDGE('',*,*,#8540,.F.);
#12600=ORIENTED_EDGE('',*,*,#8982,.F.);
#12601=ORIENTED_EDGE('',*,*,#8983,.F.);
#12602=ORIENTED_EDGE('',*,*,#8984,.F.);
#12603=ORIENTED_EDGE('',*,*,#8985,.F.);
#12604=ORIENTED_EDGE('',*,*,#8986,.F.);
#12605=ORIENTED_EDGE('',*,*,#8657,.F.);
#12606=ORIENTED_EDGE('',*,*,#8987,.F.);
#12607=ORIENTED_EDGE('',*,*,#8541,.F.);
#12608=ORIENTED_EDGE('',*,*,#8981,.T.);
#12609=ORIENTED_EDGE('',*,*,#8656,.F.);
#12610=ORIENTED_EDGE('',*,*,#8988,.F.);
#12611=ORIENTED_EDGE('',*,*,#8989,.F.);
#12612=ORIENTED_EDGE('',*,*,#8990,.F.);
#12613=ORIENTED_EDGE('',*,*,#8991,.F.);
#12614=ORIENTED_EDGE('',*,*,#8992,.F.);
#12615=ORIENTED_EDGE('',*,*,#8542,.F.);
#12616=ORIENTED_EDGE('',*,*,#8987,.T.);
#12617=ORIENTED_EDGE('',*,*,#8972,.T.);
#12618=ORIENTED_EDGE('',*,*,#8659,.F.);
#12619=ORIENTED_EDGE('',*,*,#8986,.T.);
#12620=ORIENTED_EDGE('',*,*,#8993,.T.);
#12621=ORIENTED_EDGE('',*,*,#8973,.T.);
#12622=ORIENTED_EDGE('',*,*,#8993,.F.);
#12623=ORIENTED_EDGE('',*,*,#8985,.T.);
#12624=ORIENTED_EDGE('',*,*,#8994,.T.);
#12625=ORIENTED_EDGE('',*,*,#8974,.T.);
#12626=ORIENTED_EDGE('',*,*,#8994,.F.);
#12627=ORIENTED_EDGE('',*,*,#8984,.T.);
#12628=ORIENTED_EDGE('',*,*,#8995,.T.);
#12629=ORIENTED_EDGE('',*,*,#8975,.T.);
#12630=ORIENTED_EDGE('',*,*,#8995,.F.);
#12631=ORIENTED_EDGE('',*,*,#8983,.T.);
#12632=ORIENTED_EDGE('',*,*,#8996,.T.);
#12633=ORIENTED_EDGE('',*,*,#8976,.T.);
#12634=ORIENTED_EDGE('',*,*,#8996,.F.);
#12635=ORIENTED_EDGE('',*,*,#8982,.T.);
#12636=ORIENTED_EDGE('',*,*,#8539,.T.);
#12637=ORIENTED_EDGE('',*,*,#8654,.F.);
#12638=ORIENTED_EDGE('',*,*,#8997,.F.);
#12639=ORIENTED_EDGE('',*,*,#8544,.F.);
#12640=ORIENTED_EDGE('',*,*,#8998,.F.);
#12641=ORIENTED_EDGE('',*,*,#8999,.F.);
#12642=ORIENTED_EDGE('',*,*,#9000,.F.);
#12643=ORIENTED_EDGE('',*,*,#9001,.F.);
#12644=ORIENTED_EDGE('',*,*,#9002,.F.);
#12645=ORIENTED_EDGE('',*,*,#8653,.F.);
#12646=ORIENTED_EDGE('',*,*,#9003,.F.);
#12647=ORIENTED_EDGE('',*,*,#8545,.F.);
#12648=ORIENTED_EDGE('',*,*,#8997,.T.);
#12649=ORIENTED_EDGE('',*,*,#8652,.F.);
#12650=ORIENTED_EDGE('',*,*,#9004,.F.);
#12651=ORIENTED_EDGE('',*,*,#9005,.F.);
#12652=ORIENTED_EDGE('',*,*,#9006,.F.);
#12653=ORIENTED_EDGE('',*,*,#9007,.F.);
#12654=ORIENTED_EDGE('',*,*,#9008,.F.);
#12655=ORIENTED_EDGE('',*,*,#8546,.F.);
#12656=ORIENTED_EDGE('',*,*,#9003,.T.);
#12657=ORIENTED_EDGE('',*,*,#8988,.T.);
#12658=ORIENTED_EDGE('',*,*,#8655,.F.);
#12659=ORIENTED_EDGE('',*,*,#9002,.T.);
#12660=ORIENTED_EDGE('',*,*,#9009,.T.);
#12661=ORIENTED_EDGE('',*,*,#8989,.T.);
#12662=ORIENTED_EDGE('',*,*,#9009,.F.);
#12663=ORIENTED_EDGE('',*,*,#9001,.T.);
#12664=ORIENTED_EDGE('',*,*,#9010,.T.);
#12665=ORIENTED_EDGE('',*,*,#8990,.T.);
#12666=ORIENTED_EDGE('',*,*,#9010,.F.);
#12667=ORIENTED_EDGE('',*,*,#9000,.T.);
#12668=ORIENTED_EDGE('',*,*,#9011,.T.);
#12669=ORIENTED_EDGE('',*,*,#8991,.T.);
#12670=ORIENTED_EDGE('',*,*,#9011,.F.);
#12671=ORIENTED_EDGE('',*,*,#8999,.T.);
#12672=ORIENTED_EDGE('',*,*,#9012,.T.);
#12673=ORIENTED_EDGE('',*,*,#8992,.T.);
#12674=ORIENTED_EDGE('',*,*,#9012,.F.);
#12675=ORIENTED_EDGE('',*,*,#8998,.T.);
#12676=ORIENTED_EDGE('',*,*,#8543,.T.);
#12677=ORIENTED_EDGE('',*,*,#8650,.F.);
#12678=ORIENTED_EDGE('',*,*,#9013,.F.);
#12679=ORIENTED_EDGE('',*,*,#8548,.F.);
#12680=ORIENTED_EDGE('',*,*,#9014,.F.);
#12681=ORIENTED_EDGE('',*,*,#9015,.F.);
#12682=ORIENTED_EDGE('',*,*,#9016,.F.);
#12683=ORIENTED_EDGE('',*,*,#9017,.F.);
#12684=ORIENTED_EDGE('',*,*,#9018,.F.);
#12685=ORIENTED_EDGE('',*,*,#8649,.F.);
#12686=ORIENTED_EDGE('',*,*,#9019,.F.);
#12687=ORIENTED_EDGE('',*,*,#8549,.F.);
#12688=ORIENTED_EDGE('',*,*,#9013,.T.);
#12689=ORIENTED_EDGE('',*,*,#8648,.F.);
#12690=ORIENTED_EDGE('',*,*,#9020,.F.);
#12691=ORIENTED_EDGE('',*,*,#9021,.F.);
#12692=ORIENTED_EDGE('',*,*,#9022,.F.);
#12693=ORIENTED_EDGE('',*,*,#9023,.F.);
#12694=ORIENTED_EDGE('',*,*,#9024,.F.);
#12695=ORIENTED_EDGE('',*,*,#8550,.F.);
#12696=ORIENTED_EDGE('',*,*,#9019,.T.);
#12697=ORIENTED_EDGE('',*,*,#9004,.T.);
#12698=ORIENTED_EDGE('',*,*,#8651,.F.);
#12699=ORIENTED_EDGE('',*,*,#9018,.T.);
#12700=ORIENTED_EDGE('',*,*,#9025,.T.);
#12701=ORIENTED_EDGE('',*,*,#9005,.T.);
#12702=ORIENTED_EDGE('',*,*,#9025,.F.);
#12703=ORIENTED_EDGE('',*,*,#9017,.T.);
#12704=ORIENTED_EDGE('',*,*,#9026,.T.);
#12705=ORIENTED_EDGE('',*,*,#9006,.T.);
#12706=ORIENTED_EDGE('',*,*,#9026,.F.);
#12707=ORIENTED_EDGE('',*,*,#9016,.T.);
#12708=ORIENTED_EDGE('',*,*,#9027,.T.);
#12709=ORIENTED_EDGE('',*,*,#9007,.T.);
#12710=ORIENTED_EDGE('',*,*,#9027,.F.);
#12711=ORIENTED_EDGE('',*,*,#9015,.T.);
#12712=ORIENTED_EDGE('',*,*,#9028,.T.);
#12713=ORIENTED_EDGE('',*,*,#9008,.T.);
#12714=ORIENTED_EDGE('',*,*,#9028,.F.);
#12715=ORIENTED_EDGE('',*,*,#9014,.T.);
#12716=ORIENTED_EDGE('',*,*,#8547,.T.);
#12717=ORIENTED_EDGE('',*,*,#8646,.F.);
#12718=ORIENTED_EDGE('',*,*,#9029,.F.);
#12719=ORIENTED_EDGE('',*,*,#8552,.F.);
#12720=ORIENTED_EDGE('',*,*,#9030,.F.);
#12721=ORIENTED_EDGE('',*,*,#9031,.F.);
#12722=ORIENTED_EDGE('',*,*,#9032,.F.);
#12723=ORIENTED_EDGE('',*,*,#9033,.F.);
#12724=ORIENTED_EDGE('',*,*,#9034,.F.);
#12725=ORIENTED_EDGE('',*,*,#8645,.F.);
#12726=ORIENTED_EDGE('',*,*,#9035,.F.);
#12727=ORIENTED_EDGE('',*,*,#8553,.F.);
#12728=ORIENTED_EDGE('',*,*,#9029,.T.);
#12729=ORIENTED_EDGE('',*,*,#8644,.F.);
#12730=ORIENTED_EDGE('',*,*,#9036,.F.);
#12731=ORIENTED_EDGE('',*,*,#9037,.F.);
#12732=ORIENTED_EDGE('',*,*,#9038,.F.);
#12733=ORIENTED_EDGE('',*,*,#9039,.F.);
#12734=ORIENTED_EDGE('',*,*,#9040,.F.);
#12735=ORIENTED_EDGE('',*,*,#8554,.F.);
#12736=ORIENTED_EDGE('',*,*,#9035,.T.);
#12737=ORIENTED_EDGE('',*,*,#9020,.T.);
#12738=ORIENTED_EDGE('',*,*,#8647,.F.);
#12739=ORIENTED_EDGE('',*,*,#9034,.T.);
#12740=ORIENTED_EDGE('',*,*,#9041,.T.);
#12741=ORIENTED_EDGE('',*,*,#9021,.T.);
#12742=ORIENTED_EDGE('',*,*,#9041,.F.);
#12743=ORIENTED_EDGE('',*,*,#9033,.T.);
#12744=ORIENTED_EDGE('',*,*,#9042,.T.);
#12745=ORIENTED_EDGE('',*,*,#9022,.T.);
#12746=ORIENTED_EDGE('',*,*,#9042,.F.);
#12747=ORIENTED_EDGE('',*,*,#9032,.T.);
#12748=ORIENTED_EDGE('',*,*,#9043,.T.);
#12749=ORIENTED_EDGE('',*,*,#9023,.T.);
#12750=ORIENTED_EDGE('',*,*,#9043,.F.);
#12751=ORIENTED_EDGE('',*,*,#9031,.T.);
#12752=ORIENTED_EDGE('',*,*,#9044,.T.);
#12753=ORIENTED_EDGE('',*,*,#9024,.T.);
#12754=ORIENTED_EDGE('',*,*,#9044,.F.);
#12755=ORIENTED_EDGE('',*,*,#9030,.T.);
#12756=ORIENTED_EDGE('',*,*,#8551,.T.);
#12757=ORIENTED_EDGE('',*,*,#8642,.F.);
#12758=ORIENTED_EDGE('',*,*,#9045,.F.);
#12759=ORIENTED_EDGE('',*,*,#8556,.F.);
#12760=ORIENTED_EDGE('',*,*,#9046,.F.);
#12761=ORIENTED_EDGE('',*,*,#9047,.F.);
#12762=ORIENTED_EDGE('',*,*,#9048,.F.);
#12763=ORIENTED_EDGE('',*,*,#9049,.F.);
#12764=ORIENTED_EDGE('',*,*,#9050,.F.);
#12765=ORIENTED_EDGE('',*,*,#8641,.F.);
#12766=ORIENTED_EDGE('',*,*,#9051,.F.);
#12767=ORIENTED_EDGE('',*,*,#8557,.F.);
#12768=ORIENTED_EDGE('',*,*,#9045,.T.);
#12769=ORIENTED_EDGE('',*,*,#8640,.F.);
#12770=ORIENTED_EDGE('',*,*,#9052,.F.);
#12771=ORIENTED_EDGE('',*,*,#9053,.F.);
#12772=ORIENTED_EDGE('',*,*,#9054,.F.);
#12773=ORIENTED_EDGE('',*,*,#9055,.F.);
#12774=ORIENTED_EDGE('',*,*,#9056,.F.);
#12775=ORIENTED_EDGE('',*,*,#8558,.F.);
#12776=ORIENTED_EDGE('',*,*,#9051,.T.);
#12777=ORIENTED_EDGE('',*,*,#9036,.T.);
#12778=ORIENTED_EDGE('',*,*,#8643,.F.);
#12779=ORIENTED_EDGE('',*,*,#9050,.T.);
#12780=ORIENTED_EDGE('',*,*,#9057,.T.);
#12781=ORIENTED_EDGE('',*,*,#9037,.T.);
#12782=ORIENTED_EDGE('',*,*,#9057,.F.);
#12783=ORIENTED_EDGE('',*,*,#9049,.T.);
#12784=ORIENTED_EDGE('',*,*,#9058,.T.);
#12785=ORIENTED_EDGE('',*,*,#9038,.T.);
#12786=ORIENTED_EDGE('',*,*,#9058,.F.);
#12787=ORIENTED_EDGE('',*,*,#9048,.T.);
#12788=ORIENTED_EDGE('',*,*,#9059,.T.);
#12789=ORIENTED_EDGE('',*,*,#9039,.T.);
#12790=ORIENTED_EDGE('',*,*,#9059,.F.);
#12791=ORIENTED_EDGE('',*,*,#9047,.T.);
#12792=ORIENTED_EDGE('',*,*,#9060,.T.);
#12793=ORIENTED_EDGE('',*,*,#9040,.T.);
#12794=ORIENTED_EDGE('',*,*,#9060,.F.);
#12795=ORIENTED_EDGE('',*,*,#9046,.T.);
#12796=ORIENTED_EDGE('',*,*,#8555,.T.);
#12797=ORIENTED_EDGE('',*,*,#8638,.F.);
#12798=ORIENTED_EDGE('',*,*,#9061,.F.);
#12799=ORIENTED_EDGE('',*,*,#8560,.F.);
#12800=ORIENTED_EDGE('',*,*,#9062,.F.);
#12801=ORIENTED_EDGE('',*,*,#9063,.F.);
#12802=ORIENTED_EDGE('',*,*,#9064,.F.);
#12803=ORIENTED_EDGE('',*,*,#9065,.F.);
#12804=ORIENTED_EDGE('',*,*,#9066,.F.);
#12805=ORIENTED_EDGE('',*,*,#8637,.F.);
#12806=ORIENTED_EDGE('',*,*,#9067,.F.);
#12807=ORIENTED_EDGE('',*,*,#8561,.F.);
#12808=ORIENTED_EDGE('',*,*,#9061,.T.);
#12809=ORIENTED_EDGE('',*,*,#8636,.F.);
#12810=ORIENTED_EDGE('',*,*,#9068,.F.);
#12811=ORIENTED_EDGE('',*,*,#9069,.F.);
#12812=ORIENTED_EDGE('',*,*,#9070,.F.);
#12813=ORIENTED_EDGE('',*,*,#9071,.F.);
#12814=ORIENTED_EDGE('',*,*,#9072,.F.);
#12815=ORIENTED_EDGE('',*,*,#8562,.F.);
#12816=ORIENTED_EDGE('',*,*,#9067,.T.);
#12817=ORIENTED_EDGE('',*,*,#9052,.T.);
#12818=ORIENTED_EDGE('',*,*,#8639,.F.);
#12819=ORIENTED_EDGE('',*,*,#9066,.T.);
#12820=ORIENTED_EDGE('',*,*,#9073,.T.);
#12821=ORIENTED_EDGE('',*,*,#9053,.T.);
#12822=ORIENTED_EDGE('',*,*,#9073,.F.);
#12823=ORIENTED_EDGE('',*,*,#9065,.T.);
#12824=ORIENTED_EDGE('',*,*,#9074,.T.);
#12825=ORIENTED_EDGE('',*,*,#9054,.T.);
#12826=ORIENTED_EDGE('',*,*,#9074,.F.);
#12827=ORIENTED_EDGE('',*,*,#9064,.T.);
#12828=ORIENTED_EDGE('',*,*,#9075,.T.);
#12829=ORIENTED_EDGE('',*,*,#9055,.T.);
#12830=ORIENTED_EDGE('',*,*,#9075,.F.);
#12831=ORIENTED_EDGE('',*,*,#9063,.T.);
#12832=ORIENTED_EDGE('',*,*,#9076,.T.);
#12833=ORIENTED_EDGE('',*,*,#9056,.T.);
#12834=ORIENTED_EDGE('',*,*,#9076,.F.);
#12835=ORIENTED_EDGE('',*,*,#9062,.T.);
#12836=ORIENTED_EDGE('',*,*,#8559,.T.);
#12837=ORIENTED_EDGE('',*,*,#8634,.F.);
#12838=ORIENTED_EDGE('',*,*,#9077,.F.);
#12839=ORIENTED_EDGE('',*,*,#8564,.F.);
#12840=ORIENTED_EDGE('',*,*,#9078,.F.);
#12841=ORIENTED_EDGE('',*,*,#9079,.F.);
#12842=ORIENTED_EDGE('',*,*,#9080,.F.);
#12843=ORIENTED_EDGE('',*,*,#9081,.F.);
#12844=ORIENTED_EDGE('',*,*,#9082,.F.);
#12845=ORIENTED_EDGE('',*,*,#8633,.F.);
#12846=ORIENTED_EDGE('',*,*,#9083,.F.);
#12847=ORIENTED_EDGE('',*,*,#8565,.F.);
#12848=ORIENTED_EDGE('',*,*,#9077,.T.);
#12849=ORIENTED_EDGE('',*,*,#8632,.F.);
#12850=ORIENTED_EDGE('',*,*,#9084,.F.);
#12851=ORIENTED_EDGE('',*,*,#9085,.F.);
#12852=ORIENTED_EDGE('',*,*,#9086,.F.);
#12853=ORIENTED_EDGE('',*,*,#9087,.F.);
#12854=ORIENTED_EDGE('',*,*,#9088,.F.);
#12855=ORIENTED_EDGE('',*,*,#8566,.F.);
#12856=ORIENTED_EDGE('',*,*,#9083,.T.);
#12857=ORIENTED_EDGE('',*,*,#9068,.T.);
#12858=ORIENTED_EDGE('',*,*,#8635,.F.);
#12859=ORIENTED_EDGE('',*,*,#9082,.T.);
#12860=ORIENTED_EDGE('',*,*,#9089,.T.);
#12861=ORIENTED_EDGE('',*,*,#9069,.T.);
#12862=ORIENTED_EDGE('',*,*,#9089,.F.);
#12863=ORIENTED_EDGE('',*,*,#9081,.T.);
#12864=ORIENTED_EDGE('',*,*,#9090,.T.);
#12865=ORIENTED_EDGE('',*,*,#9070,.T.);
#12866=ORIENTED_EDGE('',*,*,#9090,.F.);
#12867=ORIENTED_EDGE('',*,*,#9080,.T.);
#12868=ORIENTED_EDGE('',*,*,#9091,.T.);
#12869=ORIENTED_EDGE('',*,*,#9071,.T.);
#12870=ORIENTED_EDGE('',*,*,#9091,.F.);
#12871=ORIENTED_EDGE('',*,*,#9079,.T.);
#12872=ORIENTED_EDGE('',*,*,#9092,.T.);
#12873=ORIENTED_EDGE('',*,*,#9072,.T.);
#12874=ORIENTED_EDGE('',*,*,#9092,.F.);
#12875=ORIENTED_EDGE('',*,*,#9078,.T.);
#12876=ORIENTED_EDGE('',*,*,#8563,.T.);
#12877=ORIENTED_EDGE('',*,*,#8630,.F.);
#12878=ORIENTED_EDGE('',*,*,#9093,.F.);
#12879=ORIENTED_EDGE('',*,*,#8568,.F.);
#12880=ORIENTED_EDGE('',*,*,#9094,.F.);
#12881=ORIENTED_EDGE('',*,*,#9095,.F.);
#12882=ORIENTED_EDGE('',*,*,#9096,.F.);
#12883=ORIENTED_EDGE('',*,*,#9097,.F.);
#12884=ORIENTED_EDGE('',*,*,#9098,.F.);
#12885=ORIENTED_EDGE('',*,*,#8629,.F.);
#12886=ORIENTED_EDGE('',*,*,#9099,.F.);
#12887=ORIENTED_EDGE('',*,*,#8569,.F.);
#12888=ORIENTED_EDGE('',*,*,#9093,.T.);
#12889=ORIENTED_EDGE('',*,*,#8628,.F.);
#12890=ORIENTED_EDGE('',*,*,#9100,.F.);
#12891=ORIENTED_EDGE('',*,*,#9101,.F.);
#12892=ORIENTED_EDGE('',*,*,#9102,.F.);
#12893=ORIENTED_EDGE('',*,*,#9103,.F.);
#12894=ORIENTED_EDGE('',*,*,#9104,.F.);
#12895=ORIENTED_EDGE('',*,*,#8570,.F.);
#12896=ORIENTED_EDGE('',*,*,#9099,.T.);
#12897=ORIENTED_EDGE('',*,*,#9084,.T.);
#12898=ORIENTED_EDGE('',*,*,#8631,.F.);
#12899=ORIENTED_EDGE('',*,*,#9098,.T.);
#12900=ORIENTED_EDGE('',*,*,#9105,.T.);
#12901=ORIENTED_EDGE('',*,*,#9085,.T.);
#12902=ORIENTED_EDGE('',*,*,#9105,.F.);
#12903=ORIENTED_EDGE('',*,*,#9097,.T.);
#12904=ORIENTED_EDGE('',*,*,#9106,.T.);
#12905=ORIENTED_EDGE('',*,*,#9086,.T.);
#12906=ORIENTED_EDGE('',*,*,#9106,.F.);
#12907=ORIENTED_EDGE('',*,*,#9096,.T.);
#12908=ORIENTED_EDGE('',*,*,#9107,.T.);
#12909=ORIENTED_EDGE('',*,*,#9087,.T.);
#12910=ORIENTED_EDGE('',*,*,#9107,.F.);
#12911=ORIENTED_EDGE('',*,*,#9095,.T.);
#12912=ORIENTED_EDGE('',*,*,#9108,.T.);
#12913=ORIENTED_EDGE('',*,*,#9088,.T.);
#12914=ORIENTED_EDGE('',*,*,#9108,.F.);
#12915=ORIENTED_EDGE('',*,*,#9094,.T.);
#12916=ORIENTED_EDGE('',*,*,#8567,.T.);
#12917=ORIENTED_EDGE('',*,*,#8626,.F.);
#12918=ORIENTED_EDGE('',*,*,#9109,.F.);
#12919=ORIENTED_EDGE('',*,*,#8572,.F.);
#12920=ORIENTED_EDGE('',*,*,#9110,.F.);
#12921=ORIENTED_EDGE('',*,*,#9111,.F.);
#12922=ORIENTED_EDGE('',*,*,#9112,.F.);
#12923=ORIENTED_EDGE('',*,*,#9113,.F.);
#12924=ORIENTED_EDGE('',*,*,#9114,.F.);
#12925=ORIENTED_EDGE('',*,*,#8625,.F.);
#12926=ORIENTED_EDGE('',*,*,#9115,.F.);
#12927=ORIENTED_EDGE('',*,*,#8573,.F.);
#12928=ORIENTED_EDGE('',*,*,#9109,.T.);
#12929=ORIENTED_EDGE('',*,*,#8624,.F.);
#12930=ORIENTED_EDGE('',*,*,#9116,.F.);
#12931=ORIENTED_EDGE('',*,*,#9117,.F.);
#12932=ORIENTED_EDGE('',*,*,#9118,.F.);
#12933=ORIENTED_EDGE('',*,*,#9119,.F.);
#12934=ORIENTED_EDGE('',*,*,#9120,.F.);
#12935=ORIENTED_EDGE('',*,*,#8574,.F.);
#12936=ORIENTED_EDGE('',*,*,#9115,.T.);
#12937=ORIENTED_EDGE('',*,*,#9100,.T.);
#12938=ORIENTED_EDGE('',*,*,#8627,.F.);
#12939=ORIENTED_EDGE('',*,*,#9114,.T.);
#12940=ORIENTED_EDGE('',*,*,#9121,.T.);
#12941=ORIENTED_EDGE('',*,*,#9101,.T.);
#12942=ORIENTED_EDGE('',*,*,#9121,.F.);
#12943=ORIENTED_EDGE('',*,*,#9113,.T.);
#12944=ORIENTED_EDGE('',*,*,#9122,.T.);
#12945=ORIENTED_EDGE('',*,*,#9102,.T.);
#12946=ORIENTED_EDGE('',*,*,#9122,.F.);
#12947=ORIENTED_EDGE('',*,*,#9112,.T.);
#12948=ORIENTED_EDGE('',*,*,#9123,.T.);
#12949=ORIENTED_EDGE('',*,*,#9103,.T.);
#12950=ORIENTED_EDGE('',*,*,#9123,.F.);
#12951=ORIENTED_EDGE('',*,*,#9111,.T.);
#12952=ORIENTED_EDGE('',*,*,#9124,.T.);
#12953=ORIENTED_EDGE('',*,*,#9104,.T.);
#12954=ORIENTED_EDGE('',*,*,#9124,.F.);
#12955=ORIENTED_EDGE('',*,*,#9110,.T.);
#12956=ORIENTED_EDGE('',*,*,#8571,.T.);
#12957=ORIENTED_EDGE('',*,*,#8622,.F.);
#12958=ORIENTED_EDGE('',*,*,#9125,.F.);
#12959=ORIENTED_EDGE('',*,*,#8576,.F.);
#12960=ORIENTED_EDGE('',*,*,#9126,.F.);
#12961=ORIENTED_EDGE('',*,*,#9127,.F.);
#12962=ORIENTED_EDGE('',*,*,#9128,.F.);
#12963=ORIENTED_EDGE('',*,*,#9129,.F.);
#12964=ORIENTED_EDGE('',*,*,#9130,.F.);
#12965=ORIENTED_EDGE('',*,*,#8621,.F.);
#12966=ORIENTED_EDGE('',*,*,#9131,.F.);
#12967=ORIENTED_EDGE('',*,*,#8577,.F.);
#12968=ORIENTED_EDGE('',*,*,#9125,.T.);
#12969=ORIENTED_EDGE('',*,*,#8620,.F.);
#12970=ORIENTED_EDGE('',*,*,#9132,.F.);
#12971=ORIENTED_EDGE('',*,*,#9133,.F.);
#12972=ORIENTED_EDGE('',*,*,#9134,.F.);
#12973=ORIENTED_EDGE('',*,*,#9135,.F.);
#12974=ORIENTED_EDGE('',*,*,#9136,.F.);
#12975=ORIENTED_EDGE('',*,*,#8578,.F.);
#12976=ORIENTED_EDGE('',*,*,#9131,.T.);
#12977=ORIENTED_EDGE('',*,*,#9116,.T.);
#12978=ORIENTED_EDGE('',*,*,#8623,.F.);
#12979=ORIENTED_EDGE('',*,*,#9130,.T.);
#12980=ORIENTED_EDGE('',*,*,#9137,.T.);
#12981=ORIENTED_EDGE('',*,*,#9117,.T.);
#12982=ORIENTED_EDGE('',*,*,#9137,.F.);
#12983=ORIENTED_EDGE('',*,*,#9129,.T.);
#12984=ORIENTED_EDGE('',*,*,#9138,.T.);
#12985=ORIENTED_EDGE('',*,*,#9118,.T.);
#12986=ORIENTED_EDGE('',*,*,#9138,.F.);
#12987=ORIENTED_EDGE('',*,*,#9128,.T.);
#12988=ORIENTED_EDGE('',*,*,#9139,.T.);
#12989=ORIENTED_EDGE('',*,*,#9119,.T.);
#12990=ORIENTED_EDGE('',*,*,#9139,.F.);
#12991=ORIENTED_EDGE('',*,*,#9127,.T.);
#12992=ORIENTED_EDGE('',*,*,#9140,.T.);
#12993=ORIENTED_EDGE('',*,*,#9120,.T.);
#12994=ORIENTED_EDGE('',*,*,#9140,.F.);
#12995=ORIENTED_EDGE('',*,*,#9126,.T.);
#12996=ORIENTED_EDGE('',*,*,#8575,.T.);
#12997=ORIENTED_EDGE('',*,*,#8618,.F.);
#12998=ORIENTED_EDGE('',*,*,#9141,.F.);
#12999=ORIENTED_EDGE('',*,*,#8580,.F.);
#13000=ORIENTED_EDGE('',*,*,#9142,.F.);
#13001=ORIENTED_EDGE('',*,*,#9143,.F.);
#13002=ORIENTED_EDGE('',*,*,#9144,.F.);
#13003=ORIENTED_EDGE('',*,*,#9145,.F.);
#13004=ORIENTED_EDGE('',*,*,#9146,.F.);
#13005=ORIENTED_EDGE('',*,*,#8617,.F.);
#13006=ORIENTED_EDGE('',*,*,#9147,.F.);
#13007=ORIENTED_EDGE('',*,*,#8581,.F.);
#13008=ORIENTED_EDGE('',*,*,#9141,.T.);
#13009=ORIENTED_EDGE('',*,*,#8616,.F.);
#13010=ORIENTED_EDGE('',*,*,#9148,.F.);
#13011=ORIENTED_EDGE('',*,*,#9149,.F.);
#13012=ORIENTED_EDGE('',*,*,#9150,.F.);
#13013=ORIENTED_EDGE('',*,*,#9151,.F.);
#13014=ORIENTED_EDGE('',*,*,#9152,.F.);
#13015=ORIENTED_EDGE('',*,*,#8582,.F.);
#13016=ORIENTED_EDGE('',*,*,#9147,.T.);
#13017=ORIENTED_EDGE('',*,*,#9132,.T.);
#13018=ORIENTED_EDGE('',*,*,#8619,.F.);
#13019=ORIENTED_EDGE('',*,*,#9146,.T.);
#13020=ORIENTED_EDGE('',*,*,#9153,.T.);
#13021=ORIENTED_EDGE('',*,*,#9133,.T.);
#13022=ORIENTED_EDGE('',*,*,#9153,.F.);
#13023=ORIENTED_EDGE('',*,*,#9145,.T.);
#13024=ORIENTED_EDGE('',*,*,#9154,.T.);
#13025=ORIENTED_EDGE('',*,*,#9134,.T.);
#13026=ORIENTED_EDGE('',*,*,#9154,.F.);
#13027=ORIENTED_EDGE('',*,*,#9144,.T.);
#13028=ORIENTED_EDGE('',*,*,#9155,.T.);
#13029=ORIENTED_EDGE('',*,*,#9135,.T.);
#13030=ORIENTED_EDGE('',*,*,#9155,.F.);
#13031=ORIENTED_EDGE('',*,*,#9143,.T.);
#13032=ORIENTED_EDGE('',*,*,#9156,.T.);
#13033=ORIENTED_EDGE('',*,*,#9136,.T.);
#13034=ORIENTED_EDGE('',*,*,#9156,.F.);
#13035=ORIENTED_EDGE('',*,*,#9142,.T.);
#13036=ORIENTED_EDGE('',*,*,#8579,.T.);
#13037=ORIENTED_EDGE('',*,*,#8614,.F.);
#13038=ORIENTED_EDGE('',*,*,#9157,.F.);
#13039=ORIENTED_EDGE('',*,*,#8584,.F.);
#13040=ORIENTED_EDGE('',*,*,#9158,.F.);
#13041=ORIENTED_EDGE('',*,*,#9159,.F.);
#13042=ORIENTED_EDGE('',*,*,#9160,.F.);
#13043=ORIENTED_EDGE('',*,*,#9161,.F.);
#13044=ORIENTED_EDGE('',*,*,#9162,.F.);
#13045=ORIENTED_EDGE('',*,*,#8613,.F.);
#13046=ORIENTED_EDGE('',*,*,#9163,.F.);
#13047=ORIENTED_EDGE('',*,*,#8585,.F.);
#13048=ORIENTED_EDGE('',*,*,#9157,.T.);
#13049=ORIENTED_EDGE('',*,*,#8612,.F.);
#13050=ORIENTED_EDGE('',*,*,#9164,.F.);
#13051=ORIENTED_EDGE('',*,*,#9165,.F.);
#13052=ORIENTED_EDGE('',*,*,#9166,.F.);
#13053=ORIENTED_EDGE('',*,*,#9167,.F.);
#13054=ORIENTED_EDGE('',*,*,#9168,.F.);
#13055=ORIENTED_EDGE('',*,*,#8586,.F.);
#13056=ORIENTED_EDGE('',*,*,#9163,.T.);
#13057=ORIENTED_EDGE('',*,*,#9148,.T.);
#13058=ORIENTED_EDGE('',*,*,#8615,.F.);
#13059=ORIENTED_EDGE('',*,*,#9162,.T.);
#13060=ORIENTED_EDGE('',*,*,#9169,.T.);
#13061=ORIENTED_EDGE('',*,*,#9164,.T.);
#13062=ORIENTED_EDGE('',*,*,#8611,.F.);
#13063=ORIENTED_EDGE('',*,*,#9170,.T.);
#13064=ORIENTED_EDGE('',*,*,#9171,.T.);
#13065=ORIENTED_EDGE('',*,*,#9149,.T.);
#13066=ORIENTED_EDGE('',*,*,#9169,.F.);
#13067=ORIENTED_EDGE('',*,*,#9161,.T.);
#13068=ORIENTED_EDGE('',*,*,#9172,.T.);
#13069=ORIENTED_EDGE('',*,*,#9150,.T.);
#13070=ORIENTED_EDGE('',*,*,#9172,.F.);
#13071=ORIENTED_EDGE('',*,*,#9160,.T.);
#13072=ORIENTED_EDGE('',*,*,#9173,.T.);
#13073=ORIENTED_EDGE('',*,*,#9151,.T.);
#13074=ORIENTED_EDGE('',*,*,#9173,.F.);
#13075=ORIENTED_EDGE('',*,*,#9159,.T.);
#13076=ORIENTED_EDGE('',*,*,#9174,.T.);
#13077=ORIENTED_EDGE('',*,*,#9152,.T.);
#13078=ORIENTED_EDGE('',*,*,#9174,.F.);
#13079=ORIENTED_EDGE('',*,*,#9158,.T.);
#13080=ORIENTED_EDGE('',*,*,#8583,.T.);
#13081=ORIENTED_EDGE('',*,*,#8610,.F.);
#13082=ORIENTED_EDGE('',*,*,#9175,.F.);
#13083=ORIENTED_EDGE('',*,*,#8588,.F.);
#13084=ORIENTED_EDGE('',*,*,#9176,.F.);
#13085=ORIENTED_EDGE('',*,*,#9177,.F.);
#13086=ORIENTED_EDGE('',*,*,#9178,.F.);
#13087=ORIENTED_EDGE('',*,*,#9179,.F.);
#13088=ORIENTED_EDGE('',*,*,#9170,.F.);
#13089=ORIENTED_EDGE('',*,*,#8609,.F.);
#13090=ORIENTED_EDGE('',*,*,#9180,.F.);
#13091=ORIENTED_EDGE('',*,*,#8589,.F.);
#13092=ORIENTED_EDGE('',*,*,#9175,.T.);
#13093=ORIENTED_EDGE('',*,*,#8608,.F.);
#13094=ORIENTED_EDGE('',*,*,#9181,.F.);
#13095=ORIENTED_EDGE('',*,*,#9182,.F.);
#13096=ORIENTED_EDGE('',*,*,#9183,.F.);
#13097=ORIENTED_EDGE('',*,*,#9184,.F.);
#13098=ORIENTED_EDGE('',*,*,#9185,.F.);
#13099=ORIENTED_EDGE('',*,*,#8590,.F.);
#13100=ORIENTED_EDGE('',*,*,#9180,.T.);
#13101=ORIENTED_EDGE('',*,*,#9181,.T.);
#13102=ORIENTED_EDGE('',*,*,#8607,.F.);
#13103=ORIENTED_EDGE('',*,*,#9186,.T.);
#13104=ORIENTED_EDGE('',*,*,#9187,.T.);
#13105=ORIENTED_EDGE('',*,*,#9165,.T.);
#13106=ORIENTED_EDGE('',*,*,#9171,.F.);
#13107=ORIENTED_EDGE('',*,*,#9179,.T.);
#13108=ORIENTED_EDGE('',*,*,#9188,.T.);
#13109=ORIENTED_EDGE('',*,*,#9182,.T.);
#13110=ORIENTED_EDGE('',*,*,#9187,.F.);
#13111=ORIENTED_EDGE('',*,*,#9189,.T.);
#13112=ORIENTED_EDGE('',*,*,#9190,.T.);
#13113=ORIENTED_EDGE('',*,*,#9168,.T.);
#13114=ORIENTED_EDGE('',*,*,#9191,.F.);
#13115=ORIENTED_EDGE('',*,*,#9176,.T.);
#13116=ORIENTED_EDGE('',*,*,#8587,.T.);
#13117=ORIENTED_EDGE('',*,*,#9166,.T.);
#13118=ORIENTED_EDGE('',*,*,#9188,.F.);
#13119=ORIENTED_EDGE('',*,*,#9178,.T.);
#13120=ORIENTED_EDGE('',*,*,#9192,.T.);
#13121=ORIENTED_EDGE('',*,*,#9167,.T.);
#13122=ORIENTED_EDGE('',*,*,#9192,.F.);
#13123=ORIENTED_EDGE('',*,*,#9177,.T.);
#13124=ORIENTED_EDGE('',*,*,#9191,.T.);
#13125=ORIENTED_EDGE('',*,*,#8606,.F.);
#13126=ORIENTED_EDGE('',*,*,#9193,.F.);
#13127=ORIENTED_EDGE('',*,*,#8592,.F.);
#13128=ORIENTED_EDGE('',*,*,#9194,.F.);
#13129=ORIENTED_EDGE('',*,*,#9195,.F.);
#13130=ORIENTED_EDGE('',*,*,#9196,.F.);
#13131=ORIENTED_EDGE('',*,*,#9189,.F.);
#13132=ORIENTED_EDGE('',*,*,#9186,.F.);
#13133=ORIENTED_EDGE('',*,*,#8605,.F.);
#13134=ORIENTED_EDGE('',*,*,#9197,.F.);
#13135=ORIENTED_EDGE('',*,*,#8593,.F.);
#13136=ORIENTED_EDGE('',*,*,#9193,.T.);
#13137=ORIENTED_EDGE('',*,*,#8604,.F.);
#13138=ORIENTED_EDGE('',*,*,#8733,.F.);
#13139=ORIENTED_EDGE('',*,*,#8735,.F.);
#13140=ORIENTED_EDGE('',*,*,#8737,.F.);
#13141=ORIENTED_EDGE('',*,*,#8739,.F.);
#13142=ORIENTED_EDGE('',*,*,#8740,.F.);
#13143=ORIENTED_EDGE('',*,*,#8594,.F.);
#13144=ORIENTED_EDGE('',*,*,#9197,.T.);
#13145=ORIENTED_EDGE('',*,*,#9184,.T.);
#13146=ORIENTED_EDGE('',*,*,#9198,.F.);
#13147=ORIENTED_EDGE('',*,*,#9195,.T.);
#13148=ORIENTED_EDGE('',*,*,#9199,.T.);
#13149=ORIENTED_EDGE('',*,*,#9183,.T.);
#13150=ORIENTED_EDGE('',*,*,#9190,.F.);
#13151=ORIENTED_EDGE('',*,*,#9196,.T.);
#13152=ORIENTED_EDGE('',*,*,#9198,.T.);
#13153=ORIENTED_EDGE('',*,*,#9185,.T.);
#13154=ORIENTED_EDGE('',*,*,#9199,.F.);
#13155=ORIENTED_EDGE('',*,*,#9194,.T.);
#13156=ORIENTED_EDGE('',*,*,#8591,.T.);
#14654=PLANE('',#16485);
#14655=PLANE('',#16518);
#15124=ADVANCED_FACE('',(#2768),#1235,.F.);
#15125=ADVANCED_FACE('',(#2769),#1446,.F.);
#15126=ADVANCED_FACE('',(#2770,#1704),#14654,.T.);
#15127=ADVANCED_FACE('',(#2771),#1236,.F.);
#15128=ADVANCED_FACE('',(#2772,#1705),#14655,.T.);
#15129=ADVANCED_FACE('',(#2773),#164,.F.);
#15130=ADVANCED_FACE('',(#2774),#165,.F.);
#15131=ADVANCED_FACE('',(#2775),#166,.F.);
#15132=ADVANCED_FACE('',(#2776),#1237,.T.);
#15133=ADVANCED_FACE('',(#2777),#1447,.T.);
#15134=ADVANCED_FACE('',(#2778),#127,.F.);
#15135=ADVANCED_FACE('',(#2779),#1448,.T.);
#15136=ADVANCED_FACE('',(#2780),#1238,.T.);
#15137=ADVANCED_FACE('',(#2781),#167,.F.);
#15138=ADVANCED_FACE('',(#2782),#168,.F.);
#15139=ADVANCED_FACE('',(#2783),#169,.F.);
#15140=ADVANCED_FACE('',(#2784),#1239,.T.);
#15141=ADVANCED_FACE('',(#2785),#1449,.T.);
#15142=ADVANCED_FACE('',(#2786),#128,.F.);
#15143=ADVANCED_FACE('',(#2787),#1450,.T.);
#15144=ADVANCED_FACE('',(#2788),#1240,.T.);
#15145=ADVANCED_FACE('',(#2789),#170,.F.);
#15146=ADVANCED_FACE('',(#2790),#171,.F.);
#15147=ADVANCED_FACE('',(#2791),#172,.F.);
#15148=ADVANCED_FACE('',(#2792),#1241,.T.);
#15149=ADVANCED_FACE('',(#2793),#1451,.T.);
#15150=ADVANCED_FACE('',(#2794),#129,.F.);
#15151=ADVANCED_FACE('',(#2795),#1452,.T.);
#15152=ADVANCED_FACE('',(#2796),#1242,.T.);
#15153=ADVANCED_FACE('',(#2797),#173,.F.);
#15154=ADVANCED_FACE('',(#2798),#174,.F.);
#15155=ADVANCED_FACE('',(#2799),#175,.F.);
#15156=ADVANCED_FACE('',(#2800),#1243,.T.);
#15157=ADVANCED_FACE('',(#2801),#1453,.T.);
#15158=ADVANCED_FACE('',(#2802),#130,.F.);
#15159=ADVANCED_FACE('',(#2803),#1454,.T.);
#15160=ADVANCED_FACE('',(#2804),#1244,.T.);
#15161=ADVANCED_FACE('',(#2805),#176,.F.);
#15162=ADVANCED_FACE('',(#2806),#177,.F.);
#15163=ADVANCED_FACE('',(#2807),#178,.F.);
#15164=ADVANCED_FACE('',(#2808),#1245,.T.);
#15165=ADVANCED_FACE('',(#2809),#1455,.T.);
#15166=ADVANCED_FACE('',(#2810),#131,.F.);
#15167=ADVANCED_FACE('',(#2811),#1456,.T.);
#15168=ADVANCED_FACE('',(#2812),#1246,.T.);
#15169=ADVANCED_FACE('',(#2813),#179,.F.);
#15170=ADVANCED_FACE('',(#2814),#180,.F.);
#15171=ADVANCED_FACE('',(#2815),#181,.F.);
#15172=ADVANCED_FACE('',(#2816),#1247,.T.);
#15173=ADVANCED_FACE('',(#2817),#1457,.T.);
#15174=ADVANCED_FACE('',(#2818),#132,.F.);
#15175=ADVANCED_FACE('',(#2819),#1458,.T.);
#15176=ADVANCED_FACE('',(#2820),#1248,.T.);
#15177=ADVANCED_FACE('',(#2821),#182,.F.);
#15178=ADVANCED_FACE('',(#2822),#183,.F.);
#15179=ADVANCED_FACE('',(#2823),#184,.F.);
#15180=ADVANCED_FACE('',(#2824),#1249,.T.);
#15181=ADVANCED_FACE('',(#2825),#1459,.T.);
#15182=ADVANCED_FACE('',(#2826),#133,.F.);
#15183=ADVANCED_FACE('',(#2827),#1460,.T.);
#15184=ADVANCED_FACE('',(#2828),#1250,.T.);
#15185=ADVANCED_FACE('',(#2829),#185,.F.);
#15186=ADVANCED_FACE('',(#2830),#186,.F.);
#15187=ADVANCED_FACE('',(#2831),#187,.F.);
#15188=ADVANCED_FACE('',(#2832),#1251,.T.);
#15189=ADVANCED_FACE('',(#2833),#1461,.T.);
#15190=ADVANCED_FACE('',(#2834),#134,.F.);
#15191=ADVANCED_FACE('',(#2835),#1462,.T.);
#15192=ADVANCED_FACE('',(#2836),#1252,.T.);
#15193=ADVANCED_FACE('',(#2837),#188,.F.);
#15194=ADVANCED_FACE('',(#2838),#189,.F.);
#15195=ADVANCED_FACE('',(#2839),#190,.F.);
#15196=ADVANCED_FACE('',(#2840),#1253,.T.);
#15197=ADVANCED_FACE('',(#2841),#1463,.T.);
#15198=ADVANCED_FACE('',(#2842),#135,.F.);
#15199=ADVANCED_FACE('',(#2843),#1464,.T.);
#15200=ADVANCED_FACE('',(#2844),#1254,.T.);
#15201=ADVANCED_FACE('',(#2845),#191,.F.);
#15202=ADVANCED_FACE('',(#2846),#192,.F.);
#15203=ADVANCED_FACE('',(#2847),#193,.F.);
#15204=ADVANCED_FACE('',(#2848),#1255,.T.);
#15205=ADVANCED_FACE('',(#2849),#1465,.T.);
#15206=ADVANCED_FACE('',(#2850),#136,.F.);
#15207=ADVANCED_FACE('',(#2851),#1466,.T.);
#15208=ADVANCED_FACE('',(#2852),#1256,.T.);
#15209=ADVANCED_FACE('',(#2853),#194,.F.);
#15210=ADVANCED_FACE('',(#2854),#195,.F.);
#15211=ADVANCED_FACE('',(#2855),#196,.F.);
#15212=ADVANCED_FACE('',(#2856),#1257,.T.);
#15213=ADVANCED_FACE('',(#2857),#1467,.T.);
#15214=ADVANCED_FACE('',(#2858),#137,.F.);
#15215=ADVANCED_FACE('',(#2859),#1468,.T.);
#15216=ADVANCED_FACE('',(#2860),#1258,.T.);
#15217=ADVANCED_FACE('',(#2861),#197,.F.);
#15218=ADVANCED_FACE('',(#2862),#198,.F.);
#15219=ADVANCED_FACE('',(#2863),#199,.F.);
#15220=ADVANCED_FACE('',(#2864),#1259,.T.);
#15221=ADVANCED_FACE('',(#2865),#1469,.T.);
#15222=ADVANCED_FACE('',(#2866),#138,.F.);
#15223=ADVANCED_FACE('',(#2867),#1470,.T.);
#15224=ADVANCED_FACE('',(#2868),#1260,.T.);
#15225=ADVANCED_FACE('',(#2869),#200,.F.);
#15226=ADVANCED_FACE('',(#2870),#201,.F.);
#15227=ADVANCED_FACE('',(#2871),#202,.F.);
#15228=ADVANCED_FACE('',(#2872),#1261,.T.);
#15229=ADVANCED_FACE('',(#2873),#1471,.T.);
#15230=ADVANCED_FACE('',(#2874),#139,.F.);
#15231=ADVANCED_FACE('',(#2875),#1472,.T.);
#15232=ADVANCED_FACE('',(#2876),#1262,.T.);
#15233=ADVANCED_FACE('',(#2877),#203,.F.);
#15234=ADVANCED_FACE('',(#2878),#204,.F.);
#15235=ADVANCED_FACE('',(#2879),#205,.F.);
#15236=ADVANCED_FACE('',(#2880),#1263,.T.);
#15237=ADVANCED_FACE('',(#2881),#1473,.T.);
#15238=ADVANCED_FACE('',(#2882),#140,.F.);
#15239=ADVANCED_FACE('',(#2883),#1474,.T.);
#15240=ADVANCED_FACE('',(#2884),#1264,.T.);
#15241=ADVANCED_FACE('',(#2885),#206,.F.);
#15242=ADVANCED_FACE('',(#2886),#207,.F.);
#15243=ADVANCED_FACE('',(#2887),#208,.F.);
#15244=ADVANCED_FACE('',(#2888),#1265,.T.);
#15245=ADVANCED_FACE('',(#2889),#1475,.T.);
#15246=ADVANCED_FACE('',(#2890),#141,.F.);
#15247=ADVANCED_FACE('',(#2891),#1476,.T.);
#15248=ADVANCED_FACE('',(#2892),#1266,.T.);
#15249=ADVANCED_FACE('',(#2893),#209,.F.);
#15250=ADVANCED_FACE('',(#2894),#210,.F.);
#15251=ADVANCED_FACE('',(#2895),#211,.F.);
#15252=ADVANCED_FACE('',(#2896),#1267,.T.);
#15253=ADVANCED_FACE('',(#2897),#1477,.T.);
#15254=ADVANCED_FACE('',(#2898),#142,.F.);
#15255=ADVANCED_FACE('',(#2899),#1478,.T.);
#15256=ADVANCED_FACE('',(#2900),#1268,.T.);
#15257=ADVANCED_FACE('',(#2901),#212,.F.);
#15258=ADVANCED_FACE('',(#2902),#213,.F.);
#15259=ADVANCED_FACE('',(#2903),#214,.F.);
#15260=ADVANCED_FACE('',(#2904),#1269,.T.);
#15261=ADVANCED_FACE('',(#2905),#1479,.T.);
#15262=ADVANCED_FACE('',(#2906),#143,.F.);
#15263=ADVANCED_FACE('',(#2907),#1480,.T.);
#15264=ADVANCED_FACE('',(#2908),#1270,.T.);
#15265=ADVANCED_FACE('',(#2909),#215,.F.);
#15266=ADVANCED_FACE('',(#2910),#216,.F.);
#15267=ADVANCED_FACE('',(#2911),#217,.F.);
#15268=ADVANCED_FACE('',(#2912),#1271,.T.);
#15269=ADVANCED_FACE('',(#2913),#1481,.T.);
#15270=ADVANCED_FACE('',(#2914),#144,.F.);
#15271=ADVANCED_FACE('',(#2915),#1482,.T.);
#15272=ADVANCED_FACE('',(#2916),#1272,.T.);
#15273=ADVANCED_FACE('',(#2917),#218,.F.);
#15274=ADVANCED_FACE('',(#2918),#219,.F.);
#15275=ADVANCED_FACE('',(#2919),#220,.F.);
#15276=ADVANCED_FACE('',(#2920),#1273,.T.);
#15277=ADVANCED_FACE('',(#2921),#1483,.T.);
#15278=ADVANCED_FACE('',(#2922),#145,.F.);
#15279=ADVANCED_FACE('',(#2923),#1484,.T.);
#15280=ADVANCED_FACE('',(#2924),#1274,.T.);
#15281=ADVANCED_FACE('',(#2925),#221,.F.);
#15282=ADVANCED_FACE('',(#2926),#222,.F.);
#15283=ADVANCED_FACE('',(#2927),#223,.F.);
#15284=ADVANCED_FACE('',(#2928),#1275,.T.);
#15285=ADVANCED_FACE('',(#2929),#1485,.T.);
#15286=ADVANCED_FACE('',(#2930),#146,.F.);
#15287=ADVANCED_FACE('',(#2931),#1486,.T.);
#15288=ADVANCED_FACE('',(#2932),#1276,.T.);
#15289=ADVANCED_FACE('',(#2933),#224,.F.);
#15290=ADVANCED_FACE('',(#2934),#225,.F.);
#15291=ADVANCED_FACE('',(#2935),#226,.F.);
#15292=ADVANCED_FACE('',(#2936),#1277,.T.);
#15293=ADVANCED_FACE('',(#2937),#1487,.T.);
#15294=ADVANCED_FACE('',(#2938),#147,.F.);
#15295=ADVANCED_FACE('',(#2939),#1488,.T.);
#15296=ADVANCED_FACE('',(#2940),#1278,.T.);
#15297=ADVANCED_FACE('',(#2941),#227,.F.);
#15298=ADVANCED_FACE('',(#2942),#228,.F.);
#15299=ADVANCED_FACE('',(#2943),#229,.F.);
#15300=ADVANCED_FACE('',(#2944),#1279,.T.);
#15301=ADVANCED_FACE('',(#2945),#1489,.T.);
#15302=ADVANCED_FACE('',(#2946),#148,.F.);
#15303=ADVANCED_FACE('',(#2947),#1490,.T.);
#15304=ADVANCED_FACE('',(#2948),#1280,.T.);
#15305=ADVANCED_FACE('',(#2949),#230,.F.);
#15306=ADVANCED_FACE('',(#2950),#231,.F.);
#15307=ADVANCED_FACE('',(#2951),#232,.F.);
#15308=ADVANCED_FACE('',(#2952),#1281,.T.);
#15309=ADVANCED_FACE('',(#2953),#1491,.T.);
#15310=ADVANCED_FACE('',(#2954),#149,.F.);
#15311=ADVANCED_FACE('',(#2955),#1492,.T.);
#15312=ADVANCED_FACE('',(#2956),#1282,.T.);
#15313=ADVANCED_FACE('',(#2957),#233,.F.);
#15314=ADVANCED_FACE('',(#2958),#234,.F.);
#15315=ADVANCED_FACE('',(#2959),#235,.F.);
#15316=ADVANCED_FACE('',(#2960),#1283,.T.);
#15317=ADVANCED_FACE('',(#2961),#1493,.T.);
#15318=ADVANCED_FACE('',(#2962),#150,.F.);
#15319=ADVANCED_FACE('',(#2963),#1494,.T.);
#15320=ADVANCED_FACE('',(#2964),#1284,.T.);
#15321=ADVANCED_FACE('',(#2965),#236,.F.);
#15322=ADVANCED_FACE('',(#2966),#237,.F.);
#15323=ADVANCED_FACE('',(#2967),#238,.F.);
#15324=ADVANCED_FACE('',(#2968),#1285,.T.);
#15325=ADVANCED_FACE('',(#2969),#1495,.T.);
#15326=ADVANCED_FACE('',(#2970),#151,.F.);
#15327=ADVANCED_FACE('',(#2971),#1496,.T.);
#15328=ADVANCED_FACE('',(#2972),#1286,.T.);
#15329=ADVANCED_FACE('',(#2973),#239,.F.);
#15330=ADVANCED_FACE('',(#2974),#240,.F.);
#15331=ADVANCED_FACE('',(#2975),#241,.F.);
#15332=ADVANCED_FACE('',(#2976),#1287,.T.);
#15333=ADVANCED_FACE('',(#2977),#1497,.T.);
#15334=ADVANCED_FACE('',(#2978),#152,.F.);
#15335=ADVANCED_FACE('',(#2979),#1498,.T.);
#15336=ADVANCED_FACE('',(#2980),#1288,.T.);
#15337=ADVANCED_FACE('',(#2981),#242,.F.);
#15338=ADVANCED_FACE('',(#2982),#243,.F.);
#15339=ADVANCED_FACE('',(#2983),#244,.F.);
#15340=ADVANCED_FACE('',(#2984),#1289,.T.);
#15341=ADVANCED_FACE('',(#2985),#1499,.T.);
#15342=ADVANCED_FACE('',(#2986),#153,.F.);
#15343=ADVANCED_FACE('',(#2987),#1500,.T.);
#15344=ADVANCED_FACE('',(#2988),#1290,.T.);
#15345=ADVANCED_FACE('',(#2989),#245,.F.);
#15346=ADVANCED_FACE('',(#2990),#246,.F.);
#15347=ADVANCED_FACE('',(#2991),#247,.F.);
#15348=ADVANCED_FACE('',(#2992),#1291,.T.);
#15349=ADVANCED_FACE('',(#2993),#1292,.T.);
#15350=ADVANCED_FACE('',(#2994),#1501,.T.);
#15351=ADVANCED_FACE('',(#2995),#154,.F.);
#15352=ADVANCED_FACE('',(#2996),#1502,.T.);
#15353=ADVANCED_FACE('',(#2997),#1293,.T.);
#15354=ADVANCED_FACE('',(#2998),#248,.F.);
#15355=ADVANCED_FACE('',(#2999),#249,.F.);
#15356=ADVANCED_FACE('',(#3000),#250,.F.);
#15357=ADVANCED_FACE('',(#3001),#1294,.T.);
#15358=ADVANCED_FACE('',(#3002),#1503,.T.);
#15359=ADVANCED_FACE('',(#3003),#1504,.T.);
#15360=ADVANCED_FACE('',(#3004),#1295,.T.);
#15361=ADVANCED_FACE('',(#3005),#155,.F.);
#15362=ADVANCED_FACE('',(#3006),#1505,.T.);
#15363=ADVANCED_FACE('',(#3007),#251,.F.);
#15364=ADVANCED_FACE('',(#3008),#252,.F.);
#15365=ADVANCED_FACE('',(#3009),#253,.F.);
#15366=ADVANCED_FACE('',(#3010),#1506,.T.);
#15367=ADVANCED_FACE('',(#3011),#156,.F.);
#15368=ADVANCED_FACE('',(#3012),#1296,.T.);
#15617=CLOSED_SHELL('',(#15124,#15125,#15126,#15127,#15128,#15129,#15130,
#15131,#15132,#15133,#15134,#15135,#15136,#15137,#15138,#15139,#15140,#15141,
#15142,#15143,#15144,#15145,#15146,#15147,#15148,#15149,#15150,#15151,#15152,
#15153,#15154,#15155,#15156,#15157,#15158,#15159,#15160,#15161,#15162,#15163,
#15164,#15165,#15166,#15167,#15168,#15169,#15170,#15171,#15172,#15173,#15174,
#15175,#15176,#15177,#15178,#15179,#15180,#15181,#15182,#15183,#15184,#15185,
#15186,#15187,#15188,#15189,#15190,#15191,#15192,#15193,#15194,#15195,#15196,
#15197,#15198,#15199,#15200,#15201,#15202,#15203,#15204,#15205,#15206,#15207,
#15208,#15209,#15210,#15211,#15212,#15213,#15214,#15215,#15216,#15217,#15218,
#15219,#15220,#15221,#15222,#15223,#15224,#15225,#15226,#15227,#15228,#15229,
#15230,#15231,#15232,#15233,#15234,#15235,#15236,#15237,#15238,#15239,#15240,
#15241,#15242,#15243,#15244,#15245,#15246,#15247,#15248,#15249,#15250,#15251,
#15252,#15253,#15254,#15255,#15256,#15257,#15258,#15259,#15260,#15261,#15262,
#15263,#15264,#15265,#15266,#15267,#15268,#15269,#15270,#15271,#15272,#15273,
#15274,#15275,#15276,#15277,#15278,#15279,#15280,#15281,#15282,#15283,#15284,
#15285,#15286,#15287,#15288,#15289,#15290,#15291,#15292,#15293,#15294,#15295,
#15296,#15297,#15298,#15299,#15300,#15301,#15302,#15303,#15304,#15305,#15306,
#15307,#15308,#15309,#15310,#15311,#15312,#15313,#15314,#15315,#15316,#15317,
#15318,#15319,#15320,#15321,#15322,#15323,#15324,#15325,#15326,#15327,#15328,
#15329,#15330,#15331,#15332,#15333,#15334,#15335,#15336,#15337,#15338,#15339,
#15340,#15341,#15342,#15343,#15344,#15345,#15346,#15347,#15348,#15349,#15350,
#15351,#15352,#15353,#15354,#15355,#15356,#15357,#15358,#15359,#15360,#15361,
#15362,#15363,#15364,#15365,#15366,#15367,#15368));
#16477=AXIS2_PLACEMENT_3D('',#26810,#19185,#19186);
#16478=AXIS2_PLACEMENT_3D('',#26811,#19187,#19188);
#16479=AXIS2_PLACEMENT_3D('',#26814,#19189,#19190);
#16480=AXIS2_PLACEMENT_3D('',#26817,#19192,#19193);
#16481=AXIS2_PLACEMENT_3D('',#26818,#19194,#19195);
#16482=AXIS2_PLACEMENT_3D('',#26819,#19196,#19197);
#16483=AXIS2_PLACEMENT_3D('',#26823,#19199,#19200);
#16484=AXIS2_PLACEMENT_3D('',#26824,#19201,#19202);
#16485=AXIS2_PLACEMENT_3D('',#26825,#19203,#19204);
#16486=AXIS2_PLACEMENT_3D('',#26848,#19205,#19206);
#16487=AXIS2_PLACEMENT_3D('',#26891,#19208,#19209);
#16488=AXIS2_PLACEMENT_3D('',#26937,#19211,#19212);
#16489=AXIS2_PLACEMENT_3D('',#26980,#19214,#19215);
#16490=AXIS2_PLACEMENT_3D('',#27026,#19217,#19218);
#16491=AXIS2_PLACEMENT_3D('',#27069,#19220,#19221);
#16492=AXIS2_PLACEMENT_3D('',#27112,#19223,#19224);
#16493=AXIS2_PLACEMENT_3D('',#27155,#19226,#19227);
#16494=AXIS2_PLACEMENT_3D('',#27195,#19229,#19230);
#16495=AXIS2_PLACEMENT_3D('',#27237,#19232,#19233);
#16496=AXIS2_PLACEMENT_3D('',#27276,#19235,#19236);
#16497=AXIS2_PLACEMENT_3D('',#27315,#19238,#19239);
#16498=AXIS2_PLACEMENT_3D('',#27356,#19241,#19242);
#16499=AXIS2_PLACEMENT_3D('',#27393,#19244,#19245);
#16500=AXIS2_PLACEMENT_3D('',#27429,#19247,#19248);
#16501=AXIS2_PLACEMENT_3D('',#27468,#19250,#19251);
#16502=AXIS2_PLACEMENT_3D('',#27506,#19253,#19254);
#16503=AXIS2_PLACEMENT_3D('',#27544,#19256,#19257);
#16504=AXIS2_PLACEMENT_3D('',#27605,#19259,#19260);
#16505=AXIS2_PLACEMENT_3D('',#27643,#19262,#19263);
#16506=AXIS2_PLACEMENT_3D('',#27683,#19265,#19266);
#16507=AXIS2_PLACEMENT_3D('',#27714,#19268,#19269);
#16508=AXIS2_PLACEMENT_3D('',#27758,#19271,#19272);
#16509=AXIS2_PLACEMENT_3D('',#27801,#19274,#19275);
#16510=AXIS2_PLACEMENT_3D('',#27848,#19277,#19278);
#16511=AXIS2_PLACEMENT_3D('',#27891,#19280,#19281);
#16512=AXIS2_PLACEMENT_3D('',#27937,#19283,#19284);
#16513=AXIS2_PLACEMENT_3D('',#27978,#19286,#19287);
#16514=AXIS2_PLACEMENT_3D('',#28021,#19289,#19290);
#16515=AXIS2_PLACEMENT_3D('',#28051,#19292,#19293);
#16516=AXIS2_PLACEMENT_3D('',#28112,#19295,#19296);
#16517=AXIS2_PLACEMENT_3D('',#28115,#19298,#19299);
#16518=AXIS2_PLACEMENT_3D('',#28116,#19300,#19301);
#16519=AXIS2_PLACEMENT_3D('',#28149,#19303,#19304);
#16520=AXIS2_PLACEMENT_3D('',#28191,#19306,#19307);
#16521=AXIS2_PLACEMENT_3D('',#28270,#19309,#19310);
#16522=AXIS2_PLACEMENT_3D('',#28300,#19312,#19313);
#16523=AXIS2_PLACEMENT_3D('',#28380,#19315,#19316);
#16524=AXIS2_PLACEMENT_3D('',#28411,#19318,#19319);
#16525=AXIS2_PLACEMENT_3D('',#28446,#19321,#19322);
#16526=AXIS2_PLACEMENT_3D('',#28517,#19324,#19325);
#16527=AXIS2_PLACEMENT_3D('',#28561,#19327,#19328);
#16528=AXIS2_PLACEMENT_3D('',#28601,#19330,#19331);
#16529=AXIS2_PLACEMENT_3D('',#28630,#19333,#19334);
#16530=AXIS2_PLACEMENT_3D('',#28659,#19336,#19337);
#16531=AXIS2_PLACEMENT_3D('',#28688,#19339,#19340);
#16532=AXIS2_PLACEMENT_3D('',#28717,#19342,#19343);
#16533=AXIS2_PLACEMENT_3D('',#28745,#19345,#19346);
#16534=AXIS2_PLACEMENT_3D('',#28806,#19348,#19349);
#16535=AXIS2_PLACEMENT_3D('',#28836,#19351,#19352);
#16536=AXIS2_PLACEMENT_3D('',#28863,#19354,#19355);
#16537=AXIS2_PLACEMENT_3D('',#28936,#19357,#19358);
#16538=AXIS2_PLACEMENT_3D('',#28999,#19360,#19361);
#16539=AXIS2_PLACEMENT_3D('',#29029,#19363,#19364);
#16540=AXIS2_PLACEMENT_3D('',#29060,#19366,#19367);
#16541=AXIS2_PLACEMENT_3D('',#29089,#19369,#19370);
#16542=AXIS2_PLACEMENT_3D('',#29120,#19372,#19373);
#16543=AXIS2_PLACEMENT_3D('',#29193,#19375,#19376);
#16544=AXIS2_PLACEMENT_3D('',#29266,#19378,#19379);
#16545=AXIS2_PLACEMENT_3D('',#29301,#19381,#19382);
#16546=AXIS2_PLACEMENT_3D('',#29333,#19384,#19385);
#16547=AXIS2_PLACEMENT_3D('',#29413,#19387,#19388);
#16548=AXIS2_PLACEMENT_3D('',#29445,#19390,#19391);
#16549=AXIS2_PLACEMENT_3D('',#30616,#19392,#19393);
#16550=AXIS2_PLACEMENT_3D('',#30618,#19394,#19395);
#16551=AXIS2_PLACEMENT_3D('',#30625,#19396,#19397);
#16552=AXIS2_PLACEMENT_3D('',#30627,#19398,#19399);
#16553=AXIS2_PLACEMENT_3D('',#30636,#19400,#19401);
#16554=AXIS2_PLACEMENT_3D('',#30638,#19402,#19403);
#16555=AXIS2_PLACEMENT_3D('',#30653,#19404,#19405);
#16556=AXIS2_PLACEMENT_3D('',#30655,#19406,#19407);
#16557=AXIS2_PLACEMENT_3D('',#30662,#19408,#19409);
#16558=AXIS2_PLACEMENT_3D('',#31931,#19410,#19411);
#16559=AXIS2_PLACEMENT_3D('',#31932,#19412,#19413);
#16560=AXIS2_PLACEMENT_3D('',#31933,#19414,#19415);
#16561=AXIS2_PLACEMENT_3D('',#31934,#19416,#19417);
#16562=AXIS2_PLACEMENT_3D('',#31935,#19418,#19419);
#16563=AXIS2_PLACEMENT_3D('',#31936,#19420,#19421);
#16564=AXIS2_PLACEMENT_3D('',#31937,#19422,#19423);
#16565=AXIS2_PLACEMENT_3D('',#31938,#19424,#19425);
#16566=AXIS2_PLACEMENT_3D('',#31939,#19426,#19427);
#16567=AXIS2_PLACEMENT_3D('',#33296,#19428,#19429);
#16568=AXIS2_PLACEMENT_3D('',#33297,#19430,#19431);
#16569=AXIS2_PLACEMENT_3D('',#33298,#19432,#19433);
#16570=AXIS2_PLACEMENT_3D('',#33299,#19434,#19435);
#16571=AXIS2_PLACEMENT_3D('',#33300,#19436,#19437);
#16572=AXIS2_PLACEMENT_3D('',#33301,#19438,#19439);
#16573=AXIS2_PLACEMENT_3D('',#33302,#19440,#19441);
#16574=AXIS2_PLACEMENT_3D('',#33303,#19442,#19443);
#16575=AXIS2_PLACEMENT_3D('',#33304,#19444,#19445);
#16576=AXIS2_PLACEMENT_3D('',#34487,#19446,#19447);
#16577=AXIS2_PLACEMENT_3D('',#34488,#19448,#19449);
#16578=AXIS2_PLACEMENT_3D('',#34489,#19450,#19451);
#16579=AXIS2_PLACEMENT_3D('',#34490,#19452,#19453);
#16580=AXIS2_PLACEMENT_3D('',#34491,#19454,#19455);
#16581=AXIS2_PLACEMENT_3D('',#34492,#19456,#19457);
#16582=AXIS2_PLACEMENT_3D('',#34493,#19458,#19459);
#16583=AXIS2_PLACEMENT_3D('',#34494,#19460,#19461);
#16584=AXIS2_PLACEMENT_3D('',#34495,#19462,#19463);
#16585=AXIS2_PLACEMENT_3D('',#35776,#19464,#19465);
#16586=AXIS2_PLACEMENT_3D('',#35777,#19466,#19467);
#16587=AXIS2_PLACEMENT_3D('',#35778,#19468,#19469);
#16588=AXIS2_PLACEMENT_3D('',#35779,#19470,#19471);
#16589=AXIS2_PLACEMENT_3D('',#35780,#19472,#19473);
#16590=AXIS2_PLACEMENT_3D('',#35781,#19474,#19475);
#16591=AXIS2_PLACEMENT_3D('',#35782,#19476,#19477);
#16592=AXIS2_PLACEMENT_3D('',#35783,#19478,#19479);
#16593=AXIS2_PLACEMENT_3D('',#35784,#19480,#19481);
#16594=AXIS2_PLACEMENT_3D('',#37059,#19482,#19483);
#16595=AXIS2_PLACEMENT_3D('',#37060,#19484,#19485);
#16596=AXIS2_PLACEMENT_3D('',#37061,#19486,#19487);
#16597=AXIS2_PLACEMENT_3D('',#37062,#19488,#19489);
#16598=AXIS2_PLACEMENT_3D('',#37063,#19490,#19491);
#16599=AXIS2_PLACEMENT_3D('',#37064,#19492,#19493);
#16600=AXIS2_PLACEMENT_3D('',#37065,#19494,#19495);
#16601=AXIS2_PLACEMENT_3D('',#37066,#19496,#19497);
#16602=AXIS2_PLACEMENT_3D('',#37067,#19498,#19499);
#16603=AXIS2_PLACEMENT_3D('',#38162,#19500,#19501);
#16604=AXIS2_PLACEMENT_3D('',#38163,#19502,#19503);
#16605=AXIS2_PLACEMENT_3D('',#38164,#19504,#19505);
#16606=AXIS2_PLACEMENT_3D('',#38165,#19506,#19507);
#16607=AXIS2_PLACEMENT_3D('',#38166,#19508,#19509);
#16608=AXIS2_PLACEMENT_3D('',#38167,#19510,#19511);
#16609=AXIS2_PLACEMENT_3D('',#38168,#19512,#19513);
#16610=AXIS2_PLACEMENT_3D('',#38169,#19514,#19515);
#16611=AXIS2_PLACEMENT_3D('',#38170,#19516,#19517);
#16612=AXIS2_PLACEMENT_3D('',#39239,#19518,#19519);
#16613=AXIS2_PLACEMENT_3D('',#39240,#19520,#19521);
#16614=AXIS2_PLACEMENT_3D('',#39241,#19522,#19523);
#16615=AXIS2_PLACEMENT_3D('',#39242,#19524,#19525);
#16616=AXIS2_PLACEMENT_3D('',#39243,#19526,#19527);
#16617=AXIS2_PLACEMENT_3D('',#39244,#19528,#19529);
#16618=AXIS2_PLACEMENT_3D('',#39245,#19530,#19531);
#16619=AXIS2_PLACEMENT_3D('',#39246,#19532,#19533);
#16620=AXIS2_PLACEMENT_3D('',#39247,#19534,#19535);
#16621=AXIS2_PLACEMENT_3D('',#40488,#19536,#19537);
#16622=AXIS2_PLACEMENT_3D('',#40489,#19538,#19539);
#16623=AXIS2_PLACEMENT_3D('',#40490,#19540,#19541);
#16624=AXIS2_PLACEMENT_3D('',#40491,#19542,#19543);
#16625=AXIS2_PLACEMENT_3D('',#40492,#19544,#19545);
#16626=AXIS2_PLACEMENT_3D('',#40493,#19546,#19547);
#16627=AXIS2_PLACEMENT_3D('',#40494,#19548,#19549);
#16628=AXIS2_PLACEMENT_3D('',#40495,#19550,#19551);
#16629=AXIS2_PLACEMENT_3D('',#40496,#19552,#19553);
#16630=AXIS2_PLACEMENT_3D('',#41589,#19554,#19555);
#16631=AXIS2_PLACEMENT_3D('',#41590,#19556,#19557);
#16632=AXIS2_PLACEMENT_3D('',#41591,#19558,#19559);
#16633=AXIS2_PLACEMENT_3D('',#41592,#19560,#19561);
#16634=AXIS2_PLACEMENT_3D('',#41593,#19562,#19563);
#16635=AXIS2_PLACEMENT_3D('',#41594,#19564,#19565);
#16636=AXIS2_PLACEMENT_3D('',#41595,#19566,#19567);
#16637=AXIS2_PLACEMENT_3D('',#41596,#19568,#19569);
#16638=AXIS2_PLACEMENT_3D('',#41597,#19570,#19571);
#16639=AXIS2_PLACEMENT_3D('',#42550,#19572,#19573);
#16640=AXIS2_PLACEMENT_3D('',#42551,#19574,#19575);
#16641=AXIS2_PLACEMENT_3D('',#42552,#19576,#19577);
#16642=AXIS2_PLACEMENT_3D('',#42553,#19578,#19579);
#16643=AXIS2_PLACEMENT_3D('',#42554,#19580,#19581);
#16644=AXIS2_PLACEMENT_3D('',#42555,#19582,#19583);
#16645=AXIS2_PLACEMENT_3D('',#42556,#19584,#19585);
#16646=AXIS2_PLACEMENT_3D('',#42557,#19586,#19587);
#16647=AXIS2_PLACEMENT_3D('',#42558,#19588,#19589);
#16648=AXIS2_PLACEMENT_3D('',#43585,#19590,#19591);
#16649=AXIS2_PLACEMENT_3D('',#43586,#19592,#19593);
#16650=AXIS2_PLACEMENT_3D('',#43587,#19594,#19595);
#16651=AXIS2_PLACEMENT_3D('',#43588,#19596,#19597);
#16652=AXIS2_PLACEMENT_3D('',#43589,#19598,#19599);
#16653=AXIS2_PLACEMENT_3D('',#43590,#19600,#19601);
#16654=AXIS2_PLACEMENT_3D('',#43591,#19602,#19603);
#16655=AXIS2_PLACEMENT_3D('',#43592,#19604,#19605);
#16656=AXIS2_PLACEMENT_3D('',#43593,#19606,#19607);
#16657=AXIS2_PLACEMENT_3D('',#44690,#19608,#19609);
#16658=AXIS2_PLACEMENT_3D('',#44691,#19610,#19611);
#16659=AXIS2_PLACEMENT_3D('',#44692,#19612,#19613);
#16660=AXIS2_PLACEMENT_3D('',#44693,#19614,#19615);
#16661=AXIS2_PLACEMENT_3D('',#44694,#19616,#19617);
#16662=AXIS2_PLACEMENT_3D('',#44695,#19618,#19619);
#16663=AXIS2_PLACEMENT_3D('',#44696,#19620,#19621);
#16664=AXIS2_PLACEMENT_3D('',#44697,#19622,#19623);
#16665=AXIS2_PLACEMENT_3D('',#44698,#19624,#19625);
#16666=AXIS2_PLACEMENT_3D('',#45633,#19626,#19627);
#16667=AXIS2_PLACEMENT_3D('',#45634,#19628,#19629);
#16668=AXIS2_PLACEMENT_3D('',#45635,#19630,#19631);
#16669=AXIS2_PLACEMENT_3D('',#45636,#19632,#19633);
#16670=AXIS2_PLACEMENT_3D('',#45637,#19634,#19635);
#16671=AXIS2_PLACEMENT_3D('',#45638,#19636,#19637);
#16672=AXIS2_PLACEMENT_3D('',#45639,#19638,#19639);
#16673=AXIS2_PLACEMENT_3D('',#45640,#19640,#19641);
#16674=AXIS2_PLACEMENT_3D('',#45641,#19642,#19643);
#16675=AXIS2_PLACEMENT_3D('',#46558,#19644,#19645);
#16676=AXIS2_PLACEMENT_3D('',#46559,#19646,#19647);
#16677=AXIS2_PLACEMENT_3D('',#46560,#19648,#19649);
#16678=AXIS2_PLACEMENT_3D('',#46561,#19650,#19651);
#16679=AXIS2_PLACEMENT_3D('',#46562,#19652,#19653);
#16680=AXIS2_PLACEMENT_3D('',#46563,#19654,#19655);
#16681=AXIS2_PLACEMENT_3D('',#46564,#19656,#19657);
#16682=AXIS2_PLACEMENT_3D('',#46565,#19658,#19659);
#16683=AXIS2_PLACEMENT_3D('',#46566,#19660,#19661);
#16684=AXIS2_PLACEMENT_3D('',#47583,#19662,#19663);
#16685=AXIS2_PLACEMENT_3D('',#47584,#19664,#19665);
#16686=AXIS2_PLACEMENT_3D('',#47585,#19666,#19667);
#16687=AXIS2_PLACEMENT_3D('',#47586,#19668,#19669);
#16688=AXIS2_PLACEMENT_3D('',#47587,#19670,#19671);
#16689=AXIS2_PLACEMENT_3D('',#47588,#19672,#19673);
#16690=AXIS2_PLACEMENT_3D('',#47589,#19674,#19675);
#16691=AXIS2_PLACEMENT_3D('',#47590,#19676,#19677);
#16692=AXIS2_PLACEMENT_3D('',#47591,#19678,#19679);
#16693=AXIS2_PLACEMENT_3D('',#48524,#19680,#19681);
#16694=AXIS2_PLACEMENT_3D('',#48525,#19682,#19683);
#16695=AXIS2_PLACEMENT_3D('',#48526,#19684,#19685);
#16696=AXIS2_PLACEMENT_3D('',#48527,#19686,#19687);
#16697=AXIS2_PLACEMENT_3D('',#48528,#19688,#19689);
#16698=AXIS2_PLACEMENT_3D('',#48529,#19690,#19691);
#16699=AXIS2_PLACEMENT_3D('',#48530,#19692,#19693);
#16700=AXIS2_PLACEMENT_3D('',#48531,#19694,#19695);
#16701=AXIS2_PLACEMENT_3D('',#48532,#19696,#19697);
#16702=AXIS2_PLACEMENT_3D('',#49577,#19698,#19699);
#16703=AXIS2_PLACEMENT_3D('',#49578,#19700,#19701);
#16704=AXIS2_PLACEMENT_3D('',#49579,#19702,#19703);
#16705=AXIS2_PLACEMENT_3D('',#49580,#19704,#19705);
#16706=AXIS2_PLACEMENT_3D('',#49581,#19706,#19707);
#16707=AXIS2_PLACEMENT_3D('',#49582,#19708,#19709);
#16708=AXIS2_PLACEMENT_3D('',#49583,#19710,#19711);
#16709=AXIS2_PLACEMENT_3D('',#49584,#19712,#19713);
#16710=AXIS2_PLACEMENT_3D('',#49585,#19714,#19715);
#16711=AXIS2_PLACEMENT_3D('',#50544,#19716,#19717);
#16712=AXIS2_PLACEMENT_3D('',#50545,#19718,#19719);
#16713=AXIS2_PLACEMENT_3D('',#50546,#19720,#19721);
#16714=AXIS2_PLACEMENT_3D('',#50547,#19722,#19723);
#16715=AXIS2_PLACEMENT_3D('',#50548,#19724,#19725);
#16716=AXIS2_PLACEMENT_3D('',#50549,#19726,#19727);
#16717=AXIS2_PLACEMENT_3D('',#50550,#19728,#19729);
#16718=AXIS2_PLACEMENT_3D('',#50551,#19730,#19731);
#16719=AXIS2_PLACEMENT_3D('',#50552,#19732,#19733);
#16720=AXIS2_PLACEMENT_3D('',#51493,#19734,#19735);
#16721=AXIS2_PLACEMENT_3D('',#51494,#19736,#19737);
#16722=AXIS2_PLACEMENT_3D('',#51495,#19738,#19739);
#16723=AXIS2_PLACEMENT_3D('',#51496,#19740,#19741);
#16724=AXIS2_PLACEMENT_3D('',#51497,#19742,#19743);
#16725=AXIS2_PLACEMENT_3D('',#51498,#19744,#19745);
#16726=AXIS2_PLACEMENT_3D('',#51499,#19746,#19747);
#16727=AXIS2_PLACEMENT_3D('',#51500,#19748,#19749);
#16728=AXIS2_PLACEMENT_3D('',#51501,#19750,#19751);
#16729=AXIS2_PLACEMENT_3D('',#52712,#19752,#19753);
#16730=AXIS2_PLACEMENT_3D('',#52713,#19754,#19755);
#16731=AXIS2_PLACEMENT_3D('',#52714,#19756,#19757);
#16732=AXIS2_PLACEMENT_3D('',#52715,#19758,#19759);
#16733=AXIS2_PLACEMENT_3D('',#52716,#19760,#19761);
#16734=AXIS2_PLACEMENT_3D('',#52717,#19762,#19763);
#16735=AXIS2_PLACEMENT_3D('',#52718,#19764,#19765);
#16736=AXIS2_PLACEMENT_3D('',#52719,#19766,#19767);
#16737=AXIS2_PLACEMENT_3D('',#52720,#19768,#19769);
#16738=AXIS2_PLACEMENT_3D('',#53757,#19770,#19771);
#16739=AXIS2_PLACEMENT_3D('',#53758,#19772,#19773);
#16740=AXIS2_PLACEMENT_3D('',#53759,#19774,#19775);
#16741=AXIS2_PLACEMENT_3D('',#53760,#19776,#19777);
#16742=AXIS2_PLACEMENT_3D('',#53761,#19778,#19779);
#16743=AXIS2_PLACEMENT_3D('',#53762,#19780,#19781);
#16744=AXIS2_PLACEMENT_3D('',#53763,#19782,#19783);
#16745=AXIS2_PLACEMENT_3D('',#53764,#19784,#19785);
#16746=AXIS2_PLACEMENT_3D('',#53765,#19786,#19787);
#16747=AXIS2_PLACEMENT_3D('',#54808,#19788,#19789);
#16748=AXIS2_PLACEMENT_3D('',#54809,#19790,#19791);
#16749=AXIS2_PLACEMENT_3D('',#54810,#19792,#19793);
#16750=AXIS2_PLACEMENT_3D('',#54811,#19794,#19795);
#16751=AXIS2_PLACEMENT_3D('',#54812,#19796,#19797);
#16752=AXIS2_PLACEMENT_3D('',#54813,#19798,#19799);
#16753=AXIS2_PLACEMENT_3D('',#54814,#19800,#19801);
#16754=AXIS2_PLACEMENT_3D('',#54815,#19802,#19803);
#16755=AXIS2_PLACEMENT_3D('',#54816,#19804,#19805);
#16756=AXIS2_PLACEMENT_3D('',#55887,#19806,#19807);
#16757=AXIS2_PLACEMENT_3D('',#55888,#19808,#19809);
#16758=AXIS2_PLACEMENT_3D('',#55889,#19810,#19811);
#16759=AXIS2_PLACEMENT_3D('',#55890,#19812,#19813);
#16760=AXIS2_PLACEMENT_3D('',#55891,#19814,#19815);
#16761=AXIS2_PLACEMENT_3D('',#55892,#19816,#19817);
#16762=AXIS2_PLACEMENT_3D('',#55893,#19818,#19819);
#16763=AXIS2_PLACEMENT_3D('',#55894,#19820,#19821);
#16764=AXIS2_PLACEMENT_3D('',#55895,#19822,#19823);
#16765=AXIS2_PLACEMENT_3D('',#57234,#19824,#19825);
#16766=AXIS2_PLACEMENT_3D('',#57235,#19826,#19827);
#16767=AXIS2_PLACEMENT_3D('',#57236,#19828,#19829);
#16768=AXIS2_PLACEMENT_3D('',#57237,#19830,#19831);
#16769=AXIS2_PLACEMENT_3D('',#57238,#19832,#19833);
#16770=AXIS2_PLACEMENT_3D('',#57239,#19834,#19835);
#16771=AXIS2_PLACEMENT_3D('',#57240,#19836,#19837);
#16772=AXIS2_PLACEMENT_3D('',#57241,#19838,#19839);
#16773=AXIS2_PLACEMENT_3D('',#57242,#19840,#19841);
#16774=AXIS2_PLACEMENT_3D('',#58291,#19842,#19843);
#16775=AXIS2_PLACEMENT_3D('',#58292,#19844,#19845);
#16776=AXIS2_PLACEMENT_3D('',#58293,#19846,#19847);
#16777=AXIS2_PLACEMENT_3D('',#58294,#19848,#19849);
#16778=AXIS2_PLACEMENT_3D('',#58295,#19850,#19851);
#16779=AXIS2_PLACEMENT_3D('',#58296,#19852,#19853);
#16780=AXIS2_PLACEMENT_3D('',#58297,#19854,#19855);
#16781=AXIS2_PLACEMENT_3D('',#58298,#19856,#19857);
#16782=AXIS2_PLACEMENT_3D('',#58299,#19858,#19859);
#16783=AXIS2_PLACEMENT_3D('',#59644,#19860,#19861);
#16784=AXIS2_PLACEMENT_3D('',#59645,#19862,#19863);
#16785=AXIS2_PLACEMENT_3D('',#59646,#19864,#19865);
#16786=AXIS2_PLACEMENT_3D('',#59647,#19866,#19867);
#16787=AXIS2_PLACEMENT_3D('',#59648,#19868,#19869);
#16788=AXIS2_PLACEMENT_3D('',#59649,#19870,#19871);
#16789=AXIS2_PLACEMENT_3D('',#59650,#19872,#19873);
#16790=AXIS2_PLACEMENT_3D('',#59651,#19874,#19875);
#16791=AXIS2_PLACEMENT_3D('',#59652,#19876,#19877);
#16792=AXIS2_PLACEMENT_3D('',#60751,#19878,#19879);
#16793=AXIS2_PLACEMENT_3D('',#60752,#19880,#19881);
#16794=AXIS2_PLACEMENT_3D('',#60753,#19882,#19883);
#16795=AXIS2_PLACEMENT_3D('',#60765,#19884,#19885);
#16796=AXIS2_PLACEMENT_3D('',#60766,#19886,#19887);
#16797=AXIS2_PLACEMENT_3D('',#60767,#19888,#19889);
#16798=AXIS2_PLACEMENT_3D('',#60768,#19890,#19891);
#16799=AXIS2_PLACEMENT_3D('',#60769,#19892,#19893);
#16800=AXIS2_PLACEMENT_3D('',#60770,#19894,#19895);
#16801=AXIS2_PLACEMENT_3D('',#60771,#19896,#19897);
#16802=AXIS2_PLACEMENT_3D('',#60772,#19898,#19899);
#16803=AXIS2_PLACEMENT_3D('',#62084,#19900,#19901);
#16804=AXIS2_PLACEMENT_3D('',#62092,#19902,#19903);
#16805=AXIS2_PLACEMENT_3D('',#62093,#19904,#19905);
#16806=AXIS2_PLACEMENT_3D('',#62094,#19906,#19907);
#16807=AXIS2_PLACEMENT_3D('',#62095,#19908,#19909);
#16808=AXIS2_PLACEMENT_3D('',#62103,#19910,#19911);
#16809=AXIS2_PLACEMENT_3D('',#62104,#19912,#19913);
#16810=AXIS2_PLACEMENT_3D('',#62105,#19914,#19915);
#16811=AXIS2_PLACEMENT_3D('',#62106,#19916,#19917);
#16812=AXIS2_PLACEMENT_3D('',#62107,#19918,#19919);
#16813=AXIS2_PLACEMENT_3D('',#62108,#19920,#19921);
#16814=AXIS2_PLACEMENT_3D('',#63077,#19922,#19923);
#16815=AXIS2_PLACEMENT_3D('',#63078,#19924,#19925);
#16816=AXIS2_PLACEMENT_3D('',#63079,#19926,#19927);
#16817=AXIS2_PLACEMENT_3D('',#63080,#19928,#19929);
#16818=AXIS2_PLACEMENT_3D('',#63081,#19930,#19931);
#19185=DIRECTION('axis',(0.,0.,1.));
#19186=DIRECTION('refdir',(1.,0.,0.));
#19187=DIRECTION('center_axis',(0.,-1.,0.));
#19188=DIRECTION('ref_axis',(0.,0.,-1.));
#19189=DIRECTION('center_axis',(0.,1.,0.));
#19190=DIRECTION('ref_axis',(0.,0.,-1.));
#19191=DIRECTION('',(-8.65956056235491E-17,-0.707106781186549,0.707106781186546));
#19192=DIRECTION('center_axis',(0.,-1.,0.));
#19193=DIRECTION('ref_axis',(0.,0.,-1.));
#19194=DIRECTION('center_axis',(0.,1.,0.));
#19195=DIRECTION('ref_axis',(0.,0.,-1.));
#19196=DIRECTION('center_axis',(0.,1.,0.));
#19197=DIRECTION('ref_axis',(0.,0.,1.));
#19198=DIRECTION('',(0.,1.,0.));
#19199=DIRECTION('center_axis',(0.,-1.,0.));
#19200=DIRECTION('ref_axis',(0.,0.,-1.));
#19201=DIRECTION('center_axis',(0.,-1.,0.));
#19202=DIRECTION('ref_axis',(0.,0.,-1.));
#19203=DIRECTION('center_axis',(0.,-1.,0.));
#19204=DIRECTION('ref_axis',(0.,0.,-1.));
#19205=DIRECTION('center_axis',(0.,1.,0.));
#19206=DIRECTION('ref_axis',(1.,0.,0.));
#19207=DIRECTION('',(-0.904527495480339,0.,-0.426415302164528));
#19208=DIRECTION('center_axis',(0.,1.,0.));
#19209=DIRECTION('ref_axis',(1.,0.,0.));
#19210=DIRECTION('',(-0.79610467303825,0.,-0.605158945704896));
#19211=DIRECTION('center_axis',(0.,1.,0.));
#19212=DIRECTION('ref_axis',(1.,0.,0.));
#19213=DIRECTION('',(-0.652888256250524,0.,-0.757454239442984));
#19214=DIRECTION('center_axis',(0.,1.,0.));
#19215=DIRECTION('ref_axis',(1.,0.,0.));
#19216=DIRECTION('',(-0.481137489758913,0.,-0.876645148248989));
#19217=DIRECTION('center_axis',(0.,1.,0.));
#19218=DIRECTION('ref_axis',(1.,0.,0.));
#19219=DIRECTION('',(-0.288358706211123,0.,-0.957522457466271));
#19220=DIRECTION('center_axis',(0.,1.,0.));
#19221=DIRECTION('ref_axis',(1.,0.,0.));
#19222=DIRECTION('',(-0.0829772635033118,0.,-0.996551440589748));
#19223=DIRECTION('center_axis',(0.,1.,0.));
#19224=DIRECTION('ref_axis',(1.,0.,0.));
#19225=DIRECTION('',(0.126030683788683,0.,-0.992026343775082));
#19226=DIRECTION('center_axis',(0.,1.,0.));
#19227=DIRECTION('ref_axis',(1.,0.,0.));
#19228=DIRECTION('',(0.329530485436752,0.,-0.944144935466912));
#19229=DIRECTION('center_axis',(0.,1.,0.));
#19230=DIRECTION('ref_axis',(1.,0.,0.));
#19231=DIRECTION('',(0.518628223608573,0.,-0.854999862968771));
#19232=DIRECTION('center_axis',(0.,1.,0.));
#19233=DIRECTION('ref_axis',(1.,0.,0.));
#19234=DIRECTION('',(0.685059419754336,0.,-0.728487193714379));
#19235=DIRECTION('center_axis',(0.,1.,0.));
#19236=DIRECTION('ref_axis',(1.,0.,0.));
#19237=DIRECTION('',(0.821550231977042,0.,-0.570136138425262));
#19238=DIRECTION('center_axis',(0.,1.,0.));
#19239=DIRECTION('ref_axis',(1.,0.,0.));
#19240=DIRECTION('',(0.922135356826958,0.,-0.386867398070217));
#19241=DIRECTION('center_axis',(0.,1.,0.));
#19242=DIRECTION('ref_axis',(1.,0.,0.));
#19243=DIRECTION('',(0.98241874168714,0.,-0.186690696023813));
#19244=DIRECTION('center_axis',(0.,1.,0.));
#19245=DIRECTION('ref_axis',(1.,0.,0.));
#19246=DIRECTION('',(0.999765713367456,0.,0.0216452852802363));
#19247=DIRECTION('center_axis',(0.,1.,0.));
#19248=DIRECTION('ref_axis',(1.,0.,0.));
#19249=DIRECTION('',(0.973418125965458,0.,0.229035263751885));
#19250=DIRECTION('center_axis',(0.,1.,0.));
#19251=DIRECTION('ref_axis',(1.,0.,0.));
#19252=DIRECTION('',(0.904527495480356,0.,0.426415302164492));
#19253=DIRECTION('center_axis',(0.,1.,0.));
#19254=DIRECTION('ref_axis',(1.,0.,0.));
#19255=DIRECTION('',(0.79610467303827,0.,0.605158945704869));
#19256=DIRECTION('center_axis',(0.,1.,0.));
#19257=DIRECTION('ref_axis',(1.,0.,0.));
#19258=DIRECTION('',(0.652888256250397,0.,0.757454239443094));
#19259=DIRECTION('center_axis',(0.,1.,0.));
#19260=DIRECTION('ref_axis',(1.,0.,0.));
#19261=DIRECTION('',(0.481137489758878,0.,0.876645148249008));
#19262=DIRECTION('center_axis',(0.,1.,0.));
#19263=DIRECTION('ref_axis',(1.,0.,0.));
#19264=DIRECTION('',(0.288358706211123,0.,0.957522457466271));
#19265=DIRECTION('center_axis',(0.,1.,0.));
#19266=DIRECTION('ref_axis',(1.,0.,0.));
#19267=DIRECTION('',(0.0829772635033118,0.,0.996551440589748));
#19268=DIRECTION('center_axis',(0.,1.,0.));
#19269=DIRECTION('ref_axis',(1.,0.,0.));
#19270=DIRECTION('',(-0.126030683788684,0.,0.992026343775082));
#19271=DIRECTION('center_axis',(0.,1.,0.));
#19272=DIRECTION('ref_axis',(1.,0.,0.));
#19273=DIRECTION('',(-0.329530485436752,0.,0.944144935466912));
#19274=DIRECTION('center_axis',(0.,1.,0.));
#19275=DIRECTION('ref_axis',(1.,0.,0.));
#19276=DIRECTION('',(-0.518628223608573,0.,0.854999862968771));
#19277=DIRECTION('center_axis',(0.,1.,0.));
#19278=DIRECTION('ref_axis',(1.,0.,0.));
#19279=DIRECTION('',(-0.685059419754315,0.,0.728487193714399));
#19280=DIRECTION('center_axis',(0.,1.,0.));
#19281=DIRECTION('ref_axis',(1.,0.,0.));
#19282=DIRECTION('',(-0.821550231977102,0.,0.570136138425175));
#19283=DIRECTION('center_axis',(0.,1.,0.));
#19284=DIRECTION('ref_axis',(1.,0.,0.));
#19285=DIRECTION('',(-0.922135356827004,0.,0.386867398070107));
#19286=DIRECTION('center_axis',(0.,1.,0.));
#19287=DIRECTION('ref_axis',(1.,0.,0.));
#19288=DIRECTION('',(-0.98241874168718,0.,0.186690696023607));
#19289=DIRECTION('center_axis',(0.,1.,0.));
#19290=DIRECTION('ref_axis',(1.,0.,0.));
#19291=DIRECTION('',(-0.99976571336746,0.,-0.021645285280017));
#19292=DIRECTION('center_axis',(0.,1.,0.));
#19293=DIRECTION('ref_axis',(1.,0.,0.));
#19294=DIRECTION('',(-0.973418125965487,0.,-0.229035263751761));
#19295=DIRECTION('center_axis',(0.,1.,0.));
#19296=DIRECTION('ref_axis',(0.,0.,-1.));
#19297=DIRECTION('',(8.65956056235493E-17,0.707106781186548,0.707106781186547));
#19298=DIRECTION('center_axis',(0.,1.,0.));
#19299=DIRECTION('ref_axis',(0.,0.,-1.));
#19300=DIRECTION('center_axis',(0.,1.,0.));
#19301=DIRECTION('ref_axis',(0.,0.,1.));
#19302=DIRECTION('',(0.98241874168718,0.,0.186690696023607));
#19303=DIRECTION('center_axis',(0.,1.,0.));
#19304=DIRECTION('ref_axis',(1.,0.,0.));
#19305=DIRECTION('',(0.99976571336746,0.,-0.021645285280017));
#19306=DIRECTION('center_axis',(0.,1.,0.));
#19307=DIRECTION('ref_axis',(1.,0.,0.));
#19308=DIRECTION('',(0.973418125965488,0.,-0.22903526375176));
#19309=DIRECTION('center_axis',(0.,1.,0.));
#19310=DIRECTION('ref_axis',(1.,0.,0.));
#19311=DIRECTION('',(0.904527495480339,0.,-0.426415302164528));
#19312=DIRECTION('center_axis',(0.,1.,0.));
#19313=DIRECTION('ref_axis',(1.,0.,0.));
#19314=DIRECTION('',(0.79610467303825,0.,-0.605158945704896));
#19315=DIRECTION('center_axis',(0.,1.,0.));
#19316=DIRECTION('ref_axis',(1.,0.,0.));
#19317=DIRECTION('',(0.652888256250524,0.,-0.757454239442984));
#19318=DIRECTION('center_axis',(0.,1.,0.));
#19319=DIRECTION('ref_axis',(1.,0.,0.));
#19320=DIRECTION('',(0.481137489758913,0.,-0.876645148248989));
#19321=DIRECTION('center_axis',(0.,1.,0.));
#19322=DIRECTION('ref_axis',(1.,0.,0.));
#19323=DIRECTION('',(0.288358706211123,0.,-0.957522457466271));
#19324=DIRECTION('center_axis',(0.,1.,0.));
#19325=DIRECTION('ref_axis',(1.,0.,0.));
#19326=DIRECTION('',(0.0829772635033118,0.,-0.996551440589748));
#19327=DIRECTION('center_axis',(0.,1.,0.));
#19328=DIRECTION('ref_axis',(1.,0.,0.));
#19329=DIRECTION('',(-0.126030683788638,0.,-0.992026343775088));
#19330=DIRECTION('center_axis',(0.,1.,0.));
#19331=DIRECTION('ref_axis',(1.,0.,0.));
#19332=DIRECTION('',(-0.32953048543679,0.,-0.944144935466898));
#19333=DIRECTION('center_axis',(0.,1.,0.));
#19334=DIRECTION('ref_axis',(1.,0.,0.));
#19335=DIRECTION('',(-0.518628223608571,0.,-0.854999862968772));
#19336=DIRECTION('center_axis',(0.,1.,0.));
#19337=DIRECTION('ref_axis',(1.,0.,0.));
#19338=DIRECTION('',(-0.685059419754336,0.,-0.728487193714379));
#19339=DIRECTION('center_axis',(0.,1.,0.));
#19340=DIRECTION('ref_axis',(1.,0.,0.));
#19341=DIRECTION('',(-0.821550231977042,0.,-0.570136138425262));
#19342=DIRECTION('center_axis',(0.,1.,0.));
#19343=DIRECTION('ref_axis',(1.,0.,0.));
#19344=DIRECTION('',(-0.922135356826964,0.,-0.386867398070201));
#19345=DIRECTION('center_axis',(0.,1.,0.));
#19346=DIRECTION('ref_axis',(1.,0.,0.));
#19347=DIRECTION('',(-0.98241874168714,0.,-0.186690696023813));
#19348=DIRECTION('center_axis',(0.,1.,0.));
#19349=DIRECTION('ref_axis',(1.,0.,0.));
#19350=DIRECTION('',(-0.999765713367456,0.,0.0216452852801921));
#19351=DIRECTION('center_axis',(0.,1.,0.));
#19352=DIRECTION('ref_axis',(1.,0.,0.));
#19353=DIRECTION('',(-0.973418125965457,0.,0.229035263751892));
#19354=DIRECTION('center_axis',(0.,1.,0.));
#19355=DIRECTION('ref_axis',(1.,0.,0.));
#19356=DIRECTION('',(-0.904527495480356,0.,0.426415302164492));
#19357=DIRECTION('center_axis',(0.,1.,0.));
#19358=DIRECTION('ref_axis',(1.,0.,0.));
#19359=DIRECTION('',(-0.796104673038291,0.,0.605158945704842));
#19360=DIRECTION('center_axis',(0.,1.,0.));
#19361=DIRECTION('ref_axis',(1.,0.,0.));
#19362=DIRECTION('',(-0.652888256250376,0.,0.757454239443112));
#19363=DIRECTION('center_axis',(0.,1.,0.));
#19364=DIRECTION('ref_axis',(1.,0.,0.));
#19365=DIRECTION('',(-0.481137489758911,0.,0.87664514824899));
#19366=DIRECTION('center_axis',(0.,1.,0.));
#19367=DIRECTION('ref_axis',(1.,0.,0.));
#19368=DIRECTION('',(-0.288358706211123,0.,0.957522457466271));
#19369=DIRECTION('center_axis',(0.,1.,0.));
#19370=DIRECTION('ref_axis',(1.,0.,0.));
#19371=DIRECTION('',(-0.0829772635033118,0.,0.996551440589748));
#19372=DIRECTION('center_axis',(0.,1.,0.));
#19373=DIRECTION('ref_axis',(1.,0.,0.));
#19374=DIRECTION('',(0.126030683788633,0.,0.992026343775088));
#19375=DIRECTION('center_axis',(0.,1.,0.));
#19376=DIRECTION('ref_axis',(1.,0.,0.));
#19377=DIRECTION('',(0.32953048543679,0.,0.944144935466898));
#19378=DIRECTION('center_axis',(0.,1.,0.));
#19379=DIRECTION('ref_axis',(1.,0.,0.));
#19380=DIRECTION('',(0.518628223608571,0.,0.854999862968772));
#19381=DIRECTION('center_axis',(0.,1.,0.));
#19382=DIRECTION('ref_axis',(1.,0.,0.));
#19383=DIRECTION('',(0.685059419754315,0.,0.728487193714399));
#19384=DIRECTION('center_axis',(0.,1.,0.));
#19385=DIRECTION('ref_axis',(1.,0.,0.));
#19386=DIRECTION('',(0.821550231977102,0.,0.570136138425175));
#19387=DIRECTION('center_axis',(0.,1.,0.));
#19388=DIRECTION('ref_axis',(1.,0.,0.));
#19389=DIRECTION('',(0.922135356827004,0.,0.386867398070107));
#19390=DIRECTION('center_axis',(0.,1.,0.));
#19391=DIRECTION('ref_axis',(1.,0.,0.));
#19392=DIRECTION('center_axis',(0.,-1.,0.));
#19393=DIRECTION('ref_axis',(0.,0.,1.));
#19394=DIRECTION('center_axis',(0.,1.,0.));
#19395=DIRECTION('ref_axis',(1.,0.,0.));
#19396=DIRECTION('center_axis',(0.,1.,0.));
#19397=DIRECTION('ref_axis',(0.,0.,1.));
#19398=DIRECTION('center_axis',(0.,1.,0.));
#19399=DIRECTION('ref_axis',(1.,0.,0.));
#19400=DIRECTION('center_axis',(0.,1.,0.));
#19401=DIRECTION('ref_axis',(0.,0.,1.));
#19402=DIRECTION('center_axis',(0.,1.,0.));
#19403=DIRECTION('ref_axis',(1.,0.,0.));
#19404=DIRECTION('center_axis',(0.,1.,0.));
#19405=DIRECTION('ref_axis',(0.,0.,1.));
#19406=DIRECTION('center_axis',(0.,1.,0.));
#19407=DIRECTION('ref_axis',(1.,0.,0.));
#19408=DIRECTION('center_axis',(0.,1.,0.));
#19409=DIRECTION('ref_axis',(0.,0.,1.));
#19410=DIRECTION('center_axis',(0.,-1.,0.));
#19411=DIRECTION('ref_axis',(0.,0.,1.));
#19412=DIRECTION('center_axis',(0.,1.,0.));
#19413=DIRECTION('ref_axis',(1.,0.,0.));
#19414=DIRECTION('center_axis',(0.,1.,0.));
#19415=DIRECTION('ref_axis',(0.,0.,1.));
#19416=DIRECTION('center_axis',(0.,1.,0.));
#19417=DIRECTION('ref_axis',(1.,0.,0.));
#19418=DIRECTION('center_axis',(0.,1.,0.));
#19419=DIRECTION('ref_axis',(0.,0.,1.));
#19420=DIRECTION('center_axis',(0.,1.,0.));
#19421=DIRECTION('ref_axis',(1.,0.,0.));
#19422=DIRECTION('center_axis',(0.,1.,0.));
#19423=DIRECTION('ref_axis',(0.,0.,1.));
#19424=DIRECTION('center_axis',(0.,1.,0.));
#19425=DIRECTION('ref_axis',(1.,0.,0.));
#19426=DIRECTION('center_axis',(0.,1.,0.));
#19427=DIRECTION('ref_axis',(0.,0.,1.));
#19428=DIRECTION('center_axis',(0.,-1.,0.));
#19429=DIRECTION('ref_axis',(0.,0.,1.));
#19430=DIRECTION('center_axis',(0.,1.,0.));
#19431=DIRECTION('ref_axis',(1.,0.,0.));
#19432=DIRECTION('center_axis',(0.,1.,0.));
#19433=DIRECTION('ref_axis',(0.,0.,1.));
#19434=DIRECTION('center_axis',(0.,1.,0.));
#19435=DIRECTION('ref_axis',(1.,0.,0.));
#19436=DIRECTION('center_axis',(0.,1.,0.));
#19437=DIRECTION('ref_axis',(0.,0.,1.));
#19438=DIRECTION('center_axis',(0.,1.,0.));
#19439=DIRECTION('ref_axis',(1.,0.,0.));
#19440=DIRECTION('center_axis',(0.,1.,0.));
#19441=DIRECTION('ref_axis',(0.,0.,1.));
#19442=DIRECTION('center_axis',(0.,1.,0.));
#19443=DIRECTION('ref_axis',(1.,0.,0.));
#19444=DIRECTION('center_axis',(0.,1.,0.));
#19445=DIRECTION('ref_axis',(0.,0.,1.));
#19446=DIRECTION('center_axis',(0.,-1.,0.));
#19447=DIRECTION('ref_axis',(0.,0.,1.));
#19448=DIRECTION('center_axis',(0.,1.,0.));
#19449=DIRECTION('ref_axis',(1.,0.,0.));
#19450=DIRECTION('center_axis',(0.,1.,0.));
#19451=DIRECTION('ref_axis',(0.,0.,1.));
#19452=DIRECTION('center_axis',(0.,1.,0.));
#19453=DIRECTION('ref_axis',(1.,0.,0.));
#19454=DIRECTION('center_axis',(0.,1.,0.));
#19455=DIRECTION('ref_axis',(0.,0.,1.));
#19456=DIRECTION('center_axis',(0.,1.,0.));
#19457=DIRECTION('ref_axis',(1.,0.,0.));
#19458=DIRECTION('center_axis',(0.,1.,0.));
#19459=DIRECTION('ref_axis',(0.,0.,1.));
#19460=DIRECTION('center_axis',(0.,1.,0.));
#19461=DIRECTION('ref_axis',(1.,0.,0.));
#19462=DIRECTION('center_axis',(0.,1.,0.));
#19463=DIRECTION('ref_axis',(0.,0.,1.));
#19464=DIRECTION('center_axis',(0.,-1.,0.));
#19465=DIRECTION('ref_axis',(0.,0.,1.));
#19466=DIRECTION('center_axis',(0.,1.,0.));
#19467=DIRECTION('ref_axis',(1.,0.,0.));
#19468=DIRECTION('center_axis',(0.,1.,0.));
#19469=DIRECTION('ref_axis',(0.,0.,1.));
#19470=DIRECTION('center_axis',(0.,1.,0.));
#19471=DIRECTION('ref_axis',(1.,0.,0.));
#19472=DIRECTION('center_axis',(0.,1.,0.));
#19473=DIRECTION('ref_axis',(0.,0.,1.));
#19474=DIRECTION('center_axis',(0.,1.,0.));
#19475=DIRECTION('ref_axis',(1.,0.,0.));
#19476=DIRECTION('center_axis',(0.,1.,0.));
#19477=DIRECTION('ref_axis',(0.,0.,1.));
#19478=DIRECTION('center_axis',(0.,1.,0.));
#19479=DIRECTION('ref_axis',(1.,0.,0.));
#19480=DIRECTION('center_axis',(0.,1.,0.));
#19481=DIRECTION('ref_axis',(0.,0.,1.));
#19482=DIRECTION('center_axis',(0.,-1.,0.));
#19483=DIRECTION('ref_axis',(0.,0.,1.));
#19484=DIRECTION('center_axis',(0.,1.,0.));
#19485=DIRECTION('ref_axis',(1.,0.,0.));
#19486=DIRECTION('center_axis',(0.,1.,0.));
#19487=DIRECTION('ref_axis',(0.,0.,1.));
#19488=DIRECTION('center_axis',(0.,1.,0.));
#19489=DIRECTION('ref_axis',(1.,0.,0.));
#19490=DIRECTION('center_axis',(0.,1.,0.));
#19491=DIRECTION('ref_axis',(0.,0.,1.));
#19492=DIRECTION('center_axis',(0.,1.,0.));
#19493=DIRECTION('ref_axis',(1.,0.,0.));
#19494=DIRECTION('center_axis',(0.,1.,0.));
#19495=DIRECTION('ref_axis',(0.,0.,1.));
#19496=DIRECTION('center_axis',(0.,1.,0.));
#19497=DIRECTION('ref_axis',(1.,0.,0.));
#19498=DIRECTION('center_axis',(0.,1.,0.));
#19499=DIRECTION('ref_axis',(0.,0.,1.));
#19500=DIRECTION('center_axis',(0.,-1.,0.));
#19501=DIRECTION('ref_axis',(0.,0.,1.));
#19502=DIRECTION('center_axis',(0.,1.,0.));
#19503=DIRECTION('ref_axis',(1.,0.,0.));
#19504=DIRECTION('center_axis',(0.,1.,0.));
#19505=DIRECTION('ref_axis',(0.,0.,1.));
#19506=DIRECTION('center_axis',(0.,1.,0.));
#19507=DIRECTION('ref_axis',(1.,0.,0.));
#19508=DIRECTION('center_axis',(0.,1.,0.));
#19509=DIRECTION('ref_axis',(0.,0.,1.));
#19510=DIRECTION('center_axis',(0.,1.,0.));
#19511=DIRECTION('ref_axis',(1.,0.,0.));
#19512=DIRECTION('center_axis',(0.,1.,0.));
#19513=DIRECTION('ref_axis',(0.,0.,1.));
#19514=DIRECTION('center_axis',(0.,1.,0.));
#19515=DIRECTION('ref_axis',(1.,0.,0.));
#19516=DIRECTION('center_axis',(0.,1.,0.));
#19517=DIRECTION('ref_axis',(0.,0.,1.));
#19518=DIRECTION('center_axis',(0.,-1.,0.));
#19519=DIRECTION('ref_axis',(0.,0.,1.));
#19520=DIRECTION('center_axis',(0.,1.,0.));
#19521=DIRECTION('ref_axis',(1.,0.,0.));
#19522=DIRECTION('center_axis',(0.,1.,0.));
#19523=DIRECTION('ref_axis',(0.,0.,1.));
#19524=DIRECTION('center_axis',(0.,1.,0.));
#19525=DIRECTION('ref_axis',(1.,0.,0.));
#19526=DIRECTION('center_axis',(0.,1.,0.));
#19527=DIRECTION('ref_axis',(0.,0.,1.));
#19528=DIRECTION('center_axis',(0.,1.,0.));
#19529=DIRECTION('ref_axis',(1.,0.,0.));
#19530=DIRECTION('center_axis',(0.,1.,0.));
#19531=DIRECTION('ref_axis',(0.,0.,1.));
#19532=DIRECTION('center_axis',(0.,1.,0.));
#19533=DIRECTION('ref_axis',(1.,0.,0.));
#19534=DIRECTION('center_axis',(0.,1.,0.));
#19535=DIRECTION('ref_axis',(0.,0.,1.));
#19536=DIRECTION('center_axis',(0.,-1.,0.));
#19537=DIRECTION('ref_axis',(0.,0.,1.));
#19538=DIRECTION('center_axis',(0.,1.,0.));
#19539=DIRECTION('ref_axis',(1.,0.,0.));
#19540=DIRECTION('center_axis',(0.,1.,0.));
#19541=DIRECTION('ref_axis',(0.,0.,1.));
#19542=DIRECTION('center_axis',(0.,1.,0.));
#19543=DIRECTION('ref_axis',(1.,0.,0.));
#19544=DIRECTION('center_axis',(0.,1.,0.));
#19545=DIRECTION('ref_axis',(0.,0.,1.));
#19546=DIRECTION('center_axis',(0.,1.,0.));
#19547=DIRECTION('ref_axis',(1.,0.,0.));
#19548=DIRECTION('center_axis',(0.,1.,0.));
#19549=DIRECTION('ref_axis',(0.,0.,1.));
#19550=DIRECTION('center_axis',(0.,1.,0.));
#19551=DIRECTION('ref_axis',(1.,0.,0.));
#19552=DIRECTION('center_axis',(0.,1.,0.));
#19553=DIRECTION('ref_axis',(0.,0.,1.));
#19554=DIRECTION('center_axis',(0.,-1.,0.));
#19555=DIRECTION('ref_axis',(0.,0.,1.));
#19556=DIRECTION('center_axis',(0.,1.,0.));
#19557=DIRECTION('ref_axis',(1.,0.,0.));
#19558=DIRECTION('center_axis',(0.,1.,0.));
#19559=DIRECTION('ref_axis',(0.,0.,1.));
#19560=DIRECTION('center_axis',(0.,1.,0.));
#19561=DIRECTION('ref_axis',(1.,0.,0.));
#19562=DIRECTION('center_axis',(0.,1.,0.));
#19563=DIRECTION('ref_axis',(0.,0.,1.));
#19564=DIRECTION('center_axis',(0.,1.,0.));
#19565=DIRECTION('ref_axis',(1.,0.,0.));
#19566=DIRECTION('center_axis',(0.,1.,0.));
#19567=DIRECTION('ref_axis',(0.,0.,1.));
#19568=DIRECTION('center_axis',(0.,1.,0.));
#19569=DIRECTION('ref_axis',(1.,0.,0.));
#19570=DIRECTION('center_axis',(0.,1.,0.));
#19571=DIRECTION('ref_axis',(0.,0.,1.));
#19572=DIRECTION('center_axis',(0.,-1.,0.));
#19573=DIRECTION('ref_axis',(0.,0.,1.));
#19574=DIRECTION('center_axis',(0.,1.,0.));
#19575=DIRECTION('ref_axis',(1.,0.,0.));
#19576=DIRECTION('center_axis',(0.,1.,0.));
#19577=DIRECTION('ref_axis',(0.,0.,1.));
#19578=DIRECTION('center_axis',(0.,1.,0.));
#19579=DIRECTION('ref_axis',(1.,0.,0.));
#19580=DIRECTION('center_axis',(0.,1.,0.));
#19581=DIRECTION('ref_axis',(0.,0.,1.));
#19582=DIRECTION('center_axis',(0.,1.,0.));
#19583=DIRECTION('ref_axis',(1.,0.,0.));
#19584=DIRECTION('center_axis',(0.,1.,0.));
#19585=DIRECTION('ref_axis',(0.,0.,1.));
#19586=DIRECTION('center_axis',(0.,1.,0.));
#19587=DIRECTION('ref_axis',(1.,0.,0.));
#19588=DIRECTION('center_axis',(0.,1.,0.));
#19589=DIRECTION('ref_axis',(0.,0.,1.));
#19590=DIRECTION('center_axis',(0.,-1.,0.));
#19591=DIRECTION('ref_axis',(0.,0.,1.));
#19592=DIRECTION('center_axis',(0.,1.,0.));
#19593=DIRECTION('ref_axis',(1.,0.,0.));
#19594=DIRECTION('center_axis',(0.,1.,0.));
#19595=DIRECTION('ref_axis',(0.,0.,1.));
#19596=DIRECTION('center_axis',(0.,1.,0.));
#19597=DIRECTION('ref_axis',(1.,0.,0.));
#19598=DIRECTION('center_axis',(0.,1.,0.));
#19599=DIRECTION('ref_axis',(0.,0.,1.));
#19600=DIRECTION('center_axis',(0.,1.,0.));
#19601=DIRECTION('ref_axis',(1.,0.,0.));
#19602=DIRECTION('center_axis',(0.,1.,0.));
#19603=DIRECTION('ref_axis',(0.,0.,1.));
#19604=DIRECTION('center_axis',(0.,1.,0.));
#19605=DIRECTION('ref_axis',(1.,0.,0.));
#19606=DIRECTION('center_axis',(0.,1.,0.));
#19607=DIRECTION('ref_axis',(0.,0.,1.));
#19608=DIRECTION('center_axis',(0.,-1.,0.));
#19609=DIRECTION('ref_axis',(0.,0.,1.));
#19610=DIRECTION('center_axis',(0.,1.,0.));
#19611=DIRECTION('ref_axis',(1.,0.,0.));
#19612=DIRECTION('center_axis',(0.,1.,0.));
#19613=DIRECTION('ref_axis',(0.,0.,1.));
#19614=DIRECTION('center_axis',(0.,1.,0.));
#19615=DIRECTION('ref_axis',(1.,0.,0.));
#19616=DIRECTION('center_axis',(0.,1.,0.));
#19617=DIRECTION('ref_axis',(0.,0.,1.));
#19618=DIRECTION('center_axis',(0.,1.,0.));
#19619=DIRECTION('ref_axis',(1.,0.,0.));
#19620=DIRECTION('center_axis',(0.,1.,0.));
#19621=DIRECTION('ref_axis',(0.,0.,1.));
#19622=DIRECTION('center_axis',(0.,1.,0.));
#19623=DIRECTION('ref_axis',(1.,0.,0.));
#19624=DIRECTION('center_axis',(0.,1.,0.));
#19625=DIRECTION('ref_axis',(0.,0.,1.));
#19626=DIRECTION('center_axis',(0.,-1.,0.));
#19627=DIRECTION('ref_axis',(0.,0.,1.));
#19628=DIRECTION('center_axis',(0.,1.,0.));
#19629=DIRECTION('ref_axis',(1.,0.,0.));
#19630=DIRECTION('center_axis',(0.,1.,0.));
#19631=DIRECTION('ref_axis',(0.,0.,1.));
#19632=DIRECTION('center_axis',(0.,1.,0.));
#19633=DIRECTION('ref_axis',(1.,0.,0.));
#19634=DIRECTION('center_axis',(0.,1.,0.));
#19635=DIRECTION('ref_axis',(0.,0.,1.));
#19636=DIRECTION('center_axis',(0.,1.,0.));
#19637=DIRECTION('ref_axis',(1.,0.,0.));
#19638=DIRECTION('center_axis',(0.,1.,0.));
#19639=DIRECTION('ref_axis',(0.,0.,1.));
#19640=DIRECTION('center_axis',(0.,1.,0.));
#19641=DIRECTION('ref_axis',(1.,0.,0.));
#19642=DIRECTION('center_axis',(0.,1.,0.));
#19643=DIRECTION('ref_axis',(0.,0.,1.));
#19644=DIRECTION('center_axis',(0.,-1.,0.));
#19645=DIRECTION('ref_axis',(0.,0.,1.));
#19646=DIRECTION('center_axis',(0.,1.,0.));
#19647=DIRECTION('ref_axis',(1.,0.,0.));
#19648=DIRECTION('center_axis',(0.,1.,0.));
#19649=DIRECTION('ref_axis',(0.,0.,1.));
#19650=DIRECTION('center_axis',(0.,1.,0.));
#19651=DIRECTION('ref_axis',(1.,0.,0.));
#19652=DIRECTION('center_axis',(0.,1.,0.));
#19653=DIRECTION('ref_axis',(0.,0.,1.));
#19654=DIRECTION('center_axis',(0.,1.,0.));
#19655=DIRECTION('ref_axis',(1.,0.,0.));
#19656=DIRECTION('center_axis',(0.,1.,0.));
#19657=DIRECTION('ref_axis',(0.,0.,1.));
#19658=DIRECTION('center_axis',(0.,1.,0.));
#19659=DIRECTION('ref_axis',(1.,0.,0.));
#19660=DIRECTION('center_axis',(0.,1.,0.));
#19661=DIRECTION('ref_axis',(0.,0.,1.));
#19662=DIRECTION('center_axis',(0.,-1.,0.));
#19663=DIRECTION('ref_axis',(0.,0.,1.));
#19664=DIRECTION('center_axis',(0.,1.,0.));
#19665=DIRECTION('ref_axis',(1.,0.,0.));
#19666=DIRECTION('center_axis',(0.,1.,0.));
#19667=DIRECTION('ref_axis',(0.,0.,1.));
#19668=DIRECTION('center_axis',(0.,1.,0.));
#19669=DIRECTION('ref_axis',(1.,0.,0.));
#19670=DIRECTION('center_axis',(0.,1.,0.));
#19671=DIRECTION('ref_axis',(0.,0.,1.));
#19672=DIRECTION('center_axis',(0.,1.,0.));
#19673=DIRECTION('ref_axis',(1.,0.,0.));
#19674=DIRECTION('center_axis',(0.,1.,0.));
#19675=DIRECTION('ref_axis',(0.,0.,1.));
#19676=DIRECTION('center_axis',(0.,1.,0.));
#19677=DIRECTION('ref_axis',(1.,0.,0.));
#19678=DIRECTION('center_axis',(0.,1.,0.));
#19679=DIRECTION('ref_axis',(0.,0.,1.));
#19680=DIRECTION('center_axis',(0.,-1.,0.));
#19681=DIRECTION('ref_axis',(0.,0.,1.));
#19682=DIRECTION('center_axis',(0.,1.,0.));
#19683=DIRECTION('ref_axis',(1.,0.,0.));
#19684=DIRECTION('center_axis',(0.,1.,0.));
#19685=DIRECTION('ref_axis',(0.,0.,1.));
#19686=DIRECTION('center_axis',(0.,1.,0.));
#19687=DIRECTION('ref_axis',(1.,0.,0.));
#19688=DIRECTION('center_axis',(0.,1.,0.));
#19689=DIRECTION('ref_axis',(0.,0.,1.));
#19690=DIRECTION('center_axis',(0.,1.,0.));
#19691=DIRECTION('ref_axis',(1.,0.,0.));
#19692=DIRECTION('center_axis',(0.,1.,0.));
#19693=DIRECTION('ref_axis',(0.,0.,1.));
#19694=DIRECTION('center_axis',(0.,1.,0.));
#19695=DIRECTION('ref_axis',(1.,0.,0.));
#19696=DIRECTION('center_axis',(0.,1.,0.));
#19697=DIRECTION('ref_axis',(0.,0.,1.));
#19698=DIRECTION('center_axis',(0.,-1.,0.));
#19699=DIRECTION('ref_axis',(0.,0.,1.));
#19700=DIRECTION('center_axis',(0.,1.,0.));
#19701=DIRECTION('ref_axis',(1.,0.,0.));
#19702=DIRECTION('center_axis',(0.,1.,0.));
#19703=DIRECTION('ref_axis',(0.,0.,1.));
#19704=DIRECTION('center_axis',(0.,1.,0.));
#19705=DIRECTION('ref_axis',(1.,0.,0.));
#19706=DIRECTION('center_axis',(0.,1.,0.));
#19707=DIRECTION('ref_axis',(0.,0.,1.));
#19708=DIRECTION('center_axis',(0.,1.,0.));
#19709=DIRECTION('ref_axis',(1.,0.,0.));
#19710=DIRECTION('center_axis',(0.,1.,0.));
#19711=DIRECTION('ref_axis',(0.,0.,1.));
#19712=DIRECTION('center_axis',(0.,1.,0.));
#19713=DIRECTION('ref_axis',(1.,0.,0.));
#19714=DIRECTION('center_axis',(0.,1.,0.));
#19715=DIRECTION('ref_axis',(0.,0.,1.));
#19716=DIRECTION('center_axis',(0.,-1.,0.));
#19717=DIRECTION('ref_axis',(0.,0.,1.));
#19718=DIRECTION('center_axis',(0.,1.,0.));
#19719=DIRECTION('ref_axis',(1.,0.,0.));
#19720=DIRECTION('center_axis',(0.,1.,0.));
#19721=DIRECTION('ref_axis',(0.,0.,1.));
#19722=DIRECTION('center_axis',(0.,1.,0.));
#19723=DIRECTION('ref_axis',(1.,0.,0.));
#19724=DIRECTION('center_axis',(0.,1.,0.));
#19725=DIRECTION('ref_axis',(0.,0.,1.));
#19726=DIRECTION('center_axis',(0.,1.,0.));
#19727=DIRECTION('ref_axis',(1.,0.,0.));
#19728=DIRECTION('center_axis',(0.,1.,0.));
#19729=DIRECTION('ref_axis',(0.,0.,1.));
#19730=DIRECTION('center_axis',(0.,1.,0.));
#19731=DIRECTION('ref_axis',(1.,0.,0.));
#19732=DIRECTION('center_axis',(0.,1.,0.));
#19733=DIRECTION('ref_axis',(0.,0.,1.));
#19734=DIRECTION('center_axis',(0.,-1.,0.));
#19735=DIRECTION('ref_axis',(0.,0.,1.));
#19736=DIRECTION('center_axis',(0.,1.,0.));
#19737=DIRECTION('ref_axis',(1.,0.,0.));
#19738=DIRECTION('center_axis',(0.,1.,0.));
#19739=DIRECTION('ref_axis',(0.,0.,1.));
#19740=DIRECTION('center_axis',(0.,1.,0.));
#19741=DIRECTION('ref_axis',(1.,0.,0.));
#19742=DIRECTION('center_axis',(0.,1.,0.));
#19743=DIRECTION('ref_axis',(0.,0.,1.));
#19744=DIRECTION('center_axis',(0.,1.,0.));
#19745=DIRECTION('ref_axis',(1.,0.,0.));
#19746=DIRECTION('center_axis',(0.,1.,0.));
#19747=DIRECTION('ref_axis',(0.,0.,1.));
#19748=DIRECTION('center_axis',(0.,1.,0.));
#19749=DIRECTION('ref_axis',(1.,0.,0.));
#19750=DIRECTION('center_axis',(0.,1.,0.));
#19751=DIRECTION('ref_axis',(0.,0.,1.));
#19752=DIRECTION('center_axis',(0.,-1.,0.));
#19753=DIRECTION('ref_axis',(0.,0.,1.));
#19754=DIRECTION('center_axis',(0.,1.,0.));
#19755=DIRECTION('ref_axis',(1.,0.,0.));
#19756=DIRECTION('center_axis',(0.,1.,0.));
#19757=DIRECTION('ref_axis',(0.,0.,1.));
#19758=DIRECTION('center_axis',(0.,1.,0.));
#19759=DIRECTION('ref_axis',(1.,0.,0.));
#19760=DIRECTION('center_axis',(0.,1.,0.));
#19761=DIRECTION('ref_axis',(0.,0.,1.));
#19762=DIRECTION('center_axis',(0.,1.,0.));
#19763=DIRECTION('ref_axis',(1.,0.,0.));
#19764=DIRECTION('center_axis',(0.,1.,0.));
#19765=DIRECTION('ref_axis',(0.,0.,1.));
#19766=DIRECTION('center_axis',(0.,1.,0.));
#19767=DIRECTION('ref_axis',(1.,0.,0.));
#19768=DIRECTION('center_axis',(0.,1.,0.));
#19769=DIRECTION('ref_axis',(0.,0.,1.));
#19770=DIRECTION('center_axis',(0.,-1.,0.));
#19771=DIRECTION('ref_axis',(0.,0.,1.));
#19772=DIRECTION('center_axis',(0.,1.,0.));
#19773=DIRECTION('ref_axis',(1.,0.,0.));
#19774=DIRECTION('center_axis',(0.,1.,0.));
#19775=DIRECTION('ref_axis',(0.,0.,1.));
#19776=DIRECTION('center_axis',(0.,1.,0.));
#19777=DIRECTION('ref_axis',(1.,0.,0.));
#19778=DIRECTION('center_axis',(0.,1.,0.));
#19779=DIRECTION('ref_axis',(0.,0.,1.));
#19780=DIRECTION('center_axis',(0.,1.,0.));
#19781=DIRECTION('ref_axis',(1.,0.,0.));
#19782=DIRECTION('center_axis',(0.,1.,0.));
#19783=DIRECTION('ref_axis',(0.,0.,1.));
#19784=DIRECTION('center_axis',(0.,1.,0.));
#19785=DIRECTION('ref_axis',(1.,0.,0.));
#19786=DIRECTION('center_axis',(0.,1.,0.));
#19787=DIRECTION('ref_axis',(0.,0.,1.));
#19788=DIRECTION('center_axis',(0.,-1.,0.));
#19789=DIRECTION('ref_axis',(0.,0.,1.));
#19790=DIRECTION('center_axis',(0.,1.,0.));
#19791=DIRECTION('ref_axis',(1.,0.,0.));
#19792=DIRECTION('center_axis',(0.,1.,0.));
#19793=DIRECTION('ref_axis',(0.,0.,1.));
#19794=DIRECTION('center_axis',(0.,1.,0.));
#19795=DIRECTION('ref_axis',(1.,0.,0.));
#19796=DIRECTION('center_axis',(0.,1.,0.));
#19797=DIRECTION('ref_axis',(0.,0.,1.));
#19798=DIRECTION('center_axis',(0.,1.,0.));
#19799=DIRECTION('ref_axis',(1.,0.,0.));
#19800=DIRECTION('center_axis',(0.,1.,0.));
#19801=DIRECTION('ref_axis',(0.,0.,1.));
#19802=DIRECTION('center_axis',(0.,1.,0.));
#19803=DIRECTION('ref_axis',(1.,0.,0.));
#19804=DIRECTION('center_axis',(0.,1.,0.));
#19805=DIRECTION('ref_axis',(0.,0.,1.));
#19806=DIRECTION('center_axis',(0.,-1.,0.));
#19807=DIRECTION('ref_axis',(0.,0.,1.));
#19808=DIRECTION('center_axis',(0.,1.,0.));
#19809=DIRECTION('ref_axis',(1.,0.,0.));
#19810=DIRECTION('center_axis',(0.,1.,0.));
#19811=DIRECTION('ref_axis',(0.,0.,1.));
#19812=DIRECTION('center_axis',(0.,1.,0.));
#19813=DIRECTION('ref_axis',(1.,0.,0.));
#19814=DIRECTION('center_axis',(0.,1.,0.));
#19815=DIRECTION('ref_axis',(0.,0.,1.));
#19816=DIRECTION('center_axis',(0.,1.,0.));
#19817=DIRECTION('ref_axis',(1.,0.,0.));
#19818=DIRECTION('center_axis',(0.,1.,0.));
#19819=DIRECTION('ref_axis',(0.,0.,1.));
#19820=DIRECTION('center_axis',(0.,1.,0.));
#19821=DIRECTION('ref_axis',(1.,0.,0.));
#19822=DIRECTION('center_axis',(0.,1.,0.));
#19823=DIRECTION('ref_axis',(0.,0.,1.));
#19824=DIRECTION('center_axis',(0.,-1.,0.));
#19825=DIRECTION('ref_axis',(0.,0.,1.));
#19826=DIRECTION('center_axis',(0.,1.,0.));
#19827=DIRECTION('ref_axis',(1.,0.,0.));
#19828=DIRECTION('center_axis',(0.,1.,0.));
#19829=DIRECTION('ref_axis',(0.,0.,1.));
#19830=DIRECTION('center_axis',(0.,1.,0.));
#19831=DIRECTION('ref_axis',(1.,0.,0.));
#19832=DIRECTION('center_axis',(0.,1.,0.));
#19833=DIRECTION('ref_axis',(0.,0.,1.));
#19834=DIRECTION('center_axis',(0.,1.,0.));
#19835=DIRECTION('ref_axis',(1.,0.,0.));
#19836=DIRECTION('center_axis',(0.,1.,0.));
#19837=DIRECTION('ref_axis',(0.,0.,1.));
#19838=DIRECTION('center_axis',(0.,1.,0.));
#19839=DIRECTION('ref_axis',(1.,0.,0.));
#19840=DIRECTION('center_axis',(0.,1.,0.));
#19841=DIRECTION('ref_axis',(0.,0.,1.));
#19842=DIRECTION('center_axis',(0.,-1.,0.));
#19843=DIRECTION('ref_axis',(0.,0.,1.));
#19844=DIRECTION('center_axis',(0.,1.,0.));
#19845=DIRECTION('ref_axis',(1.,0.,0.));
#19846=DIRECTION('center_axis',(0.,1.,0.));
#19847=DIRECTION('ref_axis',(0.,0.,1.));
#19848=DIRECTION('center_axis',(0.,1.,0.));
#19849=DIRECTION('ref_axis',(1.,0.,0.));
#19850=DIRECTION('center_axis',(0.,1.,0.));
#19851=DIRECTION('ref_axis',(0.,0.,1.));
#19852=DIRECTION('center_axis',(0.,1.,0.));
#19853=DIRECTION('ref_axis',(1.,0.,0.));
#19854=DIRECTION('center_axis',(0.,1.,0.));
#19855=DIRECTION('ref_axis',(0.,0.,1.));
#19856=DIRECTION('center_axis',(0.,1.,0.));
#19857=DIRECTION('ref_axis',(1.,0.,0.));
#19858=DIRECTION('center_axis',(0.,1.,0.));
#19859=DIRECTION('ref_axis',(0.,0.,1.));
#19860=DIRECTION('center_axis',(0.,-1.,0.));
#19861=DIRECTION('ref_axis',(0.,0.,1.));
#19862=DIRECTION('center_axis',(0.,1.,0.));
#19863=DIRECTION('ref_axis',(1.,0.,0.));
#19864=DIRECTION('center_axis',(0.,1.,0.));
#19865=DIRECTION('ref_axis',(0.,0.,1.));
#19866=DIRECTION('center_axis',(0.,1.,0.));
#19867=DIRECTION('ref_axis',(1.,0.,0.));
#19868=DIRECTION('center_axis',(0.,1.,0.));
#19869=DIRECTION('ref_axis',(0.,0.,1.));
#19870=DIRECTION('center_axis',(0.,1.,0.));
#19871=DIRECTION('ref_axis',(1.,0.,0.));
#19872=DIRECTION('center_axis',(0.,1.,0.));
#19873=DIRECTION('ref_axis',(0.,0.,1.));
#19874=DIRECTION('center_axis',(0.,1.,0.));
#19875=DIRECTION('ref_axis',(1.,0.,0.));
#19876=DIRECTION('center_axis',(0.,1.,0.));
#19877=DIRECTION('ref_axis',(0.,0.,1.));
#19878=DIRECTION('center_axis',(0.,-1.,0.));
#19879=DIRECTION('ref_axis',(0.,0.,1.));
#19880=DIRECTION('center_axis',(0.,1.,0.));
#19881=DIRECTION('ref_axis',(1.,0.,0.));
#19882=DIRECTION('center_axis',(0.,-1.,0.));
#19883=DIRECTION('ref_axis',(0.,0.,1.));
#19884=DIRECTION('center_axis',(0.,1.,0.));
#19885=DIRECTION('ref_axis',(1.,0.,0.));
#19886=DIRECTION('center_axis',(0.,1.,0.));
#19887=DIRECTION('ref_axis',(0.,0.,1.));
#19888=DIRECTION('center_axis',(0.,1.,0.));
#19889=DIRECTION('ref_axis',(1.,0.,0.));
#19890=DIRECTION('center_axis',(0.,1.,0.));
#19891=DIRECTION('ref_axis',(0.,0.,1.));
#19892=DIRECTION('center_axis',(0.,1.,0.));
#19893=DIRECTION('ref_axis',(1.,0.,0.));
#19894=DIRECTION('center_axis',(0.,1.,0.));
#19895=DIRECTION('ref_axis',(0.,0.,1.));
#19896=DIRECTION('center_axis',(0.,1.,0.));
#19897=DIRECTION('ref_axis',(1.,0.,0.));
#19898=DIRECTION('center_axis',(0.,1.,0.));
#19899=DIRECTION('ref_axis',(0.,0.,1.));
#19900=DIRECTION('center_axis',(0.,-1.,0.));
#19901=DIRECTION('ref_axis',(0.,0.,1.));
#19902=DIRECTION('center_axis',(0.,1.,0.));
#19903=DIRECTION('ref_axis',(1.,0.,0.));
#19904=DIRECTION('center_axis',(0.,1.,0.));
#19905=DIRECTION('ref_axis',(0.,0.,1.));
#19906=DIRECTION('center_axis',(0.,1.,0.));
#19907=DIRECTION('ref_axis',(1.,0.,0.));
#19908=DIRECTION('center_axis',(0.,1.,0.));
#19909=DIRECTION('ref_axis',(0.,0.,1.));
#19910=DIRECTION('center_axis',(0.,1.,0.));
#19911=DIRECTION('ref_axis',(1.,0.,0.));
#19912=DIRECTION('center_axis',(0.,1.,0.));
#19913=DIRECTION('ref_axis',(0.,0.,1.));
#19914=DIRECTION('center_axis',(0.,1.,0.));
#19915=DIRECTION('ref_axis',(1.,0.,0.));
#19916=DIRECTION('center_axis',(0.,1.,0.));
#19917=DIRECTION('ref_axis',(0.,0.,1.));
#19918=DIRECTION('center_axis',(0.,1.,0.));
#19919=DIRECTION('ref_axis',(1.,0.,0.));
#19920=DIRECTION('center_axis',(0.,1.,0.));
#19921=DIRECTION('ref_axis',(0.,0.,1.));
#19922=DIRECTION('center_axis',(0.,1.,0.));
#19923=DIRECTION('ref_axis',(0.,0.,1.));
#19924=DIRECTION('center_axis',(0.,1.,0.));
#19925=DIRECTION('ref_axis',(1.,0.,0.));
#19926=DIRECTION('center_axis',(0.,1.,0.));
#19927=DIRECTION('ref_axis',(1.,0.,0.));
#19928=DIRECTION('center_axis',(0.,1.,0.));
#19929=DIRECTION('ref_axis',(0.,0.,1.));
#19930=DIRECTION('center_axis',(0.,1.,0.));
#19931=DIRECTION('ref_axis',(0.,0.,1.));
#26810=CARTESIAN_POINT('',(0.,0.,0.));
#26811=CARTESIAN_POINT('Origin',(0.,-1.275,7.2));
#26812=CARTESIAN_POINT('',(-4.04133443718627E-16,-1.25,3.9));
#26813=CARTESIAN_POINT('',(-4.04133443718627E-16,-1.25,10.5));
#26814=CARTESIAN_POINT('Origin',(0.,-1.25,7.2));
#26815=CARTESIAN_POINT('',(-4.10256677714363E-16,-1.3,10.55));
#26816=CARTESIAN_POINT('',(-4.07195060716495E-16,-1.275,10.525));
#26817=CARTESIAN_POINT('Origin',(0.,-1.3,7.2));
#26818=CARTESIAN_POINT('Origin',(0.,-1.25,7.2));
#26819=CARTESIAN_POINT('Origin',(0.,0.,7.2));
#26820=CARTESIAN_POINT('',(-4.04133443718627E-16,1.25,3.9));
#26821=CARTESIAN_POINT('',(-4.04133443718627E-16,0.,3.9));
#26822=CARTESIAN_POINT('',(-4.04133443718627E-16,1.25,10.5));
#26823=CARTESIAN_POINT('Origin',(0.,1.25,7.2));
#26824=CARTESIAN_POINT('Origin',(0.,1.25,7.2));
#26825=CARTESIAN_POINT('Origin',(0.,-1.3,12.05));
#26826=CARTESIAN_POINT('',(-1.16079736048698,-1.3,11.6306327026976));
#26827=CARTESIAN_POINT('',(-1.35212230766397,-1.30000000000017,11.857710302833));
#26828=CARTESIAN_POINT('Ctrl Pts',(-1.16079736048698,-1.3,11.6306327026976));
#26829=CARTESIAN_POINT('Ctrl Pts',(-1.16756547280972,-1.3,11.6361811764316));
#26830=CARTESIAN_POINT('Ctrl Pts',(-1.17433759800592,-1.30000000000001,
11.6464116794416));
#26831=CARTESIAN_POINT('Ctrl Pts',(-1.18440586374552,-1.30000000000002,
11.6613628993828));
#26832=CARTESIAN_POINT('Ctrl Pts',(-1.19298536144484,-1.30000000000003,
11.6736347004975));
#26833=CARTESIAN_POINT('Ctrl Pts',(-1.2010525651233,-1.30000000000005,11.6846776130522));
#26834=CARTESIAN_POINT('Ctrl Pts',(-1.20689949924857,-1.30000000000005,
11.6917782430971));
#26835=CARTESIAN_POINT('Ctrl Pts',(-1.21290364438206,-1.30000000000005,
11.6988352552442));
#26836=CARTESIAN_POINT('Ctrl Pts',(-1.22618519864767,-1.30000000000005,
11.7171839141227));
#26837=CARTESIAN_POINT('Ctrl Pts',(-1.24813860795808,-1.30000000000018,
11.742992785695));
#26838=CARTESIAN_POINT('Ctrl Pts',(-1.26978166142649,-1.30000000000021,
11.7689185967307));
#26839=CARTESIAN_POINT('Ctrl Pts',(-1.28621507340024,-1.30000000000022,
11.7874440086064));
#26840=CARTESIAN_POINT('Ctrl Pts',(-1.29884778522716,-1.30000000000025,
11.8011898160839));
#26841=CARTESIAN_POINT('Ctrl Pts',(-1.30959903943822,-1.30000000000028,
11.8125295228686));
#26842=CARTESIAN_POINT('Ctrl Pts',(-1.31760194267198,-1.30000000000028,
11.8218663161003));
#26843=CARTESIAN_POINT('Ctrl Pts',(-1.33044578595539,-1.30000000000034,
11.835492648863));
#26844=CARTESIAN_POINT('Ctrl Pts',(-1.34223778779766,-1.30000000000035,
11.8472929513181));
#26845=CARTESIAN_POINT('Ctrl Pts',(-1.35147403673712,-1.30000000000039,
11.857025688592));
#26846=CARTESIAN_POINT('Ctrl Pts',(-1.3521223074938,-1.30000000000039,11.8577103026533));
#26847=CARTESIAN_POINT('',(-1.85488174067955,-1.30000000000031,11.6812848300933));
#26848=CARTESIAN_POINT('Origin',(0.,-1.3,7.2));
#26849=CARTESIAN_POINT('',(-1.84783999216022,-1.3,11.390889146273));
#26850=CARTESIAN_POINT('Ctrl Pts',(-1.85488174055135,-1.29999999999962,
11.6812848304777));
#26851=CARTESIAN_POINT('Ctrl Pts',(-1.85492628499207,-1.29999999999962,
11.6802652801082));
#26852=CARTESIAN_POINT('Ctrl Pts',(-1.85520261176984,-1.29999999999962,
11.6731568182642));
#26853=CARTESIAN_POINT('Ctrl Pts',(-1.85517328864456,-1.29999999999968,
11.6601079860047));
#26854=CARTESIAN_POINT('Ctrl Pts',(-1.85677772263879,-1.29999999999968,
11.6415847248257));
#26855=CARTESIAN_POINT('Ctrl Pts',(-1.8559372933276,-1.29999999999972,11.6267230412807));
#26856=CARTESIAN_POINT('Ctrl Pts',(-1.85699869963993,-1.29999999999972,
11.6143622964798));
#26857=CARTESIAN_POINT('Ctrl Pts',(-1.85707299808147,-1.29999999999975,
11.5962359591743));
#26858=CARTESIAN_POINT('Ctrl Pts',(-1.85782405239374,-1.29999999999978,
11.5718563713308));
#26859=CARTESIAN_POINT('Ctrl Pts',(-1.85678181360665,-1.29999999999981,
11.5479686431211));
#26860=CARTESIAN_POINT('Ctrl Pts',(-1.85646792992201,-1.29999999999983,
11.5238562660423));
#26861=CARTESIAN_POINT('Ctrl Pts',(-1.85497966222552,-1.29999999999992,
11.5031261449632));
#26862=CARTESIAN_POINT('Ctrl Pts',(-1.85439311555543,-1.29999999999991,
11.4790463022061));
#26863=CARTESIAN_POINT('Ctrl Pts',(-1.85283978068161,-1.29999999999994,
11.4613539877648));
#26864=CARTESIAN_POINT('Ctrl Pts',(-1.85127630062445,-1.29999999999995,
11.4435752287495));
#26865=CARTESIAN_POINT('Ctrl Pts',(-1.84999209718951,-1.29999999999997,
11.42887504109));
#26866=CARTESIAN_POINT('Ctrl Pts',(-1.84771283470267,-1.29999999999997,
11.411322510041));
#26867=CARTESIAN_POINT('Ctrl Pts',(-1.84624880074883,-1.3,11.3993427675272));
#26868=CARTESIAN_POINT('Ctrl Pts',(-1.84783999216022,-1.3,11.390889146273));
#26869=CARTESIAN_POINT('',(-2.05661148970878,-1.3,11.2924694059607));
#26870=CARTESIAN_POINT('',(-1.84783999216022,-1.3,11.390889146273));
#26871=CARTESIAN_POINT('',(-2.29123854954719,-1.29999999999661,11.4746609113891));
#26872=CARTESIAN_POINT('Ctrl Pts',(-2.05661148970878,-1.3,11.2924694059607));
#26873=CARTESIAN_POINT('Ctrl Pts',(-2.06438529509424,-1.3,11.2964894625547));
#26874=CARTESIAN_POINT('Ctrl Pts',(-2.07310405152088,-1.29999999999976,
11.3051109272566));
#26875=CARTESIAN_POINT('Ctrl Pts',(-2.08604767365932,-1.29999999999967,
11.3176494774367));
#26876=CARTESIAN_POINT('Ctrl Pts',(-2.09697218826213,-1.2999999999995,11.3278871439685));
#26877=CARTESIAN_POINT('Ctrl Pts',(-2.10826479557385,-1.29999999999936,
11.3380338755579));
#26878=CARTESIAN_POINT('Ctrl Pts',(-2.11798686606834,-1.29999999999925,
11.3455803565384));
#26879=CARTESIAN_POINT('Ctrl Pts',(-2.12751552334166,-1.29999999999917,
11.353305425036));
#26880=CARTESIAN_POINT('Ctrl Pts',(-2.14304910682454,-1.2999999999991,11.3675618927394));
#26881=CARTESIAN_POINT('Ctrl Pts',(-2.16816701100081,-1.29999999999791,
11.3858847423419));
#26882=CARTESIAN_POINT('Ctrl Pts',(-2.19197084033902,-1.2999999999976,11.4050757262928));
#26883=CARTESIAN_POINT('Ctrl Pts',(-2.21194072996125,-1.29999999999725,
11.4197523880556));
#26884=CARTESIAN_POINT('Ctrl Pts',(-2.22718477672532,-1.2999999999971,11.4305479831049));
#26885=CARTESIAN_POINT('Ctrl Pts',(-2.24236803062252,-1.29999999999635,
11.4413662490843));
#26886=CARTESIAN_POINT('Ctrl Pts',(-2.26249397180294,-1.29999999999583,
11.4558744789577));
#26887=CARTESIAN_POINT('Ctrl Pts',(-2.27915093949768,-1.29999999999501,
11.4666835569465));
#26888=CARTESIAN_POINT('Ctrl Pts',(-2.29043543302869,-1.29999999999466,
11.4741293822945));
#26889=CARTESIAN_POINT('Ctrl Pts',(-2.29123854934731,-1.29999999999464,
11.4746609111665));
#26890=CARTESIAN_POINT('',(-2.74606098184731,-1.30000000000043,11.1977054774281));
#26891=CARTESIAN_POINT('Origin',(0.,-1.3,7.2));
#26892=CARTESIAN_POINT('',(-2.67879510330291,-1.3,10.9151206262376));
#26893=CARTESIAN_POINT('Ctrl Pts',(-2.74606098180075,-1.30000000000052,
11.1977054778115));
#26894=CARTESIAN_POINT('Ctrl Pts',(-2.74589257547025,-1.30000000000052,
11.1966989891297));
#26895=CARTESIAN_POINT('Ctrl Pts',(-2.74468488647704,-1.30000000000052,
11.1896884723293));
#26896=CARTESIAN_POINT('Ctrl Pts',(-2.74194313468275,-1.30000000000045,
11.1769309522019));
#26897=CARTESIAN_POINT('Ctrl Pts',(-2.73966116432262,-1.30000000000044,
11.1584789426609));
#26898=CARTESIAN_POINT('Ctrl Pts',(-2.73574909450226,-1.30000000000039,
11.1441167944129));
#26899=CARTESIAN_POINT('Ctrl Pts',(-2.73421733091279,-1.30000000000039,
11.1318054961784));
#26900=CARTESIAN_POINT('Ctrl Pts',(-2.73052114637807,-1.30000000000036,
11.1140598974805));
#26901=CARTESIAN_POINT('Ctrl Pts',(-2.72618669292026,-1.3000000000003,11.0900570416951));
#26902=CARTESIAN_POINT('Ctrl Pts',(-2.72020047826994,-1.30000000000025,
11.0669081106693));
#26903=CARTESIAN_POINT('Ctrl Pts',(-2.71488010558258,-1.30000000000023,
11.0433879560159));
#26904=CARTESIAN_POINT('Ctrl Pts',(-2.70911402584219,-1.30000000000012,
11.0234204248471));
#26905=CARTESIAN_POINT('Ctrl Pts',(-2.70353383063923,-1.30000000000011,
10.9999887293472));
#26906=CARTESIAN_POINT('Ctrl Pts',(-2.69833596654804,-1.30000000000008,
10.983006039634));
#26907=CARTESIAN_POINT('Ctrl Pts',(-2.69311023072124,-1.30000000000006,
10.9659408795863));
#26908=CARTESIAN_POINT('Ctrl Pts',(-2.6887977871431,-1.30000000000005,10.9518289492138));
#26909=CARTESIAN_POINT('Ctrl Pts',(-2.6829189620321,-1.30000000000003,10.9351338813408));
#26910=CARTESIAN_POINT('Ctrl Pts',(-2.67899628993004,-1.3,10.9237203428817));
#26911=CARTESIAN_POINT('Ctrl Pts',(-2.67879510330291,-1.3,10.9151206262376));
#26912=CARTESIAN_POINT('',(-2.86254182811346,-1.3,10.7754455583364));
#26913=CARTESIAN_POINT('',(-2.67879510330291,-1.3,10.9151206262376));
#26914=CARTESIAN_POINT('',(-3.12979327626143,-1.29999999999956,10.9049823276056));
#26915=CARTESIAN_POINT('Ctrl Pts',(-2.86254182811346,-1.3,10.7754455583364));
#26916=CARTESIAN_POINT('Ctrl Pts',(-2.87098157396347,-1.3,10.7777615020268));
#26917=CARTESIAN_POINT('Ctrl Pts',(-2.88130799910635,-1.29999999999995,
10.7843752712055));
#26918=CARTESIAN_POINT('Ctrl Pts',(-2.89657675896672,-1.29999999999994,
10.7939475114029));
#26919=CARTESIAN_POINT('Ctrl Pts',(-2.90939733936898,-1.29999999999989,
10.8016830781138));
#26920=CARTESIAN_POINT('Ctrl Pts',(-2.92255067730088,-1.29999999999988,
10.8092626647234));
#26921=CARTESIAN_POINT('Ctrl Pts',(-2.93364134797163,-1.29999999999984,
10.8146096561709));
#26922=CARTESIAN_POINT('Ctrl Pts',(-2.94454127932451,-1.29999999999984,
10.8202105050095));
#26923=CARTESIAN_POINT('Ctrl Pts',(-2.96280984633302,-1.29999999999977,
10.8308072518358));
#26924=CARTESIAN_POINT('Ctrl Pts',(-2.99104878850524,-1.29999999999969,
10.8436673431889));
#26925=CARTESIAN_POINT('Ctrl Pts',(-3.01834269857632,-1.29999999999954,
10.8574591123471));
#26926=CARTESIAN_POINT('Ctrl Pts',(-3.04099809512408,-1.29999999999947,
10.8675872666515));
#26927=CARTESIAN_POINT('Ctrl Pts',(-3.05375053744491,-1.29999999999936,
10.8732488581604));
#26928=CARTESIAN_POINT('Ctrl Pts',(-3.06242055860219,-1.29999999999936,
10.8768361729214));
#26929=CARTESIAN_POINT('Ctrl Pts',(-3.06815466520311,-1.29999999999934,
10.879276631911));
#26930=CARTESIAN_POINT('Ctrl Pts',(-3.07523784637398,-1.29999999999934,
10.8824189159387));
#26931=CARTESIAN_POINT('Ctrl Pts',(-3.0835896561049,-1.29999999999931,10.8863527724723));
#26932=CARTESIAN_POINT('Ctrl Pts',(-3.10080971693874,-1.29999999999922,
10.893634162511));
#26933=CARTESIAN_POINT('Ctrl Pts',(-3.11640268293853,-1.29999999999909,
10.899617481341));
#26934=CARTESIAN_POINT('Ctrl Pts',(-3.12890931112008,-1.29999999999898,
10.9046274841548));
#26935=CARTESIAN_POINT('Ctrl Pts',(-3.12979327620054,-1.29999999999897,
10.9049823275812));
#26936=CARTESIAN_POINT('',(-3.51715555718115,-1.30000000000215,10.5394702475537));
#26937=CARTESIAN_POINT('Origin',(0.,-1.3,7.2));
#26938=CARTESIAN_POINT('',(-3.39267401414619,-1.3,10.2769835077089));
#26939=CARTESIAN_POINT('Ctrl Pts',(-3.51715323192894,-1.30000000000206,
10.5394644239228));
#26940=CARTESIAN_POINT('Ctrl Pts',(-3.5167751163261,-1.30000000000204,10.5385174606946));
#26941=CARTESIAN_POINT('Ctrl Pts',(-3.51412021591145,-1.30000000000197,
10.5319251070686));
#26942=CARTESIAN_POINT('Ctrl Pts',(-3.51014479419029,-1.30000000000177,
10.5226552577284));
#26943=CARTESIAN_POINT('Ctrl Pts',(-3.50627111332769,-1.30000000000177,
10.51267580137));
#26944=CARTESIAN_POINT('Ctrl Pts',(-3.50442220663016,-1.30000000000176,
10.5076132694342));
#26945=CARTESIAN_POINT('Ctrl Pts',(-3.50332286786836,-1.30000000000176,
10.5047548383451));
#26946=CARTESIAN_POINT('Ctrl Pts',(-3.49802816243003,-1.30000000000167,
10.4921711193908));
#26947=CARTESIAN_POINT('Ctrl Pts',(-3.48397706310364,-1.30000000000133,
10.4576138699548));
#26948=CARTESIAN_POINT('Ctrl Pts',(-3.46377916361693,-1.30000000000061,
10.4138557361379));
#26949=CARTESIAN_POINT('Ctrl Pts',(-3.44488287358282,-1.30000000000045,
10.3765723257512));
#26950=CARTESIAN_POINT('Ctrl Pts',(-3.43444272475379,-1.30000000000036,
10.3549066020539));
#26951=CARTESIAN_POINT('Ctrl Pts',(-3.4258722715172,-1.30000000000023,10.3393534519172));
#26952=CARTESIAN_POINT('Ctrl Pts',(-3.41721009436118,-1.30000000000019,
10.3237432942191));
#26953=CARTESIAN_POINT('Ctrl Pts',(-3.41007224859402,-1.30000000000012,
10.3108264414936));
#26954=CARTESIAN_POINT('Ctrl Pts',(-3.4008540684495,-1.30000000000008,10.2957145443332));
#26955=CARTESIAN_POINT('Ctrl Pts',(-3.39465878599086,-1.3,10.2853534708595));
#26956=CARTESIAN_POINT('Ctrl Pts',(-3.39267401414619,-1.3,10.2769835077089));
#26957=CARTESIAN_POINT('',(-3.54336535262991,-1.3,10.1021575829215));
#26958=CARTESIAN_POINT('',(-3.39267401414619,-1.3,10.2769835077089));
#26959=CARTESIAN_POINT('',(-3.83170332429324,-1.30000000000003,10.1733061790875));
#26960=CARTESIAN_POINT('Ctrl Pts',(-3.54336535262991,-1.3,10.1021575829215));
#26961=CARTESIAN_POINT('Ctrl Pts',(-3.55210218155242,-1.3,10.1026681958559));
#26962=CARTESIAN_POINT('Ctrl Pts',(-3.56359990094073,-1.3,10.1069613837583));
#26963=CARTESIAN_POINT('Ctrl Pts',(-3.58052453593301,-1.3,10.1131512829018));
#26964=CARTESIAN_POINT('Ctrl Pts',(-3.5947099922829,-1.30000000000002,10.1179996604393));
#26965=CARTESIAN_POINT('Ctrl Pts',(-3.6091175106494,-1.30000000000001,10.122729572639));
#26966=CARTESIAN_POINT('Ctrl Pts',(-3.62418184228238,-1.30000000000001,
10.1262166523165));
#26967=CARTESIAN_POINT('Ctrl Pts',(-3.64724297519883,-1.30000000000001,
10.1335969392187));
#26968=CARTESIAN_POINT('Ctrl Pts',(-3.67397691592533,-1.30000000000002,
10.1404382070294));
#26969=CARTESIAN_POINT('Ctrl Pts',(-3.70101609997419,-1.30000000000003,
10.1467971727461));
#26970=CARTESIAN_POINT('Ctrl Pts',(-3.71878759513276,-1.30000000000003,
10.1514335393157));
#26971=CARTESIAN_POINT('Ctrl Pts',(-3.73401038434217,-1.30000000000004,
10.1545818971217));
#26972=CARTESIAN_POINT('Ctrl Pts',(-3.74458338262459,-1.30000000000004,
10.1569162443582));
#26973=CARTESIAN_POINT('Ctrl Pts',(-3.75070071224819,-1.30000000000004,
10.1581177840759));
#26974=CARTESIAN_POINT('Ctrl Pts',(-3.76607211082019,-1.30000000000004,
10.1609742455453));
#26975=CARTESIAN_POINT('Ctrl Pts',(-3.79159121371509,-1.30000000000004,
10.166868855423));
#26976=CARTESIAN_POINT('Ctrl Pts',(-3.81751020820494,-1.30000000000005,
10.1708055317158));
#26977=CARTESIAN_POINT('Ctrl Pts',(-3.83076636902639,-1.30000000000006,
10.1731399950341));
#26978=CARTESIAN_POINT('Ctrl Pts',(-3.83170332419124,-1.30000000000006,
10.1733061790695));
#26979=CARTESIAN_POINT('',(-4.13458745388079,-1.30000000000005,9.73526890803374));
#26980=CARTESIAN_POINT('Origin',(0.,-1.3,7.2));
#26981=CARTESIAN_POINT('',(-3.95827679071515,-1.3,9.50436744488836));
#26982=CARTESIAN_POINT('Ctrl Pts',(-4.13458133514455,-1.30000000000001,
9.73525952971052));
#26983=CARTESIAN_POINT('Ctrl Pts',(-4.13402211860173,-1.30000000000001,
9.73440240093009));
#26984=CARTESIAN_POINT('Ctrl Pts',(-4.12678253409857,-1.30000000000001,
9.7232969089459));
#26985=CARTESIAN_POINT('Ctrl Pts',(-4.11635470812671,-1.30000000000001,
9.70687190739251));
#26986=CARTESIAN_POINT('Ctrl Pts',(-4.10202300360556,-1.30000000000001,
9.68751099507706));
#26987=CARTESIAN_POINT('Ctrl Pts',(-4.0922355048406,-1.30000000000001,9.6718006770301));
#26988=CARTESIAN_POINT('Ctrl Pts',(-4.08088288391458,-1.29999999999999,
9.65800792817637));
#26989=CARTESIAN_POINT('Ctrl Pts',(-4.07272838886398,-1.3,9.64488009164316));
#26990=CARTESIAN_POINT('Ctrl Pts',(-4.06138621253064,-1.3,9.63106202969796));
#26991=CARTESIAN_POINT('Ctrl Pts',(-4.04716422159604,-1.3,9.61149186781034));
#26992=CARTESIAN_POINT('Ctrl Pts',(-4.02999794901947,-1.3,9.59094278729833));
#26993=CARTESIAN_POINT('Ctrl Pts',(-4.01715577671304,-1.3,9.57427610753465));
#26994=CARTESIAN_POINT('Ctrl Pts',(-4.01049046738455,-1.3,9.56625472662842));
#26995=CARTESIAN_POINT('Ctrl Pts',(-4.00659335599276,-1.3,9.56178696274009));
#26996=CARTESIAN_POINT('Ctrl Pts',(-4.00072166766439,-1.3,9.55514362730498));
#26997=CARTESIAN_POINT('Ctrl Pts',(-3.99198996060064,-1.3,9.54496247330593));
#26998=CARTESIAN_POINT('Ctrl Pts',(-3.98223602054924,-1.3,9.53389065551681));
#26999=CARTESIAN_POINT('Ctrl Pts',(-3.97422670435759,-1.3,9.52527149172313));
#27000=CARTESIAN_POINT('Ctrl Pts',(-3.96589174422145,-1.3,9.51663189767497));
#27001=CARTESIAN_POINT('Ctrl Pts',(-3.96073119938755,-1.3,9.50955037962426));
#27002=CARTESIAN_POINT('Ctrl Pts',(-3.95827679071515,-1.3,9.50436744488836));
#27003=CARTESIAN_POINT('',(-4.06932680828303,-1.3,9.30203139503569));
#27004=CARTESIAN_POINT('',(-3.95827679071515,-1.3,9.50436744488836));
#27005=CARTESIAN_POINT('',(-4.36615556544121,-1.29999999999999,9.31167837948083));
#27006=CARTESIAN_POINT('Ctrl Pts',(-4.06932680828303,-1.3,9.30203139503569));
#27007=CARTESIAN_POINT('Ctrl Pts',(-4.07797887893014,-1.3,9.30071436097879));
#27008=CARTESIAN_POINT('Ctrl Pts',(-4.09011797873215,-1.3,9.30252364569424));
#27009=CARTESIAN_POINT('Ctrl Pts',(-4.10795972277923,-1.3,9.30505955869223));
#27010=CARTESIAN_POINT('Ctrl Pts',(-4.12284323459949,-1.3,9.30685293138333));
#27011=CARTESIAN_POINT('Ctrl Pts',(-4.13791931153359,-1.3,9.30848411321574));
#27012=CARTESIAN_POINT('Ctrl Pts',(-4.15337942684459,-1.3,9.30876317496534));
#27013=CARTESIAN_POINT('Ctrl Pts',(-4.177471105744,-1.3,9.3111874364075));
#27014=CARTESIAN_POINT('Ctrl Pts',(-4.2050428800799,-1.29999999999999,9.31232210003487));
#27015=CARTESIAN_POINT('Ctrl Pts',(-4.23281323594795,-1.29999999999999,
9.31292054619228));
#27016=CARTESIAN_POINT('Ctrl Pts',(-4.25116029379092,-1.29999999999997,
9.31376081103432));
#27017=CARTESIAN_POINT('Ctrl Pts',(-4.26670499109767,-1.29999999999998,
9.31367542306717));
#27018=CARTESIAN_POINT('Ctrl Pts',(-4.27753228080538,-1.29999999999998,
9.31376050379772));
#27019=CARTESIAN_POINT('Ctrl Pts',(-4.28376574468317,-1.29999999999998,
9.31366392579328));
#27020=CARTESIAN_POINT('Ctrl Pts',(-4.29939513404249,-1.29999999999998,
9.31326205030653));
#27021=CARTESIAN_POINT('Ctrl Pts',(-4.32558216921343,-1.29999999999998,
9.31372186269267));
#27022=CARTESIAN_POINT('Ctrl Pts',(-4.35175307577712,-1.29999999999997,
9.31218345558017));
#27023=CARTESIAN_POINT('Ctrl Pts',(-4.36520473933644,-1.29999999999997,
9.31171063592312));
#27024=CARTESIAN_POINT('Ctrl Pts',(-4.36615556533234,-1.29999999999997,
9.31167837948453));
#27025=CARTESIAN_POINT('',(-4.57138092645551,-1.29999999999936,8.82016913292346));
#27026=CARTESIAN_POINT('Origin',(0.,-1.3,7.2));
#27027=CARTESIAN_POINT('',(-4.35088387761047,-1.3,8.63103946714436));
#27028=CARTESIAN_POINT('Ctrl Pts',(-4.57137830133415,-1.29999999999872,
8.82016777346892));
#27029=CARTESIAN_POINT('Ctrl Pts',(-4.5706499710557,-1.29999999999873,8.81945142449021));
#27030=CARTESIAN_POINT('Ctrl Pts',(-4.56555294905792,-1.2999999999988,8.81448624478641));
#27031=CARTESIAN_POINT('Ctrl Pts',(-4.55583799175273,-1.29999999999884,
8.80577096598508));
#27032=CARTESIAN_POINT('Ctrl Pts',(-4.54314694081162,-1.29999999999898,
8.79218277495142));
#27033=CARTESIAN_POINT('Ctrl Pts',(-4.53154583913746,-1.29999999999902,
8.78285112053941));
#27034=CARTESIAN_POINT('Ctrl Pts',(-4.5230641316617,-1.29999999999905,8.77380443519591));
#27035=CARTESIAN_POINT('Ctrl Pts',(-4.50966808728349,-1.29999999999912,
8.76156795041169));
#27036=CARTESIAN_POINT('Ctrl Pts',(-4.48972114667047,-1.29999999999927,
8.7428644163535));
#27037=CARTESIAN_POINT('Ctrl Pts',(-4.46225757065887,-1.29999999999944,
8.71958453597246));
#27038=CARTESIAN_POINT('Ctrl Pts',(-4.43911310247342,-1.29999999999973,
8.70074230118687));
#27039=CARTESIAN_POINT('Ctrl Pts',(-4.42075431675779,-1.29999999999974,
8.68521657502575));
#27040=CARTESIAN_POINT('Ctrl Pts',(-4.4065970852679,-1.29999999999981,8.6744687837598));
#27041=CARTESIAN_POINT('Ctrl Pts',(-4.39232901723895,-1.29999999999987,
8.663754809807));
#27042=CARTESIAN_POINT('Ctrl Pts',(-4.38055136998726,-1.29999999999991,
8.65486034483265));
#27043=CARTESIAN_POINT('Ctrl Pts',(-4.36598120515464,-1.29999999999993,
8.64481132314781));
#27044=CARTESIAN_POINT('Ctrl Pts',(-4.35610142762816,-1.3,8.63787852952385));
#27045=CARTESIAN_POINT('Ctrl Pts',(-4.35088387761047,-1.3,8.63103946714436));
#27046=CARTESIAN_POINT('',(-4.41743915561768,-1.3,8.41003634852114));
#27047=CARTESIAN_POINT('',(-4.35088387761047,-1.3,8.63103946714436));
#27048=CARTESIAN_POINT('',(-4.70981757133242,-1.29999999999615,8.35763484922072));
#27049=CARTESIAN_POINT('Ctrl Pts',(-4.41743915561768,-1.3,8.41003634852114));
#27050=CARTESIAN_POINT('Ctrl Pts',(-4.42289860586251,-1.3,8.40797826829437));
#27051=CARTESIAN_POINT('Ctrl Pts',(-4.4316817112443,-1.29999999999974,8.40635777334174));
#27052=CARTESIAN_POINT('Ctrl Pts',(-4.44386598092803,-1.29999999999974,
8.40580624828125));
#27053=CARTESIAN_POINT('Ctrl Pts',(-4.45581389180353,-1.29999999999952,
8.40486348086199));
#27054=CARTESIAN_POINT('Ctrl Pts',(-4.47075640156682,-1.29999999999934,
8.4036633250798));
#27055=CARTESIAN_POINT('Ctrl Pts',(-4.48584345896485,-1.29999999999907,
8.40202163820225));
#27056=CARTESIAN_POINT('Ctrl Pts',(-4.49796178305987,-1.29999999999891,
8.39985529775274));
#27057=CARTESIAN_POINT('Ctrl Pts',(-4.51007860939437,-1.29999999999879,
8.39793835227947));
#27058=CARTESIAN_POINT('Ctrl Pts',(-4.53106911976877,-1.29999999999867,
8.39593541505635));
#27059=CARTESIAN_POINT('Ctrl Pts',(-4.56150565653829,-1.29999999999687,
8.3894994098264));
#27060=CARTESIAN_POINT('Ctrl Pts',(-4.5916993973255,-1.29999999999631,8.38463466234546));
#27061=CARTESIAN_POINT('Ctrl Pts',(-4.6159708325463,-1.29999999999587,8.37961235158075));
#27062=CARTESIAN_POINT('Ctrl Pts',(-4.63419695389511,-1.29999999999542,
8.37547771778002));
#27063=CARTESIAN_POINT('Ctrl Pts',(-4.65239690742476,-1.29999999999488,
8.37146876966047));
#27064=CARTESIAN_POINT('Ctrl Pts',(-4.67662765556342,-1.29999999999398,
8.36638064005625));
#27065=CARTESIAN_POINT('Ctrl Pts',(-4.69579249083398,-1.29999999999256,
8.36144353805949));
#27066=CARTESIAN_POINT('Ctrl Pts',(-4.70888530574064,-1.29999999999208,
8.35788592377707));
#27067=CARTESIAN_POINT('Ctrl Pts',(-4.70981757125868,-1.29999999999204,
8.3576348491941));
#27068=CARTESIAN_POINT('',(-4.80833510396185,-1.3000000000003,7.83433302999821));
#27069=CARTESIAN_POINT('Origin',(0.,-1.3,7.2));
#27070=CARTESIAN_POINT('',(-4.55333646119701,-1.3,7.69516819779691));
#27071=CARTESIAN_POINT('Ctrl Pts',(-4.80833173373481,-1.30000000000022,
7.83433088232518));
#27072=CARTESIAN_POINT('Ctrl Pts',(-4.80747027295148,-1.30000000000022,
7.83378193252291));
#27073=CARTESIAN_POINT('Ctrl Pts',(-4.80145165647202,-1.30000000000022,
7.82998687887007));
#27074=CARTESIAN_POINT('Ctrl Pts',(-4.79013869260298,-1.30000000000018,
7.82347634664022));
#27075=CARTESIAN_POINT('Ctrl Pts',(-4.77489914987298,-1.30000000000019,
7.81282546636897));
#27076=CARTESIAN_POINT('Ctrl Pts',(-4.76161182290262,-1.30000000000016,
7.80610825536316));
#27077=CARTESIAN_POINT('Ctrl Pts',(-4.75143447025795,-1.30000000000017,
7.79902289403953));
#27078=CARTESIAN_POINT('Ctrl Pts',(-4.7357871929817,-1.30000000000014,7.78983839804539));
#27079=CARTESIAN_POINT('Ctrl Pts',(-4.71238759485038,-1.30000000000014,
7.77568997553474));
#27080=CARTESIAN_POINT('Ctrl Pts',(-4.68068425748567,-1.30000000000009,
7.75862761062045));
#27081=CARTESIAN_POINT('Ctrl Pts',(-4.65412859982376,-1.30000000000005,
7.74500676190757));
#27082=CARTESIAN_POINT('Ctrl Pts',(-4.63294304514747,-1.30000000000005,
7.73363723320237));
#27083=CARTESIAN_POINT('Ctrl Pts',(-4.61686083285171,-1.30000000000004,
7.72606704168879));
#27084=CARTESIAN_POINT('Ctrl Pts',(-4.60067713755889,-1.30000000000003,
7.71855328487673));
#27085=CARTESIAN_POINT('Ctrl Pts',(-4.58730781279961,-1.30000000000002,
7.71230138859932));
#27086=CARTESIAN_POINT('Ctrl Pts',(-4.57096682812081,-1.3,7.70550102152382));
#27087=CARTESIAN_POINT('Ctrl Pts',(-4.55986191625143,-1.3,7.70077302060858));
#27088=CARTESIAN_POINT('Ctrl Pts',(-4.55333646119701,-1.3,7.69516819779691));
#27089=CARTESIAN_POINT('',(-4.57248821462698,-1.3,7.4651569071776));
#27090=CARTESIAN_POINT('',(-4.55333646119701,-1.3,7.69516819779691));
#27091=CARTESIAN_POINT('',(-4.84757993445123,-1.30000000000002,7.35319523199426));
#27092=CARTESIAN_POINT('Ctrl Pts',(-4.57248821462698,-1.3,7.4651569071776));
#27093=CARTESIAN_POINT('Ctrl Pts',(-4.57985658845472,-1.3,7.46043462252668));
#27094=CARTESIAN_POINT('Ctrl Pts',(-4.59168342474763,-1.3,7.45718163914689));
#27095=CARTESIAN_POINT('Ctrl Pts',(-4.60901429870377,-1.3,7.45223840664112));
#27096=CARTESIAN_POINT('Ctrl Pts',(-4.6233426492548,-1.3,7.44788165467972));
#27097=CARTESIAN_POINT('Ctrl Pts',(-4.63777744145292,-1.30000000000001,
7.44317884815646));
#27098=CARTESIAN_POINT('Ctrl Pts',(-4.64917211308579,-1.30000000000001,
7.43850439917718));
#27099=CARTESIAN_POINT('Ctrl Pts',(-4.66062967398901,-1.30000000000001,
7.4341698631728));
#27100=CARTESIAN_POINT('Ctrl Pts',(-4.68072279072001,-1.30000000000001,
7.427597316889));
#27101=CARTESIAN_POINT('Ctrl Pts',(-4.72058200346441,-1.30000000000001,
7.41055955717716));
#27102=CARTESIAN_POINT('Ctrl Pts',(-4.75619240536045,-1.30000000000002,
7.39667294505808));
#27103=CARTESIAN_POINT('Ctrl Pts',(-4.78159245634837,-1.30000000000002,
7.3845295394818));
#27104=CARTESIAN_POINT('Ctrl Pts',(-4.78724263544855,-1.30000000000002,
7.38189848275632));
#27105=CARTESIAN_POINT('Ctrl Pts',(-4.79573463031575,-1.30000000000002,
7.37812243727754));
#27106=CARTESIAN_POINT('Ctrl Pts',(-4.80424392564078,-1.30000000000002,
7.37453487689564));
#27107=CARTESIAN_POINT('Ctrl Pts',(-4.82116392366521,-1.30000000000002,
7.3664890641967));
#27108=CARTESIAN_POINT('Ctrl Pts',(-4.83462057271346,-1.30000000000004,
7.35948972770122));
#27109=CARTESIAN_POINT('Ctrl Pts',(-4.84672316806408,-1.30000000000005,
7.35361004877818));
#27110=CARTESIAN_POINT('Ctrl Pts',(-4.84757993437554,-1.30000000000005,
7.3531952320309));
#27111=CARTESIAN_POINT('',(-4.83515073502711,-1.30000000000003,6.82076739205056));
#27112=CARTESIAN_POINT('Origin',(0.,-1.3,7.2));
#27113=CARTESIAN_POINT('',(-4.55678639209675,-1.3,6.73765570212511));
#27114=CARTESIAN_POINT('Ctrl Pts',(-4.83515073557977,-1.30000000000001,
6.82076739235878));
#27115=CARTESIAN_POINT('Ctrl Pts',(-4.83419429812713,-1.30000000000001,
6.82040545606944));
#27116=CARTESIAN_POINT('Ctrl Pts',(-4.82180430644273,-1.30000000000001,
6.81574194544304));
#27117=CARTESIAN_POINT('Ctrl Pts',(-4.79795229094081,-1.29999999999999,
6.80742687526405));
#27118=CARTESIAN_POINT('Ctrl Pts',(-4.77218237162954,-1.3,6.79773450848217));
#27119=CARTESIAN_POINT('Ctrl Pts',(-4.75492703857423,-1.3,6.79270521874687));
#27120=CARTESIAN_POINT('Ctrl Pts',(-4.74343177047669,-1.3,6.78894839353199));
#27121=CARTESIAN_POINT('Ctrl Pts',(-4.72910106576434,-1.3,6.78356480038482));
#27122=CARTESIAN_POINT('Ctrl Pts',(-4.71179979755839,-1.3,6.77906526523394));
#27123=CARTESIAN_POINT('Ctrl Pts',(-4.6859192007466,-1.3,6.77087890474239));
#27124=CARTESIAN_POINT('Ctrl Pts',(-4.65706796695327,-1.3,6.76297007363099));
#27125=CARTESIAN_POINT('Ctrl Pts',(-4.62824128498159,-1.3,6.75514249224118));
#27126=CARTESIAN_POINT('Ctrl Pts',(-4.60795779379671,-1.3,6.75077046400056));
#27127=CARTESIAN_POINT('Ctrl Pts',(-4.59357758309321,-1.3,6.7473262596935));
#27128=CARTESIAN_POINT('Ctrl Pts',(-4.57618074025563,-1.3,6.74410801342416));
#27129=CARTESIAN_POINT('Ctrl Pts',(-4.56433455848945,-1.3,6.74178132771716));
#27130=CARTESIAN_POINT('Ctrl Pts',(-4.55678639209675,-1.3,6.73765570212511));
#27131=CARTESIAN_POINT('',(-4.52769759742429,-1.3,6.50868883662639));
#27132=CARTESIAN_POINT('',(-4.55678639209675,-1.3,6.73765570212511));
#27133=CARTESIAN_POINT('',(-4.77349769916151,-1.30000000000004,6.34196753202475));
#27134=CARTESIAN_POINT('Ctrl Pts',(-4.52769759742428,-1.3,6.50868883662639));
#27135=CARTESIAN_POINT('Ctrl Pts',(-4.53392313641892,-1.3,6.50253777416401));
#27136=CARTESIAN_POINT('Ctrl Pts',(-4.54481358953488,-1.3,6.49689772508412));
#27137=CARTESIAN_POINT('Ctrl Pts',(-4.56073742191181,-1.30000000000001,
6.48845909030186));
#27138=CARTESIAN_POINT('Ctrl Pts',(-4.57384637687987,-1.30000000000001,
6.48122083117138));
#27139=CARTESIAN_POINT('Ctrl Pts',(-4.58698656110021,-1.30000000000001,
6.47361713730408));
#27140=CARTESIAN_POINT('Ctrl Pts',(-4.5971617191533,-1.30000000000001,6.46668272213463));
#27141=CARTESIAN_POINT('Ctrl Pts',(-4.60746225289102,-1.30000000000001,
6.46004353502867));
#27142=CARTESIAN_POINT('Ctrl Pts',(-4.62576982567744,-1.30000000000001,
6.449508799198));
#27143=CARTESIAN_POINT('Ctrl Pts',(-4.65102959463077,-1.30000000000003,
6.43149214233013));
#27144=CARTESIAN_POINT('Ctrl Pts',(-4.67660141835911,-1.30000000000004,
6.4146923842508));
#27145=CARTESIAN_POINT('Ctrl Pts',(-4.69671938666191,-1.30000000000004,
6.40019410542733));
#27146=CARTESIAN_POINT('Ctrl Pts',(-4.70923780804923,-1.30000000000005,
6.39102177259885));
#27147=CARTESIAN_POINT('Ctrl Pts',(-4.71915423906947,-1.30000000000005,
6.38338868641418));
#27148=CARTESIAN_POINT('Ctrl Pts',(-4.72667488592069,-1.30000000000005,
6.37792955793699));
#27149=CARTESIAN_POINT('Ctrl Pts',(-4.73425539759128,-1.30000000000006,
6.37265708709588));
#27150=CARTESIAN_POINT('Ctrl Pts',(-4.74915526276079,-1.30000000000005,
6.36133152319305));
#27151=CARTESIAN_POINT('Ctrl Pts',(-4.76218569011346,-1.30000000000008,
6.35098992646152));
#27152=CARTESIAN_POINT('Ctrl Pts',(-4.77274896536852,-1.30000000000009,
6.34256409538153));
#27153=CARTESIAN_POINT('Ctrl Pts',(-4.77349769914136,-1.30000000000009,
6.34196753204081));
#27154=CARTESIAN_POINT('',(-4.65066919172074,-1.3000000000019,5.8238996459718));
#27155=CARTESIAN_POINT('Origin',(0.,-1.3,7.2));
#27156=CARTESIAN_POINT('',(-4.36108289177477,-1.3,5.80034987084453));
#27157=CARTESIAN_POINT('Ctrl Pts',(-4.65065521504301,-1.30000000000123,
5.82389742331003));
#27158=CARTESIAN_POINT('Ctrl Pts',(-4.64964365411225,-1.30000000000123,
5.82373656278459));
#27159=CARTESIAN_POINT('Ctrl Pts',(-4.63654304374248,-1.30000000000123,
5.82165956670231));
#27160=CARTESIAN_POINT('Ctrl Pts',(-4.61140095727319,-1.30000000000098,
5.81803205132024));
#27161=CARTESIAN_POINT('Ctrl Pts',(-4.57222382486577,-1.30000000000091,
5.81294014075723));
#27162=CARTESIAN_POINT('Ctrl Pts',(-4.54217763126687,-1.30000000000045,
5.80967119057755));
#27163=CARTESIAN_POINT('Ctrl Pts',(-4.51828305614626,-1.30000000000046,
5.8081247804399));
#27164=CARTESIAN_POINT('Ctrl Pts',(-4.49429427127261,-1.30000000000038,
5.80593985674244));
#27165=CARTESIAN_POINT('Ctrl Pts',(-4.46442169461025,-1.30000000000015,
5.80418837180128));
#27166=CARTESIAN_POINT('Ctrl Pts',(-4.43460530968231,-1.30000000000015,
5.80256316172568));
#27167=CARTESIAN_POINT('Ctrl Pts',(-4.41385708995417,-1.30000000000008,
5.80251373424002));
#27168=CARTESIAN_POINT('Ctrl Pts',(-4.39907707321173,-1.30000000000007,
5.80214342814169));
#27169=CARTESIAN_POINT('Ctrl Pts',(-4.38139208292371,-1.30000000000003,
5.80261733027065));
#27170=CARTESIAN_POINT('Ctrl Pts',(-4.36932387841423,-1.3,5.80281598958163));
#27171=CARTESIAN_POINT('Ctrl Pts',(-4.36108289177477,-1.3,5.80034987084453));
#27172=CARTESIAN_POINT('',(-4.28502486891058,-1.3,5.58243438119362));
#27173=CARTESIAN_POINT('',(-4.36108289177477,-1.3,5.80034987084453));
#27174=CARTESIAN_POINT('',(-4.49074858706858,-1.30000000000336,5.36815088613614));
#27175=CARTESIAN_POINT('Ctrl Pts',(-4.28502486891058,-1.3,5.58243438119362));
#27176=CARTESIAN_POINT('Ctrl Pts',(-4.28983548714458,-1.3,5.57512337186545));
#27177=CARTESIAN_POINT('Ctrl Pts',(-4.29926460392035,-1.30000000000005,
5.56730754668058));
#27178=CARTESIAN_POINT('Ctrl Pts',(-4.31087898979562,-1.30000000000006,
5.55775119234793));
#27179=CARTESIAN_POINT('Ctrl Pts',(-4.31756355119799,-1.30000000000007,
5.55178320730578));
#27180=CARTESIAN_POINT('Ctrl Pts',(-4.32673222276919,-1.30000000000009,
5.54396284373672));
#27181=CARTESIAN_POINT('Ctrl Pts',(-4.33567044487514,-1.30000000000012,
5.53578209594158));
#27182=CARTESIAN_POINT('Ctrl Pts',(-4.34632504743019,-1.30000000000015,
5.52463757271538));
#27183=CARTESIAN_POINT('Ctrl Pts',(-4.35515498779034,-1.30000000000018,
5.51626230029439));
#27184=CARTESIAN_POINT('Ctrl Pts',(-4.37078301239806,-1.30000000000019,
5.50197740006243));
#27185=CARTESIAN_POINT('Ctrl Pts',(-4.3895491469188,-1.30000000000043,5.48121690616271));
#27186=CARTESIAN_POINT('Ctrl Pts',(-4.41112472456535,-1.30000000000049,
5.45954571059707));
#27187=CARTESIAN_POINT('Ctrl Pts',(-4.42782422204148,-1.30000000000057,
5.44124473191616));
#27188=CARTESIAN_POINT('Ctrl Pts',(-4.44012243041892,-1.3000000000006,5.42715703615339));
#27189=CARTESIAN_POINT('Ctrl Pts',(-4.45464562208433,-1.30000000000083,
5.41105919281666));
#27190=CARTESIAN_POINT('Ctrl Pts',(-4.47094525801375,-1.30000000000091,
5.3921662715124));
#27191=CARTESIAN_POINT('Ctrl Pts',(-4.48355136291131,-1.30000000000109,
5.37693009060612));
#27192=CARTESIAN_POINT('Ctrl Pts',(-4.49013572864496,-1.30000000000116,
5.36889672578802));
#27193=CARTESIAN_POINT('Ctrl Pts',(-4.49074754412175,-1.30000000000116,
5.36815157839931));
#27194=CARTESIAN_POINT('',(-4.26288026203271,-1.30000000000046,4.88691723606622));
#27195=CARTESIAN_POINT('Origin',(0.,-1.3,7.2));
#27196=CARTESIAN_POINT('',(-3.97477914228473,-1.3,4.92421546647452));
#27197=CARTESIAN_POINT('Ctrl Pts',(-4.26288026262664,-1.30000000000002,
4.88691723612453));
#27198=CARTESIAN_POINT('Ctrl Pts',(-4.26185925374181,-1.30000000000002,
4.88697560743987));
#27199=CARTESIAN_POINT('Ctrl Pts',(-4.24864351689439,-1.30000000000002,
4.88775469182251));
#27200=CARTESIAN_POINT('Ctrl Pts',(-4.22347137391457,-1.30000000000002,
4.8898598443532));
#27201=CARTESIAN_POINT('Ctrl Pts',(-4.19598697828258,-1.30000000000001,
4.89148680791329));
#27202=CARTESIAN_POINT('Ctrl Pts',(-4.17817781145144,-1.30000000000001,
4.89391064073123));
#27203=CARTESIAN_POINT('Ctrl Pts',(-4.16614832183902,-1.30000000000001,
4.89515416503415));
#27204=CARTESIAN_POINT('Ctrl Pts',(-4.15086691685344,-1.30000000000001,
4.89606494834232));
#27205=CARTESIAN_POINT('Ctrl Pts',(-4.13323139050141,-1.30000000000001,
4.89899172467465));
#27206=CARTESIAN_POINT('Ctrl Pts',(-4.10625889988789,-1.30000000000001,
4.90204030255357));
#27207=CARTESIAN_POINT('Ctrl Pts',(-4.07668616191853,-1.30000000000001,
4.90655222883004));
#27208=CARTESIAN_POINT('Ctrl Pts',(-4.04716803737915,-1.30000000000001,
4.9111262375198));
#27209=CARTESIAN_POINT('Ctrl Pts',(-4.02686024311824,-1.30000000000001,
4.91538283693502));
#27210=CARTESIAN_POINT('Ctrl Pts',(-4.01232252274933,-1.3,4.91808539201506));
#27211=CARTESIAN_POINT('Ctrl Pts',(-3.99512086302587,-1.3,4.92222147175324));
#27212=CARTESIAN_POINT('Ctrl Pts',(-3.98335277851019,-1.3,4.92491429713412));
#27213=CARTESIAN_POINT('Ctrl Pts',(-3.97477914228473,-1.3,4.92421546647452));
#27214=CARTESIAN_POINT('',(-3.85507599179486,-1.3,4.7268753052437));
#27215=CARTESIAN_POINT('',(-3.97477914228473,-1.3,4.92421546647452));
#27216=CARTESIAN_POINT('',(-4.01183482598956,-1.30000000000004,4.47462271804852));
#27217=CARTESIAN_POINT('Ctrl Pts',(-3.85507599179486,-1.3,4.7268753052437));
#27218=CARTESIAN_POINT('Ctrl Pts',(-3.85719962537661,-1.3,4.72144101857423));
#27219=CARTESIAN_POINT('Ctrl Pts',(-3.86187573129448,-1.3,4.71383403293719));
#27220=CARTESIAN_POINT('Ctrl Pts',(-3.86961810893469,-1.3,4.70440940889751));
#27221=CARTESIAN_POINT('Ctrl Pts',(-3.87691755596589,-1.3,4.69490664118851));
#27222=CARTESIAN_POINT('Ctrl Pts',(-3.88601526735224,-1.3,4.68298671678656));
#27223=CARTESIAN_POINT('Ctrl Pts',(-3.89491361629376,-1.30000000000001,
4.67070753187996));
#27224=CARTESIAN_POINT('Ctrl Pts',(-3.90299367365694,-1.30000000000001,
4.65757823073424));
#27225=CARTESIAN_POINT('Ctrl Pts',(-3.90989779693671,-1.30000000000001,
4.64755288062265));
#27226=CARTESIAN_POINT('Ctrl Pts',(-3.92221206525842,-1.30000000000001,
4.6303305021881));
#27227=CARTESIAN_POINT('Ctrl Pts',(-3.93623661697013,-1.30000000000003,
4.60609932986893));
#27228=CARTESIAN_POINT('Ctrl Pts',(-3.95284745610302,-1.30000000000004,
4.58042969910381));
#27229=CARTESIAN_POINT('Ctrl Pts',(-3.96535170192481,-1.30000000000004,
4.55902748517642));
#27230=CARTESIAN_POINT('Ctrl Pts',(-3.97449901676931,-1.30000000000004,
4.54274237531139));
#27231=CARTESIAN_POINT('Ctrl Pts',(-3.98365558285502,-1.30000000000005,
4.52648867384939));
#27232=CARTESIAN_POINT('Ctrl Pts',(-3.99622589356068,-1.30000000000007,
4.50522626952481));
#27233=CARTESIAN_POINT('Ctrl Pts',(-4.0051093795642,-1.30000000000007,4.48739495292359));
#27234=CARTESIAN_POINT('Ctrl Pts',(-4.01138931711436,-1.30000000000008,
4.47546647684066));
#27235=CARTESIAN_POINT('Ctrl Pts',(-4.01183482595518,-1.30000000000008,
4.47462271811364));
#27236=CARTESIAN_POINT('',(-3.68874885777913,-1.30000000000003,4.05109036897819));
#27237=CARTESIAN_POINT('Origin',(0.,-1.3,7.2));
#27238=CARTESIAN_POINT('',(-3.4147584711704,-1.3,4.14754376664537));
#27239=CARTESIAN_POINT('Ctrl Pts',(-3.68874885789501,-1.29999999999998,
4.05109036897745));
#27240=CARTESIAN_POINT('Ctrl Pts',(-3.68777058327918,-1.29999999999998,
4.0513661006271));
#27241=CARTESIAN_POINT('Ctrl Pts',(-3.68094176684541,-1.29999999999998,
4.05331905207122));
#27242=CARTESIAN_POINT('Ctrl Pts',(-3.67135789241846,-1.29999999999998,
4.05637552490222));
#27243=CARTESIAN_POINT('Ctrl Pts',(-3.65953806887845,-1.29999999999998,
4.05956467038679));
#27244=CARTESIAN_POINT('Ctrl Pts',(-3.64763149426095,-1.29999999999998,
4.06262355022671));
#27245=CARTESIAN_POINT('Ctrl Pts',(-3.63356070629898,-1.29999999999998,
4.06771912618173));
#27246=CARTESIAN_POINT('Ctrl Pts',(-3.61556442432801,-1.29999999999998,
4.07212390020612));
#27247=CARTESIAN_POINT('Ctrl Pts',(-3.58711823022726,-1.29999999999998,
4.08187617918609));
#27248=CARTESIAN_POINT('Ctrl Pts',(-3.55260469525794,-1.29999999999999,
4.0930731351417));
#27249=CARTESIAN_POINT('Ctrl Pts',(-3.51930456141974,-1.29999999999999,
4.10610119875621));
#27250=CARTESIAN_POINT('Ctrl Pts',(-3.49661091395695,-1.3,4.11413655268901));
#27251=CARTESIAN_POINT('Ctrl Pts',(-3.48026786811637,-1.3,4.12106457332588));
#27252=CARTESIAN_POINT('Ctrl Pts',(-3.46382778992352,-1.3,4.12803241400126));
#27253=CARTESIAN_POINT('Ctrl Pts',(-3.45023815468816,-1.3,4.1337844199917));
#27254=CARTESIAN_POINT('Ctrl Pts',(-3.4342434803328,-1.3,4.14136931465002));
#27255=CARTESIAN_POINT('Ctrl Pts',(-3.42329004793791,-1.3,4.14644476697428));
#27256=CARTESIAN_POINT('Ctrl Pts',(-3.4147584711704,-1.3,4.14754376664537));
#27257=CARTESIAN_POINT('',(-3.2566417951307,-1.3,3.97940364582357));
#27258=CARTESIAN_POINT('',(-3.4147584711704,-1.3,4.14754376664537));
#27259=CARTESIAN_POINT('',(-3.35764585633179,-1.3,3.70018367575412));
#27260=CARTESIAN_POINT('Ctrl Pts',(-3.2566417951307,-1.3,3.97940364582357));
#27261=CARTESIAN_POINT('Ctrl Pts',(-3.25806285817519,-1.3,3.97076805174943));
#27262=CARTESIAN_POINT('Ctrl Pts',(-3.26355683793739,-1.3,3.9597981722457));
#27263=CARTESIAN_POINT('Ctrl Pts',(-3.27139143944837,-1.3,3.94354916079683));
#27264=CARTESIAN_POINT('Ctrl Pts',(-3.2779598506316,-1.3,3.93013440106242));
#27265=CARTESIAN_POINT('Ctrl Pts',(-3.2859599492917,-1.3,3.91027551688124));
#27266=CARTESIAN_POINT('Ctrl Pts',(-3.29748931314118,-1.3,3.88213052763898));
#27267=CARTESIAN_POINT('Ctrl Pts',(-3.30875979616856,-1.3,3.85378158569074));
#27268=CARTESIAN_POINT('Ctrl Pts',(-3.32193490364989,-1.3,3.81588673765676));
#27269=CARTESIAN_POINT('Ctrl Pts',(-3.33101474967438,-1.3,3.78965575124683));
#27270=CARTESIAN_POINT('Ctrl Pts',(-3.33990624483581,-1.30000000000001,
3.7596865043912));
#27271=CARTESIAN_POINT('Ctrl Pts',(-3.34788849600103,-1.30000000000001,
3.73634894724736));
#27272=CARTESIAN_POINT('Ctrl Pts',(-3.35378355466238,-1.30000000000001,
3.71409631543785));
#27273=CARTESIAN_POINT('Ctrl Pts',(-3.35739217057375,-1.30000000000001,
3.70109535582529));
#27274=CARTESIAN_POINT('Ctrl Pts',(-3.35764585626408,-1.30000000000001,
3.70018367599751));
#27275=CARTESIAN_POINT('',(-2.95346134572195,-1.29999999999997,3.35297958421177));
#27276=CARTESIAN_POINT('Origin',(0.,-1.3,7.2));
#27277=CARTESIAN_POINT('',(-2.70549646903679,-1.3,3.50427905152391));
#27278=CARTESIAN_POINT('Ctrl Pts',(-2.95346134606173,-1.29999999999991,
3.35297958415421));
#27279=CARTESIAN_POINT('Ctrl Pts',(-2.95255499004324,-1.29999999999991,
3.3534507668553));
#27280=CARTESIAN_POINT('Ctrl Pts',(-2.94625709387801,-1.29999999999991,
3.35676322322326));
#27281=CARTESIAN_POINT('Ctrl Pts',(-2.93496317665334,-1.29999999999991,
3.36330631593411));
#27282=CARTESIAN_POINT('Ctrl Pts',(-2.91812360584104,-1.29999999999993,
3.37118251970181));
#27283=CARTESIAN_POINT('Ctrl Pts',(-2.9056493229959,-1.29999999999993,3.37931771926192));
#27284=CARTESIAN_POINT('Ctrl Pts',(-2.89444547446341,-1.29999999999993,
3.38460967377963));
#27285=CARTESIAN_POINT('Ctrl Pts',(-2.87330971922866,-1.29999999999993,
3.39645550931664));
#27286=CARTESIAN_POINT('Ctrl Pts',(-2.84986342692002,-1.29999999999996,
3.41016373782286));
#27287=CARTESIAN_POINT('Ctrl Pts',(-2.81674957134943,-1.29999999999996,
3.43070471365395));
#27288=CARTESIAN_POINT('Ctrl Pts',(-2.7913038555555,-1.29999999999999,3.44659963092752));
#27289=CARTESIAN_POINT('Ctrl Pts',(-2.76631964265224,-1.29999999999999,
3.46290077644007));
#27290=CARTESIAN_POINT('Ctrl Pts',(-2.74946991434189,-1.29999999999999,
3.47502052021695));
#27291=CARTESIAN_POINT('Ctrl Pts',(-2.73730164354868,-1.3,3.48341371040722));
#27292=CARTESIAN_POINT('Ctrl Pts',(-2.72326627312498,-1.3,3.49418507966832));
#27293=CARTESIAN_POINT('Ctrl Pts',(-2.71361311550261,-1.3,3.50143025308134));
#27294=CARTESIAN_POINT('Ctrl Pts',(-2.70549646903679,-1.3,3.50427905152391));
#27295=CARTESIAN_POINT('',(-2.5158767249182,-1.3,3.37268750121688));
#27296=CARTESIAN_POINT('',(-2.70549646903679,-1.3,3.50427905152391));
#27297=CARTESIAN_POINT('',(-2.55662924076281,-1.30000000000006,3.07857464882883));
#27298=CARTESIAN_POINT('Ctrl Pts',(-2.5158767249182,-1.3,3.37268750121688));
#27299=CARTESIAN_POINT('Ctrl Pts',(-2.51547129336049,-1.3,3.36394515997202));
#27300=CARTESIAN_POINT('Ctrl Pts',(-2.51853827080766,-1.3,3.35206487686083));
#27301=CARTESIAN_POINT('Ctrl Pts',(-2.52292752087393,-1.3,3.33458767675194));
#27302=CARTESIAN_POINT('Ctrl Pts',(-2.52626319062591,-1.30000000000002,
3.31997332758446));
#27303=CARTESIAN_POINT('Ctrl Pts',(-2.52947109631152,-1.30000000000001,
3.30515554054866));
#27304=CARTESIAN_POINT('Ctrl Pts',(-2.53134877776937,-1.30000000000001,
3.28980202777013));
#27305=CARTESIAN_POINT('Ctrl Pts',(-2.53635588003665,-1.30000000000001,
3.26613435433942));
#27306=CARTESIAN_POINT('Ctrl Pts',(-2.54098117524229,-1.30000000000006,
3.23262551129745));
#27307=CARTESIAN_POINT('Ctrl Pts',(-2.54607194775842,-1.30000000000005,
3.19608939128866));
#27308=CARTESIAN_POINT('Ctrl Pts',(-2.54893825527277,-1.30000000000007,
3.1715295558732));
#27309=CARTESIAN_POINT('Ctrl Pts',(-2.5504386619693,-1.30000000000007,3.15283126618667));
#27310=CARTESIAN_POINT('Ctrl Pts',(-2.55358415559025,-1.3000000000001,3.12519350169639));
#27311=CARTESIAN_POINT('Ctrl Pts',(-2.55521193746924,-1.30000000000012,
3.09918410423394));
#27312=CARTESIAN_POINT('Ctrl Pts',(-2.55656438877201,-1.30000000000014,
3.07951611690942));
#27313=CARTESIAN_POINT('Ctrl Pts',(-2.55662924075641,-1.30000000000014,
3.07857464892167));
#27314=CARTESIAN_POINT('',(-2.08924672297676,-1.30000000000088,2.82308040495193));
#27315=CARTESIAN_POINT('Origin',(0.,-1.3,7.2));
#27316=CARTESIAN_POINT('',(-1.87799128879384,-1.3,3.02253507588753));
#27317=CARTESIAN_POINT('Ctrl Pts',(-2.08923581516041,-1.29999999999997,
2.82308924799323));
#27318=CARTESIAN_POINT('Ctrl Pts',(-2.08844045325633,-1.29999999999997,
2.82373405682108));
#27319=CARTESIAN_POINT('Ctrl Pts',(-2.07814240117949,-1.29999999999997,
2.83208780541099));
#27320=CARTESIAN_POINT('Ctrl Pts',(-2.05852013350784,-1.29999999999997,
2.84828080309984));
#27321=CARTESIAN_POINT('Ctrl Pts',(-2.0312350900644,-1.29999999999999,2.87227242206314));
#27322=CARTESIAN_POINT('Ctrl Pts',(-2.00791251142451,-1.29999999999999,
2.89191456471751));
#27323=CARTESIAN_POINT('Ctrl Pts',(-1.99091305460766,-1.29999999999999,
2.90872364328326));
#27324=CARTESIAN_POINT('Ctrl Pts',(-1.96891126495497,-1.29999999999999,
2.92924299368149));
#27325=CARTESIAN_POINT('Ctrl Pts',(-1.94765865101366,-1.3,2.95030374733538));
#27326=CARTESIAN_POINT('Ctrl Pts',(-1.92692142534669,-1.3,2.97161824960676));
#27327=CARTESIAN_POINT('Ctrl Pts',(-1.91488873767411,-1.3,2.98475844866707));
#27328=CARTESIAN_POINT('Ctrl Pts',(-1.90476633611182,-1.3,2.99551287590898));
#27329=CARTESIAN_POINT('Ctrl Pts',(-1.89326780681826,-1.3,3.00896395652652));
#27330=CARTESIAN_POINT('Ctrl Pts',(-1.8853382685594,-1.3,3.01806098483551));
#27331=CARTESIAN_POINT('Ctrl Pts',(-1.87799128879384,-1.3,3.02253507588753));
#27332=CARTESIAN_POINT('',(-1.66515576931082,-1.3,2.93324327829));
#27333=CARTESIAN_POINT('',(-1.87799128879384,-1.3,3.02253507588753));
#27334=CARTESIAN_POINT('',(-1.64377746965492,-1.30000000000001,2.63705187074685));
#27335=CARTESIAN_POINT('Ctrl Pts',(-1.66515576931082,-1.3,2.93324327829));
#27336=CARTESIAN_POINT('Ctrl Pts',(-1.66294156245546,-1.3,2.9247762721372));
#27337=CARTESIAN_POINT('Ctrl Pts',(-1.66343058758897,-1.3,2.91253818382604));
#27338=CARTESIAN_POINT('Ctrl Pts',(-1.66409924349391,-1.3,2.89751233934794));
#27339=CARTESIAN_POINT('Ctrl Pts',(-1.66413304228543,-1.3,2.88855088157155));
#27340=CARTESIAN_POINT('Ctrl Pts',(-1.66445586874793,-1.3,2.87650429183671));
#27341=CARTESIAN_POINT('Ctrl Pts',(-1.664349847888,-1.3,2.86438665854254));
#27342=CARTESIAN_POINT('Ctrl Pts',(-1.66319395735112,-1.3,2.84901103609996));
#27343=CARTESIAN_POINT('Ctrl Pts',(-1.66287285385496,-1.3,2.83684381205863));
#27344=CARTESIAN_POINT('Ctrl Pts',(-1.66271526553416,-1.3,2.81567174026611));
#27345=CARTESIAN_POINT('Ctrl Pts',(-1.65979832631147,-1.3,2.78782357681355));
#27346=CARTESIAN_POINT('Ctrl Pts',(-1.65813795427161,-1.30000000000001,
2.75729053581771));
#27347=CARTESIAN_POINT('Ctrl Pts',(-1.65570779467889,-1.30000000000001,
2.7326332827021));
#27348=CARTESIAN_POINT('Ctrl Pts',(-1.65357606588014,-1.30000000000001,
2.71409163860543));
#27349=CARTESIAN_POINT('Ctrl Pts',(-1.65142819925291,-1.30000000000001,
2.69555803570244));
#27350=CARTESIAN_POINT('Ctrl Pts',(-1.64970395610008,-1.30000000000003,
2.67712374665253));
#27351=CARTESIAN_POINT('Ctrl Pts',(-1.6466789368294,-1.30000000000002,2.65843106406553));
#27352=CARTESIAN_POINT('Ctrl Pts',(-1.64484418585986,-1.30000000000002,
2.64511356192673));
#27353=CARTESIAN_POINT('Ctrl Pts',(-1.64390164626195,-1.30000000000002,
2.63799122361867));
#27354=CARTESIAN_POINT('Ctrl Pts',(-1.6437774696566,-1.30000000000002,2.63705187075953));
#27355=CARTESIAN_POINT('',(-1.13359858633549,-1.30000000000068,2.48435531028948));
#27356=CARTESIAN_POINT('Origin',(0.,-1.3,7.2));
#27357=CARTESIAN_POINT('',(-0.96840887762858,-1.3,2.72336636313561));
#27358=CARTESIAN_POINT('Ctrl Pts',(-1.13358785818362,-1.30000000000001,
2.48436857277337));
#27359=CARTESIAN_POINT('Ctrl Pts',(-1.13294391371556,-1.30000000000001,
2.48516464283889));
#27360=CARTESIAN_POINT('Ctrl Pts',(-1.12460746651562,-1.30000000000001,
2.49547678508334));
#27361=CARTESIAN_POINT('Ctrl Pts',(-1.10877976373829,-1.30000000000001,
2.51539512337677));
#27362=CARTESIAN_POINT('Ctrl Pts',(-1.08708000619847,-1.30000000000001,
2.54453579145496));
#27363=CARTESIAN_POINT('Ctrl Pts',(-1.06835320849415,-1.30000000000001,
2.56859872678717));
#27364=CARTESIAN_POINT('Ctrl Pts',(-1.05521937382472,-1.3,2.58857464167053));
#27365=CARTESIAN_POINT('Ctrl Pts',(-1.03796310307449,-1.30000000000001,
2.61321937129878));
#27366=CARTESIAN_POINT('Ctrl Pts',(-1.02154978498818,-1.3,2.63823699667523));
#27367=CARTESIAN_POINT('Ctrl Pts',(-1.00569178470079,-1.3,2.66339442294084));
#27368=CARTESIAN_POINT('Ctrl Pts',(-0.996652854808831,-1.3,2.67874859209711));
#27369=CARTESIAN_POINT('Ctrl Pts',(-0.988985336877536,-1.3,2.69137107011216));
#27370=CARTESIAN_POINT('Ctrl Pts',(-0.980533804017512,-1.3,2.7069183409826));
#27371=CARTESIAN_POINT('Ctrl Pts',(-0.974665092423394,-1.3,2.71746251872214));
#27372=CARTESIAN_POINT('Ctrl Pts',(-0.96840887762858,-1.3,2.72336636313561));
#27373=CARTESIAN_POINT('',(-0.741659516280667,-1.3,2.68027679827216));
#27374=CARTESIAN_POINT('',(-0.96840887762858,-1.3,2.72336636313561));
#27375=CARTESIAN_POINT('',(-0.65920976572758,-1.3,2.39500858640003));
#27376=CARTESIAN_POINT('Ctrl Pts',(-0.741659516280667,-1.3,2.68027679827216));
#27377=CARTESIAN_POINT('Ctrl Pts',(-0.737733305592168,-1.3,2.67245517600954));
#27378=CARTESIAN_POINT('Ctrl Pts',(-0.735709753270853,-1.3,2.66035632699759));
#27379=CARTESIAN_POINT('Ctrl Pts',(-0.732581199673119,-1.3,2.64260536769193));
#27380=CARTESIAN_POINT('Ctrl Pts',(-0.729771743392392,-1.3,2.62789816097751));
#27381=CARTESIAN_POINT('Ctrl Pts',(-0.726505469227191,-1.3,2.61305804659458));
#27382=CARTESIAN_POINT('Ctrl Pts',(-0.718203659447295,-1.3,2.58347432518374));
#27383=CARTESIAN_POINT('Ctrl Pts',(-0.711759248151159,-1.3,2.55392799989943));
#27384=CARTESIAN_POINT('Ctrl Pts',(-0.701409308678931,-1.3,2.52143083639189));
#27385=CARTESIAN_POINT('Ctrl Pts',(-0.695015042608168,-1.3,2.49781259678565));
#27386=CARTESIAN_POINT('Ctrl Pts',(-0.684471546903469,-1.3,2.46831190594928));
#27387=CARTESIAN_POINT('Ctrl Pts',(-0.67426120931563,-1.3,2.43590191982579));
#27388=CARTESIAN_POINT('Ctrl Pts',(-0.665650684226192,-1.3,2.41236448965118));
#27389=CARTESIAN_POINT('Ctrl Pts',(-0.660928574120142,-1.3,2.3997238538199));
#27390=CARTESIAN_POINT('Ctrl Pts',(-0.659532670840085,-1.3,2.39589740264602));
#27391=CARTESIAN_POINT('Ctrl Pts',(-0.659209765837711,-1.3,2.39500858670318));
#27392=CARTESIAN_POINT('',(-0.128233641545422,-1.30000000000026,2.35170117785791));
#27393=CARTESIAN_POINT('Origin',(0.,-1.3,7.2));
#27394=CARTESIAN_POINT('',(-0.0165023515695832,-1.3,2.61984802158616));
#27395=CARTESIAN_POINT('Ctrl Pts',(-0.128230808431501,-1.3,2.35170674040144));
#27396=CARTESIAN_POINT('Ctrl Pts',(-0.12776606171,-1.3,2.35261922867771));
#27397=CARTESIAN_POINT('Ctrl Pts',(-0.116201754712566,-1.3,2.37534516765435));
#27398=CARTESIAN_POINT('Ctrl Pts',(-0.10245981594267,-1.3,2.40364627470203));
#27399=CARTESIAN_POINT('Ctrl Pts',(-0.0865550189115516,-1.3,2.43952180316647));
#27400=CARTESIAN_POINT('Ctrl Pts',(-0.0768451818344749,-1.3,2.46162868799538));
#27401=CARTESIAN_POINT('Ctrl Pts',(-0.0646419694895632,-1.3,2.49219986215438));
#27402=CARTESIAN_POINT('Ctrl Pts',(-0.0519913323925687,-1.3,2.52275042090917));
#27403=CARTESIAN_POINT('Ctrl Pts',(-0.0414484880037243,-1.3,2.55063756703338));
#27404=CARTESIAN_POINT('Ctrl Pts',(-0.0349002835201714,-1.3,2.57033915626984));
#27405=CARTESIAN_POINT('Ctrl Pts',(-0.0299922130720366,-1.3,2.58428069475804));
#27406=CARTESIAN_POINT('Ctrl Pts',(-0.0249600309789548,-1.3,2.60124271611068));
#27407=CARTESIAN_POINT('Ctrl Pts',(-0.0213943747864753,-1.3,2.6127724501419));
#27408=CARTESIAN_POINT('Ctrl Pts',(-0.0165023515695832,-1.3,2.61984802158616));
#27409=CARTESIAN_POINT('',(0.214250816488161,-1.3,2.62484391020801));
#27410=CARTESIAN_POINT('',(-0.0165023515695832,-1.3,2.61984802158616));
#27411=CARTESIAN_POINT('',(0.35416429646195,-1.3,2.36294845478037));
#27412=CARTESIAN_POINT('Ctrl Pts',(0.214250816488161,-1.3,2.62484391020801));
#27413=CARTESIAN_POINT('Ctrl Pts',(0.219717436762652,-1.3,2.61800951426072));
#27414=CARTESIAN_POINT('Ctrl Pts',(0.224226242429556,-1.3,2.60660085910045));
#27415=CARTESIAN_POINT('Ctrl Pts',(0.230949458773341,-1.3,2.58988253450941));
#27416=CARTESIAN_POINT('Ctrl Pts',(0.236845399224574,-1.3,2.57610161912971));
#27417=CARTESIAN_POINT('Ctrl Pts',(0.242960861231531,-1.3,2.56222898063722));
#27418=CARTESIAN_POINT('Ctrl Pts',(0.250471543071847,-1.3,2.54870591804817));
#27419=CARTESIAN_POINT('Ctrl Pts',(0.260324786692121,-1.30000000000003,
2.52661415542702));
#27420=CARTESIAN_POINT('Ctrl Pts',(0.276326377533022,-1.29999999999998,
2.49679480815956));
#27421=CARTESIAN_POINT('Ctrl Pts',(0.292202396494612,-1.3,2.46694851625356));
#27422=CARTESIAN_POINT('Ctrl Pts',(0.304272576971148,-1.3,2.44537989334913));
#27423=CARTESIAN_POINT('Ctrl Pts',(0.313919337066705,-1.3,2.42933896783766));
#27424=CARTESIAN_POINT('Ctrl Pts',(0.329357357760238,-1.3,2.40248830163039));
#27425=CARTESIAN_POINT('Ctrl Pts',(0.343163853228179,-1.3,2.3804482950595));
#27426=CARTESIAN_POINT('Ctrl Pts',(0.353661239603825,-1.3,2.3637484532088));
#27427=CARTESIAN_POINT('Ctrl Pts',(0.354164296458132,-1.3,2.36294845478644));
#27428=CARTESIAN_POINT('',(0.882693729895366,-1.30000000000117,2.43100096678543));
#27429=CARTESIAN_POINT('Origin',(0.,-1.3,7.2));
#27430=CARTESIAN_POINT('',(0.936125406440075,-1.3,2.71650429950101));
#27431=CARTESIAN_POINT('Ctrl Pts',(0.88269372985561,-1.30000000000001,2.43100096679471));
#27432=CARTESIAN_POINT('Ctrl Pts',(0.882952787962226,-1.30000000000001,
2.43198921795854));
#27433=CARTESIAN_POINT('Ctrl Pts',(0.884755223318824,-1.30000000000001,
2.43888799591159));
#27434=CARTESIAN_POINT('Ctrl Pts',(0.889558734078043,-1.30000000000001,
2.45759430808911));
#27435=CARTESIAN_POINT('Ctrl Pts',(0.89478682500609,-1.3,2.4812180822005));
#27436=CARTESIAN_POINT('Ctrl Pts',(0.900920744454363,-1.3,2.5048946782523));
#27437=CARTESIAN_POINT('Ctrl Pts',(0.903919282745227,-1.3,2.52258106593104));
#27438=CARTESIAN_POINT('Ctrl Pts',(0.909809170318803,-1.3,2.54627243685644));
#27439=CARTESIAN_POINT('Ctrl Pts',(0.915082652483101,-1.3,2.57870764115585));
#27440=CARTESIAN_POINT('Ctrl Pts',(0.920469044817052,-1.3,2.60822457195672));
#27441=CARTESIAN_POINT('Ctrl Pts',(0.923992559502828,-1.3,2.62890061695527));
#27442=CARTESIAN_POINT('Ctrl Pts',(0.92529189916004,-1.3,2.63775451220869));
#27443=CARTESIAN_POINT('Ctrl Pts',(0.926611318159081,-1.3,2.64948665818481));
#27444=CARTESIAN_POINT('Ctrl Pts',(0.928513761893331,-1.3,2.66427335298964));
#27445=CARTESIAN_POINT('Ctrl Pts',(0.930286002589081,-1.3,2.67890363859173));
#27446=CARTESIAN_POINT('Ctrl Pts',(0.931729064678959,-1.3,2.69655002042693));
#27447=CARTESIAN_POINT('Ctrl Pts',(0.932811379690214,-1.3,2.70856623745045));
#27448=CARTESIAN_POINT('Ctrl Pts',(0.936125406440075,-1.3,2.71650429950101));
#27449=CARTESIAN_POINT('',(1.16079736048698,-1.3,2.76936729730244));
#27450=CARTESIAN_POINT('',(0.936125406440075,-1.3,2.71650429950101));
#27451=CARTESIAN_POINT('',(1.35237060322927,-1.30000000000175,2.54236178404915));
#27452=CARTESIAN_POINT('Ctrl Pts',(1.16079736048698,-1.3,2.76936729730244));
#27453=CARTESIAN_POINT('Ctrl Pts',(1.16756547280971,-1.3,2.76381882356845));
#27454=CARTESIAN_POINT('Ctrl Pts',(1.17429750653111,-1.3,2.75357268161998));
#27455=CARTESIAN_POINT('Ctrl Pts',(1.18440293490914,-1.3,2.73864158445797));
#27456=CARTESIAN_POINT('Ctrl Pts',(1.19282025714294,-1.3,2.72628875413437));
#27457=CARTESIAN_POINT('Ctrl Pts',(1.20387629867366,-1.3,2.71172082727262));
#27458=CARTESIAN_POINT('Ctrl Pts',(1.22295971290217,-1.3,2.68787251266423));
#27459=CARTESIAN_POINT('Ctrl Pts',(1.24182813440028,-1.3,2.66390221260837));
#27460=CARTESIAN_POINT('Ctrl Pts',(1.26205481118708,-1.3,2.6405729968529));
#27461=CARTESIAN_POINT('Ctrl Pts',(1.2776175603498,-1.3,2.62164579396719));
#27462=CARTESIAN_POINT('Ctrl Pts',(1.2989775139145,-1.30000000000002,2.59886823472894));
#27463=CARTESIAN_POINT('Ctrl Pts',(1.32380250697419,-1.30000000000001,2.57121941147867));
#27464=CARTESIAN_POINT('Ctrl Pts',(1.34201514395952,-1.30000000000001,2.55258581820719));
#27465=CARTESIAN_POINT('Ctrl Pts',(1.35168394483177,-1.30000000000001,2.54304278699951));
#27466=CARTESIAN_POINT('Ctrl Pts',(1.35237060320572,-1.30000000000001,2.54236178414845));
#27467=CARTESIAN_POINT('',(1.8548768629636,-1.30000000000053,2.71871315099399));
#27468=CARTESIAN_POINT('Origin',(0.,-1.3,7.2));
#27469=CARTESIAN_POINT('',(1.84783999216022,-1.3,3.009110853727));
#27470=CARTESIAN_POINT('Ctrl Pts',(1.85487686288809,-1.3,2.71871315085827));
#27471=CARTESIAN_POINT('Ctrl Pts',(1.8549270845609,-1.3,2.71973140281124));
#27472=CARTESIAN_POINT('Ctrl Pts',(1.85584912980544,-1.3,2.73905781529638));
#27473=CARTESIAN_POINT('Ctrl Pts',(1.85622336316485,-1.3,2.76429054728935));
#27474=CARTESIAN_POINT('Ctrl Pts',(1.85720708657456,-1.3,2.79473457766745));
#27475=CARTESIAN_POINT('Ctrl Pts',(1.85717700294328,-1.3,2.82191251964874));
#27476=CARTESIAN_POINT('Ctrl Pts',(1.85685021732853,-1.3,2.84599119375483));
#27477=CARTESIAN_POINT('Ctrl Pts',(1.85632123702888,-1.3,2.87004577464698));
#27478=CARTESIAN_POINT('Ctrl Pts',(1.85516825338145,-1.3,2.89087649959048));
#27479=CARTESIAN_POINT('Ctrl Pts',(1.85462998338858,-1.3,2.91496806145217));
#27480=CARTESIAN_POINT('Ctrl Pts',(1.85283789437454,-1.3,2.9386502765753));
#27481=CARTESIAN_POINT('Ctrl Pts',(1.85121289296164,-1.3,2.956407355506));
#27482=CARTESIAN_POINT('Ctrl Pts',(1.84997378187088,-1.3,2.97112153527195));
#27483=CARTESIAN_POINT('Ctrl Pts',(1.84769026538568,-1.3,2.98867205329545));
#27484=CARTESIAN_POINT('Ctrl Pts',(1.84624880074882,-1.3,3.00065723247277));
#27485=CARTESIAN_POINT('Ctrl Pts',(1.84783999216022,-1.3,3.009110853727));
#27486=CARTESIAN_POINT('',(2.05661148970878,-1.3,3.10753059403928));
#27487=CARTESIAN_POINT('',(1.84783999216022,-1.3,3.009110853727));
#27488=CARTESIAN_POINT('',(2.29124606287429,-1.30000000000005,2.92534725798923));
#27489=CARTESIAN_POINT('Ctrl Pts',(2.05661148970878,-1.3,3.10753059403928));
#27490=CARTESIAN_POINT('Ctrl Pts',(2.06438529509424,-1.3,3.10351053744535));
#27491=CARTESIAN_POINT('Ctrl Pts',(2.07311117400896,-1.3,3.09489607890758));
#27492=CARTESIAN_POINT('Ctrl Pts',(2.08606699867075,-1.3,3.08237024088461));
#27493=CARTESIAN_POINT('Ctrl Pts',(2.09696957937697,-1.3,3.07210722196283));
#27494=CARTESIAN_POINT('Ctrl Pts',(2.11058813200124,-1.3,3.06000397880414));
#27495=CARTESIAN_POINT('Ctrl Pts',(2.12535537170441,-1.3,3.04879480129421));
#27496=CARTESIAN_POINT('Ctrl Pts',(2.14303983420991,-1.3,3.03242748668087));
#27497=CARTESIAN_POINT('Ctrl Pts',(2.16828207977003,-1.30000000000002,3.01421432900305));
#27498=CARTESIAN_POINT('Ctrl Pts',(2.19672991623475,-1.30000000000001,2.99108833318567));
#27499=CARTESIAN_POINT('Ctrl Pts',(2.22228736155764,-1.30000000000002,2.97318805622786));
#27500=CARTESIAN_POINT('Ctrl Pts',(2.24737536599506,-1.30000000000003,2.95499905098218));
#27501=CARTESIAN_POINT('Ctrl Pts',(2.26798132103125,-1.30000000000003,2.94084734176461));
#27502=CARTESIAN_POINT('Ctrl Pts',(2.28447669320673,-1.30000000000004,2.92993182453429));
#27503=CARTESIAN_POINT('Ctrl Pts',(2.29044867842997,-1.30000000000004,2.92588845519796));
#27504=CARTESIAN_POINT('Ctrl Pts',(2.29124265273508,-1.30000000000004,2.92534957251983));
#27505=CARTESIAN_POINT('',(2.74606318254088,-1.30000000000086,3.20229603426228));
#27506=CARTESIAN_POINT('Origin',(0.,-1.3,7.2));
#27507=CARTESIAN_POINT('',(2.67879510330291,-1.3,3.48487937376242));
#27508=CARTESIAN_POINT('Ctrl Pts',(2.74606318249062,-1.29999999999992,3.20229603390921));
#27509=CARTESIAN_POINT('Ctrl Pts',(2.74589513931379,-1.29999999999992,3.20330365007811));
#27510=CARTESIAN_POINT('Ctrl Pts',(2.74469097079251,-1.29999999999992,3.2103169281617));
#27511=CARTESIAN_POINT('Ctrl Pts',(2.74195814600035,-1.29999999999994,3.22308002651851));
#27512=CARTESIAN_POINT('Ctrl Pts',(2.73967118082232,-1.29999999999994,3.24152929711112));
#27513=CARTESIAN_POINT('Ctrl Pts',(2.73578893667096,-1.29999999999994,3.25590696673797));
#27514=CARTESIAN_POINT('Ctrl Pts',(2.73421818102307,-1.29999999999994,3.26819776747556));
#27515=CARTESIAN_POINT('Ctrl Pts',(2.72948351347016,-1.29999999999994,3.29195966295173));
#27516=CARTESIAN_POINT('Ctrl Pts',(2.72369170179234,-1.29999999999997,3.3184945491252));
#27517=CARTESIAN_POINT('Ctrl Pts',(2.7143890244755,-1.29999999999997,3.35633531279436));
#27518=CARTESIAN_POINT('Ctrl Pts',(2.70713559815793,-1.29999999999998,3.38544760191399));
#27519=CARTESIAN_POINT('Ctrl Pts',(2.69935280611399,-1.29999999999999,3.41424635971549));
#27520=CARTESIAN_POINT('Ctrl Pts',(2.6930331868878,-1.3,3.43401667925856));
#27521=CARTESIAN_POINT('Ctrl Pts',(2.68881095174019,-1.3,3.44818305017517));
#27522=CARTESIAN_POINT('Ctrl Pts',(2.68290395206009,-1.3,3.46486003904829));
#27523=CARTESIAN_POINT('Ctrl Pts',(2.67899628993004,-1.3,3.47627965711833));
#27524=CARTESIAN_POINT('Ctrl Pts',(2.67879510330291,-1.3,3.48487937376242));
#27525=CARTESIAN_POINT('',(2.86254182811346,-1.3,3.62455444166361));
#27526=CARTESIAN_POINT('',(2.67879510330291,-1.3,3.48487937376242));
#27527=CARTESIAN_POINT('',(3.12987662692929,-1.30000000000176,3.49508808472698));
#27528=CARTESIAN_POINT('Ctrl Pts',(2.86254182811346,-1.3,3.62455444166361));
#27529=CARTESIAN_POINT('Ctrl Pts',(2.87098157396346,-1.3,3.62223849797319));
#27530=CARTESIAN_POINT('Ctrl Pts',(2.88130082124863,-1.3,3.61561587077067));
#27531=CARTESIAN_POINT('Ctrl Pts',(2.89657701929705,-1.3,3.60605436272742));
#27532=CARTESIAN_POINT('Ctrl Pts',(2.90936639790833,-1.29999999999998,3.59827482204039));
#27533=CARTESIAN_POINT('Ctrl Pts',(2.92520978215673,-1.29999999999999,3.58926377762022));
#27534=CARTESIAN_POINT('Ctrl Pts',(2.94195211701841,-1.29999999999997,3.58135635188596));
#27535=CARTESIAN_POINT('Ctrl Pts',(2.96275287235917,-1.29999999999999,3.56912187057544));
#27536=CARTESIAN_POINT('Ctrl Pts',(2.99103081011587,-1.29999999999996,3.55633083166688));
#27537=CARTESIAN_POINT('Ctrl Pts',(3.02374000248103,-1.29999999999995,3.53970490348805));
#27538=CARTESIAN_POINT('Ctrl Pts',(3.0581134518176,-1.29999999999992,3.52497819970328));
#27539=CARTESIAN_POINT('Ctrl Pts',(3.09205625616746,-1.2999999999999,3.50984328348542));
#27540=CARTESIAN_POINT('Ctrl Pts',(3.11631138545393,-1.29999999999988,3.50027215599398));
#27541=CARTESIAN_POINT('Ctrl Pts',(3.12897487608527,-1.29999999999987,3.49543223771777));
#27542=CARTESIAN_POINT('Ctrl Pts',(3.12987662694986,-1.29999999999987,3.495088084751));
#27543=CARTESIAN_POINT('',(3.5171326127652,-1.30000000000045,3.86049731487559));
#27544=CARTESIAN_POINT('Origin',(0.,-1.3,7.2));
#27545=CARTESIAN_POINT('',(3.39267401414619,-1.3,4.12301649229108));
#27546=CARTESIAN_POINT('Ctrl Pts',(3.51713261273951,-1.3,3.86049731486587));
#27547=CARTESIAN_POINT('Ctrl Pts',(3.51688288217038,-1.3,3.86115709724913));
#27548=CARTESIAN_POINT('Ctrl Pts',(3.51650668153201,-1.3,3.86212544904999));
#27549=CARTESIAN_POINT('Ctrl Pts',(3.5160121348391,-1.3,3.86337613530466));
#27550=CARTESIAN_POINT('Ctrl Pts',(3.51367923070723,-1.3,3.86927594450976));
#27551=CARTESIAN_POINT('Ctrl Pts',(3.50890708207116,-1.3,3.88153385811727));
#27552=CARTESIAN_POINT('Ctrl Pts',(3.50248870255892,-1.3,3.89738608899958));
#27553=CARTESIAN_POINT('Ctrl Pts',(3.49843132749079,-1.3,3.90740706800735));
#27554=CARTESIAN_POINT('Ctrl Pts',(3.49368714677763,-1.3,3.91885284427876));
#27555=CARTESIAN_POINT('Ctrl Pts',(3.48842221216129,-1.3,3.93100743587123));
#27556=CARTESIAN_POINT('Ctrl Pts',(3.48607767189504,-1.3,3.93642002529257));
#27557=CARTESIAN_POINT('Ctrl Pts',(3.48362945784637,-1.3,3.94197283731675));
#27558=CARTESIAN_POINT('Ctrl Pts',(3.48111675437825,-1.3,3.94761334202975));
#27559=CARTESIAN_POINT('Ctrl Pts',(3.47392079620689,-1.3,3.96376679447454));
#27560=CARTESIAN_POINT('Ctrl Pts',(3.46610202845713,-1.3,3.98081946477663));
#27561=CARTESIAN_POINT('Ctrl Pts',(3.45829100003881,-1.3,3.99674657305018));
#27562=CARTESIAN_POINT('Ctrl Pts',(3.45203318383949,-1.3,4.00950659782858));
#27563=CARTESIAN_POINT('Ctrl Pts',(3.44681974798713,-1.3,4.01966078645757));
#27564=CARTESIAN_POINT('Ctrl Pts',(3.44229346403023,-1.3,4.02889359280264));
#27565=CARTESIAN_POINT('Ctrl Pts',(3.43952648034535,-1.3,4.03453774256563));
#27566=CARTESIAN_POINT('Ctrl Pts',(3.43698933358003,-1.3,4.03982671919313));
#27567=CARTESIAN_POINT('Ctrl Pts',(3.4343179304055,-1.3,4.04500372655646));
#27568=CARTESIAN_POINT('Ctrl Pts',(3.43163432866176,-1.3,4.05020437396154));
#27569=CARTESIAN_POINT('Ctrl Pts',(3.42878588057214,-1.3,4.05534933711627));
#27570=CARTESIAN_POINT('Ctrl Pts',(3.42583988757771,-1.3,4.060679557033));
#27571=CARTESIAN_POINT('Ctrl Pts',(3.42266805467712,-1.3,4.06641839175911));
#27572=CARTESIAN_POINT('Ctrl Pts',(3.41981353336582,-1.3,4.07159530558462));
#27573=CARTESIAN_POINT('Ctrl Pts',(3.417220711055,-1.3,4.07625699048129));
#27574=CARTESIAN_POINT('Ctrl Pts',(3.41568434131801,-1.3,4.07901925905972));
#27575=CARTESIAN_POINT('Ctrl Pts',(3.4142406922337,-1.3,4.08160108673217));
#27576=CARTESIAN_POINT('Ctrl Pts',(3.41288349055858,-1.3,4.08401513033096));
#27577=CARTESIAN_POINT('Ctrl Pts',(3.41132416451107,-1.3,4.08678869090963));
#27578=CARTESIAN_POINT('Ctrl Pts',(3.4098759552894,-1.3,4.08933910003031));
#27579=CARTESIAN_POINT('Ctrl Pts',(3.40850271524696,-1.3,4.09167097319111));
#27580=CARTESIAN_POINT('Ctrl Pts',(3.40683923872879,-1.3,4.09449569146794));
#27581=CARTESIAN_POINT('Ctrl Pts',(3.40529659274212,-1.3,4.09700575372786));
#27582=CARTESIAN_POINT('Ctrl Pts',(3.403919606175,-1.3,4.09926954672169));
#27583=CARTESIAN_POINT('Ctrl Pts',(3.39276510850083,-1.3,4.11760776024346));
#27584=CARTESIAN_POINT('Ctrl Pts',(3.39333976027048,-1.3,4.12020898041362));
#27585=CARTESIAN_POINT('Ctrl Pts',(3.39267401414619,-1.3,4.12301649229108));
#27586=CARTESIAN_POINT('',(3.54336535262991,-1.3,4.29784241707854));
#27587=CARTESIAN_POINT('',(3.39267401414619,-1.3,4.12301649229108));
#27588=CARTESIAN_POINT('',(3.83160559593893,-1.30000000000002,4.22656788267061));
#27589=CARTESIAN_POINT('Ctrl Pts',(3.54336535262991,-1.3,4.29784241707854));
#27590=CARTESIAN_POINT('Ctrl Pts',(3.5521021815524,-1.3,4.29733180414408));
#27591=CARTESIAN_POINT('Ctrl Pts',(3.56358560401283,-1.3,4.29301250933079));
#27592=CARTESIAN_POINT('Ctrl Pts',(3.58056423090154,-1.3,4.28691857619117));
#27593=CARTESIAN_POINT('Ctrl Pts',(3.59459177663706,-1.3,4.2817873486781));
#27594=CARTESIAN_POINT('Ctrl Pts',(3.61517717129019,-1.3,4.27590496591539));
#27595=CARTESIAN_POINT('Ctrl Pts',(3.64437267289781,-1.30000000000002,4.26737943677047));
#27596=CARTESIAN_POINT('Ctrl Pts',(3.67374206987082,-1.30000000000001,4.25912999654611));
#27597=CARTESIAN_POINT('Ctrl Pts',(3.71280539583391,-1.30000000000003,4.24998612818397));
#27598=CARTESIAN_POINT('Ctrl Pts',(3.73984169575344,-1.30000000000003,4.24369792702497));
#27599=CARTESIAN_POINT('Ctrl Pts',(3.77057621024761,-1.30000000000003,4.23798792710164));
#27600=CARTESIAN_POINT('Ctrl Pts',(3.79462037248639,-1.30000000000005,4.23248904186298));
#27601=CARTESIAN_POINT('Ctrl Pts',(3.81736692655516,-1.30000000000004,4.22895365433709));
#27602=CARTESIAN_POINT('Ctrl Pts',(3.83067329395874,-1.30000000000005,4.22672467388769));
#27603=CARTESIAN_POINT('Ctrl Pts',(3.83160559566069,-1.30000000000005,4.2265678827174));
#27604=CARTESIAN_POINT('',(4.13470146325513,-1.3,4.66489767272486));
#27605=CARTESIAN_POINT('Origin',(0.,-1.3,7.2));
#27606=CARTESIAN_POINT('',(3.95827679071515,-1.3,4.89563255511164));
#27607=CARTESIAN_POINT('Ctrl Pts',(4.1347014632565,-1.30000000000001,4.66489767272278));
#27608=CARTESIAN_POINT('Ctrl Pts',(4.13414034057423,-1.30000000000001,4.66574651526749));
#27609=CARTESIAN_POINT('Ctrl Pts',(4.1301921985072,-1.30000000000001,4.67166339544529));
#27610=CARTESIAN_POINT('Ctrl Pts',(4.1225478980385,-1.30000000000001,4.68226017949025));
#27611=CARTESIAN_POINT('Ctrl Pts',(4.11277136635636,-1.30000000000001,4.69795681868009));
#27612=CARTESIAN_POINT('Ctrl Pts',(4.10185652815243,-1.30000000000001,4.71227111163331));
#27613=CARTESIAN_POINT('Ctrl Pts',(4.08853169252855,-1.30000000000001,4.73287853781571));
#27614=CARTESIAN_POINT('Ctrl Pts',(4.07049950580513,-1.29999999999999,4.75697072422904));
#27615=CARTESIAN_POINT('Ctrl Pts',(4.04694899362191,-1.3,4.7882155432056));
#27616=CARTESIAN_POINT('Ctrl Pts',(4.02820350434482,-1.3,4.8114248769198));
#27617=CARTESIAN_POINT('Ctrl Pts',(4.01343459617974,-1.3,4.83038036764205));
#27618=CARTESIAN_POINT('Ctrl Pts',(4.00369573333177,-1.3,4.84150363159022));
#27619=CARTESIAN_POINT('Ctrl Pts',(3.99200513405257,-1.3,4.855004766164));
#27620=CARTESIAN_POINT('Ctrl Pts',(3.9823266250081,-1.3,4.86614166803621));
#27621=CARTESIAN_POINT('Ctrl Pts',(3.97017242189078,-1.3,4.87901196281535));
#27622=CARTESIAN_POINT('Ctrl Pts',(3.96195840372374,-1.3,4.88785815300778));
#27623=CARTESIAN_POINT('Ctrl Pts',(3.95827679071515,-1.3,4.89563255511164));
#27624=CARTESIAN_POINT('',(4.06932680828302,-1.3,5.09796860496431));
#27625=CARTESIAN_POINT('',(3.95827679071515,-1.3,4.89563255511164));
#27626=CARTESIAN_POINT('',(4.36619448174045,-1.30000000000001,5.08840208666063));
#27627=CARTESIAN_POINT('Ctrl Pts',(4.06932680828302,-1.3,5.09796860496431));
#27628=CARTESIAN_POINT('Ctrl Pts',(4.07797887893015,-1.3,5.09928563902122));
#27629=CARTESIAN_POINT('Ctrl Pts',(4.09010264837494,-1.3,5.09742818248793));
#27630=CARTESIAN_POINT('Ctrl Pts',(4.10794777737397,-1.3,5.09490870018088));
#27631=CARTESIAN_POINT('Ctrl Pts',(4.1227984853887,-1.3,5.092996965449));
#27632=CARTESIAN_POINT('Ctrl Pts',(4.14093676471961,-1.3,5.09122327296695));
#27633=CARTESIAN_POINT('Ctrl Pts',(4.15945674239661,-1.3,5.09077853240722));
#27634=CARTESIAN_POINT('Ctrl Pts',(4.18342557961069,-1.3,5.08805332370513));
#27635=CARTESIAN_POINT('Ctrl Pts',(4.22679133883137,-1.3,5.0875445379173));
#27636=CARTESIAN_POINT('Ctrl Pts',(4.26662860959371,-1.30000000000001,5.08602638006159));
#27637=CARTESIAN_POINT('Ctrl Pts',(4.3041267131296,-1.30000000000001,5.08697688034838));
#27638=CARTESIAN_POINT('Ctrl Pts',(4.32877752354222,-1.30000000000001,5.08656709641376));
#27639=CARTESIAN_POINT('Ctrl Pts',(4.35175885165174,-1.30000000000001,5.08779880743945));
#27640=CARTESIAN_POINT('Ctrl Pts',(4.36524030569969,-1.30000000000002,5.08836278683076));
#27641=CARTESIAN_POINT('Ctrl Pts',(4.3661944817394,-1.30000000000002,5.08840208666059));
#27642=CARTESIAN_POINT('',(4.5712854650164,-1.30000000000092,5.57960782188225));
#27643=CARTESIAN_POINT('Origin',(0.,-1.3,7.2));
#27644=CARTESIAN_POINT('',(4.35088387761047,-1.3,5.76896053285564));
#27645=CARTESIAN_POINT('Ctrl Pts',(4.57127105643491,-1.30000000000025,5.57962221793917));
#27646=CARTESIAN_POINT('Ctrl Pts',(4.57054672674967,-1.30000000000025,5.58034591264246));
#27647=CARTESIAN_POINT('Ctrl Pts',(4.56116348515715,-1.30000000000025,5.58971564859421));
#27648=CARTESIAN_POINT('Ctrl Pts',(4.54301380784618,-1.30000000000019,5.60754561873787));
#27649=CARTESIAN_POINT('Ctrl Pts',(4.51629897299144,-1.30000000000017,5.63216227364949));
#27650=CARTESIAN_POINT('Ctrl Pts',(4.49433855488318,-1.30000000000009,5.65331652551982));
#27651=CARTESIAN_POINT('Ctrl Pts',(4.47582949985366,-1.3000000000001,5.66843433384021));
#27652=CARTESIAN_POINT('Ctrl Pts',(4.45542493556535,-1.30000000000008,5.68625771326949));
#27653=CARTESIAN_POINT('Ctrl Pts',(4.43225268787841,-1.30000000000004,5.70516072474142));
#27654=CARTESIAN_POINT('Ctrl Pts',(4.40908517600157,-1.30000000000003,5.72400020051142));
#27655=CARTESIAN_POINT('Ctrl Pts',(4.39231891341255,-1.30000000000002,5.73621537749316));
#27656=CARTESIAN_POINT('Ctrl Pts',(4.38057663395205,-1.30000000000002,5.74519668890453));
#27657=CARTESIAN_POINT('Ctrl Pts',(4.36598759938307,-1.3,5.75520187083905));
#27658=CARTESIAN_POINT('Ctrl Pts',(4.35610142762816,-1.3,5.76212147047616));
#27659=CARTESIAN_POINT('Ctrl Pts',(4.35088387761047,-1.3,5.76896053285564));
#27660=CARTESIAN_POINT('',(4.41743915561768,-1.3,5.98996365147886));
#27661=CARTESIAN_POINT('',(4.35088387761047,-1.3,5.76896053285564));
#27662=CARTESIAN_POINT('',(4.70981332849669,-1.30000000000085,6.04234788887652));
#27663=CARTESIAN_POINT('Ctrl Pts',(4.41743915561768,-1.3,5.98996365147887));
#27664=CARTESIAN_POINT('Ctrl Pts',(4.42562833098492,-1.3,5.99305077181904));
#27665=CARTESIAN_POINT('Ctrl Pts',(4.43787121888721,-1.29999999999999,5.99376524194451));
#27666=CARTESIAN_POINT('Ctrl Pts',(4.45585041430517,-1.29999999999998,5.99501197237366));
#27667=CARTESIAN_POINT('Ctrl Pts',(4.47077112054749,-1.29999999999998,5.99624136741251));
#27668=CARTESIAN_POINT('Ctrl Pts',(4.48888549481281,-1.29999999999996,5.99826902796312));
#27669=CARTESIAN_POINT('Ctrl Pts',(4.50708052400253,-1.29999999999994,6.00172835399205));
#27670=CARTESIAN_POINT('Ctrl Pts',(4.53109886254277,-1.29999999999994,6.00406302153201));
#27671=CARTESIAN_POINT('Ctrl Pts',(4.5554207795094,-1.29999999999991,6.00910658184204));
#27672=CARTESIAN_POINT('Ctrl Pts',(4.57961335592168,-1.2999999999999,6.01326169023657));
#27673=CARTESIAN_POINT('Ctrl Pts',(4.60381579105576,-1.29999999999988,6.01754841177145));
#27674=CARTESIAN_POINT('Ctrl Pts',(4.62354611479138,-1.29999999999983,6.02187971789091));
#27675=CARTESIAN_POINT('Ctrl Pts',(4.63874413860124,-1.29999999999982,6.02548249806524));
#27676=CARTESIAN_POINT('Ctrl Pts',(4.6448207916927,-1.29999999999982,6.02690740127392));
#27677=CARTESIAN_POINT('Ctrl Pts',(4.65541484816387,-1.29999999999982,6.02904115986987));
#27678=CARTESIAN_POINT('Ctrl Pts',(4.67663673184222,-1.2999999999998,6.03366080550892));
#27679=CARTESIAN_POINT('Ctrl Pts',(4.6957990883815,-1.29999999999975,6.03866730859026));
#27680=CARTESIAN_POINT('Ctrl Pts',(4.70888266080627,-1.29999999999972,6.04210425716953));
#27681=CARTESIAN_POINT('Ctrl Pts',(4.70981332848442,-1.29999999999972,6.04234788890545));
#27682=CARTESIAN_POINT('',(4.80833879015672,-1.30000000000006,6.56566721647533));
#27683=CARTESIAN_POINT('Origin',(0.,-1.3,7.2));
#27684=CARTESIAN_POINT('',(4.55333646119701,-1.3,6.70483180220308));
#27685=CARTESIAN_POINT('Ctrl Pts',(4.80833879058776,-1.30000000000005,6.56566721608982));
#27686=CARTESIAN_POINT('Ctrl Pts',(4.80747844806735,-1.30000000000005,6.56622014166603));
#27687=CARTESIAN_POINT('Ctrl Pts',(4.79632873311919,-1.30000000000005,6.5733579152029));
#27688=CARTESIAN_POINT('Ctrl Pts',(4.77472662307004,-1.30000000000003,6.58645074781878));
#27689=CARTESIAN_POINT('Ctrl Pts',(4.7515349646246,-1.30000000000003,6.60128956561561));
#27690=CARTESIAN_POINT('Ctrl Pts',(4.73570235451819,-1.30000000000002,6.60979664855893));
#27691=CARTESIAN_POINT('Ctrl Pts',(4.72523936468665,-1.30000000000002,6.61586137002473));
#27692=CARTESIAN_POINT('Ctrl Pts',(4.71234108790908,-1.30000000000002,6.62410664981093));
#27693=CARTESIAN_POINT('Ctrl Pts',(4.69635329463586,-1.30000000000002,6.63210460558043));
#27694=CARTESIAN_POINT('Ctrl Pts',(4.67274012394597,-1.30000000000002,6.64549193416047));
#27695=CARTESIAN_POINT('Ctrl Pts',(4.64616298310549,-1.30000000000001,6.65922290148753));
#27696=CARTESIAN_POINT('Ctrl Pts',(4.61959384082978,-1.30000000000001,6.67287273622477));
#27697=CARTESIAN_POINT('Ctrl Pts',(4.60066248946865,-1.30000000000001,6.68136532610089));
#27698=CARTESIAN_POINT('Ctrl Pts',(4.58731275561843,-1.3,6.68772391623228));
#27699=CARTESIAN_POINT('Ctrl Pts',(4.57096519811773,-1.3,6.69448853267874));
#27700=CARTESIAN_POINT('Ctrl Pts',(4.55986191625143,-1.3,6.69922697939143));
#27701=CARTESIAN_POINT('Ctrl Pts',(4.55333646119701,-1.3,6.70483180220308));
#27702=CARTESIAN_POINT('',(4.57248821462698,-1.3,6.9348430928224));
#27703=CARTESIAN_POINT('',(4.55333646119701,-1.3,6.70483180220308));
#27704=CARTESIAN_POINT('',(4.84757809483801,-1.3,7.04674656791213));
#27705=CARTESIAN_POINT('Ctrl Pts',(4.57248821462698,-1.3,6.9348430928224));
#27706=CARTESIAN_POINT('Ctrl Pts',(4.58686099902111,-1.3,6.94405440331263));
#27707=CARTESIAN_POINT('Ctrl Pts',(4.60907421143989,-1.30000000000024,6.94591557225086));
#27708=CARTESIAN_POINT('Ctrl Pts',(4.66591701788673,-1.30000000000024,6.9677865529423));
#27709=CARTESIAN_POINT('Ctrl Pts',(4.68947396446559,-1.30000000000016,6.97660500882556));
#27710=CARTESIAN_POINT('Ctrl Pts',(4.75859274645512,-1.30000000000016,7.00421340848844));
#27711=CARTESIAN_POINT('Ctrl Pts',(4.80332270094286,-1.3,7.02507116583801));
#27712=CARTESIAN_POINT('Ctrl Pts',(4.84757809483801,-1.3,7.04674656791213));
#27713=CARTESIAN_POINT('',(4.83514958407044,-1.30000000000004,7.57915194386478));
#27714=CARTESIAN_POINT('Origin',(0.,-1.3,7.2));
#27715=CARTESIAN_POINT('',(4.55678639209675,-1.3,7.66234429787489));
#27716=CARTESIAN_POINT('Ctrl Pts',(4.83514187469075,-1.30000000000002,7.57915490962811));
#27717=CARTESIAN_POINT('Ctrl Pts',(4.83418604828034,-1.30000000000002,7.57952260918312));
#27718=CARTESIAN_POINT('Ctrl Pts',(4.8218053910255,-1.30000000000002,7.58427928601273));
#27719=CARTESIAN_POINT('Ctrl Pts',(4.80369703210634,-1.30000000000002,7.59113993557893));
#27720=CARTESIAN_POINT('Ctrl Pts',(4.78072070206189,-1.30000000000001,7.59826996426714));
#27721=CARTESIAN_POINT('Ctrl Pts',(4.76786499505704,-1.30000000000001,7.60368176740184));
#27722=CARTESIAN_POINT('Ctrl Pts',(4.75923927618335,-1.30000000000001,7.60624853723847));
#27723=CARTESIAN_POINT('Ctrl Pts',(4.75348070600745,-1.30000000000001,7.60784584718063));
#27724=CARTESIAN_POINT('Ctrl Pts',(4.74343057879298,-1.30000000000001,7.61127081391062));
#27725=CARTESIAN_POINT('Ctrl Pts',(4.7290926957189,-1.30000000000001,7.61656804117484));
#27726=CARTESIAN_POINT('Ctrl Pts',(4.71179724858882,-1.30000000000001,7.62108876395165));
#27727=CARTESIAN_POINT('Ctrl Pts',(4.68590468587277,-1.30000000000001,7.62938620214825));
#27728=CARTESIAN_POINT('Ctrl Pts',(4.65997285225601,-1.3,7.63611399060629));
#27729=CARTESIAN_POINT('Ctrl Pts',(4.63687848316794,-1.3,7.64278362359797));
#27730=CARTESIAN_POINT('Ctrl Pts',(4.62245430981319,-1.3,7.64588206265252));
#27731=CARTESIAN_POINT('Ctrl Pts',(4.60795019531382,-1.30000000000002,7.64934885674979));
#27732=CARTESIAN_POINT('Ctrl Pts',(4.59357906309857,-1.3,7.65261768781225));
#27733=CARTESIAN_POINT('Ctrl Pts',(4.57617941896521,-1.3,7.65590048748505));
#27734=CARTESIAN_POINT('Ctrl Pts',(4.56433455848945,-1.3,7.65821867228284));
#27735=CARTESIAN_POINT('Ctrl Pts',(4.55678639209675,-1.3,7.66234429787489));
#27736=CARTESIAN_POINT('',(4.52769759742429,-1.3,7.89131116337361));
#27737=CARTESIAN_POINT('',(4.55678639209675,-1.3,7.66234429787489));
#27738=CARTESIAN_POINT('',(4.77352143851607,-1.29999999999998,8.05790038817306));
#27739=CARTESIAN_POINT('Ctrl Pts',(4.52769759742428,-1.3,7.89131116337361));
#27740=CARTESIAN_POINT('Ctrl Pts',(4.53392313641892,-1.3,7.89746222583599));
#27741=CARTESIAN_POINT('Ctrl Pts',(4.54480756131904,-1.3,7.90313131042928));
#27742=CARTESIAN_POINT('Ctrl Pts',(4.56073300810662,-1.3,7.91156448348519));
#27743=CARTESIAN_POINT('Ctrl Pts',(4.57382741729707,-1.3,7.91886372538035));
#27744=CARTESIAN_POINT('Ctrl Pts',(4.58698548913663,-1.29999999999999,7.92639668444809));
#27745=CARTESIAN_POINT('Ctrl Pts',(4.59965290245868,-1.29999999999999,7.93527268020086));
#27746=CARTESIAN_POINT('Ctrl Pts',(4.62058857472471,-1.29999999999999,7.94740044967715));
#27747=CARTESIAN_POINT('Ctrl Pts',(4.64859413441977,-1.29999999999999,7.96634699488997));
#27748=CARTESIAN_POINT('Ctrl Pts',(4.6816555228702,-1.29999999999997,7.98886506857447));
#27749=CARTESIAN_POINT('Ctrl Pts',(4.70425563008658,-1.29999999999998,8.00520911535576));
#27750=CARTESIAN_POINT('Ctrl Pts',(4.71911478157114,-1.29999999999997,8.01670270298284));
#27751=CARTESIAN_POINT('Ctrl Pts',(4.72917527752168,-1.29999999999997,8.02388370350348));
#27752=CARTESIAN_POINT('Ctrl Pts',(4.74172894757691,-1.29999999999997,8.03290675645269));
#27753=CARTESIAN_POINT('Ctrl Pts',(4.75646184909153,-1.29999999999997,8.04470262929097));
#27754=CARTESIAN_POINT('Ctrl Pts',(4.7670715443958,-1.29999999999996,8.05295673069625));
#27755=CARTESIAN_POINT('Ctrl Pts',(4.77277075263192,-1.29999999999996,8.05732553818437));
#27756=CARTESIAN_POINT('Ctrl Pts',(4.77352143846884,-1.29999999999996,8.05790038813689));
#27757=CARTESIAN_POINT('',(4.65060554698675,-1.30000000000011,8.57636043474658));
#27758=CARTESIAN_POINT('Origin',(0.,-1.3,7.2));
#27759=CARTESIAN_POINT('',(4.36108289177477,-1.3,8.59965012915547));
#27760=CARTESIAN_POINT('Ctrl Pts',(4.65060554698679,-1.30000000000024,8.57636043474659));
#27761=CARTESIAN_POINT('Ctrl Pts',(4.64959949726022,-1.30000000000024,8.57651340723713));
#27762=CARTESIAN_POINT('Ctrl Pts',(4.63651671604971,-1.30000000000024,8.57849253071906));
#27763=CARTESIAN_POINT('Ctrl Pts',(4.62194387170408,-1.30000000000018,8.58059186454646));
#27764=CARTESIAN_POINT('Ctrl Pts',(4.60387932238256,-1.30000000000017,8.58288177294578));
#27765=CARTESIAN_POINT('Ctrl Pts',(4.5949397787931,-1.30000000000016,8.58342037655297));
#27766=CARTESIAN_POINT('Ctrl Pts',(4.58581707049659,-1.30000000000016,8.58509868341759));
#27767=CARTESIAN_POINT('Ctrl Pts',(4.57976379072862,-1.30000000000016,8.5860410540558));
#27768=CARTESIAN_POINT('Ctrl Pts',(4.5527239583302,-1.30000000000016,8.58902013595488));
#27769=CARTESIAN_POINT('Ctrl Pts',(4.51519255717782,-1.30000000000006,8.59274412866406));
#27770=CARTESIAN_POINT('Ctrl Pts',(4.47343222775836,-1.30000000000005,8.59504533441449));
#27771=CARTESIAN_POINT('Ctrl Pts',(4.45248023997978,-1.30000000000004,8.59655638746876));
#27772=CARTESIAN_POINT('Ctrl Pts',(4.44055346921642,-1.30000000000004,8.59708300700705));
#27773=CARTESIAN_POINT('Ctrl Pts',(4.42874610728168,-1.30000000000002,8.59716779009615));
#27774=CARTESIAN_POINT('Ctrl Pts',(4.41383823973776,-1.30000000000004,8.59752605734575));
#27775=CARTESIAN_POINT('Ctrl Pts',(4.39909825262232,-1.30000000000002,8.59776299484744));
#27776=CARTESIAN_POINT('Ctrl Pts',(4.38139541625276,-1.3,8.59735867632484));
#27777=CARTESIAN_POINT('Ctrl Pts',(4.36932387841423,-1.3,8.59718401041836));
#27778=CARTESIAN_POINT('Ctrl Pts',(4.36108289177477,-1.3,8.59965012915547));
#27779=CARTESIAN_POINT('',(4.28502486891058,-1.3,8.81756561880638));
#27780=CARTESIAN_POINT('',(4.36108289177477,-1.3,8.59965012915547));
#27781=CARTESIAN_POINT('',(4.4908419881269,-1.30000000000001,9.03162175071067));
#27782=CARTESIAN_POINT('Ctrl Pts',(4.28502486891058,-1.3,8.81756561880638));
#27783=CARTESIAN_POINT('Ctrl Pts',(4.28983548714458,-1.3,8.82487662813455));
#27784=CARTESIAN_POINT('Ctrl Pts',(4.29930376072647,-1.3,8.8326846148834));
#27785=CARTESIAN_POINT('Ctrl Pts',(4.31312792074243,-1.3,8.84424454248958));
#27786=CARTESIAN_POINT('Ctrl Pts',(4.32441879715599,-1.3,8.85410663225913));
#27787=CARTESIAN_POINT('Ctrl Pts',(4.33572321977293,-1.3,8.86421064164099));
#27788=CARTESIAN_POINT('Ctrl Pts',(4.34626852229515,-1.3,8.87552627071934));
#27789=CARTESIAN_POINT('Ctrl Pts',(4.3642252122643,-1.3,8.89174180979169));
#27790=CARTESIAN_POINT('Ctrl Pts',(4.38767994763106,-1.3,8.91609640196863));
#27791=CARTESIAN_POINT('Ctrl Pts',(4.41533706763616,-1.30000000000001,8.94499626631874));
#27792=CARTESIAN_POINT('Ctrl Pts',(4.43404520828785,-1.30000000000001,8.96568188496965));
#27793=CARTESIAN_POINT('Ctrl Pts',(4.44619000963143,-1.30000000000001,8.98001366847381));
#27794=CARTESIAN_POINT('Ctrl Pts',(4.45453765168017,-1.30000000000001,8.9891294252702));
#27795=CARTESIAN_POINT('Ctrl Pts',(4.46494103395469,-1.30000000000001,9.00056527592794));
#27796=CARTESIAN_POINT('Ctrl Pts',(4.47689956689865,-1.30000000000001,9.0151663505764));
#27797=CARTESIAN_POINT('Ctrl Pts',(4.48556119107646,-1.30000000000001,9.02544560667773));
#27798=CARTESIAN_POINT('Ctrl Pts',(4.49022739352167,-1.30000000000001,9.0309035988107));
#27799=CARTESIAN_POINT('Ctrl Pts',(4.49084198808645,-1.30000000000001,9.0316217506634));
#27800=CARTESIAN_POINT('',(4.2628448153366,-1.30000000000019,9.51314808875148));
#27801=CARTESIAN_POINT('Origin',(0.,-1.3,7.2));
#27802=CARTESIAN_POINT('',(3.97477914228473,-1.3,9.47578453352548));
#27803=CARTESIAN_POINT('Ctrl Pts',(4.26284481543292,-1.29999999999937,9.5131480887536));
#27804=CARTESIAN_POINT('Ctrl Pts',(4.26220643334429,-1.29999999999937,9.51311720919109));
#27805=CARTESIAN_POINT('Ctrl Pts',(4.26156824485443,-1.29999999999937,9.51308588793707));
#27806=CARTESIAN_POINT('Ctrl Pts',(4.26054883619775,-1.29999999999937,9.51303248016318));
#27807=CARTESIAN_POINT('Ctrl Pts',(4.260166989794,-1.29999999999937,9.5130120882434));
#27808=CARTESIAN_POINT('Ctrl Pts',(4.25368275115679,-1.29999999999938,9.51264762263276));
#27809=CARTESIAN_POINT('Ctrl Pts',(4.24178124330855,-1.29999999999946,9.51117036285086));
#27810=CARTESIAN_POINT('Ctrl Pts',(4.22320612684214,-1.2999999999995,9.51079938881588));
#27811=CARTESIAN_POINT('Ctrl Pts',(4.20544580882674,-1.29999999999956,9.50826165136631));
#27812=CARTESIAN_POINT('Ctrl Pts',(4.186869367981,-1.29999999999961,9.50784799049426));
#27813=CARTESIAN_POINT('Ctrl Pts',(4.16917315735985,-1.29999999999964,9.50510377777432));
#27814=CARTESIAN_POINT('Ctrl Pts',(4.15072826469995,-1.2999999999997,9.50428049865621));
#27815=CARTESIAN_POINT('Ctrl Pts',(4.13311774283479,-1.29999999999972,9.50129808886395));
#27816=CARTESIAN_POINT('Ctrl Pts',(4.10903671786789,-1.29999999999976,9.49882516426723));
#27817=CARTESIAN_POINT('Ctrl Pts',(4.08562660246456,-1.29999999999985,9.49464937055402));
#27818=CARTESIAN_POINT('Ctrl Pts',(4.06476527097454,-1.29999999999987,9.49189931303716));
#27819=CARTESIAN_POINT('Ctrl Pts',(4.05300830437223,-1.29999999999988,9.48988652188621));
#27820=CARTESIAN_POINT('Ctrl Pts',(4.04144316270787,-1.2999999999999,9.48751020962115));
#27821=CARTESIAN_POINT('Ctrl Pts',(4.02679641464904,-1.29999999999993,9.48473812544654));
#27822=CARTESIAN_POINT('Ctrl Pts',(4.01233725084337,-1.29999999999994,9.4818865708566));
#27823=CARTESIAN_POINT('Ctrl Pts',(3.99511068658323,-1.29999999999998,9.47779791444728));
#27824=CARTESIAN_POINT('Ctrl Pts',(3.98335277851019,-1.3,9.47508570286587));
#27825=CARTESIAN_POINT('Ctrl Pts',(3.97477914228473,-1.3,9.47578453352548));
#27826=CARTESIAN_POINT('',(3.85507599179486,-1.3,9.6731246947563));
#27827=CARTESIAN_POINT('',(3.97477914228473,-1.3,9.47578453352548));
#27828=CARTESIAN_POINT('',(4.01179369694655,-1.29999999999766,9.92543782412063));
#27829=CARTESIAN_POINT('Ctrl Pts',(3.85507599179486,-1.3,9.6731246947563));
#27830=CARTESIAN_POINT('Ctrl Pts',(3.85826144216748,-1.3,9.6812761247605));
#27831=CARTESIAN_POINT('Ctrl Pts',(3.86592075441167,-1.29999999999977,9.69085660595971));
#27832=CARTESIAN_POINT('Ctrl Pts',(3.87702049239362,-1.29999999999969,9.70505728721368));
#27833=CARTESIAN_POINT('Ctrl Pts',(3.88609751225379,-1.29999999999954,9.71696191407332));
#27834=CARTESIAN_POINT('Ctrl Pts',(3.89668925414945,-1.29999999999939,9.73180622961143));
#27835=CARTESIAN_POINT('Ctrl Pts',(3.90634129735435,-1.29999999999907,9.74759065323404));
#27836=CARTESIAN_POINT('Ctrl Pts',(3.92055275904235,-1.29999999999887,9.76714384265834));
#27837=CARTESIAN_POINT('Ctrl Pts',(3.9429340522804,-1.29999999999834,9.80416499781408));
#27838=CARTESIAN_POINT('Ctrl Pts',(3.96875291306392,-1.29999999999679,9.84603918270465));
#27839=CARTESIAN_POINT('Ctrl Pts',(3.9873515828036,-1.29999999999548,9.87931932511112));
#27840=CARTESIAN_POINT('Ctrl Pts',(3.99403512297734,-1.29999999999538,9.89169252950719));
#27841=CARTESIAN_POINT('Ctrl Pts',(3.99548245121696,-1.29999999999538,9.89448355290195));
#27842=CARTESIAN_POINT('Ctrl Pts',(3.99797166780201,-1.29999999999536,9.89941379417338));
#27843=CARTESIAN_POINT('Ctrl Pts',(4.00320446632786,-1.29999999999526,9.90899225940416));
#27844=CARTESIAN_POINT('Ctrl Pts',(4.00794236274215,-1.29999999999492,9.91824630352297));
#27845=CARTESIAN_POINT('Ctrl Pts',(4.01134148578579,-1.29999999999461,9.92459663707328));
#27846=CARTESIAN_POINT('Ctrl Pts',(4.01179369694582,-1.29999999999457,9.92543782411959));
#27847=CARTESIAN_POINT('',(3.68876499470921,-1.2999999999998,10.3488907275642));
#27848=CARTESIAN_POINT('Origin',(0.,-1.3,7.2));
#27849=CARTESIAN_POINT('',(3.4147584711704,-1.3,10.2524562333546));
#27850=CARTESIAN_POINT('Ctrl Pts',(3.68876499511134,-1.29999999999967,10.3488907275609));
#27851=CARTESIAN_POINT('Ctrl Pts',(3.68778157068785,-1.29999999999968,10.3486180302189));
#27852=CARTESIAN_POINT('Ctrl Pts',(3.68093562331016,-1.29999999999968,10.34668418986));
#27853=CARTESIAN_POINT('Ctrl Pts',(3.66853450170539,-1.29999999999972,10.342623977583));
#27854=CARTESIAN_POINT('Ctrl Pts',(3.65042204492734,-1.29999999999974,10.3384258601431));
#27855=CARTESIAN_POINT('Ctrl Pts',(3.63654746083435,-1.29999999999975,10.333034031973));
#27856=CARTESIAN_POINT('Ctrl Pts',(3.62446370502866,-1.29999999999976,10.3302238019511));
#27857=CARTESIAN_POINT('Ctrl Pts',(3.60720160452375,-1.29999999999979,10.3246930658666));
#27858=CARTESIAN_POINT('Ctrl Pts',(3.58378319929591,-1.29999999999981,10.3178735693703));
#27859=CARTESIAN_POINT('Ctrl Pts',(3.5613867219776,-1.29999999999984,10.309500573553));
#27860=CARTESIAN_POINT('Ctrl Pts',(3.53855149764872,-1.29999999999986,10.3017508966992));
#27861=CARTESIAN_POINT('Ctrl Pts',(3.51929591785349,-1.29999999999993,10.2939294651204));
#27862=CARTESIAN_POINT('Ctrl Pts',(3.49657587699449,-1.29999999999993,10.2859305508819));
#27863=CARTESIAN_POINT('Ctrl Pts',(3.48022950006539,-1.29999999999995,10.2789860295796));
#27864=CARTESIAN_POINT('Ctrl Pts',(3.46380404043213,-1.29999999999997,10.2720051436094));
#27865=CARTESIAN_POINT('Ctrl Pts',(3.4502201710553,-1.29999999999997,10.2662412177574));
#27866=CARTESIAN_POINT('Ctrl Pts',(3.43423105359296,-1.29999999999999,10.258649491102));
#27867=CARTESIAN_POINT('Ctrl Pts',(3.42329004793793,-1.3,10.2535552330257));
#27868=CARTESIAN_POINT('Ctrl Pts',(3.4147584711704,-1.3,10.2524562333546));
#27869=CARTESIAN_POINT('',(3.2566417951307,-1.3,10.4205963541764));
#27870=CARTESIAN_POINT('',(3.4147584711704,-1.3,10.2524562333546));
#27871=CARTESIAN_POINT('',(3.35750201349686,-1.30000000000001,10.6999543181825));
#27872=CARTESIAN_POINT('Ctrl Pts',(3.2566417951307,-1.3,10.4205963541764));
#27873=CARTESIAN_POINT('Ctrl Pts',(3.25806285817521,-1.3,10.4292319482506));
#27874=CARTESIAN_POINT('Ctrl Pts',(3.26356969889493,-1.3,10.4401936173529));
#27875=CARTESIAN_POINT('Ctrl Pts',(3.27142362945852,-1.3,10.4564287702392));
#27876=CARTESIAN_POINT('Ctrl Pts',(3.27796208619394,-1.3,10.4698652030682));
#27877=CARTESIAN_POINT('Ctrl Pts',(3.2860779275434,-1.3,10.4896409410859));
#27878=CARTESIAN_POINT('Ctrl Pts',(3.29502533151807,-1.3,10.5123524713942));
#27879=CARTESIAN_POINT('Ctrl Pts',(3.30450367753534,-1.3,10.5347011036463));
#27880=CARTESIAN_POINT('Ctrl Pts',(3.31134556628297,-1.30000000000001,10.5553067937749));
#27881=CARTESIAN_POINT('Ctrl Pts',(3.31769888764456,-1.30000000000001,10.5725971040919));
#27882=CARTESIAN_POINT('Ctrl Pts',(3.32402656077159,-1.30000000000001,10.5898959986511));
#27883=CARTESIAN_POINT('Ctrl Pts',(3.32983519550124,-1.30000000000001,10.6075611244656));
#27884=CARTESIAN_POINT('Ctrl Pts',(3.33543431689405,-1.30000000000001,10.6253660208349));
#27885=CARTESIAN_POINT('Ctrl Pts',(3.34094149524616,-1.30000000000001,10.6432126996063));
#27886=CARTESIAN_POINT('Ctrl Pts',(3.34862517899022,-1.30000000000001,10.6667657263109));
#27887=CARTESIAN_POINT('Ctrl Pts',(3.35346931197927,-1.30000000000001,10.6861420881869));
#27888=CARTESIAN_POINT('Ctrl Pts',(3.35723434756309,-1.30000000000001,10.6990438624022));
#27889=CARTESIAN_POINT('Ctrl Pts',(3.35750201347149,-1.30000000000001,10.6999543180962));
#27890=CARTESIAN_POINT('',(2.95346386085648,-1.30000000000038,11.0470184848632));
#27891=CARTESIAN_POINT('Origin',(0.,-1.3,7.2));
#27892=CARTESIAN_POINT('',(2.70549646903679,-1.3,10.8957209484761));
#27893=CARTESIAN_POINT('Ctrl Pts',(2.95346386122922,-1.30000000000034,11.0470184849348));
#27894=CARTESIAN_POINT('Ctrl Pts',(2.95255855788318,-1.30000000000034,11.046547241464));
#27895=CARTESIAN_POINT('Ctrl Pts',(2.9462642246173,-1.30000000000027,11.0432322378643));
#27896=CARTESIAN_POINT('Ctrl Pts',(2.93497824004344,-1.30000000000034,11.0366822995913));
#27897=CARTESIAN_POINT('Ctrl Pts',(2.91813452753453,-1.30000000000025,11.0288099698744));
#27898=CARTESIAN_POINT('Ctrl Pts',(2.90568427085911,-1.30000000000026,11.0206511408273));
#27899=CARTESIAN_POINT('Ctrl Pts',(2.8944488945071,-1.30000000000025,11.0153899166468));
#27900=CARTESIAN_POINT('Ctrl Pts',(2.87871424024048,-1.30000000000023,11.0063906910495));
#27901=CARTESIAN_POINT('Ctrl Pts',(2.85722596337419,-1.3000000000002,10.994850673871));
#27902=CARTESIAN_POINT('Ctrl Pts',(2.83706008972697,-1.30000000000017,10.9820037922093));
#27903=CARTESIAN_POINT('Ctrl Pts',(2.81633525801823,-1.30000000000013,10.9696756101453));
#27904=CARTESIAN_POINT('Ctrl Pts',(2.7991269778593,-1.30000000000009,10.9580213491863));
#27905=CARTESIAN_POINT('Ctrl Pts',(2.77856646432003,-1.30000000000008,10.9454735069678));
#27906=CARTESIAN_POINT('Ctrl Pts',(2.76402116993851,-1.30000000000005,10.9352822600267));
#27907=CARTESIAN_POINT('Ctrl Pts',(2.74940605748609,-1.30000000000005,10.9250389677111));
#27908=CARTESIAN_POINT('Ctrl Pts',(2.73731735276373,-1.30000000000003,10.9165770042152));
#27909=CARTESIAN_POINT('Ctrl Pts',(2.72325603000415,-1.30000000000001,10.9058269403026));
#27910=CARTESIAN_POINT('Ctrl Pts',(2.71361311550261,-1.3,10.8985697469187));
#27911=CARTESIAN_POINT('Ctrl Pts',(2.70549646903679,-1.3,10.8957209484761));
#27912=CARTESIAN_POINT('',(2.5158767249182,-1.3,11.0273124987831));
#27913=CARTESIAN_POINT('',(2.70549646903679,-1.3,10.8957209484761));
#27914=CARTESIAN_POINT('',(2.55649102449489,-1.30000000000196,11.3215110871707));
#27915=CARTESIAN_POINT('Ctrl Pts',(2.5158767249182,-1.3,11.0273124987831));
#27916=CARTESIAN_POINT('Ctrl Pts',(2.51547129336049,-1.3,11.036054840028));
#27917=CARTESIAN_POINT('Ctrl Pts',(2.5185714677897,-1.30000000000023,11.0479195112411));
#27918=CARTESIAN_POINT('Ctrl Pts',(2.52295716596346,-1.30000000000031,11.06539891157));
#27919=CARTESIAN_POINT('Ctrl Pts',(2.52635301603749,-1.30000000000046,11.0799823544973));
#27920=CARTESIAN_POINT('Ctrl Pts',(2.52949729038838,-1.30000000000058,11.0948340954078));
#27921=CARTESIAN_POINT('Ctrl Pts',(2.53115568101867,-1.3000000000007,11.1070342157947));
#27922=CARTESIAN_POINT('Ctrl Pts',(2.53311426036291,-1.30000000000078,11.1191314014661));
#27923=CARTESIAN_POINT('Ctrl Pts',(2.53754735173857,-1.30000000000096,11.139780364975));
#27924=CARTESIAN_POINT('Ctrl Pts',(2.54105191070822,-1.30000000000149,11.1706110977417));
#27925=CARTESIAN_POINT('Ctrl Pts',(2.54573452006113,-1.30000000000204,11.2008309367231));
#27926=CARTESIAN_POINT('Ctrl Pts',(2.54836608072526,-1.30000000000237,11.2255071987807));
#27927=CARTESIAN_POINT('Ctrl Pts',(2.54980989363996,-1.30000000000288,11.2393849186443));
#27928=CARTESIAN_POINT('Ctrl Pts',(2.55054244654306,-1.30000000000289,11.2487391367418));
#27929=CARTESIAN_POINT('Ctrl Pts',(2.55109152476666,-1.30000000000291,11.2549467364804));
#27930=CARTESIAN_POINT('Ctrl Pts',(2.55189116477319,-1.30000000000301,11.262654253516));
#27931=CARTESIAN_POINT('Ctrl Pts',(2.55305163254523,-1.30000000000305,11.2718129170801));
#27932=CARTESIAN_POINT('Ctrl Pts',(2.55465518880789,-1.30000000000349,11.2904402301689));
#27933=CARTESIAN_POINT('Ctrl Pts',(2.55552695808368,-1.30000000000399,11.3071186494231));
#27934=CARTESIAN_POINT('Ctrl Pts',(2.55642674563612,-1.30000000000449,11.3205610386322));
#27935=CARTESIAN_POINT('Ctrl Pts',(2.55649102449025,-1.30000000000453,11.3215110871003));
#27936=CARTESIAN_POINT('',(2.08915688129593,-1.30000000000187,11.576970137216));
#27937=CARTESIAN_POINT('Origin',(0.,-1.3,7.2));
#27938=CARTESIAN_POINT('',(1.87799128879385,-1.3,11.3774649241125));
#27939=CARTESIAN_POINT('Ctrl Pts',(2.08915200586581,-1.30000000000102,11.576966073662));
#27940=CARTESIAN_POINT('Ctrl Pts',(2.08836889275514,-1.30000000000101,11.5763133523961));
#27941=CARTESIAN_POINT('Ctrl Pts',(2.0829231840913,-1.30000000000101,11.5717486188595));
#27942=CARTESIAN_POINT('Ctrl Pts',(2.07532697621286,-1.30000000000088,11.5651096373284));
#27943=CARTESIAN_POINT('Ctrl Pts',(2.0670360910251,-1.30000000000089,11.5583394095983));
#27944=CARTESIAN_POINT('Ctrl Pts',(2.06279202116117,-1.30000000000088,11.5550170835899));
#27945=CARTESIAN_POINT('Ctrl Pts',(2.06041334439402,-1.30000000000088,11.5530881430355));
#27946=CARTESIAN_POINT('Ctrl Pts',(2.05008175662487,-1.30000000000087,11.5441639496953));
#27947=CARTESIAN_POINT('Ctrl Pts',(2.02156140521154,-1.3000000000006,11.5201193794785));
#27948=CARTESIAN_POINT('Ctrl Pts',(1.98618970204262,-1.30000000000032,11.4873857546922));
#27949=CARTESIAN_POINT('Ctrl Pts',(1.95657107896346,-1.30000000000022,11.4578927873005));
#27950=CARTESIAN_POINT('Ctrl Pts',(1.9391923383441,-1.30000000000018,11.4412683292772));
#27951=CARTESIAN_POINT('Ctrl Pts',(1.9270492632946,-1.30000000000012,11.4283111506914));
#27952=CARTESIAN_POINT('Ctrl Pts',(1.91488011008762,-1.30000000000009,11.4152490614082));
#27953=CARTESIAN_POINT('Ctrl Pts',(1.90480129625264,-1.30000000000006,11.4044692218263));
#27954=CARTESIAN_POINT('Ctrl Pts',(1.89327770969982,-1.30000000000004,11.3910324012891));
#27955=CARTESIAN_POINT('Ctrl Pts',(1.88533826855939,-1.3,11.3819390151645));
#27956=CARTESIAN_POINT('Ctrl Pts',(1.87799128879384,-1.3,11.3774649241125));
#27957=CARTESIAN_POINT('',(1.66515576931082,-1.3,11.46675672171));
#27958=CARTESIAN_POINT('',(1.87799128879384,-1.3,11.3774649241125));
#27959=CARTESIAN_POINT('',(1.64376583932815,-1.3,11.7629523189989));
#27960=CARTESIAN_POINT('Ctrl Pts',(1.66515576931082,-1.3,11.46675672171));
#27961=CARTESIAN_POINT('Ctrl Pts',(1.66294156245546,-1.3,11.4752237278628));
#27962=CARTESIAN_POINT('Ctrl Pts',(1.66352992364857,-1.3,11.4874744137729));
#27963=CARTESIAN_POINT('Ctrl Pts',(1.66410716288398,-1.3,11.505499322124));
#27964=CARTESIAN_POINT('Ctrl Pts',(1.66462615833061,-1.3,11.5204313880075));
#27965=CARTESIAN_POINT('Ctrl Pts',(1.66400832169345,-1.3,11.5417962198324));
#27966=CARTESIAN_POINT('Ctrl Pts',(1.6629753934554,-1.3,11.5661771710961));
#27967=CARTESIAN_POINT('Ctrl Pts',(1.66253954923371,-1.29999999999999,11.5904501135858));
#27968=CARTESIAN_POINT('Ctrl Pts',(1.66047989040796,-1.29999999999999,11.6120422433131));
#27969=CARTESIAN_POINT('Ctrl Pts',(1.65917440129576,-1.29999999999999,11.6304388748568));
#27970=CARTESIAN_POINT('Ctrl Pts',(1.65825661873327,-1.29999999999999,11.6457250585537));
#27971=CARTESIAN_POINT('Ctrl Pts',(1.65692536543947,-1.3,11.6580787419226));
#27972=CARTESIAN_POINT('Ctrl Pts',(1.65574912520357,-1.3,11.6703942470278));
#27973=CARTESIAN_POINT('Ctrl Pts',(1.6519973873214,-1.29999999999997,11.704362262037));
#27974=CARTESIAN_POINT('Ctrl Pts',(1.64727440390851,-1.29999999999999,11.7363420669453));
#27975=CARTESIAN_POINT('Ctrl Pts',(1.64388919338363,-1.29999999999999,11.7620157535565));
#27976=CARTESIAN_POINT('Ctrl Pts',(1.64376583933432,-1.29999999999999,11.7629523189521));
#27977=CARTESIAN_POINT('',(1.13367999186515,-1.30000000000007,11.9156231271707));
#27978=CARTESIAN_POINT('Origin',(0.,-1.3,7.2));
#27979=CARTESIAN_POINT('',(0.968408877628581,-1.3,11.6766336368644));
#27980=CARTESIAN_POINT('Ctrl Pts',(1.13366791254867,-1.30000000000001,11.9156081970114));
#27981=CARTESIAN_POINT('Ctrl Pts',(1.13302390437827,-1.30000000000001,11.9148121906901));
#27982=CARTESIAN_POINT('Ctrl Pts',(1.12468637038362,-1.30000000000001,11.9045010017064));
#27983=CARTESIAN_POINT('Ctrl Pts',(1.10885180968865,-1.30000000000001,11.884587008504));
#27984=CARTESIAN_POINT('Ctrl Pts',(1.08716165682344,-1.3,11.855446045349));
#27985=CARTESIAN_POINT('Ctrl Pts',(1.06841695418305,-1.3,11.8313959298596));
#27986=CARTESIAN_POINT('Ctrl Pts',(1.05531692441144,-1.3,11.8114079524741));
#27987=CARTESIAN_POINT('Ctrl Pts',(1.03972439720481,-1.3,11.7892518976243));
#27988=CARTESIAN_POINT('Ctrl Pts',(1.0233484645155,-1.3,11.7642300009282));
#27989=CARTESIAN_POINT('Ctrl Pts',(1.00703467199694,-1.3,11.739219370099));
#27990=CARTESIAN_POINT('Ctrl Pts',(0.996639789377799,-1.3,11.7212674543396));
#27991=CARTESIAN_POINT('Ctrl Pts',(0.988936150867075,-1.3,11.7086498444923));
#27992=CARTESIAN_POINT('Ctrl Pts',(0.980511229803915,-1.3,11.6930945208311));
#27993=CARTESIAN_POINT('Ctrl Pts',(0.974665092423395,-1.3,11.6825374812779));
#27994=CARTESIAN_POINT('Ctrl Pts',(0.968408877628581,-1.3,11.6766336368644));
#27995=CARTESIAN_POINT('',(0.741659516280668,-1.3,11.7197232017278));
#27996=CARTESIAN_POINT('',(0.968408877628581,-1.3,11.6766336368644));
#27997=CARTESIAN_POINT('',(0.659062828598954,-1.29999999999948,12.0050115700132));
#27998=CARTESIAN_POINT('Ctrl Pts',(0.741659516280668,-1.3,11.7197232017278));
#27999=CARTESIAN_POINT('Ctrl Pts',(0.739042042488337,-1.3,11.7249376165696));
#28000=CARTESIAN_POINT('Ctrl Pts',(0.736513353027037,-1.29999999999997,
11.7335029101655));
#28001=CARTESIAN_POINT('Ctrl Pts',(0.734690372091585,-1.29999999999996,
11.7455625251115));
#28002=CARTESIAN_POINT('Ctrl Pts',(0.732507359893533,-1.29999999999992,
11.7573468723061));
#28003=CARTESIAN_POINT('Ctrl Pts',(0.729739714965371,-1.2999999999999,11.7720784210858));
#28004=CARTESIAN_POINT('Ctrl Pts',(0.726871111169886,-1.29999999999987,
11.7854327933035));
#28005=CARTESIAN_POINT('Ctrl Pts',(0.724391632493095,-1.29999999999985,
11.7943012189907));
#28006=CARTESIAN_POINT('Ctrl Pts',(0.722742798682037,-1.29999999999985,
11.8002248077555));
#28007=CARTESIAN_POINT('Ctrl Pts',(0.719941170551377,-1.2999999999998,11.8105870027121));
#28008=CARTESIAN_POINT('Ctrl Pts',(0.715773049841678,-1.29999999999985,
11.8312567595427));
#28009=CARTESIAN_POINT('Ctrl Pts',(0.708106339592658,-1.29999999999956,
11.854933747163));
#28010=CARTESIAN_POINT('Ctrl Pts',(0.701392717589497,-1.29999999999949,
11.8785605604877));
#28011=CARTESIAN_POINT('Ctrl Pts',(0.696379212651565,-1.29999999999946,
11.896276690909));
#28012=CARTESIAN_POINT('Ctrl Pts',(0.690660095299637,-1.29999999999939,
11.9139835115396));
#28013=CARTESIAN_POINT('Ctrl Pts',(0.68477416176603,-1.29999999999933,11.9316792283626));
#28014=CARTESIAN_POINT('Ctrl Pts',(0.678549186698806,-1.29999999999919,
11.9493585018481));
#28015=CARTESIAN_POINT('Ctrl Pts',(0.674222718308847,-1.29999999999909,
11.9640876094411));
#28016=CARTESIAN_POINT('Ctrl Pts',(0.667369721617829,-1.29999999999903,
11.9817468175655));
#28017=CARTESIAN_POINT('Ctrl Pts',(0.663034818602077,-1.29999999999887,
11.9943987309871));
#28018=CARTESIAN_POINT('Ctrl Pts',(0.659399632431257,-1.29999999999879,
12.0041138042021));
#28019=CARTESIAN_POINT('Ctrl Pts',(0.659062828590475,-1.29999999999879,
12.0050115700357));
#28020=CARTESIAN_POINT('',(0.128218778230027,-1.30000000000009,12.0483048527994));
#28021=CARTESIAN_POINT('Origin',(0.,-1.3,7.2));
#28022=CARTESIAN_POINT('',(0.0165023515695838,-1.3,11.7801519784138));
#28023=CARTESIAN_POINT('Ctrl Pts',(0.12821877865013,-1.30000000000002,12.0483048532947));
#28024=CARTESIAN_POINT('Ctrl Pts',(0.127767437989379,-1.30000000000002,
12.0473919903599));
#28025=CARTESIAN_POINT('Ctrl Pts',(0.124640289790951,-1.30000000000002,
12.0410103084665));
#28026=CARTESIAN_POINT('Ctrl Pts',(0.120462273527711,-1.30000000000002,
12.0318473446916));
#28027=CARTESIAN_POINT('Ctrl Pts',(0.114879864456106,-1.30000000000002,
12.0209362197056));
#28028=CARTESIAN_POINT('Ctrl Pts',(0.109188261488994,-1.30000000000002,
12.0100407684408));
#28029=CARTESIAN_POINT('Ctrl Pts',(0.103562192797069,-1.3,11.996174288113));
#28030=CARTESIAN_POINT('Ctrl Pts',(0.0947946336556477,-1.30000000000001,
11.9798529787365));
#28031=CARTESIAN_POINT('Ctrl Pts',(0.0830130309314115,-1.3,11.9521871509241));
#28032=CARTESIAN_POINT('Ctrl Pts',(0.0682437123210014,-1.30000000000001,
11.9190458604758));
#28033=CARTESIAN_POINT('Ctrl Pts',(0.0556483962277135,-1.3,11.8855803936));
#28034=CARTESIAN_POINT('Ctrl Pts',(0.0464357783186146,-1.3,11.8633387174799));
#28035=CARTESIAN_POINT('Ctrl Pts',(0.0406518797624009,-1.3,11.8465564726808));
#28036=CARTESIAN_POINT('Ctrl Pts',(0.0348304131678258,-1.3,11.8296763358228));
#28037=CARTESIAN_POINT('Ctrl Pts',(0.0300137202382597,-1.3,11.8157274242518));
#28038=CARTESIAN_POINT('Ctrl Pts',(0.0249486472265611,-1.3,11.798765411714));
#28039=CARTESIAN_POINT('Ctrl Pts',(0.0213943747864759,-1.3,11.7872275498581));
#28040=CARTESIAN_POINT('Ctrl Pts',(0.0165023515695838,-1.3,11.7801519784138));
#28041=CARTESIAN_POINT('',(-0.214250816488161,-1.3,11.775156089792));
#28042=CARTESIAN_POINT('',(0.0165023515695838,-1.3,11.7801519784138));
#28043=CARTESIAN_POINT('',(-0.354232945953444,-1.3,12.0370465182796));
#28044=CARTESIAN_POINT('Ctrl Pts',(-0.214250816488157,-1.3,11.775156089792));
#28045=CARTESIAN_POINT('Ctrl Pts',(-0.226776816940669,-1.3,11.7908161580662));
#28046=CARTESIAN_POINT('Ctrl Pts',(-0.229117821703532,-1.29999999999933,
11.816545516841));
#28047=CARTESIAN_POINT('Ctrl Pts',(-0.314361841081013,-1.29999999999933,
11.9736092487021));
#28048=CARTESIAN_POINT('Ctrl Pts',(-0.33156106808883,-1.3,11.9999679942315));
#28049=CARTESIAN_POINT('Ctrl Pts',(-0.354232945953442,-1.3,12.0370465182796));
#28050=CARTESIAN_POINT('',(-0.882581877102588,-1.30000000000383,11.9690197346898));
#28051=CARTESIAN_POINT('Origin',(0.,-1.3,7.2));
#28052=CARTESIAN_POINT('',(-0.936125406440075,-1.3,11.683495700499));
#28053=CARTESIAN_POINT('Ctrl Pts',(-0.882581877071048,-1.3,11.9690197346817));
#28054=CARTESIAN_POINT('Ctrl Pts',(-0.882808795626795,-1.3,11.9681439377607));
#28055=CARTESIAN_POINT('Ctrl Pts',(-0.883062784706584,-1.3,11.9671488844407));
#28056=CARTESIAN_POINT('Ctrl Pts',(-0.88333561661655,-1.3,11.9660476844872));
#28057=CARTESIAN_POINT('Ctrl Pts',(-0.88444610261044,-1.3,11.96156555802));
#28058=CARTESIAN_POINT('Ctrl Pts',(-0.885768767111217,-1.3,11.955301283602));
#28059=CARTESIAN_POINT('Ctrl Pts',(-0.887564373833532,-1.3,11.9483389250401));
#28060=CARTESIAN_POINT('Ctrl Pts',(-0.889007412258535,-1.3,11.942743629139));
#28061=CARTESIAN_POINT('Ctrl Pts',(-0.890845883878463,-1.3,11.9367181788242));
#28062=CARTESIAN_POINT('Ctrl Pts',(-0.89225592342973,-1.3,11.9305935570264));
#28063=CARTESIAN_POINT('Ctrl Pts',(-0.893647676455054,-1.3,11.9245483642455));
#28064=CARTESIAN_POINT('Ctrl Pts',(-0.894627819898128,-1.3,11.9184090511601));
#28065=CARTESIAN_POINT('Ctrl Pts',(-0.896030179377485,-1.3,11.912883875931));
#28066=CARTESIAN_POINT('Ctrl Pts',(-0.896833031705652,-1.3,11.9097207070992));
#28067=CARTESIAN_POINT('Ctrl Pts',(-0.89773423291985,-1.3,11.9067490121674));
#28068=CARTESIAN_POINT('Ctrl Pts',(-0.898453790759213,-1.3,11.9039975125493));
#28069=CARTESIAN_POINT('Ctrl Pts',(-0.899333475274128,-1.3,11.9006337084541));
#28070=CARTESIAN_POINT('Ctrl Pts',(-0.89998356318908,-1.3,11.8976091563924));
#28071=CARTESIAN_POINT('Ctrl Pts',(-0.900535947202928,-1.3,11.8951297300085));
#28072=CARTESIAN_POINT('Ctrl Pts',(-0.901673468155476,-1.3,11.8900238627289));
#28073=CARTESIAN_POINT('Ctrl Pts',(-0.902046559818047,-1.3,11.8883980818041));
#28074=CARTESIAN_POINT('Ctrl Pts',(-0.902341267799144,-1.3,11.8870932461531));
#28075=CARTESIAN_POINT('Ctrl Pts',(-0.902635975780242,-1.3,11.8857884105021));
#28076=CARTESIAN_POINT('Ctrl Pts',(-0.902931032114102,-1.3,11.8844836710949));
#28077=CARTESIAN_POINT('Ctrl Pts',(-0.903225882890785,-1.3,11.8831788717348));
#28078=CARTESIAN_POINT('Ctrl Pts',(-0.903815584444153,-1.3,11.8805692730148));
#28079=CARTESIAN_POINT('Ctrl Pts',(-0.904404468432412,-1.3,11.8779594230048));
#28080=CARTESIAN_POINT('Ctrl Pts',(-0.904988061452789,-1.3,11.8753482266002));
#28081=CARTESIAN_POINT('Ctrl Pts',(-0.906155247493544,-1.3,11.8701258337912));
#28082=CARTESIAN_POINT('Ctrl Pts',(-0.907301396337968,-1.3,11.8648979451309));
#28083=CARTESIAN_POINT('Ctrl Pts',(-0.908389551665395,-1.3,11.8596576184927));
#28084=CARTESIAN_POINT('Ctrl Pts',(-0.910831876163998,-1.3,11.8478958986293));
#28085=CARTESIAN_POINT('Ctrl Pts',(-0.912979520196815,-1.3,11.8360733641414));
#28086=CARTESIAN_POINT('Ctrl Pts',(-0.915007770053264,-1.3,11.8242316349802));
#28087=CARTESIAN_POINT('Ctrl Pts',(-0.917028179777949,-1.3,11.8124356796258));
#28088=CARTESIAN_POINT('Ctrl Pts',(-0.918931529702551,-1.3,11.8006199242949));
#28089=CARTESIAN_POINT('Ctrl Pts',(-0.920981332184873,-1.3,11.7888327519991));
#28090=CARTESIAN_POINT('Ctrl Pts',(-0.921072479857284,-1.3,11.7883086169527));
#28091=CARTESIAN_POINT('Ctrl Pts',(-0.92116391556169,-1.3,11.7877845386678));
#28092=CARTESIAN_POINT('Ctrl Pts',(-0.921255506017709,-1.3,11.7872604942856));
#28093=CARTESIAN_POINT('Ctrl Pts',(-0.921599708986489,-1.3,11.785291100967));
#28094=CARTESIAN_POINT('Ctrl Pts',(-0.922341321043407,-1.3,11.781792726034));
#28095=CARTESIAN_POINT('Ctrl Pts',(-0.923980128118824,-1.3,11.7711124286227));
#28096=CARTESIAN_POINT('Ctrl Pts',(-0.924788538415726,-1.3,11.7658439241533));
#28097=CARTESIAN_POINT('Ctrl Pts',(-0.925589291106062,-1.3,11.7596504825016));
#28098=CARTESIAN_POINT('Ctrl Pts',(-0.92635697777491,-1.3,11.7534461585483));
#28099=CARTESIAN_POINT('Ctrl Pts',(-0.927121899806116,-1.3,11.7472641779653));
#28100=CARTESIAN_POINT('Ctrl Pts',(-0.927871372060883,-1.3,11.741073829877));
#28101=CARTESIAN_POINT('Ctrl Pts',(-0.928520999957708,-1.3,11.7357687097838));
#28102=CARTESIAN_POINT('Ctrl Pts',(-0.929364645543441,-1.3,11.7288791639835));
#28103=CARTESIAN_POINT('Ctrl Pts',(-0.930049426493481,-1.3,11.7231571743506));
#28104=CARTESIAN_POINT('Ctrl Pts',(-0.93052372837535,-1.3,11.7181547759627));
#28105=CARTESIAN_POINT('Ctrl Pts',(-0.930834677160099,-1.3,11.7148752407995));
#28106=CARTESIAN_POINT('Ctrl Pts',(-0.931065957287747,-1.3,11.7119438225555));
#28107=CARTESIAN_POINT('Ctrl Pts',(-0.931282157598271,-1.3,11.7093208443881));
#28108=CARTESIAN_POINT('Ctrl Pts',(-0.932829264363458,-1.3,11.6905510875003));
#28109=CARTESIAN_POINT('Ctrl Pts',(-0.934376840494585,-1.3,11.6876840266721));
#28110=CARTESIAN_POINT('Ctrl Pts',(-0.936125406440076,-1.3,11.683495700499));
#28111=CARTESIAN_POINT('',(-0.936125406440075,-1.3,11.683495700499));
#28112=CARTESIAN_POINT('Origin',(0.,1.275,7.2));
#28113=CARTESIAN_POINT('',(4.10256677714363E-16,1.3,10.55));
#28114=CARTESIAN_POINT('',(4.07195060716495E-16,1.275,10.525));
#28115=CARTESIAN_POINT('Origin',(0.,1.3,7.2));
#28116=CARTESIAN_POINT('Origin',(0.,1.3,10.5));
#28117=CARTESIAN_POINT('',(-1.13329432476672,1.3,11.9157336622684));
#28118=CARTESIAN_POINT('',(-0.968408877628584,1.3,11.6766336368644));
#28119=CARTESIAN_POINT('Ctrl Pts',(-1.13329432476672,1.3,11.9157336622684));
#28120=CARTESIAN_POINT('Ctrl Pts',(-1.09357982029352,1.3,11.8656069040482));
#28121=CARTESIAN_POINT('Ctrl Pts',(-1.03481352213628,1.30000000000027,11.78447477828));
#28122=CARTESIAN_POINT('Ctrl Pts',(-0.993644753278957,1.30000000000027,
11.7162670765878));
#28123=CARTESIAN_POINT('Ctrl Pts',(-0.992137613505443,1.30000000000026,
11.7141259017487));
#28124=CARTESIAN_POINT('Ctrl Pts',(-0.980066579642223,1.30000000000026,
11.6923013287743));
#28125=CARTESIAN_POINT('Ctrl Pts',(-0.975396089277502,1.3,11.6832273059784));
#28126=CARTESIAN_POINT('Ctrl Pts',(-0.968408877628581,1.3,11.6766336368644));
#28127=CARTESIAN_POINT('',(-0.741659516280671,1.3,11.7197232017278));
#28128=CARTESIAN_POINT('',(-0.968408877628584,1.3,11.6766336368644));
#28129=CARTESIAN_POINT('',(-0.659151153699352,1.29999999999999,12.0049994543784));
#28130=CARTESIAN_POINT('Ctrl Pts',(-0.741659516280671,1.3,11.7197232017278));
#28131=CARTESIAN_POINT('Ctrl Pts',(-0.737733305603289,1.3,11.727544824049));
#28132=CARTESIAN_POINT('Ctrl Pts',(-0.735751588984198,1.3,11.7396469846747));
#28133=CARTESIAN_POINT('Ctrl Pts',(-0.732635446296485,1.3,11.7573965790848));
#28134=CARTESIAN_POINT('Ctrl Pts',(-0.72985761739672,1.3,11.7721099993479));
#28135=CARTESIAN_POINT('Ctrl Pts',(-0.725954358660486,1.3,11.7899072742885));
#28136=CARTESIAN_POINT('Ctrl Pts',(-0.720616710375773,1.3,11.8076573420007));
#28137=CARTESIAN_POINT('Ctrl Pts',(-0.715898913230529,1.3,11.8312928575073));
#28138=CARTESIAN_POINT('Ctrl Pts',(-0.706317872537295,1.29999999999998,
11.8608672626166));
#28139=CARTESIAN_POINT('Ctrl Pts',(-0.696599728536621,1.29999999999999,
11.8962911605939));
#28140=CARTESIAN_POINT('Ctrl Pts',(-0.687924960193452,1.29999999999998,
11.9228443737029));
#28141=CARTESIAN_POINT('Ctrl Pts',(-0.681633248701518,1.29999999999998,
11.9405257597102));
#28142=CARTESIAN_POINT('Ctrl Pts',(-0.677918881824272,1.29999999999998,
11.9523134141152));
#28143=CARTESIAN_POINT('Ctrl Pts',(-0.673216514165749,1.29999999999998,
11.9670400942954));
#28144=CARTESIAN_POINT('Ctrl Pts',(-0.666547092405337,1.29999999999998,
11.9846968609246));
#28145=CARTESIAN_POINT('Ctrl Pts',(-0.661903094886713,1.29999999999998,
11.9973370975437));
#28146=CARTESIAN_POINT('Ctrl Pts',(-0.659471134965142,1.29999999999998,
12.00410729267));
#28147=CARTESIAN_POINT('Ctrl Pts',(-0.659151153717024,1.29999999999998,
12.0049994543292));
#28148=CARTESIAN_POINT('',(-0.128158081915158,1.30000000000259,12.0483064575425));
#28149=CARTESIAN_POINT('Origin',(0.,1.3,7.2));
#28150=CARTESIAN_POINT('',(-0.0165023515695838,1.3,11.7801519784138));
#28151=CARTESIAN_POINT('Ctrl Pts',(-0.128158082004638,1.30000000000001,
12.0483064576567));
#28152=CARTESIAN_POINT('Ctrl Pts',(-0.127706543597735,1.30000000000001,
12.0473941560219));
#28153=CARTESIAN_POINT('Ctrl Pts',(-0.124585249997123,1.30000000000001,
12.0410104377584));
#28154=CARTESIAN_POINT('Ctrl Pts',(-0.119344627363001,1.30000000000001,
12.0290727474592));
#28155=CARTESIAN_POINT('Ctrl Pts',(-0.110353620477029,1.30000000000001,
12.0128019553342));
#28156=CARTESIAN_POINT('Ctrl Pts',(-0.10505905347749,1.30000000000001,11.9988853872125));
#28157=CARTESIAN_POINT('Ctrl Pts',(-0.0990805943072033,1.30000000000001,
11.9880225704775));
#28158=CARTESIAN_POINT('Ctrl Pts',(-0.0915248950042503,1.30000000000001,
11.9715091494637));
#28159=CARTESIAN_POINT('Ctrl Pts',(-0.0802434788763688,1.29999999999999,
11.946707478996));
#28160=CARTESIAN_POINT('Ctrl Pts',(-0.065394987617947,1.30000000000001,
11.9106252544473));
#28161=CARTESIAN_POINT('Ctrl Pts',(-0.0532333790268668,1.3,11.8800519932815));
#28162=CARTESIAN_POINT('Ctrl Pts',(-0.0443578084944021,1.3,11.8577582069453));
#28163=CARTESIAN_POINT('Ctrl Pts',(-0.039728294969975,1.3,11.8437419949466));
#28164=CARTESIAN_POINT('Ctrl Pts',(-0.0347820509500467,1.3,11.8296771141586));
#28165=CARTESIAN_POINT('Ctrl Pts',(-0.0300196112300812,1.3,11.8157273049924));
#28166=CARTESIAN_POINT('Ctrl Pts',(-0.0249390517352318,1.3,11.798765550829));
#28167=CARTESIAN_POINT('Ctrl Pts',(-0.0213943747864967,1.3,11.7872275498223));
#28168=CARTESIAN_POINT('Ctrl Pts',(-0.0165023515695838,1.3,11.7801519784138));
#28169=CARTESIAN_POINT('',(0.214250816488161,1.3,11.775156089792));
#28170=CARTESIAN_POINT('',(-0.0165023515695838,1.3,11.7801519784138));
#28171=CARTESIAN_POINT('',(0.354270609538462,1.30000000000001,12.0370437599031));
#28172=CARTESIAN_POINT('Ctrl Pts',(0.214250816488161,1.3,11.775156089792));
#28173=CARTESIAN_POINT('Ctrl Pts',(0.219717436763954,1.3,11.7819904857988));
#28174=CARTESIAN_POINT('Ctrl Pts',(0.224173980653817,1.3,11.7934174209104));
#28175=CARTESIAN_POINT('Ctrl Pts',(0.23091560441885,1.3,11.8101320480681));
#28176=CARTESIAN_POINT('Ctrl Pts',(0.236687800958387,1.3,11.8239457500398));
#28177=CARTESIAN_POINT('Ctrl Pts',(0.244221948540284,1.3,11.8405462034363));
#28178=CARTESIAN_POINT('Ctrl Pts',(0.253104343833752,1.3,11.8567896804809));
#28179=CARTESIAN_POINT('Ctrl Pts',(0.262803958219338,1.3,11.8789010314179));
#28180=CARTESIAN_POINT('Ctrl Pts',(0.281070358318964,1.3,11.9113009100025));
#28181=CARTESIAN_POINT('Ctrl Pts',(0.29785247370303,1.30000000000001,11.9439420582747));
#28182=CARTESIAN_POINT('Ctrl Pts',(0.313963477925296,1.30000000000001,11.9706688915201));
#28183=CARTESIAN_POINT('Ctrl Pts',(0.323566005429044,1.30000000000001,11.9867005582315));
#28184=CARTESIAN_POINT('Ctrl Pts',(0.330874530740489,1.30000000000001,12.000206898768));
#28185=CARTESIAN_POINT('Ctrl Pts',(0.337855133813077,1.30000000000001,12.0107554280267));
#28186=CARTESIAN_POINT('Ctrl Pts',(0.344387552689543,1.30000000000001,12.0213987101841));
#28187=CARTESIAN_POINT('Ctrl Pts',(0.349955872658189,1.30000000000001,12.0301352547577));
#28188=CARTESIAN_POINT('Ctrl Pts',(0.353770133775808,1.30000000000001,12.03624110066));
#28189=CARTESIAN_POINT('Ctrl Pts',(0.354270609436508,1.30000000000001,12.0370437597396));
#28190=CARTESIAN_POINT('',(0.882649956952474,1.30000000000121,11.9690071349479));
#28191=CARTESIAN_POINT('Origin',(0.,1.3,7.2));
#28192=CARTESIAN_POINT('',(0.936125406440073,1.3,11.683495700499));
#28193=CARTESIAN_POINT('Ctrl Pts',(0.88264995692282,1.3,11.96900713494));
#28194=CARTESIAN_POINT('Ctrl Pts',(0.882911955670296,1.3,11.968026127732));
#28195=CARTESIAN_POINT('Ctrl Pts',(0.883173297900691,1.3,11.9670365544159));
#28196=CARTESIAN_POINT('Ctrl Pts',(0.883432313455179,1.3,11.9660383664123));
#28197=CARTESIAN_POINT('Ctrl Pts',(0.885606849944969,1.3,11.9576581892382));
#28198=CARTESIAN_POINT('Ctrl Pts',(0.887575729343874,1.3,11.9486660469659));
#28199=CARTESIAN_POINT('Ctrl Pts',(0.890061999938986,1.3,11.9394534486077));
#28200=CARTESIAN_POINT('Ctrl Pts',(0.890851962988844,1.3,11.9365263286432));
#28201=CARTESIAN_POINT('Ctrl Pts',(0.891699082744094,1.3,11.9335773147197));
#28202=CARTESIAN_POINT('Ctrl Pts',(0.892445456246523,1.3,11.9305767538767));
#28203=CARTESIAN_POINT('Ctrl Pts',(0.893884265071105,1.3,11.9247924737467));
#28204=CARTESIAN_POINT('Ctrl Pts',(0.894920505793652,1.3,11.9188138340153));
#28205=CARTESIAN_POINT('Ctrl Pts',(0.896299792001618,1.3,11.9128615900811));
#28206=CARTESIAN_POINT('Ctrl Pts',(0.897667983545716,1.3,11.9069572246403));
#28207=CARTESIAN_POINT('Ctrl Pts',(0.899382403484439,1.3,11.9010763914123));
#28208=CARTESIAN_POINT('Ctrl Pts',(0.9007277698223,1.3,11.8951124219187));
#28209=CARTESIAN_POINT('Ctrl Pts',(0.902056064238301,1.3,11.8892241317537));
#28210=CARTESIAN_POINT('Ctrl Pts',(0.903014046033323,1.3,11.883255972996));
#28211=CARTESIAN_POINT('Ctrl Pts',(0.904274193813204,1.3,11.8773973930454));
#28212=CARTESIAN_POINT('Ctrl Pts',(0.905564059685733,1.3,11.8714006500757));
#28213=CARTESIAN_POINT('Ctrl Pts',(0.907156121579215,1.3,11.8655127074693));
#28214=CARTESIAN_POINT('Ctrl Pts',(0.908366580665661,1.3,11.8596450271036));
#28215=CARTESIAN_POINT('Ctrl Pts',(0.909600827504593,1.3,11.8536620360018));
#28216=CARTESIAN_POINT('Ctrl Pts',(0.910447978388727,1.3,11.8477046062916));
#28217=CARTESIAN_POINT('Ctrl Pts',(0.911488139022433,1.3,11.8419426014754));
#28218=CARTESIAN_POINT('Ctrl Pts',(0.912592827853641,1.3,11.8358231405388));
#28219=CARTESIAN_POINT('Ctrl Pts',(0.913887769999808,1.3,11.8299167744627));
#28220=CARTESIAN_POINT('Ctrl Pts',(0.914982579148,1.3,11.8242119452305));
#28221=CARTESIAN_POINT('Ctrl Pts',(0.917527897789361,1.3,11.8109488041483));
#28222=CARTESIAN_POINT('Ctrl Pts',(0.919180222565221,1.3,11.7988189649137));
#28223=CARTESIAN_POINT('Ctrl Pts',(0.920881722724676,1.3,11.7888075686438));
#28224=CARTESIAN_POINT('Ctrl Pts',(0.922057503612529,1.3,11.7818894332975));
#28225=CARTESIAN_POINT('Ctrl Pts',(0.923102561601193,1.3,11.7762464130738));
#28226=CARTESIAN_POINT('Ctrl Pts',(0.923921465389292,1.3,11.771085056656));
#28227=CARTESIAN_POINT('Ctrl Pts',(0.924403404177455,1.3,11.7680475107398));
#28228=CARTESIAN_POINT('Ctrl Pts',(0.924828219757713,1.3,11.7651004509153));
#28229=CARTESIAN_POINT('Ctrl Pts',(0.925198336031033,1.3,11.7622401659214));
#28230=CARTESIAN_POINT('Ctrl Pts',(0.925391797231251,1.3,11.7607450839491));
#28231=CARTESIAN_POINT('Ctrl Pts',(0.92557043456165,1.3,11.7592737494426));
#28232=CARTESIAN_POINT('Ctrl Pts',(0.925741442489917,1.3,11.7578264931109));
#28233=CARTESIAN_POINT('Ctrl Pts',(0.925918111930927,1.3,11.7563313228593));
#28234=CARTESIAN_POINT('Ctrl Pts',(0.926086696269529,1.3,11.754861862917));
#28235=CARTESIAN_POINT('Ctrl Pts',(0.926256816181442,1.3,11.7534184302241));
#28236=CARTESIAN_POINT('Ctrl Pts',(0.927007261063928,1.3,11.7470510587308));
#28237=CARTESIAN_POINT('Ctrl Pts',(0.927774594433632,1.3,11.7411851682608));
#28238=CARTESIAN_POINT('Ctrl Pts',(0.928446980256554,1.3,11.7357385420547));
#28239=CARTESIAN_POINT('Ctrl Pts',(0.929240499769501,1.3,11.7293106787253));
#28240=CARTESIAN_POINT('Ctrl Pts',(0.929908251832915,1.3,11.7234706008434));
#28241=CARTESIAN_POINT('Ctrl Pts',(0.930436366319506,1.3,11.7181271863582));
#28242=CARTESIAN_POINT('Ctrl Pts',(0.930742894038522,1.3,11.7150257666936));
#28243=CARTESIAN_POINT('Ctrl Pts',(0.931003610509611,1.3,11.7120920765099));
#28244=CARTESIAN_POINT('Ctrl Pts',(0.931226895192046,1.3,11.7093048944438));
#28245=CARTESIAN_POINT('Ctrl Pts',(0.931479130591859,1.3,11.7061563310262));
#28246=CARTESIAN_POINT('Ctrl Pts',(0.931693185616966,1.3,11.7031937822063));
#28247=CARTESIAN_POINT('Ctrl Pts',(0.932017858608567,1.3,11.7004007314288));
#28248=CARTESIAN_POINT('Ctrl Pts',(0.932766403025875,1.3,11.69396125965));
#28249=CARTESIAN_POINT('Ctrl Pts',(0.934064984191208,1.3,11.6884310135751));
#28250=CARTESIAN_POINT('Ctrl Pts',(0.936125406440064,1.3,11.683495700499));
#28251=CARTESIAN_POINT('',(1.16079736048698,1.3,11.6306327026976));
#28252=CARTESIAN_POINT('',(0.936125406440074,1.3,11.683495700499));
#28253=CARTESIAN_POINT('',(1.35226619965017,1.3,11.8576685288847));
#28254=CARTESIAN_POINT('Ctrl Pts',(1.16079736048698,1.3,11.6306327026976));
#28255=CARTESIAN_POINT('Ctrl Pts',(1.16756547282336,1.3,11.6361811764895));
#28256=CARTESIAN_POINT('Ctrl Pts',(1.17431337124345,1.3,11.6464259698444));
#28257=CARTESIAN_POINT('Ctrl Pts',(1.1844641184857,1.3,11.6613370682762));
#28258=CARTESIAN_POINT('Ctrl Pts',(1.19279885226841,1.3,11.6737320721675));
#28259=CARTESIAN_POINT('Ctrl Pts',(1.20597861208497,1.3,11.6905975515117));
#28260=CARTESIAN_POINT('Ctrl Pts',(1.22462455149233,1.3,11.7146389274155));
#28261=CARTESIAN_POINT('Ctrl Pts',(1.24342566547099,1.3,11.7386228662457));
#28262=CARTESIAN_POINT('Ctrl Pts',(1.26170958390841,1.30000000000001,11.7595856095273));
#28263=CARTESIAN_POINT('Ctrl Pts',(1.27727352044057,1.30000000000001,11.7785119326797));
#28264=CARTESIAN_POINT('Ctrl Pts',(1.29877215077146,1.30000000000001,11.8012267330547));
#28265=CARTESIAN_POINT('Ctrl Pts',(1.32365521531308,1.30000000000001,11.8288485325488));
#28266=CARTESIAN_POINT('Ctrl Pts',(1.34190888454235,1.30000000000001,11.8474571703315));
#28267=CARTESIAN_POINT('Ctrl Pts',(1.35158289478778,1.30000000000001,11.856991850512));
#28268=CARTESIAN_POINT('Ctrl Pts',(1.35226619956941,1.30000000000001,11.8576685288047));
#28269=CARTESIAN_POINT('',(1.85479302526307,1.30000000000044,11.6813215498401));
#28270=CARTESIAN_POINT('Origin',(0.,1.3,7.2));
#28271=CARTESIAN_POINT('',(1.84783999216022,1.3,11.390889146273));
#28272=CARTESIAN_POINT('Ctrl Pts',(1.85479302522491,1.3,11.6813215498385));
#28273=CARTESIAN_POINT('Ctrl Pts',(1.85749249844584,1.3,11.6158578696262));
#28274=CARTESIAN_POINT('Ctrl Pts',(1.85870424358163,1.3,11.5263025468982));
#28275=CARTESIAN_POINT('Ctrl Pts',(1.84829934772273,1.3,11.4112520763645));
#28276=CARTESIAN_POINT('Ctrl Pts',(1.8458590678981,1.3,11.4014133252669));
#28277=CARTESIAN_POINT('Ctrl Pts',(1.84783999216022,1.3,11.390889146273));
#28278=CARTESIAN_POINT('',(2.05661148970878,1.3,11.2924694059607));
#28279=CARTESIAN_POINT('',(1.84783999216022,1.3,11.390889146273));
#28280=CARTESIAN_POINT('',(2.2911613629891,1.30000000000044,11.4747022830537));
#28281=CARTESIAN_POINT('Ctrl Pts',(2.05661148970878,1.3,11.2924694059607));
#28282=CARTESIAN_POINT('Ctrl Pts',(2.06438529511966,1.3,11.2964894626086));
#28283=CARTESIAN_POINT('Ctrl Pts',(2.07311280409283,1.30000000000005,11.3051080086582));
#28284=CARTESIAN_POINT('Ctrl Pts',(2.08607547837362,1.30000000000005,11.3176312713285));
#28285=CARTESIAN_POINT('Ctrl Pts',(2.09696615016092,1.3000000000001,11.3279028086908));
#28286=CARTESIAN_POINT('Ctrl Pts',(2.11062203159441,1.30000000000011,11.3399881418636));
#28287=CARTESIAN_POINT('Ctrl Pts',(2.12531111485264,1.30000000000018,11.3512371203303));
#28288=CARTESIAN_POINT('Ctrl Pts',(2.14327171669124,1.30000000000022,11.3674145634971));
#28289=CARTESIAN_POINT('Ctrl Pts',(2.17775045539098,1.30000000000032,11.3935430635717));
#28290=CARTESIAN_POINT('Ctrl Pts',(2.21669657645957,1.30000000000061,11.4235975293954));
#28291=CARTESIAN_POINT('Ctrl Pts',(2.24785024885108,1.30000000000087,11.4455731525381));
#28292=CARTESIAN_POINT('Ctrl Pts',(2.25945701905641,1.30000000000088,11.4535134605502));
#28293=CARTESIAN_POINT('Ctrl Pts',(2.26208146734059,1.30000000000088,11.4552446005424));
#28294=CARTESIAN_POINT('Ctrl Pts',(2.2667245028145,1.3000000000009,11.4582355351721));
#28295=CARTESIAN_POINT('Ctrl Pts',(2.27570351210482,1.30000000000087,11.4644408982048));
#28296=CARTESIAN_POINT('Ctrl Pts',(2.28441167791373,1.30000000000097,11.4701202167479));
#28297=CARTESIAN_POINT('Ctrl Pts',(2.2903719830358,1.30000000000101,11.4741645710873));
#28298=CARTESIAN_POINT('Ctrl Pts',(2.29116136298823,1.30000000000102,11.4747022830531));
#28299=CARTESIAN_POINT('',(2.74612652659283,1.3,11.1976604533081));
#28300=CARTESIAN_POINT('Origin',(0.,1.3,7.2));
#28301=CARTESIAN_POINT('',(2.67879510330291,1.3,10.9151206262376));
#28302=CARTESIAN_POINT('Ctrl Pts',(2.74612652659282,1.3,11.1976604533081));
#28303=CARTESIAN_POINT('Ctrl Pts',(2.74596451589451,1.3,11.19665402888));
#28304=CARTESIAN_POINT('Ctrl Pts',(2.74580163938371,1.3,11.1956477001141));
#28305=CARTESIAN_POINT('Ctrl Pts',(2.74563797152551,1.3,11.1946414582487));
#28306=CARTESIAN_POINT('Ctrl Pts',(2.74368370235821,1.3,11.1826264696363));
#28307=CARTESIAN_POINT('Ctrl Pts',(2.74161741958818,1.3,11.1706227867786));
#28308=CARTESIAN_POINT('Ctrl Pts',(2.73928525122789,1.3,11.1586662116773));
#28309=CARTESIAN_POINT('Ctrl Pts',(2.73870662877036,1.3,11.1556997265013));
#28310=CARTESIAN_POINT('Ctrl Pts',(2.7381117435708,1.3,11.1527361231565));
#28311=CARTESIAN_POINT('Ctrl Pts',(2.73746409185162,1.3,11.1497825766952));
#28312=CARTESIAN_POINT('Ctrl Pts',(2.73681764724266,1.3,11.1468345351311));
#28313=CARTESIAN_POINT('Ctrl Pts',(2.73611954983319,1.3,11.1438967384406));
#28314=CARTESIAN_POINT('Ctrl Pts',(2.73557366467298,1.3,11.1409300364769));
#28315=CARTESIAN_POINT('Ctrl Pts',(2.73501877686395,1.3,11.1379144081495));
#28316=CARTESIAN_POINT('Ctrl Pts',(2.73461628430988,1.3,11.1348691468756));
#28317=CARTESIAN_POINT('Ctrl Pts',(2.73415960583626,1.3,11.1318333756012));
#28318=CARTESIAN_POINT('Ctrl Pts',(2.73393195089181,1.3,11.1303200387992));
#28319=CARTESIAN_POINT('Ctrl Pts',(2.73369124569482,1.3,11.1288090442376));
#28320=CARTESIAN_POINT('Ctrl Pts',(2.73341248846247,1.3,11.1273055115503));
#28321=CARTESIAN_POINT('Ctrl Pts',(2.73313667795592,1.3,11.1258178726158));
#28322=CARTESIAN_POINT('Ctrl Pts',(2.73282314053844,1.3,11.1243376848035));
#28323=CARTESIAN_POINT('Ctrl Pts',(2.73250766432533,1.3,11.1228579486607));
#28324=CARTESIAN_POINT('Ctrl Pts',(2.73124858845734,1.3,11.1169522733956));
#28325=CARTESIAN_POINT('Ctrl Pts',(2.72996157700056,1.3,11.1110529795643));
#28326=CARTESIAN_POINT('Ctrl Pts',(2.72872025058404,1.3,11.1051442288111));
#28327=CARTESIAN_POINT('Ctrl Pts',(2.72747735620529,1.3,11.099228014511));
#28328=CARTESIAN_POINT('Ctrl Pts',(2.72628009813441,1.3,11.0933015722916));
#28329=CARTESIAN_POINT('Ctrl Pts',(2.72498683323779,1.3,11.0873959758342));
#28330=CARTESIAN_POINT('Ctrl Pts',(2.72241841329655,1.3,11.0756674801904));
#28331=CARTESIAN_POINT('Ctrl Pts',(2.71946779623975,1.3,11.0640269669922));
#28332=CARTESIAN_POINT('Ctrl Pts',(2.71652343305083,1.3,11.0523920562829));
#28333=CARTESIAN_POINT('Ctrl Pts',(2.71358373997865,1.3,11.0407755999517));
#28334=CARTESIAN_POINT('Ctrl Pts',(2.71065147471426,1.3,11.0291615051628));
#28335=CARTESIAN_POINT('Ctrl Pts',(2.70771716723947,1.3,11.0175458216236));
#28336=CARTESIAN_POINT('Ctrl Pts',(2.70625043780106,1.3,11.0117396594745));
#28337=CARTESIAN_POINT('Ctrl Pts',(2.70478323191785,1.3,11.0059327406934));
#28338=CARTESIAN_POINT('Ctrl Pts',(2.70323987718174,1.3,11.0001465555415));
#28339=CARTESIAN_POINT('Ctrl Pts',(2.70247147803797,1.3,10.9972657533433));
#28340=CARTESIAN_POINT('Ctrl Pts',(2.70168438254399,1.3,10.9943900335713));
#28341=CARTESIAN_POINT('Ctrl Pts',(2.70083970447103,1.3,10.9915311919127));
#28342=CARTESIAN_POINT('Ctrl Pts',(2.70000086668158,1.3,10.9886921168923));
#28343=CARTESIAN_POINT('Ctrl Pts',(2.69910470091314,1.3,10.9858700981927));
#28344=CARTESIAN_POINT('Ctrl Pts',(2.69822575948921,1.3,10.98304354175));
#28345=CARTESIAN_POINT('Ctrl Pts',(2.69625160085045,1.3,10.9766949152462));
#28346=CARTESIAN_POINT('Ctrl Pts',(2.69437215817735,1.3,10.9703739764371));
#28347=CARTESIAN_POINT('Ctrl Pts',(2.69304746703953,1.3,10.9659932897602));
#28348=CARTESIAN_POINT('Ctrl Pts',(2.69119548416497,1.3,10.9598688759457));
#28349=CARTESIAN_POINT('Ctrl Pts',(2.68998601190985,1.3,10.9558289925951));
#28350=CARTESIAN_POINT('Ctrl Pts',(2.68772315303807,1.3,10.9490869229178));
#28351=CARTESIAN_POINT('Ctrl Pts',(2.68687354912832,1.3,10.9465555724969));
#28352=CARTESIAN_POINT('Ctrl Pts',(2.68580897072893,1.3,10.9435039196507));
#28353=CARTESIAN_POINT('Ctrl Pts',(2.68483500056766,1.3,10.9407017314786));
#28354=CARTESIAN_POINT('Ctrl Pts',(2.68164275703609,1.3,10.9315173976843));
#28355=CARTESIAN_POINT('Ctrl Pts',(2.67898731875167,1.3,10.9233368709496));
#28356=CARTESIAN_POINT('Ctrl Pts',(2.67879510330291,1.3,10.9151206262376));
#28357=CARTESIAN_POINT('',(2.86254182811346,1.3,10.7754455583364));
#28358=CARTESIAN_POINT('',(2.67879510330291,1.3,10.9151206262376));
#28359=CARTESIAN_POINT('',(3.1297306010244,1.30000000000014,10.9050352717634));
#28360=CARTESIAN_POINT('Ctrl Pts',(2.86254182811346,1.3,10.7754455583364));
#28361=CARTESIAN_POINT('Ctrl Pts',(2.87098157399952,1.3,10.7777615020743));
#28362=CARTESIAN_POINT('Ctrl Pts',(2.88129518337835,1.30000000000003,10.7843931284862));
#28363=CARTESIAN_POINT('Ctrl Pts',(2.89656867358042,1.30000000000002,10.7939563838538));
#28364=CARTESIAN_POINT('Ctrl Pts',(2.90935734036008,1.30000000000004,10.8017417133146));
#28365=CARTESIAN_POINT('Ctrl Pts',(2.92519160082833,1.30000000000006,10.8107532722469));
#28366=CARTESIAN_POINT('Ctrl Pts',(2.94194585038891,1.30000000000006,10.8186721958535));
#28367=CARTESIAN_POINT('Ctrl Pts',(2.96266976928765,1.30000000000008,10.8309787346033));
#28368=CARTESIAN_POINT('Ctrl Pts',(2.98251244358946,1.30000000000014,10.8398773562819));
#28369=CARTESIAN_POINT('Ctrl Pts',(3.00474611284772,1.30000000000016,10.8505077189706));
#28370=CARTESIAN_POINT('Ctrl Pts',(3.02671111250602,1.3000000000002,10.8614078746728));
#28371=CARTESIAN_POINT('Ctrl Pts',(3.04946200615208,1.30000000000022,10.8714147740806));
#28372=CARTESIAN_POINT('Ctrl Pts',(3.06679325766632,1.30000000000024,10.8785906567429));
#28373=CARTESIAN_POINT('Ctrl Pts',(3.07804152851698,1.30000000000026,10.8837146344997));
#28374=CARTESIAN_POINT('Ctrl Pts',(3.09212660927841,1.30000000000026,10.8900802463094));
#28375=CARTESIAN_POINT('Ctrl Pts',(3.10970701250653,1.30000000000029,10.8969430220631));
#28376=CARTESIAN_POINT('Ctrl Pts',(3.12220207956528,1.30000000000031,10.9019527342208));
#28377=CARTESIAN_POINT('Ctrl Pts',(3.12885620798913,1.30000000000033,10.9046768064315));
#28378=CARTESIAN_POINT('Ctrl Pts',(3.12973060094966,1.30000000000033,10.9050352717328));
#28379=CARTESIAN_POINT('',(3.51702417252248,1.30000000000004,10.5396168896264));
#28380=CARTESIAN_POINT('Origin',(0.,1.3,7.2));
#28381=CARTESIAN_POINT('',(3.39267401414619,1.3,10.2769835077089));
#28382=CARTESIAN_POINT('Ctrl Pts',(3.51702417248271,1.3,10.5396168896419));
#28383=CARTESIAN_POINT('Ctrl Pts',(3.49672647112758,1.3,10.4875123140426));
#28384=CARTESIAN_POINT('Ctrl Pts',(3.46275940082978,1.3,10.4051664173467));
#28385=CARTESIAN_POINT('Ctrl Pts',(3.4011770434785,1.3,10.2950140468319));
#28386=CARTESIAN_POINT('Ctrl Pts',(3.39510833417347,1.3,10.2872492564874));
#28387=CARTESIAN_POINT('Ctrl Pts',(3.39267401414619,1.3,10.276983507709));
#28388=CARTESIAN_POINT('',(3.54336535262991,1.3,10.1021575829215));
#28389=CARTESIAN_POINT('',(3.39267401414619,1.3,10.2769835077089));
#28390=CARTESIAN_POINT('',(3.8316570030416,1.29999999999986,10.1733658723814));
#28391=CARTESIAN_POINT('Ctrl Pts',(3.54336535262991,1.3,10.1021575829215));
#28392=CARTESIAN_POINT('Ctrl Pts',(3.55210218159755,1.3,10.1026681958948));
#28393=CARTESIAN_POINT('Ctrl Pts',(3.56356899629571,1.29999999999999,10.1070114760009));
#28394=CARTESIAN_POINT('Ctrl Pts',(3.58049697517908,1.29999999999998,10.113190435319));
#28395=CARTESIAN_POINT('Ctrl Pts',(3.59462471573536,1.29999999999995,10.1181472229321));
#28396=CARTESIAN_POINT('Ctrl Pts',(3.61198647845491,1.29999999999995,10.12367003144));
#28397=CARTESIAN_POINT('Ctrl Pts',(3.63002093128387,1.29999999999992,10.1279329457953));
#28398=CARTESIAN_POINT('Ctrl Pts',(3.65285062374733,1.29999999999992,10.1356618793807));
#28399=CARTESIAN_POINT('Ctrl Pts',(3.67410984172058,1.29999999999985,10.1402406910406));
#28400=CARTESIAN_POINT('Ctrl Pts',(3.6980678619775,1.29999999999983,10.1460160834464));
#28401=CARTESIAN_POINT('Ctrl Pts',(3.72181914762373,1.29999999999981,10.1521112671248));
#28402=CARTESIAN_POINT('Ctrl Pts',(3.74615344929343,1.29999999999978,10.1571692337866));
#28403=CARTESIAN_POINT('Ctrl Pts',(3.76459792690676,1.29999999999976,10.1605848969376));
#28404=CARTESIAN_POINT('Ctrl Pts',(3.77666573049054,1.29999999999974,10.1632582465006));
#28405=CARTESIAN_POINT('Ctrl Pts',(3.79176649230709,1.29999999999974,10.1665562922193));
#28406=CARTESIAN_POINT('Ctrl Pts',(3.81038957161618,1.2999999999997,10.1696138666325));
#28407=CARTESIAN_POINT('Ctrl Pts',(3.82365280763186,1.29999999999968,10.1719161377918));
#28408=CARTESIAN_POINT('Ctrl Pts',(3.83072754430228,1.29999999999967,10.173197107173));
#28409=CARTESIAN_POINT('Ctrl Pts',(3.83165700295789,1.29999999999967,10.1733658723663));
#28410=CARTESIAN_POINT('',(4.13460022854383,1.2999999999976,9.7352069526073));
#28411=CARTESIAN_POINT('Origin',(0.,1.3,7.2));
#28412=CARTESIAN_POINT('',(3.95827679071515,1.3,9.50436744488836));
#28413=CARTESIAN_POINT('Ctrl Pts',(4.13458086813857,1.3,9.73517804740468));
#28414=CARTESIAN_POINT('Ctrl Pts',(4.08546280420686,1.3,9.66185452740355));
#28415=CARTESIAN_POINT('Ctrl Pts',(4.04234444364633,1.3,9.6029319619877));
#28416=CARTESIAN_POINT('Ctrl Pts',(3.96268006345613,1.3,9.511257093339));
#28417=CARTESIAN_POINT('Ctrl Pts',(3.96053997251118,1.3,9.50914656897965));
#28418=CARTESIAN_POINT('Ctrl Pts',(3.95827679071515,1.3,9.50436744488836));
#28419=CARTESIAN_POINT('',(4.06932680828303,1.3,9.30203139503569));
#28420=CARTESIAN_POINT('',(3.95827679071515,1.3,9.50436744488836));
#28421=CARTESIAN_POINT('',(4.36609756959125,1.29999999999973,9.31179828885486));
#28422=CARTESIAN_POINT('Ctrl Pts',(4.06932680828303,1.3,9.30203139503569));
#28423=CARTESIAN_POINT('Ctrl Pts',(4.07797887898238,1.3,9.30071436100745));
#28424=CARTESIAN_POINT('Ctrl Pts',(4.09011069171085,1.29999999999996,9.30253751130118));
#28425=CARTESIAN_POINT('Ctrl Pts',(4.10795583415653,1.29999999999994,9.30506364957931));
#28426=CARTESIAN_POINT('Ctrl Pts',(4.12281928798903,1.29999999999992,9.30690417832915));
#28427=CARTESIAN_POINT('Ctrl Pts',(4.13792366935278,1.29999999999991,9.30846318087845));
#28428=CARTESIAN_POINT('Ctrl Pts',(4.15023209615125,1.29999999999988,9.3088328818803));
#28429=CARTESIAN_POINT('Ctrl Pts',(4.16247876162117,1.29999999999988,9.30949047140628));
#28430=CARTESIAN_POINT('Ctrl Pts',(4.18345672109247,1.29999999999984,9.31179756901066));
#28431=CARTESIAN_POINT('Ctrl Pts',(4.20827437817346,1.29999999999976,9.31201935419063));
#28432=CARTESIAN_POINT('Ctrl Pts',(4.23283302083266,1.29999999999972,9.3128856552204));
#28433=CARTESIAN_POINT('Ctrl Pts',(4.25122160285819,1.29999999999969,9.31361866027968));
#28434=CARTESIAN_POINT('Ctrl Pts',(4.26981671664902,1.29999999999964,9.31368244807499));
#28435=CARTESIAN_POINT('Ctrl Pts',(4.28847502205149,1.29999999999959,9.31351820624347));
#28436=CARTESIAN_POINT('Ctrl Pts',(4.30716480650586,1.29999999999956,9.31320732627316));
#28437=CARTESIAN_POINT('Ctrl Pts',(4.32563404344978,1.29999999999949,9.31355938218807));
#28438=CARTESIAN_POINT('Ctrl Pts',(4.34458714565271,1.29999999999946,9.31234956827253));
#28439=CARTESIAN_POINT('Ctrl Pts',(4.35714349439214,1.29999999999938,9.31234301972474));
#28440=CARTESIAN_POINT('Ctrl Pts',(4.36384001426254,1.29999999999937,9.31193092960279));
#28441=CARTESIAN_POINT('Ctrl Pts',(4.36462701760224,1.29999999999937,9.31188523907631));
#28442=CARTESIAN_POINT('Ctrl Pts',(4.3653799997326,1.29999999999937,9.31183950868406));
#28443=CARTESIAN_POINT('Ctrl Pts',(4.36593552968483,1.29999999999937,9.31180750976769));
#28444=CARTESIAN_POINT('Ctrl Pts',(4.36609756959125,1.29999999999937,9.31179828885486));
#28445=CARTESIAN_POINT('',(4.57140911793407,1.30000000000128,8.82009835380608));
#28446=CARTESIAN_POINT('Origin',(0.,1.3,7.2));
#28447=CARTESIAN_POINT('',(4.35088387761047,1.3,8.63103946714436));
#28448=CARTESIAN_POINT('Ctrl Pts',(4.57140911790143,1.3,8.82009835383949));
#28449=CARTESIAN_POINT('Ctrl Pts',(4.5706814231909,1.3,8.81938742440423));
#28450=CARTESIAN_POINT('Ctrl Pts',(4.56995109704004,1.3,8.81868077650572));
#28451=CARTESIAN_POINT('Ctrl Pts',(4.56921748737933,1.3,8.81797917609138));
#28452=CARTESIAN_POINT('Ctrl Pts',(4.56480235883729,1.3,8.81375669078291));
#28453=CARTESIAN_POINT('Ctrl Pts',(4.56027147065103,1.3,8.80971586453579));
#28454=CARTESIAN_POINT('Ctrl Pts',(4.55597042156158,1.3,8.80551114442447));
#28455=CARTESIAN_POINT('Ctrl Pts',(4.5515560546328,1.3,8.80119564441083));
#28456=CARTESIAN_POINT('Ctrl Pts',(4.54737114764275,1.3,8.79671564866395));
#28457=CARTESIAN_POINT('Ctrl Pts',(4.54294046767687,1.3,8.79259015797614));
#28458=CARTESIAN_POINT('Ctrl Pts',(4.53847171520424,1.3,8.78842921725059));
#28459=CARTESIAN_POINT('Ctrl Pts',(4.53376239388215,1.3,8.78462570418076));
#28460=CARTESIAN_POINT('Ctrl Pts',(4.52949040409136,1.3,8.78046646176674));
#28461=CARTESIAN_POINT('Ctrl Pts',(4.52727670177039,1.3,8.77831118400713));
#28462=CARTESIAN_POINT('Ctrl Pts',(4.52517288265194,1.3,8.77606700032968));
#28463=CARTESIAN_POINT('Ctrl Pts',(4.52300760269494,1.3,8.77392186038719));
#28464=CARTESIAN_POINT('Ctrl Pts',(4.52083180190261,1.3,8.77176629746728));
#28465=CARTESIAN_POINT('Ctrl Pts',(4.51859492702336,1.3,8.76971040774127));
#28466=CARTESIAN_POINT('Ctrl Pts',(4.51637518841834,1.3,8.76767197520911));
#28467=CARTESIAN_POINT('Ctrl Pts',(4.50713124681152,1.3,8.7591830696893));
#28468=CARTESIAN_POINT('Ctrl Pts',(4.49817607520628,1.3,8.75100076229712));
#28469=CARTESIAN_POINT('Ctrl Pts',(4.48948341155244,1.3,8.74333183809486));
#28470=CARTESIAN_POINT('Ctrl Pts',(4.47994963627258,1.3,8.73492086041367));
#28471=CARTESIAN_POINT('Ctrl Pts',(4.47074451497491,1.3,8.72711603709132));
#28472=CARTESIAN_POINT('Ctrl Pts',(4.46212271757076,1.3,8.71986344315658));
#28473=CARTESIAN_POINT('Ctrl Pts',(4.4491396707095,1.3,8.70894219756165));
#28474=CARTESIAN_POINT('Ctrl Pts',(4.43747485629493,1.3,8.69927577567235));
#28475=CARTESIAN_POINT('Ctrl Pts',(4.42761872805175,1.3,8.69109174442388));
#28476=CARTESIAN_POINT('Ctrl Pts',(4.42252179250726,1.3,8.68685950649654));
#28477=CARTESIAN_POINT('Ctrl Pts',(4.41788967791717,1.3,8.68304533279346));
#28478=CARTESIAN_POINT('Ctrl Pts',(4.41368050107165,1.3,8.6798232258243));
#28479=CARTESIAN_POINT('Ctrl Pts',(4.4111202398016,1.3,8.67786335671357));
#28480=CARTESIAN_POINT('Ctrl Pts',(4.4087266150474,1.3,8.67611069656105));
#28481=CARTESIAN_POINT('Ctrl Pts',(4.40656831116804,1.3,8.67450505586071));
#28482=CARTESIAN_POINT('Ctrl Pts',(4.40006247096172,1.3,8.66966512487367));
#28483=CARTESIAN_POINT('Ctrl Pts',(4.39588688861348,1.3,8.6664490557388));
#28484=CARTESIAN_POINT('Ctrl Pts',(4.39234740865121,1.3,8.66377079335119));
#28485=CARTESIAN_POINT('Ctrl Pts',(4.38738609061361,1.3,8.66001665103798));
#28486=CARTESIAN_POINT('Ctrl Pts',(4.38385031613455,1.3,8.65733159560148));
#28487=CARTESIAN_POINT('Ctrl Pts',(4.37809180956932,1.3,8.65323937484063));
#28488=CARTESIAN_POINT('Ctrl Pts',(4.37589487582872,1.3,8.65167814750474));
#28489=CARTESIAN_POINT('Ctrl Pts',(4.37324823329501,1.3,8.64984331524573));
#28490=CARTESIAN_POINT('Ctrl Pts',(4.3708229365894,1.3,8.64815914175065));
#28491=CARTESIAN_POINT('Ctrl Pts',(4.36278432406233,1.3,8.64257697189741));
#28492=CARTESIAN_POINT('Ctrl Pts',(4.35585193117194,1.3,8.63755149448732));
#28493=CARTESIAN_POINT('Ctrl Pts',(4.35088387761047,1.3,8.63103946714436));
#28494=CARTESIAN_POINT('',(4.41743915561768,1.3,8.41003634852114));
#28495=CARTESIAN_POINT('',(4.35088387761047,1.3,8.63103946714436));
#28496=CARTESIAN_POINT('',(4.70979663593526,1.3000000000001,8.35772002147866));
#28497=CARTESIAN_POINT('Ctrl Pts',(4.41743915561768,1.3,8.41003634852114));
#28498=CARTESIAN_POINT('Ctrl Pts',(4.42562833104196,1.3,8.40694922819813));
#28499=CARTESIAN_POINT('Ctrl Pts',(4.43787350489845,1.30000000000001,8.40622766486505));
#28500=CARTESIAN_POINT('Ctrl Pts',(4.45585351305901,1.30000000000001,8.40499606910573));
#28501=CARTESIAN_POINT('Ctrl Pts',(4.47077483084096,1.30000000000003,8.40371437127723));
#28502=CARTESIAN_POINT('Ctrl Pts',(4.48587205596936,1.30000000000003,8.40211582040918));
#28503=CARTESIAN_POINT('Ctrl Pts',(4.4979897136352,1.30000000000004,8.39991299338427));
#28504=CARTESIAN_POINT('Ctrl Pts',(4.51009815468572,1.30000000000004,8.39805546525287));
#28505=CARTESIAN_POINT('Ctrl Pts',(4.53111879558693,1.30000000000004,8.39580460547943));
#28506=CARTESIAN_POINT('Ctrl Pts',(4.57364955024891,1.30000000000008,8.38742647237147));
#28507=CARTESIAN_POINT('Ctrl Pts',(4.61136873806362,1.30000000000014,8.38124836466501));
#28508=CARTESIAN_POINT('Ctrl Pts',(4.63873844454836,1.30000000000016,8.37465149171448));
#28509=CARTESIAN_POINT('Ctrl Pts',(4.64481218242238,1.30000000000016,8.37325265104856));
#28510=CARTESIAN_POINT('Ctrl Pts',(4.65390368130274,1.30000000000016,8.37132464930544));
#28511=CARTESIAN_POINT('Ctrl Pts',(4.66297291571428,1.30000000000017,8.36958456723215));
#28512=CARTESIAN_POINT('Ctrl Pts',(4.68119597547622,1.30000000000017,8.36523210052763));
#28513=CARTESIAN_POINT('Ctrl Pts',(4.6958131149506,1.30000000000022,8.3611827857283));
#28514=CARTESIAN_POINT('Ctrl Pts',(4.70887301296434,1.30000000000024,8.35794751342532));
#28515=CARTESIAN_POINT('Ctrl Pts',(4.70979663583784,1.30000000000024,8.35772002150267));
#28516=CARTESIAN_POINT('',(4.80835060743154,1.3,7.83424319963977));
#28517=CARTESIAN_POINT('Origin',(0.,1.3,7.2));
#28518=CARTESIAN_POINT('',(4.55333646119701,1.3,7.69516819779692));
#28519=CARTESIAN_POINT('Ctrl Pts',(4.80835060754372,1.29999999999996,7.8342431997438));
#28520=CARTESIAN_POINT('Ctrl Pts',(4.80749051866453,1.29999999999996,7.83369878716171));
#28521=CARTESIAN_POINT('Ctrl Pts',(4.80146805113317,1.29999999999996,7.8299273448685));
#28522=CARTESIAN_POINT('Ctrl Pts',(4.79014356570026,1.29999999999996,7.82346765255662));
#28523=CARTESIAN_POINT('Ctrl Pts',(4.7749017311504,1.29999999999998,7.81282514770577));
#28524=CARTESIAN_POINT('Ctrl Pts',(4.76161483790886,1.29999999999997,7.80610490563682));
#28525=CARTESIAN_POINT('Ctrl Pts',(4.75143645340678,1.29999999999997,7.79902370870334));
#28526=CARTESIAN_POINT('Ctrl Pts',(4.73580330060841,1.29999999999997,7.78978321737489));
#28527=CARTESIAN_POINT('Ctrl Pts',(4.7123168197138,1.29999999999999,7.77597081284977));
#28528=CARTESIAN_POINT('Ctrl Pts',(4.67798440200463,1.29999999999997,7.75743185110967));
#28529=CARTESIAN_POINT('Ctrl Pts',(4.64884999722387,1.29999999999999,7.74214044075126));
#28530=CARTESIAN_POINT('Ctrl Pts',(4.62760606760101,1.29999999999999,7.73098319622892));
#28531=CARTESIAN_POINT('Ctrl Pts',(4.61415054115611,1.29999999999999,7.72491389336459));
#28532=CARTESIAN_POINT('Ctrl Pts',(4.60067972068881,1.29999999999999,7.71852453663296));
#28533=CARTESIAN_POINT('Ctrl Pts',(4.5873040871705,1.29999999999999,7.71233002722669));
#28534=CARTESIAN_POINT('Ctrl Pts',(4.5709662969739,1.29999999999999,7.70550430059969));
#28535=CARTESIAN_POINT('Ctrl Pts',(4.55986191621585,1.3,7.70077302060486));
#28536=CARTESIAN_POINT('Ctrl Pts',(4.55333646119701,1.3,7.69516819779692));
#28537=CARTESIAN_POINT('',(4.57248821462698,1.3,7.4651569071776));
#28538=CARTESIAN_POINT('',(4.55333646119701,1.3,7.69516819779692));
#28539=CARTESIAN_POINT('',(4.84757646506369,1.30000000000001,7.35330497500277));
#28540=CARTESIAN_POINT('Ctrl Pts',(4.57248821462698,1.3,7.4651569071776));
#28541=CARTESIAN_POINT('Ctrl Pts',(4.5798565885141,1.3,7.46043462253162));
#28542=CARTESIAN_POINT('Ctrl Pts',(4.59168078261245,1.3,7.45714429554202));
#28543=CARTESIAN_POINT('Ctrl Pts',(4.60901113594043,1.3,7.45220225290281));
#28544=CARTESIAN_POINT('Ctrl Pts',(4.62333650359118,1.3,7.44778282836643));
#28545=CARTESIAN_POINT('Ctrl Pts',(4.63777227980167,1.3,7.44313876891633));
#28546=CARTESIAN_POINT('Ctrl Pts',(4.65200864708552,1.3,7.4371009858883));
#28547=CARTESIAN_POINT('Ctrl Pts',(4.67500366927394,1.3,7.42951895371871));
#28548=CARTESIAN_POINT('Ctrl Pts',(4.70065028211382,1.3,7.41931266872196));
#28549=CARTESIAN_POINT('Ctrl Pts',(4.72626264033617,1.30000000000001,7.40855923000075));
#28550=CARTESIAN_POINT('Ctrl Pts',(4.74336478500948,1.30000000000001,7.40185875322679));
#28551=CARTESIAN_POINT('Ctrl Pts',(4.75753064369248,1.30000000000001,7.39545690322073));
#28552=CARTESIAN_POINT('Ctrl Pts',(4.76745636601093,1.3,7.39112846433222));
#28553=CARTESIAN_POINT('Ctrl Pts',(4.77311161413793,1.30000000000001,7.38850648431319));
#28554=CARTESIAN_POINT('Ctrl Pts',(4.78158028238953,1.3,7.38446389233093));
#28555=CARTESIAN_POINT('Ctrl Pts',(4.79431947529819,1.30000000000002,7.37881277574729));
#28556=CARTESIAN_POINT('Ctrl Pts',(4.81695502355809,1.3,7.36871994814812));
#28557=CARTESIAN_POINT('Ctrl Pts',(4.8346427283241,1.30000000000002,7.35972960775616));
#28558=CARTESIAN_POINT('Ctrl Pts',(4.84672489359485,1.30000000000002,7.35372750798776));
#28559=CARTESIAN_POINT('Ctrl Pts',(4.84757646497524,1.30000000000002,7.35330497504666));
#28560=CARTESIAN_POINT('',(4.83514813889957,1.30000000000181,6.82074434979023));
#28561=CARTESIAN_POINT('Origin',(0.,1.3,7.2));
#28562=CARTESIAN_POINT('',(4.55678639209675,1.3,6.73765570212511));
#28563=CARTESIAN_POINT('Ctrl Pts',(4.83514655110529,1.30000000000047,6.82074421646102));
#28564=CARTESIAN_POINT('Ctrl Pts',(4.83418984233378,1.30000000000046,6.82039257937535));
#28565=CARTESIAN_POINT('Ctrl Pts',(4.8275141099345,1.30000000000046,6.8179659614836));
#28566=CARTESIAN_POINT('Ctrl Pts',(4.81795999365544,1.30000000000042,6.81478799676167));
#28567=CARTESIAN_POINT('Ctrl Pts',(4.80653088510641,1.30000000000041,6.81028270647152));
#28568=CARTESIAN_POINT('Ctrl Pts',(4.78936219347766,1.30000000000041,6.80389947355039));
#28569=CARTESIAN_POINT('Ctrl Pts',(4.75783769436201,1.30000000000029,6.79269374504301));
#28570=CARTESIAN_POINT('Ctrl Pts',(4.72334918205181,1.30000000000017,6.78192834281718));
#28571=CARTESIAN_POINT('Ctrl Pts',(4.68878647838757,1.30000000000016,6.77165051357849));
#28572=CARTESIAN_POINT('Ctrl Pts',(4.66573214590264,1.30000000000009,6.76556506981444));
#28573=CARTESIAN_POINT('Ctrl Pts',(4.64264412228767,1.30000000000009,6.75875338894064));
#28574=CARTESIAN_POINT('Ctrl Pts',(4.62535152074713,1.30000000000006,6.7547381568986));
#28575=CARTESIAN_POINT('Ctrl Pts',(4.60795448968299,1.30000000000004,6.75071584500925));
#28576=CARTESIAN_POINT('Ctrl Pts',(4.59357902902068,1.30000000000003,6.74737894430936));
#28577=CARTESIAN_POINT('Ctrl Pts',(4.576180400044,1.30000000000001,6.74411411083726));
#28578=CARTESIAN_POINT('Ctrl Pts',(4.56433455845385,1.3,6.74178132772091));
#28579=CARTESIAN_POINT('Ctrl Pts',(4.55678639209675,1.3,6.73765570212512));
#28580=CARTESIAN_POINT('',(4.52769759742429,1.3,6.50868883662639));
#28581=CARTESIAN_POINT('',(4.55678639209675,1.3,6.73765570212511));
#28582=CARTESIAN_POINT('',(4.77352764767188,1.30000000000002,6.34213416147271));
#28583=CARTESIAN_POINT('Ctrl Pts',(4.52769759742429,1.3,6.50868883662639));
#28584=CARTESIAN_POINT('Ctrl Pts',(4.53392313647801,1.3,6.50253777415649));
#28585=CARTESIAN_POINT('Ctrl Pts',(4.54481208542156,1.3,6.49688052366386));
#28586=CARTESIAN_POINT('Ctrl Pts',(4.56070008160091,1.3,6.488336502504));
#28587=CARTESIAN_POINT('Ctrl Pts',(4.57389579341099,1.3,6.48133398930416));
#28588=CARTESIAN_POINT('Ctrl Pts',(4.59203923906489,1.30000000000002,6.46996823620903));
#28589=CARTESIAN_POINT('Ctrl Pts',(4.61789381187435,1.3,6.45392159180597));
#28590=CARTESIAN_POINT('Ctrl Pts',(4.64368961597031,1.30000000000002,6.43767322775346));
#28591=CARTESIAN_POINT('Ctrl Pts',(4.66641984978595,1.30000000000002,6.42158632818792));
#28592=CARTESIAN_POINT('Ctrl Pts',(4.68178015411769,1.30000000000002,6.41154489129323));
#28593=CARTESIAN_POINT('Ctrl Pts',(4.69428702464384,1.30000000000003,6.40228578094019));
#28594=CARTESIAN_POINT('Ctrl Pts',(4.70437021285367,1.30000000000003,6.39513336563024));
#28595=CARTESIAN_POINT('Ctrl Pts',(4.71922603638813,1.30000000000003,6.38361239688257));
#28596=CARTESIAN_POINT('Ctrl Pts',(4.74196049006546,1.30000000000003,6.36773979185516));
#28597=CARTESIAN_POINT('Ctrl Pts',(4.76217237674818,1.30000000000005,6.35099061182857));
#28598=CARTESIAN_POINT('Ctrl Pts',(4.77278114106614,1.30000000000005,6.34271479237717));
#28599=CARTESIAN_POINT('Ctrl Pts',(4.77352764741212,1.30000000000005,6.34213416167476));
#28600=CARTESIAN_POINT('',(4.65067750872513,1.30000000000116,5.82388274136382));
#28601=CARTESIAN_POINT('Origin',(0.,1.3,7.2));
#28602=CARTESIAN_POINT('',(4.36108289177478,1.3,5.80034987084453));
#28603=CARTESIAN_POINT('Ctrl Pts',(4.65067750872023,1.3,5.8238827413956));
#28604=CARTESIAN_POINT('Ctrl Pts',(4.57567439558732,1.3,5.8123200324086));
#28605=CARTESIAN_POINT('Ctrl Pts',(4.49988238082424,1.3,5.80395796558544));
#28606=CARTESIAN_POINT('Ctrl Pts',(4.40454586996321,1.3,5.80228572656157));
#28607=CARTESIAN_POINT('Ctrl Pts',(4.40191545967668,1.3,5.80217462217108));
#28608=CARTESIAN_POINT('Ctrl Pts',(4.38054048224239,1.3,5.80258762524379));
#28609=CARTESIAN_POINT('Ctrl Pts',(4.3703146143467,1.3,5.80311246775222));
#28610=CARTESIAN_POINT('Ctrl Pts',(4.36108289177478,1.3,5.80034987084453));
#28611=CARTESIAN_POINT('',(4.28502486891058,1.3,5.58243438119362));
#28612=CARTESIAN_POINT('',(4.36108289177478,1.3,5.80034987084453));
#28613=CARTESIAN_POINT('',(4.49080284932952,1.30000000000011,5.368282290184));
#28614=CARTESIAN_POINT('Ctrl Pts',(4.28502486891058,1.3,5.58243438119362));
#28615=CARTESIAN_POINT('Ctrl Pts',(4.2898354872008,1.3,5.57512337184582));
#28616=CARTESIAN_POINT('Ctrl Pts',(4.29931642282797,1.30000000000001,5.56733888639131));
#28617=CARTESIAN_POINT('Ctrl Pts',(4.3130840388909,1.30000000000001,5.55568404800534));
#28618=CARTESIAN_POINT('Ctrl Pts',(4.32453875212957,1.30000000000003,5.54609803841767));
#28619=CARTESIAN_POINT('Ctrl Pts',(4.33993231883246,1.30000000000003,5.53122457501866));
#28620=CARTESIAN_POINT('Ctrl Pts',(4.36189159450452,1.30000000000003,5.51016616730234));
#28621=CARTESIAN_POINT('Ctrl Pts',(4.38377554191331,1.30000000000007,5.48895426241472));
#28622=CARTESIAN_POINT('Ctrl Pts',(4.40271175336488,1.3000000000001,5.46857812868943));
#28623=CARTESIAN_POINT('Ctrl Pts',(4.41990733032772,1.3000000000001,5.45112073570275));
#28624=CARTESIAN_POINT('Ctrl Pts',(4.44025594115488,1.30000000000016,5.4273732287603));
#28625=CARTESIAN_POINT('Ctrl Pts',(4.46512770529739,1.3000000000002,5.39974222775974));
#28626=CARTESIAN_POINT('Ctrl Pts',(4.48173090221287,1.30000000000024,5.37965091509962));
#28627=CARTESIAN_POINT('Ctrl Pts',(4.49020148419593,1.30000000000025,5.36903242764666));
#28628=CARTESIAN_POINT('Ctrl Pts',(4.49080284925142,1.30000000000025,5.36828229028143));
#28629=CARTESIAN_POINT('',(4.26287719558135,1.3000000000006,4.88691158511914));
#28630=CARTESIAN_POINT('Origin',(0.,1.3,7.2));
#28631=CARTESIAN_POINT('',(3.97477914228473,1.3,4.92421546647452));
#28632=CARTESIAN_POINT('Ctrl Pts',(4.26287719558322,1.3,4.88691158515324));
#28633=CARTESIAN_POINT('Ctrl Pts',(4.16750758322341,1.3,4.89212562971692));
#28634=CARTESIAN_POINT('Ctrl Pts',(4.09236051848986,1.3,4.90259779459969));
#28635=CARTESIAN_POINT('Ctrl Pts',(3.98404709074897,1.3,4.92363634735652));
#28636=CARTESIAN_POINT('Ctrl Pts',(3.98077132219638,1.3,4.92470388458002));
#28637=CARTESIAN_POINT('Ctrl Pts',(3.97477914228474,1.3,4.92421546647452));
#28638=CARTESIAN_POINT('',(3.85507599179487,1.3,4.7268753052437));
#28639=CARTESIAN_POINT('',(3.97477914228474,1.3,4.92421546647452));
#28640=CARTESIAN_POINT('',(4.01191463394249,1.3,4.47474020138297));
#28641=CARTESIAN_POINT('Ctrl Pts',(3.85507599179487,1.3,4.7268753052437));
#28642=CARTESIAN_POINT('Ctrl Pts',(3.85826144221842,1.3,4.7187238752086));
#28643=CARTESIAN_POINT('Ctrl Pts',(3.86591529009691,1.3,4.70913672804832));
#28644=CARTESIAN_POINT('Ctrl Pts',(3.87702448920013,1.3,4.69494766196105));
#28645=CARTESIAN_POINT('Ctrl Pts',(3.88606867189398,1.3,4.68300308818325));
#28646=CARTESIAN_POINT('Ctrl Pts',(3.89672887394469,1.3,4.66824246157762));
#28647=CARTESIAN_POINT('Ctrl Pts',(3.90461453552397,1.3,4.65489605906055));
#28648=CARTESIAN_POINT('Ctrl Pts',(3.91888415578993,1.3,4.63540334932576));
#28649=CARTESIAN_POINT('Ctrl Pts',(3.93483759407892,1.3,4.60896349398333));
#28650=CARTESIAN_POINT('Ctrl Pts',(3.9561473127133,1.3,4.57524814942806));
#28651=CARTESIAN_POINT('Ctrl Pts',(3.97147745303166,1.30000000000001,4.54819353159721));
#28652=CARTESIAN_POINT('Ctrl Pts',(3.98359299015971,1.30000000000001,4.52641657168413));
#28653=CARTESIAN_POINT('Ctrl Pts',(3.99308905203255,1.3,4.51055005634327));
#28654=CARTESIAN_POINT('Ctrl Pts',(4.00172238876483,1.3,4.49374975302448));
#28655=CARTESIAN_POINT('Ctrl Pts',(4.00805516521168,1.30000000000001,4.48189586303462));
#28656=CARTESIAN_POINT('Ctrl Pts',(4.01146644254775,1.3,4.47557094656382));
#28657=CARTESIAN_POINT('Ctrl Pts',(4.01191463393987,1.3,4.47474020138783));
#28658=CARTESIAN_POINT('',(3.68882920336369,1.30000000000049,4.05118449127588));
#28659=CARTESIAN_POINT('Origin',(0.,1.3,7.2));
#28660=CARTESIAN_POINT('',(3.4147584711704,1.3,4.14754376664537));
#28661=CARTESIAN_POINT('Ctrl Pts',(3.68882920337514,1.3,4.05118449131822));
#28662=CARTESIAN_POINT('Ctrl Pts',(3.65850555103085,1.3,4.05938588383362));
#28663=CARTESIAN_POINT('Ctrl Pts',(3.55713888853847,1.3,4.08790905610615));
#28664=CARTESIAN_POINT('Ctrl Pts',(3.43637430894292,1.3,4.13982506353119));
#28665=CARTESIAN_POINT('Ctrl Pts',(3.42618793094316,1.3,4.1460714746367));
#28666=CARTESIAN_POINT('Ctrl Pts',(3.4147584711704,1.3,4.14754376664537));
#28667=CARTESIAN_POINT('',(3.25664179513071,1.3,3.97940364582358));
#28668=CARTESIAN_POINT('',(3.4147584711704,1.3,4.14754376664537));
#28669=CARTESIAN_POINT('',(3.35740649851691,1.30000000000134,3.69995637892978));
#28670=CARTESIAN_POINT('Ctrl Pts',(3.25664179513071,1.3,3.97940364582358));
#28671=CARTESIAN_POINT('Ctrl Pts',(3.25806285821859,1.3,3.9707680517086));
#28672=CARTESIAN_POINT('Ctrl Pts',(3.26349509695928,1.3,3.95978804109145));
#28673=CARTESIAN_POINT('Ctrl Pts',(3.2702247202651,1.3,3.94633814773344));
#28674=CARTESIAN_POINT('Ctrl Pts',(3.27389249918462,1.3,3.93815813999823));
#28675=CARTESIAN_POINT('Ctrl Pts',(3.27911491145038,1.3,3.92730408899227));
#28676=CARTESIAN_POINT('Ctrl Pts',(3.28506288912775,1.3,3.91334417124239));
#28677=CARTESIAN_POINT('Ctrl Pts',(3.29127623046883,1.3,3.8959033209131));
#28678=CARTESIAN_POINT('Ctrl Pts',(3.30120174405925,1.30000000000002,3.87389948305366));
#28679=CARTESIAN_POINT('Ctrl Pts',(3.31308542169651,1.3,3.83865271317822));
#28680=CARTESIAN_POINT('Ctrl Pts',(3.32618522651639,1.30000000000001,3.80439139269443));
#28681=CARTESIAN_POINT('Ctrl Pts',(3.33701682672449,1.30000000000001,3.76851394130066));
#28682=CARTESIAN_POINT('Ctrl Pts',(3.34674839854031,1.30000000000003,3.73916815385308));
#28683=CARTESIAN_POINT('Ctrl Pts',(3.3533947067203,1.30000000000002,3.71491322535318));
#28684=CARTESIAN_POINT('Ctrl Pts',(3.3569075990033,1.30000000000002,3.70182795548531));
#28685=CARTESIAN_POINT('Ctrl Pts',(3.3571574986747,1.30000000000002,3.70089472823323));
#28686=CARTESIAN_POINT('Ctrl Pts',(3.35740469928613,1.30000000000002,3.69995929704989));
#28687=CARTESIAN_POINT('',(2.95357407114036,1.30000000000001,3.35306612923546));
#28688=CARTESIAN_POINT('Origin',(0.,1.3,7.2));
#28689=CARTESIAN_POINT('',(2.70549646903679,1.3,3.50427905152391));
#28690=CARTESIAN_POINT('Ctrl Pts',(2.95357407115217,1.3,3.35306612925858));
#28691=CARTESIAN_POINT('Ctrl Pts',(2.88599776229586,1.3,3.38758551557036));
#28692=CARTESIAN_POINT('Ctrl Pts',(2.8198851485551,1.3,3.42559236828672));
#28693=CARTESIAN_POINT('Ctrl Pts',(2.71359164015416,1.3,3.50008522613048));
#28694=CARTESIAN_POINT('Ctrl Pts',(2.71105385687628,1.3,3.50232850732212));
#28695=CARTESIAN_POINT('Ctrl Pts',(2.7054964690368,1.3,3.50427905152391));
#28696=CARTESIAN_POINT('',(2.5158767249182,1.3,3.37268750121688));
#28697=CARTESIAN_POINT('',(2.70549646903679,1.3,3.50427905152391));
#28698=CARTESIAN_POINT('',(2.55661739137892,1.29999999999997,3.0785672983659));
#28699=CARTESIAN_POINT('Ctrl Pts',(2.5158767249182,1.3,3.37268750121688));
#28700=CARTESIAN_POINT('Ctrl Pts',(2.51547129339445,1.3,3.36394515992304));
#28701=CARTESIAN_POINT('Ctrl Pts',(2.51855424420958,1.3,3.35207075092507));
#28702=CARTESIAN_POINT('Ctrl Pts',(2.52283590576821,1.3,3.33454697355417));
#28703=CARTESIAN_POINT('Ctrl Pts',(2.52646568091669,1.29999999999998,3.32005827780177));
#28704=CARTESIAN_POINT('Ctrl Pts',(2.53015462701597,1.3,3.29896774216744));
#28705=CARTESIAN_POINT('Ctrl Pts',(2.53556382481435,1.29999999999996,3.26903445978772));
#28706=CARTESIAN_POINT('Ctrl Pts',(2.54069414220718,1.29999999999997,3.23896280698673));
#28707=CARTESIAN_POINT('Ctrl Pts',(2.54562846964274,1.29999999999995,3.19912449820451));
#28708=CARTESIAN_POINT('Ctrl Pts',(2.5491865482161,1.29999999999994,3.17163804176601));
#28709=CARTESIAN_POINT('Ctrl Pts',(2.55097589650377,1.29999999999994,3.14662539106063));
#28710=CARTESIAN_POINT('Ctrl Pts',(2.55239378124017,1.29999999999994,3.13435370671797));
#28711=CARTESIAN_POINT('Ctrl Pts',(2.55405997194999,1.29999999999994,3.11897444393603));
#28712=CARTESIAN_POINT('Ctrl Pts',(2.55513657431493,1.29999999999992,3.1001254150743));
#28713=CARTESIAN_POINT('Ctrl Pts',(2.55602160759642,1.29999999999992,3.08668496437601));
#28714=CARTESIAN_POINT('Ctrl Pts',(2.55654773472364,1.29999999999992,3.07951048822781));
#28715=CARTESIAN_POINT('Ctrl Pts',(2.55661739137288,1.29999999999992,3.0785672984477));
#28716=CARTESIAN_POINT('',(2.08911835436551,1.30000000000047,2.82300508328796));
#28717=CARTESIAN_POINT('Origin',(0.,1.3,7.2));
#28718=CARTESIAN_POINT('',(1.87799128879385,1.3,3.02253507588753));
#28719=CARTESIAN_POINT('Ctrl Pts',(2.08911835439991,1.3,2.82300508332989));
#28720=CARTESIAN_POINT('Ctrl Pts',(2.03046284013333,1.3,2.87112862669476));
#28721=CARTESIAN_POINT('Ctrl Pts',(1.97359865399671,1.3,2.92188244262196));
#28722=CARTESIAN_POINT('Ctrl Pts',(1.88576178563236,1.3,3.01598267558689));
#28723=CARTESIAN_POINT('Ctrl Pts',(1.8835507587602,1.3,3.01914952488677));
#28724=CARTESIAN_POINT('Ctrl Pts',(1.87799128879385,1.3,3.02253507588753));
#28725=CARTESIAN_POINT('',(1.66515576931082,1.3,2.93324327828999));
#28726=CARTESIAN_POINT('',(1.87799128879385,1.3,3.02253507588753));
#28727=CARTESIAN_POINT('',(1.64381178161171,1.3,2.63706423159009));
#28728=CARTESIAN_POINT('Ctrl Pts',(1.66515576931082,1.3,2.93324327829));
#28729=CARTESIAN_POINT('Ctrl Pts',(1.66294156247849,1.3,2.92477627208227));
#28730=CARTESIAN_POINT('Ctrl Pts',(1.66351030995394,1.3,2.9125249551468));
#28731=CARTESIAN_POINT('Ctrl Pts',(1.66412261980249,1.3,2.89450855944385));
#28732=CARTESIAN_POINT('Ctrl Pts',(1.66452629020269,1.3,2.87955334577841));
#28733=CARTESIAN_POINT('Ctrl Pts',(1.66423539774643,1.3,2.86129400510938));
#28734=CARTESIAN_POINT('Ctrl Pts',(1.66273115025757,1.3,2.83678667555902));
#28735=CARTESIAN_POINT('Ctrl Pts',(1.6626944242077,1.3,2.81260856801406));
#28736=CARTESIAN_POINT('Ctrl Pts',(1.6605733140711,1.3,2.79100115316553));
#28737=CARTESIAN_POINT('Ctrl Pts',(1.65871139278267,1.3,2.76644084839449));
#28738=CARTESIAN_POINT('Ctrl Pts',(1.65715322685088,1.3,2.74196829601108));
#28739=CARTESIAN_POINT('Ctrl Pts',(1.65352500342455,1.3,2.71406419108784));
#28740=CARTESIAN_POINT('Ctrl Pts',(1.6504187223115,1.3,2.68327445254122));
#28741=CARTESIAN_POINT('Ctrl Pts',(1.64675072801477,1.3,2.65752408921042));
#28742=CARTESIAN_POINT('Ctrl Pts',(1.64394619751435,1.3,2.63799905453949));
#28743=CARTESIAN_POINT('Ctrl Pts',(1.64381178161338,1.3,2.63706423160175));
#28744=CARTESIAN_POINT('',(1.13357773497359,1.30000000000006,2.48433445646712));
#28745=CARTESIAN_POINT('Origin',(0.,1.3,7.2));
#28746=CARTESIAN_POINT('',(0.968408877628583,1.3,2.72336636313561));
#28747=CARTESIAN_POINT('Ctrl Pts',(1.13357773499831,1.3,2.4843344564871));
#28748=CARTESIAN_POINT('Ctrl Pts',(1.13293652139485,1.3,2.48512733677124));
#28749=CARTESIAN_POINT('Ctrl Pts',(1.1322867097125,1.3,2.48593132009101));
#28750=CARTESIAN_POINT('Ctrl Pts',(1.13162887637119,1.3,2.48674634991899));
#28751=CARTESIAN_POINT('Ctrl Pts',(1.12479465001758,1.3,2.49521368956197));
#28752=CARTESIAN_POINT('Ctrl Pts',(1.11708786724918,1.3,2.5048693306749));
#28753=CARTESIAN_POINT('Ctrl Pts',(1.10893902398972,1.3,2.51546374956644));
#28754=CARTESIAN_POINT('Ctrl Pts',(1.10193451489362,1.3,2.52457040447816));
#28755=CARTESIAN_POINT('Ctrl Pts',(1.09462362918233,1.3,2.53438290697181));
#28756=CARTESIAN_POINT('Ctrl Pts',(1.08693530229986,1.3,2.54448550662487));
#28757=CARTESIAN_POINT('Ctrl Pts',(1.07978720725581,1.3,2.55387823193637));
#28758=CARTESIAN_POINT('Ctrl Pts',(1.07228148729113,1.3,2.56350592466692));
#28759=CARTESIAN_POINT('Ctrl Pts',(1.06521521123111,1.3,2.57365000947087));
#28760=CARTESIAN_POINT('Ctrl Pts',(1.06180540316093,1.3,2.57854500393971));
#28761=CARTESIAN_POINT('Ctrl Pts',(1.05850493335534,1.3,2.58356304708329));
#28762=CARTESIAN_POINT('Ctrl Pts',(1.05512786151265,1.3,2.5885393160823));
#28763=CARTESIAN_POINT('Ctrl Pts',(1.0517557761572,1.3,2.5935082372655));
#28764=CARTESIAN_POINT('Ctrl Pts',(1.04830595503031,1.3,2.59843593972442));
#28765=CARTESIAN_POINT('Ctrl Pts',(1.04490139855508,1.3,2.6033778059502));
#28766=CARTESIAN_POINT('Ctrl Pts',(1.0345032720822,1.3,2.61847115229406));
#28767=CARTESIAN_POINT('Ctrl Pts',(1.02453521099312,1.3,2.63369301355648));
#28768=CARTESIAN_POINT('Ctrl Pts',(1.01523157341463,1.3,2.648306025813));
#28769=CARTESIAN_POINT('Ctrl Pts',(1.01197415980419,1.3,2.65342237139422));
#28770=CARTESIAN_POINT('Ctrl Pts',(1.0087985257201,1.3,2.65846528371442));
#28771=CARTESIAN_POINT('Ctrl Pts',(1.00576925730934,1.3,2.66343712573536));
#28772=CARTESIAN_POINT('Ctrl Pts',(1.00250701753485,1.3,2.66879133625551));
#28773=CARTESIAN_POINT('Ctrl Pts',(0.99938314075874,1.3,2.67410046903923));
#28774=CARTESIAN_POINT('Ctrl Pts',(0.996624580065918,1.3,2.67871368637101));
#28775=CARTESIAN_POINT('Ctrl Pts',(0.993116511760298,1.3,2.68458032601054));
#28776=CARTESIAN_POINT('Ctrl Pts',(0.990100803084034,1.3,2.68958524992309));
#28777=CARTESIAN_POINT('Ctrl Pts',(0.987617586884602,1.3,2.6939842956337));
#28778=CARTESIAN_POINT('Ctrl Pts',(0.986011479870618,1.3,2.69682953245692));
#28779=CARTESIAN_POINT('Ctrl Pts',(0.984612560913104,1.3,2.69941205955226));
#28780=CARTESIAN_POINT('Ctrl Pts',(0.983335702194529,1.3,2.70174695396398));
#28781=CARTESIAN_POINT('Ctrl Pts',(0.976916590415545,1.3,2.713485095391));
#28782=CARTESIAN_POINT('Ctrl Pts',(0.973272619642238,1.3,2.7187765629255));
#28783=CARTESIAN_POINT('Ctrl Pts',(0.968408877628585,1.3,2.72336636313561));
#28784=CARTESIAN_POINT('',(0.74165951628067,1.3,2.68027679827216));
#28785=CARTESIAN_POINT('',(0.968408877628583,1.3,2.72336636313561));
#28786=CARTESIAN_POINT('',(0.659051978146154,1.3,2.39498694173454));
#28787=CARTESIAN_POINT('Ctrl Pts',(0.74165951628067,1.3,2.68027679827216));
#28788=CARTESIAN_POINT('Ctrl Pts',(0.737733305603287,1.3,2.67245517595099));
#28789=CARTESIAN_POINT('Ctrl Pts',(0.735713875635836,1.3,2.66035957958182));
#28790=CARTESIAN_POINT('Ctrl Pts',(0.732597760872633,1.3,2.64260793958377));
#28791=CARTESIAN_POINT('Ctrl Pts',(0.729765699114481,1.3,2.62790692781172));
#28792=CARTESIAN_POINT('Ctrl Pts',(0.726557820517931,1.3,2.61305934494932));
#28793=CARTESIAN_POINT('Ctrl Pts',(0.723151878203878,1.3,2.60124260806693));
#28794=CARTESIAN_POINT('Ctrl Pts',(0.720709138865025,1.3,2.59235073662494));
#28795=CARTESIAN_POINT('Ctrl Pts',(0.71634712092609,1.3,2.57167599474918));
#28796=CARTESIAN_POINT('Ctrl Pts',(0.707491994511335,1.3,2.54210786089461));
#28797=CARTESIAN_POINT('Ctrl Pts',(0.69816516774291,1.3,2.50962744616599));
#28798=CARTESIAN_POINT('Ctrl Pts',(0.690779760699569,1.3,2.48601858192387));
#28799=CARTESIAN_POINT('Ctrl Pts',(0.684623565179564,1.3,2.46832269985239));
#28800=CARTESIAN_POINT('Ctrl Pts',(0.676935095157866,1.3,2.44474912633269));
#28801=CARTESIAN_POINT('Ctrl Pts',(0.669050883568352,1.3,2.42118640333502));
#28802=CARTESIAN_POINT('Ctrl Pts',(0.661798923496942,1.30000000000001,2.40266552561176));
#28803=CARTESIAN_POINT('Ctrl Pts',(0.659371426705916,1.30000000000001,2.39588686093049));
#28804=CARTESIAN_POINT('Ctrl Pts',(0.659051978154449,1.30000000000001,2.39498694175791));
#28805=CARTESIAN_POINT('',(0.128170675781554,1.30000000000107,2.35169387542681));
#28806=CARTESIAN_POINT('Origin',(0.,1.3,7.2));
#28807=CARTESIAN_POINT('',(0.0165023515695843,1.3,2.61984802158616));
#28808=CARTESIAN_POINT('Ctrl Pts',(0.128170675807936,1.3,2.35169387544013));
#28809=CARTESIAN_POINT('Ctrl Pts',(0.10619951312427,1.3,2.39523277512288));
#28810=CARTESIAN_POINT('Ctrl Pts',(0.0854073494869826,1.29999999999995,
2.43946186308817));
#28811=CARTESIAN_POINT('Ctrl Pts',(0.0585207374510833,1.29999999999995,
2.50734591272452));
#28812=CARTESIAN_POINT('Ctrl Pts',(0.0487206764552959,1.29999999999993,
2.52957674635612));
#28813=CARTESIAN_POINT('Ctrl Pts',(0.0354428122597672,1.29999999999993,
2.56889180573038));
#28814=CARTESIAN_POINT('Ctrl Pts',(0.0324836161788516,1.29999999999993,
2.5767603968036));
#28815=CARTESIAN_POINT('Ctrl Pts',(0.0251452812246871,1.29999999999993,
2.60004278591798));
#28816=CARTESIAN_POINT('Ctrl Pts',(0.022543073780594,1.3,2.61111103088363));
#28817=CARTESIAN_POINT('Ctrl Pts',(0.0165023515695844,1.3,2.61984802158616));
#28818=CARTESIAN_POINT('',(-0.214250816488161,1.3,2.624843910208));
#28819=CARTESIAN_POINT('',(0.0165023515695843,1.3,2.61984802158616));
#28820=CARTESIAN_POINT('',(-0.354392897366409,1.3,2.36296519815122));
#28821=CARTESIAN_POINT('Ctrl Pts',(-0.21425081648816,1.3,2.624843910208));
#28822=CARTESIAN_POINT('Ctrl Pts',(-0.219717436763953,1.3,2.61800951420116));
#28823=CARTESIAN_POINT('Ctrl Pts',(-0.224209275765746,1.3,2.606595622045));
#28824=CARTESIAN_POINT('Ctrl Pts',(-0.231052456917044,1.3,2.58990382504299));
#28825=CARTESIAN_POINT('Ctrl Pts',(-0.236623358264727,1.3,2.57604856509846));
#28826=CARTESIAN_POINT('Ctrl Pts',(-0.2460751938082,1.3,2.55682624237417));
#28827=CARTESIAN_POINT('Ctrl Pts',(-0.259183769683128,1.3,2.52940909662549));
#28828=CARTESIAN_POINT('Ctrl Pts',(-0.274355810881998,1.3,2.49938890693942));
#28829=CARTESIAN_POINT('Ctrl Pts',(-0.290586106563452,1.3,2.46962310770296));
#28830=CARTESIAN_POINT('Ctrl Pts',(-0.302397069786213,1.29999999999999,
2.44799378564757));
#28831=CARTESIAN_POINT('Ctrl Pts',(-0.323310367858908,1.3,2.41324546052299));
#28832=CARTESIAN_POINT('Ctrl Pts',(-0.33939401831521,1.3,2.38564120596506));
#28833=CARTESIAN_POINT('Ctrl Pts',(-0.353861208044329,1.3,2.36377256592943));
#28834=CARTESIAN_POINT('Ctrl Pts',(-0.354392897361749,1.3,2.3629651981583));
#28835=CARTESIAN_POINT('',(-0.882736269392908,1.3,2.43100884057243));
#28836=CARTESIAN_POINT('Origin',(0.,1.3,7.2));
#28837=CARTESIAN_POINT('',(-0.936125406440072,1.3,2.71650429950101));
#28838=CARTESIAN_POINT('Ctrl Pts',(-0.882736269392908,1.3,2.43100884057243));
#28839=CARTESIAN_POINT('Ctrl Pts',(-0.890585516016561,1.3,2.46173198670934));
#28840=CARTESIAN_POINT('Ctrl Pts',(-0.914120009049791,1.29999999996271,
2.56513894027015));
#28841=CARTESIAN_POINT('Ctrl Pts',(-0.931163753333676,1.29999999996271,
2.67599020345154));
#28842=CARTESIAN_POINT('Ctrl Pts',(-0.929449820781408,1.3,2.70051432210213));
#28843=CARTESIAN_POINT('Ctrl Pts',(-0.936125406440074,1.3,2.716504299501));
#28844=CARTESIAN_POINT('',(-1.16079736048697,1.3,2.76936729730244));
#28845=CARTESIAN_POINT('',(-0.936125406440072,1.3,2.71650429950101));
#28846=CARTESIAN_POINT('',(-1.3523957842154,1.30000000000138,2.54237068259109));
#28847=CARTESIAN_POINT('Ctrl Pts',(-1.16079736048697,1.3,2.76936729730244));
#28848=CARTESIAN_POINT('Ctrl Pts',(-1.16756547282336,1.3,2.76381882351047));
#28849=CARTESIAN_POINT('Ctrl Pts',(-1.17429793045071,1.3,2.75357283179475));
#28850=CARTESIAN_POINT('Ctrl Pts',(-1.18440354486965,1.3,2.7386418212914));
#28851=CARTESIAN_POINT('Ctrl Pts',(-1.19282120230342,1.3,2.72628912988518));
#28852=CARTESIAN_POINT('Ctrl Pts',(-1.20387759611253,1.3,2.71172137984579));
#28853=CARTESIAN_POINT('Ctrl Pts',(-1.22296240651216,1.3,2.68787374759291));
#28854=CARTESIAN_POINT('Ctrl Pts',(-1.24183231204913,1.3,2.66390421538196));
#28855=CARTESIAN_POINT('Ctrl Pts',(-1.26206094764912,1.30000000000001,2.64057600636631));
#28856=CARTESIAN_POINT('Ctrl Pts',(-1.27762376107936,1.30000000000001,2.62164883825251));
#28857=CARTESIAN_POINT('Ctrl Pts',(-1.29899075380456,1.29999999999999,2.59887488144818));
#28858=CARTESIAN_POINT('Ctrl Pts',(-1.32381937982074,1.3,2.57122791399148));
#28859=CARTESIAN_POINT('Ctrl Pts',(-1.34203682692771,1.30000000000001,2.55259610655428));
#28860=CARTESIAN_POINT('Ctrl Pts',(-1.35170736374796,1.30000000000001,2.5430533015253));
#28861=CARTESIAN_POINT('Ctrl Pts',(-1.3523945461556,1.30000000000001,2.54237191022484));
#28862=CARTESIAN_POINT('',(-1.85490568625463,1.30000000000046,2.7187250815555));
#28863=CARTESIAN_POINT('Origin',(0.,1.3,7.2));
#28864=CARTESIAN_POINT('',(-1.84783999216021,1.3,3.00911085372699));
#28865=CARTESIAN_POINT('Ctrl Pts',(-1.85490568621173,1.3,2.71872508155732));
#28866=CARTESIAN_POINT('Ctrl Pts',(-1.85494906266401,1.3,2.71974586259111));
#28867=CARTESIAN_POINT('Ctrl Pts',(-1.85498765318356,1.3,2.7207652106144));
#28868=CARTESIAN_POINT('Ctrl Pts',(-1.85502062869155,1.3,2.72178310517736));
#28869=CARTESIAN_POINT('Ctrl Pts',(-1.85521915454548,1.3,2.72791124086604));
#28870=CARTESIAN_POINT('Ctrl Pts',(-1.85521812104922,1.3,2.73398519666606));
#28871=CARTESIAN_POINT('Ctrl Pts',(-1.85546360136794,1.3,2.73998240712142));
#28872=CARTESIAN_POINT('Ctrl Pts',(-1.85571689038058,1.3,2.74617038798602));
#28873=CARTESIAN_POINT('Ctrl Pts',(-1.85621651005613,1.3,2.75228028849141));
#28874=CARTESIAN_POINT('Ctrl Pts',(-1.85637531506373,1.3,2.75831933810552));
#28875=CARTESIAN_POINT('Ctrl Pts',(-1.85653649953747,1.3,2.76444887424915));
#28876=CARTESIAN_POINT('Ctrl Pts',(-1.85635497434812,1.3,2.77050160335946));
#28877=CARTESIAN_POINT('Ctrl Pts',(-1.85649256135086,1.3,2.77645639068877));
#28878=CARTESIAN_POINT('Ctrl Pts',(-1.85663595615561,1.3,2.7826625406115));
#28879=CARTESIAN_POINT('Ctrl Pts',(-1.85709812605095,1.3,2.7887665601669));
#28880=CARTESIAN_POINT('Ctrl Pts',(-1.85723117976892,1.3,2.79476573133978));
#28881=CARTESIAN_POINT('Ctrl Pts',(-1.85736766436802,1.3,2.80091959524531));
#28882=CARTESIAN_POINT('Ctrl Pts',(-1.85717181951977,1.3,2.80695968052047));
#28883=CARTESIAN_POINT('Ctrl Pts',(-1.85717055652404,1.3,2.81287274002393));
#28884=CARTESIAN_POINT('Ctrl Pts',(-1.85716923144163,1.3,2.8190764753326));
#28885=CARTESIAN_POINT('Ctrl Pts',(-1.85736110288761,1.3,2.82514297239297));
#28886=CARTESIAN_POINT('Ctrl Pts',(-1.85737655537845,1.3,2.83105817463949));
#28887=CARTESIAN_POINT('Ctrl Pts',(-1.85740983197251,1.3,2.84379643062085));
#28888=CARTESIAN_POINT('Ctrl Pts',(-1.85670509444853,1.3,2.85582368886185));
#28889=CARTESIAN_POINT('Ctrl Pts',(-1.85623323659832,1.3,2.86702301390781));
#28890=CARTESIAN_POINT('Ctrl Pts',(-1.85567755293928,1.3,2.88021190526076));
#28891=CARTESIAN_POINT('Ctrl Pts',(-1.85534153484999,1.3,2.89225944470745));
#28892=CARTESIAN_POINT('Ctrl Pts',(-1.85491006186869,1.3,2.90295344320832));
#28893=CARTESIAN_POINT('Ctrl Pts',(-1.85478465332402,1.3,2.90606167674066));
#28894=CARTESIAN_POINT('Ctrl Pts',(-1.85465444606568,1.3,2.90905549205128));
#28895=CARTESIAN_POINT('Ctrl Pts',(-1.85453421931241,1.3,2.91193055999209));
#28896=CARTESIAN_POINT('Ctrl Pts',(-1.85425731305134,1.3,2.91855241654326));
#28897=CARTESIAN_POINT('Ctrl Pts',(-1.85400169649198,1.3,2.92454378031362));
#28898=CARTESIAN_POINT('Ctrl Pts',(-1.85357635954475,1.3,2.92982815978896));
#28899=CARTESIAN_POINT('Ctrl Pts',(-1.85331787482462,1.3,2.93303956984536));
#28900=CARTESIAN_POINT('Ctrl Pts',(-1.85301417358302,1.3,2.9359903706631));
#28901=CARTESIAN_POINT('Ctrl Pts',(-1.85276389577182,1.3,2.93867303583745));
#28902=CARTESIAN_POINT('Ctrl Pts',(-1.85203942456943,1.3,2.9464384612068));
#28903=CARTESIAN_POINT('Ctrl Pts',(-1.85165865380786,1.3,2.95166509583937));
#28904=CARTESIAN_POINT('Ctrl Pts',(-1.85124074681822,1.3,2.95641359523244));
#28905=CARTESIAN_POINT('Ctrl Pts',(-1.85096598292866,1.3,2.9595356204562));
#28906=CARTESIAN_POINT('Ctrl Pts',(-1.85069885767855,1.3,2.96237084157569));
#28907=CARTESIAN_POINT('Ctrl Pts',(-1.85042671469841,1.3,2.96526229133589));
#28908=CARTESIAN_POINT('Ctrl Pts',(-1.85016557442577,1.3,2.96803684013488));
#28909=CARTESIAN_POINT('Ctrl Pts',(-1.84990350496385,1.3,2.9708641856712));
#28910=CARTESIAN_POINT('Ctrl Pts',(-1.84954418939433,1.3,2.97403920416527));
#28911=CARTESIAN_POINT('Ctrl Pts',(-1.84923315994381,1.3,2.97678755225074));
#28912=CARTESIAN_POINT('Ctrl Pts',(-1.84882683041588,1.3,2.97989392199881));
#28913=CARTESIAN_POINT('Ctrl Pts',(-1.84844777243925,1.3,2.98284440587253));
#28914=CARTESIAN_POINT('Ctrl Pts',(-1.84725567213586,1.3,2.99212338939983));
#28915=CARTESIAN_POINT('Ctrl Pts',(-1.8462860297191,1.3,3.00085502123862));
#28916=CARTESIAN_POINT('Ctrl Pts',(-1.84783999216021,1.3,3.00911085372699));
#28917=CARTESIAN_POINT('',(-2.05661148970878,1.3,3.10753059403928));
#28918=CARTESIAN_POINT('',(-1.84783999216022,1.3,3.00911085372699));
#28919=CARTESIAN_POINT('',(-2.29120499210816,1.30000000000064,2.92532110174576));
#28920=CARTESIAN_POINT('Ctrl Pts',(-2.05661148970878,1.3,3.10753059403928));
#28921=CARTESIAN_POINT('Ctrl Pts',(-2.06438529511965,1.3,3.10351053739145));
#28922=CARTESIAN_POINT('Ctrl Pts',(-2.07309811100438,1.3,3.09488481470888));
#28923=CARTESIAN_POINT('Ctrl Pts',(-2.08608645028851,1.3,3.08238039314201));
#28924=CARTESIAN_POINT('Ctrl Pts',(-2.09688680253806,1.3,3.07204590157201));
#28925=CARTESIAN_POINT('Ctrl Pts',(-2.11072923711644,1.3,3.06009427260729));
#28926=CARTESIAN_POINT('Ctrl Pts',(-2.13435227632379,1.3,3.0407328914854));
#28927=CARTESIAN_POINT('Ctrl Pts',(-2.15779105518433,1.29999999999999,3.02120880625423));
#28928=CARTESIAN_POINT('Ctrl Pts',(-2.18242600362798,1.29999999999999,3.00259488826929));
#28929=CARTESIAN_POINT('Ctrl Pts',(-2.20158377310446,1.29999999999999,2.98731694105395));
#28930=CARTESIAN_POINT('Ctrl Pts',(-2.22721864903229,1.29999999999999,2.96948359344277));
#28931=CARTESIAN_POINT('Ctrl Pts',(-2.25725367801875,1.29999999999997,2.94760389756073));
#28932=CARTESIAN_POINT('Ctrl Pts',(-2.27894790606329,1.29999999999997,2.93316799584485));
#28933=CARTESIAN_POINT('Ctrl Pts',(-2.29039127170519,1.29999999999997,2.92584463101117));
#28934=CARTESIAN_POINT('Ctrl Pts',(-2.29120499200655,1.29999999999997,2.92532110186514));
#28935=CARTESIAN_POINT('',(-2.74608525937212,1.30000000000049,3.202311199222));
#28936=CARTESIAN_POINT('Origin',(0.,1.3,7.2));
#28937=CARTESIAN_POINT('',(-2.67879510330291,1.3,3.48487937376242));
#28938=CARTESIAN_POINT('Ctrl Pts',(-2.74608525933252,1.3,3.20231119921555));
#28939=CARTESIAN_POINT('Ctrl Pts',(-2.74592314706517,1.3,3.20330586994931));
#28940=CARTESIAN_POINT('Ctrl Pts',(-2.74575725588899,1.3,3.20431266911));
#28941=CARTESIAN_POINT('Ctrl Pts',(-2.745587413402,1.3,3.20533113938524));
#28942=CARTESIAN_POINT('Ctrl Pts',(-2.74297531402366,1.3,3.22099474405838));
#28943=CARTESIAN_POINT('Ctrl Pts',(-2.73928848452582,1.3,3.23938453120443));
#28944=CARTESIAN_POINT('Ctrl Pts',(-2.73586109861741,1.3,3.25921559597869));
#28945=CARTESIAN_POINT('Ctrl Pts',(-2.73484312557184,1.3,3.26510565036547));
#28946=CARTESIAN_POINT('Ctrl Pts',(-2.73386685344387,1.3,3.2711284112336));
#28947=CARTESIAN_POINT('Ctrl Pts',(-2.73254890665973,1.3,3.27716215918157));
#28948=CARTESIAN_POINT('Ctrl Pts',(-2.73191131995472,1.3,3.28008112185844));
#28949=CARTESIAN_POINT('Ctrl Pts',(-2.73119017390953,1.3,3.28300152537924));
#28950=CARTESIAN_POINT('Ctrl Pts',(-2.73051127150851,1.3,3.28594500588927));
#28951=CARTESIAN_POINT('Ctrl Pts',(-2.72849187055887,1.3,3.29470041363015));
#28952=CARTESIAN_POINT('Ctrl Pts',(-2.72685428417164,1.3,3.30366556692271));
#28953=CARTESIAN_POINT('Ctrl Pts',(-2.72492380642212,1.3,3.31257530148778));
#28954=CARTESIAN_POINT('Ctrl Pts',(-2.72236580737704,1.3,3.32438123528583));
#28955=CARTESIAN_POINT('Ctrl Pts',(-2.71928291517288,1.3,3.33607991251617));
#28956=CARTESIAN_POINT('Ctrl Pts',(-2.71638775539464,1.3,3.34754495029874));
#28957=CARTESIAN_POINT('Ctrl Pts',(-2.71255125582638,1.3,3.36273776032373));
#28958=CARTESIAN_POINT('Ctrl Pts',(-2.70901769291549,1.3,3.377521969348));
#28959=CARTESIAN_POINT('Ctrl Pts',(-2.70554870841793,1.3,3.39118652568365));
#28960=CARTESIAN_POINT('Ctrl Pts',(-2.7040218274528,1.3,3.39720100945563));
#28961=CARTESIAN_POINT('Ctrl Pts',(-2.70250594885501,1.3,3.40299854130969));
#28962=CARTESIAN_POINT('Ctrl Pts',(-2.70087427516177,1.3,3.40848409353771));
#28963=CARTESIAN_POINT('Ctrl Pts',(-2.70000778040026,1.3,3.41139717737869));
#28964=CARTESIAN_POINT('Ctrl Pts',(-2.69911190347081,1.3,3.41422269682275));
#28965=CARTESIAN_POINT('Ctrl Pts',(-2.69825737393594,1.3,3.41697217111659));
#28966=CARTESIAN_POINT('Ctrl Pts',(-2.69618031045467,1.3,3.4236551848866));
#28967=CARTESIAN_POINT('Ctrl Pts',(-2.69436074527778,1.3,3.42976051800602));
#28968=CARTESIAN_POINT('Ctrl Pts',(-2.69306997616279,1.3,3.43401819985236));
#28969=CARTESIAN_POINT('Ctrl Pts',(-2.69114011425413,1.3,3.44038396884935));
#28970=CARTESIAN_POINT('Ctrl Pts',(-2.68999653222302,1.3,3.44420087101193));
#28971=CARTESIAN_POINT('Ctrl Pts',(-2.68773832472882,1.3,3.45092138645622));
#28972=CARTESIAN_POINT('Ctrl Pts',(-2.68689484823012,1.3,3.45343160611094));
#28973=CARTESIAN_POINT('Ctrl Pts',(-2.68582412772417,1.3,3.45649798649749));
#28974=CARTESIAN_POINT('Ctrl Pts',(-2.68484689460198,1.3,3.4593048285032));
#28975=CARTESIAN_POINT('Ctrl Pts',(-2.68164638744206,1.3,3.46849743335057));
#28976=CARTESIAN_POINT('Ctrl Pts',(-2.67898720638086,1.3,3.47666793233799));
#28977=CARTESIAN_POINT('Ctrl Pts',(-2.6787951033029,1.3,3.48487937376242));
#28978=CARTESIAN_POINT('',(-2.86254182811346,1.3,3.6245544416636));
#28979=CARTESIAN_POINT('',(-2.67879510330291,1.3,3.48487937376242));
#28980=CARTESIAN_POINT('',(-3.12967817046588,1.29999999999996,3.49492043954391));
#28981=CARTESIAN_POINT('Ctrl Pts',(-2.86254182811346,1.3,3.6245544416636));
#28982=CARTESIAN_POINT('Ctrl Pts',(-2.87098157399952,1.3,3.62223849792578));
#28983=CARTESIAN_POINT('Ctrl Pts',(-2.88132223312521,1.3,3.61563726783235));
#28984=CARTESIAN_POINT('Ctrl Pts',(-2.8966652799432,1.3,3.60615009400148));
#28985=CARTESIAN_POINT('Ctrl Pts',(-2.90932323850128,1.29999999999998,3.59822082837081));
#28986=CARTESIAN_POINT('Ctrl Pts',(-2.92824173701722,1.29999999999999,3.58819528871223));
#28987=CARTESIAN_POINT('Ctrl Pts',(-2.95503853269752,1.29999999999997,3.57380109025187));
#28988=CARTESIAN_POINT('Ctrl Pts',(-2.98205336859788,1.29999999999997,3.55962955254953));
#28989=CARTESIAN_POINT('Ctrl Pts',(-3.01841720312939,1.29999999999995,3.54262615901524));
#28990=CARTESIAN_POINT('Ctrl Pts',(-3.0434588220131,1.29999999999994,3.53074835161772));
#28991=CARTESIAN_POINT('Ctrl Pts',(-3.06669431743405,1.29999999999993,3.52131722426942));
#28992=CARTESIAN_POINT('Ctrl Pts',(-3.07792722226869,1.29999999999993,3.51617656284746));
#28993=CARTESIAN_POINT('Ctrl Pts',(-3.0920388719552,1.29999999999991,3.50983944286351));
#28994=CARTESIAN_POINT('Ctrl Pts',(-3.10963261570923,1.29999999999992,3.50299078553603));
#28995=CARTESIAN_POINT('Ctrl Pts',(-3.12214179520417,1.29999999999991,3.49799566328401));
#28996=CARTESIAN_POINT('Ctrl Pts',(-3.12880259493956,1.29999999999991,3.4952781850355));
#28997=CARTESIAN_POINT('Ctrl Pts',(-3.12967817039088,1.29999999999991,3.49492043957456));
#28998=CARTESIAN_POINT('',(-3.51715936790342,1.30000000000004,3.86052549337951));
#28999=CARTESIAN_POINT('Origin',(0.,1.3,7.2));
#29000=CARTESIAN_POINT('',(-3.39267401414619,1.3,4.12301649229107));
#29001=CARTESIAN_POINT('Ctrl Pts',(-3.51715936786488,1.3,3.86052549336462));
#29002=CARTESIAN_POINT('Ctrl Pts',(-3.50582685066179,1.3,3.88984355757898));
#29003=CARTESIAN_POINT('Ctrl Pts',(-3.46685584273537,1.3,3.98767483334669));
#29004=CARTESIAN_POINT('Ctrl Pts',(-3.40261508876044,1.3,4.10231519737892));
#29005=CARTESIAN_POINT('Ctrl Pts',(-3.39533368135243,1.3,4.11180043398003));
#29006=CARTESIAN_POINT('Ctrl Pts',(-3.3926740141462,1.3,4.12301649229107));
#29007=CARTESIAN_POINT('',(-3.54336535262991,1.3,4.29784241707854));
#29008=CARTESIAN_POINT('',(-3.39267401414619,1.3,4.12301649229107));
#29009=CARTESIAN_POINT('',(-3.83164255228946,1.29999999999999,4.22661550568205));
#29010=CARTESIAN_POINT('Ctrl Pts',(-3.54336535262991,1.3,4.29784241707854));
#29011=CARTESIAN_POINT('Ctrl Pts',(-3.55210218159752,1.3,4.29733180410519));
#29012=CARTESIAN_POINT('Ctrl Pts',(-3.56357804858823,1.3,4.29300353001696));
#29013=CARTESIAN_POINT('Ctrl Pts',(-3.58051111276238,1.3,4.28683090345647));
#29014=CARTESIAN_POINT('Ctrl Pts',(-3.5946404397042,1.3,4.281881159061));
#29015=CARTESIAN_POINT('Ctrl Pts',(-3.61201924717445,1.3,4.27637436927279));
#29016=CARTESIAN_POINT('Ctrl Pts',(-3.63003664337434,1.3,4.27211248343673));
#29017=CARTESIAN_POINT('Ctrl Pts',(-3.65295986932128,1.29999999999998,4.26452737687587));
#29018=CARTESIAN_POINT('Ctrl Pts',(-3.6892645645786,1.3,4.25643069318791));
#29019=CARTESIAN_POINT('Ctrl Pts',(-3.72475552906397,1.29999999999999,4.24706883683854));
#29020=CARTESIAN_POINT('Ctrl Pts',(-3.75540297439471,1.29999999999998,4.24116675613968));
#29021=CARTESIAN_POINT('Ctrl Pts',(-3.77374429985487,1.29999999999998,4.23757924625996));
#29022=CARTESIAN_POINT('Ctrl Pts',(-3.78867292218785,1.29999999999998,4.23397473293131));
#29023=CARTESIAN_POINT('Ctrl Pts',(-3.80118619929376,1.29999999999998,4.23210976365254));
#29024=CARTESIAN_POINT('Ctrl Pts',(-3.81344027727322,1.29999999999998,4.22979565281318));
#29025=CARTESIAN_POINT('Ctrl Pts',(-3.82363173700113,1.29999999999997,4.2280429461226));
#29026=CARTESIAN_POINT('Ctrl Pts',(-3.83071366500148,1.29999999999997,4.22678143362433));
#29027=CARTESIAN_POINT('Ctrl Pts',(-3.83164255214012,1.29999999999997,4.22661550570873));
#29028=CARTESIAN_POINT('',(-4.13466409677445,1.30000000000152,4.66483672982034));
#29029=CARTESIAN_POINT('Origin',(0.,1.3,7.2));
#29030=CARTESIAN_POINT('',(-3.95827679071515,1.3,4.89563255511164));
#29031=CARTESIAN_POINT('Ctrl Pts',(-4.13466409674311,1.3,4.66483672979985));
#29032=CARTESIAN_POINT('Ctrl Pts',(-4.09315488056353,1.3,4.72833921195976));
#29033=CARTESIAN_POINT('Ctrl Pts',(-4.0481896741846,1.30000000000031,4.78987080268933));
#29034=CARTESIAN_POINT('Ctrl Pts',(-3.99253637143538,1.30000000000031,4.85426406366701));
#29035=CARTESIAN_POINT('Ctrl Pts',(-3.98559379871555,1.3000000000003,4.86240513433244));
#29036=CARTESIAN_POINT('Ctrl Pts',(-3.96923168411537,1.3000000000003,4.88009738329383));
#29037=CARTESIAN_POINT('Ctrl Pts',(-3.96254124756276,1.3,4.88662737113017));
#29038=CARTESIAN_POINT('Ctrl Pts',(-3.95827679071516,1.3,4.89563255511163));
#29039=CARTESIAN_POINT('',(-4.06932680828303,1.3,5.09796860496431));
#29040=CARTESIAN_POINT('',(-3.95827679071515,1.3,4.89563255511164));
#29041=CARTESIAN_POINT('',(-4.36610424565707,1.30000000000001,5.0882155138236));
#29042=CARTESIAN_POINT('Ctrl Pts',(-4.06932680828303,1.3,5.09796860496431));
#29043=CARTESIAN_POINT('Ctrl Pts',(-4.07797887898237,1.3,5.09928563899255));
#29044=CARTESIAN_POINT('Ctrl Pts',(-4.09011340671472,1.3,5.09746151167884));
#29045=CARTESIAN_POINT('Ctrl Pts',(-4.10798906787033,1.3,5.09503481582656));
#29046=CARTESIAN_POINT('Ctrl Pts',(-4.12278056955995,1.3,5.09294345303559));
#29047=CARTESIAN_POINT('Ctrl Pts',(-4.14413938009718,1.3,5.091473450798));
#29048=CARTESIAN_POINT('Ctrl Pts',(-4.17448812907648,1.3,5.08925827165076));
#29049=CARTESIAN_POINT('Ctrl Pts',(-4.20490736605425,1.3,5.08723936162841));
#29050=CARTESIAN_POINT('Ctrl Pts',(-4.23275200389569,1.30000000000001,5.08689293279717));
#29051=CARTESIAN_POINT('Ctrl Pts',(-4.25108091289331,1.30000000000001,5.08598794103597));
#29052=CARTESIAN_POINT('Ctrl Pts',(-4.26664152659686,1.30000000000001,5.08612728928339));
#29053=CARTESIAN_POINT('Ctrl Pts',(-4.27900308121979,1.30000000000001,5.08598697165463));
#29054=CARTESIAN_POINT('Ctrl Pts',(-4.29779355786982,1.30000000000001,5.08657564277857));
#29055=CARTESIAN_POINT('Ctrl Pts',(-4.32551587266611,1.30000000000003,5.08605420816759));
#29056=CARTESIAN_POINT('Ctrl Pts',(-4.35171241440574,1.30000000000002,5.08772479474994));
#29057=CARTESIAN_POINT('Ctrl Pts',(-4.36515927599734,1.30000000000002,5.08818455598542));
#29058=CARTESIAN_POINT('Ctrl Pts',(-4.36610424531595,1.30000000000002,5.08821551381243));
#29059=CARTESIAN_POINT('',(-4.57136452277826,1.30000000000254,5.57977581816781));
#29060=CARTESIAN_POINT('Origin',(0.,1.3,7.2));
#29061=CARTESIAN_POINT('',(-4.35088387761047,1.3,5.76896053285564));
#29062=CARTESIAN_POINT('Ctrl Pts',(-4.57136452274418,1.3,5.57977581813352));
#29063=CARTESIAN_POINT('Ctrl Pts',(-4.51754002640381,1.3,5.63325957053971));
#29064=CARTESIAN_POINT('Ctrl Pts',(-4.46083948717456,1.30000000000647,5.68419491725153));
#29065=CARTESIAN_POINT('Ctrl Pts',(-4.38996093886439,1.30000000000647,5.73802002909746));
#29066=CARTESIAN_POINT('Ctrl Pts',(-4.38483171389866,1.30000000000651,5.74208126366599));
#29067=CARTESIAN_POINT('Ctrl Pts',(-4.36574496082626,1.30000000000651,5.75538076255523));
#29068=CARTESIAN_POINT('Ctrl Pts',(-4.35689160691752,1.3,5.76108571890034));
#29069=CARTESIAN_POINT('Ctrl Pts',(-4.35088387761047,1.3,5.76896053285564));
#29070=CARTESIAN_POINT('',(-4.41743915561768,1.3,5.98996365147886));
#29071=CARTESIAN_POINT('',(-4.35088387761047,1.3,5.76896053285564));
#29072=CARTESIAN_POINT('',(-4.70979325221238,1.30000000000053,6.04226621306406));
#29073=CARTESIAN_POINT('Ctrl Pts',(-4.41743915561768,1.3,5.98996365147886));
#29074=CARTESIAN_POINT('Ctrl Pts',(-4.42562833104198,1.3,5.99305077180187));
#29075=CARTESIAN_POINT('Ctrl Pts',(-4.43787410397313,1.30000000000004,5.99377070921043));
#29076=CARTESIAN_POINT('Ctrl Pts',(-4.45586248406724,1.30000000000007,5.99510260510018));
#29077=CARTESIAN_POINT('Ctrl Pts',(-4.47076472138646,1.30000000000009,5.99612876774796));
#29078=CARTESIAN_POINT('Ctrl Pts',(-4.49195835498715,1.30000000000015,5.99908948996134));
#29079=CARTESIAN_POINT('Ctrl Pts',(-4.52210835638369,1.30000000000015,6.00327770721702));
#29080=CARTESIAN_POINT('Ctrl Pts',(-4.55226320816141,1.30000000000036,6.00741263999137));
#29081=CARTESIAN_POINT('Ctrl Pts',(-4.57654950949712,1.30000000000046,6.01237589346951));
#29082=CARTESIAN_POINT('Ctrl Pts',(-4.60070795159453,1.30000000000046,6.0162343787984));
#29083=CARTESIAN_POINT('Ctrl Pts',(-4.6311368113507,1.30000000000088,6.02353250784579));
#29084=CARTESIAN_POINT('Ctrl Pts',(-4.67053008929459,1.30000000000101,6.0319106295725));
#29085=CARTESIAN_POINT('Ctrl Pts',(-4.69577141109484,1.30000000000119,6.0384019209567));
#29086=CARTESIAN_POINT('Ctrl Pts',(-4.70886570174723,1.30000000000123,6.04201282916357));
#29087=CARTESIAN_POINT('Ctrl Pts',(-4.70979325209678,1.30000000000123,6.04226621303244));
#29088=CARTESIAN_POINT('',(-4.80835019122325,1.30000000000007,6.56575364560707));
#29089=CARTESIAN_POINT('Origin',(0.,1.3,7.2));
#29090=CARTESIAN_POINT('',(-4.55333646119701,1.3,6.70483180220308));
#29091=CARTESIAN_POINT('Ctrl Pts',(-4.80835019119519,1.3,6.56575364556359));
#29092=CARTESIAN_POINT('Ctrl Pts',(-4.7434061141498,1.3,6.60767583956299));
#29093=CARTESIAN_POINT('Ctrl Pts',(-4.72650779342684,1.29999999999997,6.61707548172361));
#29094=CARTESIAN_POINT('Ctrl Pts',(-4.6403689076869,1.29999999999997,6.66208434195179));
#29095=CARTESIAN_POINT('Ctrl Pts',(-4.63296554263347,1.29999999999999,6.66644578587599));
#29096=CARTESIAN_POINT('Ctrl Pts',(-4.57698227389077,1.29999999999999,6.69210759502936));
#29097=CARTESIAN_POINT('Ctrl Pts',(-4.56282896282898,1.3,6.6966785332743));
#29098=CARTESIAN_POINT('Ctrl Pts',(-4.55333646119701,1.3,6.70483180220308));
#29099=CARTESIAN_POINT('',(-4.57248821462698,1.3,6.9348430928224));
#29100=CARTESIAN_POINT('',(-4.55333646119701,1.3,6.70483180220308));
#29101=CARTESIAN_POINT('',(-4.84757460734146,1.3,7.04663629419473));
#29102=CARTESIAN_POINT('Ctrl Pts',(-4.57248821462698,1.3,6.9348430928224));
#29103=CARTESIAN_POINT('Ctrl Pts',(-4.5798565885141,1.3,6.93956537746838));
#29104=CARTESIAN_POINT('Ctrl Pts',(-4.59168429755987,1.3,6.94283346090675));
#29105=CARTESIAN_POINT('Ctrl Pts',(-4.60900164344958,1.3,6.94788682421139));
#29106=CARTESIAN_POINT('Ctrl Pts',(-4.62336514575569,1.3,6.95199202349994));
#29107=CARTESIAN_POINT('Ctrl Pts',(-4.64347549796415,1.3,6.95933528312236));
#29108=CARTESIAN_POINT('Ctrl Pts',(-4.67210160956593,1.3,6.96965511487844));
#29109=CARTESIAN_POINT('Ctrl Pts',(-4.70071250038716,1.3,6.98017995874042));
#29110=CARTESIAN_POINT('Ctrl Pts',(-4.72629088154586,1.3,6.99118791773456));
#29111=CARTESIAN_POINT('Ctrl Pts',(-4.74340328278023,1.3,6.99781595031789));
#29112=CARTESIAN_POINT('Ctrl Pts',(-4.75756194704263,1.3,7.00427217122634));
#29113=CARTESIAN_POINT('Ctrl Pts',(-4.76891185654316,1.3,7.00917189133043));
#29114=CARTESIAN_POINT('Ctrl Pts',(-4.78583835543268,1.3,7.01735252591455));
#29115=CARTESIAN_POINT('Ctrl Pts',(-4.81137590685574,1.3,7.02815247242249));
#29116=CARTESIAN_POINT('Ctrl Pts',(-4.83462754895962,1.3,7.04033440400255));
#29117=CARTESIAN_POINT('Ctrl Pts',(-4.84672437123211,1.3,7.04622385103896));
#29118=CARTESIAN_POINT('Ctrl Pts',(-4.84757460701277,1.3,7.04663629403529));
#29119=CARTESIAN_POINT('',(-4.83514000566344,1.30000000008923,7.57936937611262));
#29120=CARTESIAN_POINT('Origin',(0.,1.3,7.2));
#29121=CARTESIAN_POINT('',(-4.55678639209675,1.3,7.66234429787488));
#29122=CARTESIAN_POINT('Ctrl Pts',(-4.83514000561781,1.3,7.57936937599151));
#29123=CARTESIAN_POINT('Ctrl Pts',(-4.83419097024645,1.3,7.57972696234589));
#29124=CARTESIAN_POINT('Ctrl Pts',(-4.83323821194189,1.3,7.58008513247196));
#29125=CARTESIAN_POINT('Ctrl Pts',(-4.83228194790045,1.3,7.58044402446448));
#29126=CARTESIAN_POINT('Ctrl Pts',(-4.82124539004742,1.3,7.58458611500299));
#29127=CARTESIAN_POINT('Ctrl Pts',(-4.80974201417162,1.3,7.58882670514177));
#29128=CARTESIAN_POINT('Ctrl Pts',(-4.79795307756342,1.3,7.59296283947731));
#29129=CARTESIAN_POINT('Ctrl Pts',(-4.79652635944612,1.3,7.59346340182557));
#29130=CARTESIAN_POINT('Ctrl Pts',(-4.79509548726416,1.3,7.59396253106982));
#29131=CARTESIAN_POINT('Ctrl Pts',(-4.7936535395449,1.3,7.59443920076872));
#29132=CARTESIAN_POINT('Ctrl Pts',(-4.78938085605041,1.3,7.59585163668968));
#29133=CARTESIAN_POINT('Ctrl Pts',(-4.78501089289788,1.3,7.59706283538183));
#29134=CARTESIAN_POINT('Ctrl Pts',(-4.78073579922085,1.3,7.5985929666076));
#29135=CARTESIAN_POINT('Ctrl Pts',(-4.77785428940659,1.3,7.59962430965578));
#29136=CARTESIAN_POINT('Ctrl Pts',(-4.77501388452526,1.3,7.60079734333637));
#29137=CARTESIAN_POINT('Ctrl Pts',(-4.77215073536344,1.3,7.60191808577717));
#29138=CARTESIAN_POINT('Ctrl Pts',(-4.77072659903648,1.3,7.60247554538996));
#29139=CARTESIAN_POINT('Ctrl Pts',(-4.769296968437,1.3,7.6030202762138));
#29140=CARTESIAN_POINT('Ctrl Pts',(-4.76785580911974,1.3,7.60353277750965));
#29141=CARTESIAN_POINT('Ctrl Pts',(-4.76642912909357,1.3,7.60404012971798));
#29142=CARTESIAN_POINT('Ctrl Pts',(-4.76499106435748,1.3,7.60451551720438));
#29143=CARTESIAN_POINT('Ctrl Pts',(-4.76355258318755,1.3,7.60498986104352));
#29144=CARTESIAN_POINT('Ctrl Pts',(-4.74038334903627,1.3,7.61262999127744));
#29145=CARTESIAN_POINT('Ctrl Pts',(-4.71743823325545,1.3,7.61992997683004));
#29146=CARTESIAN_POINT('Ctrl Pts',(-4.69454547239695,1.3,7.62649274471369));
#29147=CARTESIAN_POINT('Ctrl Pts',(-4.68209916288128,1.3,7.6300607827002));
#29148=CARTESIAN_POINT('Ctrl Pts',(-4.67003039171006,1.3,7.63333245595284));
#29149=CARTESIAN_POINT('Ctrl Pts',(-4.65995652632322,1.3,7.63618341831681));
#29150=CARTESIAN_POINT('Ctrl Pts',(-4.65313633315566,1.3,7.6381135725614));
#29151=CARTESIAN_POINT('Ctrl Pts',(-4.64721746850589,1.3,7.63980698908736));
#29152=CARTESIAN_POINT('Ctrl Pts',(-4.64265064572876,1.3,7.64103597342789));
#29153=CARTESIAN_POINT('Ctrl Pts',(-4.63895509819979,1.3,7.6420304876152));
#29154=CARTESIAN_POINT('Ctrl Pts',(-4.63651780229139,1.3,7.64264706904322));
#29155=CARTESIAN_POINT('Ctrl Pts',(-4.63398843337283,1.3,7.64325317280513));
#29156=CARTESIAN_POINT('Ctrl Pts',(-4.63111165446774,1.3,7.64394252519803));
#29157=CARTESIAN_POINT('Ctrl Pts',(-4.62821644281675,1.3,7.64457987313622));
#29158=CARTESIAN_POINT('Ctrl Pts',(-4.62533042545875,1.3,7.64523212643175));
#29159=CARTESIAN_POINT('Ctrl Pts',(-4.61948156938312,1.3,7.64655399500605));
#29160=CARTESIAN_POINT('Ctrl Pts',(-4.6136656043277,1.3,7.64793750472749));
#29161=CARTESIAN_POINT('Ctrl Pts',(-4.60797408626637,1.3,7.64926722192711));
#29162=CARTESIAN_POINT('Ctrl Pts',(-4.60203015483469,1.3,7.65065591080993));
#29163=CARTESIAN_POINT('Ctrl Pts',(-4.59622578392498,1.3,7.65198073034883));
#29164=CARTESIAN_POINT('Ctrl Pts',(-4.59066919321539,1.3,7.65310460254942));
#29165=CARTESIAN_POINT('Ctrl Pts',(-4.58768770325936,1.3,7.65370763664947));
#29166=CARTESIAN_POINT('Ctrl Pts',(-4.58477730158393,1.3,7.65425612837712));
#29167=CARTESIAN_POINT('Ctrl Pts',(-4.58196278725844,1.3,7.65479373462267));
#29168=CARTESIAN_POINT('Ctrl Pts',(-4.57189339261782,1.3,7.65671711067325));
#29169=CARTESIAN_POINT('Ctrl Pts',(-4.56309464195952,1.3,7.65889637743072));
#29170=CARTESIAN_POINT('Ctrl Pts',(-4.55678639209676,1.3,7.66234429787489));
#29171=CARTESIAN_POINT('',(-4.52769759742429,1.3,7.89131116337361));
#29172=CARTESIAN_POINT('',(-4.55678639209675,1.3,7.66234429787488));
#29173=CARTESIAN_POINT('',(-4.77350315750453,1.30000000000009,8.05800210098462));
#29174=CARTESIAN_POINT('Ctrl Pts',(-4.52769759742429,1.3,7.89131116337361));
#29175=CARTESIAN_POINT('Ctrl Pts',(-4.53392313647801,1.3,7.8974622258435));
#29176=CARTESIAN_POINT('Ctrl Pts',(-4.54481935244901,1.30000000000001,7.90309006287113));
#29177=CARTESIAN_POINT('Ctrl Pts',(-4.56073685668485,1.30000000000002,7.91153981038679));
#29178=CARTESIAN_POINT('Ctrl Pts',(-4.57387095253533,1.30000000000002,7.91873059084141));
#29179=CARTESIAN_POINT('Ctrl Pts',(-4.58959025693521,1.30000000000004,7.927944597891));
#29180=CARTESIAN_POINT('Ctrl Pts',(-4.60482087637025,1.30000000000004,7.93850976730446));
#29181=CARTESIAN_POINT('Ctrl Pts',(-4.62584154984425,1.30000000000006,7.95030089779444));
#29182=CARTESIAN_POINT('Ctrl Pts',(-4.65100328639092,1.30000000000009,7.96856552395811));
#29183=CARTESIAN_POINT('Ctrl Pts',(-4.68168781869127,1.30000000000013,7.98876229901975));
#29184=CARTESIAN_POINT('Ctrl Pts',(-4.70425849103461,1.30000000000015,8.00522489773813));
#29185=CARTESIAN_POINT('Ctrl Pts',(-4.71912910902609,1.30000000000016,8.0166759369683));
#29186=CARTESIAN_POINT('Ctrl Pts',(-4.72919200083095,1.30000000000016,8.02385128590682));
#29187=CARTESIAN_POINT('Ctrl Pts',(-4.74174314804138,1.30000000000018,8.03287907296244));
#29188=CARTESIAN_POINT('Ctrl Pts',(-4.75647533498549,1.3000000000002,8.04467732548915));
#29189=CARTESIAN_POINT('Ctrl Pts',(-4.76705952279732,1.30000000000021,8.05301621943483));
#29190=CARTESIAN_POINT('Ctrl Pts',(-4.77275066854619,1.30000000000022,8.05742047528334));
#29191=CARTESIAN_POINT('Ctrl Pts',(-4.77350315748042,1.30000000000022,8.05800210096597));
#29192=CARTESIAN_POINT('',(-4.65061125535824,1.29999999999665,8.57625414053201));
#29193=CARTESIAN_POINT('Origin',(0.,1.3,7.2));
#29194=CARTESIAN_POINT('',(-4.36108289177478,1.3,8.59965012915547));
#29195=CARTESIAN_POINT('Ctrl Pts',(-4.65058430230005,1.3,8.57625821131574));
#29196=CARTESIAN_POINT('Ctrl Pts',(-4.6495875835157,1.3,8.57640874172956));
#29197=CARTESIAN_POINT('Ctrl Pts',(-4.6485907689512,1.3,8.57655893939737));
#29198=CARTESIAN_POINT('Ctrl Pts',(-4.6475939573955,1.3,8.57670945662017));
#29199=CARTESIAN_POINT('Ctrl Pts',(-4.6355533009042,1.3,8.57852757978046));
#29200=CARTESIAN_POINT('Ctrl Pts',(-4.6235110513442,1.3,8.58039535440588));
#29201=CARTESIAN_POINT('Ctrl Pts',(-4.61140829826703,1.3,8.58183234538072));
#29202=CARTESIAN_POINT('Ctrl Pts',(-4.60539370804484,1.3,8.58254647313426));
#29203=CARTESIAN_POINT('Ctrl Pts',(-4.59936562178916,1.3,8.58315349116365));
#29204=CARTESIAN_POINT('Ctrl Pts',(-4.59336338090833,1.3,8.58396597893305));
#29205=CARTESIAN_POINT('Ctrl Pts',(-4.58732043535485,1.3,8.5847839766527));
#29206=CARTESIAN_POINT('Ctrl Pts',(-4.58130099734447,1.3,8.58580835441553));
#29207=CARTESIAN_POINT('Ctrl Pts',(-4.57524472399301,1.3,8.58653298671471));
#29208=CARTESIAN_POINT('Ctrl Pts',(-4.56925971555996,1.3,8.5872490921759));
#29209=CARTESIAN_POINT('Ctrl Pts',(-4.56324090758591,1.3,8.58766473828875));
#29210=CARTESIAN_POINT('Ctrl Pts',(-4.55724511852431,1.3,8.58827649344112));
#29211=CARTESIAN_POINT('Ctrl Pts',(-4.5512176382313,1.3,8.58889148207517));
#29212=CARTESIAN_POINT('Ctrl Pts',(-4.54521048860568,1.3,8.58970340650068));
#29213=CARTESIAN_POINT('Ctrl Pts',(-4.53918575032511,1.3,8.590349951669));
#29214=CARTESIAN_POINT('Ctrl Pts',(-4.52725372665985,1.3,8.59163043754072));
#29215=CARTESIAN_POINT('Ctrl Pts',(-4.51526184714999,1.3,8.59224977873498));
#29216=CARTESIAN_POINT('Ctrl Pts',(-4.5032919926851,1.3,8.59300958029857));
#29217=CARTESIAN_POINT('Ctrl Pts',(-4.49132452209666,1.3,8.5937692305426));
#29218=CARTESIAN_POINT('Ctrl Pts',(-4.47937209380073,1.3,8.59467395052153));
#29219=CARTESIAN_POINT('Ctrl Pts',(-4.46741124492339,1.3,8.59549545051039));
#29220=CARTESIAN_POINT('Ctrl Pts',(-4.46143603156469,1.3,8.59590584259527));
#29221=CARTESIAN_POINT('Ctrl Pts',(-4.45545887627245,1.3,8.596295629844));
#29222=CARTESIAN_POINT('Ctrl Pts',(-4.44947791681133,1.3,8.59660698982628));
#29223=CARTESIAN_POINT('Ctrl Pts',(-4.44650105055845,1.3,8.59676196111973));
#29224=CARTESIAN_POINT('Ctrl Pts',(-4.44352321944155,1.3,8.59689768988603));
#29225=CARTESIAN_POINT('Ctrl Pts',(-4.44054357105003,1.3,8.59697309156111));
#29226=CARTESIAN_POINT('Ctrl Pts',(-4.43758401047722,1.3,8.59704798490266));
#29227=CARTESIAN_POINT('Ctrl Pts',(-4.43462290252627,1.3,8.5970627433161));
#29228=CARTESIAN_POINT('Ctrl Pts',(-4.43166289976314,1.3,8.59709880909697));
#29229=CARTESIAN_POINT('Ctrl Pts',(-4.4258852251388,1.3,8.59716920644575));
#29230=CARTESIAN_POINT('Ctrl Pts',(-4.42019491457939,1.3,8.59732137622975));
#29231=CARTESIAN_POINT('Ctrl Pts',(-4.41384885731029,1.3,8.59744228461716));
#29232=CARTESIAN_POINT('Ctrl Pts',(-4.40828798224256,1.3,8.59754823330444));
#29233=CARTESIAN_POINT('Ctrl Pts',(-4.40235627801372,1.3,8.5976248940948));
#29234=CARTESIAN_POINT('Ctrl Pts',(-4.3961230007992,1.3,8.59759099519588));
#29235=CARTESIAN_POINT('Ctrl Pts',(-4.39315805428831,1.3,8.59757487070492));
#29236=CARTESIAN_POINT('Ctrl Pts',(-4.39009395819138,1.3,8.59753057587581));
#29237=CARTESIAN_POINT('Ctrl Pts',(-4.38726532243509,1.3,8.59746198288177));
#29238=CARTESIAN_POINT('Ctrl Pts',(-4.38411848835464,1.3,8.59738567373845));
#29239=CARTESIAN_POINT('Ctrl Pts',(-4.38116136924875,1.3,8.59728836610966));
#29240=CARTESIAN_POINT('Ctrl Pts',(-4.37832669149765,1.3,8.59732091390751));
#29241=CARTESIAN_POINT('Ctrl Pts',(-4.3722147640682,1.3,8.59739109111845));
#29242=CARTESIAN_POINT('Ctrl Pts',(-4.36669022745341,1.3,8.59797213156775));
#29243=CARTESIAN_POINT('Ctrl Pts',(-4.36108289177478,1.3,8.59965012915547));
#29244=CARTESIAN_POINT('',(-4.28502486891058,1.3,8.81756561880638));
#29245=CARTESIAN_POINT('',(-4.36108289177478,1.3,8.59965012915547));
#29246=CARTESIAN_POINT('',(-4.49082727704381,1.29999999999945,9.03165781950697));
#29247=CARTESIAN_POINT('Ctrl Pts',(-4.28502486891058,1.3,8.81756561880638));
#29248=CARTESIAN_POINT('Ctrl Pts',(-4.2898354872008,1.3,8.8248766281542));
#29249=CARTESIAN_POINT('Ctrl Pts',(-4.29932549685833,1.29999999999993,8.83264384777641));
#29250=CARTESIAN_POINT('Ctrl Pts',(-4.31313904561508,1.29999999999991,8.84421728449725));
#29251=CARTESIAN_POINT('Ctrl Pts',(-4.32449237549068,1.29999999999986,8.8539796218888));
#29252=CARTESIAN_POINT('Ctrl Pts',(-4.33795366492192,1.29999999999982,8.86625855451921));
#29253=CARTESIAN_POINT('Ctrl Pts',(-4.35065688898753,1.29999999999975,8.87975609279067));
#29254=CARTESIAN_POINT('Ctrl Pts',(-4.36876695393333,1.29999999999971,8.89565957397917));
#29255=CARTESIAN_POINT('Ctrl Pts',(-4.38958862281826,1.29999999999944,8.91874421566872));
#29256=CARTESIAN_POINT('Ctrl Pts',(-4.41540753427271,1.29999999999926,8.94487233749321));
#29257=CARTESIAN_POINT('Ctrl Pts',(-4.43406590057313,1.29999999999911,8.96566151560513));
#29258=CARTESIAN_POINT('Ctrl Pts',(-4.44623256960715,1.29999999999905,8.97995099359928));
#29259=CARTESIAN_POINT('Ctrl Pts',(-4.45458379296231,1.29999999999901,8.98906155763134));
#29260=CARTESIAN_POINT('Ctrl Pts',(-4.46498628653592,1.29999999999898,9.00049726618221));
#29261=CARTESIAN_POINT('Ctrl Pts',(-4.47694277519802,1.29999999999885,9.01510154466921));
#29262=CARTESIAN_POINT('Ctrl Pts',(-4.48556751235134,1.29999999999877,9.02544344919194));
#29263=CARTESIAN_POINT('Ctrl Pts',(-4.49021466107917,1.29999999999873,9.03093465841783));
#29264=CARTESIAN_POINT('Ctrl Pts',(-4.4908272770097,1.29999999999872,9.03165781946676));
#29265=CARTESIAN_POINT('',(-4.26286793815783,1.30000000000209,9.51310547565977));
#29266=CARTESIAN_POINT('Origin',(0.,1.3,7.2));
#29267=CARTESIAN_POINT('',(-3.97477914228474,1.3,9.47578453352548));
#29268=CARTESIAN_POINT('Ctrl Pts',(-4.2628679381595,1.3,9.51310547563085));
#29269=CARTESIAN_POINT('Ctrl Pts',(-4.18712155066313,1.3,9.50872478499194));
#29270=CARTESIAN_POINT('Ctrl Pts',(-4.11130619555387,1.30000000000629,9.5009205299035));
#29271=CARTESIAN_POINT('Ctrl Pts',(-4.02380326491958,1.30000000000629,9.48408990538011));
#29272=CARTESIAN_POINT('Ctrl Pts',(-4.01872677589918,1.3000000000063,9.4833016605151));
#29273=CARTESIAN_POINT('Ctrl Pts',(-3.99411124458743,1.3000000000063,9.47759067102414));
#29274=CARTESIAN_POINT('Ctrl Pts',(-3.98430478699325,1.3,9.47500810534561));
#29275=CARTESIAN_POINT('Ctrl Pts',(-3.97477914228474,1.3,9.47578453352547));
#29276=CARTESIAN_POINT('',(-3.85507599179487,1.3,9.6731246947563));
#29277=CARTESIAN_POINT('',(-3.97477914228474,1.3,9.47578453352548));
#29278=CARTESIAN_POINT('',(-4.01176129273638,1.30000000000074,9.92548471807191));
#29279=CARTESIAN_POINT('Ctrl Pts',(-3.85507599179487,1.3,9.6731246947563));
#29280=CARTESIAN_POINT('Ctrl Pts',(-3.85719962541057,1.3,9.67855898144637));
#29281=CARTESIAN_POINT('Ctrl Pts',(-3.86187591307552,1.3,9.68616633802149));
#29282=CARTESIAN_POINT('Ctrl Pts',(-3.86961829094849,1.3,9.69559038157922));
#29283=CARTESIAN_POINT('Ctrl Pts',(-3.87691775533033,1.3,9.70509517032314));
#29284=CARTESIAN_POINT('Ctrl Pts',(-3.88601575983783,1.3,9.71700697516693));
#29285=CARTESIAN_POINT('Ctrl Pts',(-3.89402362564178,1.3,9.72807138563928));
#29286=CARTESIAN_POINT('Ctrl Pts',(-3.89895590723415,1.3,9.73584729023011));
#29287=CARTESIAN_POINT('Ctrl Pts',(-3.90225564380959,1.3,9.74103523695475));
#29288=CARTESIAN_POINT('Ctrl Pts',(-3.90808032589377,1.3,9.75005250397545));
#29289=CARTESIAN_POINT('Ctrl Pts',(-3.92066850316574,1.3,9.76696249005104));
#29290=CARTESIAN_POINT('Ctrl Pts',(-3.93465792264323,1.3,9.79123516446284));
#29291=CARTESIAN_POINT('Ctrl Pts',(-3.94790798782012,1.3,9.8118165641029));
#29292=CARTESIAN_POINT('Ctrl Pts',(-3.95754151618004,1.30000000000002,9.82759293428611));
#29293=CARTESIAN_POINT('Ctrl Pts',(-3.96543595276435,1.29999999999999,9.84087661025074));
#29294=CARTESIAN_POINT('Ctrl Pts',(-3.97449492745696,1.3,9.8572589811272));
#29295=CARTESIAN_POINT('Ctrl Pts',(-3.98377635983763,1.3,9.87337467813515));
#29296=CARTESIAN_POINT('Ctrl Pts',(-3.99612389890649,1.30000000000002,9.89487963847089));
#29297=CARTESIAN_POINT('Ctrl Pts',(-4.00523044215879,1.30000000000001,9.91248203324778));
#29298=CARTESIAN_POINT('Ctrl Pts',(-4.01132444103615,1.30000000000001,9.92462053118691));
#29299=CARTESIAN_POINT('Ctrl Pts',(-4.01176063670267,1.30000000000001,9.92548407605884));
#29300=CARTESIAN_POINT('',(-3.68879127699578,1.3000000000002,10.3488599388502));
#29301=CARTESIAN_POINT('Origin',(0.,1.3,7.2));
#29302=CARTESIAN_POINT('',(-3.4147584711704,1.3,10.2524562333546));
#29303=CARTESIAN_POINT('Ctrl Pts',(-3.68879127700292,1.3,10.3488599388241));
#29304=CARTESIAN_POINT('Ctrl Pts',(-3.61561107823774,1.3,10.3288266201356));
#29305=CARTESIAN_POINT('Ctrl Pts',(-3.5430756359792,1.30000000000053,10.3054288287531));
#29306=CARTESIAN_POINT('Ctrl Pts',(-3.46098540050118,1.30000000000053,10.270773167704));
#29307=CARTESIAN_POINT('Ctrl Pts',(-3.45618327613316,1.30000000000052,10.2689465255546));
#29308=CARTESIAN_POINT('Ctrl Pts',(-3.43329266685346,1.30000000000052,10.2582422684741));
#29309=CARTESIAN_POINT('Ctrl Pts',(-3.42423747329421,1.3,10.2536772761121));
#29310=CARTESIAN_POINT('Ctrl Pts',(-3.4147584711704,1.3,10.2524562333546));
#29311=CARTESIAN_POINT('',(-3.25664179513071,1.3,10.4205963541764));
#29312=CARTESIAN_POINT('',(-3.4147584711704,1.3,10.2524562333546));
#29313=CARTESIAN_POINT('',(-3.35750281628615,1.30000000000089,10.6999535480671));
#29314=CARTESIAN_POINT('Ctrl Pts',(-3.25664179513071,1.3,10.4205963541764));
#29315=CARTESIAN_POINT('Ctrl Pts',(-3.25806285821861,1.3,10.4292319482914));
#29316=CARTESIAN_POINT('Ctrl Pts',(-3.26356414651618,1.30000000000008,10.4401950374537));
#29317=CARTESIAN_POINT('Ctrl Pts',(-3.27146918596613,1.30000000000012,10.4563930038539));
#29318=CARTESIAN_POINT('Ctrl Pts',(-3.27787351976156,1.30000000000018,10.4699243752486));
#29319=CARTESIAN_POINT('Ctrl Pts',(-3.2851479844364,1.30000000000024,10.486646198898));
#29320=CARTESIAN_POINT('Ctrl Pts',(-3.29130852430374,1.30000000000035,10.5040919019837));
#29321=CARTESIAN_POINT('Ctrl Pts',(-3.30114479310941,1.30000000000045,10.5261721228317));
#29322=CARTESIAN_POINT('Ctrl Pts',(-3.31534105722496,1.30000000000063,10.5670370259464));
#29323=CARTESIAN_POINT('Ctrl Pts',(-3.33189443614984,1.30000000000123,10.6133610002865));
#29324=CARTESIAN_POINT('Ctrl Pts',(-3.34316994757927,1.30000000000171,10.649779142451));
#29325=CARTESIAN_POINT('Ctrl Pts',(-3.34713592831131,1.30000000000175,10.6632708594138));
#29326=CARTESIAN_POINT('Ctrl Pts',(-3.34797075229533,1.30000000000177,10.6663022138394));
#29327=CARTESIAN_POINT('Ctrl Pts',(-3.34938363968462,1.30000000000175,10.6716401187348));
#29328=CARTESIAN_POINT('Ctrl Pts',(-3.35249794888383,1.30000000000182,10.6821059278266));
#29329=CARTESIAN_POINT('Ctrl Pts',(-3.35524625903208,1.30000000000193,10.6921138091528));
#29330=CARTESIAN_POINT('Ctrl Pts',(-3.35723820844024,1.30000000000204,10.6990377857127));
#29331=CARTESIAN_POINT('Ctrl Pts',(-3.35750281627144,1.30000000000205,10.699953548016));
#29332=CARTESIAN_POINT('',(-2.95338171769359,1.3,11.0470815470423));
#29333=CARTESIAN_POINT('Origin',(0.,1.3,7.2));
#29334=CARTESIAN_POINT('',(-2.70549646903679,1.3,10.8957209484761));
#29335=CARTESIAN_POINT('Ctrl Pts',(-2.95338171769359,1.3,11.0470815470423));
#29336=CARTESIAN_POINT('Ctrl Pts',(-2.95247588339834,1.3,11.0466168870669));
#29337=CARTESIAN_POINT('Ctrl Pts',(-2.95157040531699,1.3,11.0461514383438));
#29338=CARTESIAN_POINT('Ctrl Pts',(-2.95066525202913,1.3,11.0456852690531));
#29339=CARTESIAN_POINT('Ctrl Pts',(-2.93984365977446,1.3,11.0401119655544));
#29340=CARTESIAN_POINT('Ctrl Pts',(-2.92906721124797,1.3,11.0344361051911));
#29341=CARTESIAN_POINT('Ctrl Pts',(-2.9184176123353,1.3,11.028522211404));
#29342=CARTESIAN_POINT('Ctrl Pts',(-2.91577535418661,1.3,11.0270549229007));
#29343=CARTESIAN_POINT('Ctrl Pts',(-2.91314085605255,1.3,11.0255730743499));
#29344=CARTESIAN_POINT('Ctrl Pts',(-2.91053216609454,1.3,11.0240442761547));
#29345=CARTESIAN_POINT('Ctrl Pts',(-2.90792830457153,1.3,11.0225183076183));
#29346=CARTESIAN_POINT('Ctrl Pts',(-2.9053500848189,1.3,11.0209465056074));
#29347=CARTESIAN_POINT('Ctrl Pts',(-2.90269735027348,1.3,11.0195104701681));
#29348=CARTESIAN_POINT('Ctrl Pts',(-2.90000088688124,1.3,11.0180507624869));
#29349=CARTESIAN_POINT('Ctrl Pts',(-2.89722916133843,1.3,11.0167267722398));
#29350=CARTESIAN_POINT('Ctrl Pts',(-2.89448316298046,1.3,11.0153542728071));
#29351=CARTESIAN_POINT('Ctrl Pts',(-2.89311426908746,1.3,11.0146700749867));
#29352=CARTESIAN_POINT('Ctrl Pts',(-2.8917516247831,1.3,11.0139742120426));
#29353=CARTESIAN_POINT('Ctrl Pts',(-2.89040783878869,1.3,11.0132444682025));
#29354=CARTESIAN_POINT('Ctrl Pts',(-2.88907825445049,1.3,11.012522436581));
#29355=CARTESIAN_POINT('Ctrl Pts',(-2.88776741760646,1.3,11.0117668298678));
#29356=CARTESIAN_POINT('Ctrl Pts',(-2.88645763555239,1.3,11.0110094722585));
#29357=CARTESIAN_POINT('Ctrl Pts',(-2.88123035456337,1.3,11.0079868922648));
#29358=CARTESIAN_POINT('Ctrl Pts',(-2.87601819521636,1.3,11.0049389767175));
#29359=CARTESIAN_POINT('Ctrl Pts',(-2.87078275582546,1.3,11.001931888515));
#29360=CARTESIAN_POINT('Ctrl Pts',(-2.86554067077328,1.3,10.9989209832329));
#29361=CARTESIAN_POINT('Ctrl Pts',(-2.86027458446436,1.3,10.9959506173958));
#29362=CARTESIAN_POINT('Ctrl Pts',(-2.85505801286341,1.3,10.992895365571));
#29363=CARTESIAN_POINT('Ctrl Pts',(-2.84469787685817,1.3,10.9868276209185));
#29364=CARTESIAN_POINT('Ctrl Pts',(-2.83453960901062,1.3,10.9804234935907));
#29365=CARTESIAN_POINT('Ctrl Pts',(-2.82438475466521,1.3,10.9740270330777));
#29366=CARTESIAN_POINT('Ctrl Pts',(-2.81424599834958,1.3,10.9676407125833));
#29367=CARTESIAN_POINT('Ctrl Pts',(-2.80410721467228,1.3,10.9612621771574));
#29368=CARTESIAN_POINT('Ctrl Pts',(-2.79396737066265,1.3,10.9548814931131));
#29369=CARTESIAN_POINT('Ctrl Pts',(-2.78889889682822,1.3,10.9516920623789));
#29370=CARTESIAN_POINT('Ctrl Pts',(-2.78382980480467,1.3,10.9485020149995));
#29371=CARTESIAN_POINT('Ctrl Pts',(-2.77880393234839,1.3,10.945245998842));
#29372=CARTESIAN_POINT('Ctrl Pts',(-2.77630166727939,1.3,10.9436249040836));
#29373=CARTESIAN_POINT('Ctrl Pts',(-2.77381000561899,1.3,10.9419876101408));
#29374=CARTESIAN_POINT('Ctrl Pts',(-2.77135220271479,1.3,10.9403007518256));
#29375=CARTESIAN_POINT('Ctrl Pts',(-2.76891140135738,1.3,10.9386255621437));
#29376=CARTESIAN_POINT('Ctrl Pts',(-2.76650454967012,1.3,10.9369011054413));
#29377=CARTESIAN_POINT('Ctrl Pts',(-2.76408805554562,1.3,10.9351916308035));
#29378=CARTESIAN_POINT('Ctrl Pts',(-2.75866098844093,1.3,10.9313524186659));
#29379=CARTESIAN_POINT('Ctrl Pts',(-2.75323113168416,1.3,10.9276119632866));
#29380=CARTESIAN_POINT('Ctrl Pts',(-2.74947315280486,1.3,10.9249974102865));
#29381=CARTESIAN_POINT('Ctrl Pts',(-2.74422322745703,1.3,10.9213448596709));
#29382=CARTESIAN_POINT('Ctrl Pts',(-2.740751784517,1.3,10.9189437652169));
#29383=CARTESIAN_POINT('Ctrl Pts',(-2.73504020153367,1.3,10.9147088809601));
#29384=CARTESIAN_POINT('Ctrl Pts',(-2.73289496744276,1.3,10.9131182854797));
#29385=CARTESIAN_POINT('Ctrl Pts',(-2.73032184179771,1.3,10.9111628383304));
#29386=CARTESIAN_POINT('Ctrl Pts',(-2.72795814059379,1.3,10.9093707518815));
#29387=CARTESIAN_POINT('Ctrl Pts',(-2.720208752911,1.3,10.9034954015496));
#29388=CARTESIAN_POINT('Ctrl Pts',(-2.71325047752261,1.3,10.8984424674216));
#29389=CARTESIAN_POINT('Ctrl Pts',(-2.70549646903679,1.3,10.8957209484761));
#29390=CARTESIAN_POINT('',(-2.5158767249182,1.3,11.0273124987831));
#29391=CARTESIAN_POINT('',(-2.70549646903679,1.3,10.8957209484761));
#29392=CARTESIAN_POINT('',(-2.55655914734361,1.30000000000023,11.321468831149));
#29393=CARTESIAN_POINT('Ctrl Pts',(-2.5158767249182,1.3,11.0273124987831));
#29394=CARTESIAN_POINT('Ctrl Pts',(-2.51547129339445,1.3,11.036054840077));
#29395=CARTESIAN_POINT('Ctrl Pts',(-2.51859198142745,1.30000000000003,11.0479128654031));
#29396=CARTESIAN_POINT('Ctrl Pts',(-2.52296758356098,1.30000000000005,11.0653939986377));
#29397=CARTESIAN_POINT('Ctrl Pts',(-2.5264203539551,1.30000000000005,11.079962490987));
#29398=CARTESIAN_POINT('Ctrl Pts',(-2.53009803158022,1.30000000000008,11.0978064517128));
#29399=CARTESIAN_POINT('Ctrl Pts',(-2.53245235259751,1.30000000000011,11.116187731106));
#29400=CARTESIAN_POINT('Ctrl Pts',(-2.53775258378681,1.30000000000011,11.1397002573066));
#29401=CARTESIAN_POINT('Ctrl Pts',(-2.54008393448627,1.30000000000022,11.1613216668819));
#29402=CARTESIAN_POINT('Ctrl Pts',(-2.54332335680958,1.30000000000025,11.1857521422222));
#29403=CARTESIAN_POINT('Ctrl Pts',(-2.5469023959529,1.30000000000031,11.2100104540124));
#29404=CARTESIAN_POINT('Ctrl Pts',(-2.54938896734332,1.30000000000036,11.2347401697883));
#29405=CARTESIAN_POINT('Ctrl Pts',(-2.55085790609064,1.30000000000038,11.2534406531382));
#29406=CARTESIAN_POINT('Ctrl Pts',(-2.55225517129,1.3000000000004,11.2657217926828));
#29407=CARTESIAN_POINT('Ctrl Pts',(-2.55395665763029,1.30000000000042,11.2810845819828));
#29408=CARTESIAN_POINT('Ctrl Pts',(-2.55505077960984,1.30000000000047,11.2999252661264));
#29409=CARTESIAN_POINT('Ctrl Pts',(-2.55595402588115,1.30000000000049,11.3133566528398));
#29410=CARTESIAN_POINT('Ctrl Pts',(-2.55648845398831,1.30000000000052,11.3205266804514));
#29411=CARTESIAN_POINT('Ctrl Pts',(-2.5565591473374,1.30000000000052,11.3214688310659));
#29412=CARTESIAN_POINT('',(-2.08914039445814,1.29999999999929,11.5769470743903));
#29413=CARTESIAN_POINT('Origin',(0.,1.3,7.2));
#29414=CARTESIAN_POINT('',(-1.87799128879385,1.3,11.3774649241125));
#29415=CARTESIAN_POINT('Ctrl Pts',(-2.08911157607092,1.3,11.5769235068739));
#29416=CARTESIAN_POINT('Ctrl Pts',(-2.03039281675241,1.3,11.5289034585235));
#29417=CARTESIAN_POINT('Ctrl Pts',(-1.97366330051107,1.30000000000335,11.4780295569611));
#29418=CARTESIAN_POINT('Ctrl Pts',(-1.91186458013702,1.30000000000335,11.4120146246155));
#29419=CARTESIAN_POINT('Ctrl Pts',(-1.90903631482672,1.30000000000332,11.4092617389519));
#29420=CARTESIAN_POINT('Ctrl Pts',(-1.8926160488693,1.30000000000332,11.390333398815));
#29421=CARTESIAN_POINT('Ctrl Pts',(-1.88617869194126,1.3,11.3824508078545));
#29422=CARTESIAN_POINT('Ctrl Pts',(-1.87799128879385,1.3,11.3774649241125));
#29423=CARTESIAN_POINT('',(-1.66515576931083,1.3,11.46675672171));
#29424=CARTESIAN_POINT('',(-1.87799128879385,1.3,11.3774649241125));
#29425=CARTESIAN_POINT('',(-1.64379217587214,1.29999999999984,11.7629428313909));
#29426=CARTESIAN_POINT('Ctrl Pts',(-1.66515576931083,1.3,11.46675672171));
#29427=CARTESIAN_POINT('Ctrl Pts',(-1.6629415624785,1.3,11.4752237279177));
#29428=CARTESIAN_POINT('Ctrl Pts',(-1.66352894105859,1.29999999999999,11.4874714735657));
#29429=CARTESIAN_POINT('Ctrl Pts',(-1.66417447630822,1.29999999999996,11.5054803428951));
#29430=CARTESIAN_POINT('Ctrl Pts',(-1.66452301405315,1.29999999999996,11.5204483587987));
#29431=CARTESIAN_POINT('Ctrl Pts',(-1.66441047704251,1.29999999999995,11.5386670191183));
#29432=CARTESIAN_POINT('Ctrl Pts',(-1.66289185486147,1.29999999999991,11.5571361197397));
#29433=CARTESIAN_POINT('Ctrl Pts',(-1.66318775374981,1.29999999999991,11.5812368181191));
#29434=CARTESIAN_POINT('Ctrl Pts',(-1.66097302460095,1.29999999999983,11.6028704763946));
#29435=CARTESIAN_POINT('Ctrl Pts',(-1.65906230940226,1.29999999999982,11.6274406048554));
#29436=CARTESIAN_POINT('Ctrl Pts',(-1.65751962363572,1.29999999999978,11.6519129358666));
#29437=CARTESIAN_POINT('Ctrl Pts',(-1.65481031308637,1.29999999999973,11.6766192287848));
#29438=CARTESIAN_POINT('Ctrl Pts',(-1.65235914007452,1.29999999999972,11.6952164665527));
#29439=CARTESIAN_POINT('Ctrl Pts',(-1.6511724890373,1.29999999999972,11.7075197398047));
#29440=CARTESIAN_POINT('Ctrl Pts',(-1.6496427241954,1.29999999999968,11.7229005682395));
#29441=CARTESIAN_POINT('Ctrl Pts',(-1.64679579483565,1.29999999999966,11.7415570091161));
#29442=CARTESIAN_POINT('Ctrl Pts',(-1.64488682205169,1.29999999999964,11.7548824893073));
#29443=CARTESIAN_POINT('Ctrl Pts',(-1.64391888364001,1.29999999999962,11.7620067583755));
#29444=CARTESIAN_POINT('Ctrl Pts',(-1.64379217588362,1.29999999999962,11.7629428313061));
#29445=CARTESIAN_POINT('Origin',(0.,1.3,7.2));
#29446=CARTESIAN_POINT('Ctrl Pts',(-0.815761714370199,-1.30000000001152,
12.1782561896344));
#29447=CARTESIAN_POINT('Ctrl Pts',(-0.774949037065984,-1.18514270861958,
12.1904765350853));
#29448=CARTESIAN_POINT('Ctrl Pts',(-0.740987950522033,-1.06847604194908,
12.1899531249505));
#29449=CARTESIAN_POINT('Ctrl Pts',(-0.678359592026837,-0.794772684000851,
12.1593033180494));
#29450=CARTESIAN_POINT('Ctrl Pts',(-0.662111769290086,-0.636309800095197,
12.0912247185297));
#29451=CARTESIAN_POINT('Ctrl Pts',(-0.623796234000798,-0.319434907277159,
12.0277447643888));
#29452=CARTESIAN_POINT('Ctrl Pts',(-0.614857791974962,-0.158333333333332,
11.9827589718232));
#29453=CARTESIAN_POINT('Ctrl Pts',(-0.581221077760458,0.158333333333334,
11.9868187308147));
#29454=CARTESIAN_POINT('Ctrl Pts',(-0.55498717214331,0.319434907277167,
12.0359668790066));
#29455=CARTESIAN_POINT('Ctrl Pts',(-0.527915117225984,0.636309800095206,
12.1075072879431));
#29456=CARTESIAN_POINT('Ctrl Pts',(-0.508441992410805,0.79477268400084,
12.1792483945391));
#29457=CARTESIAN_POINT('Ctrl Pts',(-0.5254047727039,1.06847604194527,12.2173269808048));
#29458=CARTESIAN_POINT('Ctrl Pts',(-0.542940786614001,1.1851427086121,12.2211942845391));
#29459=CARTESIAN_POINT('Ctrl Pts',(-0.570670255378274,1.30000000000048,
12.2124460829639));
#29460=CARTESIAN_POINT('Ctrl Pts',(-0.82013686250475,-1.30000000001152,
12.1665018705585));
#29461=CARTESIAN_POINT('Ctrl Pts',(-0.780090946642151,-1.18514270861958,
12.1764721061336));
#29462=CARTESIAN_POINT('Ctrl Pts',(-0.746715246716433,-1.06847604194908,
12.1743051424724));
#29463=CARTESIAN_POINT('Ctrl Pts',(-0.685020236289605,-0.794772684000851,
12.141259664642));
#29464=CARTESIAN_POINT('Ctrl Pts',(-0.66882498757232,-0.636309800095197,
12.0736176643627));
#29465=CARTESIAN_POINT('Ctrl Pts',(-0.630650969306314,-0.319434907277159,
12.0100782700739));
#29466=CARTESIAN_POINT('Ctrl Pts',(-0.621210414483327,-0.158333333333332,
11.9658130254479));
#29467=CARTESIAN_POINT('Ctrl Pts',(-0.588041432022333,0.158333333333334,
11.9699175322922));
#29468=CARTESIAN_POINT('Ctrl Pts',(-0.562926419586644,0.319434907277167,
12.0183993675339));
#29469=CARTESIAN_POINT('Ctrl Pts',(-0.53636198222106,0.636309800095206,
12.0900710401584));
#29470=CARTESIAN_POINT('Ctrl Pts',(-0.517059899028168,0.79477268400084,
12.161414267525));
#29471=CARTESIAN_POINT('Ctrl Pts',(-0.533012642916803,1.06847604194527,
12.2018952309815));
#29472=CARTESIAN_POINT('Ctrl Pts',(-0.54980559533789,1.1851427086121,12.2073958498195));
#29473=CARTESIAN_POINT('Ctrl Pts',(-0.576486148458089,1.30000000000048,
12.2008743783825));
#29474=CARTESIAN_POINT('Ctrl Pts',(-0.828301885813206,-1.3000000000115,
12.1430419168349));
#29475=CARTESIAN_POINT('Ctrl Pts',(-0.791470154233991,-1.18514270861957,
12.148526329752));
#29476=CARTESIAN_POINT('Ctrl Pts',(-0.760221087829436,-1.06847604194906,
12.1430741928524));
#29477=CARTESIAN_POINT('Ctrl Pts',(-0.700926566443512,-0.794772684000842,
12.1052130479931));
#29478=CARTESIAN_POINT('Ctrl Pts',(-0.682086780735323,-0.636309800095188,
12.0383657208095));
#29479=CARTESIAN_POINT('Ctrl Pts',(-0.643454278021432,-0.319434907277154,
11.9746814174566));
#29480=CARTESIAN_POINT('Ctrl Pts',(-0.634003199425879,-0.15833333333333,
11.9319085201582));
#29481=CARTESIAN_POINT('Ctrl Pts',(-0.601473370738099,0.158333333333332,
11.9360713376515));
#29482=CARTESIAN_POINT('Ctrl Pts',(-0.57745577938292,0.319434907277162,
11.9831275324594));
#29483=CARTESIAN_POINT('Ctrl Pts',(-0.551739715339017,0.636309800095197,
12.0550457861955));
#29484=CARTESIAN_POINT('Ctrl Pts',(-0.533839936831245,0.794772684000831,
12.1256672596271));
#29485=CARTESIAN_POINT('Ctrl Pts',(-0.547735885685927,1.06847604194526,
12.1709700838584));
#29486=CARTESIAN_POINT('Ctrl Pts',(-0.562829352204696,1.18514270861208,
12.1797357114804));
#29487=CARTESIAN_POINT('Ctrl Pts',(-0.587001243878688,1.30000000000045,
12.1776570527497));
#29488=CARTESIAN_POINT('Ctrl Pts',(-0.836707147794769,-1.30000000001149,
12.1192702708369));
#29489=CARTESIAN_POINT('Ctrl Pts',(-0.80043188440398,-1.18514270861956,
12.1201835583254));
#29490=CARTESIAN_POINT('Ctrl Pts',(-0.769771336481297,-1.06847604194905,
12.1113955021284));
#29491=CARTESIAN_POINT('Ctrl Pts',(-0.711910453110691,-0.794772684000834,
12.068681289609));
#29492=CARTESIAN_POINT('Ctrl Pts',(-0.694489271114953,-0.636309800095183,
12.0027480164002));
#29493=CARTESIAN_POINT('Ctrl Pts',(-0.656588678792395,-0.319434907277153,
11.9389505469321));
#29494=CARTESIAN_POINT('Ctrl Pts',(-0.64612829689688,-0.158333333333329,
11.8976409947032));
#29495=CARTESIAN_POINT('Ctrl Pts',(-0.614289353194816,0.15833333333333,
11.9018599735325));
#29496=CARTESIAN_POINT('Ctrl Pts',(-0.591653888851498,0.319434907277157,
11.9474876088037));
#29497=CARTESIAN_POINT('Ctrl Pts',(-0.567261065300381,0.636309800095191,
12.0196769662247));
#29498=CARTESIAN_POINT('Ctrl Pts',(-0.551340534525828,0.794772684000825,
12.0895982646898));
#29499=CARTESIAN_POINT('Ctrl Pts',(-0.563310045646076,1.06847604194525,
12.139782144358));
#29500=CARTESIAN_POINT('Ctrl Pts',(-0.576630193529321,1.18514270861207,
12.1518448274832));
#29501=CARTESIAN_POINT('Ctrl Pts',(-0.598089331445952,1.30000000000045,
12.1542474517214));
#29502=CARTESIAN_POINT('Ctrl Pts',(-0.840896249733202,-1.30000000001149,
12.1071345222084));
#29503=CARTESIAN_POINT('Ctrl Pts',(-0.80590565072756,-1.18514270861955,
12.1057161795362));
#29504=CARTESIAN_POINT('Ctrl Pts',(-0.776118041671117,-1.06847604194905,
12.0952223523448));
#29505=CARTESIAN_POINT('Ctrl Pts',(-0.719322653398249,-0.794772684000831,
12.0500133274667));
#29506=CARTESIAN_POINT('Ctrl Pts',(-0.701147360363495,-0.636309800095182,
11.9845133106775));
#29507=CARTESIAN_POINT('Ctrl Pts',(-0.662937063965583,-0.319434907277152,
11.9206373392581));
#29508=CARTESIAN_POINT('Ctrl Pts',(-0.651850096865466,-0.158333333333328,
11.880076238071));
#29509=CARTESIAN_POINT('Ctrl Pts',(-0.620348320308299,0.15833333333333,
11.8843214312355));
#29510=CARTESIAN_POINT('Ctrl Pts',(-0.598936484134056,0.319434907277156,
11.929235417687));
#29511=CARTESIAN_POINT('Ctrl Pts',(-0.575010801522814,0.636309800095188,
12.0015391808645));
#29512=CARTESIAN_POINT('Ctrl Pts',(-0.559119512271139,0.794772684000824,
12.0710311232064));
#29513=CARTESIAN_POINT('Ctrl Pts',(-0.57010620639343,1.06847604194525,12.1237185482583));
#29514=CARTESIAN_POINT('Ctrl Pts',(-0.582732606004582,1.18514270861207,
12.1374883996074));
#29515=CARTESIAN_POINT('Ctrl Pts',(-0.60322967243848,1.30000000000044,12.1422216682623));
#29516=CARTESIAN_POINT('Ctrl Pts',(-0.84108366557138,-1.30000000001149,
12.106582879579));
#29517=CARTESIAN_POINT('Ctrl Pts',(-0.806151169153311,-1.18514270861955,
12.1050584818237));
#29518=CARTESIAN_POINT('Ctrl Pts',(-0.776403200212559,-1.06847604194905,
12.0944870720756));
#29519=CARTESIAN_POINT('Ctrl Pts',(-0.719656736533463,-0.794772684000831,
12.0491645932037));
#29520=CARTESIAN_POINT('Ctrl Pts',(-0.701449230989593,-0.636309800095182,
11.9836843524763));
#29521=CARTESIAN_POINT('Ctrl Pts',(-0.663224451229675,-0.319434907277152,
11.9198047781588));
#29522=CARTESIAN_POINT('Ctrl Pts',(-0.652106150378969,-0.158333333333328,
11.8792775941036));
#29523=CARTESIAN_POINT('Ctrl Pts',(-0.62061947737185,0.15833333333333,11.8835239547376));
#29524=CARTESIAN_POINT('Ctrl Pts',(-0.599265114264511,0.319434907277156,
11.9284055424065));
#29525=CARTESIAN_POINT('Ctrl Pts',(-0.575362200797949,0.636309800095188,
12.0007145718174));
#29526=CARTESIAN_POINT('Ctrl Pts',(-0.559473301158497,0.794772684000824,
12.07018707444));
#29527=CARTESIAN_POINT('Ctrl Pts',(-0.570415763160731,1.06847604194525,
12.1229883507983));
#29528=CARTESIAN_POINT('Ctrl Pts',(-0.583010559332848,1.18514270861207,
12.1368358144636));
#29529=CARTESIAN_POINT('Ctrl Pts',(-0.603463565334488,1.30000000000044,
12.1416750257389));
#29530=CARTESIAN_POINT('Ctrl Pts',(-0.841271106653579,-1.30000000001149,
12.1060312225867));
#29531=CARTESIAN_POINT('Ctrl Pts',(-0.806396138358098,-1.18514270861955,
12.1044007736908));
#29532=CARTESIAN_POINT('Ctrl Pts',(-0.776687427737685,-1.06847604194905,
12.0937517836326));
#29533=CARTESIAN_POINT('Ctrl Pts',(-0.719989451734108,-0.794772684000831,
12.0483158520383));
#29534=CARTESIAN_POINT('Ctrl Pts',(-0.701749841759635,-0.636309800095182,
11.9828553699663));
#29535=CARTESIAN_POINT('Ctrl Pts',(-0.66351134192088,-0.319434907277152,
11.9189722126188));
#29536=CARTESIAN_POINT('Ctrl Pts',(-0.652363265515954,-0.158333333333328,
11.8784790007643));
#29537=CARTESIAN_POINT('Ctrl Pts',(-0.620891783947901,0.15833333333333,
11.8827265264074));
#29538=CARTESIAN_POINT('Ctrl Pts',(-0.599593227881866,0.319434907277156,
11.9275756469084));
#29539=CARTESIAN_POINT('Ctrl Pts',(-0.575712897964395,0.636309800095188,
11.9998899397845));
#29540=CARTESIAN_POINT('Ctrl Pts',(-0.559827649734273,0.794772684000824,
12.06934306953));
#29541=CARTESIAN_POINT('Ctrl Pts',(-0.570726051352478,1.06847604194525,
12.1222582011948));
#29542=CARTESIAN_POINT('Ctrl Pts',(-0.583289129579976,1.18514270861207,
12.1361832670831));
#29543=CARTESIAN_POINT('Ctrl Pts',(-0.603697771800025,1.30000000000044,
12.141128399061));
#29544=CARTESIAN_POINT('Ctrl Pts',(-0.8416433382849,-1.30000000001149,12.1049278686445));
#29545=CARTESIAN_POINT('Ctrl Pts',(-0.806882159906077,-1.18514270861955,
12.1030852573022));
#29546=CARTESIAN_POINT('Ctrl Pts',(-0.777251289156161,-1.06847604194905,
12.0922810672687));
#29547=CARTESIAN_POINT('Ctrl Pts',(-0.720650087026833,-0.794772684000831,
12.0466181873869));
#29548=CARTESIAN_POINT('Ctrl Pts',(-0.702348630569117,-0.636309800095182,
11.981197280085));
#29549=CARTESIAN_POINT('Ctrl Pts',(-0.66408356520117,-0.319434907277152,
11.9173069588674));
#29550=CARTESIAN_POINT('Ctrl Pts',(-0.652875601867588,-0.158333333333328,
11.8768816785607));
#29551=CARTESIAN_POINT('Ctrl Pts',(-0.621434367058539,0.15833333333333,
11.8811315066939));
#29552=CARTESIAN_POINT('Ctrl Pts',(-0.600246478406182,0.319434907277156,
11.9259156187069));
#29553=CARTESIAN_POINT('Ctrl Pts',(-0.576412498766739,0.636309800095188,
11.998240501404));
#29554=CARTESIAN_POINT('Ctrl Pts',(-0.560537751889447,0.794772684000824,
12.0676550804845));
#29555=CARTESIAN_POINT('Ctrl Pts',(-0.571348643291286,1.06847604194525,
12.1207979754241));
#29556=CARTESIAN_POINT('Ctrl Pts',(-0.583847946343261,1.18514270861207,
12.1348782360536));
#29557=CARTESIAN_POINT('Ctrl Pts',(-0.604166918142359,1.30000000000044,
12.1400351672316));
#29558=CARTESIAN_POINT('Ctrl Pts',(-0.842440411811635,-1.30000000001149,
12.1025370321507));
#29559=CARTESIAN_POINT('Ctrl Pts',(-0.807917893314191,-1.18514270861955,
12.1002345213527));
#29560=CARTESIAN_POINT('Ctrl Pts',(-0.778451084354395,-1.06847604194905,
12.0890939250708));
#29561=CARTESIAN_POINT('Ctrl Pts',(-0.722056561266581,-0.794772684000831,
12.0429391734713));
#29562=CARTESIAN_POINT('Ctrl Pts',(-0.703631014770677,-0.636309800095182,
11.9776041650572));
#29563=CARTESIAN_POINT('Ctrl Pts',(-0.665315562999388,-0.319434907277152,
11.9136984391799));
#29564=CARTESIAN_POINT('Ctrl Pts',(-0.653984050577437,-0.158333333333328,
11.8734205623712));
#29565=CARTESIAN_POINT('Ctrl Pts',(-0.622608333470667,0.15833333333333,
11.8776752669074));
#29566=CARTESIAN_POINT('Ctrl Pts',(-0.60164873732673,0.319434907277157,
11.9223179126499));
#29567=CARTESIAN_POINT('Ctrl Pts',(-0.577918698969977,0.636309800095188,
11.9946659720654));
#29568=CARTESIAN_POINT('Ctrl Pts',(-0.562084540976334,0.794772684000824,
12.0639981026217));
#29569=CARTESIAN_POINT('Ctrl Pts',(-0.572709027367301,1.06847604194525,
12.1176347043536));
#29570=CARTESIAN_POINT('Ctrl Pts',(-0.58506843023964,1.18514270861207,12.13205113149));
#29571=CARTESIAN_POINT('Ctrl Pts',(-0.605188289501683,1.30000000000044,
12.1376666883049));
#29572=CARTESIAN_POINT('Ctrl Pts',(-0.8436279850576,-1.30000000001149,12.098857420753));
#29573=CARTESIAN_POINT('Ctrl Pts',(-0.8094239679675,-1.18514270861955,12.0958463896222));
#29574=CARTESIAN_POINT('Ctrl Pts',(-0.780181208795663,-1.06847604194905,
12.0841876400619));
#29575=CARTESIAN_POINT('Ctrl Pts',(-0.724086083403273,-0.794772684000831,
12.0372756367114));
#29576=CARTESIAN_POINT('Ctrl Pts',(-0.705529966296978,-0.636309800095182,
11.9720736371635));
#29577=CARTESIAN_POINT('Ctrl Pts',(-0.667182604758452,-0.319434907277152,
11.9081451757437));
#29578=CARTESIAN_POINT('Ctrl Pts',(-0.655703716817061,-0.158333333333328,
11.8680957195148));
#29579=CARTESIAN_POINT('Ctrl Pts',(-0.624426688156065,0.15833333333333,
11.872357314027));
#29580=CARTESIAN_POINT('Ctrl Pts',(-0.603741085139811,0.319434907277157,
11.9167783358466));
#29581=CARTESIAN_POINT('Ctrl Pts',(-0.580187088115549,0.636309800095188,
11.9891633552736));
#29582=CARTESIAN_POINT('Ctrl Pts',(-0.564525011791283,0.794772684000824,
12.0583754013928));
#29583=CARTESIAN_POINT('Ctrl Pts',(-0.574876802233916,1.06847604194525,
12.1127725326272));
#29584=CARTESIAN_POINT('Ctrl Pts',(-0.587007286654078,1.18514270861207,
12.1277053380453));
#29585=CARTESIAN_POINT('Ctrl Pts',(-0.606787348983421,1.30000000000044,
12.1340244463825));
#29586=CARTESIAN_POINT('Ctrl Pts',(-0.844998182644887,-1.30000000001148,
12.0944389846615));
#29587=CARTESIAN_POINT('Ctrl Pts',(-0.81108280355128,-1.18514270861955,
12.090576012288));
#29588=CARTESIAN_POINT('Ctrl Pts',(-0.782053207345806,-1.06847604194905,
12.0782944298942));
#29589=CARTESIAN_POINT('Ctrl Pts',(-0.726276168630486,-0.794772684000832,
12.0304728443595));
#29590=CARTESIAN_POINT('Ctrl Pts',(-0.707666075200391,-0.636309800095182,
11.9654317870864));
#29591=CARTESIAN_POINT('Ctrl Pts',(-0.669369958673357,-0.319434907277152,
11.9014782233589));
#29592=CARTESIAN_POINT('Ctrl Pts',(-0.65781344964472,-0.158333333333328,
11.8617068390375));
#29593=CARTESIAN_POINT('Ctrl Pts',(-0.626654186829892,0.15833333333333,
11.8659756293417));
#29594=CARTESIAN_POINT('Ctrl Pts',(-0.606142384063235,0.319434907277157,
11.9101225137041));
#29595=CARTESIAN_POINT('Ctrl Pts',(-0.582820993097351,0.636309800095189,
11.982553935868));
#29596=CARTESIAN_POINT('Ctrl Pts',(-0.567560619655728,0.794772684000824,
12.0516344476837));
#29597=CARTESIAN_POINT('Ctrl Pts',(-0.577613545939296,1.06847604194525,
12.1069460957049));
#29598=CARTESIAN_POINT('Ctrl Pts',(-0.589447841868061,1.18514270861207,
12.1224971408499));
#29599=CARTESIAN_POINT('Ctrl Pts',(-0.608764894435061,1.30000000000044,
12.1296568682101));
#29600=CARTESIAN_POINT('Ctrl Pts',(-0.846782212613889,-1.30000000001149,
12.0885449248653));
#29601=CARTESIAN_POINT('Ctrl Pts',(-0.813168584017232,-1.18514270861955,
12.0835445222219));
#29602=CARTESIAN_POINT('Ctrl Pts',(-0.784372570115393,-1.06847604194905,
12.0704315727545));
#29603=CARTESIAN_POINT('Ctrl Pts',(-0.728977671085883,-0.794772684000831,
12.0213964301765));
#29604=CARTESIAN_POINT('Ctrl Pts',(-0.710379940056297,-0.636309800095182,
11.9565711544317));
#29605=CARTESIAN_POINT('Ctrl Pts',(-0.672221392006236,-0.319434907277152,
11.8925859612815));
#29606=CARTESIAN_POINT('Ctrl Pts',(-0.660639528873272,-0.158333333333328,
11.8531887947527));
#29607=CARTESIAN_POINT('Ctrl Pts',(-0.629635528222297,0.15833333333333,
11.8574659748541));
#29608=CARTESIAN_POINT('Ctrl Pts',(-0.609228998788056,0.319434907277157,
11.9012398803746));
#29609=CARTESIAN_POINT('Ctrl Pts',(-0.586239765328994,0.636309800095188,
11.9737345871329));
#29610=CARTESIAN_POINT('Ctrl Pts',(-0.571684072982041,0.794772684000824,
12.0426503161413));
#29611=CARTESIAN_POINT('Ctrl Pts',(-0.581362316142963,1.06847604194525,
12.0991830970244));
#29612=CARTESIAN_POINT('Ctrl Pts',(-0.592782232184672,1.18514270861207,
12.1155574251084));
#29613=CARTESIAN_POINT('Ctrl Pts',(-0.611432711417976,1.30000000000044,
12.1238351351779));
#29614=CARTESIAN_POINT('Ctrl Pts',(-0.849022524491501,-1.30000000001149,
12.0811753213131));
#29615=CARTESIAN_POINT('Ctrl Pts',(-0.815790792839271,-1.18514270861955,
12.0747521792439));
#29616=CARTESIAN_POINT('Ctrl Pts',(-0.7872803364692,-1.06847604194905,12.0605992294231));
#29617=CARTESIAN_POINT('Ctrl Pts',(-0.732322569147779,-0.794772684000832,
12.0100456818012));
#29618=CARTESIAN_POINT('Ctrl Pts',(-0.713659524061526,-0.636309800095182,
11.9454896346112));
#29619=CARTESIAN_POINT('Ctrl Pts',(-0.675628672060576,-0.319434907277152,
11.881464252745));
#29620=CARTESIAN_POINT('Ctrl Pts',(-0.664012556063606,-0.158333333333328,
11.8425350941018));
#29621=CARTESIAN_POINT('Ctrl Pts',(-0.633230004184434,0.15833333333333,
11.8468222411214));
#29622=CARTESIAN_POINT('Ctrl Pts',(-0.613036617821267,0.319434907277157,
11.890130257037));
#29623=CARTESIAN_POINT('Ctrl Pts',(-0.590457452248467,0.636309800095189,
11.9627014415155));
#29624=CARTESIAN_POINT('Ctrl Pts',(-0.576648844760399,0.794772684000824,
12.0314043836306));
#29625=CARTESIAN_POINT('Ctrl Pts',(-0.585895284402455,1.06847604194525,
12.0894658356194));
#29626=CARTESIAN_POINT('Ctrl Pts',(-0.596847578942501,1.18514270861207,
12.1068723220005));
#29627=CARTESIAN_POINT('Ctrl Pts',(-0.614749726915899,1.30000000000044,
12.1165526435854));
#29628=CARTESIAN_POINT('Ctrl Pts',(-0.852869513329444,-1.30000000001149,
12.0693893749476));
#29629=CARTESIAN_POINT('Ctrl Pts',(-0.820647185601926,-1.18514270861956,
12.0606941221766));
#29630=CARTESIAN_POINT('Ctrl Pts',(-0.792815469737626,-1.06847604194905,
12.0448792800955));
#29631=CARTESIAN_POINT('Ctrl Pts',(-0.738661830119352,-0.794772684000832,
11.9918961555659));
#29632=CARTESIAN_POINT('Ctrl Pts',(-0.719381690621249,-0.636309800095182,
11.927765607536));
#29633=CARTESIAN_POINT('Ctrl Pts',(-0.681009666211855,-0.319434907277152,
11.8636640896346));
#29634=CARTESIAN_POINT('Ctrl Pts',(-0.668721509130177,-0.158333333333328,
11.8254656175414));
#29635=CARTESIAN_POINT('Ctrl Pts',(-0.638266505472543,0.15833333333333,
11.8297692452917));
#29636=CARTESIAN_POINT('Ctrl Pts',(-0.619251838548418,0.319434907277157,
11.8723633623647));
#29637=CARTESIAN_POINT('Ctrl Pts',(-0.597316162344372,0.636309800095189,
11.9450436276509));
#29638=CARTESIAN_POINT('Ctrl Pts',(-0.583841371506697,0.794772684000823,
12.0133455370274));
#29639=CARTESIAN_POINT('Ctrl Pts',(-0.59230706893329,1.06847604194525,12.0738508224656));
#29640=CARTESIAN_POINT('Ctrl Pts',(-0.602621019135524,1.18514270861207,
12.0929205048113));
#29641=CARTESIAN_POINT('Ctrl Pts',(-0.619584432809021,1.30000000000044,
12.1048693733783));
#29642=CARTESIAN_POINT('Ctrl Pts',(-0.857756263455172,-1.30000000001149,
12.0546463002434));
#29643=CARTESIAN_POINT('Ctrl Pts',(-0.826777915563002,-1.18514270861955,
12.0431077053763));
#29644=CARTESIAN_POINT('Ctrl Pts',(-0.799791193187777,-1.06847604194905,
12.0252135500953));
#29645=CARTESIAN_POINT('Ctrl Pts',(-0.746667919292781,-0.794772684000831,
11.9691918557023));
#29646=CARTESIAN_POINT('Ctrl Pts',(-0.726684243680441,-0.636309800095182,
11.9055952862092));
#29647=CARTESIAN_POINT('Ctrl Pts',(-0.687953766670922,-0.319434907277152,
11.8414036063792));
#29648=CARTESIAN_POINT('Ctrl Pts',(-0.674928204569495,-0.158333333333329,
11.8041281373097));
#29649=CARTESIAN_POINT('Ctrl Pts',(-0.644786943020532,0.15833333333333,
11.8084501671754));
#29650=CARTESIAN_POINT('Ctrl Pts',(-0.626886079124035,0.319434907277158,
11.8501324015904));
#29651=CARTESIAN_POINT('Ctrl Pts',(-0.605820300049983,0.63630980009519,
11.9229551449895));
#29652=CARTESIAN_POINT('Ctrl Pts',(-0.593236695086667,0.794772684000823,
11.9907870809948));
#29653=CARTESIAN_POINT('Ctrl Pts',(-0.600902941546169,1.06847604194525,
12.0543534139577));
#29654=CARTESIAN_POINT('Ctrl Pts',(-0.610435718320796,1.18514270861207,
12.0754994900718));
#29655=CARTESIAN_POINT('Ctrl Pts',(-0.626182837840153,1.30000000000045,
12.090276132125));
#29656=CARTESIAN_POINT('Ctrl Pts',(-0.864644628449034,-1.3000000000115,
12.0310472553246));
#29657=CARTESIAN_POINT('Ctrl Pts',(-0.834955202509833,-1.18514270861956,
12.0149459412788));
#29658=CARTESIAN_POINT('Ctrl Pts',(-0.808856027738995,-1.06847604194906,
11.9937159067301));
#29659=CARTESIAN_POINT('Ctrl Pts',(-0.756855911323515,-0.794772684000833,
11.9328219095113));
#29660=CARTESIAN_POINT('Ctrl Pts',(-0.736034398151118,-0.636309800095184,
11.870088231716));
#29661=CARTESIAN_POINT('Ctrl Pts',(-0.697391884991225,-0.319434907277153,
11.8057563938321));
#29662=CARTESIAN_POINT('Ctrl Pts',(-0.684176003430856,-0.158333333333329,
11.7699635731805));
#29663=CARTESIAN_POINT('Ctrl Pts',(-0.655128309893531,0.158333333333331,
11.7743144927794));
#29664=CARTESIAN_POINT('Ctrl Pts',(-0.639098183310164,0.319434907277159,
11.8145449842146));
#29665=CARTESIAN_POINT('Ctrl Pts',(-0.618976588811999,0.636309800095192,
11.8875626261278));
#29666=CARTESIAN_POINT('Ctrl Pts',(-0.606686062383306,0.794772684000826,
11.9545666974269));
#29667=CARTESIAN_POINT('Ctrl Pts',(-0.612704837274032,1.06847604194525,
12.0230303781235));
#29668=CARTESIAN_POINT('Ctrl Pts',(-0.62101138188125,1.18514270861208,12.0475164781124));
#29669=CARTESIAN_POINT('Ctrl Pts',(-0.635019166463077,1.30000000000045,
12.066853287546));
#29670=CARTESIAN_POINT('Ctrl Pts',(-0.871823313020447,-1.3000000000115,
12.0074165305344));
#29671=CARTESIAN_POINT('Ctrl Pts',(-0.843419365115712,-1.18514270861956,
11.9867520917804));
#29672=CARTESIAN_POINT('Ctrl Pts',(-0.818264588190346,-1.06847604194906,
11.9621852591644));
#29673=CARTESIAN_POINT('Ctrl Pts',(-0.767658256254581,-0.794772684000836,
11.896415650752));
#29674=CARTESIAN_POINT('Ctrl Pts',(-0.746661656345003,-0.636309800095187,
11.8345383396903));
#29675=CARTESIAN_POINT('Ctrl Pts',(-0.708018162750769,-0.319434907277156,
11.7700665973413));
#29676=CARTESIAN_POINT('Ctrl Pts',(-0.694138943110603,-0.15833333333333,
11.7357745430453));
#29677=CARTESIAN_POINT('Ctrl Pts',(-0.665269484383368,0.158333333333332,
11.7401347217955));
#29678=CARTESIAN_POINT('Ctrl Pts',(-0.649849813569892,0.319434907277161,
11.7788574661797));
#29679=CARTESIAN_POINT('Ctrl Pts',(-0.630563019913342,0.636309800095195,
11.8520669521813));
#29680=CARTESIAN_POINT('Ctrl Pts',(-0.619731947798664,0.794772684000831,
11.9182908531853));
#29681=CARTESIAN_POINT('Ctrl Pts',(-0.624903674483712,1.06847604194526,
11.9916814007995));
#29682=CARTESIAN_POINT('Ctrl Pts',(-0.63229108230308,1.18514270861208,12.0195178447586));
#29683=CARTESIAN_POINT('Ctrl Pts',(-0.644827249091217,1.30000000000046,
12.0434226840024));
#29684=CARTESIAN_POINT('Ctrl Pts',(-0.878501924149539,-1.3000000000115,
11.9837919824015));
#29685=CARTESIAN_POINT('Ctrl Pts',(-0.851593849899919,-1.18514270861957,
11.9585435767857));
#29686=CARTESIAN_POINT('Ctrl Pts',(-0.827318970973691,-1.06847604194906,
11.9306273219391));
#29687=CARTESIAN_POINT('Ctrl Pts',(-0.777322352448109,-0.794772684000837,
11.8599719231924));
#29688=CARTESIAN_POINT('Ctrl Pts',(-0.754045433093823,-0.636309800095185,
11.7989833086607));
#29689=CARTESIAN_POINT('Ctrl Pts',(-0.715008483530921,-0.319434907277153,
11.7343686089337));
#29690=CARTESIAN_POINT('Ctrl Pts',(-0.701574831806603,-0.158333333333329,
11.7015525526237));
#29691=CARTESIAN_POINT('Ctrl Pts',(-0.673894849027944,0.158333333333331,
11.7059103525462));
#29692=CARTESIAN_POINT('Ctrl Pts',(-0.65976531894143,0.319434907277161,
11.7431259723976));
#29693=CARTESIAN_POINT('Ctrl Pts',(-0.642182221447585,0.636309800095194,
11.8165321273102));
#29694=CARTESIAN_POINT('Ctrl Pts',(-0.633533642865829,0.794772684000825,
11.8819903817194));
#29695=CARTESIAN_POINT('Ctrl Pts',(-0.637513538252151,1.06847604194525,
11.9603096822764));
#29696=CARTESIAN_POINT('Ctrl Pts',(-0.643530336300666,1.18514270861208,
11.9914944048591));
#29697=CARTESIAN_POINT('Ctrl Pts',(-0.653841183154614,1.30000000000046,
12.0199623268296));
#29698=CARTESIAN_POINT('Ctrl Pts',(-0.883557620031031,-1.3000000000115,
11.9660343263365));
#29699=CARTESIAN_POINT('Ctrl Pts',(-0.856845494787491,-1.18514270861957,
11.9373706087656));
#29700=CARTESIAN_POINT('Ctrl Pts',(-0.832849332419673,-1.06847604194906,
11.9069544151971));
#29701=CARTESIAN_POINT('Ctrl Pts',(-0.78368781450453,-0.794772684000841,
11.8326383531807));
#29702=CARTESIAN_POINT('Ctrl Pts',(-0.761796018154491,-0.63630980009519,
11.7722658357778));
#29703=CARTESIAN_POINT('Ctrl Pts',(-0.722736188073244,-0.319434907277156,
11.7075445931099));
#29704=CARTESIAN_POINT('Ctrl Pts',(-0.707613932029028,-0.158333333333331,
11.6758783453701));
#29705=CARTESIAN_POINT('Ctrl Pts',(-0.679765481684038,0.158333333333332,
11.6802412589297));
#29706=CARTESIAN_POINT('Ctrl Pts',(-0.666795618498137,0.319434907277163,
11.7163157384279));
#29707=CARTESIAN_POINT('Ctrl Pts',(-0.649626496355868,0.636309800095198,
11.7898316119687));
#29708=CARTESIAN_POINT('Ctrl Pts',(-0.64091936790216,0.794772684000834,
11.8546401172946));
#29709=CARTESIAN_POINT('Ctrl Pts',(-0.644477404575823,1.06847604194526,
11.936664901596));
#29710=CARTESIAN_POINT('Ctrl Pts',(-0.650189127781039,1.18514270861208,
11.9703850564661));
#29711=CARTESIAN_POINT('Ctrl Pts',(-0.66007243195369,1.30000000000046,12.0023198763999));
#29712=CARTESIAN_POINT('Ctrl Pts',(-0.887281295441576,-1.3000000000115,
11.9483568191932));
#29713=CARTESIAN_POINT('Ctrl Pts',(-0.861806181848091,-1.18514270861957,
11.9162326705626));
#29714=CARTESIAN_POINT('Ctrl Pts',(-0.838516494444084,-1.06847604194906,
11.8832903206437));
#29715=CARTESIAN_POINT('Ctrl Pts',(-0.789761429146444,-0.79477268400084,
11.8052966935815));
#29716=CARTESIAN_POINT('Ctrl Pts',(-0.765800673218215,-0.636309800095188,
11.7456175979226));
#29717=CARTESIAN_POINT('Ctrl Pts',(-0.726343628275416,-0.319434907277154,
11.6807914709022));
#29718=CARTESIAN_POINT('Ctrl Pts',(-0.711403458489195,-0.15833333333333,
11.6502281095496));
#29719=CARTESIAN_POINT('Ctrl Pts',(-0.685078224489192,0.158333333333332,
11.6545703789146));
#29720=CARTESIAN_POINT('Ctrl Pts',(-0.674269857923319,0.319434907277163,
11.6894882681703));
#29721=CARTESIAN_POINT('Ctrl Pts',(-0.658929605102686,0.636309800095197,
11.7631343154741));
#29722=CARTESIAN_POINT('Ctrl Pts',(-0.651505739224311,0.794772684000829,
11.8273679692787));
#29723=CARTESIAN_POINT('Ctrl Pts',(-0.653946884062025,1.06847604194526,
11.9130946810947));
#29724=CARTESIAN_POINT('Ctrl Pts',(-0.658499180558779,1.18514270861208,
11.9493313800572));
#29725=CARTESIAN_POINT('Ctrl Pts',(-0.666547092405371,1.30000000000046,
11.9846968609247));
#29726=CARTESIAN_POINT('Ctrl Pts',(-0.892703441219226,-1.30000000001151,
11.9305719471507));
#29727=CARTESIAN_POINT('Ctrl Pts',(-0.867861945427389,-1.18514270861957,
11.8950149270867));
#29728=CARTESIAN_POINT('Ctrl Pts',(-0.844983347403223,-1.06847604194906,
11.859564292742));
#29729=CARTESIAN_POINT('Ctrl Pts',(-0.796663895640123,-0.794772684000841,
11.7779120078267));
#29730=CARTESIAN_POINT('Ctrl Pts',(-0.772227335557577,-0.636309800095189,
11.7188940920834));
#29731=CARTESIAN_POINT('Ctrl Pts',(-0.732424394074677,-0.319434907277156,
11.6539705401567));
#29732=CARTESIAN_POINT('Ctrl Pts',(-0.717112193228731,-0.158333333333331,
11.6245378964453));
#29733=CARTESIAN_POINT('Ctrl Pts',(-0.690622206064707,0.158333333333332,
11.6288726611887));
#29734=CARTESIAN_POINT('Ctrl Pts',(-0.679713770617353,0.319434907277163,
11.6626385810088));
#29735=CARTESIAN_POINT('Ctrl Pts',(-0.66500986725975,0.636309800095199,
11.7363947688458));
#29736=CARTESIAN_POINT('Ctrl Pts',(-0.659065939520507,0.794772684000833,
11.7999938191272));
#29737=CARTESIAN_POINT('Ctrl Pts',(-0.661570434056588,1.06847604194526,
11.8894333440492));
#29738=CARTESIAN_POINT('Ctrl Pts',(-0.665813828387652,1.18514270861208,
11.9282072795572));
#29739=CARTESIAN_POINT('Ctrl Pts',(-0.673216514165779,1.30000000000046,
11.9670400942955));
#29740=CARTESIAN_POINT('Ctrl Pts',(-0.894984307098906,-1.3000000000115,
11.9158592698447));
#29741=CARTESIAN_POINT('Ctrl Pts',(-0.87060412226304,-1.18514270861957,
11.877430347329));
#29742=CARTESIAN_POINT('Ctrl Pts',(-0.848070591674411,-1.06847604194906,
11.8398786914086));
#29743=CARTESIAN_POINT('Ctrl Pts',(-0.800279768931258,-0.79477268400084,
11.7551535153833));
#29744=CARTESIAN_POINT('Ctrl Pts',(-0.775870214390773,-0.63630980009519,
11.6966683639025));
#29745=CARTESIAN_POINT('Ctrl Pts',(-0.736016130791778,-0.319434907277156,
11.6316498793278));
#29746=CARTESIAN_POINT('Ctrl Pts',(-0.720069234314568,-0.158333333333331,
11.6031686722742));
#29747=CARTESIAN_POINT('Ctrl Pts',(-0.694043459634896,0.158333333333332,
11.6074850335135));
#29748=CARTESIAN_POINT('Ctrl Pts',(-0.684234636903101,0.319434907277163,
11.6402707573857));
#29749=CARTESIAN_POINT('Ctrl Pts',(-0.67052600784846,0.636309800095199,
11.7141054852488));
#29750=CARTESIAN_POINT('Ctrl Pts',(-0.665408068045094,0.794772684000834,
11.7771791444796));
#29751=CARTESIAN_POINT('Ctrl Pts',(-0.66757080607668,1.06847604194526,11.8697080313361));
#29752=CARTESIAN_POINT('Ctrl Pts',(-0.671332221044731,1.18514270861209,
11.9105939344582));
#29753=CARTESIAN_POINT('Ctrl Pts',(-0.6779188818243,1.30000000000046,11.9523134141154));
#29754=CARTESIAN_POINT('Ctrl Pts',(-0.89857809711787,-1.30000000001151,
11.9039905526542));
#29755=CARTESIAN_POINT('Ctrl Pts',(-0.874603358219584,-1.18514270861957,
11.8632690261007));
#29756=CARTESIAN_POINT('Ctrl Pts',(-0.852274272367022,-1.06847604194906,
11.8240441276441));
#29757=CARTESIAN_POINT('Ctrl Pts',(-0.804491404877559,-0.794772684000842,
11.7368842756001));
#29758=CARTESIAN_POINT('Ctrl Pts',(-0.779337536601101,-0.63630980009519,
11.6788530360347));
#29759=CARTESIAN_POINT('Ctrl Pts',(-0.73892990170289,-0.319434907277156,
11.6137837345045));
#29760=CARTESIAN_POINT('Ctrl Pts',(-0.722441783590277,-0.158333333333331,
11.5860732558579));
#29761=CARTESIAN_POINT('Ctrl Pts',(-0.69673919586524,0.158333333333333,
11.590376212721));
#29762=CARTESIAN_POINT('Ctrl Pts',(-0.687911166797296,0.319434907277164,
11.6223606112703));
#29763=CARTESIAN_POINT('Ctrl Pts',(-0.675177329582872,0.6363098000952,11.6962538723052));
#29764=CARTESIAN_POINT('Ctrl Pts',(-0.671095145736662,0.794772684000834,
11.7589138472138));
#29765=CARTESIAN_POINT('Ctrl Pts',(-0.67283030602288,1.06847604194526,11.8539181159165));
#29766=CARTESIAN_POINT('Ctrl Pts',(-0.676014982447061,1.18514270861209,
11.8964952730699));
#29767=CARTESIAN_POINT('Ctrl Pts',(-0.681633248701541,1.30000000000046,
11.9405257597103));
#29768=CARTESIAN_POINT('Ctrl Pts',(-0.902477105871258,-1.3000000000115,
11.8862709956588));
#29769=CARTESIAN_POINT('Ctrl Pts',(-0.879221148848204,-1.18514270861957,
11.8421011623459));
#29770=CARTESIAN_POINT('Ctrl Pts',(-0.857323211941763,-1.06847604194906,
11.8003577978764));
#29771=CARTESIAN_POINT('Ctrl Pts',(-0.809871895161875,-0.79477268400084,
11.7095279036636));
#29772=CARTESIAN_POINT('Ctrl Pts',(-0.78376380919803,-0.63630980009519,
11.6521754885616));
#29773=CARTESIAN_POINT('Ctrl Pts',(-0.743059579658607,-0.319434907277157,
11.5870018840245));
#29774=CARTESIAN_POINT('Ctrl Pts',(-0.726496099759876,-0.158333333333331,
11.5604077166868));
#29775=CARTESIAN_POINT('Ctrl Pts',(-0.701225272913036,0.158333333333333,
11.564684638206));
#29776=CARTESIAN_POINT('Ctrl Pts',(-0.693057788862471,0.319434907277164,
11.5955056206572));
#29777=CARTESIAN_POINT('Ctrl Pts',(-0.681187501823921,0.6363098000952,11.6694930695212));
#29778=CARTESIAN_POINT('Ctrl Pts',(-0.677908421627274,0.794772684000835,
11.7315085139232));
#29779=CARTESIAN_POINT('Ctrl Pts',(-0.679723677487409,1.06847604194526,
11.830224032349));
#29780=CARTESIAN_POINT('Ctrl Pts',(-0.682719357389429,1.18514270861209,
11.875340909519));
#29781=CARTESIAN_POINT('Ctrl Pts',(-0.687924960193474,1.30000000000046,
11.9228443737031));
#29782=CARTESIAN_POINT('Ctrl Pts',(-0.908701175984222,-1.30000000001151,
11.8596446736958));
#29783=CARTESIAN_POINT('Ctrl Pts',(-0.885597731026704,-1.18514270861958,
11.8103494528277));
#29784=CARTESIAN_POINT('Ctrl Pts',(-0.863726842934849,-1.06847604194907,
11.7648613672129));
#29785=CARTESIAN_POINT('Ctrl Pts',(-0.816048169119225,-0.794772684000848,
11.6685700336343));
#29786=CARTESIAN_POINT('Ctrl Pts',(-0.789297210261759,-0.636309800095195,
11.6122070099515));
#29787=CARTESIAN_POINT('Ctrl Pts',(-0.748080016284346,-0.319434907277159,
11.5468882279858));
#29788=CARTESIAN_POINT('Ctrl Pts',(-0.730922493088147,-0.158333333333332,
11.5219976057089));
#29789=CARTESIAN_POINT('Ctrl Pts',(-0.706296610091351,0.158333333333333,
11.5262284547253));
#29790=CARTESIAN_POINT('Ctrl Pts',(-0.699176918679878,0.319434907277163,
11.5552723030019));
#29791=CARTESIAN_POINT('Ctrl Pts',(-0.68952274971155,0.636309800095202,
11.629367132279));
#29792=CARTESIAN_POINT('Ctrl Pts',(-0.689442245328543,0.794772684000841,
11.6903943283916));
#29793=CARTESIAN_POINT('Ctrl Pts',(-0.691123492164588,1.06847604194527,
11.7946579210228));
#29794=CARTESIAN_POINT('Ctrl Pts',(-0.6931914874416,1.18514270861209,11.843579616181));
#29795=CARTESIAN_POINT('Ctrl Pts',(-0.696599728536635,1.30000000000047,
11.8962911605941));
#29796=CARTESIAN_POINT('Ctrl Pts',(-0.915130190235684,-1.30000000001151,
11.8242205798896));
#29797=CARTESIAN_POINT('Ctrl Pts',(-0.893056339639968,-1.18514270861957,
11.7680209678601));
#29798=CARTESIAN_POINT('Ctrl Pts',(-0.871639908682559,-1.06847604194907,
11.7175023970209));
#29799=CARTESIAN_POINT('Ctrl Pts',(-0.823682439710349,-0.794772684000845,
11.6139187338168));
#29800=CARTESIAN_POINT('Ctrl Pts',(-0.794249766051324,-0.636309800095193,
11.5590155181827));
#29801=CARTESIAN_POINT('Ctrl Pts',(-0.751861014111227,-0.319434907277158,
11.4935377543236));
#29802=CARTESIAN_POINT('Ctrl Pts',(-0.734333408979958,-0.158333333333331,
11.4708919274452));
#29803=CARTESIAN_POINT('Ctrl Pts',(-0.711210673215988,0.158333333333333,
11.474997385459));
#29804=CARTESIAN_POINT('Ctrl Pts',(-0.706934100478653,0.319434907277164,
11.5015762199418));
#29805=CARTESIAN_POINT('Ctrl Pts',(-0.699537697066227,0.636309800095202,
11.5757677752393));
#29806=CARTESIAN_POINT('Ctrl Pts',(-0.70026656533437,0.794772684000837,
11.6355062348343));
#29807=CARTESIAN_POINT('Ctrl Pts',(-0.701961607982734,1.06847604194527,
11.7471880962734));
#29808=CARTESIAN_POINT('Ctrl Pts',(-0.703658269885911,1.18514270861209,
11.80119546492));
#29809=CARTESIAN_POINT('Ctrl Pts',(-0.706317872537308,1.30000000000047,
11.8608672626169));
#29810=CARTESIAN_POINT('Ctrl Pts',(-0.919875601210953,-1.30000000001151,
11.794755777199));
#29811=CARTESIAN_POINT('Ctrl Pts',(-0.897754873416259,-1.18514270861958,
11.7328980381801));
#29812=CARTESIAN_POINT('Ctrl Pts',(-0.876137226977588,-1.06847604194907,
11.6782555736647));
#29813=CARTESIAN_POINT('Ctrl Pts',(-0.827358357683314,-0.794772684000842,
11.5686892769622));
#29814=CARTESIAN_POINT('Ctrl Pts',(-0.796899762965292,-0.636309800095194,
11.5149399801506));
#29815=CARTESIAN_POINT('Ctrl Pts',(-0.753134772148241,-0.319434907277159,
11.449386078349));
#29816=CARTESIAN_POINT('Ctrl Pts',(-0.734068291732325,-0.158333333333332,
11.4287191254146));
#29817=CARTESIAN_POINT('Ctrl Pts',(-0.711489212968676,0.158333333333334,
11.4327379611124));
#29818=CARTESIAN_POINT('Ctrl Pts',(-0.708878543676851,0.319434907277166,
11.4572226251063));
#29819=CARTESIAN_POINT('Ctrl Pts',(-0.704814412254138,0.636309800095204,
11.5313722822653));
#29820=CARTESIAN_POINT('Ctrl Pts',(-0.709558684665683,0.794772684000838,
11.5898828461728));
#29821=CARTESIAN_POINT('Ctrl Pts',(-0.712685057867134,1.06847604194527,
11.7076289689314));
#29822=CARTESIAN_POINT('Ctrl Pts',(-0.714207440026723,1.1851427086121,11.7658395763296));
#29823=CARTESIAN_POINT('Ctrl Pts',(-0.715898913230535,1.30000000000048,
11.8312928575076));
#29824=CARTESIAN_POINT('Ctrl Pts',(-0.924141876334402,-1.30000000001151,
11.77109374108));
#29825=CARTESIAN_POINT('Ctrl Pts',(-0.902128626336287,-1.18514270861958,
11.7046408337731));
#29826=CARTESIAN_POINT('Ctrl Pts',(-0.880266737286765,-1.06847604194907,
11.6466664975652));
#29827=CARTESIAN_POINT('Ctrl Pts',(-0.830111074198288,-0.794772684000846,
11.5323213785717));
#29828=CARTESIAN_POINT('Ctrl Pts',(-0.796780342020798,-0.636309800095194,
11.4796953438876));
#29829=CARTESIAN_POINT('Ctrl Pts',(-0.752031508840179,-0.319434907277159,
11.414066913023));
#29830=CARTESIAN_POINT('Ctrl Pts',(-0.733948122062509,-0.158333333333332,
11.3947980763829));
#29831=CARTESIAN_POINT('Ctrl Pts',(-0.712402467902627,0.158333333333334,
11.3986851071608));
#29832=CARTESIAN_POINT('Ctrl Pts',(-0.710570449880107,0.319434907277166,
11.4215419748185));
#29833=CARTESIAN_POINT('Ctrl Pts',(-0.708111636311791,0.636309800095204,
11.4956970484854));
#29834=CARTESIAN_POINT('Ctrl Pts',(-0.714522758116903,0.794772684000838,
11.5532469192424));
#29835=CARTESIAN_POINT('Ctrl Pts',(-0.718124410207019,1.06847604194527,
11.6759178206841));
#29836=CARTESIAN_POINT('Ctrl Pts',(-0.719474850841755,1.1851427086121,11.7375308903995));
#29837=CARTESIAN_POINT('Ctrl Pts',(-0.720616710375778,1.30000000000048,
11.8076573420011));
#29838=CARTESIAN_POINT('Ctrl Pts',(-0.926371093396794,-1.30000000001152,
11.753459339287));
#29839=CARTESIAN_POINT('Ctrl Pts',(-0.904090435631733,-1.18514270861958,
11.6836508049185));
#29840=CARTESIAN_POINT('Ctrl Pts',(-0.881916612865422,-1.06847604194907,
11.623236534169));
#29841=CARTESIAN_POINT('Ctrl Pts',(-0.830937456637536,-0.794772684000847,
11.5053701111827));
#29842=CARTESIAN_POINT('Ctrl Pts',(-0.796952716130588,-0.636309800095196,
11.4534698280134));
#29843=CARTESIAN_POINT('Ctrl Pts',(-0.751203299623306,-0.31943490727716,
11.3878331944127));
#29844=CARTESIAN_POINT('Ctrl Pts',(-0.732079387725648,-0.158333333333332,
11.3697640959159));
#29845=CARTESIAN_POINT('Ctrl Pts',(-0.710840218192551,0.158333333333334,
11.3735847534848));
#29846=CARTESIAN_POINT('Ctrl Pts',(-0.71018123879766,0.319434907277167,
11.395154921514));
#29847=CARTESIAN_POINT('Ctrl Pts',(-0.709701662316501,0.636309800095206,
11.4692249373051));
#29848=CARTESIAN_POINT('Ctrl Pts',(-0.717994743494202,0.79477268400084,
11.5259919854094));
#29849=CARTESIAN_POINT('Ctrl Pts',(-0.723001082445735,1.06847604194527,
11.6522344970941));
#29850=CARTESIAN_POINT('Ctrl Pts',(-0.72470786072698,1.1851427086121,11.7163406580131));
#29851=CARTESIAN_POINT('Ctrl Pts',(-0.725954358660491,1.30000000000048,
11.7899072742888));
#29852=CARTESIAN_POINT('Ctrl Pts',(-0.928515616741265,-1.30000000001152,
11.7357458531039));
#29853=CARTESIAN_POINT('Ctrl Pts',(-0.906220595951806,-1.18514270861958,
11.6624050656068));
#29854=CARTESIAN_POINT('Ctrl Pts',(-0.883726917173569,-1.06847604194907,
11.5994386109857));
#29855=CARTESIAN_POINT('Ctrl Pts',(-0.831303079656328,-0.794772684000849,
11.4779402887388));
#29856=CARTESIAN_POINT('Ctrl Pts',(-0.79401622890383,-0.636309800095196,
11.4270499306769));
#29857=CARTESIAN_POINT('Ctrl Pts',(-0.748443991722638,-0.31943490727716,
11.3612517013318));
#29858=CARTESIAN_POINT('Ctrl Pts',(-0.732895889171905,-0.158333333333333,
11.3439307342967));
#29859=CARTESIAN_POINT('Ctrl Pts',(-0.712854812281222,0.158333333333334,
11.3475845935226));
#29860=CARTESIAN_POINT('Ctrl Pts',(-0.710580569151887,0.319434907277167,
11.3681203190846));
#29861=CARTESIAN_POINT('Ctrl Pts',(-0.710811179990112,0.636309800095207,
11.4422556130938));
#29862=CARTESIAN_POINT('Ctrl Pts',(-0.721190875660884,0.794772684000841,
11.4982216430212));
#29863=CARTESIAN_POINT('Ctrl Pts',(-0.727041576108211,1.06847604194527,
11.6282345327963));
#29864=CARTESIAN_POINT('Ctrl Pts',(-0.728824440348993,1.1851427086121,11.6949522758241));
#29865=CARTESIAN_POINT('Ctrl Pts',(-0.729857617396724,1.30000000000048,
11.7721099993483));
#29866=CARTESIAN_POINT('Ctrl Pts',(-0.930329635621813,-1.30000000001152,
11.7210988980544));
#29867=CARTESIAN_POINT('Ctrl Pts',(-0.907076845997319,-1.18514270861958,
11.6451431370766));
#29868=CARTESIAN_POINT('Ctrl Pts',(-0.884085358419116,-1.06847604194908,
11.5802500565896));
#29869=CARTESIAN_POINT('Ctrl Pts',(-0.831574082683346,-0.794772684000852,
11.455891063866));
#29870=CARTESIAN_POINT('Ctrl Pts',(-0.796125283318549,-0.636309800095196,
11.4053623224109));
#29871=CARTESIAN_POINT('Ctrl Pts',(-0.75140068947891,-0.319434907277159,
11.3394432860062));
#29872=CARTESIAN_POINT('Ctrl Pts',(-0.736139894754654,-0.158333333333332,
11.3230376354443));
#29873=CARTESIAN_POINT('Ctrl Pts',(-0.715467336234378,0.158333333333334,
11.3267399924723));
#29874=CARTESIAN_POINT('Ctrl Pts',(-0.711333498127357,0.319434907277167,
11.3464993960691));
#29875=CARTESIAN_POINT('Ctrl Pts',(-0.711346536120014,0.636309800095206,
11.4206699483946));
#29876=CARTESIAN_POINT('Ctrl Pts',(-0.723269722424154,0.794772684000839,
11.4759041572379));
#29877=CARTESIAN_POINT('Ctrl Pts',(-0.729727433914076,1.06847604194527,
11.6087621891132));
#29878=CARTESIAN_POINT('Ctrl Pts',(-0.731628539382279,1.1851427086121,11.6774767588117));
#29879=CARTESIAN_POINT('Ctrl Pts',(-0.73263544629649,1.30000000000048,11.7573965790852));
#29880=CARTESIAN_POINT('Ctrl Pts',(-0.931747258687475,-1.30000000001152,
11.7034562621613));
#29881=CARTESIAN_POINT('Ctrl Pts',(-0.90733877716988,-1.18514270861958,
11.6239757801627));
#29882=CARTESIAN_POINT('Ctrl Pts',(-0.883910231356362,-1.06847604194908,
11.5564438916877));
#29883=CARTESIAN_POINT('Ctrl Pts',(-0.832049451175459,-0.794772684000851,
11.4280353609519));
#29884=CARTESIAN_POINT('Ctrl Pts',(-0.799951516477764,-0.636309800095196,
11.3776840270139));
#29885=CARTESIAN_POINT('Ctrl Pts',(-0.757363875886255,-0.319434907277159,
11.3113557017931));
#29886=CARTESIAN_POINT('Ctrl Pts',(-0.742707262105031,-0.158333333333332,
11.2961489921131));
#29887=CARTESIAN_POINT('Ctrl Pts',(-0.722150626445397,0.158333333333334,
11.299816574206));
#29888=CARTESIAN_POINT('Ctrl Pts',(-0.717216708376096,0.319434907277167,
11.3183579084001));
#29889=CARTESIAN_POINT('Ctrl Pts',(-0.715964078358445,0.636309800095206,
11.3928350448839));
#29890=CARTESIAN_POINT('Ctrl Pts',(-0.726336336909195,0.79477268400084,
11.447716025051));
#29891=CARTESIAN_POINT('Ctrl Pts',(-0.732307490535758,1.06847604194527,
11.5846602431266));
#29892=CARTESIAN_POINT('Ctrl Pts',(-0.734317087069204,1.1851427086121,11.65608184955));
#29893=CARTESIAN_POINT('Ctrl Pts',(-0.735751588984204,1.30000000000048,
11.739646984675));
#29894=CARTESIAN_POINT('Ctrl Pts',(-0.932811379692883,-1.30000000001152,
11.6914337625578));
#29895=CARTESIAN_POINT('Ctrl Pts',(-0.90624835288135,-1.18514270861958,
11.6096869608822));
#29896=CARTESIAN_POINT('Ctrl Pts',(-0.882011643627204,-1.06847604194908,
11.5404979069991));
#29897=CARTESIAN_POINT('Ctrl Pts',(-0.831394255649799,-0.794772684000851,
11.409668260878));
#29898=CARTESIAN_POINT('Ctrl Pts',(-0.805863671216798,-0.636309800095197,
11.3596728386796));
#29899=CARTESIAN_POINT('Ctrl Pts',(-0.76676614190522,-0.319434907277159,
11.2934131620907));
#29900=CARTESIAN_POINT('Ctrl Pts',(-0.7519939500761,-0.158333333333332,
11.2792748470613));
#29901=CARTESIAN_POINT('Ctrl Pts',(-0.731604230888437,0.158333333333334,
11.2829625198157));
#29902=CARTESIAN_POINT('Ctrl Pts',(-0.726824245390955,0.319434907277167,
11.3005329620478));
#29903=CARTESIAN_POINT('Ctrl Pts',(-0.722683372359804,0.636309800095206,
11.3748246904046));
#29904=CARTESIAN_POINT('Ctrl Pts',(-0.72755043150687,0.79477268400084,11.4289715802577));
#29905=CARTESIAN_POINT('Ctrl Pts',(-0.732217053984718,1.06847604194527,
11.5683538364568));
#29906=CARTESIAN_POINT('Ctrl Pts',(-0.734729140509331,1.1851427086121,11.6415286370167));
#29907=CARTESIAN_POINT('Ctrl Pts',(-0.737733305603302,1.30000000000048,
11.7275448240494));
#29908=CARTESIAN_POINT('Ctrl Pts',(-0.936125406442746,-1.30000000001152,
11.6834957005072));
#29909=CARTESIAN_POINT('Ctrl Pts',(-0.909492919288004,-1.18514270861958,
11.6019904180297));
#29910=CARTESIAN_POINT('Ctrl Pts',(-0.885532801702577,-1.06847604194908,
11.5330073325074));
#29911=CARTESIAN_POINT('Ctrl Pts',(-0.836353845186883,-0.794772684000851,
11.4025713849577));
#29912=CARTESIAN_POINT('Ctrl Pts',(-0.813383183475108,-0.636309800095197,
11.3527487599227));
#29913=CARTESIAN_POINT('Ctrl Pts',(-0.77596280188267,-0.319434907277159,
11.2866672191688));
#29914=CARTESIAN_POINT('Ctrl Pts',(-0.761169784372622,-0.158333333333332,
11.2724808787964));
#29915=CARTESIAN_POINT('Ctrl Pts',(-0.74101228662764,0.158333333333334,
11.2762150307074));
#29916=CARTESIAN_POINT('Ctrl Pts',(-0.736764158587383,0.319434907277167,
11.2939064508864));
#29917=CARTESIAN_POINT('Ctrl Pts',(-0.730851239620766,0.636309800095206,
11.368060793598));
#29918=CARTESIAN_POINT('Ctrl Pts',(-0.732075357025827,0.79477268400084,
11.421994282357));
#29919=CARTESIAN_POINT('Ctrl Pts',(-0.735457044102353,1.06847604194527,
11.5609770187779));
#29920=CARTESIAN_POINT('Ctrl Pts',(-0.738012470505655,1.1851427086121,11.6339459053542));
#29921=CARTESIAN_POINT('Ctrl Pts',(-0.741659516280686,1.30000000000048,
11.7197232017282));
#29922=CARTESIAN_POINT('Ctrl Pts',(-0.936125406440075,-1.3,11.683495700499));
#29923=CARTESIAN_POINT('Ctrl Pts',(-0.909492919286402,-1.18514270861178,
11.6019904180251));
#29924=CARTESIAN_POINT('Ctrl Pts',(-0.885532801701866,-1.06847604194512,
11.5330073325055));
#29925=CARTESIAN_POINT('Ctrl Pts',(-0.836353845186883,-0.794772684000851,
11.4025713849577));
#29926=CARTESIAN_POINT('Ctrl Pts',(-0.813383183475108,-0.636309800095197,
11.3527487599227));
#29927=CARTESIAN_POINT('Ctrl Pts',(-0.775962801882671,-0.319434907277159,
11.2866672191688));
#29928=CARTESIAN_POINT('Ctrl Pts',(-0.761169784372622,-0.158333333333332,
11.2724808787964));
#29929=CARTESIAN_POINT('Ctrl Pts',(-0.741012286627641,0.158333333333334,
11.2762150307074));
#29930=CARTESIAN_POINT('Ctrl Pts',(-0.736764158587383,0.319434907277167,
11.2939064508864));
#29931=CARTESIAN_POINT('Ctrl Pts',(-0.730851239620766,0.636309800095206,
11.368060793598));
#29932=CARTESIAN_POINT('Ctrl Pts',(-0.732075357025827,0.79477268400084,
11.421994282357));
#29933=CARTESIAN_POINT('Ctrl Pts',(-0.735457044102351,1.06847604194511,
11.5609770187778));
#29934=CARTESIAN_POINT('Ctrl Pts',(-0.738012470505648,1.18514270861177,
11.633945905354));
#29935=CARTESIAN_POINT('Ctrl Pts',(-0.741659516280671,1.3,11.7197232017278));
#29936=CARTESIAN_POINT('',(-0.818977267421107,-1.2,12.0817800273514));
#29937=CARTESIAN_POINT('Ctrl Pts',(-0.818977267421108,-1.2,12.0817800273514));
#29938=CARTESIAN_POINT('Ctrl Pts',(-0.829590878647036,-1.21693989154628,
12.0628228500606));
#29939=CARTESIAN_POINT('Ctrl Pts',(-0.841157631026617,-1.23347875773062,
12.0440503378966));
#29940=CARTESIAN_POINT('Ctrl Pts',(-0.857159462862295,-1.25898780506585,
12.0153221239789));
#29941=CARTESIAN_POINT('Ctrl Pts',(-0.862316329350737,-1.26708707076649,
12.0061721287558));
#29942=CARTESIAN_POINT('Ctrl Pts',(-0.871215005322769,-1.28134030327299,
11.9900791870324));
#29943=CARTESIAN_POINT('Ctrl Pts',(-0.877883425044479,-1.29212373571783,
11.9778974543232));
#29944=CARTESIAN_POINT('Ctrl Pts',(-0.881788403109014,-1.29865542294387,
11.9705339008578));
#29945=CARTESIAN_POINT('Ctrl Pts',(-0.882187409448981,-1.29932801060554,
11.9697761372506));
#29946=CARTESIAN_POINT('Ctrl Pts',(-0.88258187706403,-1.3000000000115,11.9690197347219));
#29947=CARTESIAN_POINT('',(-0.664237986899246,-0.653834841416763,12.1052306670025));
#29948=CARTESIAN_POINT('Ctrl Pts',(-0.664237986905426,-0.653834841416077,
12.105230667028));
#29949=CARTESIAN_POINT('Ctrl Pts',(-0.680353745117992,-0.717928623971185,
12.1030483641927));
#29950=CARTESIAN_POINT('Ctrl Pts',(-0.693482797353694,-0.763796716852745,
12.1012100657869));
#29951=CARTESIAN_POINT('Ctrl Pts',(-0.744781546673584,-0.949538510163098,
12.0937752011493));
#29952=CARTESIAN_POINT('Ctrl Pts',(-0.772317944299114,-1.0477587126458,
12.0896076895435));
#29953=CARTESIAN_POINT('Ctrl Pts',(-0.818977267421107,-1.2,12.0817800273514));
#29954=CARTESIAN_POINT('',(-0.525742999964556,0.653834841531101,12.1220010461182));
#29955=CARTESIAN_POINT('Ctrl Pts',(-0.525742999964555,0.653834841531117,
12.1220010461182));
#29956=CARTESIAN_POINT('Ctrl Pts',(-0.539180494581549,0.575791384517359,
12.0825525341831));
#29957=CARTESIAN_POINT('Ctrl Pts',(-0.551088168076891,0.493917938905458,
12.0497160696344));
#29958=CARTESIAN_POINT('Ctrl Pts',(-0.570743025184575,0.338198422468042,
12.0029892655978));
#29959=CARTESIAN_POINT('Ctrl Pts',(-0.578836711827597,0.265710408106597,
11.987005961632));
#29960=CARTESIAN_POINT('Ctrl Pts',(-0.593510978022751,0.129738985434452,
11.9674960160308));
#29961=CARTESIAN_POINT('Ctrl Pts',(-0.600113893017226,0.0666402976695767,
11.9624924648463));
#29962=CARTESIAN_POINT('Ctrl Pts',(-0.613310308940931,-0.0595494045754736,
11.9605197921755));
#29963=CARTESIAN_POINT('Ctrl Pts',(-0.620002378829859,-0.122795601055212,
11.9635188907578));
#29964=CARTESIAN_POINT('Ctrl Pts',(-0.633837957101957,-0.260143441971975,
11.9789765523794));
#29965=CARTESIAN_POINT('Ctrl Pts',(-0.640844580997494,-0.333940897156081,
11.9930593600372));
#29966=CARTESIAN_POINT('Ctrl Pts',(-0.653894554419043,-0.491228500515348,
12.0359708867721));
#29967=CARTESIAN_POINT('Ctrl Pts',(-0.659731921577109,-0.574163620766454,
12.0669021452979));
#29968=CARTESIAN_POINT('Ctrl Pts',(-0.664237986928543,-0.653834841428476,
12.1052306669747));
#29969=CARTESIAN_POINT('',(-0.597447978578511,1.2,12.1138127673826));
#29970=CARTESIAN_POINT('Ctrl Pts',(-0.597447978578509,1.2,12.1138127673826));
#29971=CARTESIAN_POINT('Ctrl Pts',(-0.585248394446679,1.13497002128492,
12.1152960589169));
#29972=CARTESIAN_POINT('Ctrl Pts',(-0.568988293295729,1.03881507655241,
12.1172252340192));
#29973=CARTESIAN_POINT('Ctrl Pts',(-0.537251997267457,0.795009267531881,
12.120775755352));
#29974=CARTESIAN_POINT('Ctrl Pts',(-0.53228169119802,0.741767795577442,
12.1213026165338));
#29975=CARTESIAN_POINT('Ctrl Pts',(-0.525742999964558,0.653834841531101,
12.1220010461182));
#29976=CARTESIAN_POINT('Ctrl Pts',(-0.659151153699351,1.29999999999999,
12.0049994543784));
#29977=CARTESIAN_POINT('Ctrl Pts',(-0.649082664482629,1.28244937374245,
12.0240956466888));
#29978=CARTESIAN_POINT('Ctrl Pts',(-0.638073668917069,1.2652022482834,12.0429614950135));
#29979=CARTESIAN_POINT('Ctrl Pts',(-0.622388419312196,1.23914419848352,
12.071260359206));
#29980=CARTESIAN_POINT('Ctrl Pts',(-0.610683834550175,1.2193232684228,12.0927379078));
#29981=CARTESIAN_POINT('Ctrl Pts',(-0.597447978578509,1.2,12.1138127673826));
#29982=CARTESIAN_POINT('Ctrl Pts',(-0.936125406440075,-1.3,11.683495700499));
#29983=CARTESIAN_POINT('Ctrl Pts',(-0.909492919286402,-1.18514270861178,
11.6019904180251));
#29984=CARTESIAN_POINT('Ctrl Pts',(-0.885532801701865,-1.06847604194512,
11.5330073325055));
#29985=CARTESIAN_POINT('Ctrl Pts',(-0.836353845186884,-0.794772684000851,
11.4025713849577));
#29986=CARTESIAN_POINT('Ctrl Pts',(-0.813383183475109,-0.636309800095197,
11.3527487599227));
#29987=CARTESIAN_POINT('Ctrl Pts',(-0.775962801882671,-0.319434907277159,
11.2866672191688));
#29988=CARTESIAN_POINT('Ctrl Pts',(-0.761169784372622,-0.158333333333333,
11.2724808787964));
#29989=CARTESIAN_POINT('Ctrl Pts',(-0.741012286627641,0.158333333333334,
11.2762150307074));
#29990=CARTESIAN_POINT('Ctrl Pts',(-0.736764158587383,0.319434907277167,
11.2939064508864));
#29991=CARTESIAN_POINT('Ctrl Pts',(-0.730851239620767,0.636309800095206,
11.368060793598));
#29992=CARTESIAN_POINT('Ctrl Pts',(-0.732075357025827,0.79477268400084,
11.421994282357));
#29993=CARTESIAN_POINT('Ctrl Pts',(-0.735457044102351,1.06847604194511,
11.5609770187778));
#29994=CARTESIAN_POINT('Ctrl Pts',(-0.738012470505648,1.18514270861178,
11.633945905354));
#29995=CARTESIAN_POINT('Ctrl Pts',(-0.741659516280671,1.3,11.7197232017278));
#29996=CARTESIAN_POINT('Ctrl Pts',(-1.01101605778904,-1.3,11.6658747012318));
#29997=CARTESIAN_POINT('Ctrl Pts',(-0.982742057194053,-1.18514270861178,
11.5849228973736));
#29998=CARTESIAN_POINT('Ctrl Pts',(-0.95765377154039,-1.06847604194512,
11.5163675802146));
#29999=CARTESIAN_POINT('Ctrl Pts',(-0.90705445160062,-0.794772684000851,
11.386629447317));
#30000=CARTESIAN_POINT('Ctrl Pts',(-0.884801197368707,-0.636309800095197,
11.3368248349354));
#30001=CARTESIAN_POINT('Ctrl Pts',(-0.847999940077956,-0.319434907277159,
11.270991020387));
#30002=CARTESIAN_POINT('Ctrl Pts',(-0.834445726094756,-0.158333333333333,
11.2567221110703));
#30003=CARTESIAN_POINT('Ctrl Pts',(-0.814362858626307,0.158333333333334,
11.2608073708274));
#30004=CARTESIAN_POINT('Ctrl Pts',(-0.808949443435951,0.319434907277167,
11.2789272273103));
#30005=CARTESIAN_POINT('Ctrl Pts',(-0.802571685601039,0.636309800095206,
11.3535596997118));
#30006=CARTESIAN_POINT('Ctrl Pts',(-0.803147745067787,0.79477268400084,
11.4078014397586));
#30007=CARTESIAN_POINT('Ctrl Pts',(-0.808110825487516,1.06847604194511,
11.5468439477319));
#30008=CARTESIAN_POINT('Ctrl Pts',(-0.811870873772818,1.18514270861178,
11.6197447528576));
#30009=CARTESIAN_POINT('Ctrl Pts',(-0.817242636729975,1.3,11.70536001344));
#30010=CARTESIAN_POINT('Ctrl Pts',(-1.08590670913801,-1.3,11.6482537019647));
#30011=CARTESIAN_POINT('Ctrl Pts',(-1.05599119510171,-1.18514270861178,
11.5678553767222));
#30012=CARTESIAN_POINT('Ctrl Pts',(-1.02977474137891,-1.06847604194512,
11.4997278279237));
#30013=CARTESIAN_POINT('Ctrl Pts',(-0.977755058014356,-0.794772684000851,
11.3706875096762));
#30014=CARTESIAN_POINT('Ctrl Pts',(-0.956219211262306,-0.636309800095197,
11.3209009099481));
#30015=CARTESIAN_POINT('Ctrl Pts',(-0.920037078273243,-0.319434907277159,
11.2553148216052));
#30016=CARTESIAN_POINT('Ctrl Pts',(-0.90772166781689,-0.158333333333333,
11.2409633433442));
#30017=CARTESIAN_POINT('Ctrl Pts',(-0.887713430624973,0.158333333333334,
11.2453997109473));
#30018=CARTESIAN_POINT('Ctrl Pts',(-0.881134728284519,0.319434907277167,
11.2639480037341));
#30019=CARTESIAN_POINT('Ctrl Pts',(-0.874292131581311,0.636309800095206,
11.3390586058255));
#30020=CARTESIAN_POINT('Ctrl Pts',(-0.874220133109747,0.79477268400084,
11.3936085971601));
#30021=CARTESIAN_POINT('Ctrl Pts',(-0.880764606872681,1.06847604194511,
11.5327108766861));
#30022=CARTESIAN_POINT('Ctrl Pts',(-0.885729277039988,1.18514270861178,
11.6055436003612));
#30023=CARTESIAN_POINT('Ctrl Pts',(-0.892825757179279,1.3,11.6909968251522));
#30024=CARTESIAN_POINT('Ctrl Pts',(-1.16079736048698,-1.3,11.6306327026976));
#30025=CARTESIAN_POINT('Ctrl Pts',(-1.12924033300936,-1.18514270861178,
11.5507878560707));
#30026=CARTESIAN_POINT('Ctrl Pts',(-1.10189571121744,-1.06847604194512,
11.4830880756329));
#30027=CARTESIAN_POINT('Ctrl Pts',(-1.04845566442809,-0.794772684000851,
11.3547455720355));
#30028=CARTESIAN_POINT('Ctrl Pts',(-1.0276372251559,-0.636309800095197,
11.3049769849608));
#30029=CARTESIAN_POINT('Ctrl Pts',(-0.992074216468528,-0.319434907277159,
11.2396386228234));
#30030=CARTESIAN_POINT('Ctrl Pts',(-0.980997609539023,-0.158333333333333,
11.2252045756181));
#30031=CARTESIAN_POINT('Ctrl Pts',(-0.961064002623639,0.158333333333334,
11.2299920510673));
#30032=CARTESIAN_POINT('Ctrl Pts',(-0.953320013133087,0.319434907277167,
11.248968780158));
#30033=CARTESIAN_POINT('Ctrl Pts',(-0.946012577561583,0.636309800095206,
11.3245575119393));
#30034=CARTESIAN_POINT('Ctrl Pts',(-0.945292521151708,0.79477268400084,
11.3794157545617));
#30035=CARTESIAN_POINT('Ctrl Pts',(-0.953418388257847,1.06847604194511,
11.5185778056402));
#30036=CARTESIAN_POINT('Ctrl Pts',(-0.959587680307158,1.18514270861178,
11.5913424478648));
#30037=CARTESIAN_POINT('Ctrl Pts',(-0.968408877628584,1.3,11.6766336368644));
#30038=CARTESIAN_POINT('Ctrl Pts',(-1.16079736048698,-1.3,11.6306327026976));
#30039=CARTESIAN_POINT('Ctrl Pts',(-1.12924033300936,-1.18514270861178,
11.5507878560707));
#30040=CARTESIAN_POINT('Ctrl Pts',(-1.10189571121744,-1.06847604194512,
11.4830880756329));
#30041=CARTESIAN_POINT('Ctrl Pts',(-1.04845566442809,-0.794772684000851,
11.3547455720355));
#30042=CARTESIAN_POINT('Ctrl Pts',(-1.0276372251559,-0.636309800095197,
11.3049769849608));
#30043=CARTESIAN_POINT('Ctrl Pts',(-0.992074216468528,-0.319434907277159,
11.2396386228234));
#30044=CARTESIAN_POINT('Ctrl Pts',(-0.980997609539023,-0.158333333333332,
11.2252045756181));
#30045=CARTESIAN_POINT('Ctrl Pts',(-0.961064002623638,0.158333333333334,
11.2299920510673));
#30046=CARTESIAN_POINT('Ctrl Pts',(-0.953320013133087,0.319434907277167,
11.248968780158));
#30047=CARTESIAN_POINT('Ctrl Pts',(-0.946012577561583,0.636309800095206,
11.3245575119393));
#30048=CARTESIAN_POINT('Ctrl Pts',(-0.945292521151708,0.79477268400084,
11.3794157545617));
#30049=CARTESIAN_POINT('Ctrl Pts',(-0.953418388257847,1.06847604194511,
11.5185778056402));
#30050=CARTESIAN_POINT('Ctrl Pts',(-0.959587680307158,1.18514270861178,
11.5913424478648));
#30051=CARTESIAN_POINT('Ctrl Pts',(-0.968408877628584,1.3,11.6766336368644));
#30052=CARTESIAN_POINT('Ctrl Pts',(-1.16079736048729,-1.30000000000112,
11.6306327026983));
#30053=CARTESIAN_POINT('Ctrl Pts',(-1.12924033300954,-1.18514270861254,
11.5507878560712));
#30054=CARTESIAN_POINT('Ctrl Pts',(-1.10189571121751,-1.0684760419455,11.483088075633));
#30055=CARTESIAN_POINT('Ctrl Pts',(-1.04845566442809,-0.794772684000851,
11.3547455720355));
#30056=CARTESIAN_POINT('Ctrl Pts',(-1.0276372251559,-0.636309800095196,
11.3049769849608));
#30057=CARTESIAN_POINT('Ctrl Pts',(-0.992074216468527,-0.319434907277159,
11.2396386228234));
#30058=CARTESIAN_POINT('Ctrl Pts',(-0.980997609539022,-0.158333333333332,
11.2252045756181));
#30059=CARTESIAN_POINT('Ctrl Pts',(-0.961064002623638,0.158333333333334,
11.2299920510673));
#30060=CARTESIAN_POINT('Ctrl Pts',(-0.953320013133086,0.319434907277167,
11.248968780158));
#30061=CARTESIAN_POINT('Ctrl Pts',(-0.946012577561583,0.636309800095206,
11.3245575119393));
#30062=CARTESIAN_POINT('Ctrl Pts',(-0.945292521151708,0.79477268400084,
11.3794157545617));
#30063=CARTESIAN_POINT('Ctrl Pts',(-0.953418388257849,1.06847604194519,
11.5185778056402));
#30064=CARTESIAN_POINT('Ctrl Pts',(-0.959587680307166,1.18514270861193,
11.5913424478649));
#30065=CARTESIAN_POINT('Ctrl Pts',(-0.968408877628601,1.30000000000022,
11.6766336368646));
#30066=CARTESIAN_POINT('Ctrl Pts',(-1.16756547281003,-1.30000000000112,
11.6361811764323));
#30067=CARTESIAN_POINT('Ctrl Pts',(-1.13532397902382,-1.18514270861254,
11.5563795754664));
#30068=CARTESIAN_POINT('Ctrl Pts',(-1.10785601152158,-1.0684760419455,11.488509311166));
#30069=CARTESIAN_POINT('Ctrl Pts',(-1.05542731230007,-0.794772684000851,
11.3592791977852));
#30070=CARTESIAN_POINT('Ctrl Pts',(-1.03785006786609,-0.636309800095196,
11.3078339412244));
#30071=CARTESIAN_POINT('Ctrl Pts',(-1.00385002391231,-0.319434907277159,
11.2416493150162));
#30072=CARTESIAN_POINT('Ctrl Pts',(-0.992336747169047,-0.158333333333332,
11.2275421125221));
#30073=CARTESIAN_POINT('Ctrl Pts',(-0.972209900186257,0.158333333333334,
11.2324665017675));
#30074=CARTESIAN_POINT('Ctrl Pts',(-0.964465402249317,0.319434907277167,
11.2513908870207));
#30075=CARTESIAN_POINT('Ctrl Pts',(-0.955698270375139,0.636309800095206,
11.3278245114471));
#30076=CARTESIAN_POINT('Ctrl Pts',(-0.952709891127445,0.79477268400084,
11.3838818264982));
#30077=CARTESIAN_POINT('Ctrl Pts',(-0.959681817340565,1.06847604194519,
11.5239886018995));
#30078=CARTESIAN_POINT('Ctrl Pts',(-0.965682205206487,1.18514270861193,
11.5970539055485));
#30079=CARTESIAN_POINT('Ctrl Pts',(-0.974665092415997,1.30000000000022,
11.682537481243));
#30080=CARTESIAN_POINT('Ctrl Pts',(-1.17433759800624,-1.30000000000114,
11.6464116794424));
#30081=CARTESIAN_POINT('Ctrl Pts',(-1.14166436485374,-1.18514270861256,
11.5694808106212));
#30082=CARTESIAN_POINT('Ctrl Pts',(-1.11444976981747,-1.06847604194552,
11.5034134250506));
#30083=CARTESIAN_POINT('Ctrl Pts',(-1.06418915706796,-0.794772684000863,
11.3758813671891));
#30084=CARTESIAN_POINT('Ctrl Pts',(-1.0513091229464,-0.636309800095205,
11.3215414692882));
#30085=CARTESIAN_POINT('Ctrl Pts',(-1.01984359533584,-0.319434907277162,
11.2540237958508));
#30086=CARTESIAN_POINT('Ctrl Pts',(-1.0077743357193,-0.158333333333334,
11.2391008731644));
#30087=CARTESIAN_POINT('Ctrl Pts',(-0.987512099007357,0.158333333333336,
11.2441073694368));
#30088=CARTESIAN_POINT('Ctrl Pts',(-0.980345522160174,0.319434907277171,
11.2639439027508));
#30089=CARTESIAN_POINT('Ctrl Pts',(-0.968447629115628,0.636309800095215,
11.3418486499862));
#30090=CARTESIAN_POINT('Ctrl Pts',(-0.959621049662965,0.79477268400085,
11.4008963472683));
#30091=CARTESIAN_POINT('Ctrl Pts',(-0.964471525893826,1.0684760419452,11.5393026757461));
#30092=CARTESIAN_POINT('Ctrl Pts',(-0.970529496012491,1.18514270861194,
11.610531299113));
#30093=CARTESIAN_POINT('Ctrl Pts',(-0.980545844817339,1.30000000000024,
11.6930775747087));
#30094=CARTESIAN_POINT('Ctrl Pts',(-1.18440586374583,-1.30000000000115,
11.6613628993834));
#30095=CARTESIAN_POINT('Ctrl Pts',(-1.15281179463886,-1.18514270861256,
11.5879487744173));
#30096=CARTESIAN_POINT('Ctrl Pts',(-1.12658990680956,-1.06847604194552,
11.524407622229));
#30097=CARTESIAN_POINT('Ctrl Pts',(-1.07842291370587,-0.794772684000867,
11.4004233915087));
#30098=CARTESIAN_POINT('Ctrl Pts',(-1.06681408259705,-0.636309800095209,
11.3451288299006));
#30099=CARTESIAN_POINT('Ctrl Pts',(-1.03664169893558,-0.319434907277165,
11.2773712449188));
#30100=CARTESIAN_POINT('Ctrl Pts',(-1.02481278861994,-0.158333333333335,
11.2610028855051));
#30101=CARTESIAN_POINT('Ctrl Pts',(-1.0044850652804,0.158333333333337,11.2660078555499));
#30102=CARTESIAN_POINT('Ctrl Pts',(-0.997358728970921,0.319434907277173,
11.2871590926494));
#30103=CARTESIAN_POINT('Ctrl Pts',(-0.983329367588696,0.636309800095218,
11.3655638273867));
#30104=CARTESIAN_POINT('Ctrl Pts',(-0.97135393304074,0.794772684000856,
11.4261862920945));
#30105=CARTESIAN_POINT('Ctrl Pts',(-0.973948227190362,1.06847604194521,
11.5611531693971));
#30106=CARTESIAN_POINT('Ctrl Pts',(-0.979354787992951,1.18514270861195,
11.6297802214725));
#30107=CARTESIAN_POINT('Ctrl Pts',(-0.989044935788829,1.30000000000025,
11.7086121654545));
#30108=CARTESIAN_POINT('Ctrl Pts',(-1.19298536144512,-1.30000000000116,
11.6736347004981));
#30109=CARTESIAN_POINT('Ctrl Pts',(-1.16257956592102,-1.18514270861257,
11.6026906475997));
#30110=CARTESIAN_POINT('Ctrl Pts',(-1.13708399446326,-1.06847604194553,
11.5409940674741));
#30111=CARTESIAN_POINT('Ctrl Pts',(-1.0895277239045,-0.794772684000875,
11.4198261370814));
#30112=CARTESIAN_POINT('Ctrl Pts',(-1.07616291886583,-0.636309800095215,
11.3645178040103));
#30113=CARTESIAN_POINT('Ctrl Pts',(-1.046127413614,-0.319434907277168,11.2967346480581));
#30114=CARTESIAN_POINT('Ctrl Pts',(-1.0356366171024,-0.158333333333337,
11.2789326233998));
#30115=CARTESIAN_POINT('Ctrl Pts',(-1.01578267670476,0.158333333333339,
11.2837609183981));
#30116=CARTESIAN_POINT('Ctrl Pts',(-1.00856388451852,0.319434907277175,
11.3059044815962));
#30117=CARTESIAN_POINT('Ctrl Pts',(-0.993790452697415,0.636309800095223,
11.3845140146692));
#30118=CARTESIAN_POINT('Ctrl Pts',(-0.980710833423847,0.794772684000864,
11.446079999681));
#30119=CARTESIAN_POINT('Ctrl Pts',(-0.982257391046026,1.06847604194522,
11.5784182630752));
#30120=CARTESIAN_POINT('Ctrl Pts',(-0.987267620003271,1.18514270861196,
11.6451250692127));
#30121=CARTESIAN_POINT('Ctrl Pts',(-0.996618630428724,1.30000000000026,
11.7212543508803));
#30122=CARTESIAN_POINT('Ctrl Pts',(-1.20105256512359,-1.30000000000117,
11.6846776130528));
#30123=CARTESIAN_POINT('Ctrl Pts',(-1.17182076003448,-1.18514270861259,
11.6161968728078));
#30124=CARTESIAN_POINT('Ctrl Pts',(-1.14702653796543,-1.06847604194554,
11.5563595354834));
#30125=CARTESIAN_POINT('Ctrl Pts',(-1.0999986294307,-0.794772684000881,
11.4380913056996));
#30126=CARTESIAN_POINT('Ctrl Pts',(-1.08498990472442,-0.636309800095221,
11.3828473439718));
#30127=CARTESIAN_POINT('Ctrl Pts',(-1.05457956671436,-0.319434907277171,
11.3152877377322));
#30128=CARTESIAN_POINT('Ctrl Pts',(-1.04492763006788,-0.158333333333338,
11.2962396194479));
#30129=CARTESIAN_POINT('Ctrl Pts',(-1.02445048342747,0.15833333333334,11.3012437581198));
#30130=CARTESIAN_POINT('Ctrl Pts',(-1.01546159798066,0.319434907277179,
11.3248855867104));
#30131=CARTESIAN_POINT('Ctrl Pts',(-1.00042100180492,0.63630980009523,11.4034742761441));
#30132=CARTESIAN_POINT('Ctrl Pts',(-0.989132095493053,0.794772684000872,
11.4649686187968));
#30133=CARTESIAN_POINT('Ctrl Pts',(-0.990490881115352,1.06847604194523,
11.594349776762));
#30134=CARTESIAN_POINT('Ctrl Pts',(-0.995057162532792,1.18514270861197,
11.6591412225012));
#30135=CARTESIAN_POINT('Ctrl Pts',(-1.00360155741975,1.30000000000027,11.7327198047409));
#30136=CARTESIAN_POINT('Ctrl Pts',(-1.20689949924884,-1.30000000000117,
11.6917782430978));
#30137=CARTESIAN_POINT('Ctrl Pts',(-1.17845243113741,-1.18514270861259,
11.6248282543793));
#30138=CARTESIAN_POINT('Ctrl Pts',(-1.15410150400538,-1.06847604194554,
11.5661579127043));
#30139=CARTESIAN_POINT('Ctrl Pts',(-1.10730889603686,-0.794772684000884,
11.4497453274811));
#30140=CARTESIAN_POINT('Ctrl Pts',(-1.09120924295904,-0.636309800095223,
11.3945642230668));
#30141=CARTESIAN_POINT('Ctrl Pts',(-1.06001205148635,-0.319434907277172,
11.327335922249));
#30142=CARTESIAN_POINT('Ctrl Pts',(-1.05000648532554,-0.158333333333339,
11.3078132435952));
#30143=CARTESIAN_POINT('Ctrl Pts',(-1.0289822678563,0.158333333333341,11.3129700474019));
#30144=CARTESIAN_POINT('Ctrl Pts',(-1.01946870924847,0.31943490727718,11.337318972364));
#30145=CARTESIAN_POINT('Ctrl Pts',(-1.00477531806935,0.636309800095232,
11.4157246330572));
#30146=CARTESIAN_POINT('Ctrl Pts',(-0.995163031930164,0.794772684000874,
11.4770283488341));
#30147=CARTESIAN_POINT('Ctrl Pts',(-0.996348460080219,1.06847604194523,
11.6045910634879));
#30148=CARTESIAN_POINT('Ctrl Pts',(-1.00044163242317,1.18514270861198,11.6682499633972));
#30149=CARTESIAN_POINT('Ctrl Pts',(-1.00811484918735,1.30000000000028,11.7403505907066));
#30150=CARTESIAN_POINT('Ctrl Pts',(-1.21290364438232,-1.30000000000118,
11.698835255245));
#30151=CARTESIAN_POINT('Ctrl Pts',(-1.18517186067427,-1.18514270861259,
11.6334762032491));
#30152=CARTESIAN_POINT('Ctrl Pts',(-1.16120472180641,-1.06847604194555,
11.5760187052981));
#30153=CARTESIAN_POINT('Ctrl Pts',(-1.11453291910748,-0.794772684000885,
11.461534561243));
#30154=CARTESIAN_POINT('Ctrl Pts',(-1.09730001002919,-0.636309800095224,
11.4064183653184));
#30155=CARTESIAN_POINT('Ctrl Pts',(-1.06524461600585,-0.319434907277173,
11.3395345033929));
#30156=CARTESIAN_POINT('Ctrl Pts',(-1.05468161482419,-0.158333333333339,
11.3195732647092));
#30157=CARTESIAN_POINT('Ctrl Pts',(-1.03344222170005,0.158333333333341,
11.3247807857825));
#30158=CARTESIAN_POINT('Ctrl Pts',(-1.02429992110725,0.319434907277181,
11.3495874441969));
#30159=CARTESIAN_POINT('Ctrl Pts',(-1.00996736700274,0.636309800095234,
11.4278162259574));
#30160=CARTESIAN_POINT('Ctrl Pts',(-1.00099482485428,0.794772684000876,
11.489260778002));
#30161=CARTESIAN_POINT('Ctrl Pts',(-1.00187182097402,1.06847604194523,11.6150124880496));
#30162=CARTESIAN_POINT('Ctrl Pts',(-1.00560365754974,1.18514270861198,11.677478729188));
#30163=CARTESIAN_POINT('Ctrl Pts',(-1.01268771157684,1.30000000000028,11.7479779557451));
#30164=CARTESIAN_POINT('Ctrl Pts',(-1.22618519864795,-1.30000000000117,
11.7171839141231));
#30165=CARTESIAN_POINT('Ctrl Pts',(-1.20029820969549,-1.18514270861259,
11.6557804959295));
#30166=CARTESIAN_POINT('Ctrl Pts',(-1.1774891576665,-1.06847604194555,11.6012816521569));
#30167=CARTESIAN_POINT('Ctrl Pts',(-1.13190633457677,-0.794772684000887,
11.491329368754));
#30168=CARTESIAN_POINT('Ctrl Pts',(-1.11309362995195,-0.636309800095223,
11.4359111902228));
#30169=CARTESIAN_POINT('Ctrl Pts',(-1.07962100664597,-0.319434907277172,
11.3696324319088));
#30170=CARTESIAN_POINT('Ctrl Pts',(-1.06755959380154,-0.158333333333339,
11.3486314227978));
#30171=CARTESIAN_POINT('Ctrl Pts',(-1.04563975760617,0.158333333333341,
11.354033649905));
#30172=CARTESIAN_POINT('Ctrl Pts',(-1.03692233361866,0.319434907277181,
11.3801842515533));
#30173=CARTESIAN_POINT('Ctrl Pts',(-1.02342169532662,0.636309800095234,
11.4579815559397));
#30174=CARTESIAN_POINT('Ctrl Pts',(-1.01646829809711,0.794772684000875,
11.5195861143864));
#30175=CARTESIAN_POINT('Ctrl Pts',(-1.01666663265259,1.06847604194523,11.6407453923103));
#30176=CARTESIAN_POINT('Ctrl Pts',(-1.01948091312335,1.18514270861198,11.7002238250183));
#30177=CARTESIAN_POINT('Ctrl Pts',(-1.02502362238482,1.30000000000028,11.7667353284147));
#30178=CARTESIAN_POINT('Ctrl Pts',(-1.24813860795827,-1.30000000000129,
11.7429927856957));
#30179=CARTESIAN_POINT('Ctrl Pts',(-1.2264525293792,-1.18514270861269,11.6866859516542));
#30180=CARTESIAN_POINT('Ctrl Pts',(-1.20615493716576,-1.06847604194564,
11.6361391300789));
#30181=CARTESIAN_POINT('Ctrl Pts',(-1.16247111990375,-0.794772684000951,
11.5326726414666));
#30182=CARTESIAN_POINT('Ctrl Pts',(-1.13883908333676,-0.636309800095283,
11.4779589372101));
#30183=CARTESIAN_POINT('Ctrl Pts',(-1.10197370831211,-0.319434907277205,
11.4131688831434));
#30184=CARTESIAN_POINT('Ctrl Pts',(-1.08738397050814,-0.158333333333354,
11.3908083257058));
#30185=CARTESIAN_POINT('Ctrl Pts',(-1.06439414201174,0.158333333333356,
11.3965200012287));
#30186=CARTESIAN_POINT('Ctrl Pts',(-1.05691133021397,0.319434907277209,
11.4243254506344));
#30187=CARTESIAN_POINT('Ctrl Pts',(-1.04507964885187,0.636309800095292,
11.5012931953789));
#30188=CARTESIAN_POINT('Ctrl Pts',(-1.0416738801892,0.794772684000951,11.562919855076));
#30189=CARTESIAN_POINT('Ctrl Pts',(-1.04039339555115,1.06847604194533,11.6775759855885));
#30190=CARTESIAN_POINT('Ctrl Pts',(-1.04138798256821,1.18514270861209,11.7328848202995));
#30191=CARTESIAN_POINT('Ctrl Pts',(-1.04393143095552,1.3000000000004,11.793872099251));
#30192=CARTESIAN_POINT('Ctrl Pts',(-1.26978166142668,-1.30000000000132,
11.7689185967311));
#30193=CARTESIAN_POINT('Ctrl Pts',(-1.25073245999804,-1.18514270861273,
11.718424664199));
#30194=CARTESIAN_POINT('Ctrl Pts',(-1.23223782137633,-1.06847604194567,
11.6721762443729));
#30195=CARTESIAN_POINT('Ctrl Pts',(-1.19079265734443,-0.794772684000976,
11.575141126273));
#30196=CARTESIAN_POINT('Ctrl Pts',(-1.16623243927054,-0.636309800095297,
11.5195123009208));
#30197=CARTESIAN_POINT('Ctrl Pts',(-1.12774217801638,-0.319434907277209,
11.4555287799354));
#30198=CARTESIAN_POINT('Ctrl Pts',(-1.11016030267911,-0.158333333333357,
11.4320233662326));
#30199=CARTESIAN_POINT('Ctrl Pts',(-1.08625156130612,0.158333333333359,
11.4380535962252));
#30200=CARTESIAN_POINT('Ctrl Pts',(-1.08045831900887,0.319434907277216,
11.4674483189564));
#30201=CARTESIAN_POINT('Ctrl Pts',(-1.06916124243966,0.636309800095305,
11.5440020301027));
#30202=CARTESIAN_POINT('Ctrl Pts',(-1.06704328315777,0.794772684000967,
11.6063846328021));
#30203=CARTESIAN_POINT('Ctrl Pts',(-1.06311483577445,1.06847604194535,11.7148788223867));
#30204=CARTESIAN_POINT('Ctrl Pts',(-1.06207708456856,1.18514270861211,11.7660573346459));
#30205=CARTESIAN_POINT('Ctrl Pts',(-1.06170206146569,1.30000000000043,11.8214512445991));
#30206=CARTESIAN_POINT('Ctrl Pts',(-1.28621507340038,-1.30000000000135,
11.787444008607));
#30207=CARTESIAN_POINT('Ctrl Pts',(-1.27068858339734,-1.18514270861275,
11.7404565922239));
#30208=CARTESIAN_POINT('Ctrl Pts',(-1.25446887060034,-1.06847604194569,
11.6969042378102));
#30209=CARTESIAN_POINT('Ctrl Pts',(-1.21539660596413,-0.794772684000991,
11.6042252668273));
#30210=CARTESIAN_POINT('Ctrl Pts',(-1.1880682889676,-0.636309800095309,
11.5488823476501));
#30211=CARTESIAN_POINT('Ctrl Pts',(-1.14767980214843,-0.319434907277216,
11.4858445626509));
#30212=CARTESIAN_POINT('Ctrl Pts',(-1.1281592556255,-0.15833333333336,11.4614541561878));
#30213=CARTESIAN_POINT('Ctrl Pts',(-1.10345103237585,0.158333333333362,
11.4677753839338));
#30214=CARTESIAN_POINT('Ctrl Pts',(-1.09857321173,0.319434907277223,11.4983919872682));
#30215=CARTESIAN_POINT('Ctrl Pts',(-1.08800167231434,0.636309800095319,
11.574499229092));
#30216=CARTESIAN_POINT('Ctrl Pts',(-1.08784105687488,0.794772684000983,
11.6370517121057));
#30217=CARTESIAN_POINT('Ctrl Pts',(-1.08213675247853,1.06847604194537,11.7410213750434));
#30218=CARTESIAN_POINT('Ctrl Pts',(-1.07948736551723,1.18514270861213,11.7892559936534));
#30219=CARTESIAN_POINT('Ctrl Pts',(-1.07665777360248,1.30000000000045,11.8407206162434));
#30220=CARTESIAN_POINT('Ctrl Pts',(-1.2988477852273,-1.30000000000137,11.8011898160843));
#30221=CARTESIAN_POINT('Ctrl Pts',(-1.28496304689735,-1.18514270861276,
11.7572780526074));
#30222=CARTESIAN_POINT('Ctrl Pts',(-1.26981948734302,-1.0684760419457,11.7160274702605));
#30223=CARTESIAN_POINT('Ctrl Pts',(-1.23192670645918,-0.794772684001,11.626878233666));
#30224=CARTESIAN_POINT('Ctrl Pts',(-1.20339270808647,-0.636309800095317,
11.5713448845443));
#30225=CARTESIAN_POINT('Ctrl Pts',(-1.16227892917472,-0.31943490727722,
11.5087171233327));
#30226=CARTESIAN_POINT('Ctrl Pts',(-1.14202028849874,-0.158333333333362,
11.4833758052458));
#30227=CARTESIAN_POINT('Ctrl Pts',(-1.11698880932356,0.158333333333364,
11.4898111602895));
#30228=CARTESIAN_POINT('Ctrl Pts',(-1.11265992653266,0.319434907277227,
11.5214253283881));
#30229=CARTESIAN_POINT('Ctrl Pts',(-1.10188207887894,0.636309800095326,
11.5974924555126));
#30230=CARTESIAN_POINT('Ctrl Pts',(-1.10178142294354,0.794772684000993,
11.6607002318859));
#30231=CARTESIAN_POINT('Ctrl Pts',(-1.0944826956649,1.06847604194539,11.7613683248178));
#30232=CARTESIAN_POINT('Ctrl Pts',(-1.09080071657814,1.18514270861215,11.8073233566545));
#30233=CARTESIAN_POINT('Ctrl Pts',(-1.08659610699906,1.30000000000047,11.855657933018));
#30234=CARTESIAN_POINT('Ctrl Pts',(-1.30959903943834,-1.3000000000014,11.8125295228691));
#30235=CARTESIAN_POINT('Ctrl Pts',(-1.2975816101224,-1.1851427086128,11.7709505876381));
#30236=CARTESIAN_POINT('Ctrl Pts',(-1.28368627549302,-1.06847604194573,
11.7314592499347));
#30237=CARTESIAN_POINT('Ctrl Pts',(-1.24724693579931,-0.794772684001022,
11.6450491275368));
#30238=CARTESIAN_POINT('Ctrl Pts',(-1.21760067785406,-0.636309800095336,
11.5894346271556));
#30239=CARTESIAN_POINT('Ctrl Pts',(-1.17564743019148,-0.319434907277229,
11.5272668765828));
#30240=CARTESIAN_POINT('Ctrl Pts',(-1.15418812004909,-0.158333333333367,
11.5013861396723));
#30241=CARTESIAN_POINT('Ctrl Pts',(-1.12885531704681,0.158333333333369,
11.5079362390012));
#30242=CARTESIAN_POINT('Ctrl Pts',(-1.12525652825615,0.319434907277237,
11.5402551178548));
#30243=CARTESIAN_POINT('Ctrl Pts',(-1.11504912781576,0.636309800095346,
11.615992998271));
#30244=CARTESIAN_POINT('Ctrl Pts',(-1.11630139094869,0.794772684001016,
11.6792370475013));
#30245=CARTESIAN_POINT('Ctrl Pts',(-1.10760457044329,1.06847604194542,11.7771924105374));
#30246=CARTESIAN_POINT('Ctrl Pts',(-1.10269037666985,1.18514270861218,11.8214012181949));
#30247=CARTESIAN_POINT('Ctrl Pts',(-1.09662652047079,1.3000000000005,11.8674175864555));
#30248=CARTESIAN_POINT('Ctrl Pts',(-1.31760194267207,-1.30000000000141,
11.8218663161006));
#30249=CARTESIAN_POINT('Ctrl Pts',(-1.30740878936986,-1.1851427086128,11.7820012977114));
#30250=CARTESIAN_POINT('Ctrl Pts',(-1.29473728074604,-1.06847604194573,
11.7438139784362));
#30251=CARTESIAN_POINT('Ctrl Pts',(-1.25973806431227,-0.794772684001023,
11.6594694521398));
#30252=CARTESIAN_POINT('Ctrl Pts',(-1.22907848423481,-0.636309800095337,
11.6038553909907));
#30253=CARTESIAN_POINT('Ctrl Pts',(-1.18625025075386,-0.31943490727723,
11.5421425696291));
#30254=CARTESIAN_POINT('Ctrl Pts',(-1.1635032970347,-0.158333333333367,
11.5159615935396));
#30255=CARTESIAN_POINT('Ctrl Pts',(-1.13773612695948,0.158333333333369,
11.5226872205802));
#30256=CARTESIAN_POINT('Ctrl Pts',(-1.13489948120314,0.319434907277237,
11.555508014619));
#30257=CARTESIAN_POINT('Ctrl Pts',(-1.12486792444456,0.636309800095347,
11.6310952409414));
#30258=CARTESIAN_POINT('Ctrl Pts',(-1.12656133963866,0.794772684001018,
11.6946178963244));
#30259=CARTESIAN_POINT('Ctrl Pts',(-1.11669649677285,1.06847604194542,11.7904131544161));
#30260=CARTESIAN_POINT('Ctrl Pts',(-1.11091640428911,1.18514270861219,11.8331719559363));
#30261=CARTESIAN_POINT('Ctrl Pts',(-1.1036263442698,1.30000000000051,11.8772233413129));
#30262=CARTESIAN_POINT('Ctrl Pts',(-1.33044578595549,-1.30000000000145,
11.8354926488634));
#30263=CARTESIAN_POINT('Ctrl Pts',(-1.32211288865797,-1.18514270861284,
11.7986019247905));
#30264=CARTESIAN_POINT('Ctrl Pts',(-1.31068800059481,-1.06847604194577,
11.7626398529816));
#30265=CARTESIAN_POINT('Ctrl Pts',(-1.27715110640868,-0.794772684001048,
11.6817056454209));
#30266=CARTESIAN_POINT('Ctrl Pts',(-1.2453022793547,-0.636309800095356,
11.6259099815901));
#30267=CARTESIAN_POINT('Ctrl Pts',(-1.20186071890905,-0.319434907277239,
11.5645749966149));
#30268=CARTESIAN_POINT('Ctrl Pts',(-1.17821381724787,-0.158333333333372,
11.5375213000565));
#30269=CARTESIAN_POINT('Ctrl Pts',(-1.15255006747905,0.158333333333374,
11.5441900625005));
#30270=CARTESIAN_POINT('Ctrl Pts',(-1.15106019695707,0.319434907277248,
11.577668514768));
#30271=CARTESIAN_POINT('Ctrl Pts',(-1.14115313157659,0.636309800095367,
11.6530843128247));
#30272=CARTESIAN_POINT('Ctrl Pts',(-1.14280855344883,0.794772684001041,
11.7173201381379));
#30273=CARTESIAN_POINT('Ctrl Pts',(-1.13081458063189,1.06847604194545,11.810038109084));
#30274=CARTESIAN_POINT('Ctrl Pts',(-1.12363899130074,1.18514270861222,11.8506655484021));
#30275=CARTESIAN_POINT('Ctrl Pts',(-1.11447955905041,1.30000000000055,11.8917862529552));
#30276=CARTESIAN_POINT('Ctrl Pts',(-1.34601296172094,-1.30000000000148,
11.8510707826578));
#30277=CARTESIAN_POINT('Ctrl Pts',(-1.34132286698166,-1.18514270861287,
11.8169387564616));
#30278=CARTESIAN_POINT('Ctrl Pts',(-1.33229750149764,-1.0684760419458,11.7831228063995));
#30279=CARTESIAN_POINT('Ctrl Pts',(-1.30143175902319,-0.794772684001073,
11.705731395999));
#30280=CARTESIAN_POINT('Ctrl Pts',(-1.26715729948021,-0.636309800095377,
11.6502915199856));
#30281=CARTESIAN_POINT('Ctrl Pts',(-1.22185490916071,-0.31943490727725,
11.5899544953272));
#30282=CARTESIAN_POINT('Ctrl Pts',(-1.19616941707238,-0.158333333333377,
11.5623270871317));
#30283=CARTESIAN_POINT('Ctrl Pts',(-1.16909862965114,0.158333333333379,
11.5695937788591));
#30284=CARTESIAN_POINT('Ctrl Pts',(-1.16747959347913,0.319434907277257,
11.6045326774201));
#30285=CARTESIAN_POINT('Ctrl Pts',(-1.15811685224228,0.636309800095386,
11.679580178308));
#30286=CARTESIAN_POINT('Ctrl Pts',(-1.16292009703033,0.794772684001067,
11.7433177695099));
#30287=CARTESIAN_POINT('Ctrl Pts',(-1.1489448495103,1.06847604194549,11.8322318725625));
#30288=CARTESIAN_POINT('Ctrl Pts',(-1.13981020907389,1.18514270861226,11.8705080987032));
#30289=CARTESIAN_POINT('Ctrl Pts',(-1.12759029501853,1.30000000000059,11.9085729303654));
#30290=CARTESIAN_POINT('Ctrl Pts',(-1.36294346109262,-1.30000000000156,
11.8692837620561));
#30291=CARTESIAN_POINT('Ctrl Pts',(-1.36085923751846,-1.18514270861294,
11.8390475820273));
#30292=CARTESIAN_POINT('Ctrl Pts',(-1.35373219611573,-1.06847604194586,
11.8080843650971));
#30293=CARTESIAN_POINT('Ctrl Pts',(-1.32561738671945,-0.794772684001115,
11.7348735391328));
#30294=CARTESIAN_POINT('Ctrl Pts',(-1.29114039687238,-0.63630980009541,
11.6785797244191));
#30295=CARTESIAN_POINT('Ctrl Pts',(-1.24520756634855,-0.319434907277266,
11.6186826600773));
#30296=CARTESIAN_POINT('Ctrl Pts',(-1.21710945792495,-0.158333333333386,
11.5904617895211));
#30297=CARTESIAN_POINT('Ctrl Pts',(-1.18990665017216,0.158333333333388,
11.5977907775527));
#30298=CARTESIAN_POINT('Ctrl Pts',(-1.19077150633563,0.319434907277275,
11.6332977744102));
#30299=CARTESIAN_POINT('Ctrl Pts',(-1.18135618940353,0.636309800095421,
11.7082107659264));
#30300=CARTESIAN_POINT('Ctrl Pts',(-1.185167714955,0.794772684001107,11.7732961672384));
#30301=CARTESIAN_POINT('Ctrl Pts',(-1.16816485771141,1.06847604194554,11.8582057977702));
#30302=CARTESIAN_POINT('Ctrl Pts',(-1.15725060624733,1.18514270861232,11.8936182187079));
#30303=CARTESIAN_POINT('Ctrl Pts',(-1.14278201020198,1.30000000000066,11.9276888277378));
#30304=CARTESIAN_POINT('Ctrl Pts',(-1.38080148305821,-1.30000000000158,
11.8870097673586));
#30305=CARTESIAN_POINT('Ctrl Pts',(-1.38268370064567,-1.18514270861296,
11.8599975752852));
#30306=CARTESIAN_POINT('Ctrl Pts',(-1.37819135820682,-1.06847604194587,
11.8315245282412));
#30307=CARTESIAN_POINT('Ctrl Pts',(-1.35308663959594,-0.794772684001128,
11.7623712263315));
#30308=CARTESIAN_POINT('Ctrl Pts',(-1.31591355523754,-0.636309800095421,
11.7064557387738));
#30309=CARTESIAN_POINT('Ctrl Pts',(-1.26851148105121,-0.319434907277273,
11.6474327241946));
#30310=CARTESIAN_POINT('Ctrl Pts',(-1.23889908635022,-0.158333333333388,
11.6182288910649));
#30311=CARTESIAN_POINT('Ctrl Pts',(-1.21089672311666,0.15833333333339,11.6259113968901));
#30312=CARTESIAN_POINT('Ctrl Pts',(-1.2122289967891,0.319434907277279,11.6628308932153));
#30313=CARTESIAN_POINT('Ctrl Pts',(-1.20315804593487,0.636309800095431,
11.7374350798258));
#30314=CARTESIAN_POINT('Ctrl Pts',(-1.20910091955257,0.794772684001122,
11.8025396611556));
#30315=CARTESIAN_POINT('Ctrl Pts',(-1.1894709900496,1.06847604194556,11.8832732309525));
#30316=CARTESIAN_POINT('Ctrl Pts',(-1.1763930513816,1.18514270861235,11.9159850016308));
#30317=CARTESIAN_POINT('Ctrl Pts',(-1.15873424316685,1.30000000000068,11.9464619720958));
#30318=CARTESIAN_POINT('Ctrl Pts',(-1.40367537834943,-1.30000000000185,
11.9089012603341));
#30319=CARTESIAN_POINT('Ctrl Pts',(-1.40935748512326,-1.18514270861321,
11.8864595634616));
#30320=CARTESIAN_POINT('Ctrl Pts',(-1.40753829200455,-1.0684760419461,11.8613849877698));
#30321=CARTESIAN_POINT('Ctrl Pts',(-1.38600608859034,-0.794772684001295,
11.797375224992));
#30322=CARTESIAN_POINT('Ctrl Pts',(-1.34749195158982,-0.636309800095552,
11.7409488864709));
#30323=CARTESIAN_POINT('Ctrl Pts',(-1.29928584878208,-0.319434907277337,
11.6825333798681));
#30324=CARTESIAN_POINT('Ctrl Pts',(-1.26776917595437,-0.158333333333421,
11.652128053469));
#30325=CARTESIAN_POINT('Ctrl Pts',(-1.23919953259728,0.158333333333423,
11.6600812250877));
#30326=CARTESIAN_POINT('Ctrl Pts',(-1.24175730414977,0.319434907277347,
11.6985117560777));
#30327=CARTESIAN_POINT('Ctrl Pts',(-1.23256199087342,0.636309800095563,
11.7729805746429));
#30328=CARTESIAN_POINT('Ctrl Pts',(-1.23944606917772,0.794772684001284,
11.8388334060565));
#30329=CARTESIAN_POINT('Ctrl Pts',(-1.21591616791004,1.06847604194578,11.9146313246069));
#30330=CARTESIAN_POINT('Ctrl Pts',(-1.20012062657232,1.18514270861259,11.9439876297299));
#30331=CARTESIAN_POINT('Ctrl Pts',(-1.17871476628688,1.30000000000095,11.9698901296249));
#30332=CARTESIAN_POINT('Ctrl Pts',(-1.42403899407475,-1.30000000000203,
11.928642082633));
#30333=CARTESIAN_POINT('Ctrl Pts',(-1.43380199579919,-1.18514270861337,
11.9099752094577));
#30334=CARTESIAN_POINT('Ctrl Pts',(-1.43486664397214,-1.06847604194625,
11.8877166093531));
#30335=CARTESIAN_POINT('Ctrl Pts',(-1.41723125743024,-0.794772684001406,
11.8279971825649));
#30336=CARTESIAN_POINT('Ctrl Pts',(-1.37753694095029,-0.636309800095641,
11.7711162197193));
#30337=CARTESIAN_POINT('Ctrl Pts',(-1.32822206778928,-0.319434907277382,
11.7134532616262));
#30338=CARTESIAN_POINT('Ctrl Pts',(-1.29406704705413,-0.158333333333443,
11.6824351194661));
#30339=CARTESIAN_POINT('Ctrl Pts',(-1.26458135603709,0.158333333333445,
11.6908365801527));
#30340=CARTESIAN_POINT('Ctrl Pts',(-1.26843559089466,0.319434907277389,
11.7305157631943));
#30341=CARTESIAN_POINT('Ctrl Pts',(-1.2593505240363,0.63630980009565,11.8047631456141));
#30342=CARTESIAN_POINT('Ctrl Pts',(-1.26759011506683,0.794772684001396,
11.8710693152954));
#30343=CARTESIAN_POINT('Ctrl Pts',(-1.24048368122056,1.06847604194593,11.9424659259234));
#30344=CARTESIAN_POINT('Ctrl Pts',(-1.22207813922907,1.18514270861276,11.9688815272328));
#30345=CARTESIAN_POINT('Ctrl Pts',(-1.19700042606577,1.30000000000113,11.9908077826161));
#30346=CARTESIAN_POINT('Ctrl Pts',(-1.43801335595633,-1.30000000000206,
11.9415958604667));
#30347=CARTESIAN_POINT('Ctrl Pts',(-1.45045410381386,-1.1851427086134,11.9254578817525));
#30348=CARTESIAN_POINT('Ctrl Pts',(-1.4533968558968,-1.06847604194628,11.9050925216825));
#30349=CARTESIAN_POINT('Ctrl Pts',(-1.43825293159713,-0.794772684001427,
11.8482783692284));
#30350=CARTESIAN_POINT('Ctrl Pts',(-1.39770343358077,-0.63630980009566,
11.7911317326));
#30351=CARTESIAN_POINT('Ctrl Pts',(-1.34753037301524,-0.319434907277392,
11.7340335593344));
#30352=CARTESIAN_POINT('Ctrl Pts',(-1.31138241616195,-0.158333333333447,
11.7027255806159));
#30353=CARTESIAN_POINT('Ctrl Pts',(-1.2815345070826,0.158333333333449,11.7113147339748));
#30354=CARTESIAN_POINT('Ctrl Pts',(-1.28684467285541,0.319434907277397,
11.7515472889145));
#30355=CARTESIAN_POINT('Ctrl Pts',(-1.27823601010953,0.636309800095668,
11.8254577169132));
#30356=CARTESIAN_POINT('Ctrl Pts',(-1.2875886999882,0.79477268400142,11.8919654946004));
#30357=CARTESIAN_POINT('Ctrl Pts',(-1.25784477511212,1.06847604194596,11.9605474333257));
#30358=CARTESIAN_POINT('Ctrl Pts',(-1.23745341248982,1.18514270861279,11.9851188877207));
#30359=CARTESIAN_POINT('Ctrl Pts',(-1.20954573020305,1.30000000000117,12.0045752164476));
#30360=CARTESIAN_POINT('Ctrl Pts',(-1.44396187751701,-1.30000000000207,
11.9469208090408));
#30361=CARTESIAN_POINT('Ctrl Pts',(-1.45765536941502,-1.18514270861341,
11.9317612245756));
#30362=CARTESIAN_POINT('Ctrl Pts',(-1.46144721273248,-1.06847604194628,
11.9121479982828));
#30363=CARTESIAN_POINT('Ctrl Pts',(-1.44733234031239,-0.794772684001432,
11.8565487183647));
#30364=CARTESIAN_POINT('Ctrl Pts',(-1.4060424781856,-0.636309800095663,
11.7994964200841));
#30365=CARTESIAN_POINT('Ctrl Pts',(-1.35553317450774,-0.319434907277393,
11.742630923621));
#30366=CARTESIAN_POINT('Ctrl Pts',(-1.31898795487292,-0.158333333333448,
11.7109906847985));
#30367=CARTESIAN_POINT('Ctrl Pts',(-1.28892906680916,0.15833333333345,11.7196848459155));
#30368=CARTESIAN_POINT('Ctrl Pts',(-1.29444895487496,0.319434907277399,
11.7603361927813));
#30369=CARTESIAN_POINT('Ctrl Pts',(-1.28569904371272,0.636309800095671,
11.8342654713718));
#30370=CARTESIAN_POINT('Ctrl Pts',(-1.29521836752735,0.794772684001424,
11.9009938121065));
#30371=CARTESIAN_POINT('Ctrl Pts',(-1.26446650997392,1.06847604194597,11.9683622590465));
#30372=CARTESIAN_POINT('Ctrl Pts',(-1.2433984560899,1.18514270861279,11.9920964705687));
#30373=CARTESIAN_POINT('Ctrl Pts',(-1.21457368798812,1.30000000000117,12.0104035891798));
#30374=CARTESIAN_POINT('Ctrl Pts',(-1.44878160869613,-1.30000000000208,
11.9511471654546));
#30375=CARTESIAN_POINT('Ctrl Pts',(-1.46353970026319,-1.18514270861342,
11.9367371319072));
#30376=CARTESIAN_POINT('Ctrl Pts',(-1.46804432840997,-1.06847604194629,
11.9177076628513));
#30377=CARTESIAN_POINT('Ctrl Pts',(-1.45476336887771,-0.794772684001439,
11.8630739623605));
#30378=CARTESIAN_POINT('Ctrl Pts',(-1.41275083453451,-0.636309800095669,
11.8061639179291));
#30379=CARTESIAN_POINT('Ctrl Pts',(-1.36196014505706,-0.319434907277397,
11.7494932131841));
#30380=CARTESIAN_POINT('Ctrl Pts',(-1.32517039522566,-0.158333333333449,
11.7175531446848));
#30381=CARTESIAN_POINT('Ctrl Pts',(-1.29497962595988,0.158333333333452,
11.7263151673183));
#30382=CARTESIAN_POINT('Ctrl Pts',(-1.30068393443965,0.319434907277402,
11.7672942672444));
#30383=CARTESIAN_POINT('Ctrl Pts',(-1.29180058335059,0.636309800095677,
11.8412483342407));
#30384=CARTESIAN_POINT('Ctrl Pts',(-1.30139627601783,0.794772684001432,
11.9081786650871));
#30385=CARTESIAN_POINT('Ctrl Pts',(-1.26979718785685,1.06847604194598,11.9745958920687));
#30386=CARTESIAN_POINT('Ctrl Pts',(-1.2481741555375,1.18514270861281,11.9976671741239));
#30387=CARTESIAN_POINT('Ctrl Pts',(-1.21860616530208,1.30000000000119,12.0150601816748));
#30388=CARTESIAN_POINT('Ctrl Pts',(-1.45176259299563,-1.30000000000209,
11.9538042732137));
#30389=CARTESIAN_POINT('Ctrl Pts',(-1.46715758972206,-1.18514270861342,
11.9398775948973));
#30390=CARTESIAN_POINT('Ctrl Pts',(-1.47209725699402,-1.0684760419463,11.9212184413938));
#30391=CARTESIAN_POINT('Ctrl Pts',(-1.45935497394801,-0.794772684001442,
11.867179099639));
#30392=CARTESIAN_POINT('Ctrl Pts',(-1.41699570354255,-0.636309800095672,
11.8103031424495));
#30393=CARTESIAN_POINT('Ctrl Pts',(-1.36604424570276,-0.319434907277398,
11.7537462514445));
#30394=CARTESIAN_POINT('Ctrl Pts',(-1.32902683726316,-0.15833333333345,
11.7216575833153));
#30395=CARTESIAN_POINT('Ctrl Pts',(-1.29874790973121,0.158333333333452,
11.7304654392766));
#30396=CARTESIAN_POINT('Ctrl Pts',(-1.30460577039528,0.319434907277404,
11.7716298189423));
#30397=CARTESIAN_POINT('Ctrl Pts',(-1.29567499303704,0.63630980009568,11.8455820758332));
#30398=CARTESIAN_POINT('Ctrl Pts',(-1.30536656523558,0.794772684001435,
11.9126164899123));
#30399=CARTESIAN_POINT('Ctrl Pts',(-1.27321744712993,1.06847604194598,11.9784488600289));
#30400=CARTESIAN_POINT('Ctrl Pts',(-1.25122125180277,1.18514270861281,12.0011181309178));
#30401=CARTESIAN_POINT('Ctrl Pts',(-1.22114502313416,1.30000000000119,12.0179602790019));
#30402=CARTESIAN_POINT('Ctrl Pts',(-1.45412628658392,-1.30000000000209,
11.9559408461953));
#30403=CARTESIAN_POINT('Ctrl Pts',(-1.47000738429716,-1.18514270861343,
11.9424131581336));
#30404=CARTESIAN_POINT('Ctrl Pts',(-1.47528578223223,-1.0684760419463,11.9240551310158));
#30405=CARTESIAN_POINT('Ctrl Pts',(-1.46298557985177,-0.794772684001444,
11.8704853663371));
#30406=CARTESIAN_POINT('Ctrl Pts',(-1.42043011327194,-0.636309800095673,
11.8135940727104));
#30407=CARTESIAN_POINT('Ctrl Pts',(-1.3693582354536,-0.319434907277399,
11.7571235736978));
#30408=CARTESIAN_POINT('Ctrl Pts',(-1.33209230895348,-0.15833333333345,
11.7249498649193));
#30409=CARTESIAN_POINT('Ctrl Pts',(-1.30174447208215,0.158333333333453,
11.7337942228324));
#30410=CARTESIAN_POINT('Ctrl Pts',(-1.30777075626328,0.319434907277404,
11.7750844319782));
#30411=CARTESIAN_POINT('Ctrl Pts',(-1.29884281897625,0.636309800095681,
11.8490159166609));
#30412=CARTESIAN_POINT('Ctrl Pts',(-1.30865687160089,0.794772684001436,
11.9161124935271));
#30413=CARTESIAN_POINT('Ctrl Pts',(-1.27604818827047,1.06847604194599,11.9814861394346));
#30414=CARTESIAN_POINT('Ctrl Pts',(-1.25372777969796,1.18514270861281,12.0038457928843));
#30415=CARTESIAN_POINT('Ctrl Pts',(-1.22320205329589,1.30000000000119,12.0202672708026));
#30416=CARTESIAN_POINT('Ctrl Pts',(-1.45559309281896,-1.30000000000209,
11.9572815917638));
#30417=CARTESIAN_POINT('Ctrl Pts',(-1.47176684857772,-1.18514270861343,
11.9440091015764));
#30418=CARTESIAN_POINT('Ctrl Pts',(-1.47725243245924,-1.0684760419463,11.9258416345089));
#30419=CARTESIAN_POINT('Ctrl Pts',(-1.46523341341502,-0.794772684001445,
11.8725627753639));
#30420=CARTESIAN_POINT('Ctrl Pts',(-1.42259258598767,-0.636309800095674,
11.8156424353714));
#30421=CARTESIAN_POINT('Ctrl Pts',(-1.37145024444862,-0.319434907277399,
11.7592232784206));
#30422=CARTESIAN_POINT('Ctrl Pts',(-1.3340014901361,-0.158333333333451,
11.7270104289212));
#30423=CARTESIAN_POINT('Ctrl Pts',(-1.30360964329911,0.158333333333453,
11.7358782684999));
#30424=CARTESIAN_POINT('Ctrl Pts',(-1.30975675245054,0.319434907277405,
11.7772393990036));
#30425=CARTESIAN_POINT('Ctrl Pts',(-1.30084628394672,0.636309800095682,
11.8511504676796));
#30426=CARTESIAN_POINT('Ctrl Pts',(-1.31075692417128,0.794772684001437,
11.9182766599752));
#30427=CARTESIAN_POINT('Ctrl Pts',(-1.27785446166952,1.06847604194599,11.9833667142888));
#30428=CARTESIAN_POINT('Ctrl Pts',(-1.2553216991526,1.18514270861281,12.0055374169981));
#30429=CARTESIAN_POINT('Ctrl Pts',(-1.22449843097937,1.3000000000012,12.0217037497287));
#30430=CARTESIAN_POINT('Ctrl Pts',(-1.45676183409782,-1.30000000000209,
11.9583565852924));
#30431=CARTESIAN_POINT('Ctrl Pts',(-1.47316443878281,-1.18514270861343,
11.9452909967571));
#30432=CARTESIAN_POINT('Ctrl Pts',(-1.47881367935989,-1.0684760419463,11.9272770581855));
#30433=CARTESIAN_POINT('Ctrl Pts',(-1.46702213292725,-0.794772684001445,
11.8742295779112));
#30434=CARTESIAN_POINT('Ctrl Pts',(-1.42433097171468,-0.636309800095674,
11.8172766283104));
#30435=CARTESIAN_POINT('Ctrl Pts',(-1.37313484211759,-0.319434907277399,
11.7608971357158));
#30436=CARTESIAN_POINT('Ctrl Pts',(-1.33552682586702,-0.158333333333451,
11.728659596914));
#30437=CARTESIAN_POINT('Ctrl Pts',(-1.3050996718648,0.158333333333453,11.7375463919935));
#30438=CARTESIAN_POINT('Ctrl Pts',(-1.31135108710863,0.319434907277405,
11.7789604974073));
#30439=CARTESIAN_POINT('Ctrl Pts',(-1.30246251145676,0.636309800095682,
11.8528515079605));
#30440=CARTESIAN_POINT('Ctrl Pts',(-1.31246056688986,0.794772684001438,
11.9199967060572));
#30441=CARTESIAN_POINT('Ctrl Pts',(-1.27931974389209,1.06847604194599,11.9848614994968));
#30442=CARTESIAN_POINT('Ctrl Pts',(-1.25661216601513,1.18514270861282,12.0068833729769));
#30443=CARTESIAN_POINT('Ctrl Pts',(-1.22554244454843,1.3000000000012,12.0228495543345));
#30444=CARTESIAN_POINT('Ctrl Pts',(-1.4576362468158,-1.3000000000021,11.959163908753));
#30445=CARTESIAN_POINT('Ctrl Pts',(-1.4742081978252,-1.18514270861343,11.9462546785736));
#30446=CARTESIAN_POINT('Ctrl Pts',(-1.4799792929871,-1.0684760419463,11.9283563400937));
#30447=CARTESIAN_POINT('Ctrl Pts',(-1.46835953960324,-0.794772684001445,
11.8754817594131));
#30448=CARTESIAN_POINT('Ctrl Pts',(-1.42563846320108,-0.636309800095674,
11.8185002733194));
#30449=CARTESIAN_POINT('Ctrl Pts',(-1.37440343715322,-0.319434907277399,
11.7621497596797));
#30450=CARTESIAN_POINT('Ctrl Pts',(-1.33667091322058,-0.158333333333451,
11.7298962906598));
#30451=CARTESIAN_POINT('Ctrl Pts',(-1.30621714597304,0.158333333333453,
11.7387974184199));
#30452=CARTESIAN_POINT('Ctrl Pts',(-1.31254933061953,0.319434907277405,
11.7802500019729));
#30453=CARTESIAN_POINT('Ctrl Pts',(-1.30368032461536,0.636309800095682,
11.8541244943568));
#30454=CARTESIAN_POINT('Ctrl Pts',(-1.31374852051673,0.794772684001438,
11.9212818216884));
#30455=CARTESIAN_POINT('Ctrl Pts',(-1.28042768257437,1.06847604194599,11.9859782900626));
#30456=CARTESIAN_POINT('Ctrl Pts',(-1.25758697978893,1.18514270861282,12.0078895053538));
#30457=CARTESIAN_POINT('Ctrl Pts',(-1.22632893030456,1.3000000000012,12.0237072320175));
#30458=CARTESIAN_POINT('Ctrl Pts',(-1.45836365863242,-1.3000000000021,11.9598373036628));
#30459=CARTESIAN_POINT('Ctrl Pts',(-1.47507522896852,-1.18514270861343,
11.9470591421206));
#30460=CARTESIAN_POINT('Ctrl Pts',(-1.48094730564884,-1.0684760419463,11.9292574217479));
#30461=CARTESIAN_POINT('Ctrl Pts',(-1.46947157870716,-0.794772684001446,
11.8765264606078));
#30462=CARTESIAN_POINT('Ctrl Pts',(-1.42673088476929,-0.636309800095674,
11.819518434425));
#30463=CARTESIAN_POINT('Ctrl Pts',(-1.37546443483945,-0.319434907277399,
11.7631915487841));
#30464=CARTESIAN_POINT('Ctrl Pts',(-1.33762471405457,-0.158333333333451,
11.7309265675717));
#30465=CARTESIAN_POINT('Ctrl Pts',(-1.30714867482229,0.158333333333453,
11.7398397251137));
#30466=CARTESIAN_POINT('Ctrl Pts',(-1.31354993392347,0.319434907277405,
11.7813235032592));
#30467=CARTESIAN_POINT('Ctrl Pts',(-1.30469927152157,0.636309800095682,
11.8551832836116));
#30468=CARTESIAN_POINT('Ctrl Pts',(-1.31482873251949,0.794772684001438,
11.922349417857));
#30469=CARTESIAN_POINT('Ctrl Pts',(-1.28135710266374,1.06847604194599,11.9869060154245));
#30470=CARTESIAN_POINT('Ctrl Pts',(-1.2584042056035,1.18514270861282,12.0087256230431));
#30471=CARTESIAN_POINT('Ctrl Pts',(-1.22698703980146,1.3000000000012,12.0244206792509));
#30472=CARTESIAN_POINT('Ctrl Pts',(-1.45887229050876,-1.3000000000021,11.9603089447196));
#30473=CARTESIAN_POINT('Ctrl Pts',(-1.47568111425946,-1.18514270861343,
11.9476227686205));
#30474=CARTESIAN_POINT('Ctrl Pts',(-1.4816237270335,-1.0684760419463,11.9298887510696));
#30475=CARTESIAN_POINT('Ctrl Pts',(-1.47024923022303,-0.794772684001445,
11.8772580992783));
#30476=CARTESIAN_POINT('Ctrl Pts',(-1.42749660001604,-0.636309800095674,
11.8202305657825));
#30477=CARTESIAN_POINT('Ctrl Pts',(-1.37620887221738,-0.319434907277399,
11.7639198533448));
#30478=CARTESIAN_POINT('Ctrl Pts',(-1.33829358685617,-0.158333333333451,
11.7316470933858));
#30479=CARTESIAN_POINT('Ctrl Pts',(-1.3078020088344,0.158333333333453,11.7405686639439));
#30480=CARTESIAN_POINT('Ctrl Pts',(-1.31425157265155,0.319434907277405,
11.7820743088889));
#30481=CARTESIAN_POINT('Ctrl Pts',(-1.30541441170054,0.636309800095682,
11.8559234931048));
#30482=CARTESIAN_POINT('Ctrl Pts',(-1.31558828822311,0.794772684001438,
11.9230950654863));
#30483=CARTESIAN_POINT('Ctrl Pts',(-1.28201086412561,1.06847604194599,11.9875538956265));
#30484=CARTESIAN_POINT('Ctrl Pts',(-1.25897891196976,1.18514270861282,12.0093096412464));
#30485=CARTESIAN_POINT('Ctrl Pts',(-1.22744943038369,1.3000000000012,12.0249192933534));
#30486=CARTESIAN_POINT('Ctrl Pts',(-1.45916293603873,-1.3000000000021,11.9605784516738));
#30487=CARTESIAN_POINT('Ctrl Pts',(-1.47602712731174,-1.18514270861343,
11.9479449470715));
#30488=CARTESIAN_POINT('Ctrl Pts',(-1.4820099641168,-1.0684760419463,11.9302496611076));
#30489=CARTESIAN_POINT('Ctrl Pts',(-1.47069340837042,-0.794772684001446,
11.8776762830501));
#30490=CARTESIAN_POINT('Ctrl Pts',(-1.42793473453064,-0.636309800095675,
11.8206372037096));
#30491=CARTESIAN_POINT('Ctrl Pts',(-1.3766347835925,-0.319434907277399,
11.7643357655358));
#30492=CARTESIAN_POINT('Ctrl Pts',(-1.33867549238525,-0.158333333333451,
11.7320589818148));
#30493=CARTESIAN_POINT('Ctrl Pts',(-1.30817489300452,0.158333333333453,
11.7409854326848));
#30494=CARTESIAN_POINT('Ctrl Pts',(-1.31465257256766,0.319434907277405,
11.7825033107204));
#30495=CARTESIAN_POINT('Ctrl Pts',(-1.30582325002853,0.636309800095683,
11.8563463805486));
#30496=CARTESIAN_POINT('Ctrl Pts',(-1.31602229180613,0.794772684001438,
11.9235211783992));
#30497=CARTESIAN_POINT('Ctrl Pts',(-1.28238440586926,1.06847604194599,11.9879241441032));
#30498=CARTESIAN_POINT('Ctrl Pts',(-1.25930730372606,1.18514270861282,12.0096433818638));
#30499=CARTESIAN_POINT('Ctrl Pts',(-1.22771369385523,1.3000000000012,12.025204199897));
#30500=CARTESIAN_POINT('Ctrl Pts',(-1.46859907610557,-1.30000000000203,
11.9693420881502));
#30501=CARTESIAN_POINT('Ctrl Pts',(-1.48726728132861,-1.18514270861337,
11.9584176006989));
#30502=CARTESIAN_POINT('Ctrl Pts',(-1.49456034141824,-1.06847604194625,
11.9419792378749));
#30503=CARTESIAN_POINT('Ctrl Pts',(-1.48512990834886,-0.794772684001404,
11.8912651761098));
#30504=CARTESIAN_POINT('Ctrl Pts',(-1.44215958086142,-0.636309800095641,
11.8338586014427));
#30505=CARTESIAN_POINT('Ctrl Pts',(-1.3904826145155,-0.319434907277382,
11.777848370173));
#30506=CARTESIAN_POINT('Ctrl Pts',(-1.35113949190814,-0.158333333333443,
11.7454174913081));
#30507=CARTESIAN_POINT('Ctrl Pts',(-1.32035617945323,0.158333333333445,
11.7544976139884));
#30508=CARTESIAN_POINT('Ctrl Pts',(-1.3277105057882,0.319434907277389,11.796432143158));
#30509=CARTESIAN_POINT('Ctrl Pts',(-1.31913956487404,0.636309800095649,
11.8700752352614));
#30510=CARTESIAN_POINT('Ctrl Pts',(-1.33020018471009,0.794772684001394,
11.9373330247913));
#30511=CARTESIAN_POINT('Ctrl Pts',(-1.29459393804896,1.06847604194593,11.999922806806));
#30512=CARTESIAN_POINT('Ctrl Pts',(-1.27003842655761,1.18514270861275,12.0204614781535));
#30513=CARTESIAN_POINT('Ctrl Pts',(-1.23634002841306,1.30000000000113,12.0344460233943));
#30514=CARTESIAN_POINT('Ctrl Pts',(-1.48344548007622,-1.30000000000141,
11.9818935927946));
#30515=CARTESIAN_POINT('Ctrl Pts',(-1.50529278229764,-1.18514270861281,
11.9732243738687));
#30516=CARTESIAN_POINT('Ctrl Pts',(-1.51477839333627,-1.06847604194574,
11.9585096316802));
#30517=CARTESIAN_POINT('Ctrl Pts',(-1.50813407284541,-0.794772684001029,
11.9105492654116));
#30518=CARTESIAN_POINT('Ctrl Pts',(-1.46364588916581,-0.636309800095337,
11.8532367545533));
#30519=CARTESIAN_POINT('Ctrl Pts',(-1.41117822787962,-0.319434907277229,
11.7977990691333));
#30520=CARTESIAN_POINT('Ctrl Pts',(-1.37050240246276,-0.158333333333367,
11.7647942347192));
#30521=CARTESIAN_POINT('Ctrl Pts',(-1.33921855852028,0.15833333333337,11.7741509880921));
#30522=CARTESIAN_POINT('Ctrl Pts',(-1.34760773600743,0.319434907277239,
11.8168336365887));
#30523=CARTESIAN_POINT('Ctrl Pts',(-1.33839509921198,0.636309800095348,
11.8906763773722));
#30524=CARTESIAN_POINT('Ctrl Pts',(-1.34861122908608,0.794772684001016,
11.9590558215034));
#30525=CARTESIAN_POINT('Ctrl Pts',(-1.31066005266653,1.06847604194542,12.0187173448594));
#30526=CARTESIAN_POINT('Ctrl Pts',(-1.28480044480139,1.18514270861219,12.0371059865518));
#30527=CARTESIAN_POINT('Ctrl Pts',(-1.24950888711346,1.30000000000051,12.0480580071529));
#30528=CARTESIAN_POINT('Ctrl Pts',(-1.50230543268038,-1.3000000000014,11.9989352575912));
#30529=CARTESIAN_POINT('Ctrl Pts',(-1.52838553185008,-1.1851427086128,11.9932437652798));
#30530=CARTESIAN_POINT('Ctrl Pts',(-1.54081146658877,-1.06847604194573,
11.9807964322698));
#30531=CARTESIAN_POINT('Ctrl Pts',(-1.537974010293,-0.794772684001022,11.9364332594215));
#30532=CARTESIAN_POINT('Ctrl Pts',(-1.49159955480665,-0.636309800095334,
11.8791998869732));
#30533=CARTESIAN_POINT('Ctrl Pts',(-1.43824443615658,-0.319434907277227,
11.8244360270167));
#30534=CARTESIAN_POINT('Ctrl Pts',(-1.39578979224414,-0.158333333333366,
11.7906539395304));
#30535=CARTESIAN_POINT('Ctrl Pts',(-1.36413285231675,0.158333333333369,
11.8002225466957));
#30536=CARTESIAN_POINT('Ctrl Pts',(-1.37377190540379,0.319434907277236,
11.8439539537967));
#30537=CARTESIAN_POINT('Ctrl Pts',(-1.36500420525066,0.636309800095344,
11.9174328937395));
#30538=CARTESIAN_POINT('Ctrl Pts',(-1.37741180114805,0.794772684001012,
11.9857353250915));
#30539=CARTESIAN_POINT('Ctrl Pts',(-1.33520760996577,1.06847604194542,12.0420131895444));
#30540=CARTESIAN_POINT('Ctrl Pts',(-1.30610077108674,1.18514270861218,12.0582428261529));
#30541=CARTESIAN_POINT('Ctrl Pts',(-1.26615572387209,1.3000000000005,12.0663414971487));
#30542=CARTESIAN_POINT('Ctrl Pts',(-1.51240241427839,-1.30000000000112,
12.007106984072));
#30543=CARTESIAN_POINT('Ctrl Pts',(-1.54036079622444,-1.18514270861254,
12.0030164794702));
#30544=CARTESIAN_POINT('Ctrl Pts',(-1.5541361931653,-1.0684760419455,11.9917560436576));
#30545=CARTESIAN_POINT('Ctrl Pts',(-1.55319458319894,-0.794772684000851,
11.9491782088514));
#30546=CARTESIAN_POINT('Ctrl Pts',(-1.50638430478292,-0.636309800095196,
11.8917068361181));
#30547=CARTESIAN_POINT('Ctrl Pts',(-1.45275981718469,-0.319434907277159,
11.8371994262208));
#30548=CARTESIAN_POINT('Ctrl Pts',(-1.40945018590222,-0.158333333333332,
11.8030474555539));
#30549=CARTESIAN_POINT('Ctrl Pts',(-1.37727481249132,0.158333333333334,
11.8129044039714));
#30550=CARTESIAN_POINT('Ctrl Pts',(-1.3870306215781,0.319434907277167,11.8574095495264));
#30551=CARTESIAN_POINT('Ctrl Pts',(-1.37792399116514,0.636309800095206,
11.9309840760347));
#30552=CARTESIAN_POINT('Ctrl Pts',(-1.39070615145891,0.79477268400084,11.9995754377232));
#30553=CARTESIAN_POINT('Ctrl Pts',(-1.34687223012689,1.06847604194519,12.0539531416098));
#30554=CARTESIAN_POINT('Ctrl Pts',(-1.31666175922729,1.18514270861193,12.0688762002392));
#30555=CARTESIAN_POINT('Ctrl Pts',(-1.27521489776587,1.30000000000022,12.075184224378));
#30556=CARTESIAN_POINT('Ctrl Pts',(-1.51741227377083,-1.30000000000112,
12.0112098547444));
#30557=CARTESIAN_POINT('Ctrl Pts',(-1.54630261814581,-1.18514270861254,
12.0079231435191));
#30558=CARTESIAN_POINT('Ctrl Pts',(-1.56074958986041,-1.0684760419455,11.99725764633));
#30559=CARTESIAN_POINT('Ctrl Pts',(-1.56075790439565,-0.794772684000851,
11.9555717425004));
#30560=CARTESIAN_POINT('Ctrl Pts',(-1.51378858280601,-0.636309800095196,
11.8979534138563));
#30561=CARTESIAN_POINT('Ctrl Pts',(-1.45995892423166,-0.319434907277159,
11.8436091949709));
#30562=CARTESIAN_POINT('Ctrl Pts',(-1.41600270611002,-0.158333333333332,
11.8093804181447));
#30563=CARTESIAN_POINT('Ctrl Pts',(-1.38362278588542,0.158333333333334,
11.8193529279827));
#30564=CARTESIAN_POINT('Ctrl Pts',(-1.39375448302884,0.319434907277167,
11.8640850863445));
#30565=CARTESIAN_POINT('Ctrl Pts',(-1.38457112325774,0.636309800095206,
11.9376612423013));
#30566=CARTESIAN_POINT('Ctrl Pts',(-1.39741805963304,0.79477268400084,12.0064627225285));
#30567=CARTESIAN_POINT('Ctrl Pts',(-1.3526706067805,1.06847604194519,12.0599359626955));
#30568=CARTESIAN_POINT('Ctrl Pts',(-1.32185850051433,1.18514270861193,12.0742273399833));
#30569=CARTESIAN_POINT('Ctrl Pts',(-1.27960380226532,1.30000000000022,12.0796635102695));
#30570=CARTESIAN_POINT('',(-1.2373438536101,1.2,11.9928572050431));
#30571=CARTESIAN_POINT('Ctrl Pts',(-1.2373438536101,1.2,11.9928572050431));
#30572=CARTESIAN_POINT('Ctrl Pts',(-1.22007242234924,1.21680886307926,11.9799560961046));
#30573=CARTESIAN_POINT('Ctrl Pts',(-1.20198017112036,1.23320396068793,11.9676320090486));
#30574=CARTESIAN_POINT('Ctrl Pts',(-1.17510185254842,1.25911304880667,11.9476275708389));
#30575=CARTESIAN_POINT('Ctrl Pts',(-1.15950113852676,1.27356500001449,11.9366232467277));
#30576=CARTESIAN_POINT('Ctrl Pts',(-1.13329432476672,1.3,11.9157336622684));
#30577=CARTESIAN_POINT('',(-1.38832547963881,0.653834841382538,11.9513211175694));
#30578=CARTESIAN_POINT('Ctrl Pts',(-1.38832547962899,0.653834841377511,
11.9513211176064));
#30579=CARTESIAN_POINT('Ctrl Pts',(-1.37327925638861,0.715637047620691,
11.9557175906252));
#30580=CARTESIAN_POINT('Ctrl Pts',(-1.35934876819983,0.767437339736555,
11.9597189842502));
#30581=CARTESIAN_POINT('Ctrl Pts',(-1.32827629350109,0.882054338936367,
11.9684850281746));
#30582=CARTESIAN_POINT('Ctrl Pts',(-1.31342061390376,0.939294188357158,
11.9726076783957));
#30583=CARTESIAN_POINT('Ctrl Pts',(-1.28552565669992,1.03700621393207,11.9801698223984));
#30584=CARTESIAN_POINT('Ctrl Pts',(-1.28427849821935,1.04065632268877,11.9805295350603));
#30585=CARTESIAN_POINT('Ctrl Pts',(-1.2563560598427,1.13599421849374,11.9879204304765));
#30586=CARTESIAN_POINT('Ctrl Pts',(-1.24755393031006,1.16618572853348,11.9902213293829));
#30587=CARTESIAN_POINT('Ctrl Pts',(-1.2373438536101,1.2,11.9928572050431));
#30588=CARTESIAN_POINT('',(-1.52166805320966,-0.653834841531101,11.9103106411192));
#30589=CARTESIAN_POINT('Ctrl Pts',(-1.52166805320967,-0.653834841531079,
11.9103106411192));
#30590=CARTESIAN_POINT('Ctrl Pts',(-1.49332370940493,-0.575726829001172,
11.8797128649133));
#30591=CARTESIAN_POINT('Ctrl Pts',(-1.46878742733875,-0.493694691894675,
11.8546066668147));
#30592=CARTESIAN_POINT('Ctrl Pts',(-1.43181654628555,-0.338084133530092,
11.8199726365178));
#30593=CARTESIAN_POINT('Ctrl Pts',(-1.4178771777781,-0.26562576409014,11.8086841555559));
#30594=CARTESIAN_POINT('Ctrl Pts',(-1.3965041256658,-0.129694174089561,
11.7968486800664));
#30595=CARTESIAN_POINT('Ctrl Pts',(-1.38847548152787,-0.0666412200678742,
11.794956151289));
#30596=CARTESIAN_POINT('Ctrl Pts',(-1.37567108574927,0.0594771285402088,
11.7985011872496));
#30597=CARTESIAN_POINT('Ctrl Pts',(-1.37080511110895,0.122680285497012,
11.8039458214053));
#30598=CARTESIAN_POINT('Ctrl Pts',(-1.36460604093124,0.260050375630151,
11.8236401506711));
#30599=CARTESIAN_POINT('Ctrl Pts',(-1.36403934238603,0.333912938648628,
11.8393326465065));
#30600=CARTESIAN_POINT('Ctrl Pts',(-1.36976405159761,0.491493501735914,
11.8838745599282));
#30601=CARTESIAN_POINT('Ctrl Pts',(-1.37696041957445,0.574885173904325,
11.914805991444));
#30602=CARTESIAN_POINT('Ctrl Pts',(-1.38832547957248,0.653834841398299,
11.9513211175559));
#30603=CARTESIAN_POINT('',(-1.45267111627981,-1.2,11.9320446561636));
#30604=CARTESIAN_POINT('Ctrl Pts',(-1.45267111627981,-1.2,11.9320446561636));
#30605=CARTESIAN_POINT('Ctrl Pts',(-1.46243409420727,-1.14592853623335,
11.9290475593324));
#30606=CARTESIAN_POINT('Ctrl Pts',(-1.47710331673422,-1.06261597021533,
11.9245259227913));
#30607=CARTESIAN_POINT('Ctrl Pts',(-1.50949341520291,-0.803846334503223,
11.9142418008359));
#30608=CARTESIAN_POINT('Ctrl Pts',(-1.51508125140246,-0.746395744507367,
11.9124385105203));
#30609=CARTESIAN_POINT('Ctrl Pts',(-1.52166805320967,-0.653834841531101,
11.9103106411192));
#30610=CARTESIAN_POINT('Ctrl Pts',(-1.35212230766396,-1.30000000000011,
11.857710302833));
#30611=CARTESIAN_POINT('Ctrl Pts',(-1.36853533305804,-1.28287864461177,
11.8707738366094));
#30612=CARTESIAN_POINT('Ctrl Pts',(-1.38567851507679,-1.26604242834882,
11.88327852373));
#30613=CARTESIAN_POINT('Ctrl Pts',(-1.42483729732607,-1.22709161555245,
11.9122329332583));
#30614=CARTESIAN_POINT('Ctrl Pts',(-1.43804978907626,-1.21370565301587,
11.9221962700843));
#30615=CARTESIAN_POINT('Ctrl Pts',(-1.45267111627981,-1.2,11.9320446561636));
#30616=CARTESIAN_POINT('Origin',(0.,1.25,7.2));
#30617=CARTESIAN_POINT('',(-0.213828345914065,1.2,12.1453794028855));
#30618=CARTESIAN_POINT('Origin',(0.,1.2,7.2));
#30619=CARTESIAN_POINT('Ctrl Pts',(-0.213828345914065,1.2,12.1453794028855));
#30620=CARTESIAN_POINT('Ctrl Pts',(-0.195742251015914,1.22112918552691,
12.1250124824944));
#30621=CARTESIAN_POINT('Ctrl Pts',(-0.177075057844756,1.24197036598625,
12.1048648021315));
#30622=CARTESIAN_POINT('Ctrl Pts',(-0.148630873366042,1.27532127191025,
12.0724226989563));
#30623=CARTESIAN_POINT('Ctrl Pts',(-0.138144362293013,1.28756858937727,
12.0604782373989));
#30624=CARTESIAN_POINT('Ctrl Pts',(-0.128158081937606,1.2999999999995,12.0483064575209));
#30625=CARTESIAN_POINT('Origin',(0.,0.92691742076555,7.2));
#30626=CARTESIAN_POINT('',(-0.370132012290736,0.653834841366703,12.1361424506498));
#30627=CARTESIAN_POINT('Origin',(0.,0.653834841531101,7.2));
#30628=CARTESIAN_POINT('Ctrl Pts',(-0.370132012288497,0.653834841365421,
12.1361424506875));
#30629=CARTESIAN_POINT('Ctrl Pts',(-0.354138141111788,0.717049709819526,
12.1373417361178));
#30630=CARTESIAN_POINT('Ctrl Pts',(-0.332832873908772,0.792929369312527,
12.1388326360144));
#30631=CARTESIAN_POINT('Ctrl Pts',(-0.30692609112432,0.885929226741259,
12.1404808169553));
#30632=CARTESIAN_POINT('Ctrl Pts',(-0.300394671658448,0.909292265434727,
12.1408823708037));
#30633=CARTESIAN_POINT('Ctrl Pts',(-0.267850169499559,1.02405695792837,
12.1428118183178));
#30634=CARTESIAN_POINT('Ctrl Pts',(-0.241222096346408,1.1121531011995,12.1441949517309));
#30635=CARTESIAN_POINT('Ctrl Pts',(-0.213828345914064,1.2,12.1453794028854));
#30636=CARTESIAN_POINT('Origin',(0.,0.,7.2));
#30637=CARTESIAN_POINT('',(-0.509087305688324,-0.653834841531101,12.1237516301279));
#30638=CARTESIAN_POINT('Origin',(0.,-0.653834841531101,7.2));
#30639=CARTESIAN_POINT('Ctrl Pts',(-0.509087305688305,-0.65383484153111,
12.1237516301279));
#30640=CARTESIAN_POINT('Ctrl Pts',(-0.487796603721125,-0.575992320405206,
12.0880511292075));
#30641=CARTESIAN_POINT('Ctrl Pts',(-0.469123782926452,-0.493632669726353,
12.05824203318));
#30642=CARTESIAN_POINT('Ctrl Pts',(-0.440222124607192,-0.338115839260951,
12.0166878970055));
#30643=CARTESIAN_POINT('Ctrl Pts',(-0.42902720878148,-0.265637866641146,
12.0027380166553));
#30644=CARTESIAN_POINT('Ctrl Pts',(-0.410675091361661,-0.129696817563903,
11.9867099771911));
#30645=CARTESIAN_POINT('Ctrl Pts',(-0.403190326971112,-0.0666113386779936,
11.9831897465878));
#30646=CARTESIAN_POINT('Ctrl Pts',(-0.389888857045734,0.0595467574157433,
11.9840034138292));
#30647=CARTESIAN_POINT('Ctrl Pts',(-0.38397462719954,0.122772045581972,
11.9883261664178));
#30648=CARTESIAN_POINT('Ctrl Pts',(-0.373658687761304,0.260120772719706,
12.0063186578358));
#30649=CARTESIAN_POINT('Ctrl Pts',(-0.369728507767857,0.33394176338759,
12.0215544969233));
#30650=CARTESIAN_POINT('Ctrl Pts',(-0.365884250931941,0.49120341452778,
12.0662377985978));
#30651=CARTESIAN_POINT('Ctrl Pts',(-0.366579556882535,0.574345839355596,
12.0978024686969));
#30652=CARTESIAN_POINT('Ctrl Pts',(-0.370132012239985,0.653834841383583,
12.1361424506195));
#30653=CARTESIAN_POINT('Origin',(0.,-0.926917420765551,7.2));
#30654=CARTESIAN_POINT('',(-0.437059572605786,-1.2,12.1306671891331));
#30655=CARTESIAN_POINT('Origin',(0.,-1.2,7.2));
#30656=CARTESIAN_POINT('Ctrl Pts',(-0.43705957260579,-1.2,12.1306671891331));
#30657=CARTESIAN_POINT('Ctrl Pts',(-0.449850978802582,-1.13143558342973,
12.1295333453122));
#30658=CARTESIAN_POINT('Ctrl Pts',(-0.463535154438354,-1.05442944320354,
12.1282924278181));
#30659=CARTESIAN_POINT('Ctrl Pts',(-0.497848612890372,-0.79255450235333,
12.1249197851749));
#30660=CARTESIAN_POINT('Ctrl Pts',(-0.50276625626291,-0.738810704696317,
12.1244051899056));
#30661=CARTESIAN_POINT('Ctrl Pts',(-0.509087305688302,-0.6538348415311,
12.1237516301279));
#30662=CARTESIAN_POINT('Origin',(0.,-1.25,7.2));
#30663=CARTESIAN_POINT('Ctrl Pts',(-0.354232945953443,-1.3,12.0370465182796));
#30664=CARTESIAN_POINT('Ctrl Pts',(-0.369830978971964,-1.27998847667344,
12.0559693362845));
#30665=CARTESIAN_POINT('Ctrl Pts',(-0.383310654693955,-1.26450440150284,
12.0704526234879));
#30666=CARTESIAN_POINT('Ctrl Pts',(-0.410365222815302,-1.23095282611831,
12.1019135168529));
#30667=CARTESIAN_POINT('Ctrl Pts',(-0.423468395372474,-1.21538387848804,
12.1164277278777));
#30668=CARTESIAN_POINT('Ctrl Pts',(-0.43705957260579,-1.2,12.1306671891331));
#30669=CARTESIAN_POINT('Ctrl Pts',(-1.83297302538937,-1.30000000000171,
11.8998629503917));
#30670=CARTESIAN_POINT('Ctrl Pts',(-1.7955929556911,-1.18514270861294,11.9203016847184));
#30671=CARTESIAN_POINT('Ctrl Pts',(-1.76226517728477,-1.0684760419457,11.9268506192756));
#30672=CARTESIAN_POINT('Ctrl Pts',(-1.69463294550958,-0.794772684000851,
11.9098917521005));
#30673=CARTESIAN_POINT('Ctrl Pts',(-1.66458583994784,-0.636309800095197,
11.8466789456163));
#30674=CARTESIAN_POINT('Ctrl Pts',(-1.61390936643532,-0.319434907277159,
11.7925524285052));
#30675=CARTESIAN_POINT('Ctrl Pts',(-1.59581317861837,-0.158333333333332,
11.750408090035));
#30676=CARTESIAN_POINT('Ctrl Pts',(-1.56375557866912,0.158333333333334,
11.761372599678));
#30677=CARTESIAN_POINT('Ctrl Pts',(-1.54831342142296,0.319434907277167,
11.814901078586));
#30678=CARTESIAN_POINT('Ctrl Pts',(-1.53670704324243,0.636309800095206,
11.8905067546545));
#30679=CARTESIAN_POINT('Ctrl Pts',(-1.53257526769918,0.79477268400084,11.9647288362512));
#30680=CARTESIAN_POINT('Ctrl Pts',(-1.55708435379914,1.0684760419458,11.9984485537147));
#30681=CARTESIAN_POINT('Ctrl Pts',(-1.57504122139016,1.18514270861313,11.9985854052814));
#30682=CARTESIAN_POINT('Ctrl Pts',(-1.60034588135063,1.300000000002,11.9842630921634));
#30683=CARTESIAN_POINT('Ctrl Pts',(-1.83389086553798,-1.30000000000171,
11.8936593986674));
#30684=CARTESIAN_POINT('Ctrl Pts',(-1.79665188669752,-1.18514270861294,
11.912917953872));
#30685=CARTESIAN_POINT('Ctrl Pts',(-1.76343954855294,-1.0684760419457,11.9186022150992));
#30686=CARTESIAN_POINT('Ctrl Pts',(-1.69601474886784,-0.794772684000853,
11.9003746610507));
#30687=CARTESIAN_POINT('Ctrl Pts',(-1.66603874292474,-0.636309800095198,
11.8373699184396));
#30688=CARTESIAN_POINT('Ctrl Pts',(-1.6154253025298,-0.319434907277159,
11.7831996191878));
#30689=CARTESIAN_POINT('Ctrl Pts',(-1.59715844966913,-0.158333333333333,
11.7414598793969));
#30690=CARTESIAN_POINT('Ctrl Pts',(-1.56533425686699,0.158333333333334,
11.7523976505925));
#30691=CARTESIAN_POINT('Ctrl Pts',(-1.55037005383525,0.319434907277167,
11.8054839378072));
#30692=CARTESIAN_POINT('Ctrl Pts',(-1.53902558372754,0.636309800095206,
11.8811010416947));
#30693=CARTESIAN_POINT('Ctrl Pts',(-1.53493609828886,0.794772684000841,
11.9551107502081));
#30694=CARTESIAN_POINT('Ctrl Pts',(-1.55920094319785,1.0684760419458,11.9901104066026));
#30695=CARTESIAN_POINT('Ctrl Pts',(-1.57696419153494,1.18514270861314,11.9911233153795));
#30696=CARTESIAN_POINT('Ctrl Pts',(-1.60198733594911,1.30000000000201,11.9779990785452));
#30697=CARTESIAN_POINT('Ctrl Pts',(-1.83599972161534,-1.30000000000147,
11.8811871414573));
#30698=CARTESIAN_POINT('Ctrl Pts',(-1.79892582936594,-1.18514270861273,
11.8981141035431));
#30699=CARTESIAN_POINT('Ctrl Pts',(-1.76583960086258,-1.06847604194551,
11.9020927398455));
#30700=CARTESIAN_POINT('Ctrl Pts',(-1.69861609512545,-0.794772684000711,
11.8813709627645));
#30701=CARTESIAN_POINT('Ctrl Pts',(-1.66849527243313,-0.636309800095083,
11.8188239975564));
#30702=CARTESIAN_POINT('Ctrl Pts',(-1.61822051779594,-0.319434907277102,
11.7645294437215));
#30703=CARTESIAN_POINT('Ctrl Pts',(-1.60033540285054,-0.158333333333304,
11.7234771864337));
#30704=CARTESIAN_POINT('Ctrl Pts',(-1.56911125276349,0.158333333333306,
11.7343403832408));
#30705=CARTESIAN_POINT('Ctrl Pts',(-1.55462119255688,0.31943490727711,11.7866261268805));
#30706=CARTESIAN_POINT('Ctrl Pts',(-1.54363915686094,0.636309800095092,
11.862293977294));
#30707=CARTESIAN_POINT('Ctrl Pts',(-1.53974920062094,0.794772684000699,
11.9358578924444));
#30708=CARTESIAN_POINT('Ctrl Pts',(-1.56351982816593,1.06847604194561,11.9734175763765));
#30709=CARTESIAN_POINT('Ctrl Pts',(-1.58088572421911,1.18514270861292,11.9761840272521));
#30710=CARTESIAN_POINT('Ctrl Pts',(-1.60532809244977,1.30000000000177,11.9654587335524));
#30711=CARTESIAN_POINT('Ctrl Pts',(-1.83871875022158,-1.30000000000147,
11.8566111165687));
#30712=CARTESIAN_POINT('Ctrl Pts',(-1.80373143478885,-1.18514270861272,
11.8684945970647));
#30713=CARTESIAN_POINT('Ctrl Pts',(-1.77200267054075,-1.06847604194551,
11.8688179909996));
#30714=CARTESIAN_POINT('Ctrl Pts',(-1.70623078291767,-0.794772684000706,
11.8428589831409));
#30715=CARTESIAN_POINT('Ctrl Pts',(-1.67429344241067,-0.636309800095081,
11.7815375882988));
#30716=CARTESIAN_POINT('Ctrl Pts',(-1.62344550695782,-0.3194349072771,11.7272100904621));
#30717=CARTESIAN_POINT('Ctrl Pts',(-1.60516508839733,-0.158333333333303,
11.6877409305584));
#30718=CARTESIAN_POINT('Ctrl Pts',(-1.5743680048027,0.158333333333305,11.6985560603514));
#30719=CARTESIAN_POINT('Ctrl Pts',(-1.56086158634495,0.319434907277107,
11.7491672409098));
#30720=CARTESIAN_POINT('Ctrl Pts',(-1.55099413643843,0.636309800095088,
11.8248585262712));
#30721=CARTESIAN_POINT('Ctrl Pts',(-1.54867609147355,0.794772684000694,
11.897377874003));
#30722=CARTESIAN_POINT('Ctrl Pts',(-1.57148108477577,1.0684760419456,11.9400854010788));
#30723=CARTESIAN_POINT('Ctrl Pts',(-1.58780090005551,1.18514270861292,11.9464145067419));
#30724=CARTESIAN_POINT('Ctrl Pts',(-1.61056909402271,1.30000000000177,11.9405862120668));
#30725=CARTESIAN_POINT('Ctrl Pts',(-1.84133699429135,-1.30000000000095,
11.8377753162936));
#30726=CARTESIAN_POINT('Ctrl Pts',(-1.80586113471466,-1.18514270861225,
11.8462507052803));
#30727=CARTESIAN_POINT('Ctrl Pts',(-1.77392632328359,-1.06847604194508,
11.8440552614294));
#30728=CARTESIAN_POINT('Ctrl Pts',(-1.70833104994145,-0.794772684000392,
11.8143315883892));
#30729=CARTESIAN_POINT('Ctrl Pts',(-1.67771417480332,-0.636309800094828,
11.7534325233558));
#30730=CARTESIAN_POINT('Ctrl Pts',(-1.62752369412159,-0.319434907276974,
11.6988831504611));
#30731=CARTESIAN_POINT('Ctrl Pts',(-1.60889275025167,-0.158333333333241,
11.6606177782961));
#30732=CARTESIAN_POINT('Ctrl Pts',(-1.57869038857939,0.158333333333243,
11.6713553018697));
#30733=CARTESIAN_POINT('Ctrl Pts',(-1.56592675366209,0.319434907276982,
11.7207153472662));
#30734=CARTESIAN_POINT('Ctrl Pts',(-1.55702565868022,0.636309800094838,
11.7964087944155));
#30735=CARTESIAN_POINT('Ctrl Pts',(-1.55596803316826,0.79477268400038,11.8681143540736));
#30736=CARTESIAN_POINT('Ctrl Pts',(-1.57811230023751,1.06847604194518,11.9147102504626));
#30737=CARTESIAN_POINT('Ctrl Pts',(-1.5936603129417,1.18514270861245,11.9237367188749));
#30738=CARTESIAN_POINT('Ctrl Pts',(-1.61517090566172,1.30000000000125,11.9216200187009));
#30739=CARTESIAN_POINT('Ctrl Pts',(-1.84289452093225,-1.30000000000092,
11.8250381337617));
#30740=CARTESIAN_POINT('Ctrl Pts',(-1.80820933111375,-1.18514270861222,
11.8309617575969));
#30741=CARTESIAN_POINT('Ctrl Pts',(-1.77678593741475,-1.06847604194505,
11.8269137155766));
#30742=CARTESIAN_POINT('Ctrl Pts',(-1.71172701329799,-0.794772684000369,
11.7945253857508));
#30743=CARTESIAN_POINT('Ctrl Pts',(-1.68045048611224,-0.636309800094811,
11.7342095024028));
#30744=CARTESIAN_POINT('Ctrl Pts',(-1.62992587645071,-0.319434907276965,
11.6796502838771));
#30745=CARTESIAN_POINT('Ctrl Pts',(-1.61081717316368,-0.158333333333236,
11.642250753783));
#30746=CARTESIAN_POINT('Ctrl Pts',(-1.58094261327684,0.158333333333238,
11.6529448537923));
#30747=CARTESIAN_POINT('Ctrl Pts',(-1.56923788348696,0.319434907276973,
11.7013502469139));
#30748=CARTESIAN_POINT('Ctrl Pts',(-1.56082258278577,0.63630980009482,11.7770575383374));
#30749=CARTESIAN_POINT('Ctrl Pts',(-1.55970762511443,0.794772684000359,
11.8483368173369));
#30750=CARTESIAN_POINT('Ctrl Pts',(-1.58141110711112,1.06847604194515,11.8975860362724));
#30751=CARTESIAN_POINT('Ctrl Pts',(-1.59663434811504,1.18514270861241,11.9084268380449));
#30752=CARTESIAN_POINT('Ctrl Pts',(-1.61768619695974,1.30000000000122,11.908790279576));
#30753=CARTESIAN_POINT('Ctrl Pts',(-1.84296348521904,-1.30000000000092,
11.8244594935074));
#30754=CARTESIAN_POINT('Ctrl Pts',(-1.80831270159826,-1.18514270861222,
11.8302673795263));
#30755=CARTESIAN_POINT('Ctrl Pts',(-1.77691170768193,-1.06847604194505,
11.8261352609154));
#30756=CARTESIAN_POINT('Ctrl Pts',(-1.71187679432357,-0.794772684000369,
11.7936258411106));
#30757=CARTESIAN_POINT('Ctrl Pts',(-1.68057311228323,-0.636309800094812,
11.7333359468922));
#30758=CARTESIAN_POINT('Ctrl Pts',(-1.63003388390691,-0.319434907276965,
11.6787761644253));
#30759=CARTESIAN_POINT('Ctrl Pts',(-1.61090199228311,-0.158333333333236,
11.6414162554122));
#30760=CARTESIAN_POINT('Ctrl Pts',(-1.58104259750264,0.158333333333238,
11.6521083364588));
#30761=CARTESIAN_POINT('Ctrl Pts',(-1.56938714187537,0.319434907276973,
11.7004701333277));
#30762=CARTESIAN_POINT('Ctrl Pts',(-1.56099510539947,0.636309800094821,
11.7761778608677));
#30763=CARTESIAN_POINT('Ctrl Pts',(-1.55987837436003,0.794772684000359,
11.8474376330947));
#30764=CARTESIAN_POINT('Ctrl Pts',(-1.58156226067329,1.06847604194515,11.8968074087413));
#30765=CARTESIAN_POINT('Ctrl Pts',(-1.59677074811116,1.18514270861241,11.9077306927128));
#30766=CARTESIAN_POINT('Ctrl Pts',(-1.61780157206904,1.30000000000122,11.9082069141089));
#30767=CARTESIAN_POINT('Ctrl Pts',(-1.84303196081658,-1.30000000000092,
11.8238809650216));
#30768=CARTESIAN_POINT('Ctrl Pts',(-1.80841559259507,-1.18514270861222,
11.8295731157283));
#30769=CARTESIAN_POINT('Ctrl Pts',(-1.77703699467618,-1.06847604194505,
11.8253569231424));
#30770=CARTESIAN_POINT('Ctrl Pts',(-1.71202605332952,-0.794772684000369,
11.7927264196592));
#30771=CARTESIAN_POINT('Ctrl Pts',(-1.68069495255617,-0.636309800094811,
11.7324625538845));
#30772=CARTESIAN_POINT('Ctrl Pts',(-1.63014140611213,-0.319434907276965,
11.677902145418));
#30773=CARTESIAN_POINT('Ctrl Pts',(-1.61098724178691,-0.158333333333236,
11.6405816925744));
#30774=CARTESIAN_POINT('Ctrl Pts',(-1.5811428723139,0.158333333333238,11.6512717653135));
#30775=CARTESIAN_POINT('Ctrl Pts',(-1.56953536178466,0.319434907276973,
11.6995901789837));
#30776=CARTESIAN_POINT('Ctrl Pts',(-1.56116656149189,0.63630980009482,11.7752983500434));
#30777=CARTESIAN_POINT('Ctrl Pts',(-1.56004940665739,0.794772684000359,
11.8465384115319));
#30778=CARTESIAN_POINT('Ctrl Pts',(-1.58171386737888,1.06847604194515,11.8960287165786));
#30779=CARTESIAN_POINT('Ctrl Pts',(-1.59690745305271,1.18514270861241,11.9070345037863));
#30780=CARTESIAN_POINT('Ctrl Pts',(-1.61791688210141,1.30000000000122,11.9076235589435));
#30781=CARTESIAN_POINT('Ctrl Pts',(-1.84316669728488,-1.30000000000092,
11.8227243210795));
#30782=CARTESIAN_POINT('Ctrl Pts',(-1.80861747574687,-1.18514270861222,
11.8281852976434));
#30783=CARTESIAN_POINT('Ctrl Pts',(-1.77728271948137,-1.06847604194505,
11.8238011194843));
#30784=CARTESIAN_POINT('Ctrl Pts',(-1.71231922184277,-0.794772684000369,
11.7909285139586));
#30785=CARTESIAN_POINT('Ctrl Pts',(-1.68093588515833,-0.636309800094812,
11.7307162099497));
#30786=CARTESIAN_POINT('Ctrl Pts',(-1.63035490044341,-0.319434907276966,
11.6761543109724));
#30787=CARTESIAN_POINT('Ctrl Pts',(-1.61115632950736,-0.158333333333236,
11.6389127476635));
#30788=CARTESIAN_POINT('Ctrl Pts',(-1.58134204256666,0.158333333333238,
11.6495987813934));
#30789=CARTESIAN_POINT('Ctrl Pts',(-1.56982924289939,0.319434907276973,
11.697830603521));
#30790=CARTESIAN_POINT('Ctrl Pts',(-1.56150796664459,0.636309800094821,
11.7735394991853));
#30791=CARTESIAN_POINT('Ctrl Pts',(-1.56039305183889,0.794772684000359,
11.8447396712156));
#30792=CARTESIAN_POINT('Ctrl Pts',(-1.58201926842724,1.06847604194515,11.8944709559761));
#30793=CARTESIAN_POINT('Ctrl Pts',(-1.59718274353702,1.18514270861241,11.9056418049324));
#30794=CARTESIAN_POINT('Ctrl Pts',(-1.61814850592577,1.30000000000122,11.9064566723979));
#30795=CARTESIAN_POINT('Ctrl Pts',(-1.84344888288028,-1.30000000000092,
11.8202201103828));
#30796=CARTESIAN_POINT('Ctrl Pts',(-1.80903791412077,-1.18514270861222,
11.8251815293551));
#30797=CARTESIAN_POINT('Ctrl Pts',(-1.77779396859234,-1.06847604194506,
11.8204341284388));
#30798=CARTESIAN_POINT('Ctrl Pts',(-1.71293066131657,-0.79477268400037,
11.7870373664222));
#30799=CARTESIAN_POINT('Ctrl Pts',(-1.68144353848663,-0.636309800094812,
11.7269349411184));
#30800=CARTESIAN_POINT('Ctrl Pts',(-1.63080972946727,-0.319434907276966,
11.6723685067135));
#30801=CARTESIAN_POINT('Ctrl Pts',(-1.61152048533865,-0.158333333333237,
11.6352968905261));
#30802=CARTESIAN_POINT('Ctrl Pts',(-1.58177113039119,0.158333333333239,
11.6459740954571));
#30803=CARTESIAN_POINT('Ctrl Pts',(-1.57045247065589,0.319434907276973,
11.6940200284722));
#30804=CARTESIAN_POINT('Ctrl Pts',(-1.56223778799716,0.636309800094821,
11.7697299649961));
#30805=CARTESIAN_POINT('Ctrl Pts',(-1.56114547527118,0.79477268400036,11.8408410521061));
#30806=CARTESIAN_POINT('Ctrl Pts',(-1.58269200483603,1.06847604194515,11.8910940125196));
#30807=CARTESIAN_POINT('Ctrl Pts',(-1.59778850945841,1.18514270861242,11.9026227716686));
#30808=CARTESIAN_POINT('Ctrl Pts',(-1.61865482443213,1.30000000000122,11.9039276454594));
#30809=CARTESIAN_POINT('Ctrl Pts',(-1.84384438076087,-1.30000000000093,
11.8163742850652));
#30810=CARTESIAN_POINT('Ctrl Pts',(-1.80959881413743,-1.18514270861223,
11.8205762115273));
#30811=CARTESIAN_POINT('Ctrl Pts',(-1.77846705385221,-1.06847604194506,
11.8152752438931));
#30812=CARTESIAN_POINT('Ctrl Pts',(-1.71373997526232,-0.794772684000375,
11.781075361793));
#30813=CARTESIAN_POINT('Ctrl Pts',(-1.68215207565877,-0.636309800094816,
11.7211303361575));
#30814=CARTESIAN_POINT('Ctrl Pts',(-1.63148140929813,-0.319434907276968,
11.6665484490828));
#30815=CARTESIAN_POINT('Ctrl Pts',(-1.61209419825319,-0.158333333333238,
11.6297311120483));
#30816=CARTESIAN_POINT('Ctrl Pts',(-1.58244234073241,0.15833333333324,11.6403946024421));
#30817=CARTESIAN_POINT('Ctrl Pts',(-1.57134630363325,0.319434907276975,
11.6881666550633));
#30818=CARTESIAN_POINT('Ctrl Pts',(-1.56331175406625,0.636309800094825,
11.763876099524));
#30819=CARTESIAN_POINT('Ctrl Pts',(-1.56236283053004,0.794772684000365,
11.8348339670287));
#30820=CARTESIAN_POINT('Ctrl Pts',(-1.58380073924108,1.06847604194516,11.8858875342653));
#30821=CARTESIAN_POINT('Ctrl Pts',(-1.59878065247063,1.18514270861242,11.8979689831355));
#30822=CARTESIAN_POINT('Ctrl Pts',(-1.61946080260151,1.30000000000122,11.9000326833401));
#30823=CARTESIAN_POINT('Ctrl Pts',(-1.84426494116142,-1.30000000000093,
11.8117677988858));
#30824=CARTESIAN_POINT('Ctrl Pts',(-1.8101257178847,-1.18514270861223,11.8150761584175));
#30825=CARTESIAN_POINT('Ctrl Pts',(-1.77907371003347,-1.06847604194507,
11.8091214978874));
#30826=CARTESIAN_POINT('Ctrl Pts',(-1.71446944519264,-0.794772684000379,
11.7739656114336));
#30827=CARTESIAN_POINT('Ctrl Pts',(-1.68286150667179,-0.63630980009482,
11.7141893826815));
#30828=CARTESIAN_POINT('Ctrl Pts',(-1.63223484958063,-0.31943490727697,
11.6595724368514));
#30829=CARTESIAN_POINT('Ctrl Pts',(-1.61282826183454,-0.158333333333238,
11.6230434385891));
#30830=CARTESIAN_POINT('Ctrl Pts',(-1.5832926406303,0.15833333333324,11.6336895451472));
#30831=CARTESIAN_POINT('Ctrl Pts',(-1.57231028315703,0.319434907276977,
11.6811571847545));
#30832=CARTESIAN_POINT('Ctrl Pts',(-1.56451316606789,0.636309800094828,
11.7568636108008));
#30833=CARTESIAN_POINT('Ctrl Pts',(-1.56392988574138,0.79477268400037,11.8276093111329));
#30834=CARTESIAN_POINT('Ctrl Pts',(-1.58526559199745,1.06847604194516,11.8796195501203));
#30835=CARTESIAN_POINT('Ctrl Pts',(-1.60008428456176,1.18514270861243,11.892367313324));
#30836=CARTESIAN_POINT('Ctrl Pts',(-1.62048623301792,1.30000000000123,11.8953495344429));
#30837=CARTESIAN_POINT('Ctrl Pts',(-1.84478245665894,-1.30000000000094,
11.8056321709388));
#30838=CARTESIAN_POINT('Ctrl Pts',(-1.81070410073275,-1.18514270861224,
11.8077647834726));
#30839=CARTESIAN_POINT('Ctrl Pts',(-1.77970915118711,-1.06847604194508,
11.8009480735919));
#30840=CARTESIAN_POINT('Ctrl Pts',(-1.71522790279083,-0.794772684000385,
11.7645253850059));
#30841=CARTESIAN_POINT('Ctrl Pts',(-1.68367560268276,-0.636309800094825,
11.7049579257604));
#30842=CARTESIAN_POINT('Ctrl Pts',(-1.63317521611877,-0.319434907276972,
11.6502817193305));
#30843=CARTESIAN_POINT('Ctrl Pts',(-1.61381918122407,-0.15833333333324,
11.6141244214084));
#30844=CARTESIAN_POINT('Ctrl Pts',(-1.58443628392345,0.158333333333242,
11.6247465764964));
#30845=CARTESIAN_POINT('Ctrl Pts',(-1.57348065202961,0.31943490727698,11.6718272551794));
#30846=CARTESIAN_POINT('Ctrl Pts',(-1.56602202900427,0.636309800094834,
11.7475264516963));
#30847=CARTESIAN_POINT('Ctrl Pts',(-1.5660937604962,0.794772684000376,11.8179645101958));
#30848=CARTESIAN_POINT('Ctrl Pts',(-1.58731685620065,1.06847604194517,11.8712470930887));
#30849=CARTESIAN_POINT('Ctrl Pts',(-1.60190135100444,1.18514270861244,11.8848862965936));
#30850=CARTESIAN_POINT('Ctrl Pts',(-1.62188364887474,1.30000000000124,11.8891006477833));
#30851=CARTESIAN_POINT('Ctrl Pts',(-1.84544014297006,-1.30000000000095,
11.7979582048086));
#30852=CARTESIAN_POINT('Ctrl Pts',(-1.81144108841217,-1.18514270861225,
11.7986194547981));
#30853=CARTESIAN_POINT('Ctrl Pts',(-1.78051023879179,-1.06847604194508,
11.7907258958039));
#30854=CARTESIAN_POINT('Ctrl Pts',(-1.71614195567161,-0.794772684000391,
11.7527268752903));
#30855=CARTESIAN_POINT('Ctrl Pts',(-1.68458079263209,-0.636309800094829,
11.6934365417342));
#30856=CARTESIAN_POINT('Ctrl Pts',(-1.63419573725037,-0.319434907276974,
11.6386946770248));
#30857=CARTESIAN_POINT('Ctrl Pts',(-1.6149017766345,-0.158333333333241,
11.6030025586446));
#30858=CARTESIAN_POINT('Ctrl Pts',(-1.58573694252356,0.158333333333243,
11.6135885063308));
#30859=CARTESIAN_POINT('Ctrl Pts',(-1.57489385088498,0.319434907276982,
11.6601689843851));
#30860=CARTESIAN_POINT('Ctrl Pts',(-1.56785257747679,0.636309800094838,
11.7358576708726));
#30861=CARTESIAN_POINT('Ctrl Pts',(-1.56861088718507,0.79477268400038,11.8059322870055));
#30862=CARTESIAN_POINT('Ctrl Pts',(-1.58972943387026,1.06847604194518,11.8607999137329));
#30863=CARTESIAN_POINT('Ctrl Pts',(-1.60407107161093,1.18514270861245,11.8755459464035));
#30864=CARTESIAN_POINT('Ctrl Pts',(-1.62361291075149,1.30000000000125,11.8812878491803));
#30865=CARTESIAN_POINT('Ctrl Pts',(-1.84674828898009,-1.30000000000098,
11.7856311373012));
#30866=CARTESIAN_POINT('Ctrl Pts',(-1.81326855991173,-1.18514270861227,
11.7838592214465));
#30867=CARTESIAN_POINT('Ctrl Pts',(-1.78265895673732,-1.0684760419451,11.774198415806));
#30868=CARTESIAN_POINT('Ctrl Pts',(-1.71857521495619,-0.794772684000405,
11.7336551085668));
#30869=CARTESIAN_POINT('Ctrl Pts',(-1.6864963870894,-0.63630980009484,11.6749097837805));
#30870=CARTESIAN_POINT('Ctrl Pts',(-1.63575839200298,-0.31943490727698,
11.6201649167908));
#30871=CARTESIAN_POINT('Ctrl Pts',(-1.61595406457843,-0.158333333333244,
11.5853280034014));
#30872=CARTESIAN_POINT('Ctrl Pts',(-1.58711121341717,0.158333333333246,
11.595862223947));
#30873=CARTESIAN_POINT('Ctrl Pts',(-1.57727524413475,0.319434907276988,
11.6414988656436));
#30874=CARTESIAN_POINT('Ctrl Pts',(-1.57088676731849,0.636309800094849,
11.7171603612028));
#30875=CARTESIAN_POINT('Ctrl Pts',(-1.57188783305683,0.794772684000394,
11.786773485769));
#30876=CARTESIAN_POINT('Ctrl Pts',(-1.5927508350306,1.0684760419452,11.8441938322081));
#30877=CARTESIAN_POINT('Ctrl Pts',(-1.60681390531366,1.18514270861247,11.8606993865044));
#30878=CARTESIAN_POINT('Ctrl Pts',(-1.62590922537573,1.30000000000128,11.868855354757));
#30879=CARTESIAN_POINT('Ctrl Pts',(-1.84845170421517,-1.30000000000104,
11.7701972347928));
#30880=CARTESIAN_POINT('Ctrl Pts',(-1.81560919139068,-1.18514270861233,
11.7653832284769));
#30881=CARTESIAN_POINT('Ctrl Pts',(-1.78540136955671,-1.06847604194516,
11.7535113896969));
#30882=CARTESIAN_POINT('Ctrl Pts',(-1.72170192132254,-0.794772684000443,
11.709780062255));
#30883=CARTESIAN_POINT('Ctrl Pts',(-1.68903913893573,-0.636309800094871,
11.6517047122135));
#30884=CARTESIAN_POINT('Ctrl Pts',(-1.63792278128934,-0.319434907276996,
11.5969476183648));
#30885=CARTESIAN_POINT('Ctrl Pts',(-1.61757610966211,-0.158333333333251,
11.5631688638252));
#30886=CARTESIAN_POINT('Ctrl Pts',(-1.58903919989458,0.158333333333253,
11.5736565072532));
#30887=CARTESIAN_POINT('Ctrl Pts',(-1.58010994835879,0.319434907277002,
11.6181683609924));
#30888=CARTESIAN_POINT('Ctrl Pts',(-1.57460399261029,0.636309800094879,
11.6937880536352));
#30889=CARTESIAN_POINT('Ctrl Pts',(-1.57637841542004,0.794772684000434,
11.7627565934282));
#30890=CARTESIAN_POINT('Ctrl Pts',(-1.59709589115024,1.06847604194525,11.8233372447497));
#30891=CARTESIAN_POINT('Ctrl Pts',(-1.61082650864359,1.18514270861253,11.8420361414989));
#30892=CARTESIAN_POINT('Ctrl Pts',(-1.6293199160448,1.30000000000134,11.8532108157745));
#30893=CARTESIAN_POINT('Ctrl Pts',(-1.85026481461886,-1.30000000000114,
11.7456866281147));
#30894=CARTESIAN_POINT('Ctrl Pts',(-1.81775194196863,-1.18514270861242,
11.7361383865919));
#30895=CARTESIAN_POINT('Ctrl Pts',(-1.78773023179206,-1.06847604194524,
11.7208168877023));
#30896=CARTESIAN_POINT('Ctrl Pts',(-1.72412915913127,-0.794772684000502,
11.6720837807585));
#30897=CARTESIAN_POINT('Ctrl Pts',(-1.69081671649123,-0.636309800094919,
11.6150284922353));
#30898=CARTESIAN_POINT('Ctrl Pts',(-1.63974375521256,-0.31943490727702,
11.5601180730225));
#30899=CARTESIAN_POINT('Ctrl Pts',(-1.61949910327857,-0.158333333333264,
11.5278321545169));
#30900=CARTESIAN_POINT('Ctrl Pts',(-1.59203020234948,0.158333333333265,
11.5381217576227));
#30901=CARTESIAN_POINT('Ctrl Pts',(-1.58463938153361,0.319434907277029,
11.5808228501109));
#30902=CARTESIAN_POINT('Ctrl Pts',(-1.58009946425156,0.63630980009493,11.6564366711393));
#30903=CARTESIAN_POINT('Ctrl Pts',(-1.58198527480658,0.794772684000494,
11.7245355748381));
#30904=CARTESIAN_POINT('Ctrl Pts',(-1.60210979666633,1.06847604194533,11.7902488369403));
#30905=CARTESIAN_POINT('Ctrl Pts',(-1.61533602454307,1.18514270861261,11.8124693688438));
#30906=CARTESIAN_POINT('Ctrl Pts',(-1.63307732047047,1.30000000000143,11.8284655964033));
#30907=CARTESIAN_POINT('Ctrl Pts',(-1.85235418101203,-1.30000000000125,
11.7210849690256));
#30908=CARTESIAN_POINT('Ctrl Pts',(-1.82016905161149,-1.18514270861252,
11.7068025046435));
#30909=CARTESIAN_POINT('Ctrl Pts',(-1.79038984220925,-1.06847604194533,
11.6880184387967));
#30910=CARTESIAN_POINT('Ctrl Pts',(-1.72715206767857,-0.794772684000574,
11.6342238890251));
#30911=CARTESIAN_POINT('Ctrl Pts',(-1.69383554820921,-0.636309800094973,
11.5780448011396));
#30912=CARTESIAN_POINT('Ctrl Pts',(-1.64271773724477,-0.319434907277046,
11.5230000209639));
#30913=CARTESIAN_POINT('Ctrl Pts',(-1.6221146343507,-0.158333333333276,
11.4923232235877));
#30914=CARTESIAN_POINT('Ctrl Pts',(-1.59481395715236,0.158333333333278,
11.5025859059677));
#30915=CARTESIAN_POINT('Ctrl Pts',(-1.58771839974174,0.319434907277054,
11.5436832251077));
#30916=CARTESIAN_POINT('Ctrl Pts',(-1.58403735989905,0.636309800094981,
11.619310842894));
#30917=CARTESIAN_POINT('Ctrl Pts',(-1.58718536137325,0.794772684000561,
11.6863443221167));
#30918=CARTESIAN_POINT('Ctrl Pts',(-1.60750575379507,1.06847604194542,11.7570527056758));
#30919=CARTESIAN_POINT('Ctrl Pts',(-1.62052991615721,1.18514270861271,11.7827411501694));
#30920=CARTESIAN_POINT('Ctrl Pts',(-1.63778229594682,1.30000000000154,11.8035109999178));
#30921=CARTESIAN_POINT('Ctrl Pts',(-1.85396790840865,-1.30000000000128,
11.6965900695597));
#30922=CARTESIAN_POINT('Ctrl Pts',(-1.82229831568687,-1.18514270861255,
11.6775119375083));
#30923=CARTESIAN_POINT('Ctrl Pts',(-1.79268711193668,-1.06847604194536,
11.6552680903094));
#30924=CARTESIAN_POINT('Ctrl Pts',(-1.72903459787654,-0.794772684000596,
11.5965669181243));
#30925=CARTESIAN_POINT('Ctrl Pts',(-1.69367106033116,-0.63630980009499,
11.5417312925321));
#30926=CARTESIAN_POINT('Ctrl Pts',(-1.64213453885132,-0.319434907277055,
11.4866290091821));
#30927=CARTESIAN_POINT('Ctrl Pts',(-1.62226661781747,-0.158333333333281,
11.4573044263621));
#30928=CARTESIAN_POINT('Ctrl Pts',(-1.59612552676786,0.158333333333283,
11.4673180137663));
#30929=CARTESIAN_POINT('Ctrl Pts',(-1.58998142544728,0.319434907277065,
11.5066725383206));
#30930=CARTESIAN_POINT('Ctrl Pts',(-1.58800752304125,0.636309800095001,
11.5821384656179));
#30931=CARTESIAN_POINT('Ctrl Pts',(-1.5931292840274,0.794772684000582,11.6479698066803));
#30932=CARTESIAN_POINT('Ctrl Pts',(-1.61330891412657,1.06847604194545,11.7237468386099));
#30933=CARTESIAN_POINT('Ctrl Pts',(-1.6256891281828,1.18514270861275,11.7529951111915));
#30934=CARTESIAN_POINT('Ctrl Pts',(-1.64171454215429,1.30000000000158,11.7786905870478));
#30935=CARTESIAN_POINT('Ctrl Pts',(-1.85521388015686,-1.30000000000133,
11.6781712661894));
#30936=CARTESIAN_POINT('Ctrl Pts',(-1.82303326346136,-1.1851427086126,11.6557103919718));
#30937=CARTESIAN_POINT('Ctrl Pts',(-1.79317972753303,-1.0684760419454,11.6309624309223));
#30938=CARTESIAN_POINT('Ctrl Pts',(-1.72958810946243,-0.794772684000624,
11.5685060619735));
#30939=CARTESIAN_POINT('Ctrl Pts',(-1.69570308906305,-0.636309800095015,
11.513986001499));
#30940=CARTESIAN_POINT('Ctrl Pts',(-1.64411605157966,-0.319434907277068,
11.4587851770889));
#30941=CARTESIAN_POINT('Ctrl Pts',(-1.62282683086726,-0.158333333333287,
11.4309375845017));
#30942=CARTESIAN_POINT('Ctrl Pts',(-1.59651906306741,0.158333333333289,
11.4409915305209));
#30943=CARTESIAN_POINT('Ctrl Pts',(-1.59127716910426,0.319434907277074,
11.4789877912314));
#30944=CARTESIAN_POINT('Ctrl Pts',(-1.58973211930582,0.636309800095022,
11.5544748376688));
#30945=CARTESIAN_POINT('Ctrl Pts',(-1.59466018316317,0.794772684000613,
11.6196833551108));
#30946=CARTESIAN_POINT('Ctrl Pts',(-1.61519706666357,1.06847604194549,11.6991726405048));
#30947=CARTESIAN_POINT('Ctrl Pts',(-1.62780582852626,1.18514270861279,11.7309642964648));
#30948=CARTESIAN_POINT('Ctrl Pts',(-1.64413369635081,1.30000000000163,11.7601396421058));
#30949=CARTESIAN_POINT('Ctrl Pts',(-1.85517328864499,-1.30000000000137,
11.6601079860051));
#30950=CARTESIAN_POINT('Ctrl Pts',(-1.82348599895047,-1.18514270861263,
11.6340049138576));
#30951=CARTESIAN_POINT('Ctrl Pts',(-1.79380062463975,-1.06847604194542,
11.6066388522111));
#30952=CARTESIAN_POINT('Ctrl Pts',(-1.72984629646174,-0.794772684000645,
11.5405000168428));
#30953=CARTESIAN_POINT('Ctrl Pts',(-1.69408509803023,-0.63630980009503,
11.4870871937377));
#30954=CARTESIAN_POINT('Ctrl Pts',(-1.64208594211023,-0.319434907277075,
11.4318663463684));
#30955=CARTESIAN_POINT('Ctrl Pts',(-1.62119743812734,-0.158333333333291,
11.4050607229264));
#30956=CARTESIAN_POINT('Ctrl Pts',(-1.59637095195443,0.158333333333293,
11.4147786545005));
#30957=CARTESIAN_POINT('Ctrl Pts',(-1.59300281218603,0.319434907277083,
11.4511946083861));
#30958=CARTESIAN_POINT('Ctrl Pts',(-1.59327147535533,0.636309800095039,
11.5264293584128));
#30959=CARTESIAN_POINT('Ctrl Pts',(-1.59933219948415,0.794772684000632,
11.5908094443692));
#30960=CARTESIAN_POINT('Ctrl Pts',(-1.6195475915525,1.06847604194552,11.674151461135));
#30961=CARTESIAN_POINT('Ctrl Pts',(-1.63154715737108,1.18514270861282,11.7086452007729));
#30962=CARTESIAN_POINT('Ctrl Pts',(-1.64679579483592,1.30000000000166,11.7415570091167));
#30963=CARTESIAN_POINT('Ctrl Pts',(-1.85677772263928,-1.3000000000014,11.6415847248261));
#30964=CARTESIAN_POINT('Ctrl Pts',(-1.82500377440488,-1.18514270861266,
11.611990513213));
#30965=CARTESIAN_POINT('Ctrl Pts',(-1.79520315411112,-1.06847604194545,
11.5820846750055));
#30966=CARTESIAN_POINT('Ctrl Pts',(-1.73091654194481,-0.794772684000666,
11.5122762863304));
#30967=CARTESIAN_POINT('Ctrl Pts',(-1.69481730670943,-0.636309800095046,
11.4596117897729));
#30968=CARTESIAN_POINT('Ctrl Pts',(-1.64245260583326,-0.319434907277083,
11.4043689251971));
#30969=CARTESIAN_POINT('Ctrl Pts',(-1.62142968933603,-0.158333333333295,
11.3787472591335));
#30970=CARTESIAN_POINT('Ctrl Pts',(-1.59644123206918,0.158333333333297,
11.3884914891901));
#30971=CARTESIAN_POINT('Ctrl Pts',(-1.59274409701337,0.319434907277091,
11.4237993865481));
#30972=CARTESIAN_POINT('Ctrl Pts',(-1.59366238655238,0.636309800095055,
11.4990086854437));
#30973=CARTESIAN_POINT('Ctrl Pts',(-1.60104000459311,0.794772684000651,
11.5624606041692));
#30974=CARTESIAN_POINT('Ctrl Pts',(-1.62208616073324,1.06847604194555,11.649421942033));
#30975=CARTESIAN_POINT('Ctrl Pts',(-1.63430838227277,1.18514270861285,11.6864622644108));
#30976=CARTESIAN_POINT('Ctrl Pts',(-1.64964272419568,1.3000000000017,11.7229005682402));
#30977=CARTESIAN_POINT('Ctrl Pts',(-1.85593729332808,-1.30000000000142,
11.6267230412812));
#30978=CARTESIAN_POINT('Ctrl Pts',(-1.82401323334643,-1.18514270861268,
11.5942255222404));
#30979=CARTESIAN_POINT('Ctrl Pts',(-1.79411233921994,-1.06847604194547,
11.5621934861307));
#30980=CARTESIAN_POINT('Ctrl Pts',(-1.72970920999285,-0.794772684000676,
11.4892684334208));
#30981=CARTESIAN_POINT('Ctrl Pts',(-1.69376723753485,-0.636309800095055,
11.4371135776616));
#30982=CARTESIAN_POINT('Ctrl Pts',(-1.64133817124265,-0.319434907277087,
11.3817866822353));
#30983=CARTESIAN_POINT('Ctrl Pts',(-1.6198859209163,-0.158333333333297,
11.3572289053674));
#30984=CARTESIAN_POINT('Ctrl Pts',(-1.59533823300359,0.158333333333299,
11.3668610697367));
#30985=CARTESIAN_POINT('Ctrl Pts',(-1.59250251305007,0.319434907277096,
11.40098490634));
#30986=CARTESIAN_POINT('Ctrl Pts',(-1.59440068043849,0.636309800095065,
11.476066477427));
#30987=CARTESIAN_POINT('Ctrl Pts',(-1.6024690900727,0.794772684000662,11.5388338827361));
#30988=CARTESIAN_POINT('Ctrl Pts',(-1.62382938818921,1.06847604194556,11.6288861795763));
#30989=CARTESIAN_POINT('Ctrl Pts',(-1.63602578233119,1.18514270861287,11.6680908004979));
#30990=CARTESIAN_POINT('Ctrl Pts',(-1.65117248903756,1.30000000000172,11.7075197398054));
#30991=CARTESIAN_POINT('Ctrl Pts',(-1.85699869964041,-1.30000000000142,
11.6143622964803));
#30992=CARTESIAN_POINT('Ctrl Pts',(-1.82500430958963,-1.18514270861268,
11.5795349643121));
#30993=CARTESIAN_POINT('Ctrl Pts',(-1.79495934551754,-1.06847604194547,
11.5458224717731));
#30994=CARTESIAN_POINT('Ctrl Pts',(-1.73005303202881,-0.79477268400068,
11.4705153724133));
#30995=CARTESIAN_POINT('Ctrl Pts',(-1.69344725687642,-0.636309800095058,
11.4189678952462));
#30996=CARTESIAN_POINT('Ctrl Pts',(-1.64045500640219,-0.319434907277089,
11.3637094229155));
#30997=CARTESIAN_POINT('Ctrl Pts',(-1.61863681283758,-0.158333333333298,
11.3400169850387));
#30998=CARTESIAN_POINT('Ctrl Pts',(-1.5944140512909,0.1583333333333,11.3495655171347));
#30999=CARTESIAN_POINT('Ctrl Pts',(-1.59238937323836,0.319434907277097,
11.382696200417));
#31000=CARTESIAN_POINT('Ctrl Pts',(-1.59526779410525,0.636309800095067,
11.4576289911575));
#31001=CARTESIAN_POINT('Ctrl Pts',(-1.60427319996494,0.794772684000666,
11.5197753878327));
#31002=CARTESIAN_POINT('Ctrl Pts',(-1.62572020818096,1.06847604194557,11.6123407970366));
#31003=CARTESIAN_POINT('Ctrl Pts',(-1.63769439053449,1.18514270861288,11.6533220654616));
#31004=CARTESIAN_POINT('Ctrl Pts',(-1.65235914007478,1.30000000000172,11.6952164665535));
#31005=CARTESIAN_POINT('Ctrl Pts',(-1.85707299808195,-1.30000000000145,
11.5962359591747));
#31006=CARTESIAN_POINT('Ctrl Pts',(-1.8250340456161,-1.1851427086127,11.5578966099453));
#31007=CARTESIAN_POINT('Ctrl Pts',(-1.79487638163994,-1.06847604194549,
11.5216352984547));
#31008=CARTESIAN_POINT('Ctrl Pts',(-1.72955229759684,-0.794772684000693,
11.4426650977481));
#31009=CARTESIAN_POINT('Ctrl Pts',(-1.69226227430237,-0.636309800095069,
11.3919488679483));
#31010=CARTESIAN_POINT('Ctrl Pts',(-1.63899399294016,-0.319434907277095,
11.3366395947736));
#31011=CARTESIAN_POINT('Ctrl Pts',(-1.6173140649551,-0.158333333333301,
11.3140597026112));
#31012=CARTESIAN_POINT('Ctrl Pts',(-1.59346344526089,0.158333333333303,
11.323505276146));
#31013=CARTESIAN_POINT('Ctrl Pts',(-1.59178184641142,0.319434907277104,
11.3553793032582));
#31014=CARTESIAN_POINT('Ctrl Pts',(-1.59547188581878,0.636309800095079,
11.4302369991131));
#31015=CARTESIAN_POINT('Ctrl Pts',(-1.60509054103872,0.794772684000681,
11.4915906889066));
#31016=CARTESIAN_POINT('Ctrl Pts',(-1.62742089479516,1.06847604194558,11.5877592904259));
#31017=CARTESIAN_POINT('Ctrl Pts',(-1.63977269513233,1.1851427086129,11.6312552112791));
#31018=CARTESIAN_POINT('Ctrl Pts',(-1.65481031308663,1.30000000000174,11.6766192287855));
#31019=CARTESIAN_POINT('Ctrl Pts',(-1.85782405239422,-1.30000000000149,
11.5718563713316));
#31020=CARTESIAN_POINT('Ctrl Pts',(-1.82511466019596,-1.18514270861274,
11.5289860257926));
#31021=CARTESIAN_POINT('Ctrl Pts',(-1.79433950157869,-1.06847604194552,
11.4894453770448));
#31022=CARTESIAN_POINT('Ctrl Pts',(-1.72771119513777,-0.794772684000718,
11.405790834049));
#31023=CARTESIAN_POINT('Ctrl Pts',(-1.68954961974983,-0.636309800095088,
11.3561967971218));
#31024=CARTESIAN_POINT('Ctrl Pts',(-1.63562300718043,-0.319434907277103,
11.3009078818754));
#31025=CARTESIAN_POINT('Ctrl Pts',(-1.61379601219274,-0.158333333333305,
11.2799023853609));
#31026=CARTESIAN_POINT('Ctrl Pts',(-1.59069699733874,0.158333333333307,
11.2891319462005));
#31027=CARTESIAN_POINT('Ctrl Pts',(-1.58991024511068,0.319434907277113,
11.3191733505662));
#31028=CARTESIAN_POINT('Ctrl Pts',(-1.59579737236803,0.636309800095098,
11.3936566738865));
#31029=CARTESIAN_POINT('Ctrl Pts',(-1.60818428931505,0.794772684000702,
11.4535424940212));
#31030=CARTESIAN_POINT('Ctrl Pts',(-1.63125865236166,1.06847604194561,11.5546095191125));
#31031=CARTESIAN_POINT('Ctrl Pts',(-1.64334165504426,1.18514270861293,11.6016267147841));
#31032=CARTESIAN_POINT('Ctrl Pts',(-1.65751962363596,1.30000000000179,11.6519129358675));
#31033=CARTESIAN_POINT('Ctrl Pts',(-1.85678181360715,-1.30000000000152,
11.5479686431218));
#31034=CARTESIAN_POINT('Ctrl Pts',(-1.82362997352617,-1.18514270861277,
11.5005091509062));
#31035=CARTESIAN_POINT('Ctrl Pts',(-1.79241924785772,-1.06847604194555,
11.457642418012));
#31036=CARTESIAN_POINT('Ctrl Pts',(-1.72480059049101,-0.79477268400074,
11.3692218823769));
#31037=CARTESIAN_POINT('Ctrl Pts',(-1.68579469115041,-0.636309800095108,
11.3207420009397));
#31038=CARTESIAN_POINT('Ctrl Pts',(-1.63138961270452,-0.319434907277114,
11.265422664141));
#31039=CARTESIAN_POINT('Ctrl Pts',(-1.60961523247916,-0.15833333333331,
11.2459371441337));
#31040=CARTESIAN_POINT('Ctrl Pts',(-1.58718054123095,0.158333333333312,
11.2549647313119));
#31041=CARTESIAN_POINT('Ctrl Pts',(-1.58732163867687,0.319434907277123,
11.2831821703496));
#31042=CARTESIAN_POINT('Ctrl Pts',(-1.59439645505399,0.636309800095118,
11.3574923069509));
#31043=CARTESIAN_POINT('Ctrl Pts',(-1.60718994603995,0.79477268400073,11.4163823312034));
#31044=CARTESIAN_POINT('Ctrl Pts',(-1.63150163440477,1.06847604194565,11.5222213562515));
#31045=CARTESIAN_POINT('Ctrl Pts',(-1.64419640242279,1.18514270861297,11.5725657031935));
#31046=CARTESIAN_POINT('Ctrl Pts',(-1.65906230940252,1.30000000000182,11.6274406048564));
#31047=CARTESIAN_POINT('Ctrl Pts',(-1.85646792992249,-1.30000000000154,
11.5238562660431));
#31048=CARTESIAN_POINT('Ctrl Pts',(-1.82287519950759,-1.18514270861279,
11.4717906712953));
#31049=CARTESIAN_POINT('Ctrl Pts',(-1.79110499396969,-1.06847604194556,
11.4256234324653));
#31050=CARTESIAN_POINT('Ctrl Pts',(-1.7219198606302,-0.794772684000747,
11.3325942571756));
#31051=CARTESIAN_POINT('Ctrl Pts',(-1.68117947256001,-0.636309800095115,
11.2855035822367));
#31052=CARTESIAN_POINT('Ctrl Pts',(-1.62549156015531,-0.319434907277118,
11.2303944130328));
#31053=CARTESIAN_POINT('Ctrl Pts',(-1.60321674177326,-0.158333333333312,
11.2125995993871));
#31054=CARTESIAN_POINT('Ctrl Pts',(-1.58171314091487,0.158333333333314,
11.2213342239253));
#31055=CARTESIAN_POINT('Ctrl Pts',(-1.58370410867213,0.319434907277129,
11.247408138762));
#31056=CARTESIAN_POINT('Ctrl Pts',(-1.59310619103803,0.636309800095127,
11.3212369774957));
#31057=CARTESIAN_POINT('Ctrl Pts',(-1.60751436014146,0.794772684000738,
11.3788835799511));
#31058=CARTESIAN_POINT('Ctrl Pts',(-1.63309938464165,1.06847604194566,11.48949665088));
#31059=CARTESIAN_POINT('Ctrl Pts',(-1.6460822009907,1.18514270861298,11.5432480259809));
#31060=CARTESIAN_POINT('Ctrl Pts',(-1.66097302460121,1.30000000000184,11.6028704763956));
#31061=CARTESIAN_POINT('Ctrl Pts',(-1.85497966222603,-1.30000000000162,
11.503126144964));
#31062=CARTESIAN_POINT('Ctrl Pts',(-1.82046411571729,-1.18514270861286,
11.447225295674));
#31063=CARTESIAN_POINT('Ctrl Pts',(-1.78795658628739,-1.06847604194563,
11.3982726438186));
#31064=CARTESIAN_POINT('Ctrl Pts',(-1.71749661135009,-0.794772684000801,
11.3012339511447));
#31065=CARTESIAN_POINT('Ctrl Pts',(-1.67661303372963,-0.636309800095154,
11.2549667049729));
#31066=CARTESIAN_POINT('Ctrl Pts',(-1.62024236111357,-0.319434907277136,
11.1999267400399));
#31067=CARTESIAN_POINT('Ctrl Pts',(-1.59734283762842,-0.158333333333322,
11.1836644064143));
#31068=CARTESIAN_POINT('Ctrl Pts',(-1.57606607100608,0.158333333333324,
11.1922991148789));
#31069=CARTESIAN_POINT('Ctrl Pts',(-1.57850038582121,0.319434907277148,
11.2168226451961));
#31070=CARTESIAN_POINT('Ctrl Pts',(-1.58987873169088,0.636309800095166,
11.2902117061397));
#31071=CARTESIAN_POINT('Ctrl Pts',(-1.6066555036954,0.794772684000786,11.3464567262519));
#31072=CARTESIAN_POINT('Ctrl Pts',(-1.63423517695353,1.06847604194573,11.4609670321102));
#31073=CARTESIAN_POINT('Ctrl Pts',(-1.64786544209433,1.18514270861305,11.517579383574));
#31074=CARTESIAN_POINT('Ctrl Pts',(-1.66318775375007,1.30000000000192,11.5812368181202));
#31075=CARTESIAN_POINT('Ctrl Pts',(-1.85439311555595,-1.30000000000162,
11.479046302207));
#31076=CARTESIAN_POINT('Ctrl Pts',(-1.81905279421378,-1.18514270861286,
11.4186174863998));
#31077=CARTESIAN_POINT('Ctrl Pts',(-1.78561431754195,-1.06847604194563,
11.3664538237022));
#31078=CARTESIAN_POINT('Ctrl Pts',(-1.71275838873707,-0.794772684000798,
11.2650394846877));
#31079=CARTESIAN_POINT('Ctrl Pts',(-1.66915843970215,-0.636309800095153,
11.2205097819443));
#31080=CARTESIAN_POINT('Ctrl Pts',(-1.61171114271454,-0.319434907277136,
11.1656297732224));
#31081=CARTESIAN_POINT('Ctrl Pts',(-1.59001006088378,-0.158333333333322,
11.1505468454814));
#31082=CARTESIAN_POINT('Ctrl Pts',(-1.56976350919437,0.158333333333324,
11.1588237730732));
#31083=CARTESIAN_POINT('Ctrl Pts',(-1.57276507097241,0.319434907277148,
11.181547746742));
#31084=CARTESIAN_POINT('Ctrl Pts',(-1.58582040791484,0.636309800095165,
11.2545825061741));
#31085=CARTESIAN_POINT('Ctrl Pts',(-1.60409543978382,0.794772684000785,
11.3095345616161));
#31086=CARTESIAN_POINT('Ctrl Pts',(-1.63311358253654,1.06847604194572,11.4287799832022));
#31087=CARTESIAN_POINT('Ctrl Pts',(-1.64722663290145,1.18514270861305,11.4887710035572));
#31088=CARTESIAN_POINT('Ctrl Pts',(-1.66289185486174,1.30000000000192,11.5571361197408));
#31089=CARTESIAN_POINT('Ctrl Pts',(-1.85283978068215,-1.30000000000165,
11.4613539877658));
#31090=CARTESIAN_POINT('Ctrl Pts',(-1.81653046021035,-1.18514270861288,
11.3977033856574));
#31091=CARTESIAN_POINT('Ctrl Pts',(-1.78227987318513,-1.06847604194565,
11.3432193821066));
#31092=CARTESIAN_POINT('Ctrl Pts',(-1.70791025146048,-0.794772684000815,
11.2385271108567));
#31093=CARTESIAN_POINT('Ctrl Pts',(-1.66388043844242,-0.636309800095166,
11.1948258070879));
#31094=CARTESIAN_POINT('Ctrl Pts',(-1.60549196134081,-0.319434907277143,
11.1401340976286));
#31095=CARTESIAN_POINT('Ctrl Pts',(-1.58304092552731,-0.158333333333325,
11.1264343755906));
#31096=CARTESIAN_POINT('Ctrl Pts',(-1.56306004713795,0.158333333333327,
11.1345883393377));
#31097=CARTESIAN_POINT('Ctrl Pts',(-1.56688524947397,0.319434907277154,
11.1558281168516));
#31098=CARTESIAN_POINT('Ctrl Pts',(-1.58181398704839,0.636309800095178,
11.2283793503045));
#31099=CARTESIAN_POINT('Ctrl Pts',(-1.60173505635853,0.7947726840008,11.2821786309543));
#31100=CARTESIAN_POINT('Ctrl Pts',(-1.63288796102298,1.06847604194575,11.4046189681354));
#31101=CARTESIAN_POINT('Ctrl Pts',(-1.64789044572972,1.18514270861308,11.4669682801649));
#31102=CARTESIAN_POINT('Ctrl Pts',(-1.6644104770428,1.30000000000195,11.5386670191196));
#31103=CARTESIAN_POINT('Ctrl Pts',(-1.85127630062499,-1.30000000000166,
11.4435752287505));
#31104=CARTESIAN_POINT('Ctrl Pts',(-1.81422237239857,-1.1851427086129,11.3764712734879));
#31105=CARTESIAN_POINT('Ctrl Pts',(-1.77912863126938,-1.06847604194567,
11.3195571370201));
#31106=CARTESIAN_POINT('Ctrl Pts',(-1.70258349311097,-0.794772684000825,
11.2116146160284));
#31107=CARTESIAN_POINT('Ctrl Pts',(-1.65551483630903,-0.636309800095177,
11.1695933113041));
#31108=CARTESIAN_POINT('Ctrl Pts',(-1.5972515116615,-0.319434907277149,
11.1147106253092));
#31109=CARTESIAN_POINT('Ctrl Pts',(-1.57844403382631,-0.158333333333327,
11.1010015815054));
#31110=CARTESIAN_POINT('Ctrl Pts',(-1.55960633153799,0.158333333333329,
11.1087413101428));
#31111=CARTESIAN_POINT('Ctrl Pts',(-1.56165830827601,0.319434907277156,
11.1292984694153));
#31112=CARTESIAN_POINT('Ctrl Pts',(-1.5773092958189,0.636309800095185,11.2017625771917));
#31113=CARTESIAN_POINT('Ctrl Pts',(-1.59911202315622,0.794772684000816,
11.2543443596096));
#31114=CARTESIAN_POINT('Ctrl Pts',(-1.63186631980178,1.06847604194577,11.3802996735384));
#31115=CARTESIAN_POINT('Ctrl Pts',(-1.64747792500286,1.1851427086131,11.4451896980575));
#31116=CARTESIAN_POINT('Ctrl Pts',(-1.66452301405345,1.30000000000196,11.5204483588001));
#31117=CARTESIAN_POINT('Ctrl Pts',(-1.84999209719009,-1.30000000000168,
11.428875041091));
#31118=CARTESIAN_POINT('Ctrl Pts',(-1.81145567664774,-1.18514270861291,
11.3594133583039));
#31119=CARTESIAN_POINT('Ctrl Pts',(-1.77547447896192,-1.06847604194568,
11.3007184692798));
#31120=CARTESIAN_POINT('Ctrl Pts',(-1.69825379026308,-0.794772684000835,
11.1899949812443));
#31121=CARTESIAN_POINT('Ctrl Pts',(-1.65307034145157,-0.636309800095182,
11.1479416751912));
#31122=CARTESIAN_POINT('Ctrl Pts',(-1.59561809421317,-0.319434907277151,
11.0927623076994));
#31123=CARTESIAN_POINT('Ctrl Pts',(-1.57728391425471,-0.158333333333329,
11.0798877614763));
#31124=CARTESIAN_POINT('Ctrl Pts',(-1.55783439338415,0.158333333333331,
11.0878072633641));
#31125=CARTESIAN_POINT('Ctrl Pts',(-1.55789660512953,0.31943490727716,11.1079948388319));
#31126=CARTESIAN_POINT('Ctrl Pts',(-1.57333298878991,0.636309800095192,
11.180541002553));
#31127=CARTESIAN_POINT('Ctrl Pts',(-1.59648543095614,0.794772684000821,
11.2320874284867));
#31128=CARTESIAN_POINT('Ctrl Pts',(-1.63042741542663,1.06847604194577,11.3606986517709));
#31129=CARTESIAN_POINT('Ctrl Pts',(-1.64657384485488,1.18514270861311,11.4275162264943));
#31130=CARTESIAN_POINT('Ctrl Pts',(-1.66417447630853,1.30000000000197,11.5054803428965));
#31131=CARTESIAN_POINT('Ctrl Pts',(-1.84771283470326,-1.30000000000168,
11.4113225100421));
#31132=CARTESIAN_POINT('Ctrl Pts',(-1.80731363076414,-1.18514270861292,
11.3386533475872));
#31133=CARTESIAN_POINT('Ctrl Pts',(-1.77035638698582,-1.06847604194568,
11.2774682075166));
#31134=CARTESIAN_POINT('Ctrl Pts',(-1.69292937712006,-0.794772684000837,
11.1626486829874));
#31135=CARTESIAN_POINT('Ctrl Pts',(-1.65105873820579,-0.636309800095186,
11.120072742534));
#31136=CARTESIAN_POINT('Ctrl Pts',(-1.59560967356912,-0.319434907277153,
11.0640491644009));
#31137=CARTESIAN_POINT('Ctrl Pts',(-1.57811365915877,-0.158333333333329,
11.0522220810441));
#31138=CARTESIAN_POINT('Ctrl Pts',(-1.55877072607704,0.158333333333331,
11.0600832218156));
#31139=CARTESIAN_POINT('Ctrl Pts',(-1.55780038665591,0.319434907277161,
11.0792447767487));
#31140=CARTESIAN_POINT('Ctrl Pts',(-1.57206376052553,0.636309800095195,
11.1523537198416));
#31141=CARTESIAN_POINT('Ctrl Pts',(-1.59362547973182,0.794772684000825,
11.2038774329937));
#31142=CARTESIAN_POINT('Ctrl Pts',(-1.62793948407771,1.06847604194578,11.3365871526014));
#31143=CARTESIAN_POINT('Ctrl Pts',(-1.64475372341218,1.18514270861312,11.4060302996696));
#31144=CARTESIAN_POINT('Ctrl Pts',(-1.66352894105892,1.30000000000199,11.4874714735672));
#31145=CARTESIAN_POINT('Ctrl Pts',(-1.84624880074947,-1.30000000000171,
11.3993427675283));
#31146=CARTESIAN_POINT('Ctrl Pts',(-1.80327012405174,-1.18514270861294,
11.3249050934222));
#31147=CARTESIAN_POINT('Ctrl Pts',(-1.76517783186742,-1.0684760419457,11.2622670815724));
#31148=CARTESIAN_POINT('Ctrl Pts',(-1.68846554232873,-0.794772684000851,
11.1448203238348));
#31149=CARTESIAN_POINT('Ctrl Pts',(-1.65309822965784,-0.636309800095197,
11.1012255285408));
#31150=CARTESIAN_POINT('Ctrl Pts',(-1.60107891377445,-0.319434907277159,
11.0445426182858));
#31151=CARTESIAN_POINT('Ctrl Pts',(-1.58369000879615,-0.158333333333332,
11.0337845707418));
#31152=CARTESIAN_POINT('Ctrl Pts',(-1.56451256417064,0.158333333333334,
11.0416309199903));
#31153=CARTESIAN_POINT('Ctrl Pts',(-1.56349013317763,0.319434907277167,
11.0598112207703));
#31154=CARTESIAN_POINT('Ctrl Pts',(-1.5748858670137,0.636309800095206,11.1333404325303));
#31155=CARTESIAN_POINT('Ctrl Pts',(-1.59090434066293,0.79477268400084,11.1852921644308));
#31156=CARTESIAN_POINT('Ctrl Pts',(-1.62444818679958,1.0684760419458,11.3206583385472));
#31157=CARTESIAN_POINT('Ctrl Pts',(-1.6421192747162,1.18514270861313,11.3917118019926));
#31158=CARTESIAN_POINT('Ctrl Pts',(-1.66294156247886,1.300000000002,11.4752237279192));
#31159=CARTESIAN_POINT('Ctrl Pts',(-1.84783999216086,-1.30000000000171,
11.3908891462741));
#31160=CARTESIAN_POINT('Ctrl Pts',(-1.80484358765992,-1.18514270861294,
11.3167021552094));
#31161=CARTESIAN_POINT('Ctrl Pts',(-1.76706466618289,-1.0684760419457,11.254208104176));
#31162=CARTESIAN_POINT('Ctrl Pts',(-1.69184122946293,-0.794772684000851,
11.1368473750342));
#31163=CARTESIAN_POINT('Ctrl Pts',(-1.65901382561028,-0.636309800095197,
11.0928893630096));
#31164=CARTESIAN_POINT('Ctrl Pts',(-1.60867204426711,-0.319434907277159,
11.0360319972763));
#31165=CARTESIAN_POINT('Ctrl Pts',(-1.59125278366871,-0.158333333333332,
11.0252313037607));
#31166=CARTESIAN_POINT('Ctrl Pts',(-1.57231214945024,0.158333333333334,
11.033074834932));
#31167=CARTESIAN_POINT('Ctrl Pts',(-1.57183510628244,0.319434907277167,
11.0512628906174));
#31168=CARTESIAN_POINT('Ctrl Pts',(-1.58146895355656,0.636309800095206,
11.1250261480047));
#31169=CARTESIAN_POINT('Ctrl Pts',(-1.59387972389892,0.79477268400084,11.1775265523141));
#31170=CARTESIAN_POINT('Ctrl Pts',(-1.62608364872306,1.0684760419458,11.31276909021));
#31171=CARTESIAN_POINT('Ctrl Pts',(-1.64375431751357,1.18514270861313,11.3836121285189));
#31172=CARTESIAN_POINT('Ctrl Pts',(-1.6651557693112,1.300000000002,11.4667567217115));
#31173=CARTESIAN_POINT('Ctrl Pts',(-1.84783999216022,-1.3,11.390889146273));
#31174=CARTESIAN_POINT('Ctrl Pts',(-1.80484358765955,-1.18514270861178,
11.3167021552088));
#31175=CARTESIAN_POINT('Ctrl Pts',(-1.76706466618273,-1.06847604194512,
11.2542081041758));
#31176=CARTESIAN_POINT('Ctrl Pts',(-1.69184122946293,-0.794772684000851,
11.1368473750342));
#31177=CARTESIAN_POINT('Ctrl Pts',(-1.65901382561028,-0.636309800095197,
11.0928893630096));
#31178=CARTESIAN_POINT('Ctrl Pts',(-1.60867204426711,-0.319434907277159,
11.0360319972763));
#31179=CARTESIAN_POINT('Ctrl Pts',(-1.59125278366871,-0.158333333333332,
11.0252313037607));
#31180=CARTESIAN_POINT('Ctrl Pts',(-1.57231214945024,0.158333333333334,
11.0330748349321));
#31181=CARTESIAN_POINT('Ctrl Pts',(-1.57183510628244,0.319434907277167,
11.0512628906174));
#31182=CARTESIAN_POINT('Ctrl Pts',(-1.58146895355656,0.636309800095206,
11.1250261480047));
#31183=CARTESIAN_POINT('Ctrl Pts',(-1.59387972389892,0.79477268400084,11.1775265523141));
#31184=CARTESIAN_POINT('Ctrl Pts',(-1.62608364872298,1.06847604194511,11.3127690902096));
#31185=CARTESIAN_POINT('Ctrl Pts',(-1.64375431751336,1.18514270861178,11.3836121285181));
#31186=CARTESIAN_POINT('Ctrl Pts',(-1.66515576931083,1.3,11.46675672171));
#31187=CARTESIAN_POINT('',(-1.81605431981429,-1.2,11.8048286295457));
#31188=CARTESIAN_POINT('Ctrl Pts',(-1.81605431981429,-1.2,11.8048286295457));
#31189=CARTESIAN_POINT('Ctrl Pts',(-1.8224693082947,-1.21682682923595,11.784210539298));
#31190=CARTESIAN_POINT('Ctrl Pts',(-1.82985488839019,-1.23325265804367,
11.7635755607979));
#31191=CARTESIAN_POINT('Ctrl Pts',(-1.83949601009123,-1.25864666032482,
11.7322887234019));
#31192=CARTESIAN_POINT('Ctrl Pts',(-1.84264810997846,-1.26676758279304,
11.7222392924128));
#31193=CARTESIAN_POINT('Ctrl Pts',(-1.84816644744311,-1.28141938382527,
11.704152355739));
#31194=CARTESIAN_POINT('Ctrl Pts',(-1.85203392632938,-1.2918719144206,11.6912581966035));
#31195=CARTESIAN_POINT('Ctrl Pts',(-1.85435152969323,-1.29845760775963,
11.6831734697223));
#31196=CARTESIAN_POINT('Ctrl Pts',(-1.85461944199808,-1.29922939086495,
11.6822274140474));
#31197=CARTESIAN_POINT('Ctrl Pts',(-1.85488174056831,-1.30000000000132,
11.681284830101));
#31198=CARTESIAN_POINT('',(-1.66957757387615,-0.653834841327789,11.859936772574));
#31199=CARTESIAN_POINT('Ctrl Pts',(-1.66957757394783,-0.653834841312355,
11.8599367725936));
#31200=CARTESIAN_POINT('Ctrl Pts',(-1.68331792633201,-0.711381237877385,
11.855013833653));
#31201=CARTESIAN_POINT('Ctrl Pts',(-1.69787379089,-0.767209767909677,11.8497287246474));
#31202=CARTESIAN_POINT('Ctrl Pts',(-1.72809951098891,-0.881631787835512,
11.8385815155201));
#31203=CARTESIAN_POINT('Ctrl Pts',(-1.7425600255146,-0.939021335919122,
11.8331784821344));
#31204=CARTESIAN_POINT('Ctrl Pts',(-1.7696575090577,-1.03714199995114,11.8228685450684));
#31205=CARTESIAN_POINT('Ctrl Pts',(-1.77053344226464,-1.03956800238679,
11.8225595794184));
#31206=CARTESIAN_POINT('Ctrl Pts',(-1.79854255260691,-1.13871222069374,
11.8117107047821));
#31207=CARTESIAN_POINT('Ctrl Pts',(-1.80621282339748,-1.16608661241795,
11.8087099231875));
#31208=CARTESIAN_POINT('Ctrl Pts',(-1.81605431981429,-1.2,11.8048286295457));
#31209=CARTESIAN_POINT('',(-1.53759581372313,0.653834841531101,11.9051353980115));
#31210=CARTESIAN_POINT('Ctrl Pts',(-1.53759581372313,0.65383484153109,11.9051353980115));
#31211=CARTESIAN_POINT('Ctrl Pts',(-1.54254163045076,0.575731842989942,
11.8637235483156));
#31212=CARTESIAN_POINT('Ctrl Pts',(-1.54764148398872,0.493687693661655,
11.8289822069527));
#31213=CARTESIAN_POINT('Ctrl Pts',(-1.55719804912996,0.338068747436532,
11.77922986672));
#31214=CARTESIAN_POINT('Ctrl Pts',(-1.56183985947927,0.265610792759769,
11.7619048341106));
#31215=CARTESIAN_POINT('Ctrl Pts',(-1.57217181134277,0.129684268044095,
11.7397699428473));
#31216=CARTESIAN_POINT('Ctrl Pts',(-1.57755262396628,0.0666361292480136,
11.7335211393323));
#31217=CARTESIAN_POINT('Ctrl Pts',(-1.58999125690634,-0.0594726585747696,
11.7288642981296));
#31218=CARTESIAN_POINT('Ctrl Pts',(-1.59712426033947,-0.122669256307556,
11.7304095744559));
#31219=CARTESIAN_POINT('Ctrl Pts',(-1.6137045597392,-0.26003767749522,11.7427010308845));
#31220=CARTESIAN_POINT('Ctrl Pts',(-1.62337943103797,-0.333902462181384,
11.7550658391387));
#31221=CARTESIAN_POINT('Ctrl Pts',(-1.64492749970498,-0.491493397975319,
11.7944688143506));
#31222=CARTESIAN_POINT('Ctrl Pts',(-1.65731202392141,-0.574905812515696,
11.8237247520087));
#31223=CARTESIAN_POINT('Ctrl Pts',(-1.66957757397199,-0.653834841350482,
11.8599367724921));
#31224=CARTESIAN_POINT('',(-1.60611120272456,1.2,11.8821903853306));
#31225=CARTESIAN_POINT('Ctrl Pts',(-1.60611120272456,1.2,11.8821903853306));
#31226=CARTESIAN_POINT('Ctrl Pts',(-1.59468073958328,1.13608709176311,11.886111326897));
#31227=CARTESIAN_POINT('Ctrl Pts',(-1.57885340667937,1.03790194753826,11.8914890260236));
#31228=CARTESIAN_POINT('Ctrl Pts',(-1.54889218107653,0.796896277865386,
11.9014466204779));
#31229=CARTESIAN_POINT('Ctrl Pts',(-1.54381784356845,0.741365964363796,
11.9031020947729));
#31230=CARTESIAN_POINT('Ctrl Pts',(-1.53759581372313,0.653834841531101,
11.9051353980115));
#31231=CARTESIAN_POINT('Ctrl Pts',(-1.64379217587217,1.29999999999989,11.762942831391));
#31232=CARTESIAN_POINT('Ctrl Pts',(-1.63815094958981,1.28313650166177,11.7828994633125));
#31233=CARTESIAN_POINT('Ctrl Pts',(-1.63164049333543,1.26654456688836,11.8028295456687));
#31234=CARTESIAN_POINT('Ctrl Pts',(-1.6213586730226,1.23847789472489,11.8361962431637));
#31235=CARTESIAN_POINT('Ctrl Pts',(-1.61473656949771,1.21946613476643,11.858652114516));
#31236=CARTESIAN_POINT('Ctrl Pts',(-1.60611120272456,1.2,11.8821903853306));
#31237=CARTESIAN_POINT('Ctrl Pts',(-1.84783999216022,-1.3,11.390889146273));
#31238=CARTESIAN_POINT('Ctrl Pts',(-1.80484358765955,-1.18514270861178,
11.3167021552088));
#31239=CARTESIAN_POINT('Ctrl Pts',(-1.76706466618273,-1.06847604194512,
11.2542081041758));
#31240=CARTESIAN_POINT('Ctrl Pts',(-1.69184122946293,-0.794772684000851,
11.1368473750342));
#31241=CARTESIAN_POINT('Ctrl Pts',(-1.65901382561028,-0.636309800095197,
11.0928893630096));
#31242=CARTESIAN_POINT('Ctrl Pts',(-1.60867204426711,-0.319434907277159,
11.0360319972763));
#31243=CARTESIAN_POINT('Ctrl Pts',(-1.59125278366871,-0.158333333333332,
11.0252313037607));
#31244=CARTESIAN_POINT('Ctrl Pts',(-1.57231214945024,0.158333333333334,
11.0330748349321));
#31245=CARTESIAN_POINT('Ctrl Pts',(-1.57183510628244,0.319434907277167,
11.0512628906174));
#31246=CARTESIAN_POINT('Ctrl Pts',(-1.58146895355656,0.636309800095206,
11.1250261480047));
#31247=CARTESIAN_POINT('Ctrl Pts',(-1.59387972389892,0.79477268400084,11.1775265523141));
#31248=CARTESIAN_POINT('Ctrl Pts',(-1.62608364872297,1.06847604194511,11.3127690902096));
#31249=CARTESIAN_POINT('Ctrl Pts',(-1.64375431751336,1.18514270861178,11.3836121285181));
#31250=CARTESIAN_POINT('Ctrl Pts',(-1.66515576931083,1.3,11.46675672171));
#31251=CARTESIAN_POINT('Ctrl Pts',(-1.91743049134307,-1.3,11.3580825661689));
#31252=CARTESIAN_POINT('Ctrl Pts',(-1.87294351908303,-1.18514270861178,
11.2847782487198));
#31253=CARTESIAN_POINT('Ctrl Pts',(-1.83415002075929,-1.06847604194512,
11.2229371776131));
#31254=CARTESIAN_POINT('Ctrl Pts',(-1.75768234278715,-0.794772684000851,
11.1065543243585));
#31255=CARTESIAN_POINT('Ctrl Pts',(-1.72556041438092,-0.636309800095197,
11.0624647739656));
#31256=CARTESIAN_POINT('Ctrl Pts',(-1.67587573316224,-0.319434907277159,
11.0057209978454));
#31257=CARTESIAN_POINT('Ctrl Pts',(-1.65965103821258,-0.158333333333332,
10.9945819779792));
#31258=CARTESIAN_POINT('Ctrl Pts',(-1.64085640284598,0.158333333333334,
11.0027534279408));
#31259=CARTESIAN_POINT('Ctrl Pts',(-1.6393286137645,0.319434907277167,11.0216028343905));
#31260=CARTESIAN_POINT('Ctrl Pts',(-1.64860718876712,0.636309800095206,
11.0959304186219));
#31261=CARTESIAN_POINT('Ctrl Pts',(-1.66044815183843,0.79477268400084,11.1488670770106));
#31262=CARTESIAN_POINT('Ctrl Pts',(-1.69421133997152,1.06847604194511,11.283839290143));
#31263=CARTESIAN_POINT('Ctrl Pts',(-1.71304615183609,1.18514270861178,11.3543652797717));
#31264=CARTESIAN_POINT('Ctrl Pts',(-1.73610094247183,1.3,11.4369927891775));
#31265=CARTESIAN_POINT('Ctrl Pts',(-1.98702099052593,-1.3,11.3252759860648));
#31266=CARTESIAN_POINT('Ctrl Pts',(-1.9410434505065,-1.18514270861178,11.2528543422308));
#31267=CARTESIAN_POINT('Ctrl Pts',(-1.90123537533586,-1.06847604194512,
11.1916662510505));
#31268=CARTESIAN_POINT('Ctrl Pts',(-1.82352345611138,-0.794772684000851,
11.0762612736829));
#31269=CARTESIAN_POINT('Ctrl Pts',(-1.79210700315155,-0.636309800095197,
11.0320401849215));
#31270=CARTESIAN_POINT('Ctrl Pts',(-1.74307942205737,-0.319434907277159,
10.9754099984145));
#31271=CARTESIAN_POINT('Ctrl Pts',(-1.72804929275646,-0.158333333333332,
10.9639326521977));
#31272=CARTESIAN_POINT('Ctrl Pts',(-1.70940065624173,0.158333333333334,
10.9724320209495));
#31273=CARTESIAN_POINT('Ctrl Pts',(-1.70682212124656,0.319434907277167,
10.9919427781636));
#31274=CARTESIAN_POINT('Ctrl Pts',(-1.71574542397769,0.636309800095206,
11.0668346892391));
#31275=CARTESIAN_POINT('Ctrl Pts',(-1.72701657977795,0.79477268400084,11.1202076017071));
#31276=CARTESIAN_POINT('Ctrl Pts',(-1.76233903122006,1.06847604194511,11.2549094900764));
#31277=CARTESIAN_POINT('Ctrl Pts',(-1.78233798615881,1.18514270861178,11.3251184310253));
#31278=CARTESIAN_POINT('Ctrl Pts',(-1.80704611563284,1.3,11.407228856645));
#31279=CARTESIAN_POINT('Ctrl Pts',(-2.05661148970878,-1.3,11.2924694059607));
#31280=CARTESIAN_POINT('Ctrl Pts',(-2.00914338192998,-1.18514270861178,
11.2209304357418));
#31281=CARTESIAN_POINT('Ctrl Pts',(-1.96832072991242,-1.06847604194512,
11.1603953244878));
#31282=CARTESIAN_POINT('Ctrl Pts',(-1.88936456943561,-0.794772684000851,
11.0459682230072));
#31283=CARTESIAN_POINT('Ctrl Pts',(-1.85865359192219,-0.636309800095197,
11.0016155958775));
#31284=CARTESIAN_POINT('Ctrl Pts',(-1.8102831109525,-0.319434907277159,
10.9450989989837));
#31285=CARTESIAN_POINT('Ctrl Pts',(-1.79644754730034,-0.158333333333332,
10.9332833264162));
#31286=CARTESIAN_POINT('Ctrl Pts',(-1.77794490963747,0.158333333333334,
10.9421106139582));
#31287=CARTESIAN_POINT('Ctrl Pts',(-1.77431562872862,0.319434907277167,
10.9622827219367));
#31288=CARTESIAN_POINT('Ctrl Pts',(-1.78288365918825,0.636309800095206,
11.0377389598563));
#31289=CARTESIAN_POINT('Ctrl Pts',(-1.79358500771746,0.79477268400084,11.0915481264036));
#31290=CARTESIAN_POINT('Ctrl Pts',(-1.83046672246861,1.06847604194511,11.2259796900098));
#31291=CARTESIAN_POINT('Ctrl Pts',(-1.85162982048154,1.18514270861178,11.2958715822789));
#31292=CARTESIAN_POINT('Ctrl Pts',(-1.87799128879385,1.3,11.3774649241125));
#31293=CARTESIAN_POINT('Ctrl Pts',(-2.05661148970878,-1.3,11.2924694059607));
#31294=CARTESIAN_POINT('Ctrl Pts',(-2.00914338192998,-1.18514270861178,
11.2209304357418));
#31295=CARTESIAN_POINT('Ctrl Pts',(-1.96832072991242,-1.06847604194512,
11.1603953244878));
#31296=CARTESIAN_POINT('Ctrl Pts',(-1.88936456943561,-0.794772684000851,
11.0459682230072));
#31297=CARTESIAN_POINT('Ctrl Pts',(-1.85865359192219,-0.636309800095197,
11.0016155958775));
#31298=CARTESIAN_POINT('Ctrl Pts',(-1.8102831109525,-0.319434907277159,
10.9450989989837));
#31299=CARTESIAN_POINT('Ctrl Pts',(-1.79644754730034,-0.158333333333332,
10.9332833264162));
#31300=CARTESIAN_POINT('Ctrl Pts',(-1.77794490963747,0.158333333333334,
10.9421106139582));
#31301=CARTESIAN_POINT('Ctrl Pts',(-1.77431562872862,0.319434907277167,
10.9622827219367));
#31302=CARTESIAN_POINT('Ctrl Pts',(-1.78288365918825,0.636309800095206,
11.0377389598563));
#31303=CARTESIAN_POINT('Ctrl Pts',(-1.79358500771746,0.79477268400084,11.0915481264036));
#31304=CARTESIAN_POINT('Ctrl Pts',(-1.83046672246861,1.06847604194511,11.2259796900098));
#31305=CARTESIAN_POINT('Ctrl Pts',(-1.85162982048154,1.18514270861178,11.2958715822789));
#31306=CARTESIAN_POINT('Ctrl Pts',(-1.87799128879385,1.3,11.3774649241125));
#31307=CARTESIAN_POINT('Ctrl Pts',(-2.05661148970901,-1.30000000000056,
11.2924694059611));
#31308=CARTESIAN_POINT('Ctrl Pts',(-2.00914338193012,-1.18514270861216,
11.220930435742));
#31309=CARTESIAN_POINT('Ctrl Pts',(-1.96832072991248,-1.06847604194531,
11.1603953244879));
#31310=CARTESIAN_POINT('Ctrl Pts',(-1.88936456943561,-0.794772684000851,
11.0459682230072));
#31311=CARTESIAN_POINT('Ctrl Pts',(-1.85865359192219,-0.636309800095197,
11.0016155958775));
#31312=CARTESIAN_POINT('Ctrl Pts',(-1.8102831109525,-0.319434907277159,
10.9450989989837));
#31313=CARTESIAN_POINT('Ctrl Pts',(-1.79644754730034,-0.158333333333332,
10.9332833264162));
#31314=CARTESIAN_POINT('Ctrl Pts',(-1.77794490963747,0.158333333333334,
10.9421106139582));
#31315=CARTESIAN_POINT('Ctrl Pts',(-1.77431562872862,0.319434907277167,
10.9622827219367));
#31316=CARTESIAN_POINT('Ctrl Pts',(-1.78288365918825,0.636309800095206,
11.0377389598563));
#31317=CARTESIAN_POINT('Ctrl Pts',(-1.79358500771746,0.79477268400084,11.0915481264036));
#31318=CARTESIAN_POINT('Ctrl Pts',(-1.83046672246879,1.06847604194647,11.2259796900104));
#31319=CARTESIAN_POINT('Ctrl Pts',(-1.85162982048202,1.18514270861445,11.2958715822805));
#31320=CARTESIAN_POINT('Ctrl Pts',(-1.87799128879475,1.30000000000394,11.3774649241153));
#31321=CARTESIAN_POINT('Ctrl Pts',(-2.06438529509448,-1.30000000000056,
11.296489462555));
#31322=CARTESIAN_POINT('Ctrl Pts',(-2.01625666951673,-1.18514270861216,
11.2251351015232));
#31323=CARTESIAN_POINT('Ctrl Pts',(-1.9752779216005,-1.06847604194531,11.1644588769034));
#31324=CARTESIAN_POINT('Ctrl Pts',(-1.89712646386988,-0.794772684000851,
11.0489532910601));
#31325=CARTESIAN_POINT('Ctrl Pts',(-1.86923725412316,-0.636309800095197,
11.0022867513961));
#31326=CARTESIAN_POINT('Ctrl Pts',(-1.82221963516386,-0.319434907277159,
10.9446174246915));
#31327=CARTESIAN_POINT('Ctrl Pts',(-1.8080248988176,-0.158333333333332,
10.9332122432533));
#31328=CARTESIAN_POINT('Ctrl Pts',(-1.78936170982529,0.158333333333334,
10.9422136295658));
#31329=CARTESIAN_POINT('Ctrl Pts',(-1.78572104868508,0.319434907277167,
10.9623346432573));
#31330=CARTESIAN_POINT('Ctrl Pts',(-1.79303694376686,0.636309800095206,
11.0389207988169));
#31331=CARTESIAN_POINT('Ctrl Pts',(-1.80176883893061,0.79477268400084,11.0943744460198));
#31332=CARTESIAN_POINT('Ctrl Pts',(-1.83771824839734,1.06847604194647,11.2299700072586));
#31333=CARTESIAN_POINT('Ctrl Pts',(-1.85877864421393,1.18514270861445,11.3001911079339));
#31334=CARTESIAN_POINT('Ctrl Pts',(-1.88533826854578,1.30000000000394,11.3819390151346));
#31335=CARTESIAN_POINT('Ctrl Pts',(-2.07310405152111,-1.30000000000032,
11.3051109272569));
#31336=CARTESIAN_POINT('Ctrl Pts',(-2.02516512349642,-1.18514270861194,
11.236643173689));
#31337=CARTESIAN_POINT('Ctrl Pts',(-1.98482162956526,-1.06847604194511,
11.1776687388379));
#31338=CARTESIAN_POINT('Ctrl Pts',(-1.90916706011344,-0.794772684000704,
11.063357461904));
#31339=CARTESIAN_POINT('Ctrl Pts',(-1.8852824344217,-0.63630980009508,11.0128761490054));
#31340=CARTESIAN_POINT('Ctrl Pts',(-1.84046911413487,-0.319434907277101,
10.953375594764));
#31341=CARTESIAN_POINT('Ctrl Pts',(-1.82555504877143,-0.158333333333303,
10.941293868259));
#31342=CARTESIAN_POINT('Ctrl Pts',(-1.80675081476022,0.158333333333305,
10.9504201941717));
#31343=CARTESIAN_POINT('Ctrl Pts',(-1.80381989210835,0.319434907277107,
10.9713399291468));
#31344=CARTESIAN_POINT('Ctrl Pts',(-1.80837642663847,0.636309800095088,
11.0500174340263));
#31345=CARTESIAN_POINT('Ctrl Pts',(-1.81207156347144,0.794772684000696,
11.1095781698092));
#31346=CARTESIAN_POINT('Ctrl Pts',(-1.8455999431735,1.06847604194627,11.2439466892858));
#31347=CARTESIAN_POINT('Ctrl Pts',(-1.86632992438822,1.18514270861423,11.312362147158));
#31348=CARTESIAN_POINT('Ctrl Pts',(-1.89327669359346,1.3000000000037,11.3910299096651));
#31349=CARTESIAN_POINT('Ctrl Pts',(-2.08604767365955,-1.30000000000023,
11.317649477437));
#31350=CARTESIAN_POINT('Ctrl Pts',(-2.03990164826027,-1.18514270861186,
11.2523901800366));
#31351=CARTESIAN_POINT('Ctrl Pts',(-2.00105983312491,-1.06847604194503,
11.195674735722));
#31352=CARTESIAN_POINT('Ctrl Pts',(-1.92820165679573,-0.794772684000648,
11.0843887232898));
#31353=CARTESIAN_POINT('Ctrl Pts',(-1.90537128487983,-0.636309800095034,
11.0327047049662));
#31354=CARTESIAN_POINT('Ctrl Pts',(-1.86177167481144,-0.319434907277077,
10.9727023630987));
#31355=CARTESIAN_POINT('Ctrl Pts',(-1.84678457427543,-0.158333333333292,
10.9591640112912));
#31356=CARTESIAN_POINT('Ctrl Pts',(-1.82789737514345,0.158333333333294,
10.9683136305511));
#31357=CARTESIAN_POINT('Ctrl Pts',(-1.82524821498833,0.319434907277085,
10.990526740857));
#31358=CARTESIAN_POINT('Ctrl Pts',(-1.82782788881483,0.636309800095043,
11.0701334555425));
#31359=CARTESIAN_POINT('Ctrl Pts',(-1.82881842603555,0.794772684000638,
11.131860745249));
#31360=CARTESIAN_POINT('Ctrl Pts',(-1.85943132258683,1.06847604194619,11.2633328009558));
#31361=CARTESIAN_POINT('Ctrl Pts',(-1.87897774624833,1.18514270861414,11.3293439797425));
#31362=CARTESIAN_POINT('Ctrl Pts',(-1.9048194049738,1.30000000000361,11.4044569559198));
#31363=CARTESIAN_POINT('Ctrl Pts',(-2.09697218826236,-1.30000000000006,
11.3278871439688));
#31364=CARTESIAN_POINT('Ctrl Pts',(-2.05251089756756,-1.18514270861171,
11.2647969922648));
#31365=CARTESIAN_POINT('Ctrl Pts',(-2.0147696008548,-1.0684760419449,11.2097346947087));
#31366=CARTESIAN_POINT('Ctrl Pts',(-1.9431041857565,-0.794772684000548,
11.1010757212276));
#31367=CARTESIAN_POINT('Ctrl Pts',(-1.91854905377933,-0.636309800094954,
11.0497439167426));
#31368=CARTESIAN_POINT('Ctrl Pts',(-1.87508506278343,-0.319434907277038,
10.9896831140813));
#31369=CARTESIAN_POINT('Ctrl Pts',(-1.86111833437904,-0.158333333333272,
10.9744552860704));
#31370=CARTESIAN_POINT('Ctrl Pts',(-1.84266347705537,0.158333333333274,
10.9833318705429));
#31371=CARTESIAN_POINT('Ctrl Pts',(-1.84013583062199,0.319434907277045,
11.0065378896911));
#31372=CARTESIAN_POINT('Ctrl Pts',(-1.84201524437907,0.636309800094964,
11.0865096183245));
#31373=CARTESIAN_POINT('Ctrl Pts',(-1.84208408340377,0.794772684000538,
11.149410442407));
#31374=CARTESIAN_POINT('Ctrl Pts',(-1.87112130174078,1.06847604194606,11.2785244138799));
#31375=CARTESIAN_POINT('Ctrl Pts',(-1.88988682069309,1.185142708614,11.3427315325958));
#31376=CARTESIAN_POINT('Ctrl Pts',(-1.91484872271451,1.30000000000345,11.4152571159209));
#31377=CARTESIAN_POINT('Ctrl Pts',(-2.10826479557406,-1.29999999999992,
11.3380338755581));
#31378=CARTESIAN_POINT('Ctrl Pts',(-2.0656602099202,-1.18514270861158,11.2773274665579));
#31379=CARTESIAN_POINT('Ctrl Pts',(-2.02912223104839,-1.06847604194478,
11.2241061455424));
#31380=CARTESIAN_POINT('Ctrl Pts',(-1.95872726574397,-0.794772684000462,
11.1184462977394));
#31381=CARTESIAN_POINT('Ctrl Pts',(-1.93243426015739,-0.636309800094885,
11.0675486006443));
#31382=CARTESIAN_POINT('Ctrl Pts',(-1.8886049936113,-0.319434907277003,
11.007826746438));
#31383=CARTESIAN_POINT('Ctrl Pts',(-1.87523037933012,-0.158333333333255,
10.9910809152724));
#31384=CARTESIAN_POINT('Ctrl Pts',(-1.8560745914034,0.158333333333257,11.0003296924322));
#31385=CARTESIAN_POINT('Ctrl Pts',(-1.85186465050229,0.319434907277009,
11.0256213410938));
#31386=CARTESIAN_POINT('Ctrl Pts',(-1.85347446833627,0.636309800094893,
11.1056141666609));
#31387=CARTESIAN_POINT('Ctrl Pts',(-1.85565912734136,0.794772684000451,
11.1679143238887));
#31388=CARTESIAN_POINT('Ctrl Pts',(-1.88383366212453,1.06847604194594,11.2938576588064));
#31389=CARTESIAN_POINT('Ctrl Pts',(-1.9016515493598,1.18514270861387,11.3561085364947));
#31390=CARTESIAN_POINT('Ctrl Pts',(-1.92509161169201,1.30000000000331,11.4260940888454));
#31391=CARTESIAN_POINT('Ctrl Pts',(-2.11798686606854,-1.29999999999981,
11.3455803565388));
#31392=CARTESIAN_POINT('Ctrl Pts',(-2.07682357731144,-1.18514270861148,
11.2866450754959));
#31393=CARTESIAN_POINT('Ctrl Pts',(-2.0411712851994,-1.0684760419447,11.2348234956709));
#31394=CARTESIAN_POINT('Ctrl Pts',(-1.97153886292524,-0.794772684000398,
11.1315393523081));
#31395=CARTESIAN_POINT('Ctrl Pts',(-1.94378698956596,-0.636309800094834,
11.0810582859973));
#31396=CARTESIAN_POINT('Ctrl Pts',(-1.89890182412223,-0.319434907276977,
11.0220543656774));
#31397=CARTESIAN_POINT('Ctrl Pts',(-1.88475293497587,-0.158333333333242,
11.0048933339137));
#31398=CARTESIAN_POINT('Ctrl Pts',(-1.86498170941202,0.158333333333244,
11.014460822773));
#31399=CARTESIAN_POINT('Ctrl Pts',(-1.8605942188333,0.319434907276985,11.0406385430365));
#31400=CARTESIAN_POINT('Ctrl Pts',(-1.86269152931723,0.636309800094844,
11.1202526899541));
#31401=CARTESIAN_POINT('Ctrl Pts',(-1.86684619478339,0.794772684000388,
11.1819377459642));
#31402=CARTESIAN_POINT('Ctrl Pts',(-1.89424975777036,1.06847604194586,11.3055989377497));
#31403=CARTESIAN_POINT('Ctrl Pts',(-1.9111333875259,1.18514270861377,11.3665161841555));
#31404=CARTESIAN_POINT('Ctrl Pts',(-1.93303866002193,1.3000000000032,11.4348223291416));
#31405=CARTESIAN_POINT('Ctrl Pts',(-2.12751552334184,-1.29999999999973,
11.3533054250362));
#31406=CARTESIAN_POINT('Ctrl Pts',(-2.08768657842924,-1.1851427086114,11.2962931641647));
#31407=CARTESIAN_POINT('Ctrl Pts',(-2.05287338555443,-1.06847604194463,
11.2459610975741));
#31408=CARTESIAN_POINT('Ctrl Pts',(-1.98403533626337,-0.794772684000345,
11.145116540012));
#31409=CARTESIAN_POINT('Ctrl Pts',(-1.9550943424084,-0.636309800094793,
11.0948592576465));
#31410=CARTESIAN_POINT('Ctrl Pts',(-1.9093049904265,-0.319434907276957,
11.0364660055729));
#31411=CARTESIAN_POINT('Ctrl Pts',(-1.89412945682592,-0.158333333333232,
11.0189783706396));
#31412=CARTESIAN_POINT('Ctrl Pts',(-1.87429743956021,0.158333333333234,
11.0285649155269));
#31413=CARTESIAN_POINT('Ctrl Pts',(-1.87105358272484,0.319434907276963,
11.0549689599644));
#31414=CARTESIAN_POINT('Ctrl Pts',(-1.87356912434942,0.636309800094801,
11.1342543312433));
#31415=CARTESIAN_POINT('Ctrl Pts',(-1.87794784535936,0.794772684000338,
11.1962927526475));
#31416=CARTESIAN_POINT('Ctrl Pts',(-1.90437513697839,1.06847604194579,11.317681492603));
#31417=CARTESIAN_POINT('Ctrl Pts',(-1.92053629934561,1.18514270861369,11.3770784479341));
#31418=CARTESIAN_POINT('Ctrl Pts',(-1.94141922876575,1.30000000000312,11.4433276709655));
#31419=CARTESIAN_POINT('Ctrl Pts',(-2.14304910682474,-1.29999999999967,
11.3675618927398));
#31420=CARTESIAN_POINT('Ctrl Pts',(-2.10599876682301,-1.18514270861135,
11.3135495276944));
#31421=CARTESIAN_POINT('Ctrl Pts',(-2.07304532033494,-1.06847604194458,
11.2655198289767));
#31422=CARTESIAN_POINT('Ctrl Pts',(-2.00638091023047,-0.794772684000311,
11.1683827726755));
#31423=CARTESIAN_POINT('Ctrl Pts',(-1.97576844951589,-0.636309800094764,
11.1183053583916));
#31424=CARTESIAN_POINT('Ctrl Pts',(-1.92881021894933,-0.319434907276942,
11.0607632253031));
#31425=CARTESIAN_POINT('Ctrl Pts',(-1.91226173434354,-0.158333333333225,
11.0425358743185));
#31426=CARTESIAN_POINT('Ctrl Pts',(-1.89148266149804,0.158333333333227,
11.0526393852624));
#31427=CARTESIAN_POINT('Ctrl Pts',(-1.88795508883333,0.319434907276951,
11.0806812541267));
#31428=CARTESIAN_POINT('Ctrl Pts',(-1.89115585204907,0.636309800094775,
11.1593921695946));
#31429=CARTESIAN_POINT('Ctrl Pts',(-1.89858527717453,0.794772684000302,
11.220508860524));
#31430=CARTESIAN_POINT('Ctrl Pts',(-1.92357473296657,1.06847604194574,11.3378270584154));
#31431=CARTESIAN_POINT('Ctrl Pts',(-1.93813670352488,1.18514270861364,11.3948012445658));
#31432=CARTESIAN_POINT('Ctrl Pts',(-1.95644363517964,1.30000000000306,11.4579669160667));
#31433=CARTESIAN_POINT('Ctrl Pts',(-2.16816701100096,-1.29999999999847,
11.3858847423421));
#31434=CARTESIAN_POINT('Ctrl Pts',(-2.13557075152151,-1.18514270861026,
11.3358096331527));
#31435=CARTESIAN_POINT('Ctrl Pts',(-2.10540159865792,-1.06847604194359,
11.2909739036088));
#31436=CARTESIAN_POINT('Ctrl Pts',(-2.04131192204839,-0.794772683999578,
11.1994984141206));
#31437=CARTESIAN_POINT('Ctrl Pts',(-2.00650415050177,-0.636309800094176,
11.1509629672446));
#31438=CARTESIAN_POINT('Ctrl Pts',(-1.95663189844875,-0.319434907276646,
11.0954873096538));
#31439=CARTESIAN_POINT('Ctrl Pts',(-1.93721841919561,-0.158333333333079,
11.0767127352415));
#31440=CARTESIAN_POINT('Ctrl Pts',(-1.91601584542966,0.158333333333081,
11.0870415141348));
#31441=CARTESIAN_POINT('Ctrl Pts',(-1.91530622987097,0.319434907276658,
11.1155647611286));
#31442=CARTESIAN_POINT('Ctrl Pts',(-1.91979154489423,0.636309800094188,
11.1932610324165));
#31443=CARTESIAN_POINT('Ctrl Pts',(-1.92870254854972,0.794772683999565,
11.2546762338425));
#31444=CARTESIAN_POINT('Ctrl Pts',(-1.95083582044778,1.06847604194475,11.3666316540899));
#31445=CARTESIAN_POINT('Ctrl Pts',(-1.96311770202887,1.18514270861255,11.4201456583241));
#31446=CARTESIAN_POINT('Ctrl Pts',(-1.97810079190486,1.30000000000186,11.4787123137243));
#31447=CARTESIAN_POINT('Ctrl Pts',(-2.19197084033917,-1.29999999999816,
11.405075726293));
#31448=CARTESIAN_POINT('Ctrl Pts',(-2.16287598261759,-1.18514270860997,
11.3596211368751));
#31449=CARTESIAN_POINT('Ctrl Pts',(-2.13519097617397,-1.06847604194334,
11.3182138002111));
#31450=CARTESIAN_POINT('Ctrl Pts',(-2.07449011141456,-0.794772683999387,
11.2319045325197));
#31451=CARTESIAN_POINT('Ctrl Pts',(-2.03887330153802,-0.636309800094021,
11.1826114252657));
#31452=CARTESIAN_POINT('Ctrl Pts',(-1.98785020262338,-0.319434907276568,
11.1280752760641));
#31453=CARTESIAN_POINT('Ctrl Pts',(-1.96567353851661,-0.15833333333304,
11.1087999397335));
#31454=CARTESIAN_POINT('Ctrl Pts',(-1.943487830973,0.158333333333042,11.119713787425));
#31455=CARTESIAN_POINT('Ctrl Pts',(-1.94395647822165,0.31943490727658,11.1496725896324));
#31456=CARTESIAN_POINT('Ctrl Pts',(-1.94881586676246,0.636309800094034,
11.2269087319269));
#31457=CARTESIAN_POINT('Ctrl Pts',(-1.95970581148777,0.794772683999372,
11.2883587248095));
#31458=CARTESIAN_POINT('Ctrl Pts',(-1.97841572141238,1.06847604194449,11.3952940028233));
#31459=CARTESIAN_POINT('Ctrl Pts',(-1.98804050414247,1.18514270861226,11.445568000792));
#31460=CARTESIAN_POINT('Ctrl Pts',(-1.99919124286672,1.30000000000154,11.4998276772196));
#31461=CARTESIAN_POINT('Ctrl Pts',(-2.21194072996136,-1.29999999999782,
11.4197523880558));
#31462=CARTESIAN_POINT('Ctrl Pts',(-2.18705625067301,-1.18514270860966,
11.3769694924721));
#31463=CARTESIAN_POINT('Ctrl Pts',(-2.16217394850673,-1.06847604194305,
11.3377137699941));
#31464=CARTESIAN_POINT('Ctrl Pts',(-2.10469588240273,-0.794772683999173,
11.2551736734718));
#31465=CARTESIAN_POINT('Ctrl Pts',(-2.06636629065357,-0.636309800093855,
11.206781684638));
#31466=CARTESIAN_POINT('Ctrl Pts',(-2.01361252053818,-0.319434907276486,
11.1536123775203));
#31467=CARTESIAN_POINT('Ctrl Pts',(-1.98927994229085,-0.158333333332999,
11.1339191974918));
#31468=CARTESIAN_POINT('Ctrl Pts',(-1.96637611505289,0.158333333333001,
11.1452890494184));
#31469=CARTESIAN_POINT('Ctrl Pts',(-1.96811104626271,0.319434907276498,
11.1761945853261));
#31470=CARTESIAN_POINT('Ctrl Pts',(-1.97358770240202,0.636309800093869,
11.2528442702706));
#31471=CARTESIAN_POINT('Ctrl Pts',(-1.98631080264597,0.794772683999164,
11.3141127511188));
#31472=CARTESIAN_POINT('Ctrl Pts',(-2.00232560278451,1.06847604194421,11.416996424493));
#31473=CARTESIAN_POINT('Ctrl Pts',(-2.00977318852491,1.18514270861195,11.4647174726693));
#31474=CARTESIAN_POINT('Ctrl Pts',(-2.01773614643252,1.30000000000121,11.5156250390336));
#31475=CARTESIAN_POINT('Ctrl Pts',(-2.22718477672543,-1.29999999999765,
11.4305479831051));
#31476=CARTESIAN_POINT('Ctrl Pts',(-2.20446821519554,-1.18514270860951,
11.3904908738317));
#31477=CARTESIAN_POINT('Ctrl Pts',(-2.1810698502756,-1.06847604194292,11.3532988193024));
#31478=CARTESIAN_POINT('Ctrl Pts',(-2.12543984425841,-0.794772683999076,
11.2739965827059));
#31479=CARTESIAN_POINT('Ctrl Pts',(-2.08596510327014,-0.636309800093774,
11.2256122840007));
#31480=CARTESIAN_POINT('Ctrl Pts',(-2.03265922940549,-0.319434907276445,
11.1729441026475));
#31481=CARTESIAN_POINT('Ctrl Pts',(-2.00747278411166,-0.158333333332979,
11.1524323973261));
#31482=CARTESIAN_POINT('Ctrl Pts',(-1.98432743759838,0.158333333332981,
11.1639424191239));
#31483=CARTESIAN_POINT('Ctrl Pts',(-1.98680023512611,0.319434907276456,
11.1957039870647));
#31484=CARTESIAN_POINT('Ctrl Pts',(-1.99208136539881,0.636309800093787,
11.2723471795851));
#31485=CARTESIAN_POINT('Ctrl Pts',(-2.0050069749984,0.794772683999063,11.334249214994));
#31486=CARTESIAN_POINT('Ctrl Pts',(-2.01877976488453,1.06847604194408,11.4342362373978));
#31487=CARTESIAN_POINT('Ctrl Pts',(-2.0247430628523,1.1851427086118,11.4799430554902));
#31488=CARTESIAN_POINT('Ctrl Pts',(-2.03070792837825,1.30000000000104,11.5280760145603));
#31489=CARTESIAN_POINT('Ctrl Pts',(-2.24236803062261,-1.29999999999691,
11.4413662490845));
#31490=CARTESIAN_POINT('Ctrl Pts',(-2.22272970222264,-1.18514270860883,
11.4033485923955));
#31491=CARTESIAN_POINT('Ctrl Pts',(-2.20143912424778,-1.0684760419423,11.3677553119689));
#31492=CARTESIAN_POINT('Ctrl Pts',(-2.14843660291098,-0.794772683998616,
11.2911285079329));
#31493=CARTESIAN_POINT('Ctrl Pts',(-2.10748850912162,-0.636309800093407,
11.2430534145239));
#31494=CARTESIAN_POINT('Ctrl Pts',(-2.05311394288683,-0.31943490727626,
11.1912810537758));
#31495=CARTESIAN_POINT('Ctrl Pts',(-2.02616691220347,-0.158333333332887,
11.1705871219805));
#31496=CARTESIAN_POINT('Ctrl Pts',(-2.00238897095407,0.158333333332889,
11.1825197442794));
#31497=CARTESIAN_POINT('Ctrl Pts',(-2.00562061474378,0.319434907276271,
11.2151111091204));
#31498=CARTESIAN_POINT('Ctrl Pts',(-2.01143380800353,0.636309800093419,
11.2912610402889));
#31499=CARTESIAN_POINT('Ctrl Pts',(-2.02628200316612,0.794772683998605,
11.3526445276488));
#31500=CARTESIAN_POINT('Ctrl Pts',(-2.03777139291857,1.06847604194346,11.4497683742301));
#31501=CARTESIAN_POINT('Ctrl Pts',(-2.04181744495932,1.18514270861111,11.4937546572526));
#31502=CARTESIAN_POINT('Ctrl Pts',(-2.04493621794082,1.30000000000029,11.5396859089054));
#31503=CARTESIAN_POINT('Ctrl Pts',(-2.26249397180303,-1.29999999999639,
11.455874478958));
#31504=CARTESIAN_POINT('Ctrl Pts',(-2.24629708411541,-1.18514270860836,
11.421080626451));
#31505=CARTESIAN_POINT('Ctrl Pts',(-2.22739100720034,-1.06847604194188,
11.3879398428267));
#31506=CARTESIAN_POINT('Ctrl Pts',(-2.17745541829201,-0.794772683998302,
11.3151969226777));
#31507=CARTESIAN_POINT('Ctrl Pts',(-2.13502915182882,-0.636309800093156,
11.2671282925831));
#31508=CARTESIAN_POINT('Ctrl Pts',(-2.07969952072822,-0.319434907276135,
11.2161943144671));
#31509=CARTESIAN_POINT('Ctrl Pts',(-2.05070326474499,-0.158333333332825,
11.195046095051));
#31510=CARTESIAN_POINT('Ctrl Pts',(-2.02685371396135,0.158333333332827,
11.2070121729432));
#31511=CARTESIAN_POINT('Ctrl Pts',(-2.03237832409365,0.319434907276143,
11.239855936348));
#31512=CARTESIAN_POINT('Ctrl Pts',(-2.03835837233474,0.636309800093167,
11.3157150116269));
#31513=CARTESIAN_POINT('Ctrl Pts',(-2.05308349031875,0.794772683998294,
11.3782157436242));
#31514=CARTESIAN_POINT('Ctrl Pts',(-2.06112074423417,1.06847604194304,11.4717958121859));
#31515=CARTESIAN_POINT('Ctrl Pts',(-2.06291955728834,1.18514270861065,11.5132794028105));
#31516=CARTESIAN_POINT('Ctrl Pts',(-2.06303815398629,1.29999999999977,11.5557392398623));
#31517=CARTESIAN_POINT('Ctrl Pts',(-2.28098123996243,-1.29999999999548,
11.467871279756));
#31518=CARTESIAN_POINT('Ctrl Pts',(-2.26855348098431,-1.18514270860753,
11.4352971885243));
#31519=CARTESIAN_POINT('Ctrl Pts',(-2.25218384250273,-1.06847604194113,
11.4039495664119));
#31520=CARTESIAN_POINT('Ctrl Pts',(-2.20526017265208,-0.794772683997745,
11.3343636772815));
#31521=CARTESIAN_POINT('Ctrl Pts',(-2.16046735275002,-0.636309800092709,
11.2871715906424));
#31522=CARTESIAN_POINT('Ctrl Pts',(-2.10402724865593,-0.31943490727591,
11.2372344617707));
#31523=CARTESIAN_POINT('Ctrl Pts',(-2.07383776819597,-0.158333333332714,
11.2152981632221));
#31524=CARTESIAN_POINT('Ctrl Pts',(-2.04931561047445,0.158333333332716,
11.2277249232403));
#31525=CARTESIAN_POINT('Ctrl Pts',(-2.05506359872789,0.319434907275921,
11.26198334941));
#31526=CARTESIAN_POINT('Ctrl Pts',(-2.06138952335123,0.636309800092722,
11.3374460223415));
#31527=CARTESIAN_POINT('Ctrl Pts',(-2.07859263583547,0.794772683997734,
11.3991632269327));
#31528=CARTESIAN_POINT('Ctrl Pts',(-2.08373944708755,1.06847604194229,11.4895565975992));
#31529=CARTESIAN_POINT('Ctrl Pts',(-2.08313510061906,1.18514270860981,11.5291502348457));
#31530=CARTESIAN_POINT('Ctrl Pts',(-2.0796985437992,1.29999999999886,11.5692095685813));
#31531=CARTESIAN_POINT('Ctrl Pts',(-2.30191461963453,-1.29999999999489,
11.4817207869872));
#31532=CARTESIAN_POINT('Ctrl Pts',(-2.29295315639335,-1.185142708607,11.4523286421187));
#31533=CARTESIAN_POINT('Ctrl Pts',(-2.27910133602921,-1.06847604194065,
11.4233230213229));
#31534=CARTESIAN_POINT('Ctrl Pts',(-2.23580315667427,-0.794772683997392,
11.3572071826614));
#31535=CARTESIAN_POINT('Ctrl Pts',(-2.1907397046039,-0.636309800092424,
11.3091659470523));
#31536=CARTESIAN_POINT('Ctrl Pts',(-2.13331425086397,-0.319434907275766,
11.2601315080099));
#31537=CARTESIAN_POINT('Ctrl Pts',(-2.0999167008132,-0.158333333332642,
11.2386390748403));
#31538=CARTESIAN_POINT('Ctrl Pts',(-2.07468843330633,0.158333333332644,
11.251579126617));
#31539=CARTESIAN_POINT('Ctrl Pts',(-2.08264523630014,0.319434907275776,
11.2861132674822));
#31540=CARTESIAN_POINT('Ctrl Pts',(-2.08911533116864,0.636309800092434,
11.361298594492));
#31541=CARTESIAN_POINT('Ctrl Pts',(-2.10662134947467,0.794772683997376,
11.4238415251322));
#31542=CARTESIAN_POINT('Ctrl Pts',(-2.10824296875268,1.06847604194181,11.5107554791366));
#31543=CARTESIAN_POINT('Ctrl Pts',(-2.10526319437188,1.18514270860928,11.5479437308975));
#31544=CARTESIAN_POINT('Ctrl Pts',(-2.09860170671175,1.29999999999828,11.5846984042097));
#31545=CARTESIAN_POINT('Ctrl Pts',(-2.31440322914962,-1.29999999999441,
11.4907955972478));
#31546=CARTESIAN_POINT('Ctrl Pts',(-2.30831860217203,-1.18514270860656,
11.4628406234383));
#31547=CARTESIAN_POINT('Ctrl Pts',(-2.29642039607987,-1.06847604194026,
11.4350037608307));
#31548=CARTESIAN_POINT('Ctrl Pts',(-2.25550262902185,-0.794772683997096,
11.3709678999663));
#31549=CARTESIAN_POINT('Ctrl Pts',(-2.2086285196071,-0.63630980009219,11.3236523178589));
#31550=CARTESIAN_POINT('Ctrl Pts',(-2.15072419116017,-0.31943490727565,
11.2751115673957));
#31551=CARTESIAN_POINT('Ctrl Pts',(-2.116801471756,-0.158333333332584,11.2528240808836));
#31552=CARTESIAN_POINT('Ctrl Pts',(-2.09163308515834,0.158333333332586,
11.2657146730607));
#31553=CARTESIAN_POINT('Ctrl Pts',(-2.10047576784667,0.319434907275659,
11.3007542090159));
#31554=CARTESIAN_POINT('Ctrl Pts',(-2.10693394263024,0.636309800092201,
11.3758343691641));
#31555=CARTESIAN_POINT('Ctrl Pts',(-2.1247727595787,0.794772683997086,11.4388074749674));
#31556=CARTESIAN_POINT('Ctrl Pts',(-2.1240277074958,1.06847604194142,11.5236670809836));
#31557=CARTESIAN_POINT('Ctrl Pts',(-2.11943877826403,1.18514270860885,11.559440470131));
#31558=CARTESIAN_POINT('Ctrl Pts',(-2.11058342524029,1.2999999999978,11.5942546693395));
#31559=CARTESIAN_POINT('Ctrl Pts',(-2.33381671126052,-1.29999999999402,
11.5020369773312));
#31560=CARTESIAN_POINT('Ctrl Pts',(-2.33105482008487,-1.1851427086062,11.4766190968446));
#31561=CARTESIAN_POINT('Ctrl Pts',(-2.32150725055883,-1.06847604193994,
11.4507037635032));
#31562=CARTESIAN_POINT('Ctrl Pts',(-2.28377418050927,-0.794772683996859,
11.3896849435304));
#31563=CARTESIAN_POINT('Ctrl Pts',(-2.23600821794575,-0.636309800091998,
11.3421513828582));
#31564=CARTESIAN_POINT('Ctrl Pts',(-2.17711773843962,-0.319434907275552,
11.2945339994663));
#31565=CARTESIAN_POINT('Ctrl Pts',(-2.14099785861747,-0.158333333332536,
11.2722295838866));
#31566=CARTESIAN_POINT('Ctrl Pts',(-2.11471897948203,0.158333333332538,
11.2859386798493));
#31567=CARTESIAN_POINT('Ctrl Pts',(-2.12390517567732,0.319434907275562,
11.3223368294361));
#31568=CARTESIAN_POINT('Ctrl Pts',(-2.1306012601282,0.636309800092009,11.3970951742147));
#31569=CARTESIAN_POINT('Ctrl Pts',(-2.1508023531816,0.794772683996845,11.4593010662695));
#31570=CARTESIAN_POINT('Ctrl Pts',(-2.14716342126206,1.06847604194109,11.5409850223026));
#31571=CARTESIAN_POINT('Ctrl Pts',(-2.1402022302872,1.18514270860849,11.5748651329399));
#31572=CARTESIAN_POINT('Ctrl Pts',(-2.12785500712976,1.29999999999741,11.6072673963366));
#31573=CARTESIAN_POINT('Ctrl Pts',(-2.34670163233748,-1.29999999999275,
11.5107831115056));
#31574=CARTESIAN_POINT('Ctrl Pts',(-2.34671932800519,-1.18514270860504,
11.4868594265423));
#31575=CARTESIAN_POINT('Ctrl Pts',(-2.33907711788905,-1.06847604193889,
11.4621393907479));
#31576=CARTESIAN_POINT('Ctrl Pts',(-2.30372616898224,-0.794772683996075,
11.4031914331071));
#31577=CARTESIAN_POINT('Ctrl Pts',(-2.2542761703362,-0.636309800091375,
11.3563055316114));
#31578=CARTESIAN_POINT('Ctrl Pts',(-2.19515753628339,-0.319434907275241,
11.3090063394001));
#31579=CARTESIAN_POINT('Ctrl Pts',(-2.15873250633772,-0.158333333332381,
11.2857474611326));
#31580=CARTESIAN_POINT('Ctrl Pts',(-2.13280330580729,0.158333333332383,
11.2992036186574));
#31581=CARTESIAN_POINT('Ctrl Pts',(-2.14320558663257,0.319434907275247,
11.3358763363246));
#31582=CARTESIAN_POINT('Ctrl Pts',(-2.14969885791129,0.636309800091384,
11.4106709515121));
#31583=CARTESIAN_POINT('Ctrl Pts',(-2.16955001086733,0.794772683996067,
11.4737915836462));
#31584=CARTESIAN_POINT('Ctrl Pts',(-2.16314946430749,1.06847604194005,11.5537144851381));
#31585=CARTESIAN_POINT('Ctrl Pts',(-2.15447261846925,1.18514270860733,11.5862632140747));
#31586=CARTESIAN_POINT('Ctrl Pts',(-2.13988948623493,1.29999999999614,11.6167650093272));
#31587=CARTESIAN_POINT('Ctrl Pts',(-2.35856865684174,-1.29999999999248,
11.5184481151003));
#31588=CARTESIAN_POINT('Ctrl Pts',(-2.36094102694564,-1.1851427086048,11.4959831014653));
#31589=CARTESIAN_POINT('Ctrl Pts',(-2.35498789299465,-1.06847604193867,
11.4723582444834));
#31590=CARTESIAN_POINT('Ctrl Pts',(-2.32200138276934,-0.794772683995912,
11.4151006285611));
#31591=CARTESIAN_POINT('Ctrl Pts',(-2.27204948957197,-0.636309800091243,
11.3680128505829));
#31592=CARTESIAN_POINT('Ctrl Pts',(-2.21245168235206,-0.319434907275175,
11.3211993476087));
#31593=CARTESIAN_POINT('Ctrl Pts',(-2.17457512814538,-0.158333333332349,
11.297980516356));
#31594=CARTESIAN_POINT('Ctrl Pts',(-2.14813980789209,0.158333333332351,
11.3118224764547));
#31595=CARTESIAN_POINT('Ctrl Pts',(-2.15921124599767,0.319434907275182,
11.3490400011529));
#31596=CARTESIAN_POINT('Ctrl Pts',(-2.16571545678366,0.636309800091253,
11.4237293256518));
#31597=CARTESIAN_POINT('Ctrl Pts',(-2.18633433888062,0.794772683995904,
11.4868936219414));
#31598=CARTESIAN_POINT('Ctrl Pts',(-2.17783123474526,1.06847604193983,11.5649559143081));
#31599=CARTESIAN_POINT('Ctrl Pts',(-2.16763101665763,1.18514270860708,11.5962913793229));
#31600=CARTESIAN_POINT('Ctrl Pts',(-2.15091125919154,1.29999999999587,11.6251720354797));
#31601=CARTESIAN_POINT('Ctrl Pts',(-2.36390892297408,-1.2999999999924,11.5218051266847));
#31602=CARTESIAN_POINT('Ctrl Pts',(-2.36718189067206,-1.18514270860472,
11.5001007762633));
#31603=CARTESIAN_POINT('Ctrl Pts',(-2.36189429107058,-1.0684760419386,11.4770278263546));
#31604=CARTESIAN_POINT('Ctrl Pts',(-2.32990225521314,-0.79477268399586,
11.4205629577346));
#31605=CARTESIAN_POINT('Ctrl Pts',(-2.27992579179333,-0.636309800091202,
11.3732277329024));
#31606=CARTESIAN_POINT('Ctrl Pts',(-2.22021411103163,-0.319434907275154,
11.3265548252099));
#31607=CARTESIAN_POINT('Ctrl Pts',(-2.18172997762361,-0.158333333332338,
11.3033313636279));
#31608=CARTESIAN_POINT('Ctrl Pts',(-2.15506715175217,0.15833333333234,11.3173489222133));
#31609=CARTESIAN_POINT('Ctrl Pts',(-2.16635844001899,0.319434907275161,
11.3548663899172));
#31610=CARTESIAN_POINT('Ctrl Pts',(-2.17283947535757,0.636309800091211,
11.4295289514237));
#31611=CARTESIAN_POINT('Ctrl Pts',(-2.19382952706387,0.794772683995851,
11.4926875929646));
#31612=CARTESIAN_POINT('Ctrl Pts',(-2.18438606802361,1.06847604193976,11.5699268815541));
#31613=CARTESIAN_POINT('Ctrl Pts',(-2.17350190663026,1.18514270860701,11.6007285733569));
#31614=CARTESIAN_POINT('Ctrl Pts',(-2.15582130734746,1.29999999999578,11.6288979309297));
#31615=CARTESIAN_POINT('Ctrl Pts',(-2.3720492133645,-1.29999999999228,11.5267330346446));
#31616=CARTESIAN_POINT('Ctrl Pts',(-2.37680608844054,-1.18514270860461,
11.506060968131));
#31617=CARTESIAN_POINT('Ctrl Pts',(-2.37258429148656,-1.0684760419385,11.4837606717457));
#31618=CARTESIAN_POINT('Ctrl Pts',(-2.34208856738875,-0.794772683995788,
11.4284809892067));
#31619=CARTESIAN_POINT('Ctrl Pts',(-2.29179513196189,-0.636309800091144,
11.3810034797012));
#31620=CARTESIAN_POINT('Ctrl Pts',(-2.23181042817592,-0.319434907275125,
11.334624340559));
#31621=CARTESIAN_POINT('Ctrl Pts',(-2.19245200547176,-0.158333333332324,
11.3113608196081));
#31622=CARTESIAN_POINT('Ctrl Pts',(-2.16549565963411,0.158333333332326,
11.3256061047224));
#31623=CARTESIAN_POINT('Ctrl Pts',(-2.17720846473121,0.319434907275132,
11.3635064325329));
#31624=CARTESIAN_POINT('Ctrl Pts',(-2.18368902993222,0.636309800091154,
11.4381046901535));
#31625=CARTESIAN_POINT('Ctrl Pts',(-2.20520539861963,0.794772683995779,
11.5012787044382));
#31626=CARTESIAN_POINT('Ctrl Pts',(-2.19431129208499,1.06847604193966,11.577314022173));
#31627=CARTESIAN_POINT('Ctrl Pts',(-2.18237753636617,1.1851427086069,11.6073327529529));
#31628=CARTESIAN_POINT('Ctrl Pts',(-2.16322567998097,1.29999999999566,11.6344573428514));
#31629=CARTESIAN_POINT('Ctrl Pts',(-2.38026004860352,-1.29999999999144,
11.5315931029377));
#31630=CARTESIAN_POINT('Ctrl Pts',(-2.38672599277927,-1.18514270860384,
11.5117718614968));
#31631=CARTESIAN_POINT('Ctrl Pts',(-2.38368986891399,-1.06847604193781,
11.4901473215834));
#31632=CARTESIAN_POINT('Ctrl Pts',(-2.35472413735369,-0.794772683995274,
11.4360243281893));
#31633=CARTESIAN_POINT('Ctrl Pts',(-2.30368643572867,-0.636309800090732,
11.3887457787763));
#31634=CARTESIAN_POINT('Ctrl Pts',(-2.24327796333425,-0.319434907274918,
11.3427820318431));
#31635=CARTESIAN_POINT('Ctrl Pts',(-2.20303598723206,-0.158333333332221,
11.3194833619449));
#31636=CARTESIAN_POINT('Ctrl Pts',(-2.17598241412595,0.158333333332223,
11.3338110397047));
#31637=CARTESIAN_POINT('Ctrl Pts',(-2.1885018056849,0.319434907274926,11.3718066355807));
#31638=CARTESIAN_POINT('Ctrl Pts',(-2.19516682571112,0.636309800090742,
11.4462026984505));
#31639=CARTESIAN_POINT('Ctrl Pts',(-2.21716370777384,0.794772683995265,
11.509424941382));
#31640=CARTESIAN_POINT('Ctrl Pts',(-2.20465981764346,1.06847604193897,11.5843771335585));
#31641=CARTESIAN_POINT('Ctrl Pts',(-2.19156314759851,1.18514270860613,11.6136990798478));
#31642=CARTESIAN_POINT('Ctrl Pts',(-2.17078227823132,1.29999999999482,11.6398989456853));
#31643=CARTESIAN_POINT('Ctrl Pts',(-2.38838367499918,-1.29999999999133,
11.5365218435371));
#31644=CARTESIAN_POINT('Ctrl Pts',(-2.39641057934158,-1.18514270860375,
11.5176700758882));
#31645=CARTESIAN_POINT('Ctrl Pts',(-2.39448761826522,-1.06847604193772,
11.4967791690672));
#31646=CARTESIAN_POINT('Ctrl Pts',(-2.36705901391067,-0.794772683995211,
11.4438061756833));
#31647=CARTESIAN_POINT('Ctrl Pts',(-2.31563436231257,-0.636309800090681,
11.3964383534719));
#31648=CARTESIAN_POINT('Ctrl Pts',(-2.25488089277633,-0.319434907274892,
11.3508265038955));
#31649=CARTESIAN_POINT('Ctrl Pts',(-2.21361664280147,-0.158333333332209,
11.3276071052436));
#31650=CARTESIAN_POINT('Ctrl Pts',(-2.18637498304349,0.158333333332211,
11.342086594996));
#31651=CARTESIAN_POINT('Ctrl Pts',(-2.1996222621025,0.3194349072749,11.3802319045307));
#31652=CARTESIAN_POINT('Ctrl Pts',(-2.20646568518064,0.636309800090691,
11.4544281044756));
#31653=CARTESIAN_POINT('Ctrl Pts',(-2.22903619480044,0.794772683995201,
11.5176279418966));
#31654=CARTESIAN_POINT('Ctrl Pts',(-2.21497154076344,1.06847604193888,11.5914610534171));
#31655=CARTESIAN_POINT('Ctrl Pts',(-2.20072648927202,1.18514270860604,11.6200762175823));
#31656=CARTESIAN_POINT('Ctrl Pts',(-2.17832445387503,1.29999999999472,11.6453469277217));
#31657=CARTESIAN_POINT('Ctrl Pts',(-2.39384374823495,-1.29999999999126,
11.5397696257708));
#31658=CARTESIAN_POINT('Ctrl Pts',(-2.40293450860123,-1.18514270860368,
11.5215430360648));
#31659=CARTESIAN_POINT('Ctrl Pts',(-2.40176338657601,-1.06847604193766,
11.5011320141405));
#31660=CARTESIAN_POINT('Ctrl Pts',(-2.37535085920871,-0.794772683995164,
11.4489319948659));
#31661=CARTESIAN_POINT('Ctrl Pts',(-2.32358691483882,-0.636309800090644,
11.4015736207909));
#31662=CARTESIAN_POINT('Ctrl Pts',(-2.26260745230776,-0.319434907274874,
11.3561956820194));
#31663=CARTESIAN_POINT('Ctrl Pts',(-2.22075449856025,-0.158333333332199,
11.3329567614098));
#31664=CARTESIAN_POINT('Ctrl Pts',(-2.1933776976983,0.158333333332201,11.3475446147353));
#31665=CARTESIAN_POINT('Ctrl Pts',(-2.2070297755006,0.319434907274881,11.3858511686716));
#31666=CARTESIAN_POINT('Ctrl Pts',(-2.21392324748015,0.636309800090653,
11.4599662369897));
#31667=CARTESIAN_POINT('Ctrl Pts',(-2.23681589565793,0.794772683995154,
11.5231958510112));
#31668=CARTESIAN_POINT('Ctrl Pts',(-2.22172690592412,1.06847604193882,11.5962713636694));
#31669=CARTESIAN_POINT('Ctrl Pts',(-2.20674534455013,1.18514270860597,11.6243939658985));
#31670=CARTESIAN_POINT('Ctrl Pts',(-2.18331368635577,1.29999999999464,11.6490074886415));
#31671=CARTESIAN_POINT('Ctrl Pts',(-2.3993958962951,-1.29999999999108,11.5429379339209));
#31672=CARTESIAN_POINT('Ctrl Pts',(-2.40963711164426,-1.18514270860352,
11.5252625617807));
#31673=CARTESIAN_POINT('Ctrl Pts',(-2.40925885152419,-1.06847604193752,
11.5052961304459));
#31674=CARTESIAN_POINT('Ctrl Pts',(-2.38385188222345,-0.794772683995057,
11.4538768747274));
#31675=CARTESIAN_POINT('Ctrl Pts',(-2.33150560017621,-0.636309800090558,
11.4067303741552));
#31676=CARTESIAN_POINT('Ctrl Pts',(-2.27029307764192,-0.319434907274831,
11.3615972197224));
#31677=CARTESIAN_POINT('Ctrl Pts',(-2.22806961897634,-0.158333333332178,
11.3381674328317));
#31678=CARTESIAN_POINT('Ctrl Pts',(-2.20055719881342,0.15833333333218,11.3528635379026));
#31679=CARTESIAN_POINT('Ctrl Pts',(-2.21446773311546,0.319434907274838,
11.3914444408506));
#31680=CARTESIAN_POINT('Ctrl Pts',(-2.22127000615627,0.636309800090567,
11.4655856785406));
#31681=CARTESIAN_POINT('Ctrl Pts',(-2.24433616136474,0.794772683995047,
11.5289554442119));
#31682=CARTESIAN_POINT('Ctrl Pts',(-2.22824630643318,1.06847604193868,11.6012567828048));
#31683=CARTESIAN_POINT('Ctrl Pts',(-2.21258638767723,1.18514270860581,11.6288439582938));
#31684=CARTESIAN_POINT('Ctrl Pts',(-2.18823125217736,1.29999999999447,11.6527217388234));
#31685=CARTESIAN_POINT('Ctrl Pts',(-2.40498263771275,-1.2999999999909,11.5460747568237));
#31686=CARTESIAN_POINT('Ctrl Pts',(-2.41641862629916,-1.18514270860336,
11.5289131961289));
#31687=CARTESIAN_POINT('Ctrl Pts',(-2.41685823441742,-1.06847604193737,
11.5093701990312));
#31688=CARTESIAN_POINT('Ctrl Pts',(-2.39246997841415,-0.794772683994947,
11.4587203716772));
#31689=CARTESIAN_POINT('Ctrl Pts',(-2.33945608537769,-0.63630980009047,
11.4118556739238));
#31690=CARTESIAN_POINT('Ctrl Pts',(-2.27801195848589,-0.319434907274787,
11.3669690672671));
#31691=CARTESIAN_POINT('Ctrl Pts',(-2.23548655175409,-0.158333333332156,
11.343297255196));
#31692=CARTESIAN_POINT('Ctrl Pts',(-2.20785175166259,0.158333333332158,
11.3580926156387));
#31693=CARTESIAN_POINT('Ctrl Pts',(-2.22199769074485,0.319434907274794,
11.3969652894081));
#31694=CARTESIAN_POINT('Ctrl Pts',(-2.22866855381979,0.63630980009048,11.4711630031246));
#31695=CARTESIAN_POINT('Ctrl Pts',(-2.25185434580907,0.794772683994938,
11.5347125753992));
#31696=CARTESIAN_POINT('Ctrl Pts',(-2.23474272493949,1.06847604193853,11.6062561397551));
#31697=CARTESIAN_POINT('Ctrl Pts',(-2.21840523355752,1.18514270860564,11.6333079034982));
#31698=CARTESIAN_POINT('Ctrl Pts',(-2.19313723742002,1.29999999999429,11.6564428729249));
#31699=CARTESIAN_POINT('Ctrl Pts',(-2.40914654649501,-1.2999999999908,11.5484482846422));
#31700=CARTESIAN_POINT('Ctrl Pts',(-2.42145246870887,-1.18514270860326,
11.5316937523024));
#31701=CARTESIAN_POINT('Ctrl Pts',(-2.42249597593041,-1.06847604193728,
11.5124761826751));
#31702=CARTESIAN_POINT('Ctrl Pts',(-2.39888825469448,-0.794772683994884,
11.4623896435116));
#31703=CARTESIAN_POINT('Ctrl Pts',(-2.34547205339143,-0.636309800090419,
11.4156545845343));
#31704=CARTESIAN_POINT('Ctrl Pts',(-2.28386607035366,-0.319434907274761,
11.3709429071027));
#31705=CARTESIAN_POINT('Ctrl Pts',(-2.24103624516728,-0.158333333332144,
11.3471534745865));
#31706=CARTESIAN_POINT('Ctrl Pts',(-2.21331083745272,0.158333333332146,
11.3620235089939));
#31707=CARTESIAN_POINT('Ctrl Pts',(-2.22768593270914,0.319434907274768,
11.4010732922679));
#31708=CARTESIAN_POINT('Ctrl Pts',(-2.23430283336779,0.636309800090429,
11.4752791128073));
#31709=CARTESIAN_POINT('Ctrl Pts',(-2.25762873040171,0.794772683994874,
11.5389258277537));
#31710=CARTESIAN_POINT('Ctrl Pts',(-2.23972418478954,1.06847604193844,11.6099211871069));
#31711=CARTESIAN_POINT('Ctrl Pts',(-2.22284695037678,1.18514270860555,11.6365952450213));
#31712=CARTESIAN_POINT('Ctrl Pts',(-2.19684269591802,1.29999999999418,11.6592121004232));
#31713=CARTESIAN_POINT('Ctrl Pts',(-2.41258175685607,-1.29999999999069,
11.5504545132532));
#31714=CARTESIAN_POINT('Ctrl Pts',(-2.42557611387912,-1.18514270860317,
11.5340694313134));
#31715=CARTESIAN_POINT('Ctrl Pts',(-2.42710829624824,-1.0684760419372,11.5151351004672));
#31716=CARTESIAN_POINT('Ctrl Pts',(-2.40416802758222,-0.79477268399482,
11.4655037334637));
#31717=CARTESIAN_POINT('Ctrl Pts',(-2.35054178435821,-0.636309800090368,
11.418772956396));
#31718=CARTESIAN_POINT('Ctrl Pts',(-2.28881475441011,-0.319434907274735,
11.3741949147268));
#31719=CARTESIAN_POINT('Ctrl Pts',(-2.24563279714406,-0.158333333332131,
11.3503872817849));
#31720=CARTESIAN_POINT('Ctrl Pts',(-2.21783129393859,0.158333333332133,
11.3653210871155));
#31721=CARTESIAN_POINT('Ctrl Pts',(-2.2324594281046,0.319434907274742,11.404469400769));
#31722=CARTESIAN_POINT('Ctrl Pts',(-2.23908921925421,0.636309800090377,
11.4786377527717));
#31723=CARTESIAN_POINT('Ctrl Pts',(-2.26260060340433,0.794772683994809,
11.5423141082442));
#31724=CARTESIAN_POINT('Ctrl Pts',(-2.24400853998536,1.06847604193836,11.6128729407444));
#31725=CARTESIAN_POINT('Ctrl Pts',(-2.22664498479955,1.18514270860545,11.6392598442532));
#31726=CARTESIAN_POINT('Ctrl Pts',(-2.1999656897782,1.29999999999408,11.6614913471435));
#31727=CARTESIAN_POINT('Ctrl Pts',(-2.41479985369412,-1.29999999999066,
11.551770597191));
#31728=CARTESIAN_POINT('Ctrl Pts',(-2.42822503947843,-1.18514270860314,
11.5356393929169));
#31729=CARTESIAN_POINT('Ctrl Pts',(-2.43006810827712,-1.06847604193717,
11.5168947157906));
#31730=CARTESIAN_POINT('Ctrl Pts',(-2.40756895867542,-0.794772683994802,
11.4675531166573));
#31731=CARTESIAN_POINT('Ctrl Pts',(-2.35386136455652,-0.636309800090354,
11.4207795398731));
#31732=CARTESIAN_POINT('Ctrl Pts',(-2.29206364242793,-0.319434907274728,
11.3762815092146));
#31733=CARTESIAN_POINT('Ctrl Pts',(-2.24861335875392,-0.158333333332127,
11.3524939667356));
#31734=CARTESIAN_POINT('Ctrl Pts',(-2.2207617827267,0.158333333332129,11.3674701657722));
#31735=CARTESIAN_POINT('Ctrl Pts',(-2.23557703714212,0.319434907274735,
11.406664705906));
#31736=CARTESIAN_POINT('Ctrl Pts',(-2.2422389421051,0.636309800090363,11.4807906699131));
#31737=CARTESIAN_POINT('Ctrl Pts',(-2.26590157058328,0.794772683994792,
11.5444633217759));
#31738=CARTESIAN_POINT('Ctrl Pts',(-2.24685296736716,1.06847604193833,11.6147458579512));
#31739=CARTESIAN_POINT('Ctrl Pts',(-2.22915869582073,1.18514270860543,11.6409572171816));
#31740=CARTESIAN_POINT('Ctrl Pts',(-2.20201558723986,1.29999999999405,11.6629572299565));
#31741=CARTESIAN_POINT('Ctrl Pts',(-2.41582200093143,-1.29999999999066,
11.552379271273));
#31742=CARTESIAN_POINT('Ctrl Pts',(-2.42944422392667,-1.18514270860313,
11.5363667074415));
#31743=CARTESIAN_POINT('Ctrl Pts',(-2.43143011088096,-1.06847604193717,
11.5177100967283));
#31744=CARTESIAN_POINT('Ctrl Pts',(-2.40913564292502,-0.794772683994798,
11.4685013165023));
#31745=CARTESIAN_POINT('Ctrl Pts',(-2.3553968845436,-0.63630980009035,11.4217027331553));
#31746=CARTESIAN_POINT('Ctrl Pts',(-2.2935679446324,-0.319434907274726,
11.3772404685971));
#31747=CARTESIAN_POINT('Ctrl Pts',(-2.24999004172294,-0.158333333332126,
11.3534652817272));
#31748=CARTESIAN_POINT('Ctrl Pts',(-2.22211532483174,0.158333333332128,
11.3684611396057));
#31749=CARTESIAN_POINT('Ctrl Pts',(-2.23701876714905,0.319434907274733,
11.4076755865086));
#31750=CARTESIAN_POINT('Ctrl Pts',(-2.24369793613448,0.636309800090359,
11.4817801555651));
#31751=CARTESIAN_POINT('Ctrl Pts',(-2.26743402756379,0.794772683994788,
11.5454483435967));
#31752=CARTESIAN_POINT('Ctrl Pts',(-2.24817376393022,1.06847604193833,11.6156041394163));
#31753=CARTESIAN_POINT('Ctrl Pts',(-2.23032528206969,1.18514270860542,11.6417357041927));
#31754=CARTESIAN_POINT('Ctrl Pts',(-2.20296537281255,1.29999999999404,11.6636309892633));
#31755=CARTESIAN_POINT('Ctrl Pts',(-2.41633274985894,-1.29999999999066,
11.5526838631196));
#31756=CARTESIAN_POINT('Ctrl Pts',(-2.4300531426528,-1.18514270860313,11.5367309017281));
#31757=CARTESIAN_POINT('Ctrl Pts',(-2.43211031121549,-1.06847604193717,
11.5181184256399));
#31758=CARTESIAN_POINT('Ctrl Pts',(-2.40991840093643,-0.794772683994798,
11.4689758714796));
#31759=CARTESIAN_POINT('Ctrl Pts',(-2.35616528808526,-0.63630980009035,
11.4221637757094));
#31760=CARTESIAN_POINT('Ctrl Pts',(-2.29432104999001,-0.319434907274726,
11.3777191388923));
#31761=CARTESIAN_POINT('Ctrl Pts',(-2.25067868375102,-0.158333333332126,
11.3539506638623));
#31762=CARTESIAN_POINT('Ctrl Pts',(-2.22279239010064,0.158333333332128,
11.3689563687736));
#31763=CARTESIAN_POINT('Ctrl Pts',(-2.23774018786867,0.319434907274733,
11.4081805651302));
#31764=CARTESIAN_POINT('Ctrl Pts',(-2.2444284512897,0.636309800090359,11.4822740913695));
#31765=CARTESIAN_POINT('Ctrl Pts',(-2.26820204945816,0.794772683994787,
11.54593946188));
#31766=CARTESIAN_POINT('Ctrl Pts',(-2.24883578981785,1.06847604193833,11.6160320272022));
#31767=CARTESIAN_POINT('Ctrl Pts',(-2.230909898264,1.18514270860542,11.6421239338287));
#31768=CARTESIAN_POINT('Ctrl Pts',(-2.203441051364,1.29999999999404,11.663967272739));
#31769=CARTESIAN_POINT('Ctrl Pts',(-2.41675820700139,-1.29999999999065,
11.5529378166722));
#31770=CARTESIAN_POINT('Ctrl Pts',(-2.43056017544808,-1.18514270860313,
11.5370347104054));
#31771=CARTESIAN_POINT('Ctrl Pts',(-2.43267666240502,-1.06847604193716,
11.518459078027));
#31772=CARTESIAN_POINT('Ctrl Pts',(-2.41057037076349,-0.794772683994795,
11.4693715812357));
#31773=CARTESIAN_POINT('Ctrl Pts',(-2.35680614313646,-0.636309800090348,
11.4225475297451));
#31774=CARTESIAN_POINT('Ctrl Pts',(-2.29494934815928,-0.319434907274725,
11.3781174269183));
#31775=CARTESIAN_POINT('Ctrl Pts',(-2.25125276855931,-0.158333333332126,
11.3543549505202));
#31776=CARTESIAN_POINT('Ctrl Pts',(-2.22335681619686,0.158333333332128,
11.3693688811036));
#31777=CARTESIAN_POINT('Ctrl Pts',(-2.23834181768131,0.319434907274732,
11.4086010137786));
#31778=CARTESIAN_POINT('Ctrl Pts',(-2.24503793720342,0.636309800090357,
11.4826851317409));
#31779=CARTESIAN_POINT('Ctrl Pts',(-2.26884316755643,0.794772683994785,
11.5463478715594));
#31780=CARTESIAN_POINT('Ctrl Pts',(-2.24938848253282,1.06847604193832,11.6163878284211));
#31781=CARTESIAN_POINT('Ctrl Pts',(-2.23139792006516,1.18514270860542,11.6424468164652));
#31782=CARTESIAN_POINT('Ctrl Pts',(-2.20383800740949,1.29999999999404,11.664247090464));
#31783=CARTESIAN_POINT('Ctrl Pts',(-2.41705590659015,-1.29999999999065,
11.5531156734398));
#31784=CARTESIAN_POINT('Ctrl Pts',(-2.43091492013701,-1.18514270860313,
11.5372475088211));
#31785=CARTESIAN_POINT('Ctrl Pts',(-2.4330729216556,-1.06847604193717,11.5186976709358));
#31786=CARTESIAN_POINT('Ctrl Pts',(-2.41102665830558,-0.794772683994796,
11.4696486328263));
#31787=CARTESIAN_POINT('Ctrl Pts',(-2.3572549218525,-0.636309800090349,
11.4228159918964));
#31788=CARTESIAN_POINT('Ctrl Pts',(-2.29538951710301,-0.319434907274726,
11.3783959181394));
#31789=CARTESIAN_POINT('Ctrl Pts',(-2.25165502805312,-0.158333333332126,
11.3546376119136));
#31790=CARTESIAN_POINT('Ctrl Pts',(-2.22375232379798,0.158333333332128,
11.3696572959091));
#31791=CARTESIAN_POINT('Ctrl Pts',(-2.2387632088314,0.319434907274733,11.4088951096365));
#31792=CARTESIAN_POINT('Ctrl Pts',(-2.24546492778164,0.636309800090358,
11.4829725708656));
#31793=CARTESIAN_POINT('Ctrl Pts',(-2.26929268971541,0.794772683994786,
11.5466331714944));
#31794=CARTESIAN_POINT('Ctrl Pts',(-2.24977607999461,1.06847604193833,11.6166363340987));
#31795=CARTESIAN_POINT('Ctrl Pts',(-2.23174014485318,1.18514270860542,11.6426723646367));
#31796=CARTESIAN_POINT('Ctrl Pts',(-2.20411629175686,1.29999999999404,11.6644426504939));
#31797=CARTESIAN_POINT('Ctrl Pts',(-2.41722606302245,-1.29999999999065,
11.5532172741863));
#31798=CARTESIAN_POINT('Ctrl Pts',(-2.43111759854394,-1.18514270860313,
11.5373691393569));
#31799=CARTESIAN_POINT('Ctrl Pts',(-2.43329928412564,-1.06847604193716,
11.5188340736756));
#31800=CARTESIAN_POINT('Ctrl Pts',(-2.4112873183557,-0.794772683994793,
11.4698070162378));
#31801=CARTESIAN_POINT('Ctrl Pts',(-2.3575115020879,-0.636309800090347,
11.4229692923526));
#31802=CARTESIAN_POINT('Ctrl Pts',(-2.29564112459873,-0.319434907274725,
11.3785549922577));
#31803=CARTESIAN_POINT('Ctrl Pts',(-2.25188468402401,-0.158333333332125,
11.3547993039445));
#31804=CARTESIAN_POINT('Ctrl Pts',(-2.22397810772574,0.158333333332127,
11.3698222911059));
#31805=CARTESIAN_POINT('Ctrl Pts',(-2.23900405544359,0.319434907274732,
11.4090631384977));
#31806=CARTESIAN_POINT('Ctrl Pts',(-2.2457090050593,0.636309800090356,11.4831367708317));
#31807=CARTESIAN_POINT('Ctrl Pts',(-2.26954942789417,0.794772683994783,
11.5467963146545));
#31808=CARTESIAN_POINT('Ctrl Pts',(-2.24999742106405,1.06847604193832,11.6167784568709));
#31809=CARTESIAN_POINT('Ctrl Pts',(-2.23193558967195,1.18514270860541,11.6428013423576));
#31810=CARTESIAN_POINT('Ctrl Pts',(-2.2042752661713,1.29999999999404,11.6645544370595));
#31811=CARTESIAN_POINT('Ctrl Pts',(-2.42819110567103,-1.29999999999132,
11.559777914713));
#31812=CARTESIAN_POINT('Ctrl Pts',(-2.44418755880433,-1.18514270860374,
11.5452153494114));
#31813=CARTESIAN_POINT('Ctrl Pts',(-2.447901541625,-1.06847604193771,11.5276289970943));
#31814=CARTESIAN_POINT('Ctrl Pts',(-2.42810662139858,-0.794772683995203,
11.480015452192));
#31815=CARTESIAN_POINT('Ctrl Pts',(-2.37405249916826,-0.636309800090674,
11.4328626476282));
#31816=CARTESIAN_POINT('Ctrl Pts',(-2.31187591576949,-0.319434907274889,
11.3888090582204));
#31817=CARTESIAN_POINT('Ctrl Pts',(-2.26674213815886,-0.158333333332207,
11.3651910796362));
#31818=CARTESIAN_POINT('Ctrl Pts',(-2.238587891913,0.158333333332209,11.380425036069));
#31819=CARTESIAN_POINT('Ctrl Pts',(-2.25454393150171,0.319434907274896,
11.4198940053948));
#31820=CARTESIAN_POINT('Ctrl Pts',(-2.26145712152465,0.636309800090683,
11.4937212127157));
#31821=CARTESIAN_POINT('Ctrl Pts',(-2.28615700088231,0.794772683995192,
11.5572796140882));
#31822=CARTESIAN_POINT('Ctrl Pts',(-2.26432247843443,1.06847604193887,11.6259065144236));
#31823=CARTESIAN_POINT('Ctrl Pts',(-2.24458242658572,1.18514270860602,11.651088268924));
#31824=CARTESIAN_POINT('Ctrl Pts',(-2.21455367860727,1.2999999999947,11.6717457356466));
#31825=CARTESIAN_POINT('Ctrl Pts',(-2.4452524353986,-1.29999999999661,11.5689626063178));
#31826=CARTESIAN_POINT('Ctrl Pts',(-2.46485785577321,-1.18514270860856,
11.555909053355));
#31827=CARTESIAN_POINT('Ctrl Pts',(-2.47109284500115,-1.06847604194207,
11.5395304089526));
#31828=CARTESIAN_POINT('Ctrl Pts',(-2.45460854672865,-0.794772683998442,
11.4940108374389));
#31829=CARTESIAN_POINT('Ctrl Pts',(-2.39902048241243,-0.636309800093267,
11.4473280503375));
#31830=CARTESIAN_POINT('Ctrl Pts',(-2.33622754359863,-0.31943490727619,
11.4039687597331));
#31831=CARTESIAN_POINT('Ctrl Pts',(-2.28981669923967,-0.158333333332852,
11.3799513324971));
#31832=CARTESIAN_POINT('Ctrl Pts',(-2.26119977660626,0.158333333332854,
11.3955792241029));
#31833=CARTESIAN_POINT('Ctrl Pts',(-2.27812146022787,0.319434907276197,
11.4357148298775));
#31834=CARTESIAN_POINT('Ctrl Pts',(-2.28440047433871,0.636309800093275,
11.509908331257));
#31835=CARTESIAN_POINT('Ctrl Pts',(-2.30861800866693,0.79477268399843,11.5746559944769));
#31836=CARTESIAN_POINT('Ctrl Pts',(-2.28392282923828,1.06847604194322,11.6408880860855));
#31837=CARTESIAN_POINT('Ctrl Pts',(-2.26247078692541,1.18514270861085,11.6642386146762));
#31838=CARTESIAN_POINT('Ctrl Pts',(-2.23025633042783,1.3,11.6822702535409));
#31839=CARTESIAN_POINT('Ctrl Pts',(-2.46724316344813,-1.29999999999784,
11.5817116024117));
#31840=CARTESIAN_POINT('Ctrl Pts',(-2.49156329534275,-1.18514270860968,
11.5707273717748));
#31841=CARTESIAN_POINT('Ctrl Pts',(-2.50112410315566,-1.06847604194307,
11.5559728301234));
#31842=CARTESIAN_POINT('Ctrl Pts',(-2.48911449061508,-0.794772683999187,
11.5131767145811));
#31843=CARTESIAN_POINT('Ctrl Pts',(-2.43184874460611,-0.636309800093867,
11.4668385900733));
#31844=CARTESIAN_POINT('Ctrl Pts',(-2.36827119090855,-0.319434907276493,
11.4243665324868));
#31845=CARTESIAN_POINT('Ctrl Pts',(-2.31971696369294,-0.158333333333001,
11.4001531084736));
#31846=CARTESIAN_POINT('Ctrl Pts',(-2.29076029791301,0.158333333333003,
11.4160813995587));
#31847=CARTESIAN_POINT('Ctrl Pts',(-2.30932133201575,0.319434907276497,
11.4568243292661));
#31848=CARTESIAN_POINT('Ctrl Pts',(-2.31602757401349,0.636309800093875,
11.5305165380476));
#31849=CARTESIAN_POINT('Ctrl Pts',(-2.34232654690967,0.794772683999182,
11.5947733929765));
#31850=CARTESIAN_POINT('Ctrl Pts',(-2.3127375908089,1.06847604194423,11.6586016481313));
#31851=CARTESIAN_POINT('Ctrl Pts',(-2.287642941349,1.18514270861197,11.6805270508448));
#31852=CARTESIAN_POINT('Ctrl Pts',(-2.25026160514642,1.30000000000123,11.696748969685));
#31853=CARTESIAN_POINT('Ctrl Pts',(-2.47880653387082,-1.30000000000056,
11.5876140197912));
#31854=CARTESIAN_POINT('Ctrl Pts',(-2.5053034943636,-1.18514270861216,11.5778000280662));
#31855=CARTESIAN_POINT('Ctrl Pts',(-2.51643668958126,-1.06847604194531,
11.5639215937233));
#31856=CARTESIAN_POINT('Ctrl Pts',(-2.50666322642595,-0.794772684000851,
11.5224699584834));
#31857=CARTESIAN_POINT('Ctrl Pts',(-2.44892689462504,-0.636309800095197,
11.4759868772666));
#31858=CARTESIAN_POINT('Ctrl Pts',(-2.38514150298642,-0.319434907277159,
11.4338197429392));
#31859=CARTESIAN_POINT('Ctrl Pts',(-2.33567769709269,-0.158333333333332,
11.4094186534397));
#31860=CARTESIAN_POINT('Ctrl Pts',(-2.30625480759988,0.158333333333334,
11.4257498401733));
#31861=CARTESIAN_POINT('Ctrl Pts',(-2.32505056891377,0.319434907277167,
11.4672540947557));
#31862=CARTESIAN_POINT('Ctrl Pts',(-2.33143994443199,0.636309800095206,
11.5411142162616));
#31863=CARTESIAN_POINT('Ctrl Pts',(-2.35820372983969,0.79477268400084,11.6055491315694));
#31864=CARTESIAN_POINT('Ctrl Pts',(-2.32663344521572,1.06847604194647,11.667852136859));
#31865=CARTESIAN_POINT('Ctrl Pts',(-2.30018582393963,1.18514270861445,11.6887302009383));
#31866=CARTESIAN_POINT('Ctrl Pts',(-2.26095618780691,1.30000000000395,11.7035176666606));
#31867=CARTESIAN_POINT('Ctrl Pts',(-2.48455995069208,-1.30000000000056,
11.5905856245377));
#31868=CARTESIAN_POINT('Ctrl Pts',(-2.51213562603867,-1.18514270861216,
11.5813640954911));
#31869=CARTESIAN_POINT('Ctrl Pts',(-2.52404941520513,-1.06847604194531,
11.5679279706886));
#31870=CARTESIAN_POINT('Ctrl Pts',(-2.51539056129935,-0.794772684000851,
11.5271512751842));
#31871=CARTESIAN_POINT('Ctrl Pts',(-2.45746810794787,-0.636309800095197,
11.4805575163309));
#31872=CARTESIAN_POINT('Ctrl Pts',(-2.39351595813042,-0.319434907277159,
11.4385926643448));
#31873=CARTESIAN_POINT('Ctrl Pts',(-2.34340372597283,-0.158333333333332,
11.4142508800478));
#31874=CARTESIAN_POINT('Ctrl Pts',(-2.3138047860753,0.158333333333334,11.4307376305815));
#31875=CARTESIAN_POINT('Ctrl Pts',(-2.33301542000644,0.319434907277167,
11.4723857856749));
#31876=CARTESIAN_POINT('Ctrl Pts',(-2.3393300816685,0.636309800095206,11.5462634539526));
#31877=CARTESIAN_POINT('Ctrl Pts',(-2.36620091374559,0.79477268400084,11.6108904285002));
#31878=CARTESIAN_POINT('Ctrl Pts',(-2.33354901187538,1.06847604194647,11.6724986686556));
#31879=CARTESIAN_POINT('Ctrl Pts',(-2.30638156847317,1.18514270861445,11.6928839421724));
#31880=CARTESIAN_POINT('Ctrl Pts',(-2.26618048011623,1.30000000000395,11.706986564853));
#31881=CARTESIAN_POINT('',(-2.20682734928731,1.2,11.6308478929475));
#31882=CARTESIAN_POINT('Ctrl Pts',(-2.20682734928731,1.2,11.6308478929475));
#31883=CARTESIAN_POINT('Ctrl Pts',(-2.18722751564924,1.21680586990626,11.6218348082994));
#31884=CARTESIAN_POINT('Ctrl Pts',(-2.16687973003508,1.23316195266879,11.6136279694703));
#31885=CARTESIAN_POINT('Ctrl Pts',(-2.12794466941964,1.26665720486854,11.5953463142025));
#31886=CARTESIAN_POINT('Ctrl Pts',(-2.11129558646823,1.28061603972248,11.5878883456529));
#31887=CARTESIAN_POINT('Ctrl Pts',(-2.08916921284536,1.29999999999857,11.5769706419067));
#31888=CARTESIAN_POINT('',(-2.34584244559631,0.653834841342843,11.5588442527862));
#31889=CARTESIAN_POINT('Ctrl Pts',(-2.34584244556543,0.653834841328552,
11.5588442528477));
#31890=CARTESIAN_POINT('Ctrl Pts',(-2.33308818544499,0.710941609821211,
11.5657083395222));
#31891=CARTESIAN_POINT('Ctrl Pts',(-2.31925861336638,0.767441603499411,
11.5730759416769));
#31892=CARTESIAN_POINT('Ctrl Pts',(-2.29084677666368,0.881463280997958,
11.5880272054701));
#31893=CARTESIAN_POINT('Ctrl Pts',(-2.27703180365721,0.939232753787813,
11.5952229786298));
#31894=CARTESIAN_POINT('Ctrl Pts',(-2.25131149177042,1.03694567063666,11.6084232885134));
#31895=CARTESIAN_POINT('Ctrl Pts',(-2.25039295349595,1.03976101801352,11.6089199951471));
#31896=CARTESIAN_POINT('Ctrl Pts',(-2.22336742624557,1.1397561733151,11.6225869212586));
#31897=CARTESIAN_POINT('Ctrl Pts',(-2.21631092062426,1.16602124943616,11.6261245070176));
#31898=CARTESIAN_POINT('Ctrl Pts',(-2.20682734928732,1.2,11.6308478929475));
#31899=CARTESIAN_POINT('',(-2.46774460503229,-0.653834841531101,11.4910064745155));
#31900=CARTESIAN_POINT('Ctrl Pts',(-2.4677446050323,-0.653834841531096,
11.4910064745155));
#31901=CARTESIAN_POINT('Ctrl Pts',(-2.43366531823515,-0.575743557741863,
11.466975601479));
#31902=CARTESIAN_POINT('Ctrl Pts',(-2.40440869672623,-0.493700050753892,
11.4475328008353));
#31903=CARTESIAN_POINT('Ctrl Pts',(-2.36105542073859,-0.338105451951495,
11.4213410229621));
#31904=CARTESIAN_POINT('Ctrl Pts',(-2.34510240028127,-0.265657096721669,
11.413182399269));
#31905=CARTESIAN_POINT('Ctrl Pts',(-2.32174616561371,-0.129731483841709,
11.4060384736905));
#31906=CARTESIAN_POINT('Ctrl Pts',(-2.3134924786683,-0.0666595841288654,
11.4058576315973));
#31907=CARTESIAN_POINT('Ctrl Pts',(-2.30170738667741,0.0595017295460707,
11.4119861541816));
#31908=CARTESIAN_POINT('Ctrl Pts',(-2.2980945337294,0.122719333871996,11.4183180474692));
#31909=CARTESIAN_POINT('Ctrl Pts',(-2.29615087668656,0.260098698859542,
11.43886499628));
#31910=CARTESIAN_POINT('Ctrl Pts',(-2.29885542227659,0.333972211087808,
11.4543396536581));
#31911=CARTESIAN_POINT('Ctrl Pts',(-2.31369980548976,0.4915232539199,11.4967249168017));
#31912=CARTESIAN_POINT('Ctrl Pts',(-2.32714440364268,0.574928604049013,
11.525508188405));
#31913=CARTESIAN_POINT('Ctrl Pts',(-2.34584244548056,0.653834841363857,
11.5588442528014));
#31914=CARTESIAN_POINT('',(-2.40481962522456,-1.2,11.5265855556241));
#31915=CARTESIAN_POINT('Ctrl Pts',(-2.40481962522456,-1.2,11.5265855556241));
#31916=CARTESIAN_POINT('Ctrl Pts',(-2.41054630292152,-1.16532760456162,
11.5234025313348));
#31917=CARTESIAN_POINT('Ctrl Pts',(-2.42645100662694,-1.06865554280768,
11.5145509637945));
#31918=CARTESIAN_POINT('Ctrl Pts',(-2.46017068471683,-0.773244824243328,
11.4953835148662));
#31919=CARTESIAN_POINT('Ctrl Pts',(-2.46337028885984,-0.721311495190602,
11.4935221302712));
#31920=CARTESIAN_POINT('Ctrl Pts',(-2.4677446050323,-0.653834841531101,
11.4910064745155));
#31921=CARTESIAN_POINT('Ctrl Pts',(-2.2912385497941,-1.29999999999519,11.4746609114623));
#31922=CARTESIAN_POINT('Ctrl Pts',(-2.31023238688351,-1.28305568231735,
11.4837050274263));
#31923=CARTESIAN_POINT('Ctrl Pts',(-2.32942890430126,-1.26619847603817,
11.4924852393854));
#31924=CARTESIAN_POINT('Ctrl Pts',(-2.3518627461632,-1.24605776992158,11.5031844201827));
#31925=CARTESIAN_POINT('Ctrl Pts',(-2.36202118513148,-1.23682069842138,
11.5081629233068));
#31926=CARTESIAN_POINT('Ctrl Pts',(-2.3803328638717,-1.22104712035176,11.5160864571013));
#31927=CARTESIAN_POINT('Ctrl Pts',(-2.38516684913272,-1.21689694692977,
11.5181587343142));
#31928=CARTESIAN_POINT('Ctrl Pts',(-2.39187438277638,-1.21105168977261,
11.5211282035769));
#31929=CARTESIAN_POINT('Ctrl Pts',(-2.39877337851287,-1.205063204871,11.5241534457709));
#31930=CARTESIAN_POINT('Ctrl Pts',(-2.40481962522456,-1.2,11.5265855556241));
#31931=CARTESIAN_POINT('Origin',(0.,1.25,7.2));
#31932=CARTESIAN_POINT('Origin',(0.,1.2,7.2));
#31933=CARTESIAN_POINT('Origin',(0.,0.92691742076555,7.2));
#31934=CARTESIAN_POINT('Origin',(0.,0.653834841531101,7.2));
#31935=CARTESIAN_POINT('Origin',(0.,0.,7.2));
#31936=CARTESIAN_POINT('Origin',(0.,-0.653834841531101,7.2));
#31937=CARTESIAN_POINT('Origin',(0.,-0.926917420765551,7.2));
#31938=CARTESIAN_POINT('Origin',(0.,-1.2,7.2));
#31939=CARTESIAN_POINT('Origin',(0.,-1.25,7.2));
#31940=CARTESIAN_POINT('Ctrl Pts',(-2.77007461962166,-1.30000000000024,
11.4160631477717));
#31941=CARTESIAN_POINT('Ctrl Pts',(-2.73776084594322,-1.18514270861195,
11.4438270002089));
#31942=CARTESIAN_POINT('Ctrl Pts',(-2.70652295951427,-1.0684760419452,11.457162059593));
#31943=CARTESIAN_POINT('Ctrl Pts',(-2.63684270752248,-0.794772684000851,
11.4546353160166));
#31944=CARTESIAN_POINT('Ctrl Pts',(-2.59430952183081,-0.636309800095197,
11.39905100554));
#31945=CARTESIAN_POINT('Ctrl Pts',(-2.53348691516026,-0.319434907277159,
11.3566435139844));
#31946=CARTESIAN_POINT('Ctrl Pts',(-2.50702387179492,-0.158333333333332,
11.3191825394316));
#31947=CARTESIAN_POINT('Ctrl Pts',(-2.47794645705815,0.158333333333334,
11.3365725980411));
#31948=CARTESIAN_POINT('Ctrl Pts',(-2.47397094455433,0.319434907277167,
11.3921419562788));
#31949=CARTESIAN_POINT('Ctrl Pts',(-2.47833749753066,0.636309800095206,
11.4685085686389));
#31950=CARTESIAN_POINT('Ctrl Pts',(-2.48972764967703,0.79477268400084,11.5419677641134));
#31951=CARTESIAN_POINT('Ctrl Pts',(-2.52071187691362,1.0684760419458,11.5698548993163));
#31952=CARTESIAN_POINT('Ctrl Pts',(-2.53830479690509,1.18514270861313,11.5662553176453));
#31953=CARTESIAN_POINT('Ctrl Pts',(-2.56007871299605,1.300000000002,11.5469848467941));
#31954=CARTESIAN_POINT('Ctrl Pts',(-2.7696826118328,-1.30000000000024,11.4098043288393));
#31955=CARTESIAN_POINT('Ctrl Pts',(-2.73726147280167,-1.18514270861195,
11.436384457461));
#31956=CARTESIAN_POINT('Ctrl Pts',(-2.70595672829373,-1.0684760419452,11.4488497373219));
#31957=CARTESIAN_POINT('Ctrl Pts',(-2.63621560067023,-0.794772684000851,
11.4450389031677));
#31958=CARTESIAN_POINT('Ctrl Pts',(-2.59379521981159,-0.636309800095197,
11.3896433274275));
#31959=CARTESIAN_POINT('Ctrl Pts',(-2.53302516601485,-0.319434907277159,
11.3471799051539));
#31960=CARTESIAN_POINT('Ctrl Pts',(-2.50647930784202,-0.158333333333332,
11.3101501710864));
#31961=CARTESIAN_POINT('Ctrl Pts',(-2.47762464051037,0.158333333333334,
11.3274655474731));
#31962=CARTESIAN_POINT('Ctrl Pts',(-2.47402470095201,0.319434907277167,
11.382503004698));
#31963=CARTESIAN_POINT('Ctrl Pts',(-2.47864981465855,0.636309800095206,
11.4588263414016));
#31964=CARTESIAN_POINT('Ctrl Pts',(-2.49003717792243,0.79477268400084,11.5320690120471));
#31965=CARTESIAN_POINT('Ctrl Pts',(-2.52104861549134,1.0684760419458,11.5612588970434));
#31966=CARTESIAN_POINT('Ctrl Pts',(-2.53863428980996,1.18514270861313,11.5585564843371));
#31967=CARTESIAN_POINT('Ctrl Pts',(-2.56038193621059,1.300000000002,11.5405164393015));
#31968=CARTESIAN_POINT('Ctrl Pts',(-2.76915281737503,-1.30000000000057,
11.3971658160928));
#31969=CARTESIAN_POINT('Ctrl Pts',(-2.73640851043879,-1.18514270861224,
11.4214308270861));
#31970=CARTESIAN_POINT('Ctrl Pts',(-2.70487251583296,-1.06847604194547,
11.4322014493312));
#31971=CARTESIAN_POINT('Ctrl Pts',(-2.63480950274466,-0.794772684001051,
11.425909003821));
#31972=CARTESIAN_POINT('Ctrl Pts',(-2.59234201760466,-0.636309800095355,
11.3709915412348));
#31973=CARTESIAN_POINT('Ctrl Pts',(-2.53187715672899,-0.319434907277237,
11.3283362951877));
#31974=CARTESIAN_POINT('Ctrl Pts',(-2.50584772331639,-0.158333333333372,
11.2918997445371));
#31975=CARTESIAN_POINT('Ctrl Pts',(-2.4775646853384,0.158333333333373,11.309017362706));
#31976=CARTESIAN_POINT('Ctrl Pts',(-2.47426262756895,0.319434907277246,
11.3631728921772));
#31977=CARTESIAN_POINT('Ctrl Pts',(-2.47925260021527,0.636309800095363,
11.439470565577));
#31978=CARTESIAN_POINT('Ctrl Pts',(-2.49074116951473,0.794772684001036,
11.5122361618323));
#31979=CARTESIAN_POINT('Ctrl Pts',(-2.52180172561918,1.06847604194606,11.5440328862475));
#31980=CARTESIAN_POINT('Ctrl Pts',(-2.53936376159819,1.18514270861343,11.5431282164631));
#31981=CARTESIAN_POINT('Ctrl Pts',(-2.56104286972559,1.30000000000233,11.5275552530796));
#31982=CARTESIAN_POINT('Ctrl Pts',(-2.76670318044365,-1.30000000000057,
11.3725613695234));
#31983=CARTESIAN_POINT('Ctrl Pts',(-2.73495204203674,-1.18514270861225,
11.3914589550316));
#31984=CARTESIAN_POINT('Ctrl Pts',(-2.70398432429643,-1.06847604194547,
11.3983717895585));
#31985=CARTESIAN_POINT('Ctrl Pts',(-2.63425255970823,-0.794772684001053,
11.3866546479154));
#31986=CARTESIAN_POINT('Ctrl Pts',(-2.59026178357869,-0.636309800095359,
11.3333141793376));
#31987=CARTESIAN_POINT('Ctrl Pts',(-2.52922897848775,-0.319434907277241,
11.2907460649789));
#31988=CARTESIAN_POINT('Ctrl Pts',(-2.50314228401203,-0.158333333333373,
11.2559401072439));
#31989=CARTESIAN_POINT('Ctrl Pts',(-2.47526690486424,0.158333333333374,
11.2729219488189));
#31990=CARTESIAN_POINT('Ctrl Pts',(-2.4725788014573,0.319434907277247,11.3252350049386));
#31991=CARTESIAN_POINT('Ctrl Pts',(-2.47866351752077,0.636309800095367,
11.4013239975511));
#31992=CARTESIAN_POINT('Ctrl Pts',(-2.49147185773774,0.794772684001045,
11.4727412600865));
#31993=CARTESIAN_POINT('Ctrl Pts',(-2.52265808377612,1.06847604194607,11.5097741407791));
#31994=CARTESIAN_POINT('Ctrl Pts',(-2.53993770890259,1.18514270861343,11.5125717343214));
#31995=CARTESIAN_POINT('Ctrl Pts',(-2.56099759746704,1.30000000000233,11.5021367595577));
#31996=CARTESIAN_POINT('Ctrl Pts',(-2.76535570772393,-1.30000000000129,
11.3536900155371));
#31997=CARTESIAN_POINT('Ctrl Pts',(-2.73242312356743,-1.1851427086129,11.3693724675759));
#31998=CARTESIAN_POINT('Ctrl Pts',(-2.70073315536695,-1.06847604194605,
11.373876973312));
#31999=CARTESIAN_POINT('Ctrl Pts',(-2.63039368071025,-0.794772684001488,
11.3584599905864));
#32000=CARTESIAN_POINT('Ctrl Pts',(-2.58777591208119,-0.636309800095707,
11.30525700494));
#32001=CARTESIAN_POINT('Ctrl Pts',(-2.52733729460958,-0.319434907277415,
11.2623369202654));
#32002=CARTESIAN_POINT('Ctrl Pts',(-2.50115862889893,-0.158333333333459,
11.228775100159));
#32003=CARTESIAN_POINT('Ctrl Pts',(-2.47384647649032,0.158333333333461,
11.2455582419395));
#32004=CARTESIAN_POINT('Ctrl Pts',(-2.47162318313642,0.319434907277424,
11.2964996838724));
#32005=CARTESIAN_POINT('Ctrl Pts',(-2.47864877038137,0.636309800095716,
11.3723908330216));
#32006=CARTESIAN_POINT('Ctrl Pts',(-2.49251384879947,0.794772684001477,
11.4427560053326));
#32007=CARTESIAN_POINT('Ctrl Pts',(-2.523862159101,1.06847604194665,11.4837092803596));
#32008=CARTESIAN_POINT('Ctrl Pts',(-2.54094944198943,1.18514270861408,11.489291196615));
#32009=CARTESIAN_POINT('Ctrl Pts',(-2.56155448580606,1.30000000000305,11.482727873835));
#32010=CARTESIAN_POINT('Ctrl Pts',(-2.76425102958308,-1.30000000000134,
11.3410995400671));
#32011=CARTESIAN_POINT('Ctrl Pts',(-2.7315536663465,-1.18514270861294,11.354163665401));
#32012=CARTESIAN_POINT('Ctrl Pts',(-2.69997469370202,-1.0684760419461,11.3567798466479));
#32013=CARTESIAN_POINT('Ctrl Pts',(-2.62960465554241,-0.794772684001521,
11.3386869077486));
#32014=CARTESIAN_POINT('Ctrl Pts',(-2.58647592708129,-0.636309800095733,
11.2861786420534));
#32015=CARTESIAN_POINT('Ctrl Pts',(-2.52571622593059,-0.319434907277429,
11.2433163704505));
#32016=CARTESIAN_POINT('Ctrl Pts',(-2.4992559721307,-0.158333333333466,
11.2106859315712));
#32017=CARTESIAN_POINT('Ctrl Pts',(-2.47225107092196,0.158333333333468,
11.2273600175278));
#32018=CARTESIAN_POINT('Ctrl Pts',(-2.47085041360708,0.319434907277437,
11.277165815717));
#32019=CARTESIAN_POINT('Ctrl Pts',(-2.47834670595677,0.636309800095743,
11.3529709421115));
#32020=CARTESIAN_POINT('Ctrl Pts',(-2.49207122318901,0.794772684001511,
11.422936527734));
#32021=CARTESIAN_POINT('Ctrl Pts',(-2.52353774137249,1.0684760419467,11.4665362245579));
#32022=CARTESIAN_POINT('Ctrl Pts',(-2.54068299263077,1.18514270861413,11.473932655612));
#32023=CARTESIAN_POINT('Ctrl Pts',(-2.56135280537506,1.3000000000031,11.469852824493));
#32024=CARTESIAN_POINT('Ctrl Pts',(-2.7642249389054,-1.30000000000134,11.3408092309998));
#32025=CARTESIAN_POINT('Ctrl Pts',(-2.73153255481153,-1.18514270861294,
11.3538131019925));
#32026=CARTESIAN_POINT('Ctrl Pts',(-2.69995590010922,-1.0684760419461,11.356385794704));
#32027=CARTESIAN_POINT('Ctrl Pts',(-2.62958506895419,-0.794772684001521,
11.3382311209536));
#32028=CARTESIAN_POINT('Ctrl Pts',(-2.5864454753899,-0.636309800095733,
11.2857385089783));
#32029=CARTESIAN_POINT('Ctrl Pts',(-2.5256784289746,-0.319434907277429,
11.2428775413335));
#32030=CARTESIAN_POINT('Ctrl Pts',(-2.49921092572217,-0.158333333333466,
11.2102689026167));
#32031=CARTESIAN_POINT('Ctrl Pts',(-2.47221323526919,0.158333333333468,
11.2269404266026));
#32032=CARTESIAN_POINT('Ctrl Pts',(-2.47083231477348,0.319434907277437,
11.2767197171004));
#32033=CARTESIAN_POINT('Ctrl Pts',(-2.47833989210166,0.636309800095743,
11.3525226913348));
#32034=CARTESIAN_POINT('Ctrl Pts',(-2.49206109302992,0.794772684001511,
11.4224790800824));
#32035=CARTESIAN_POINT('Ctrl Pts',(-2.52353047072471,1.0684760419467,11.4661398071924));
#32036=CARTESIAN_POINT('Ctrl Pts',(-2.54067711801391,1.18514270861413,11.4735780966765));
#32037=CARTESIAN_POINT('Ctrl Pts',(-2.56134848504356,1.3000000000031,11.4695555646682));
#32038=CARTESIAN_POINT('Ctrl Pts',(-2.76419881448468,-1.30000000000134,
11.3405189439279));
#32039=CARTESIAN_POINT('Ctrl Pts',(-2.73151148373164,-1.18514270861294,
11.3534625344107));
#32040=CARTESIAN_POINT('Ctrl Pts',(-2.69993718519305,-1.0684760419461,11.3559917257283));
#32041=CARTESIAN_POINT('Ctrl Pts',(-2.62956556622883,-0.794772684001521,
11.3377753181702));
#32042=CARTESIAN_POINT('Ctrl Pts',(-2.58641489207281,-0.636309800095733,
11.2852984453538));
#32043=CARTESIAN_POINT('Ctrl Pts',(-2.52564057129996,-0.319434907277429,
11.2424387508086));
#32044=CARTESIAN_POINT('Ctrl Pts',(-2.49916618353628,-0.158333333333466,
11.209851762818));
#32045=CARTESIAN_POINT('Ctrl Pts',(-2.47217564283986,0.158333333333468,
11.2265207446432));
#32046=CARTESIAN_POINT('Ctrl Pts',(-2.47081397410684,0.319434907277437,
11.2762737167092));
#32047=CARTESIAN_POINT('Ctrl Pts',(-2.47833276167054,0.636309800095743,
11.3520745692275));
#32048=CARTESIAN_POINT('Ctrl Pts',(-2.49205103357898,0.794772684001511,
11.4220216158322));
#32049=CARTESIAN_POINT('Ctrl Pts',(-2.52352329202462,1.0684760419467,11.465743363105));
#32050=CARTESIAN_POINT('Ctrl Pts',(-2.54067128140231,1.18514270861413,11.4732235296063));
#32051=CARTESIAN_POINT('Ctrl Pts',(-2.56134408563865,1.3000000000031,11.4692583382648));
#32052=CARTESIAN_POINT('Ctrl Pts',(-2.7641459971008,-1.30000000000134,11.3399386075426));
#32053=CARTESIAN_POINT('Ctrl Pts',(-2.73146844378851,-1.18514270861294,
11.3527617637104));
#32054=CARTESIAN_POINT('Ctrl Pts',(-2.69989867568352,-1.0684760419461,11.3552040201509));
#32055=CARTESIAN_POINT('Ctrl Pts',(-2.62952540129104,-0.794772684001521,
11.3368641660385));
#32056=CARTESIAN_POINT('Ctrl Pts',(-2.58635315650737,-0.636309800095733,
11.2844185273025));
#32057=CARTESIAN_POINT('Ctrl Pts',(-2.5255644397242,-0.319434907277429,
11.2415613108777));
#32058=CARTESIAN_POINT('Ctrl Pts',(-2.49907605021946,-0.158333333333466,
11.2090177185494));
#32059=CARTESIAN_POINT('Ctrl Pts',(-2.47209984924853,0.158333333333468,
11.2256815971009));
#32060=CARTESIAN_POINT('Ctrl Pts',(-2.47077678021634,0.319434907277437,
11.2753818890525));
#32061=CARTESIAN_POINT('Ctrl Pts',(-2.47831827749408,0.636309800095743,
11.3511783852092));
#32062=CARTESIAN_POINT('Ctrl Pts',(-2.49203108365346,0.794772684001511,
11.4211065984287));
#32063=CARTESIAN_POINT('Ctrl Pts',(-2.52350924912019,1.0684760419467,11.4649503359398));
#32064=CARTESIAN_POINT('Ctrl Pts',(-2.5406599129494,1.18514270861413,11.4725142638776));
#32065=CARTESIAN_POINT('Ctrl Pts',(-2.5613355091582,1.3000000000031,11.4686637903551));
#32066=CARTESIAN_POINT('Ctrl Pts',(-2.76402931431754,-1.30000000000134,
11.338682172166));
#32067=CARTESIAN_POINT('Ctrl Pts',(-2.73137172231167,-1.18514270861294,
11.3512448816346));
#32068=CARTESIAN_POINT('Ctrl Pts',(-2.69981107687792,-1.0684760419461,11.3534990541753));
#32069=CARTESIAN_POINT('Ctrl Pts',(-2.62943383826546,-0.794772684001521,
11.3348918611708));
#32070=CARTESIAN_POINT('Ctrl Pts',(-2.58621659385465,-0.636309800095733,
11.2825131577169));
#32071=CARTESIAN_POINT('Ctrl Pts',(-2.52539779351564,-0.319434907277428,
11.2396608293271));
#32072=CARTESIAN_POINT('Ctrl Pts',(-2.49887984433881,-0.158333333333466,
11.2072109433244));
#32073=CARTESIAN_POINT('Ctrl Pts',(-2.47193459901702,0.158333333333468,
11.2238637817233));
#32074=CARTESIAN_POINT('Ctrl Pts',(-2.47069320506725,0.319434907277437,
11.2734506758837));
#32075=CARTESIAN_POINT('Ctrl Pts',(-2.47828473941927,0.636309800095743,
11.3492374181108));
#32076=CARTESIAN_POINT('Ctrl Pts',(-2.49198924223239,0.794772684001511,
11.4191234920776));
#32077=CARTESIAN_POINT('Ctrl Pts',(-2.52348083005594,1.0684760419467,11.4632313171438));
#32078=CARTESIAN_POINT('Ctrl Pts',(-2.5406369264164,1.18514270861413,11.4709768715931));
#32079=CARTESIAN_POINT('Ctrl Pts',(-2.5613175776468,1.3000000000031,11.4673753373765));
#32080=CARTESIAN_POINT('Ctrl Pts',(-2.76384106606497,-1.30000000000133,
11.3367528528731));
#32081=CARTESIAN_POINT('Ctrl Pts',(-2.73120756008998,-1.18514270861294,
11.3489175947374));
#32082=CARTESIAN_POINT('Ctrl Pts',(-2.69965713366755,-1.0684760419461,11.3508839572717));
#32083=CARTESIAN_POINT('Ctrl Pts',(-2.62927146742631,-0.794772684001519,
11.3318663516645));
#32084=CARTESIAN_POINT('Ctrl Pts',(-2.58599385923292,-0.636309800095732,
11.2795868603255));
#32085=CARTESIAN_POINT('Ctrl Pts',(-2.52513457515162,-0.319434907277428,
11.2367395707489));
#32086=CARTESIAN_POINT('Ctrl Pts',(-2.49857540848214,-0.158333333333466,
11.2044321215613));
#32087=CARTESIAN_POINT('Ctrl Pts',(-2.47167760241594,0.158333333333468,
11.2210679345774));
#32088=CARTESIAN_POINT('Ctrl Pts',(-2.47055269207584,0.319434907277436,
11.2704838638599));
#32089=CARTESIAN_POINT('Ctrl Pts',(-2.47822465920485,0.636309800095742,
11.3462543179259));
#32090=CARTESIAN_POINT('Ctrl Pts',(-2.49193191562207,0.79477268400151,11.416069748549));
#32091=CARTESIAN_POINT('Ctrl Pts',(-2.52344696005734,1.0684760419467,11.4605828404811));
#32092=CARTESIAN_POINT('Ctrl Pts',(-2.54060989083201,1.18514270861413,11.4686084087007));
#32093=CARTESIAN_POINT('Ctrl Pts',(-2.56129405739276,1.3000000000031,11.465391477015));
#32094=CARTESIAN_POINT('Ctrl Pts',(-2.76360061952686,-1.30000000000133,
11.3344435152267));
#32095=CARTESIAN_POINT('Ctrl Pts',(-2.73097799067002,-1.18514270861294,
11.3461382704645));
#32096=CARTESIAN_POINT('Ctrl Pts',(-2.69942932223466,-1.06847604194609,
11.3477636570441));
#32097=CARTESIAN_POINT('Ctrl Pts',(-2.62902665027813,-0.794772684001518,
11.32825636923));
#32098=CARTESIAN_POINT('Ctrl Pts',(-2.58569889268955,-0.636309800095731,
11.2760863776604));
#32099=CARTESIAN_POINT('Ctrl Pts',(-2.5248079778311,-0.319434907277428,
11.2332380172859));
#32100=CARTESIAN_POINT('Ctrl Pts',(-2.49821542392339,-0.158333333333465,
11.2010950925747));
#32101=CARTESIAN_POINT('Ctrl Pts',(-2.47137359693892,0.158333333333467,
11.2177106241918));
#32102=CARTESIAN_POINT('Ctrl Pts',(-2.47035915085401,0.319434907277435,
11.2669326531755));
#32103=CARTESIAN_POINT('Ctrl Pts',(-2.47813379914407,0.636309800095741,
11.3426813909753));
#32104=CARTESIAN_POINT('Ctrl Pts',(-2.49188611954923,0.794772684001508,
11.4123964622437));
#32105=CARTESIAN_POINT('Ctrl Pts',(-2.52343468975773,1.06847604194669,11.4573939376935));
#32106=CARTESIAN_POINT('Ctrl Pts',(-2.54060061621157,1.18514270861413,11.4657574988284));
#32107=CARTESIAN_POINT('Ctrl Pts',(-2.56127626206568,1.30000000000309,11.4630068812969));
#32108=CARTESIAN_POINT('Ctrl Pts',(-2.76309350386812,-1.30000000000133,
11.3298351473961));
#32109=CARTESIAN_POINT('Ctrl Pts',(-2.73045517154361,-1.18514270861294,
11.3406057267502));
#32110=CARTESIAN_POINT('Ctrl Pts',(-2.69888781493744,-1.06847604194609,
11.3415585026455));
#32111=CARTESIAN_POINT('Ctrl Pts',(-2.62843507430646,-0.794772684001515,
11.3210785155308));
#32112=CARTESIAN_POINT('Ctrl Pts',(-2.58504928387606,-0.636309800095729,
11.2691093968105));
#32113=CARTESIAN_POINT('Ctrl Pts',(-2.52413061301386,-0.319434907277426,
11.2262440409975));
#32114=CARTESIAN_POINT('Ctrl Pts',(-2.49750907749174,-0.158333333333465,
11.1944150527455));
#32115=CARTESIAN_POINT('Ctrl Pts',(-2.47077890822903,0.158333333333467,
11.2109896331354));
#32116=CARTESIAN_POINT('Ctrl Pts',(-2.46992453282581,0.319434907277434,
11.2598472153409));
#32117=CARTESIAN_POINT('Ctrl Pts',(-2.47791479560751,0.636309800095739,
11.3355490050596));
#32118=CARTESIAN_POINT('Ctrl Pts',(-2.49183703931886,0.794772684001506,
11.4050337736974));
#32119=CARTESIAN_POINT('Ctrl Pts',(-2.52346511529109,1.06847604194669,11.4509954167954));
#32120=CARTESIAN_POINT('Ctrl Pts',(-2.5406286591004,1.18514270861412,11.4600380519337));
#32121=CARTESIAN_POINT('Ctrl Pts',(-2.56126512456632,1.30000000000309,11.4582282299596));
#32122=CARTESIAN_POINT('Ctrl Pts',(-2.76222770959521,-1.30000000000129,
11.3229634616086));
#32123=CARTESIAN_POINT('Ctrl Pts',(-2.7293887323951,-1.1851427086129,11.3324232623684));
#32124=CARTESIAN_POINT('Ctrl Pts',(-2.69768919111629,-1.06847604194606,
11.332411528792));
#32125=CARTESIAN_POINT('Ctrl Pts',(-2.62708923421229,-0.794772684001494,
11.3105032827926));
#32126=CARTESIAN_POINT('Ctrl Pts',(-2.58382313700693,-0.636309800095712,
11.2587466220022));
#32127=CARTESIAN_POINT('Ctrl Pts',(-2.52303388877888,-0.319434907277418,
11.2157845139037));
#32128=CARTESIAN_POINT('Ctrl Pts',(-2.49654983034628,-0.158333333333461,
11.1843543637192));
#32129=CARTESIAN_POINT('Ctrl Pts',(-2.46997662326551,0.158333333333463,
11.2008695548721));
#32130=CARTESIAN_POINT('Ctrl Pts',(-2.46905368135563,0.319434907277427,
11.2492992472544));
#32131=CARTESIAN_POINT('Ctrl Pts',(-2.47741359693355,0.636309800095722,
11.324915022394));
#32132=CARTESIAN_POINT('Ctrl Pts',(-2.49199886919655,0.794772684001485,
11.39390247055));
#32133=CARTESIAN_POINT('Ctrl Pts',(-2.52379078168629,1.06847604194666,11.4412940015727));
#32134=CARTESIAN_POINT('Ctrl Pts',(-2.5408960429585,1.18514270861409,11.4513755911155));
#32135=CARTESIAN_POINT('Ctrl Pts',(-2.56134502459252,1.30000000000306,11.4510247324508));
#32136=CARTESIAN_POINT('Ctrl Pts',(-2.76108397909559,-1.30000000000128,
11.3137922130238));
#32137=CARTESIAN_POINT('Ctrl Pts',(-2.72796787036885,-1.1851427086129,11.3215064835911));
#32138=CARTESIAN_POINT('Ctrl Pts',(-2.696073175759,-1.06847604194605,11.3202154940208));
#32139=CARTESIAN_POINT('Ctrl Pts',(-2.62521176165157,-0.794772684001488,
11.2964290974375));
#32140=CARTESIAN_POINT('Ctrl Pts',(-2.58200923659833,-0.636309800095708,
11.2449978338617));
#32141=CARTESIAN_POINT('Ctrl Pts',(-2.52134186084768,-0.319434907277416,
11.2019287017981));
#32142=CARTESIAN_POINT('Ctrl Pts',(-2.4950486259072,-0.15833333333346,11.1710284212635));
#32143=CARTESIAN_POINT('Ctrl Pts',(-2.46872146847482,0.158333333333462,
11.1874470610037));
#32144=CARTESIAN_POINT('Ctrl Pts',(-2.46780018656564,0.319434907277424,
11.2352637031698));
#32145=CARTESIAN_POINT('Ctrl Pts',(-2.47664852548579,0.636309800095717,
11.3107625985471));
#32146=CARTESIAN_POINT('Ctrl Pts',(-2.49195811589145,0.79477268400148,11.3791486794266));
#32147=CARTESIAN_POINT('Ctrl Pts',(-2.52402251623276,1.06847604194666,11.4284269609544));
#32148=CARTESIAN_POINT('Ctrl Pts',(-2.54111681522227,1.18514270861408,11.4398691438539));
#32149=CARTESIAN_POINT('Ctrl Pts',(-2.56142592239663,1.30000000000305,11.4414227675198));
#32150=CARTESIAN_POINT('Ctrl Pts',(-2.75980118259079,-1.30000000000125,
11.3014623485093));
#32151=CARTESIAN_POINT('Ctrl Pts',(-2.72668885406917,-1.18514270861286,
11.3066879411516));
#32152=CARTESIAN_POINT('Ctrl Pts',(-2.69474188830154,-1.06847604194603,
11.3036011429695));
#32153=CARTESIAN_POINT('Ctrl Pts',(-2.62363022750143,-0.794772684001467,
11.2772667359641));
#32154=CARTESIAN_POINT('Ctrl Pts',(-2.58003207349033,-0.63630980009569,
11.2264773244685));
#32155=CARTESIAN_POINT('Ctrl Pts',(-2.51901724331341,-0.319434907277407,
11.1834792920214));
#32156=CARTESIAN_POINT('Ctrl Pts',(-2.49240144992841,-0.158333333333455,
11.1535220447443));
#32157=CARTESIAN_POINT('Ctrl Pts',(-2.46637898161969,0.158333333333457,
11.1698229438921));
#32158=CARTESIAN_POINT('Ctrl Pts',(-2.46624982092312,0.319434907277415,
11.2165057451712));
#32159=CARTESIAN_POINT('Ctrl Pts',(-2.47573040833367,0.6363098000957,11.2918425441167));
#32160=CARTESIAN_POINT('Ctrl Pts',(-2.49117635189392,0.794772684001457,
11.3597287085015));
#32161=CARTESIAN_POINT('Ctrl Pts',(-2.52352169135959,1.06847604194663,11.4115569527867));
#32162=CARTESIAN_POINT('Ctrl Pts',(-2.54071050140298,1.18514270861405,11.4247776534393));
#32163=CARTESIAN_POINT('Ctrl Pts',(-2.56108702254797,1.30000000000301,11.4287845282192));
#32164=CARTESIAN_POINT('Ctrl Pts',(-2.75825795813088,-1.30000000000116,
11.2860117341614));
#32165=CARTESIAN_POINT('Ctrl Pts',(-2.72513502484691,-1.18514270861278,
11.2881298178769));
#32166=CARTESIAN_POINT('Ctrl Pts',(-2.69312058453786,-1.06847604194595,
11.2827970892231));
#32167=CARTESIAN_POINT('Ctrl Pts',(-2.62172166348246,-0.794772684001413,
11.2532645521214));
#32168=CARTESIAN_POINT('Ctrl Pts',(-2.57769388327834,-0.636309800095648,
11.2032509010327));
#32169=CARTESIAN_POINT('Ctrl Pts',(-2.51630763113037,-0.319434907277386,
11.1603190736043));
#32170=CARTESIAN_POINT('Ctrl Pts',(-2.48938193806615,-0.158333333333445,
11.1315094292022));
#32171=CARTESIAN_POINT('Ctrl Pts',(-2.46364866959619,0.158333333333447,
11.1477013127868));
#32172=CARTESIAN_POINT('Ctrl Pts',(-2.46417035515022,0.319434907277394,
11.1930962285957));
#32173=CARTESIAN_POINT('Ctrl Pts',(-2.47450603941183,0.636309800095658,
11.268208454363));
#32174=CARTESIAN_POINT('Ctrl Pts',(-2.49057818975681,0.794772684001404,
11.3353018937305));
#32175=CARTESIAN_POINT('Ctrl Pts',(-2.52343815187733,1.06847604194656,11.3902517119039));
#32176=CARTESIAN_POINT('Ctrl Pts',(-2.54075694726679,1.18514270861397,11.4056872918243));
#32177=CARTESIAN_POINT('Ctrl Pts',(-2.5611706780253,1.30000000000293,11.412772711469));
#32178=CARTESIAN_POINT('Ctrl Pts',(-2.75493542354467,-1.30000000000102,
11.2616597751113));
#32179=CARTESIAN_POINT('Ctrl Pts',(-2.72115084070019,-1.18514270861265,
11.2590784416815));
#32180=CARTESIAN_POINT('Ctrl Pts',(-2.68860134985113,-1.06847604194584,
11.2503326796887));
#32181=CARTESIAN_POINT('Ctrl Pts',(-2.61625882407524,-0.794772684001327,
11.2158871567315));
#32182=CARTESIAN_POINT('Ctrl Pts',(-2.57180751599066,-0.636309800095576,
11.1670064104961));
#32183=CARTESIAN_POINT('Ctrl Pts',(-2.5104314595887,-0.319434907277349,
11.1239157330979));
#32184=CARTESIAN_POINT('Ctrl Pts',(-2.48391525623262,-0.158333333333427,
11.0965453605644));
#32185=CARTESIAN_POINT('Ctrl Pts',(-2.45918556724436,0.158333333333429,
11.1123214520548));
#32186=CARTESIAN_POINT('Ctrl Pts',(-2.46083663420726,0.319434907277358,
11.1556249158299));
#32187=CARTESIAN_POINT('Ctrl Pts',(-2.47211599134814,0.636309800095586,
11.2305305584888));
#32188=CARTESIAN_POINT('Ctrl Pts',(-2.48811501046006,0.794772684001314,
11.2967506895527));
#32189=CARTESIAN_POINT('Ctrl Pts',(-2.52146216625009,1.06847604194643,11.356844218504));
#32190=CARTESIAN_POINT('Ctrl Pts',(-2.53902007409783,1.18514270861384,11.3758292365511));
#32191=CARTESIAN_POINT('Ctrl Pts',(-2.55970114168565,1.30000000000278,11.3877870106468));
#32192=CARTESIAN_POINT('Ctrl Pts',(-2.7518637748275,-1.30000000000087,11.2371614514306));
#32193=CARTESIAN_POINT('Ctrl Pts',(-2.71741456579904,-1.18514270861252,
11.2298815778422));
#32194=CARTESIAN_POINT('Ctrl Pts',(-2.6843818772594,-1.06847604194571,11.2176986913577));
#32195=CARTESIAN_POINT('Ctrl Pts',(-2.6113422042693,-0.794772684001233,
11.1782268457664));
#32196=CARTESIAN_POINT('Ctrl Pts',(-2.56707069312648,-0.636309800095504,
11.1302032988742));
#32197=CARTESIAN_POINT('Ctrl Pts',(-2.50562348786956,-0.319434907277313,
11.0869902458595));
#32198=CARTESIAN_POINT('Ctrl Pts',(-2.47909119587275,-0.158333333333409,
11.0612684020365));
#32199=CARTESIAN_POINT('Ctrl Pts',(-2.45452022313769,0.15833333333341,11.0769832866117));
#32200=CARTESIAN_POINT('Ctrl Pts',(-2.45612570166382,0.31943490727732,11.1186569966856));
#32201=CARTESIAN_POINT('Ctrl Pts',(-2.46824842658526,0.636309800095512,
11.1933974234602));
#32202=CARTESIAN_POINT('Ctrl Pts',(-2.48526252158171,0.794772684001224,
11.2583122288779));
#32203=CARTESIAN_POINT('Ctrl Pts',(-2.51983978146043,1.06847604194631,11.3232510423267));
#32204=CARTESIAN_POINT('Ctrl Pts',(-2.53792061586775,1.1851427086137,11.3456703913735));
#32205=CARTESIAN_POINT('Ctrl Pts',(-2.55911507009457,1.30000000000263,11.3623994833453));
#32206=CARTESIAN_POINT('Ctrl Pts',(-2.74834939782952,-1.30000000000082,
11.2128663351783));
#32207=CARTESIAN_POINT('Ctrl Pts',(-2.71340728818996,-1.18514270861247,
11.2007884395455));
#32208=CARTESIAN_POINT('Ctrl Pts',(-2.67981955403308,-1.06847604194567,
11.185186462444));
#32209=CARTESIAN_POINT('Ctrl Pts',(-2.60535404723434,-0.794772684001202,
11.1410014409916));
#32210=CARTESIAN_POINT('Ctrl Pts',(-2.55935977635548,-0.636309800095478,
11.0947175057529));
#32211=CARTESIAN_POINT('Ctrl Pts',(-2.49749108140857,-0.3194349072773,11.0515352465719));
#32212=CARTESIAN_POINT('Ctrl Pts',(-2.47195891583274,-0.158333333333402,
11.0269832733524));
#32213=CARTESIAN_POINT('Ctrl Pts',(-2.44847039799177,0.158333333333404,
11.0422134181132));
#32214=CARTESIAN_POINT('Ctrl Pts',(-2.45064429522044,0.319434907277308,
11.0819845588382));
#32215=CARTESIAN_POINT('Ctrl Pts',(-2.46440326171409,0.636309800095487,
11.1562118861686));
#32216=CARTESIAN_POINT('Ctrl Pts',(-2.48309797691221,0.794772684001192,
11.219540481514));
#32217=CARTESIAN_POINT('Ctrl Pts',(-2.51859141008612,1.06847604194627,11.2894664432714));
#32218=CARTESIAN_POINT('Ctrl Pts',(-2.53678252725346,1.18514270861366,11.3155017071016));
#32219=CARTESIAN_POINT('Ctrl Pts',(-2.55780096952842,1.30000000000258,11.3373038769293));
#32220=CARTESIAN_POINT('Ctrl Pts',(-2.74573850760591,-1.30000000000075,
11.194591028711));
#32221=CARTESIAN_POINT('Ctrl Pts',(-2.70959292316076,-1.18514270861241,
11.1793106824202));
#32222=CARTESIAN_POINT('Ctrl Pts',(-2.67524735232435,-1.06847604194562,
11.1613097598791));
#32223=CARTESIAN_POINT('Ctrl Pts',(-2.60006060441201,-0.794772684001161,
11.1134389523493));
#32224=CARTESIAN_POINT('Ctrl Pts',(-2.5555787040635,-0.636309800095446,
11.0671560420463));
#32225=CARTESIAN_POINT('Ctrl Pts',(-2.49364032028975,-0.319434907277284,
11.0238878071138));
#32226=CARTESIAN_POINT('Ctrl Pts',(-2.46702495262325,-0.158333333333394,
11.0010760834182));
#32227=CARTESIAN_POINT('Ctrl Pts',(-2.44338172711316,0.158333333333396,
11.0163803880387));
#32228=CARTESIAN_POINT('Ctrl Pts',(-2.44615547867357,0.319434907277292,
11.0546354570378));
#32229=CARTESIAN_POINT('Ctrl Pts',(-2.46033842181148,0.636309800095455,
11.1287942426758));
#32230=CARTESIAN_POINT('Ctrl Pts',(-2.47871468054937,0.794772684001151,
11.1915537053767));
#32231=CARTESIAN_POINT('Ctrl Pts',(-2.51532939498739,1.06847604194622,11.2650365289296));
#32232=CARTESIAN_POINT('Ctrl Pts',(-2.53427276633016,1.1851427086136,11.2935121246627));
#32233=CARTESIAN_POINT('Ctrl Pts',(-2.55631035584431,1.30000000000251,11.3186553246197));
#32234=CARTESIAN_POINT('Ctrl Pts',(-2.74194313468282,-1.30000000000071,
11.1769309522021));
#32235=CARTESIAN_POINT('Ctrl Pts',(-2.70552266600435,-1.18514270861237,
11.1579854994345));
#32236=CARTESIAN_POINT('Ctrl Pts',(-2.67079715330622,-1.06847604194558,
11.1373887609292));
#32237=CARTESIAN_POINT('Ctrl Pts',(-2.59448995954793,-0.794772684001138,
11.0859913742256));
#32238=CARTESIAN_POINT('Ctrl Pts',(-2.54840340341899,-0.636309800095426,
11.0411814441527));
#32239=CARTESIAN_POINT('Ctrl Pts',(-2.48605786049262,-0.319434907277274,
10.9979792561164));
#32240=CARTESIAN_POINT('Ctrl Pts',(-2.46005105058619,-0.15833333333339,
10.9761034409434));
#32241=CARTESIAN_POINT('Ctrl Pts',(-2.43778685380937,0.158333333333391,
10.9907711091253));
#32242=CARTESIAN_POINT('Ctrl Pts',(-2.44206476862543,0.319434907277283,
11.0270908601629));
#32243=CARTESIAN_POINT('Ctrl Pts',(-2.45796937480046,0.636309800095436,
11.1006257587997));
#32244=CARTESIAN_POINT('Ctrl Pts',(-2.47728146775959,0.794772684001127,
11.1623393375586));
#32245=CARTESIAN_POINT('Ctrl Pts',(-2.51438276944182,1.06847604194618,11.2396575410887));
#32246=CARTESIAN_POINT('Ctrl Pts',(-2.53329203241781,1.18514270861356,11.2709028445636));
#32247=CARTESIAN_POINT('Ctrl Pts',(-2.55505077961023,1.30000000000247,11.2999252661269));
#32248=CARTESIAN_POINT('Ctrl Pts',(-2.73966116432271,-1.30000000000066,
11.158478942661));
#32249=CARTESIAN_POINT('Ctrl Pts',(-2.70242984548913,-1.18514270861233,
11.1361367519602));
#32250=CARTESIAN_POINT('Ctrl Pts',(-2.66706342795359,-1.06847604194554,
11.1130797469362));
#32251=CARTESIAN_POINT('Ctrl Pts',(-2.58966822348966,-0.794772684001105,
11.058162088708));
#32252=CARTESIAN_POINT('Ctrl Pts',(-2.54340702433661,-0.636309800095402,
11.0141542266524));
#32253=CARTESIAN_POINT('Ctrl Pts',(-2.48069951827734,-0.319434907277262,
10.9710064276511));
#32254=CARTESIAN_POINT('Ctrl Pts',(-2.45480737171722,-0.158333333333383,
10.9503166592489));
#32255=CARTESIAN_POINT('Ctrl Pts',(-2.43239017645839,0.158333333333385,
10.9650437434));
#32256=CARTESIAN_POINT('Ctrl Pts',(-2.43611575138395,0.319434907277269,
11.0003481142894));
#32257=CARTESIAN_POINT('Ctrl Pts',(-2.45265054251548,0.63630980009541,11.0737230403714));
#32258=CARTESIAN_POINT('Ctrl Pts',(-2.47305803943563,0.794772684001096,
11.1342548378043));
#32259=CARTESIAN_POINT('Ctrl Pts',(-2.51172448148075,1.06847604194614,11.2149405437268));
#32260=CARTESIAN_POINT('Ctrl Pts',(-2.53138096354022,1.18514270861351,11.2486305072769));
#32261=CARTESIAN_POINT('Ctrl Pts',(-2.55395665763067,1.30000000000242,11.2810845819833));
#32262=CARTESIAN_POINT('Ctrl Pts',(-2.73574909450234,-1.30000000000064,
11.144116794413));
#32263=CARTESIAN_POINT('Ctrl Pts',(-2.69776719162632,-1.18514270861231,
11.1189659997614));
#32264=CARTESIAN_POINT('Ctrl Pts',(-2.66186056462313,-1.06847604194552,
11.0938501329944));
#32265=CARTESIAN_POINT('Ctrl Pts',(-2.58370337557335,-0.79477268400109,
11.0359081467518));
#32266=CARTESIAN_POINT('Ctrl Pts',(-2.53770217468129,-0.63630980009539,
10.9923659965246));
#32267=CARTESIAN_POINT('Ctrl Pts',(-2.47491433420959,-0.319434907277257,
10.9491493418208));
#32268=CARTESIAN_POINT('Ctrl Pts',(-2.44882343493709,-0.158333333333381,
10.9295894777583));
#32269=CARTESIAN_POINT('Ctrl Pts',(-2.42681406751302,0.158333333333383,
10.9441153090178));
#32270=CARTESIAN_POINT('Ctrl Pts',(-2.43113598017231,0.319434907277265,
10.9780824257723));
#32271=CARTESIAN_POINT('Ctrl Pts',(-2.44860268552448,0.6363098000954,11.0511286888608));
#32272=CARTESIAN_POINT('Ctrl Pts',(-2.46954364071995,0.794772684001082,
11.1108472790484));
#32273=CARTESIAN_POINT('Ctrl Pts',(-2.50916003180598,1.06847604194612,11.1944910794941));
#32274=CARTESIAN_POINT('Ctrl Pts',(-2.52924123422387,1.18514270861349,11.2303034178588));
#32275=CARTESIAN_POINT('Ctrl Pts',(-2.55225517129041,1.3000000000024,11.2657217926835));
#32276=CARTESIAN_POINT('Ctrl Pts',(-2.73421733091288,-1.30000000000063,
11.1318054961784));
#32277=CARTESIAN_POINT('Ctrl Pts',(-2.69568219536503,-1.1851427086123,11.1043904407161));
#32278=CARTESIAN_POINT('Ctrl Pts',(-2.65928523630985,-1.06847604194552,
11.0776608026002));
#32279=CARTESIAN_POINT('Ctrl Pts',(-2.58014059514451,-0.794772684001087,
11.0174934424942));
#32280=CARTESIAN_POINT('Ctrl Pts',(-2.53361645527697,-0.636309800095386,
10.9746833759411));
#32281=CARTESIAN_POINT('Ctrl Pts',(-2.47029199881909,-0.319434907277254,
10.9316507257101));
#32282=CARTESIAN_POINT('Ctrl Pts',(-2.44402307019611,-0.15833333333338,
10.9130133743054));
#32283=CARTESIAN_POINT('Ctrl Pts',(-2.42231413633528,0.158333333333381,
10.92738984692));
#32284=CARTESIAN_POINT('Ctrl Pts',(-2.42722284933438,0.319434907277263,
10.9602169003356));
#32285=CARTESIAN_POINT('Ctrl Pts',(-2.4456174566727,0.636309800095396,11.032913828414));
#32286=CARTESIAN_POINT('Ctrl Pts',(-2.4673458530226,0.794772684001076,11.0918301551621));
#32287=CARTESIAN_POINT('Ctrl Pts',(-2.50756957285321,1.06847604194612,11.1779141208763));
#32288=CARTESIAN_POINT('Ctrl Pts',(-2.52780280322549,1.18514270861349,11.2155104846413));
#32289=CARTESIAN_POINT('Ctrl Pts',(-2.55085790609104,1.30000000000239,11.2534406531388));
#32290=CARTESIAN_POINT('Ctrl Pts',(-2.73052114637815,-1.3000000000006,11.1140598974807));
#32291=CARTESIAN_POINT('Ctrl Pts',(-2.69121203817809,-1.18514270861227,
11.0832189188306));
#32292=CARTESIAN_POINT('Ctrl Pts',(-2.65417480751361,-1.06847604194549,
11.0540196347119));
#32293=CARTESIAN_POINT('Ctrl Pts',(-2.57385988700081,-0.794772684001062,
10.9903560898885));
#32294=CARTESIAN_POINT('Ctrl Pts',(-2.52683960535164,-0.636309800095369,
10.9485012201944));
#32295=CARTESIAN_POINT('Ctrl Pts',(-2.46323476709751,-0.319434907277246,
10.905476185748));
#32296=CARTESIAN_POINT('Ctrl Pts',(-2.43733245527519,-0.158333333333376,
10.8878982928609));
#32297=CARTESIAN_POINT('Ctrl Pts',(-2.41596612209797,0.158333333333377,
10.9020966854773));
#32298=CARTESIAN_POINT('Ctrl Pts',(-2.42094900457107,0.319434907277255,
10.9336232753893));
#32299=CARTESIAN_POINT('Ctrl Pts',(-2.44012184965078,0.63630980009538,11.0060780252185));
#32300=CARTESIAN_POINT('Ctrl Pts',(-2.46228533804278,0.794772684001055,
11.0640914506206));
#32301=CARTESIAN_POINT('Ctrl Pts',(-2.50412229577207,1.06847604194609,11.1535161961697));
#32302=CARTESIAN_POINT('Ctrl Pts',(-2.52524774255897,1.18514270861345,11.1934937403211));
#32303=CARTESIAN_POINT('Ctrl Pts',(-2.54938896734375,1.30000000000236,11.234740169789));
#32304=CARTESIAN_POINT('Ctrl Pts',(-2.72618669292035,-1.30000000000054,
11.090057041695));
#32305=CARTESIAN_POINT('Ctrl Pts',(-2.6852794327094,-1.18514270861222,11.0549236063513));
#32306=CARTESIAN_POINT('Ctrl Pts',(-2.64695621782421,-1.06847604194544,
11.0226451010771));
#32307=CARTESIAN_POINT('Ctrl Pts',(-2.56439158654555,-0.794772684001033,
10.954670756188));
#32308=CARTESIAN_POINT('Ctrl Pts',(-2.51675264711951,-0.636309800095345,
10.9140945200914));
#32309=CARTESIAN_POINT('Ctrl Pts',(-2.45250838794689,-0.319434907277234,
10.8712261373627));
#32310=CARTESIAN_POINT('Ctrl Pts',(-2.42678965977914,-0.15833333333337,
10.8552187665213));
#32311=CARTESIAN_POINT('Ctrl Pts',(-2.40611359010731,0.158333333333371,
10.8690496021633));
#32312=CARTESIAN_POINT('Ctrl Pts',(-2.41159051383702,0.319434907277242,
10.8985976683053));
#32313=CARTESIAN_POINT('Ctrl Pts',(-2.43283454080145,0.636309800095355,
10.9702294623685));
#32314=CARTESIAN_POINT('Ctrl Pts',(-2.45740069161927,0.794772684001025,
11.0262315201112));
#32315=CARTESIAN_POINT('Ctrl Pts',(-2.50098392074559,1.06847604194605,11.120292932966));
#32316=CARTESIAN_POINT('Ctrl Pts',(-2.52257860080518,1.18514270861341,11.1637706734171));
#32317=CARTESIAN_POINT('Ctrl Pts',(-2.54690239595331,1.30000000000231,11.2100104540132));
#32318=CARTESIAN_POINT('Ctrl Pts',(-2.72020047827003,-1.30000000000049,
11.0669081106694));
#32319=CARTESIAN_POINT('Ctrl Pts',(-2.67790604734494,-1.18514270861218,
11.0273779174215));
#32320=CARTESIAN_POINT('Ctrl Pts',(-2.63846510872675,-1.06847604194541,
10.9919366357417));
#32321=CARTESIAN_POINT('Ctrl Pts',(-2.55394078845416,-0.794772684001004,
10.9195063887635));
#32322=CARTESIAN_POINT('Ctrl Pts',(-2.50570797655504,-0.636309800095321,
10.8801953547377));
#32323=CARTESIAN_POINT('Ctrl Pts',(-2.44098964317585,-0.319434907277222,
10.8373965721291));
#32324=CARTESIAN_POINT('Ctrl Pts',(-2.41563858417114,-0.158333333333364,
10.8228649247209));
#32325=CARTESIAN_POINT('Ctrl Pts',(-2.39557038649268,0.158333333333365,
10.8363600501206));
#32326=CARTESIAN_POINT('Ctrl Pts',(-2.40157548437834,0.31943490727723,10.8639311832623));
#32327=CARTESIAN_POINT('Ctrl Pts',(-2.42394520017597,0.636309800095331,
10.9351466698216));
#32328=CARTESIAN_POINT('Ctrl Pts',(-2.44870206327488,0.794772684000997,
10.9900901533294));
#32329=CARTESIAN_POINT('Ctrl Pts',(-2.49448776363949,1.06847604194601,11.0885620182733));
#32330=CARTESIAN_POINT('Ctrl Pts',(-2.51737260574984,1.18514270861336,11.1351670001206));
#32331=CARTESIAN_POINT('Ctrl Pts',(-2.54332335681004,1.30000000000226,11.1857521422231));
#32332=CARTESIAN_POINT('Ctrl Pts',(-2.71488010558268,-1.30000000000047,
11.0433879560159));
#32333=CARTESIAN_POINT('Ctrl Pts',(-2.67119661166076,-1.18514270861215,
10.9994440491979));
#32334=CARTESIAN_POINT('Ctrl Pts',(-2.63052212327521,-1.06847604194538,
10.9608907478844));
#32335=CARTESIAN_POINT('Ctrl Pts',(-2.54350732293959,-0.794772684000988,
10.884278286391));
#32336=CARTESIAN_POINT('Ctrl Pts',(-2.49386695147061,-0.636309800095306,
10.8466866414759));
#32337=CARTESIAN_POINT('Ctrl Pts',(-2.42793766345227,-0.319434907277213,
10.8043600799878));
#32338=CARTESIAN_POINT('Ctrl Pts',(-2.40244873322788,-0.15833333333336,
10.7915861754419));
#32339=CARTESIAN_POINT('Ctrl Pts',(-2.38323040728465,0.158333333333362,
10.8046011359007));
#32340=CARTESIAN_POINT('Ctrl Pts',(-2.39059918924259,0.319434907277223,
10.829691026249));
#32341=CARTESIAN_POINT('Ctrl Pts',(-2.41514522222375,0.636309800095316,
10.8999518861306));
#32342=CARTESIAN_POINT('Ctrl Pts',(-2.44122298675669,0.794772684000977,
10.9533434101576));
#32343=CARTESIAN_POINT('Ctrl Pts',(-2.48924678398141,1.06847604194598,11.0562202485803));
#32344=CARTESIAN_POINT('Ctrl Pts',(-2.51312174160371,1.18514270861333,11.1060979118114));
#32345=CARTESIAN_POINT('Ctrl Pts',(-2.54008393448674,1.30000000000222,11.1613216668828));
#32346=CARTESIAN_POINT('Ctrl Pts',(-2.70911402584229,-1.30000000000036,
11.0234204248473));
#32347=CARTESIAN_POINT('Ctrl Pts',(-2.66373005632073,-1.18514270861205,
10.9759171644225));
#32348=CARTESIAN_POINT('Ctrl Pts',(-2.62175498217934,-1.06847604194529,
10.9347927600077));
#32349=CARTESIAN_POINT('Ctrl Pts',(-2.53265939410329,-0.794772684000918,
10.8545235923695));
#32350=CARTESIAN_POINT('Ctrl Pts',(-2.48305062346186,-0.636309800095253,
10.8177669943221));
#32351=CARTESIAN_POINT('Ctrl Pts',(-2.41646836772196,-0.319434907277188,
10.7756498564267));
#32352=CARTESIAN_POINT('Ctrl Pts',(-2.3906874974646,-0.158333333333347,
10.7645045281972));
#32353=CARTESIAN_POINT('Ctrl Pts',(-2.37167048785909,0.158333333333348,
10.7773744834247));
#32354=CARTESIAN_POINT('Ctrl Pts',(-2.37915028861769,0.319434907277195,
10.8008558590621));
#32355=CARTESIAN_POINT('Ctrl Pts',(-2.40553794661324,0.636309800095263,
10.8702757008739));
#32356=CARTESIAN_POINT('Ctrl Pts',(-2.43364132787521,0.794772684000912,
10.9218037896078));
#32357=CARTESIAN_POINT('Ctrl Pts',(-2.48442644900942,1.06847604194589,11.0280779511531));
#32358=CARTESIAN_POINT('Ctrl Pts',(-2.50952949299033,1.18514270861324,11.0806194354338));
#32359=CARTESIAN_POINT('Ctrl Pts',(-2.5377525837873,1.30000000000212,11.1397002573077));
#32360=CARTESIAN_POINT('Ctrl Pts',(-2.70353383063933,-1.30000000000036,
10.9999887293473));
#32361=CARTESIAN_POINT('Ctrl Pts',(-2.65640171232275,-1.18514270861205,
10.9482279231614));
#32362=CARTESIAN_POINT('Ctrl Pts',(-2.61284843769618,-1.06847604194529,
10.9041562286735));
#32363=CARTESIAN_POINT('Ctrl Pts',(-2.52049950537525,-0.79477268400092,
10.8201051841181));
#32364=CARTESIAN_POINT('Ctrl Pts',(-2.46859493916104,-0.636309800095253,
10.7856129456557));
#32365=CARTESIAN_POINT('Ctrl Pts',(-2.40099281991649,-0.319434907277187,
10.7438761231169));
#32366=CARTESIAN_POINT('Ctrl Pts',(-2.37662940595917,-0.158333333333347,
10.7336352602338));
#32367=CARTESIAN_POINT('Ctrl Pts',(-2.35854571391392,0.158333333333349,
10.7459410578073));
#32368=CARTESIAN_POINT('Ctrl Pts',(-2.36620623217419,0.319434907277197,
10.7675442578828));
#32369=CARTESIAN_POINT('Ctrl Pts',(-2.39416059005098,0.636309800095264,
10.8362688648969));
#32370=CARTESIAN_POINT('Ctrl Pts',(-2.42346068791063,0.794772684000911,
10.8862207282079));
#32371=CARTESIAN_POINT('Ctrl Pts',(-2.47663733261307,1.06847604194589,10.9968274519963));
#32372=CARTESIAN_POINT('Ctrl Pts',(-2.50291507230902,1.18514270861324,11.0525733958149));
#32373=CARTESIAN_POINT('Ctrl Pts',(-2.53245235259803,1.30000000000212,11.116187731107));
#32374=CARTESIAN_POINT('Ctrl Pts',(-2.69833596654814,-1.30000000000032,
10.9830060396341));
#32375=CARTESIAN_POINT('Ctrl Pts',(-2.64958615648012,-1.18514270861202,
10.9282953727471));
#32376=CARTESIAN_POINT('Ctrl Pts',(-2.6047560693387,-1.06847604194526,10.8821229387945));
#32377=CARTESIAN_POINT('Ctrl Pts',(-2.51024494391219,-0.794772684000899,
10.7951804057463));
#32378=CARTESIAN_POINT('Ctrl Pts',(-2.45809203088939,-0.636309800095237,
10.761587928484));
#32379=CARTESIAN_POINT('Ctrl Pts',(-2.38960851425324,-0.31943490727718,
10.7202309484447));
#32380=CARTESIAN_POINT('Ctrl Pts',(-2.36479931898168,-0.158333333333342,
10.7114988387911));
#32381=CARTESIAN_POINT('Ctrl Pts',(-2.34695005012083,0.158333333333344,
10.7236290565346));
#32382=CARTESIAN_POINT('Ctrl Pts',(-2.35510759647371,0.319434907277187,
10.7436092936404));
#32383=CARTESIAN_POINT('Ctrl Pts',(-2.38479397203959,0.636309800095246,
10.8114714082294));
#32384=CARTESIAN_POINT('Ctrl Pts',(-2.41546462185311,0.794772684000892,
10.8599534127673));
#32385=CARTESIAN_POINT('Ctrl Pts',(-2.471393618411,1.06847604194587,10.9732413382738));
#32386=CARTESIAN_POINT('Ctrl Pts',(-2.49903161954639,1.18514270861321,11.0311090911607));
#32387=CARTESIAN_POINT('Ctrl Pts',(-2.53009803158076,1.30000000000209,11.097806451714));
#32388=CARTESIAN_POINT('Ctrl Pts',(-2.69311023072135,-1.3000000000003,10.9659408795865));
#32389=CARTESIAN_POINT('Ctrl Pts',(-2.64291410704766,-1.185142708612,10.9080071562898));
#32390=CARTESIAN_POINT('Ctrl Pts',(-2.59675403835677,-1.06847604194525,
10.859633017996));
#32391=CARTESIAN_POINT('Ctrl Pts',(-2.49943913981101,-0.794772684000888,
10.7699636350696));
#32392=CARTESIAN_POINT('Ctrl Pts',(-2.44466296249883,-0.636309800095227,
10.738646337535));
#32393=CARTESIAN_POINT('Ctrl Pts',(-2.37626217071313,-0.319434907277174,
10.6970765318667));
#32394=CARTESIAN_POINT('Ctrl Pts',(-2.35501508934159,-0.15833333333334,
10.6875776769682));
#32395=CARTESIAN_POINT('Ctrl Pts',(-2.33819796752328,0.158333333333342,
10.6990649893284));
#32396=CARTESIAN_POINT('Ctrl Pts',(-2.34447911271732,0.319434907277183,
10.7187462166911));
#32397=CARTESIAN_POINT('Ctrl Pts',(-2.37485390637155,0.636309800095237,
10.7863729191327));
#32398=CARTESIAN_POINT('Ctrl Pts',(-2.40711206569752,0.79477268400088,10.8332727810217));
#32399=CARTESIAN_POINT('Ctrl Pts',(-2.46533825214189,1.06847604194585,10.9496658909979));
#32400=CARTESIAN_POINT('Ctrl Pts',(-2.49410027228615,1.18514270861319,11.0098921791677));
#32401=CARTESIAN_POINT('Ctrl Pts',(-2.52642035395566,1.30000000000207,11.0799624909882));
#32402=CARTESIAN_POINT('Ctrl Pts',(-2.68879778714322,-1.30000000000028,
10.9518289492139));
#32403=CARTESIAN_POINT('Ctrl Pts',(-2.63666143001629,-1.18514270861199,
10.8918972781788));
#32404=CARTESIAN_POINT('Ctrl Pts',(-2.58926308493424,-1.06847604194523,
10.8419658485832));
#32405=CARTESIAN_POINT('Ctrl Pts',(-2.49070918144798,-0.794772684000878,
10.7497168157353));
#32406=CARTESIAN_POINT('Ctrl Pts',(-2.43777016675234,-0.636309800095217,
10.7179763783682));
#32407=CARTESIAN_POINT('Ctrl Pts',(-2.37010102182277,-0.319434907277169,
10.675947759028));
#32408=CARTESIAN_POINT('Ctrl Pts',(-2.34949050527065,-0.158333333333338,
10.6671666584067));
#32409=CARTESIAN_POINT('Ctrl Pts',(-2.33211239333941,0.158333333333339,
10.6789569746833));
#32410=CARTESIAN_POINT('Ctrl Pts',(-2.33637043201771,0.319434907277178,
10.6986904147996));
#32411=CARTESIAN_POINT('Ctrl Pts',(-2.36655247148205,0.636309800095226,
10.7664419578325));
#32412=CARTESIAN_POINT('Ctrl Pts',(-2.39991574346204,0.794772684000865,
10.8120484177623));
#32413=CARTESIAN_POINT('Ctrl Pts',(-2.45985583774373,1.06847604194583,10.930792397416));
#32414=CARTESIAN_POINT('Ctrl Pts',(-2.48954170162142,1.18514270861317,10.9927928874551));
#32415=CARTESIAN_POINT('Ctrl Pts',(-2.52296758356156,1.30000000000205,11.065393998639));
#32416=CARTESIAN_POINT('Ctrl Pts',(-2.6829189620322,-1.30000000000027,10.9351338813409));
#32417=CARTESIAN_POINT('Ctrl Pts',(-2.6282936778402,-1.18514270861197,10.8724521279875));
#32418=CARTESIAN_POINT('Ctrl Pts',(-2.57942287118579,-1.06847604194522,
10.8202878113131));
#32419=CARTESIAN_POINT('Ctrl Pts',(-2.4798155255339,-0.79477268400087,10.7240751870941));
#32420=CARTESIAN_POINT('Ctrl Pts',(-2.43000817475013,-0.636309800095212,
10.6911348221682));
#32421=CARTESIAN_POINT('Ctrl Pts',(-2.36412291257034,-0.319434907277166,
10.6478639598545));
#32422=CARTESIAN_POINT('Ctrl Pts',(-2.34455008781469,-0.158333333333336,
10.6399331146946));
#32423=CARTESIAN_POINT('Ctrl Pts',(-2.3272641458419,0.158333333333338,10.6516441590843));
#32424=CARTESIAN_POINT('Ctrl Pts',(-2.33029888248175,0.319434907277175,
10.6705886890844));
#32425=CARTESIAN_POINT('Ctrl Pts',(-2.35945060103271,0.636309800095221,
10.7391345767872));
#32426=CARTESIAN_POINT('Ctrl Pts',(-2.39125326023901,0.794772684000859,
10.7850495283766));
#32427=CARTESIAN_POINT('Ctrl Pts',(-2.45240936131587,1.06847604194582,10.907725068849));
#32428=CARTESIAN_POINT('Ctrl Pts',(-2.48329430471972,1.18514270861316,10.9721548996655));
#32429=CARTESIAN_POINT('Ctrl Pts',(-2.51859198142806,1.30000000000203,11.0479128654045));
#32430=CARTESIAN_POINT('Ctrl Pts',(-2.67899628993017,-1.30000000000024,
10.9237203428818));
#32431=CARTESIAN_POINT('Ctrl Pts',(-2.62148033775193,-1.18514270861195,
10.8598450798923));
#32432=CARTESIAN_POINT('Ctrl Pts',(-2.57119727859248,-1.0684760419452,10.8064956917622));
#32433=CARTESIAN_POINT('Ctrl Pts',(-2.47174278265131,-0.794772684000851,
10.7075648092919));
#32434=CARTESIAN_POINT('Ctrl Pts',(-2.42808446301742,-0.636309800095197,
10.6722759426476));
#32435=CARTESIAN_POINT('Ctrl Pts',(-2.3654168542827,-0.319434907277159,
10.6276471138997));
#32436=CARTESIAN_POINT('Ctrl Pts',(-2.34617121474401,-0.158333333333332,
10.6207395121414));
#32437=CARTESIAN_POINT('Ctrl Pts',(-2.32904419103437,0.158333333333334,
10.632401614771));
#32438=CARTESIAN_POINT('Ctrl Pts',(-2.3318239996864,0.319434907277167,10.6503972077161));
#32439=CARTESIAN_POINT('Ctrl Pts',(-2.35825829213826,0.636309800095206,
10.7199503234929));
#32440=CARTESIAN_POINT('Ctrl Pts',(-2.38472809612601,0.79477268400084,10.7674363574646));
#32441=CARTESIAN_POINT('Ctrl Pts',(-2.44568313888404,1.0684760419458,10.8928702981304));
#32442=CARTESIAN_POINT('Ctrl Pts',(-2.47774091685543,1.18514270861313,10.958697047156));
#32443=CARTESIAN_POINT('Ctrl Pts',(-2.5154712933951,1.300000000002,11.0360548400783));
#32444=CARTESIAN_POINT('Ctrl Pts',(-2.67879510330303,-1.30000000000024,
10.9151206262377));
#32445=CARTESIAN_POINT('Ctrl Pts',(-2.62131393065162,-1.18514270861195,
10.8514942540814));
#32446=CARTESIAN_POINT('Ctrl Pts',(-2.5713673254344,-1.0684760419452,10.7982205274448));
#32447=CARTESIAN_POINT('Ctrl Pts',(-2.4733870336565,-0.794772684000851,
10.699064243732));
#32448=CARTESIAN_POINT('Ctrl Pts',(-2.43213760273471,-0.636309800095197,
10.6628920207773));
#32449=CARTESIAN_POINT('Ctrl Pts',(-2.37107459905216,-0.319434907277159,
10.6177437697791));
#32450=CARTESIAN_POINT('Ctrl Pts',(-2.35179040064045,-0.158333333333332,
10.6108007652544));
#32451=CARTESIAN_POINT('Ctrl Pts',(-2.33489442655109,0.158333333333334,
10.6224108757364));
#32452=CARTESIAN_POINT('Ctrl Pts',(-2.33820931733128,0.319434907277167,
10.6403006616186));
#32453=CARTESIAN_POINT('Ctrl Pts',(-2.36296888549193,0.636309800095206,
10.7104490253785));
#32454=CARTESIAN_POINT('Ctrl Pts',(-2.38602389855414,0.79477268400084,10.7592218256451));
#32455=CARTESIAN_POINT('Ctrl Pts',(-2.4456425950795,1.0684760419458,10.8848134171439));
#32456=CARTESIAN_POINT('Ctrl Pts',(-2.47765621323778,1.18514270861313,10.9504344264684));
#32457=CARTESIAN_POINT('Ctrl Pts',(-2.51587672491887,1.300000000002,11.0273124987845));
#32458=CARTESIAN_POINT('Ctrl Pts',(-2.67879510330291,-1.3,10.9151206262376));
#32459=CARTESIAN_POINT('Ctrl Pts',(-2.62131393065155,-1.18514270861178,
10.8514942540813));
#32460=CARTESIAN_POINT('Ctrl Pts',(-2.57136732543437,-1.06847604194512,
10.7982205274447));
#32461=CARTESIAN_POINT('Ctrl Pts',(-2.4733870336565,-0.794772684000851,
10.699064243732));
#32462=CARTESIAN_POINT('Ctrl Pts',(-2.43213760273471,-0.636309800095197,
10.6628920207773));
#32463=CARTESIAN_POINT('Ctrl Pts',(-2.37107459905216,-0.319434907277159,
10.6177437697791));
#32464=CARTESIAN_POINT('Ctrl Pts',(-2.35179040064045,-0.158333333333332,
10.6108007652544));
#32465=CARTESIAN_POINT('Ctrl Pts',(-2.33489442655109,0.158333333333334,
10.6224108757364));
#32466=CARTESIAN_POINT('Ctrl Pts',(-2.33820931733128,0.319434907277167,
10.6403006616186));
#32467=CARTESIAN_POINT('Ctrl Pts',(-2.36296888549193,0.636309800095206,
10.7104490253786));
#32468=CARTESIAN_POINT('Ctrl Pts',(-2.38602389855414,0.79477268400084,10.7592218256451));
#32469=CARTESIAN_POINT('Ctrl Pts',(-2.44564259507935,1.06847604194511,10.8848134171436));
#32470=CARTESIAN_POINT('Ctrl Pts',(-2.47765621323741,1.18514270861178,10.9504344264676));
#32471=CARTESIAN_POINT('Ctrl Pts',(-2.5158767249182,1.3,11.0273124987831));
#32472=CARTESIAN_POINT('',(-2.73377200308821,-1.2,11.3266197589711));
#32473=CARTESIAN_POINT('Ctrl Pts',(-2.73377200308821,-1.2,11.3266197589711));
#32474=CARTESIAN_POINT('Ctrl Pts',(-2.73576236750696,-1.21682511930476,
11.305118979092));
#32475=CARTESIAN_POINT('Ctrl Pts',(-2.73869233675414,-1.23325164823463,
11.2834011551542));
#32476=CARTESIAN_POINT('Ctrl Pts',(-2.7416170980304,-1.25864690463805,11.2507925097067));
#32477=CARTESIAN_POINT('Ctrl Pts',(-2.74261046385924,-1.26676740637328,
11.2403081349856));
#32478=CARTESIAN_POINT('Ctrl Pts',(-2.74424726899164,-1.28141903494891,
11.2214696307683));
#32479=CARTESIAN_POINT('Ctrl Pts',(-2.74534902187955,-1.29187033557532,
11.2080548826955));
#32480=CARTESIAN_POINT('Ctrl Pts',(-2.74593499828894,-1.29845679859462,
11.1996640849239));
#32481=CARTESIAN_POINT('Ctrl Pts',(-2.74600037704013,-1.29922898799516,
11.1986824960205));
#32482=CARTESIAN_POINT('Ctrl Pts',(-2.74606098174262,-1.30000000000076,
11.1977054774637));
#32483=CARTESIAN_POINT('',(-2.60194863161808,-0.653834841327687,11.4109812773269));
#32484=CARTESIAN_POINT('Ctrl Pts',(-2.60194863169232,-0.653834841312246,
11.4109812773313));
#32485=CARTESIAN_POINT('Ctrl Pts',(-2.61437551623445,-0.711429103212125,
11.4033027546542));
#32486=CARTESIAN_POINT('Ctrl Pts',(-2.62750506939667,-0.767209465733077,
11.3951126019967));
#32487=CARTESIAN_POINT('Ctrl Pts',(-2.65474262170037,-0.881586813988967,
11.3779310203753));
#32488=CARTESIAN_POINT('Ctrl Pts',(-2.66777274013477,-0.939011938483551,
11.3696339333288));
#32489=CARTESIAN_POINT('Ctrl Pts',(-2.69210580986878,-1.03699387118054,
11.353933891983));
#32490=CARTESIAN_POINT('Ctrl Pts',(-2.69333142495775,-1.0411369329597,11.3531667563918));
#32491=CARTESIAN_POINT('Ctrl Pts',(-2.71810657748227,-1.13882989710818,
11.3369709263887));
#32492=CARTESIAN_POINT('Ctrl Pts',(-2.72488491396426,-1.16582599832885,
11.3325072108943));
#32493=CARTESIAN_POINT('Ctrl Pts',(-2.73377200308821,-1.2,11.3266197589711));
#32494=CARTESIAN_POINT('',(-2.48224831221869,0.653834841531101,11.4826327552672));
#32495=CARTESIAN_POINT('Ctrl Pts',(-2.48224831221869,0.653834841531094,
11.4826327552672));
#32496=CARTESIAN_POINT('Ctrl Pts',(-2.47847611081766,0.575733241027942,
11.4410983042038));
#32497=CARTESIAN_POINT('Ctrl Pts',(-2.47624165072888,0.493688711564448,
11.4060553104082));
#32498=CARTESIAN_POINT('Ctrl Pts',(-2.47524533739703,0.338070081393044,
11.3554031699183));
#32499=CARTESIAN_POINT('Ctrl Pts',(-2.47618347792561,0.265612270873024,
11.3374916856793));
#32500=CARTESIAN_POINT('Ctrl Pts',(-2.48168727921389,0.129685337361217,
11.3136922909595));
#32501=CARTESIAN_POINT('Ctrl Pts',(-2.48565124756031,0.0666366523113049,
11.3064612606332));
#32502=CARTESIAN_POINT('Ctrl Pts',(-2.49684990484168,-0.0594732938431921,
11.2993200133022));
#32503=CARTESIAN_POINT('Ctrl Pts',(-2.50414835339649,-0.122670367054008,
11.2993485456319));
#32504=CARTESIAN_POINT('Ctrl Pts',(-2.5229219596009,-0.260039449736775,
11.307924387759));
#32505=CARTESIAN_POINT('Ctrl Pts',(-2.53495623693555,-0.333904359140863,
11.318007596868));
#32506=CARTESIAN_POINT('Ctrl Pts',(-2.56422571957007,-0.49149423887964,
11.352069384849));
#32507=CARTESIAN_POINT('Ctrl Pts',(-2.58242227177419,-0.574906056387881,
11.3781108287718));
#32508=CARTESIAN_POINT('Ctrl Pts',(-2.60194863169483,-0.653834841350394,
11.4109812772268));
#32509=CARTESIAN_POINT('',(-2.54449248972722,1.2,11.4459460629784));
#32510=CARTESIAN_POINT('Ctrl Pts',(-2.54449248972723,1.2,11.4459460629784));
#32511=CARTESIAN_POINT('Ctrl Pts',(-2.53481538344241,1.14033138422225,11.4517453180558));
#32512=CARTESIAN_POINT('Ctrl Pts',(-2.52020515509785,1.04182072801943,11.4604498142848));
#32513=CARTESIAN_POINT('Ctrl Pts',(-2.4925470916887,0.79704371814103,11.4766664306308));
#32514=CARTESIAN_POINT('Ctrl Pts',(-2.48792048827851,0.741502902961087,
11.4793451165048));
#32515=CARTESIAN_POINT('Ctrl Pts',(-2.48224831221869,0.653834841531102,
11.4826327552672));
#32516=CARTESIAN_POINT('Ctrl Pts',(-2.55655914734356,1.30000000000015,11.321468831149));
#32517=CARTESIAN_POINT('Ctrl Pts',(-2.55519028108804,1.28313676905805,11.3421620017419));
#32518=CARTESIAN_POINT('Ctrl Pts',(-2.55296550889272,1.2665451586595,11.3630099517663));
#32519=CARTESIAN_POINT('Ctrl Pts',(-2.54981239277721,1.23818291853827,11.3981516985073));
#32520=CARTESIAN_POINT('Ctrl Pts',(-2.54809619279288,1.21981197361561,11.420689297303));
#32521=CARTESIAN_POINT('Ctrl Pts',(-2.54449248972723,1.2,11.4459460629784));
#32522=CARTESIAN_POINT('Ctrl Pts',(-2.67879510330291,-1.3,10.9151206262376));
#32523=CARTESIAN_POINT('Ctrl Pts',(-2.62131393065155,-1.18514270861178,
10.8514942540813));
#32524=CARTESIAN_POINT('Ctrl Pts',(-2.57136732543437,-1.06847604194512,
10.7982205274447));
#32525=CARTESIAN_POINT('Ctrl Pts',(-2.4733870336565,-0.794772684000851,
10.699064243732));
#32526=CARTESIAN_POINT('Ctrl Pts',(-2.4321376027347,-0.636309800095197,
10.6628920207773));
#32527=CARTESIAN_POINT('Ctrl Pts',(-2.37107459905216,-0.319434907277159,
10.6177437697791));
#32528=CARTESIAN_POINT('Ctrl Pts',(-2.35179040064045,-0.158333333333332,
10.6108007652544));
#32529=CARTESIAN_POINT('Ctrl Pts',(-2.33489442655109,0.158333333333334,
10.6224108757364));
#32530=CARTESIAN_POINT('Ctrl Pts',(-2.33820931733128,0.319434907277167,
10.6403006616186));
#32531=CARTESIAN_POINT('Ctrl Pts',(-2.36296888549193,0.636309800095206,
10.7104490253785));
#32532=CARTESIAN_POINT('Ctrl Pts',(-2.38602389855414,0.79477268400084,10.7592218256451));
#32533=CARTESIAN_POINT('Ctrl Pts',(-2.44564259507935,1.06847604194511,10.8848134171436));
#32534=CARTESIAN_POINT('Ctrl Pts',(-2.47765621323741,1.18514270861178,10.9504344264676));
#32535=CARTESIAN_POINT('Ctrl Pts',(-2.5158767249182,1.3,11.0273124987831));
#32536=CARTESIAN_POINT('Ctrl Pts',(-2.74004401157309,-1.3,10.8685622702705));
#32537=CARTESIAN_POINT('Ctrl Pts',(-2.68128836180793,-1.18514270861178,
10.8061091896562));
#32538=CARTESIAN_POINT('Ctrl Pts',(-2.63048511284273,-1.06847604194512,
10.7536851161556));
#32539=CARTESIAN_POINT('Ctrl Pts',(-2.53149108129824,-0.794772684000851,
10.6557440316982));
#32540=CARTESIAN_POINT('Ctrl Pts',(-2.49090436112714,-0.636309800095197,
10.6192964682111));
#32541=CARTESIAN_POINT('Ctrl Pts',(-2.43050771496334,-0.319434907277159,
10.5741227058226));
#32542=CARTESIAN_POINT('Ctrl Pts',(-2.41232163607126,-0.158333333333332,
10.5666004040259));
#32543=CARTESIAN_POINT('Ctrl Pts',(-2.39563664855869,0.158333333333334,
10.5785009126177));
#32544=CARTESIAN_POINT('Ctrl Pts',(-2.39806125730008,0.319434907277167,
10.5972560595228));
#32545=CARTESIAN_POINT('Ctrl Pts',(-2.42259064688909,0.636309800095206,
10.66803028349));
#32546=CARTESIAN_POINT('Ctrl Pts',(-2.4451790066595,0.79477268400084,10.7173482742307));
#32547=CARTESIAN_POINT('Ctrl Pts',(-2.50626668917077,1.06847604194511,10.8423512591397));
#32548=CARTESIAN_POINT('Ctrl Pts',(-2.53935309295667,1.18514270861178,10.9074201091034));
#32549=CARTESIAN_POINT('Ctrl Pts',(-2.57908330629107,1.3,10.9834486486808));
#32550=CARTESIAN_POINT('Ctrl Pts',(-2.80129291984328,-1.3,10.8220039143035));
#32551=CARTESIAN_POINT('Ctrl Pts',(-2.7412627929643,-1.18514270861178,10.7607241252311));
#32552=CARTESIAN_POINT('Ctrl Pts',(-2.68960290025109,-1.06847604194512,
10.7091497048665));
#32553=CARTESIAN_POINT('Ctrl Pts',(-2.58959512893997,-0.794772684000851,
10.6124238196643));
#32554=CARTESIAN_POINT('Ctrl Pts',(-2.54967111951957,-0.636309800095197,
10.5757009156449));
#32555=CARTESIAN_POINT('Ctrl Pts',(-2.48994083087453,-0.319434907277159,
10.530501641866));
#32556=CARTESIAN_POINT('Ctrl Pts',(-2.47285287150207,-0.158333333333332,
10.5224000427974));
#32557=CARTESIAN_POINT('Ctrl Pts',(-2.4563788705663,0.158333333333334,10.5345909494989));
#32558=CARTESIAN_POINT('Ctrl Pts',(-2.45791319726889,0.319434907277167,
10.5542114574271));
#32559=CARTESIAN_POINT('Ctrl Pts',(-2.48221240828625,0.636309800095206,
10.6256115416015));
#32560=CARTESIAN_POINT('Ctrl Pts',(-2.50433411476485,0.79477268400084,10.6754747228163));
#32561=CARTESIAN_POINT('Ctrl Pts',(-2.5668907832622,1.06847604194511,10.7998891011359));
#32562=CARTESIAN_POINT('Ctrl Pts',(-2.60104997267594,1.18514270861178,10.8644057917392));
#32563=CARTESIAN_POINT('Ctrl Pts',(-2.64228988766393,1.3,10.9395847985784));
#32564=CARTESIAN_POINT('Ctrl Pts',(-2.86254182811346,-1.3,10.7754455583364));
#32565=CARTESIAN_POINT('Ctrl Pts',(-2.80123722412068,-1.18514270861178,
10.715339060806));
#32566=CARTESIAN_POINT('Ctrl Pts',(-2.74872068765946,-1.06847604194512,
10.6646142935774));
#32567=CARTESIAN_POINT('Ctrl Pts',(-2.6476991765817,-0.794772684000851,
10.5691036076304));
#32568=CARTESIAN_POINT('Ctrl Pts',(-2.60843787791201,-0.636309800095197,
10.5321053630787));
#32569=CARTESIAN_POINT('Ctrl Pts',(-2.54937394678571,-0.319434907277159,
10.4868805779095));
#32570=CARTESIAN_POINT('Ctrl Pts',(-2.53338410693288,-0.158333333333332,
10.4781996815688));
#32571=CARTESIAN_POINT('Ctrl Pts',(-2.5171210925739,0.158333333333334,10.4906809863802));
#32572=CARTESIAN_POINT('Ctrl Pts',(-2.5177651372377,0.319434907277167,10.5111668553313));
#32573=CARTESIAN_POINT('Ctrl Pts',(-2.54183416968341,0.636309800095206,
10.5831927997129));
#32574=CARTESIAN_POINT('Ctrl Pts',(-2.5634892228702,0.79477268400084,10.6336011714019));
#32575=CARTESIAN_POINT('Ctrl Pts',(-2.62751487735363,1.06847604194511,10.757426943132));
#32576=CARTESIAN_POINT('Ctrl Pts',(-2.6627468523952,1.18514270861178,10.821391474375));
#32577=CARTESIAN_POINT('Ctrl Pts',(-2.70549646903679,1.3,10.8957209484761));
#32578=CARTESIAN_POINT('Ctrl Pts',(-2.86254182811346,-1.3,10.7754455583364));
#32579=CARTESIAN_POINT('Ctrl Pts',(-2.80123722412068,-1.18514270861178,
10.715339060806));
#32580=CARTESIAN_POINT('Ctrl Pts',(-2.74872068765946,-1.06847604194512,
10.6646142935774));
#32581=CARTESIAN_POINT('Ctrl Pts',(-2.6476991765817,-0.794772684000851,
10.5691036076304));
#32582=CARTESIAN_POINT('Ctrl Pts',(-2.60843787791201,-0.636309800095197,
10.5321053630787));
#32583=CARTESIAN_POINT('Ctrl Pts',(-2.54937394678571,-0.319434907277159,
10.4868805779095));
#32584=CARTESIAN_POINT('Ctrl Pts',(-2.53338410693288,-0.158333333333332,
10.4781996815689));
#32585=CARTESIAN_POINT('Ctrl Pts',(-2.5171210925739,0.158333333333334,10.4906809863802));
#32586=CARTESIAN_POINT('Ctrl Pts',(-2.5177651372377,0.319434907277167,10.5111668553313));
#32587=CARTESIAN_POINT('Ctrl Pts',(-2.54183416968341,0.636309800095206,
10.5831927997129));
#32588=CARTESIAN_POINT('Ctrl Pts',(-2.56348922287021,0.79477268400084,10.6336011714019));
#32589=CARTESIAN_POINT('Ctrl Pts',(-2.62751487735363,1.06847604194511,10.757426943132));
#32590=CARTESIAN_POINT('Ctrl Pts',(-2.6627468523952,1.18514270861178,10.821391474375));
#32591=CARTESIAN_POINT('Ctrl Pts',(-2.70549646903679,1.3,10.8957209484761));
#32592=CARTESIAN_POINT('Ctrl Pts',(-2.86254182811353,-1.30000000000013,
10.7754455583365));
#32593=CARTESIAN_POINT('Ctrl Pts',(-2.80123722412072,-1.18514270861187,
10.715339060806));
#32594=CARTESIAN_POINT('Ctrl Pts',(-2.74872068765947,-1.06847604194516,
10.6646142935774));
#32595=CARTESIAN_POINT('Ctrl Pts',(-2.6476991765817,-0.794772684000851,
10.5691036076304));
#32596=CARTESIAN_POINT('Ctrl Pts',(-2.60843787791201,-0.636309800095197,
10.5321053630787));
#32597=CARTESIAN_POINT('Ctrl Pts',(-2.54937394678571,-0.319434907277159,
10.4868805779095));
#32598=CARTESIAN_POINT('Ctrl Pts',(-2.53338410693289,-0.158333333333332,
10.4781996815689));
#32599=CARTESIAN_POINT('Ctrl Pts',(-2.5171210925739,0.158333333333334,10.4906809863802));
#32600=CARTESIAN_POINT('Ctrl Pts',(-2.5177651372377,0.319434907277167,10.5111668553313));
#32601=CARTESIAN_POINT('Ctrl Pts',(-2.54183416968341,0.636309800095206,
10.5831927997129));
#32602=CARTESIAN_POINT('Ctrl Pts',(-2.56348922287021,0.79477268400084,10.6336011714019));
#32603=CARTESIAN_POINT('Ctrl Pts',(-2.62751487735368,1.06847604194532,10.7574269431321));
#32604=CARTESIAN_POINT('Ctrl Pts',(-2.66274685239533,1.18514270861219,10.8213914743752));
#32605=CARTESIAN_POINT('Ctrl Pts',(-2.70549646903702,1.30000000000061,10.8957209484765));
#32606=CARTESIAN_POINT('Ctrl Pts',(-2.87098157396354,-1.30000000000013,
10.7777615020269));
#32607=CARTESIAN_POINT('Ctrl Pts',(-2.80906926847882,-1.18514270861187,
10.7179729089025));
#32608=CARTESIAN_POINT('Ctrl Pts',(-2.75637070807042,-1.06847604194516,
10.6671425661359));
#32609=CARTESIAN_POINT('Ctrl Pts',(-2.65591208554583,-0.794772684000851,
10.5704096561886));
#32610=CARTESIAN_POINT('Ctrl Pts',(-2.61892980277956,-0.636309800095197,
10.5305613851358));
#32611=CARTESIAN_POINT('Ctrl Pts',(-2.56094950437881,-0.319434907277159,
10.4839277842398));
#32612=CARTESIAN_POINT('Ctrl Pts',(-2.54469368652178,-0.158333333333332,
10.4757230850146));
#32613=CARTESIAN_POINT('Ctrl Pts',(-2.52830982643484,0.158333333333334,
10.4884080646188));
#32614=CARTESIAN_POINT('Ctrl Pts',(-2.52893211645303,0.319434907277167,
10.5088463218988));
#32615=CARTESIAN_POINT('Ctrl Pts',(-2.55201129877011,0.636309800095206,
10.5822378260926));
#32616=CARTESIAN_POINT('Ctrl Pts',(-2.57208184262635,0.79477268400084,10.6346642149685));
#32617=CARTESIAN_POINT('Ctrl Pts',(-2.6354375736483,1.06847604194532,10.7598223853577));
#32618=CARTESIAN_POINT('Ctrl Pts',(-2.67063753705888,1.18514270861219,10.8241302839999));
#32619=CARTESIAN_POINT('Ctrl Pts',(-2.71361311548183,1.30000000000061,10.8985697468901));
#32620=CARTESIAN_POINT('Ctrl Pts',(-2.88130799910642,-1.30000000000008,
10.7843752712055));
#32621=CARTESIAN_POINT('Ctrl Pts',(-2.8201751994264,-1.18514270861182,10.7273767909063));
#32622=CARTESIAN_POINT('Ctrl Pts',(-2.76844666246347,-1.06847604194512,
10.6780839335672));
#32623=CARTESIAN_POINT('Ctrl Pts',(-2.67066912201355,-0.79477268400082,
10.582009102654));
#32624=CARTESIAN_POINT('Ctrl Pts',(-2.63680377542968,-0.636309800095171,
10.5376034533262));
#32625=CARTESIAN_POINT('Ctrl Pts',(-2.58060181184424,-0.319434907277146,
10.4887166000006));
#32626=CARTESIAN_POINT('Ctrl Pts',(-2.56351360569678,-0.158333333333326,
10.4799872004688));
#32627=CARTESIAN_POINT('Ctrl Pts',(-2.54702843312608,0.158333333333328,
10.4928124384856));
#32628=CARTESIAN_POINT('Ctrl Pts',(-2.54851681421681,0.319434907277155,
10.5138783362634));
#32629=CARTESIAN_POINT('Ctrl Pts',(-2.56933627910873,0.636309800095181,
10.589884803704));
#32630=CARTESIAN_POINT('Ctrl Pts',(-2.58533128900916,0.794772684000808,
10.6473785638044));
#32631=CARTESIAN_POINT('Ctrl Pts',(-2.64606408059228,1.06847604194528,10.7718410121851));
#32632=CARTESIAN_POINT('Ctrl Pts',(-2.68056571917546,1.18514270861214,10.8344520548743));
#32633=CARTESIAN_POINT('Ctrl Pts',(-2.72328002123719,1.30000000000056,10.905798958137));
#32634=CARTESIAN_POINT('Ctrl Pts',(-2.89657675896679,-1.30000000000006,
10.7939475114029));
#32635=CARTESIAN_POINT('Ctrl Pts',(-2.83786245193787,-1.18514270861181,
10.739717112883));
#32636=CARTESIAN_POINT('Ctrl Pts',(-2.78807069208927,-1.06847604194511,
10.6923235368659));
#32637=CARTESIAN_POINT('Ctrl Pts',(-2.69365463496759,-0.794772684000811,
10.5986293228974));
#32638=CARTESIAN_POINT('Ctrl Pts',(-2.66056908699804,-0.636309800095165,
10.5528292186773));
#32639=CARTESIAN_POINT('Ctrl Pts',(-2.60545199801408,-0.319434907277143,
10.5031969108166));
#32640=CARTESIAN_POINT('Ctrl Pts',(-2.58799440475969,-0.158333333333324,
10.4930527565231));
#32641=CARTESIAN_POINT('Ctrl Pts',(-2.57143636450316,0.158333333333326,
10.505914313829));
#32642=CARTESIAN_POINT('Ctrl Pts',(-2.57346983404538,0.319434907277151,
10.5281859967145));
#32643=CARTESIAN_POINT('Ctrl Pts',(-2.59254968088905,0.636309800095174,
10.6055115343826));
#32644=CARTESIAN_POINT('Ctrl Pts',(-2.60634895807667,0.794772684000802,
10.6656876864475));
#32645=CARTESIAN_POINT('Ctrl Pts',(-2.66362773438282,1.06847604194526,10.787923442475));
#32646=CARTESIAN_POINT('Ctrl Pts',(-2.69647182859621,1.18514270861213,10.8484289414837));
#32647=CARTESIAN_POINT('Ctrl Pts',(-2.73736615714789,1.30000000000054,10.9165286099978));
#32648=CARTESIAN_POINT('Ctrl Pts',(-2.90939733936904,-1.30000000000003,
10.8016830781138));
#32649=CARTESIAN_POINT('Ctrl Pts',(-2.85277794295122,-1.18514270861178,
10.7492279012714));
#32650=CARTESIAN_POINT('Ctrl Pts',(-2.80440263622773,-1.06847604194508,
10.7032260336092));
#32651=CARTESIAN_POINT('Ctrl Pts',(-2.71169149666796,-0.794772684000791,
10.6118609518534));
#32652=CARTESIAN_POINT('Ctrl Pts',(-2.67698456243157,-0.636309800095147,
10.5667713648255));
#32653=CARTESIAN_POINT('Ctrl Pts',(-2.62198781289779,-0.319434907277134,
10.5170532377087));
#32654=CARTESIAN_POINT('Ctrl Pts',(-2.60518369447283,-0.15833333333332,
10.5050370914482));
#32655=CARTESIAN_POINT('Ctrl Pts',(-2.58900027913727,0.158333333333322,
10.5175329029115));
#32656=CARTESIAN_POINT('Ctrl Pts',(-2.59136705757064,0.319434907277142,
10.5407427661508));
#32657=CARTESIAN_POINT('Ctrl Pts',(-2.6098427255564,0.636309800095157,10.618566234201));
#32658=CARTESIAN_POINT('Ctrl Pts',(-2.6229812366886,0.794772684000779,10.6800848080548));
#32659=CARTESIAN_POINT('Ctrl Pts',(-2.67822876463443,1.06847604194523,10.800342369775));
#32660=CARTESIAN_POINT('Ctrl Pts',(-2.70993424876684,1.18514270861209,10.8592459875587));
#32661=CARTESIAN_POINT('Ctrl Pts',(-2.74943060930655,1.3000000000005,10.9249981806394));
#32662=CARTESIAN_POINT('Ctrl Pts',(-2.92255067730094,-1.3,10.8092626647235));
#32663=CARTESIAN_POINT('Ctrl Pts',(-2.86823924221959,-1.18514270861175,
10.7587576758521));
#32664=CARTESIAN_POINT('Ctrl Pts',(-2.82142143722469,-1.06847604194506,
10.7143091764557));
#32665=CARTESIAN_POINT('Ctrl Pts',(-2.73057472641195,-0.794772684000774,
10.6256159532415));
#32666=CARTESIAN_POINT('Ctrl Pts',(-2.69426049879219,-0.636309800095134,
10.5813094568819));
#32667=CARTESIAN_POINT('Ctrl Pts',(-2.63898342204987,-0.319434907277128,
10.5319919830244));
#32668=CARTESIAN_POINT('Ctrl Pts',(-2.62245246795658,-0.158333333333317,
10.5183581005772));
#32669=CARTESIAN_POINT('Ctrl Pts',(-2.60566422148455,0.158333333333319,
10.531359703171));
#32670=CARTESIAN_POINT('Ctrl Pts',(-2.60681389033176,0.319434907277137,
10.5569638279893));
#32671=CARTESIAN_POINT('Ctrl Pts',(-2.62502863909171,0.636309800095145,
10.634865436697));
#32672=CARTESIAN_POINT('Ctrl Pts',(-2.64011247630467,0.794772684000763,
10.6953567565866));
#32673=CARTESIAN_POINT('Ctrl Pts',(-2.69385664340059,1.06847604194521,10.8126926805983));
#32674=CARTESIAN_POINT('Ctrl Pts',(-2.72422830809232,1.18514270861207,10.8698798781649));
#32675=CARTESIAN_POINT('Ctrl Pts',(-2.76170777895762,1.30000000000048,10.9334638995178));
#32676=CARTESIAN_POINT('Ctrl Pts',(-2.93364134797168,-1.29999999999998,
10.8146096561709));
#32677=CARTESIAN_POINT('Ctrl Pts',(-2.88110586058543,-1.18514270861173,
10.765538855818));
#32678=CARTESIAN_POINT('Ctrl Pts',(-2.83544209508976,-1.06847604194504,
10.722278164585));
#32679=CARTESIAN_POINT('Ctrl Pts',(-2.74582471404032,-0.79477268400076,
10.6357598279408));
#32680=CARTESIAN_POINT('Ctrl Pts',(-2.70815544963049,-0.636309800095123,
10.5921789864677));
#32681=CARTESIAN_POINT('Ctrl Pts',(-2.65198788829456,-0.319434907277122,
10.5437895582696));
#32682=CARTESIAN_POINT('Ctrl Pts',(-2.63461414097152,-0.158333333333314,
10.5299086096514));
#32683=CARTESIAN_POINT('Ctrl Pts',(-2.61730002870664,0.158333333333316,
10.5433402077525));
#32684=CARTESIAN_POINT('Ctrl Pts',(-2.61847805619027,0.31943490727713,10.5698315744701));
#32685=CARTESIAN_POINT('Ctrl Pts',(-2.63709993265635,0.636309800095133,
10.6472528854295));
#32686=CARTESIAN_POINT('Ctrl Pts',(-2.65397682566829,0.794772684000749,
10.7067377621516));
#32687=CARTESIAN_POINT('Ctrl Pts',(-2.70649287215143,1.06847604194519,10.8220022733572));
#32688=CARTESIAN_POINT('Ctrl Pts',(-2.73567401252214,1.18514270861205,10.8780795065985));
#32689=CARTESIAN_POINT('Ctrl Pts',(-2.7713040426523,1.30000000000045,10.9403402371513));
#32690=CARTESIAN_POINT('Ctrl Pts',(-2.94454127932457,-1.29999999999996,
10.8202105050095));
#32691=CARTESIAN_POINT('Ctrl Pts',(-2.89370153575553,-1.18514270861172,
10.7727504801566));
#32692=CARTESIAN_POINT('Ctrl Pts',(-2.84916686915389,-1.06847604194502,
10.7307723697174));
#32693=CARTESIAN_POINT('Ctrl Pts',(-2.76084886929562,-0.794772684000748,
10.6464588558599));
#32694=CARTESIAN_POINT('Ctrl Pts',(-2.72210825231037,-0.636309800095113,
10.6033006630912));
#32695=CARTESIAN_POINT('Ctrl Pts',(-2.66520808832749,-0.319434907277117,
10.5556735424191));
#32696=CARTESIAN_POINT('Ctrl Pts',(-2.64676320471826,-0.158333333333312,
10.5416884442415));
#32697=CARTESIAN_POINT('Ctrl Pts',(-2.62938737440501,0.158333333333314,
10.5551568985966));
#32698=CARTESIAN_POINT('Ctrl Pts',(-2.63171112765893,0.319434907277125,
10.5816477591922));
#32699=CARTESIAN_POINT('Ctrl Pts',(-2.65066224292211,0.636309800095123,
10.6586700857846));
#32700=CARTESIAN_POINT('Ctrl Pts',(-2.66783258409506,0.794772684000737,
10.7184529688622));
#32701=CARTESIAN_POINT('Ctrl Pts',(-2.71892149588491,1.06847604194518,10.8316990745312));
#32702=CARTESIAN_POINT('Ctrl Pts',(-2.74708102516698,1.18514270861203,10.8864396280687));
#32703=CARTESIAN_POINT('Ctrl Pts',(-2.78128558684804,1.30000000000044,10.9469006921814));
#32704=CARTESIAN_POINT('Ctrl Pts',(-2.96280984633306,-1.29999999999991,
10.8308072518359));
#32705=CARTESIAN_POINT('Ctrl Pts',(-2.91532013949125,-1.18514270861167,
10.7856898450932));
#32706=CARTESIAN_POINT('Ctrl Pts',(-2.87307106373488,-1.06847604194498,
10.7455850031852));
#32707=CARTESIAN_POINT('Ctrl Pts',(-2.78757415303104,-0.794772684000721,
10.6645148229603));
#32708=CARTESIAN_POINT('Ctrl Pts',(-2.74709018776719,-0.636309800095094,
10.6220267483154));
#32709=CARTESIAN_POINT('Ctrl Pts',(-2.68913215432975,-0.319434907277108,
10.57556179981));
#32710=CARTESIAN_POINT('Ctrl Pts',(-2.66916152367942,-0.158333333333307,
10.5611593392128));
#32711=CARTESIAN_POINT('Ctrl Pts',(-2.65102314855752,0.158333333333309,
10.5752777094955));
#32712=CARTESIAN_POINT('Ctrl Pts',(-2.65356013672887,0.319434907277116,
10.6032946602505));
#32713=CARTESIAN_POINT('Ctrl Pts',(-2.67313611639813,0.636309800095105,
10.6795440799993));
#32714=CARTESIAN_POINT('Ctrl Pts',(-2.69305833511178,0.794772684000714,
10.737821432715));
#32715=CARTESIAN_POINT('Ctrl Pts',(-2.74189854612259,1.06847604194515,10.8473865048979));
#32716=CARTESIAN_POINT('Ctrl Pts',(-2.76799328720399,1.18514270861199,10.9000916623425));
#32717=CARTESIAN_POINT('Ctrl Pts',(-2.79904165172837,1.30000000000039,10.9580753172698));
#32718=CARTESIAN_POINT('Ctrl Pts',(-2.99104878850529,-1.2999999999998,10.843667343189));
#32719=CARTESIAN_POINT('Ctrl Pts',(-2.94861710368942,-1.18514270861157,
10.8016268124618));
#32720=CARTESIAN_POINT('Ctrl Pts',(-2.90970236271676,-1.06847604194489,
10.7641432672306));
#32721=CARTESIAN_POINT('Ctrl Pts',(-2.82792637004268,-0.794772684000651,
10.6880763273062));
#32722=CARTESIAN_POINT('Ctrl Pts',(-2.78389301348772,-0.636309800095033,
10.6477071761781));
#32723=CARTESIAN_POINT('Ctrl Pts',(-2.72376072317303,-0.319434907277076,
10.603619031765));
#32724=CARTESIAN_POINT('Ctrl Pts',(-2.70111831575195,-0.158333333333292,
10.5890402621661));
#32725=CARTESIAN_POINT('Ctrl Pts',(-2.68261307994366,0.158333333333294,
10.6034604755936));
#32726=CARTESIAN_POINT('Ctrl Pts',(-2.68774540138619,0.319434907277086,
10.6316097871425));
#32727=CARTESIAN_POINT('Ctrl Pts',(-2.70815681023057,0.636309800095044,
10.7068015876387));
#32728=CARTESIAN_POINT('Ctrl Pts',(-2.72946345267766,0.794772684000635,
10.7652017115724));
#32729=CARTESIAN_POINT('Ctrl Pts',(-2.77434485092659,1.06847604194504,10.8701458336658));
#32730=CARTESIAN_POINT('Ctrl Pts',(-2.79750261992242,1.18514270861188,10.9199136815502));
#32731=CARTESIAN_POINT('Ctrl Pts',(-2.82439066363181,1.30000000000028,10.9740229554276));
#32732=CARTESIAN_POINT('Ctrl Pts',(-3.01834269857635,-1.29999999999968,
10.8574591123472));
#32733=CARTESIAN_POINT('Ctrl Pts',(-2.98046491035473,-1.18514270861146,
10.8190105036788));
#32734=CARTESIAN_POINT('Ctrl Pts',(-2.9447942397598,-1.06847604194479,10.7842434833884));
#32735=CARTESIAN_POINT('Ctrl Pts',(-2.86748673804234,-0.794772684000576,
10.7124299170517));
#32736=CARTESIAN_POINT('Ctrl Pts',(-2.82234682309723,-0.636309800094976,
10.6716853336954));
#32737=CARTESIAN_POINT('Ctrl Pts',(-2.76109407379248,-0.319434907277048,
10.6289560348325));
#32738=CARTESIAN_POINT('Ctrl Pts',(-2.73541472162827,-0.158333333333277,
10.6146850901235));
#32739=CARTESIAN_POINT('Ctrl Pts',(-2.71600552864647,0.158333333333279,
10.6299428199933));
#32740=CARTESIAN_POINT('Ctrl Pts',(-2.72268668763626,0.319434907277056,
10.6591473057952));
#32741=CARTESIAN_POINT('Ctrl Pts',(-2.74356713133065,0.636309800094986,
10.7336158510058));
#32742=CARTESIAN_POINT('Ctrl Pts',(-2.76711068084563,0.794772684000565,
10.7913518889265));
#32743=CARTESIAN_POINT('Ctrl Pts',(-2.80768348975369,1.06847604194495,10.8920278319734));
#32744=CARTESIAN_POINT('Ctrl Pts',(-2.82754652527184,1.18514270861178,10.9392085103723));
#32745=CARTESIAN_POINT('Ctrl Pts',(-2.84971013070257,1.30000000000016,10.9899909818365));
#32746=CARTESIAN_POINT('Ctrl Pts',(-3.04099809512413,-1.2999999999996,10.8675872666515));
#32747=CARTESIAN_POINT('Ctrl Pts',(-3.00762724759638,-1.18514270861139,
10.831064390507));
#32748=CARTESIAN_POINT('Ctrl Pts',(-2.97504038096538,-1.06847604194473,
10.7979362546403));
#32749=CARTESIAN_POINT('Ctrl Pts',(-2.9015693527738,-0.794772684000529,
10.7292461626843));
#32750=CARTESIAN_POINT('Ctrl Pts',(-2.85408545169189,-0.636309800094938,
10.6897924612697));
#32751=CARTESIAN_POINT('Ctrl Pts',(-2.79158851066336,-0.319434907277029,
10.6485850969138));
#32752=CARTESIAN_POINT('Ctrl Pts',(-2.76395740512797,-0.158333333333268,
10.6341165951374));
#32753=CARTESIAN_POINT('Ctrl Pts',(-2.74396501783023,0.15833333333327,10.6499441997137));
#32754=CARTESIAN_POINT('Ctrl Pts',(-2.75189768034267,0.319434907277039,
10.6799927615318));
#32755=CARTESIAN_POINT('Ctrl Pts',(-2.77307282462227,0.63630980009495,10.7539440471771));
#32756=CARTESIAN_POINT('Ctrl Pts',(-2.79821037766364,0.794772684000518,
10.8112808656079));
#32757=CARTESIAN_POINT('Ctrl Pts',(-2.83523034666321,1.06847604194488,10.9086287951997));
#32758=CARTESIAN_POINT('Ctrl Pts',(-2.85243431226021,1.18514270861171,10.9537645467817));
#32759=CARTESIAN_POINT('Ctrl Pts',(-2.87081767059933,1.30000000000008,11.0018977383219));
#32760=CARTESIAN_POINT('Ctrl Pts',(-3.05375053744494,-1.29999999999949,
10.8732488581604));
#32761=CARTESIAN_POINT('Ctrl Pts',(-3.02253872191128,-1.18514270861129,
10.8382134400058));
#32762=CARTESIAN_POINT('Ctrl Pts',(-2.9914515894023,-1.06847604194464,10.8062588675511));
#32763=CARTESIAN_POINT('Ctrl Pts',(-2.91992213707681,-0.794772684000461,
10.7395547825784));
#32764=CARTESIAN_POINT('Ctrl Pts',(-2.87147188423377,-0.636309800094884,
10.7004414750604));
#32765=CARTESIAN_POINT('Ctrl Pts',(-2.80852967755736,-0.319434907277002,
10.6598151083373));
#32766=CARTESIAN_POINT('Ctrl Pts',(-2.77999655012691,-0.158333333333255,
10.6450279038195));
#32767=CARTESIAN_POINT('Ctrl Pts',(-2.75983985593594,0.158333333333257,
10.6610058941037));
#32768=CARTESIAN_POINT('Ctrl Pts',(-2.76857308529266,0.319434907277011,
10.6914381411507));
#32769=CARTESIAN_POINT('Ctrl Pts',(-2.78973078923156,0.636309800094895,
10.7652887142333));
#32770=CARTESIAN_POINT('Ctrl Pts',(-2.81520148560987,0.794772684000449,
10.8229710284112));
#32771=CARTESIAN_POINT('Ctrl Pts',(-2.85020824756776,1.06847604194479,10.9184715141894));
#32772=CARTESIAN_POINT('Ctrl Pts',(-2.86603439018921,1.18514270861161,10.9623435382482));
#32773=CARTESIAN_POINT('Ctrl Pts',(-2.88253354530889,1.29999999999997,11.0087489647142));
#32774=CARTESIAN_POINT('Ctrl Pts',(-3.06242055860223,-1.29999999999949,
10.8768361729215));
#32775=CARTESIAN_POINT('Ctrl Pts',(-3.03267278550666,-1.18514270861128,
10.8427724582233));
#32776=CARTESIAN_POINT('Ctrl Pts',(-3.00261276335823,-1.06847604194463,
10.8115765723584));
#32777=CARTESIAN_POINT('Ctrl Pts',(-2.93244674093124,-0.794772684000459,
10.7461330936069));
#32778=CARTESIAN_POINT('Ctrl Pts',(-2.88343100137299,-0.636309800094882,
10.7071638759166));
#32779=CARTESIAN_POINT('Ctrl Pts',(-2.82021740568332,-0.319434907277,10.666908333352));
#32780=CARTESIAN_POINT('Ctrl Pts',(-2.79105344249383,-0.158333333333254,
10.6519528326215));
#32781=CARTESIAN_POINT('Ctrl Pts',(-2.77072506317317,0.158333333333256,
10.668100025496));
#32782=CARTESIAN_POINT('Ctrl Pts',(-2.7798575468528,0.31943490727701,10.6989198683978));
#32783=CARTESIAN_POINT('Ctrl Pts',(-2.80105893402106,0.636309800094892,
10.7726422267279));
#32784=CARTESIAN_POINT('Ctrl Pts',(-2.82711707716874,0.794772684000446,
10.830181207447));
#32785=CARTESIAN_POINT('Ctrl Pts',(-2.86065357629568,1.06847604194479,10.9245703549084));
#32786=CARTESIAN_POINT('Ctrl Pts',(-2.87540107879178,1.1851427086116,10.9677570528055));
#32787=CARTESIAN_POINT('Ctrl Pts',(-2.89037937596168,1.29999999999997,11.0132728841261));
#32788=CARTESIAN_POINT('Ctrl Pts',(-3.06815466520313,-1.29999999999948,
10.879276631911));
#32789=CARTESIAN_POINT('Ctrl Pts',(-3.03946963545971,-1.18514270861128,
10.8457621660883));
#32790=CARTESIAN_POINT('Ctrl Pts',(-3.01015132615301,-1.06847604194463,
10.8150076866289));
#32791=CARTESIAN_POINT('Ctrl Pts',(-2.94095716406855,-0.794772684000456,
10.7503348072978));
#32792=CARTESIAN_POINT('Ctrl Pts',(-2.89151463437421,-0.636309800094879,
10.7115234919949));
#32793=CARTESIAN_POINT('Ctrl Pts',(-2.82805721887487,-0.319434907276999,
10.6715838103291));
#32794=CARTESIAN_POINT('Ctrl Pts',(-2.79835809901693,-0.158333333333254,
10.656633107884));
#32795=CARTESIAN_POINT('Ctrl Pts',(-2.77792811427938,0.158333333333256,
10.6728825178909));
#32796=CARTESIAN_POINT('Ctrl Pts',(-2.78745064686552,0.319434907277009,
10.7038364701324));
#32797=CARTESIAN_POINT('Ctrl Pts',(-2.80877750206969,0.63630980009489,10.7773764406106));
#32798=CARTESIAN_POINT('Ctrl Pts',(-2.83527090747759,0.794772684000444,
10.8347736190766));
#32799=CARTESIAN_POINT('Ctrl Pts',(-2.86785556647318,1.06847604194479,10.9283947091163));
#32800=CARTESIAN_POINT('Ctrl Pts',(-2.88188448559708,1.1851427086116,10.9711253407065));
#32801=CARTESIAN_POINT('Ctrl Pts',(-2.89583763234629,1.29999999999996,11.0160615030121));
#32802=CARTESIAN_POINT('Ctrl Pts',(-3.07523784637402,-1.29999999999946,
10.8824189159388));
#32803=CARTESIAN_POINT('Ctrl Pts',(-3.04796476281486,-1.18514270861126,
10.849495529204));
#32804=CARTESIAN_POINT('Ctrl Pts',(-3.01962948296483,-1.06847604194461,
10.8192292580368));
#32805=CARTESIAN_POINT('Ctrl Pts',(-2.95171543213439,-0.794772684000441,
10.7554465854091));
#32806=CARTESIAN_POINT('Ctrl Pts',(-2.90168998820482,-0.636309800094867,
10.7168934624449));
#32807=CARTESIAN_POINT('Ctrl Pts',(-2.8378908573945,-0.319434907276993,
10.6773894319303));
#32808=CARTESIAN_POINT('Ctrl Pts',(-2.80745761776207,-0.158333333333251,
10.6625105926622));
#32809=CARTESIAN_POINT('Ctrl Pts',(-2.7869115402588,0.158333333333253,10.6788774623961));
#32810=CARTESIAN_POINT('Ctrl Pts',(-2.79701271806406,0.319434907277003,
10.7099064844615));
#32811=CARTESIAN_POINT('Ctrl Pts',(-2.81852503384429,0.636309800094878,
10.7831900258582));
#32812=CARTESIAN_POINT('Ctrl Pts',(-2.84549847764126,0.794772684000428,
10.8404745189034));
#32813=CARTESIAN_POINT('Ctrl Pts',(-2.87692789917283,1.06847604194477,10.9331029465521));
#32814=CARTESIAN_POINT('Ctrl Pts',(-2.89009076804454,1.18514270861158,10.9752324838597));
#32815=CARTESIAN_POINT('Ctrl Pts',(-2.90281187378179,1.29999999999994,11.0193961443673));
#32816=CARTESIAN_POINT('Ctrl Pts',(-3.08358965610494,-1.29999999999945,
10.8863527724723));
#32817=CARTESIAN_POINT('Ctrl Pts',(-3.05804567124122,-1.18514270861125,
10.8540971838029));
#32818=CARTESIAN_POINT('Ctrl Pts',(-3.03092169320698,-1.0684760419446,10.8243795583149));
#32819=CARTESIAN_POINT('Ctrl Pts',(-2.96460977751422,-0.794772684000435,
10.7615891011136));
#32820=CARTESIAN_POINT('Ctrl Pts',(-2.91395450626128,-0.636309800094863,
10.723269875));
#32821=CARTESIAN_POINT('Ctrl Pts',(-2.84972419210867,-0.319434907276991,
10.6843118023107));
#32822=CARTESIAN_POINT('Ctrl Pts',(-2.81832933467205,-0.158333333333249,
10.6696114794886));
#32823=CARTESIAN_POINT('Ctrl Pts',(-2.79752458508349,0.158333333333252,
10.686245596063));
#32824=CARTESIAN_POINT('Ctrl Pts',(-2.8082605562833,0.319434907277001,10.7174240573484));
#32825=CARTESIAN_POINT('Ctrl Pts',(-2.8298159803707,0.636309800094874,10.7905823439847));
#32826=CARTESIAN_POINT('Ctrl Pts',(-2.85717913317588,0.794772684000423,
10.847923536905));
#32827=CARTESIAN_POINT('Ctrl Pts',(-2.88712075511869,1.06847604194476,10.9394573178082));
#32828=CARTESIAN_POINT('Ctrl Pts',(-2.89923198379483,1.18514270861157,10.9808732955023));
#32829=CARTESIAN_POINT('Ctrl Pts',(-2.91049382245449,1.29999999999993,11.0240836687982));
#32830=CARTESIAN_POINT('Ctrl Pts',(-3.10080971693876,-1.29999999999934,
10.8936341625109));
#32831=CARTESIAN_POINT('Ctrl Pts',(-3.07833566280431,-1.18514270861116,
10.8631519636631));
#32832=CARTESIAN_POINT('Ctrl Pts',(-3.05335226645189,-1.06847604194452,
10.8348485035415));
#32833=CARTESIAN_POINT('Ctrl Pts',(-2.98983854045078,-0.794772684000373,
10.7744951708851));
#32834=CARTESIAN_POINT('Ctrl Pts',(-2.93783081929769,-0.636309800094812,
10.7367262126155));
#32835=CARTESIAN_POINT('Ctrl Pts',(-2.87309042237872,-0.319434907276965,
10.6984834504311));
#32836=CARTESIAN_POINT('Ctrl Pts',(-2.84049848157009,-0.158333333333237,
10.6833694821667));
#32837=CARTESIAN_POINT('Ctrl Pts',(-2.81968402648701,0.158333333333239,
10.6999957105264));
#32838=CARTESIAN_POINT('Ctrl Pts',(-2.83180795271723,0.319434907276975,
10.7313425331747));
#32839=CARTESIAN_POINT('Ctrl Pts',(-2.85344512895899,0.636309800094823,
10.8042529998644));
#32840=CARTESIAN_POINT('Ctrl Pts',(-2.881281674652,0.794772684000359,10.8620313005373));
#32841=CARTESIAN_POINT('Ctrl Pts',(-2.90806534832747,1.06847604194467,10.9515764346143));
#32842=CARTESIAN_POINT('Ctrl Pts',(-2.91801406667886,1.18514270861147,10.9916332152446));
#32843=CARTESIAN_POINT('Ctrl Pts',(-2.92631784348045,1.29999999999982,11.0329860059375));
#32844=CARTESIAN_POINT('Ctrl Pts',(-3.12726630276597,-1.29999999999915,
10.9037860597292));
#32845=CARTESIAN_POINT('Ctrl Pts',(-3.10990415514615,-1.18514270861097,
10.8753577686408));
#32846=CARTESIAN_POINT('Ctrl Pts',(-3.08851564146291,-1.06847604194435,
10.8487258397618));
#32847=CARTESIAN_POINT('Ctrl Pts',(-3.02980218501885,-0.794772684000252,
10.7913507124168));
#32848=CARTESIAN_POINT('Ctrl Pts',(-2.97608038840538,-0.636309800094717,
10.7541285055702));
#32849=CARTESIAN_POINT('Ctrl Pts',(-2.91005610250744,-0.319434907276919,
10.7175793582741));
#32850=CARTESIAN_POINT('Ctrl Pts',(-2.87460681156947,-0.158333333333213,
10.7030529564397));
#32851=CARTESIAN_POINT('Ctrl Pts',(-2.85267880346062,0.158333333333215,
10.7208784716313));
#32852=CARTESIAN_POINT('Ctrl Pts',(-2.86590325595896,0.319434907276927,
10.7534915361801));
#32853=CARTESIAN_POINT('Ctrl Pts',(-2.88786639021945,0.636309800094727,
10.8258180357411));
#32854=CARTESIAN_POINT('Ctrl Pts',(-2.91829508521574,0.794772684000243,
10.8822638836117));
#32855=CARTESIAN_POINT('Ctrl Pts',(-2.94066922555273,1.06847604194451,10.9684855749424));
#32856=CARTESIAN_POINT('Ctrl Pts',(-2.9472024446617,1.18514270861129,11.0066882228352));
#32857=CARTESIAN_POINT('Ctrl Pts',(-2.95058394657136,1.29999999999963,11.0457713432723));
#32858=CARTESIAN_POINT('Ctrl Pts',(-3.15602901483229,-1.29999999999882,
10.9157337896772));
#32859=CARTESIAN_POINT('Ctrl Pts',(-3.14419872081014,-1.18514270861068,
10.8897313639778));
#32860=CARTESIAN_POINT('Ctrl Pts',(-3.12675169145005,-1.06847604194409,
10.8650010651328));
#32861=CARTESIAN_POINT('Ctrl Pts',(-3.07346978110733,-0.794772684000054,
10.8108079950433));
#32862=CARTESIAN_POINT('Ctrl Pts',(-3.01816370804572,-0.63630980009456,
10.7738376644295));
#32863=CARTESIAN_POINT('Ctrl Pts',(-2.95126515113379,-0.31943490727684,
10.7385805017639));
#32864=CARTESIAN_POINT('Ctrl Pts',(-2.9128355854657,-0.158333333333174,
10.7245215983797));
#32865=CARTESIAN_POINT('Ctrl Pts',(-2.8907126092539,0.158333333333176,10.7425706729707));
#32866=CARTESIAN_POINT('Ctrl Pts',(-2.90693752767169,0.319434907276845,
10.7746836223076));
#32867=CARTESIAN_POINT('Ctrl Pts',(-2.92893953297227,0.636309800094568,
10.8466953240328));
#32868=CARTESIAN_POINT('Ctrl Pts',(-2.95940461178367,0.794772684000046,
10.9046636756723));
#32869=CARTESIAN_POINT('Ctrl Pts',(-2.97635305463127,1.06847604194425,10.9877859342387));
#32870=CARTESIAN_POINT('Ctrl Pts',(-2.97933175759914,1.185142708611,11.0236997722584));
#32871=CARTESIAN_POINT('Ctrl Pts',(-2.97795281062785,1.29999999999931,11.0595469025476));
#32872=CARTESIAN_POINT('Ctrl Pts',(-3.18010320518106,-1.29999999999858,
10.924026731429));
#32873=CARTESIAN_POINT('Ctrl Pts',(-3.17259939940327,-1.18514270861046,
10.9000631165806));
#32874=CARTESIAN_POINT('Ctrl Pts',(-3.15823173270695,-1.06847604194388,
10.8769284554676));
#32875=CARTESIAN_POINT('Ctrl Pts',(-3.1091826565641,-0.794772683999902,
10.8253978091835));
#32876=CARTESIAN_POINT('Ctrl Pts',(-3.05254831786319,-0.636309800094438,
10.7886958826654));
#32877=CARTESIAN_POINT('Ctrl Pts',(-2.98507404256285,-0.319434907276779,
10.7543604678475));
#32878=CARTESIAN_POINT('Ctrl Pts',(-2.94492658220406,-0.158333333333144,
10.7399863901776));
#32879=CARTESIAN_POINT('Ctrl Pts',(-2.92202390607915,0.158333333333146,
10.7589135934266));
#32880=CARTESIAN_POINT('Ctrl Pts',(-2.93866798081304,0.319434907276787,
10.7927720313494));
#32881=CARTESIAN_POINT('Ctrl Pts',(-2.96071475589337,0.636309800094449,
10.8645259076817));
#32882=CARTESIAN_POINT('Ctrl Pts',(-2.99356858890591,0.794772683999894,
10.9211606009691));
#32883=CARTESIAN_POINT('Ctrl Pts',(-3.00641322847654,1.06847604194404,11.0015499951531));
#32884=CARTESIAN_POINT('Ctrl Pts',(-3.00624339995034,1.18514270861077,11.0359634114943));
#32885=CARTESIAN_POINT('Ctrl Pts',(-3.00034377436861,1.29999999999906,11.0699926541552));
#32886=CARTESIAN_POINT('Ctrl Pts',(-3.19317119394676,-1.29999999999844,
10.9292052586356));
#32887=CARTESIAN_POINT('Ctrl Pts',(-3.18851667721922,-1.18514270861033,
10.905888404442));
#32888=CARTESIAN_POINT('Ctrl Pts',(-3.17612823403504,-1.06847604194377,
10.8833559052778));
#32889=CARTESIAN_POINT('Ctrl Pts',(-3.12964153469845,-0.794772683999815,
10.8331133416253));
#32890=CARTESIAN_POINT('Ctrl Pts',(-3.07159540712198,-0.636309800094369,
10.7973727984909));
#32891=CARTESIAN_POINT('Ctrl Pts',(-3.00380191880827,-0.319434907276744,
10.7635677244755));
#32892=CARTESIAN_POINT('Ctrl Pts',(-2.96290447793494,-0.158333333333126,
10.7487469719282));
#32893=CARTESIAN_POINT('Ctrl Pts',(-2.94019331992949,0.158333333333128,
10.7674662572841));
#32894=CARTESIAN_POINT('Ctrl Pts',(-2.95817659293092,0.319434907276751,
10.8010990163192));
#32895=CARTESIAN_POINT('Ctrl Pts',(-2.98012260412593,0.636309800094378,
10.8728450605019));
#32896=CARTESIAN_POINT('Ctrl Pts',(-3.01278690563514,0.794772683999808,
10.930407928881));
#32897=CARTESIAN_POINT('Ctrl Pts',(-3.02287677434149,1.06847604194393,11.0097570370282));
#32898=CARTESIAN_POINT('Ctrl Pts',(-3.02095452509254,1.18514270861064,11.0433115676966));
#32899=CARTESIAN_POINT('Ctrl Pts',(-3.01274249629816,1.29999999999891,11.0760733402908));
#32900=CARTESIAN_POINT('Ctrl Pts',(-3.20195356844581,-1.2999999999984,10.9325805430825));
#32901=CARTESIAN_POINT('Ctrl Pts',(-3.19905069408776,-1.18514270861029,
10.9098723006726));
#32902=CARTESIAN_POINT('Ctrl Pts',(-3.18791928835714,-1.06847604194373,
10.8878155849971));
#32903=CARTESIAN_POINT('Ctrl Pts',(-3.14319396070667,-0.794772683999789,
10.8383653164499));
#32904=CARTESIAN_POINT('Ctrl Pts',(-3.08471467087231,-0.636309800094348,
10.8026538736212));
#32905=CARTESIAN_POINT('Ctrl Pts',(-3.01669309422378,-0.319434907276734,
10.7692132537858));
#32906=CARTESIAN_POINT('Ctrl Pts',(-2.97494273212308,-0.158333333333121,
10.7545182980031));
#32907=CARTESIAN_POINT('Ctrl Pts',(-2.95200516165176,0.158333333333123,
10.7735019500123));
#32908=CARTESIAN_POINT('Ctrl Pts',(-2.97050921264184,0.319434907276741,
10.8073876617833));
#32909=CARTESIAN_POINT('Ctrl Pts',(-2.99243749225236,0.636309800094358,
10.8790747579997));
#32910=CARTESIAN_POINT('Ctrl Pts',(-3.02556140260726,0.794772683999782,
10.9366122936397));
#32911=CARTESIAN_POINT('Ctrl Pts',(-3.03400332614396,1.06847604194389,11.0150603449401));
#32912=CARTESIAN_POINT('Ctrl Pts',(-3.03091728399067,1.18514270861061,11.0480371272504));
#32913=CARTESIAN_POINT('Ctrl Pts',(-3.02109100378915,1.29999999999887,11.0800334372497));
#32914=CARTESIAN_POINT('Ctrl Pts',(-3.2078239063885,-1.29999999999838,10.9348154145648));
#32915=CARTESIAN_POINT('Ctrl Pts',(-3.20598833312576,-1.18514270861027,
10.9126326507061));
#32916=CARTESIAN_POINT('Ctrl Pts',(-3.19564031801075,-1.06847604194372,
10.8909578856118));
#32917=CARTESIAN_POINT('Ctrl Pts',(-3.15206888939482,-0.79477268399978,
10.8420584209926));
#32918=CARTESIAN_POINT('Ctrl Pts',(-3.09348408409014,-0.63630980009434,
10.8061442607962));
#32919=CARTESIAN_POINT('Ctrl Pts',(-3.02536870892628,-0.319434907276729,
10.7728771538103));
#32920=CARTESIAN_POINT('Ctrl Pts',(-2.98301636382883,-0.158333333333119,
10.7583098517379));
#32921=CARTESIAN_POINT('Ctrl Pts',(-2.95989991999098,0.158333333333121,
10.7775035462831));
#32922=CARTESIAN_POINT('Ctrl Pts',(-2.97870729740525,0.319434907276737,
10.8116079787124));
#32923=CARTESIAN_POINT('Ctrl Pts',(-3.00060901312884,0.63630980009435,10.8832717054751));
#32924=CARTESIAN_POINT('Ctrl Pts',(-3.03406590116684,0.794772683999772,
10.9407593352451));
#32925=CARTESIAN_POINT('Ctrl Pts',(-3.04141806022352,1.06847604194388,11.0185961538684));
#32926=CARTESIAN_POINT('Ctrl Pts',(-3.03755824404923,1.18514270861059,11.0511857312301));
#32927=CARTESIAN_POINT('Ctrl Pts',(-3.02665613446937,1.29999999999886,11.0826722113098));
#32928=CARTESIAN_POINT('Ctrl Pts',(-3.21827822516881,-1.29999999999833,
10.9385053407892));
#32929=CARTESIAN_POINT('Ctrl Pts',(-3.21831827069289,-1.18514270861023,
10.9172239362435));
#32930=CARTESIAN_POINT('Ctrl Pts',(-3.20933793812708,-1.06847604194368,
10.8962162353064));
#32931=CARTESIAN_POINT('Ctrl Pts',(-3.16775269548259,-0.794772683999748,
10.8483165536558));
#32932=CARTESIAN_POINT('Ctrl Pts',(-3.10890351858294,-0.636309800094315,
10.812154606619));
#32933=CARTESIAN_POINT('Ctrl Pts',(-3.04059454137874,-0.319434907276717,
10.7792317085672));
#32934=CARTESIAN_POINT('Ctrl Pts',(-2.99722861267192,-0.158333333333113,
10.7648411723961));
#32935=CARTESIAN_POINT('Ctrl Pts',(-2.97378898691106,0.158333333333115,
10.7844153481876));
#32936=CARTESIAN_POINT('Ctrl Pts',(-2.99308256531735,0.319434907276725,
10.8189529229403));
#32937=CARTESIAN_POINT('Ctrl Pts',(-3.01493552688533,0.636309800094325,
10.8905801274358));
#32938=CARTESIAN_POINT('Ctrl Pts',(-3.04902721113827,0.79477268399974,10.9479236125522));
#32939=CARTESIAN_POINT('Ctrl Pts',(-3.05446637157062,1.06847604194384,11.0246991870321));
#32940=CARTESIAN_POINT('Ctrl Pts',(-3.04923870066583,1.18514270861055,11.0566272492481));
#32941=CARTESIAN_POINT('Ctrl Pts',(-3.03642894784585,1.29999999999881,11.0872500723032));
#32942=CARTESIAN_POINT('Ctrl Pts',(-3.2303394252439,-1.29999999999813,10.9425619026323));
#32943=CARTESIAN_POINT('Ctrl Pts',(-3.23284776163168,-1.18514270861005,
10.9219129013773));
#32944=CARTESIAN_POINT('Ctrl Pts',(-3.22560190703575,-1.06847604194352,
10.9014572922326));
#32945=CARTESIAN_POINT('Ctrl Pts',(-3.18632840089931,-0.794772683999627,
10.8546475174401));
#32946=CARTESIAN_POINT('Ctrl Pts',(-3.12654679146467,-0.636309800094216,
10.8189703475746));
#32947=CARTESIAN_POINT('Ctrl Pts',(-3.05779687329653,-0.319434907276667,
10.7867111805289));
#32948=CARTESIAN_POINT('Ctrl Pts',(-3.01327450874528,-0.158333333333088,
10.7725141623555));
#32949=CARTESIAN_POINT('Ctrl Pts',(-2.98974250299873,0.15833333333309,10.7922101819601));
#32950=CARTESIAN_POINT('Ctrl Pts',(-3.0101308637112,0.319434907276676,10.8266298115445));
#32951=CARTESIAN_POINT('Ctrl Pts',(-3.03217400730282,0.636309800094226,
10.8979357227703));
#32952=CARTESIAN_POINT('Ctrl Pts',(-3.06689565791068,0.794772683999616,
10.9552203236505));
#32953=CARTESIAN_POINT('Ctrl Pts',(-3.06993147809271,1.06847604194367,11.0310329576894));
#32954=CARTESIAN_POINT('Ctrl Pts',(-3.06299302162609,1.18514270861036,11.0623753022289));
#32955=CARTESIAN_POINT('Ctrl Pts',(-3.04780201462427,1.2999999999986,11.0922435111674));
#32956=CARTESIAN_POINT('Ctrl Pts',(-3.24079513531022,-1.29999999999806,
10.9462274915081));
#32957=CARTESIAN_POINT('Ctrl Pts',(-3.24529551818108,-1.18514270860998,
10.9263349979427));
#32958=CARTESIAN_POINT('Ctrl Pts',(-3.23948544522855,-1.06847604194346,
10.9064610579923));
#32959=CARTESIAN_POINT('Ctrl Pts',(-3.20224379885544,-0.794772683999584,
10.860591143501));
#32960=CARTESIAN_POINT('Ctrl Pts',(-3.14205158607251,-0.636309800094183,
10.8248416467196));
#32961=CARTESIAN_POINT('Ctrl Pts',(-3.07300818112779,-0.31943490727665,
10.7930499844777));
#32962=CARTESIAN_POINT('Ctrl Pts',(-3.02732746867617,-0.15833333333308,
10.7792067503446));
#32963=CARTESIAN_POINT('Ctrl Pts',(-3.00360032053142,0.158333333333082,
10.7991416781415));
#32964=CARTESIAN_POINT('Ctrl Pts',(-3.02482853615089,0.319434907276658,
10.8335848462574));
#32965=CARTESIAN_POINT('Ctrl Pts',(-3.0470189317855,0.636309800094193,10.90462795134));
#32966=CARTESIAN_POINT('Ctrl Pts',(-3.08240549912536,0.794772683999574,
10.9617301143442));
#32967=CARTESIAN_POINT('Ctrl Pts',(-3.08340009269825,1.06847604194362,11.0366323287546));
#32968=CARTESIAN_POINT('Ctrl Pts',(-3.07498480978701,1.1851427086103,11.0674414679324));
#32969=CARTESIAN_POINT('Ctrl Pts',(-3.05772372126014,1.29999999999854,11.0966373530704));
#32970=CARTESIAN_POINT('Ctrl Pts',(-3.2461042721859,-1.29999999999804,10.9479547779649));
#32971=CARTESIAN_POINT('Ctrl Pts',(-3.25166886294995,-1.18514270860997,
10.9283516942736));
#32972=CARTESIAN_POINT('Ctrl Pts',(-3.24660822507569,-1.06847604194344,
10.9087271456776));
#32973=CARTESIAN_POINT('Ctrl Pts',(-3.2103707354848,-0.794772683999574,
10.86334092432));
#32974=CARTESIAN_POINT('Ctrl Pts',(-3.14977467070274,-0.636309800094174,
10.8278074737177));
#32975=CARTESIAN_POINT('Ctrl Pts',(-3.08057765298618,-0.319434907276646,
10.7962643145884));
#32976=CARTESIAN_POINT('Ctrl Pts',(-3.03449437995621,-0.158333333333078,
10.782386020323));
#32977=CARTESIAN_POINT('Ctrl Pts',(-3.01067167508799,0.15833333333308,10.8024375578468));
#32978=CARTESIAN_POINT('Ctrl Pts',(-3.03220630719915,0.319434907276654,
10.8370269173354));
#32979=CARTESIAN_POINT('Ctrl Pts',(-3.05435686985674,0.636309800094185,
10.9080702042062));
#32980=CARTESIAN_POINT('Ctrl Pts',(-3.08995186955548,0.794772683999564,
10.9652217061407));
#32981=CARTESIAN_POINT('Ctrl Pts',(-3.08994294375201,1.0684760419436,11.0396498899755));
#32982=CARTESIAN_POINT('Ctrl Pts',(-3.08083571066518,1.18514270861028,11.0701398337137));
#32983=CARTESIAN_POINT('Ctrl Pts',(-3.0626251081411,1.29999999999852,11.0989025182441));
#32984=CARTESIAN_POINT('Ctrl Pts',(-3.24914998256638,-1.29999999999804,
10.9489257242858));
#32985=CARTESIAN_POINT('Ctrl Pts',(-3.25533657941007,-1.18514270860996,
10.929470106966));
#32986=CARTESIAN_POINT('Ctrl Pts',(-3.25071124430535,-1.06847604194344,
10.9099789462566));
#32987=CARTESIAN_POINT('Ctrl Pts',(-3.21504806919795,-0.794772683999571,
10.8648683534842));
#32988=CARTESIAN_POINT('Ctrl Pts',(-3.15418675220007,-0.636309800094172,
10.8295019440878));
#32989=CARTESIAN_POINT('Ctrl Pts',(-3.08490169855022,-0.319434907276645,
10.7981023713605));
#32990=CARTESIAN_POINT('Ctrl Pts',(-3.03861899866046,-0.158333333333077,
10.7841677328696));
#32991=CARTESIAN_POINT('Ctrl Pts',(-3.0147430786694,0.158333333333079,10.8042843725331));
#32992=CARTESIAN_POINT('Ctrl Pts',(-3.0364346996967,0.319434907276653,10.8389786262426));
#32993=CARTESIAN_POINT('Ctrl Pts',(-3.05854295057592,0.636309800094182,
10.9100446506083));
#32994=CARTESIAN_POINT('Ctrl Pts',(-3.09423482136392,0.794772683999561,
10.9672494803309));
#32995=CARTESIAN_POINT('Ctrl Pts',(-3.0936531799886,1.0684760419436,11.0414062000157));
#32996=CARTESIAN_POINT('Ctrl Pts',(-3.08415726944502,1.18514270861028,11.0717062434621));
#32997=CARTESIAN_POINT('Ctrl Pts',(-3.06541721935728,1.29999999999851,11.1002066341807));
#32998=CARTESIAN_POINT('Ctrl Pts',(-3.2522037750961,-1.29999999999803,10.9498858595903));
#32999=CARTESIAN_POINT('Ctrl Pts',(-3.25902095733855,-1.18514270860995,
10.9305666068651));
#33000=CARTESIAN_POINT('Ctrl Pts',(-3.25483534210919,-1.06847604194343,
10.9112030885064));
#33001=CARTESIAN_POINT('Ctrl Pts',(-3.21974707033794,-0.794772683999564,
10.8663672249707));
#33002=CARTESIAN_POINT('Ctrl Pts',(-3.15859991758064,-0.636309800094167,
10.8311937863848));
#33003=CARTESIAN_POINT('Ctrl Pts',(-3.089226467721,-0.319434907276642,10.799939045965));
#33004=CARTESIAN_POINT('Ctrl Pts',(-3.04276163465701,-0.158333333333076,
10.7859277402349));
#33005=CARTESIAN_POINT('Ctrl Pts',(-3.01883418833475,0.158333333333078,
10.8061076516815));
#33006=CARTESIAN_POINT('Ctrl Pts',(-3.04067416343987,0.319434907276651,
10.8409169435151));
#33007=CARTESIAN_POINT('Ctrl Pts',(-3.06272970526287,0.636309800094177,
10.9120177369764));
#33008=CARTESIAN_POINT('Ctrl Pts',(-3.09850592289566,0.794772683999555,
10.969290063757));
#33009=CARTESIAN_POINT('Ctrl Pts',(-3.09735039907804,1.06847604194359,11.0431768350281));
#33010=CARTESIAN_POINT('Ctrl Pts',(-3.08746850869887,1.18514270861027,11.0732840274282));
#33011=CARTESIAN_POINT('Ctrl Pts',(-3.06820491138482,1.2999999999985,11.1015155667196));
#33012=CARTESIAN_POINT('Ctrl Pts',(-3.25602504189697,-1.29999999999801,
10.9510798888505));
#33013=CARTESIAN_POINT('Ctrl Pts',(-3.26363685807521,-1.18514270860993,
10.9319227517664));
#33014=CARTESIAN_POINT('Ctrl Pts',(-3.2600049829205,-1.06847604194341,10.9127134541495));
#33015=CARTESIAN_POINT('Ctrl Pts',(-3.22563944848708,-0.794772683999553,
10.8682156325821));
#33016=CARTESIAN_POINT('Ctrl Pts',(-3.16412692814332,-0.636309800094157,
10.8332933902027));
#33017=CARTESIAN_POINT('Ctrl Pts',(-3.09464460637555,-0.319434907276637,
10.8022185450546));
#33018=CARTESIAN_POINT('Ctrl Pts',(-3.0479593676407,-0.158333333333074,
10.788103923345));
#33019=CARTESIAN_POINT('Ctrl Pts',(-3.02396993643298,0.158333333333076,
10.8083605668864));
#33020=CARTESIAN_POINT('Ctrl Pts',(-3.04599441333248,0.319434907276646,
10.8433144176721));
#33021=CARTESIAN_POINT('Ctrl Pts',(-3.06797944317755,0.636309800094167,
10.9144639024002));
#33022=CARTESIAN_POINT('Ctrl Pts',(-3.10385470629991,0.794772683999542,
10.9718277275117));
#33023=CARTESIAN_POINT('Ctrl Pts',(-3.10197566521276,1.06847604194357,11.0453844124093));
#33024=CARTESIAN_POINT('Ctrl Pts',(-3.09160897176982,1.18514270861025,11.0752534399488));
#33025=CARTESIAN_POINT('Ctrl Pts',(-3.07168895214525,1.29999999999848,11.1031515316794));
#33026=CARTESIAN_POINT('Ctrl Pts',(-3.25983121780103,-1.29999999999798,
10.9522921169358));
#33027=CARTESIAN_POINT('Ctrl Pts',(-3.2682232328086,-1.18514270860991,10.9333152942735));
#33028=CARTESIAN_POINT('Ctrl Pts',(-3.26514019968536,-1.0684760419434,10.914266350886));
#33029=CARTESIAN_POINT('Ctrl Pts',(-3.23150811965428,-0.79477268399954,
10.87009286763));
#33030=CARTESIAN_POINT('Ctrl Pts',(-3.16968791589892,-0.636309800094147,
10.8353486978133));
#33031=CARTESIAN_POINT('Ctrl Pts',(-3.10010376764258,-0.319434907276632,
10.8044448005871));
#33032=CARTESIAN_POINT('Ctrl Pts',(-3.05315163017489,-0.158333333333071,
10.7902851974788));
#33033=CARTESIAN_POINT('Ctrl Pts',(-3.02910177510456,0.158333333333073,
10.8106178616161));
#33034=CARTESIAN_POINT('Ctrl Pts',(-3.05134352126923,0.319434907276641,
10.8456766004499));
#33035=CARTESIAN_POINT('Ctrl Pts',(-3.0732853111402,0.636309800094157,10.9168428086852));
#33036=CARTESIAN_POINT('Ctrl Pts',(-3.10929020858042,0.794772683999529,
10.9742631704055));
#33037=CARTESIAN_POINT('Ctrl Pts',(-3.1066698378272,1.06847604194355,11.0475104035141));
#33038=CARTESIAN_POINT('Ctrl Pts',(-3.09579807220139,1.18514270861023,11.0771646918295));
#33039=CARTESIAN_POINT('Ctrl Pts',(-3.07518880235454,1.29999999999846,11.1047672553249));
#33040=CARTESIAN_POINT('Ctrl Pts',(-3.26285879810893,-1.29999999999797,
10.9532835226745));
#33041=CARTESIAN_POINT('Ctrl Pts',(-3.27185662151802,-1.1851427086099,10.9344741764721));
#33042=CARTESIAN_POINT('Ctrl Pts',(-3.26920527733258,-1.06847604194339,
10.9155628521418));
#33043=CARTESIAN_POINT('Ctrl Pts',(-3.23616823431326,-0.794772683999533,
10.8716383198648));
#33044=CARTESIAN_POINT('Ctrl Pts',(-3.17416424763992,-0.636309800094141,
10.8369578318921));
#33045=CARTESIAN_POINT('Ctrl Pts',(-3.10450550169272,-0.319434907276629,
10.8061814921185));
#33046=CARTESIAN_POINT('Ctrl Pts',(-3.05729089109247,-0.15833333333307,
10.7920463667222));
#33047=CARTESIAN_POINT('Ctrl Pts',(-3.03319235162169,0.158333333333072,
10.8124410566994));
#33048=CARTESIAN_POINT('Ctrl Pts',(-3.05563863850475,0.319434907276638,
10.8475467077765));
#33049=CARTESIAN_POINT('Ctrl Pts',(-3.07757469698629,0.636309800094151,
10.9186926267006));
#33050=CARTESIAN_POINT('Ctrl Pts',(-3.1137177384153,0.794772683999522,10.9761189313738));
#33051=CARTESIAN_POINT('Ctrl Pts',(-3.1104911948604,1.06847604194355,11.0491337572892));
#33052=CARTESIAN_POINT('Ctrl Pts',(-3.09919727000925,1.18514270861022,11.0786371083924));
#33053=CARTESIAN_POINT('Ctrl Pts',(-3.07800607145667,1.29999999999845,11.106038397926));
#33054=CARTESIAN_POINT('Ctrl Pts',(-3.26512130110185,-1.29999999999797,
10.9540372474851));
#33055=CARTESIAN_POINT('Ctrl Pts',(-3.27456462137896,-1.1851427086099,10.9353646813646));
#33056=CARTESIAN_POINT('Ctrl Pts',(-3.27223346753816,-1.06847604194338,
10.9165610678225));
#33057=CARTESIAN_POINT('Ctrl Pts',(-3.23964664513232,-0.794772683999528,
10.8728182131305));
#33058=CARTESIAN_POINT('Ctrl Pts',(-3.17753465024573,-0.636309800094137,
10.838147852488));
#33059=CARTESIAN_POINT('Ctrl Pts',(-3.10782359105474,-0.319434907276627,
10.8074623493028));
#33060=CARTESIAN_POINT('Ctrl Pts',(-3.06038943072611,-0.158333333333069,
10.7933735951485));
#33061=CARTESIAN_POINT('Ctrl Pts',(-3.03625414615705,0.158333333333071,
10.8138154556009));
#33062=CARTESIAN_POINT('Ctrl Pts',(-3.0588676056342,0.319434907276636,10.8489397238093));
#33063=CARTESIAN_POINT('Ctrl Pts',(-3.08081297157187,0.636309800094147,
10.920054595231));
#33064=CARTESIAN_POINT('Ctrl Pts',(-3.1170765070553,0.794772683999518,10.9774660881753));
#33065=CARTESIAN_POINT('Ctrl Pts',(-3.11338943202109,1.06847604194354,11.0503134887088));
#33066=CARTESIAN_POINT('Ctrl Pts',(-3.10177040926063,1.18514270861021,11.0797134368291));
#33067=CARTESIAN_POINT('Ctrl Pts',(-3.08012836190243,1.29999999999844,11.106980392641));
#33068=CARTESIAN_POINT('Ctrl Pts',(-3.26700083590201,-1.29999999999796,
10.9546726147595));
#33069=CARTESIAN_POINT('Ctrl Pts',(-3.27680898774437,-1.18514270860989,
10.9361220819641));
#33070=CARTESIAN_POINT('Ctrl Pts',(-3.27474209984817,-1.06847604194337,
10.9174114201572));
#33071=CARTESIAN_POINT('Ctrl Pts',(-3.24253345793881,-0.794772683999523,
10.8738161182781));
#33072=CARTESIAN_POINT('Ctrl Pts',(-3.18035310750234,-0.636309800094134,
10.8391269232331));
#33073=CARTESIAN_POINT('Ctrl Pts',(-3.1106016129151,-0.319434907276625,
10.8085129890696));
#33074=CARTESIAN_POINT('Ctrl Pts',(-3.06296897051024,-0.158333333333068,
10.7944820510319));
#33075=CARTESIAN_POINT('Ctrl Pts',(-3.0388028643722,0.15833333333307,10.814963736934));
#33076=CARTESIAN_POINT('Ctrl Pts',(-3.06156451504281,0.319434907276634,
10.8500928419119));
#33077=CARTESIAN_POINT('Ctrl Pts',(-3.08352719265029,0.636309800094144,
10.9211707680412));
#33078=CARTESIAN_POINT('Ctrl Pts',(-3.11990372997025,0.794772683999513,
10.9785555320188));
#33079=CARTESIAN_POINT('Ctrl Pts',(-3.11582897433454,1.06847604194353,11.051268042067));
#33080=CARTESIAN_POINT('Ctrl Pts',(-3.10393309734347,1.18514270861021,11.0805887333396));
#33081=CARTESIAN_POINT('Ctrl Pts',(-3.08190515409146,1.29999999999843,11.1077555645489));
#33082=CARTESIAN_POINT('Ctrl Pts',(-3.26822071808255,-1.29999999999796,
10.9550877927237));
#33083=CARTESIAN_POINT('Ctrl Pts',(-3.27826398910814,-1.18514270860989,
10.936619089118));
#33084=CARTESIAN_POINT('Ctrl Pts',(-3.27636811928977,-1.06847604194337,
10.9179697712191));
#33085=CARTESIAN_POINT('Ctrl Pts',(-3.24440647697536,-0.794772683999522,
10.8744688609399));
#33086=CARTESIAN_POINT('Ctrl Pts',(-3.18218878382604,-0.636309800094133,
10.8397585327295));
#33087=CARTESIAN_POINT('Ctrl Pts',(-3.11241252899853,-0.319434907276625,
10.8091891951106));
#33088=CARTESIAN_POINT('Ctrl Pts',(-3.06464662184015,-0.158333333333068,
10.7952011106947));
#33089=CARTESIAN_POINT('Ctrl Pts',(-3.0404604264161,0.15833333333307,10.8157088562877));
#33090=CARTESIAN_POINT('Ctrl Pts',(-3.06332043523314,0.319434907276634,
10.8508386805889));
#33091=CARTESIAN_POINT('Ctrl Pts',(-3.08529713446789,0.636309800094143,
10.9218894186497));
#33092=CARTESIAN_POINT('Ctrl Pts',(-3.1217513001438,0.794772683999512,10.9792520038199));
#33093=CARTESIAN_POINT('Ctrl Pts',(-3.11742350878161,1.06847604194353,11.0518781349094));
#33094=CARTESIAN_POINT('Ctrl Pts',(-3.10534591028257,1.18514270861021,11.0811494049298));
#33095=CARTESIAN_POINT('Ctrl Pts',(-3.08306405380469,1.29999999999843,11.1082547838853));
#33096=CARTESIAN_POINT('Ctrl Pts',(-3.26878350127814,-1.29999999999796,
10.9552796922352));
#33097=CARTESIAN_POINT('Ctrl Pts',(-3.27893502398191,-1.18514270860989,
10.9368490790607));
#33098=CARTESIAN_POINT('Ctrl Pts',(-3.2771179959373,-1.06847604194337,10.9182281800829));
#33099=CARTESIAN_POINT('Ctrl Pts',(-3.24527055112992,-0.794772683999522,
10.8747705800738));
#33100=CARTESIAN_POINT('Ctrl Pts',(-3.18303660409327,-0.636309800094133,
10.8400492724346));
#33101=CARTESIAN_POINT('Ctrl Pts',(-3.11324920707446,-0.319434907276625,
10.8095001642765));
#33102=CARTESIAN_POINT('Ctrl Pts',(-3.06542132947862,-0.158333333333068,
10.7955324393821));
#33103=CARTESIAN_POINT('Ctrl Pts',(-3.04122585740674,0.15833333333307,10.8160522357225));
#33104=CARTESIAN_POINT('Ctrl Pts',(-3.06413141273467,0.319434907276633,
10.851182215591));
#33105=CARTESIAN_POINT('Ctrl Pts',(-3.08611491678922,0.636309800094143,
10.9222200294419));
#33106=CARTESIAN_POINT('Ctrl Pts',(-3.12260550379441,0.794772683999512,
10.9795716923723));
#33107=CARTESIAN_POINT('Ctrl Pts',(-3.11816081934627,1.06847604194353,11.0521581036447));
#33108=CARTESIAN_POINT('Ctrl Pts',(-3.10599913119212,1.1851427086102,11.0814068304583));
#33109=CARTESIAN_POINT('Ctrl Pts',(-3.08359969408964,1.29999999999843,11.1084843162373));
#33110=CARTESIAN_POINT('Ctrl Pts',(-3.26906484675215,-1.29999999999796,
10.9553756952532));
#33111=CARTESIAN_POINT('Ctrl Pts',(-3.27927044399567,-1.18514270860989,
10.9369641894471));
#33112=CARTESIAN_POINT('Ctrl Pts',(-3.27749281955508,-1.06847604194337,
10.9183575200967));
#33113=CARTESIAN_POINT('Ctrl Pts',(-3.24570251215918,-0.794772683999522,
10.8749215248163));
#33114=CARTESIAN_POINT('Ctrl Pts',(-3.18346062881311,-0.636309800094133,
10.8401944891827));
#33115=CARTESIAN_POINT('Ctrl Pts',(-3.11366771647733,-0.319434907276625,
10.8096554267729));
#33116=CARTESIAN_POINT('Ctrl Pts',(-3.06580876385529,-0.158333333333068,
10.7956979946858));
#33117=CARTESIAN_POINT('Ctrl Pts',(-3.04160865286627,0.15833333333307,10.8162238206007));
#33118=CARTESIAN_POINT('Ctrl Pts',(-3.06453701000585,0.319434907276633,
10.8513538442853));
#33119=CARTESIAN_POINT('Ctrl Pts',(-3.08652398303935,0.636309800094143,
10.9223851210484));
#33120=CARTESIAN_POINT('Ctrl Pts',(-3.12303290043782,0.794772683999512,
10.9797311847854));
#33121=CARTESIAN_POINT('Ctrl Pts',(-3.1185297481833,1.06847604194353,11.0522977658325));
#33122=CARTESIAN_POINT('Ctrl Pts',(-3.10632597148495,1.18514270861021,11.0815352746523));
#33123=CARTESIAN_POINT('Ctrl Pts',(-3.08386766584099,1.29999999999843,11.1085989082136));
#33124=CARTESIAN_POINT('Ctrl Pts',(-3.26929927812004,-1.29999999999795,
10.9554557230908));
#33125=CARTESIAN_POINT('Ctrl Pts',(-3.27954991189458,-1.18514270860989,
10.9370601705783));
#33126=CARTESIAN_POINT('Ctrl Pts',(-3.27780511729567,-1.06847604194337,
10.9184653664804));
#33127=CARTESIAN_POINT('Ctrl Pts',(-3.24606245350732,-0.794772683999522,
10.875047338114));
#33128=CARTESIAN_POINT('Ctrl Pts',(-3.18381406354817,-0.636309800094132,
10.8403153969248));
#33129=CARTESIAN_POINT('Ctrl Pts',(-3.11401660292878,-0.319434907276625,
10.8097846479383));
#33130=CARTESIAN_POINT('Ctrl Pts',(-3.06613173190375,-0.158333333333067,
10.7958358224271));
#33131=CARTESIAN_POINT('Ctrl Pts',(-3.04192775500594,0.15833333333307,10.8163666756604));
#33132=CARTESIAN_POINT('Ctrl Pts',(-3.06487510153954,0.319434907276633,
10.8514967520241));
#33133=CARTESIAN_POINT('Ctrl Pts',(-3.08686498759334,0.636309800094142,
10.922522557656));
#33134=CARTESIAN_POINT('Ctrl Pts',(-3.1233892413128,0.794772683999511,10.9798638833143));
#33135=CARTESIAN_POINT('Ctrl Pts',(-3.11883736264261,1.06847604194353,11.0524139469481));
#33136=CARTESIAN_POINT('Ctrl Pts',(-3.10659849600036,1.1851427086102,11.0816421288434));
#33137=CARTESIAN_POINT('Ctrl Pts',(-3.08409110232845,1.29999999999843,11.1086942583318));
#33138=CARTESIAN_POINT('Ctrl Pts',(-3.26946335327275,-1.29999999999796,
10.9555117735233));
#33139=CARTESIAN_POINT('Ctrl Pts',(-3.27974548388032,-1.18514270860989,
10.9371274226514));
#33140=CARTESIAN_POINT('Ctrl Pts',(-3.27802365958171,-1.06847604194337,
10.9185409361608));
#33141=CARTESIAN_POINT('Ctrl Pts',(-3.24631436378593,-0.794772683999522,
10.8751354604371));
#33142=CARTESIAN_POINT('Ctrl Pts',(-3.18406152138737,-0.636309800094133,
10.8403999564982));
#33143=CARTESIAN_POINT('Ctrl Pts',(-3.11426089875868,-0.319434907276625,
10.8098749994742));
#33144=CARTESIAN_POINT('Ctrl Pts',(-3.06635782253387,-0.158333333333068,
10.7959322775262));
#33145=CARTESIAN_POINT('Ctrl Pts',(-3.04215113968003,0.15833333333307,10.8164666513532));
#33146=CARTESIAN_POINT('Ctrl Pts',(-3.06511180759166,0.319434907276633,
10.8515967284603));
#33147=CARTESIAN_POINT('Ctrl Pts',(-3.08710377997276,0.636309800094143,
10.9226186504884));
#33148=CARTESIAN_POINT('Ctrl Pts',(-3.12363884507739,0.794772683999512,
10.9799565735776));
#33149=CARTESIAN_POINT('Ctrl Pts',(-3.11905284184813,1.06847604194353,11.052495096842));
#33150=CARTESIAN_POINT('Ctrl Pts',(-3.10678938233382,1.1851427086102,11.0817167861432));
#33151=CARTESIAN_POINT('Ctrl Pts',(-3.08424757417498,1.29999999999843,11.1087609258417));
#33152=CARTESIAN_POINT('Ctrl Pts',(-3.26955712717019,-1.29999999999795,
10.9555437816027));
#33153=CARTESIAN_POINT('Ctrl Pts',(-3.27985727277926,-1.18514270860989,
10.9371658112677));
#33154=CARTESIAN_POINT('Ctrl Pts',(-3.2781485829776,-1.06847604194337,10.9185840677267));
#33155=CARTESIAN_POINT('Ctrl Pts',(-3.24645835555544,-0.794772683999521,
10.875185766011));
#33156=CARTESIAN_POINT('Ctrl Pts',(-3.18420292236256,-0.636309800094132,
10.8404482870144));
#33157=CARTESIAN_POINT('Ctrl Pts',(-3.11440050346004,-0.319434907276625,
10.8099266281638));
#33158=CARTESIAN_POINT('Ctrl Pts',(-3.0664870875896,-0.158333333333067,
10.7959873145624));
#33159=CARTESIAN_POINT('Ctrl Pts',(-3.04227885824284,0.15833333333307,10.8165237003086));
#33160=CARTESIAN_POINT('Ctrl Pts',(-3.06524709039278,0.319434907276633,
10.8516538385203));
#33161=CARTESIAN_POINT('Ctrl Pts',(-3.08724021216317,0.636309800094142,
10.922673591622));
#33162=CARTESIAN_POINT('Ctrl Pts',(-3.12378140786306,0.794772683999511,
10.980009621591));
#33163=CARTESIAN_POINT('Ctrl Pts',(-3.11917592303689,1.06847604194353,11.052541528731));
#33164=CARTESIAN_POINT('Ctrl Pts',(-3.10689843573048,1.1851427086102,11.0817594789404));
#33165=CARTESIAN_POINT('Ctrl Pts',(-3.08433700484887,1.29999999999843,11.1087990043302));
#33166=CARTESIAN_POINT('Ctrl Pts',(-3.27860149639123,-1.29999999999811,
10.9586383734117));
#33167=CARTESIAN_POINT('Ctrl Pts',(-3.29063514544287,-1.18514270861003,
10.9408820776598));
#33168=CARTESIAN_POINT('Ctrl Pts',(-3.29019168489462,-1.0684760419435,10.9227606023519));
#33169=CARTESIAN_POINT('Ctrl Pts',(-3.26034258310117,-0.794772683999615,
10.8800527313739));
#33170=CARTESIAN_POINT('Ctrl Pts',(-3.19785238484134,-0.636309800094207,
10.8451050522886));
#33171=CARTESIAN_POINT('Ctrl Pts',(-3.12787622340848,-0.319434907276662,
10.8149018513781));
#33172=CARTESIAN_POINT('Ctrl Pts',(-3.07894950238631,-0.158333333333086,
10.8013109843307));
#33173=CARTESIAN_POINT('Ctrl Pts',(-3.0545921000759,0.158333333333088,10.8220415825818));
#33174=CARTESIAN_POINT('Ctrl Pts',(-3.07830078447487,0.319434907276671,
10.8571643390185));
#33175=CARTESIAN_POINT('Ctrl Pts',(-3.10041572132,0.636309800094218,10.9279621035605));
#33176=CARTESIAN_POINT('Ctrl Pts',(-3.1375622532135,0.794772683999603,10.9851003389286));
#33177=CARTESIAN_POINT('Ctrl Pts',(-3.13107245976098,1.06847604194366,11.0569991517836));
#33178=CARTESIAN_POINT('Ctrl Pts',(-3.11743471538953,1.18514270861034,11.0858639693406));
#33179=CARTESIAN_POINT('Ctrl Pts',(-3.0929684177617,1.29999999999859,11.1124712724833));
#33180=CARTESIAN_POINT('Ctrl Pts',(-3.29087914694721,-1.29999999999912,
10.9624030458906));
#33181=CARTESIAN_POINT('Ctrl Pts',(-3.30552730370085,-1.18514270861095,
10.945066268376));
#33182=CARTESIAN_POINT('Ctrl Pts',(-3.3069203004573,-1.06847604194433,10.9273522227033));
#33183=CARTESIAN_POINT('Ctrl Pts',(-3.27951633035355,-0.794772684000236,
10.8855576685992));
#33184=CARTESIAN_POINT('Ctrl Pts',(-3.21585242742383,-0.636309800094705,
10.8514266221781));
#33185=CARTESIAN_POINT('Ctrl Pts',(-3.14575898006573,-0.319434907276912,
10.8215319562725));
#33186=CARTESIAN_POINT('Ctrl Pts',(-3.09649779902851,-0.15833333333321,
10.8071774067706));
#33187=CARTESIAN_POINT('Ctrl Pts',(-3.07196064508898,0.158333333333212,
10.8281430733825));
#33188=CARTESIAN_POINT('Ctrl Pts',(-3.09589251350698,0.319434907276919,
10.8641713452021));
#33189=CARTESIAN_POINT('Ctrl Pts',(-3.11761911521719,0.636309800094713,
10.935329305927));
#33190=CARTESIAN_POINT('Ctrl Pts',(-3.15506335099256,0.794772684000226,
10.9927733519278));
#33191=CARTESIAN_POINT('Ctrl Pts',(-3.14637586894705,1.06847604194449,11.0635105079469));
#33192=CARTESIAN_POINT('Ctrl Pts',(-3.1312833583335,1.18514270861127,11.0915216415227));
#33193=CARTESIAN_POINT('Ctrl Pts',(-3.10485882618096,1.2999999999996,11.1169244149035));
#33194=CARTESIAN_POINT('Ctrl Pts',(-3.30924538286601,-1.2999999999992,10.9680453426394));
#33195=CARTESIAN_POINT('Ctrl Pts',(-3.32757099145425,-1.18514270861102,
10.9516278490388));
#33196=CARTESIAN_POINT('Ctrl Pts',(-3.33159804337833,-1.06847604194439,
10.9346635406921));
#33197=CARTESIAN_POINT('Ctrl Pts',(-3.30786881262129,-0.794772684000279,
10.8942093432592));
#33198=CARTESIAN_POINT('Ctrl Pts',(-3.24331509553749,-0.63630980009474,
10.8602193379614));
#33199=CARTESIAN_POINT('Ctrl Pts',(-3.17260211198495,-0.31943490727693,
10.8313189415465));
#33200=CARTESIAN_POINT('Ctrl Pts',(-3.1212001718748,-0.158333333333219,
10.8178261868591));
#33201=CARTESIAN_POINT('Ctrl Pts',(-3.09633320761107,0.158333333333221,
10.8392273848434));
#33202=CARTESIAN_POINT('Ctrl Pts',(-3.1220499431571,0.319434907276938,10.8748551818682));
#33203=CARTESIAN_POINT('Ctrl Pts',(-3.14377740756195,0.63630980009475,10.9458534895315));
#33204=CARTESIAN_POINT('Ctrl Pts',(-3.18158047197996,0.79477268400027,11.0038982027768));
#33205=CARTESIAN_POINT('Ctrl Pts',(-3.16919220103572,1.06847604194455,11.0733388251436));
#33206=CARTESIAN_POINT('Ctrl Pts',(-3.15161288425918,1.18514270861134,11.100402316501));
#33207=CARTESIAN_POINT('Ctrl Pts',(-3.12181667416719,1.29999999999968,11.1244710268218));
#33208=CARTESIAN_POINT('Ctrl Pts',(-3.3243274772242,-1.29999999999955,10.9730006918154));
#33209=CARTESIAN_POINT('Ctrl Pts',(-3.34588851006542,-1.18514270861134,
10.9571288525117));
#33210=CARTESIAN_POINT('Ctrl Pts',(-3.35220225995525,-1.06847604194468,
10.9406718024574));
#33211=CARTESIAN_POINT('Ctrl Pts',(-3.33156401143583,-0.794772684000493,
10.9013007707052));
#33212=CARTESIAN_POINT('Ctrl Pts',(-3.26575478710962,-0.636309800094912,
10.868086218826));
#33213=CARTESIAN_POINT('Ctrl Pts',(-3.19479764779382,-0.319434907277016,
10.8396875638873));
#33214=CARTESIAN_POINT('Ctrl Pts',(-3.14252835935329,-0.158333333333261,
10.825779426311));
#33215=CARTESIAN_POINT('Ctrl Pts',(-3.11752885059753,0.158333333333263,
10.8473618163122));
#33216=CARTESIAN_POINT('Ctrl Pts',(-3.14392467480981,0.319434907277023,
10.8836346317217));
#33217=CARTESIAN_POINT('Ctrl Pts',(-3.16573979918509,0.636309800094921,
10.9544015971221));
#33218=CARTESIAN_POINT('Ctrl Pts',(-3.20491078620108,0.794772684000484,
11.0116782649417));
#33219=CARTESIAN_POINT('Ctrl Pts',(-3.18926926156555,1.06847604194484,11.0802325544955));
#33220=CARTESIAN_POINT('Ctrl Pts',(-3.16929090560949,1.18514270861166,11.106889174787));
#33221=CARTESIAN_POINT('Ctrl Pts',(-3.13610483013649,1.30000000000003,11.1305278036089));
#33222=CARTESIAN_POINT('Ctrl Pts',(-3.33687491329961,-1.30000000000013,
10.9763612687376));
#33223=CARTESIAN_POINT('Ctrl Pts',(-3.36075240801907,-1.18514270861187,
10.9612527084206));
#33224=CARTESIAN_POINT('Ctrl Pts',(-3.36875682745956,-1.06847604194516,
10.9453628297242));
#33225=CARTESIAN_POINT('Ctrl Pts',(-3.35057865835347,-0.794772684000851,
10.9068490294177));
#33226=CARTESIAN_POINT('Ctrl Pts',(-3.28443962791702,-0.636309800095197,
10.873385773417));
#33227=CARTESIAN_POINT('Ctrl Pts',(-3.21328105992889,-0.319434907277159,
10.8454018207699));
#33228=CARTESIAN_POINT('Ctrl Pts',(-3.15982488509512,-0.158333333333332,
10.8318180571383));
#33229=CARTESIAN_POINT('Ctrl Pts',(-3.13444040097792,0.158333333333334,
10.8539097309621));
#33230=CARTESIAN_POINT('Ctrl Pts',(-3.16145464955745,0.319434907277167,
10.8905991594872));
#33231=CARTESIAN_POINT('Ctrl Pts',(-3.18306078463709,0.636309800095206,
10.9615168342609));
#33232=CARTESIAN_POINT('Ctrl Pts',(-3.22263648930952,0.79477268400084,11.0189791881958));
#33233=CARTESIAN_POINT('Ctrl Pts',(-3.20470961432298,1.06847604194532,11.0864845545939));
#33234=CARTESIAN_POINT('Ctrl Pts',(-3.18318073063071,1.18514270861219,11.1124051525384));
#33235=CARTESIAN_POINT('Ctrl Pts',(-3.14788284317166,1.30000000000061,11.1350257766339));
#33236=CARTESIAN_POINT('Ctrl Pts',(-3.34312043552664,-1.30000000000013,
10.9780717341714));
#33237=CARTESIAN_POINT('Ctrl Pts',(-3.36817625250943,-1.18514270861187,
10.9633184123726));
#33238=CARTESIAN_POINT('Ctrl Pts',(-3.3770361693725,-1.06847604194516,10.9476988830842));
#33239=CARTESIAN_POINT('Ctrl Pts',(-3.36008858049118,-0.794772684000851,
10.9096135331669));
#33240=CARTESIAN_POINT('Ctrl Pts',(-3.29374448453208,-0.636309800095197,
10.876080714948));
#33241=CARTESIAN_POINT('Ctrl Pts',(-3.22246485929502,-0.319434907277159,
10.8483292952626));
#33242=CARTESIAN_POINT('Ctrl Pts',(-3.16838675811195,-0.158333333333332,
10.8349383562734));
#33243=CARTESIAN_POINT('Ctrl Pts',(-3.14286241424647,0.158333333333334,
10.8572187973924));
#33244=CARTESIAN_POINT('Ctrl Pts',(-3.17031238807969,0.319434907277167,
10.8939627249896));
#33245=CARTESIAN_POINT('Ctrl Pts',(-3.19184909015918,0.636309800095206,
10.9649130969802));
#33246=CARTESIAN_POINT('Ctrl Pts',(-3.23156943363573,0.79477268400084,11.0225410569458));
#33247=CARTESIAN_POINT('Ctrl Pts',(-3.21244012754108,1.06847604194532,11.0895917213652));
#33248=CARTESIAN_POINT('Ctrl Pts',(-3.19010469464416,1.18514270861219,11.1151799568387));
#33249=CARTESIAN_POINT('Ctrl Pts',(-3.15371419664804,1.30000000000061,11.1373326796307));
#33250=CARTESIAN_POINT('',(-3.07975929592511,1.2,11.0752525955301));
#33251=CARTESIAN_POINT('Ctrl Pts',(-3.07975929592511,1.2,11.0752525955301));
#33252=CARTESIAN_POINT('Ctrl Pts',(-3.05872636744548,1.21680769549872,11.0704989090906));
#33253=CARTESIAN_POINT('Ctrl Pts',(-3.03710141769083,1.23314403937139,11.0667390106653));
#33254=CARTESIAN_POINT('Ctrl Pts',(-2.99520540299999,1.26665353031124,11.0569415951956));
#33255=CARTESIAN_POINT('Ctrl Pts',(-2.97413477718184,1.28321842329864,11.0523060114257));
#33256=CARTESIAN_POINT('Ctrl Pts',(-2.95338171769412,1.29999999999958,11.0470815470424));
#33257=CARTESIAN_POINT('',(-3.2008348383287,0.653834841336403,10.9758649786952));
#33258=CARTESIAN_POINT('Ctrl Pts',(-3.20083483831068,0.653834841321624,
10.975864978764));
#33259=CARTESIAN_POINT('Ctrl Pts',(-3.18812833935079,0.719511596407524,
10.9866363926712));
#33260=CARTESIAN_POINT('Ctrl Pts',(-3.17771111571533,0.767412490766721,
10.9953791471888));
#33261=CARTESIAN_POINT('Ctrl Pts',(-3.13847134847367,0.94981031949708,11.0280199746604));
#33262=CARTESIAN_POINT('Ctrl Pts',(-3.11682163850512,1.04818118464467,11.0457982331948));
#33263=CARTESIAN_POINT('Ctrl Pts',(-3.07975929592511,1.2,11.0752525955301));
#33264=CARTESIAN_POINT('',(-3.3059688760626,-0.653834841531101,10.8841647344419));
#33265=CARTESIAN_POINT('Ctrl Pts',(-3.30596887606259,-0.653834841531102,
10.8841647344419));
#33266=CARTESIAN_POINT('Ctrl Pts',(-3.26765010478892,-0.575768210610585,
10.8677496595377));
#33267=CARTESIAN_POINT('Ctrl Pts',(-3.23494824939066,-0.493706163102552,
10.8548265221935));
#33268=CARTESIAN_POINT('Ctrl Pts',(-3.18709017845533,-0.337903894569622,
10.8381694530451));
#33269=CARTESIAN_POINT('Ctrl Pts',(-3.16979179495297,-0.2654146213422,10.8335054310253));
#33270=CARTESIAN_POINT('Ctrl Pts',(-3.14556133124211,-0.129502257227768,
10.831330995582));
#33271=CARTESIAN_POINT('Ctrl Pts',(-3.13750239985805,-0.0665294992617646,
10.8328438160244));
#33272=CARTESIAN_POINT('Ctrl Pts',(-3.12727067311581,0.0594283132875214,
10.8412732840013));
#33273=CARTESIAN_POINT('Ctrl Pts',(-3.1250264806205,0.122541336619068,10.8482282183473));
#33274=CARTESIAN_POINT('Ctrl Pts',(-3.12729278947957,0.25988248099301,10.8687757330099));
#33275=CARTESIAN_POINT('Ctrl Pts',(-3.13313315594363,0.333772875107173,
10.8833608794714));
#33276=CARTESIAN_POINT('Ctrl Pts',(-3.15645864391337,0.491496380642283,
10.9217822007945));
#33277=CARTESIAN_POINT('Ctrl Pts',(-3.17560601109368,0.57490233849731,10.9471353939645));
#33278=CARTESIAN_POINT('Ctrl Pts',(-3.20083483821487,0.653834841358134,
10.9758649787354));
#33279=CARTESIAN_POINT('',(-3.25181112747254,-1.2,10.9320536426002));
#33280=CARTESIAN_POINT('Ctrl Pts',(-3.25181112747254,-1.2,10.9320536426002));
#33281=CARTESIAN_POINT('Ctrl Pts',(-3.26281768457294,-1.12280248951958,
10.9224634147306));
#33282=CARTESIAN_POINT('Ctrl Pts',(-3.27215610527124,-1.0521071107758,10.9142855469299));
#33283=CARTESIAN_POINT('Ctrl Pts',(-3.30019612230759,-0.767168051992084,
10.8893756587268));
#33284=CARTESIAN_POINT('Ctrl Pts',(-3.30337667056459,-0.700407703040203,
10.8864908385427));
#33285=CARTESIAN_POINT('Ctrl Pts',(-3.30596887606259,-0.6538348415311,10.8841647344419));
#33286=CARTESIAN_POINT('Ctrl Pts',(-3.12979327626223,-1.2999999999991,10.904982327606));
#33287=CARTESIAN_POINT('Ctrl Pts',(-3.15020519847771,-1.28299035195331,
10.9100057513286));
#33288=CARTESIAN_POINT('Ctrl Pts',(-3.15975174726777,-1.27543828608662,
10.9118308894838));
#33289=CARTESIAN_POINT('Ctrl Pts',(-3.20107070619102,-1.24116690344093,
10.9215350399886));
#33290=CARTESIAN_POINT('Ctrl Pts',(-3.21071565722415,-1.23311873582876,
10.9238506811936));
#33291=CARTESIAN_POINT('Ctrl Pts',(-3.22591635566606,-1.22085268075416,
10.9269247721703));
#33292=CARTESIAN_POINT('Ctrl Pts',(-3.22669721991101,-1.22026908223654,
10.9270235897164));
#33293=CARTESIAN_POINT('Ctrl Pts',(-3.23909005932958,-1.210183748322,10.929622486052));
#33294=CARTESIAN_POINT('Ctrl Pts',(-3.24523385162528,-1.205183253303,10.9309097562926));
#33295=CARTESIAN_POINT('Ctrl Pts',(-3.25181112747254,-1.2,10.9320536426002));
#33296=CARTESIAN_POINT('Origin',(0.,1.25,7.2));
#33297=CARTESIAN_POINT('Origin',(0.,1.2,7.2));
#33298=CARTESIAN_POINT('Origin',(0.,0.92691742076555,7.2));
#33299=CARTESIAN_POINT('Origin',(0.,0.653834841531101,7.2));
#33300=CARTESIAN_POINT('Origin',(0.,0.,7.2));
#33301=CARTESIAN_POINT('Origin',(0.,-0.653834841531101,7.2));
#33302=CARTESIAN_POINT('Origin',(0.,-0.926917420765551,7.2));
#33303=CARTESIAN_POINT('Origin',(0.,-1.2,7.2));
#33304=CARTESIAN_POINT('Origin',(0.,-1.25,7.2));
#33305=CARTESIAN_POINT('Ctrl Pts',(-3.58611066068418,-1.30000000000019,
10.7480011546782));
#33306=CARTESIAN_POINT('Ctrl Pts',(-3.56027544999381,-1.18514270861191,
10.781876711649));
#33307=CARTESIAN_POINT('Ctrl Pts',(-3.53249270107504,-1.06847604194518,
10.8014150897762));
#33308=CARTESIAN_POINT('Ctrl Pts',(-3.46380979024152,-0.794772684000851,
10.8134309006175));
#33309=CARTESIAN_POINT('Ctrl Pts',(-3.41064942873151,-0.636309800095197,
10.7679043872394));
#33310=CARTESIAN_POINT('Ctrl Pts',(-3.34233892867367,-0.319434907277159,
10.7390693321139));
#33311=CARTESIAN_POINT('Ctrl Pts',(-3.30866559173879,-0.158333333333333,
10.7079289458242));
#33312=CARTESIAN_POINT('Ctrl Pts',(-3.2838391847674,0.158333333333334,10.7309845243923));
#33313=CARTESIAN_POINT('Ctrl Pts',(-3.29150406597897,0.319434907277167,
10.7861661143534));
#33314=CARTESIAN_POINT('Ctrl Pts',(-3.31165271079404,0.636309800095206,
10.8599560755972));
#33315=CARTESIAN_POINT('Ctrl Pts',(-3.33806698632524,0.79477268400084,10.929441865611));
#33316=CARTESIAN_POINT('Ctrl Pts',(-3.37417219528941,1.06847604194587,10.9502776169276));
#33317=CARTESIAN_POINT('Ctrl Pts',(-3.39063227265752,1.18514270861327,10.9430989210106));
#33318=CARTESIAN_POINT('Ctrl Pts',(-3.40792382026295,1.30000000000221,10.9197225044723));
#33319=CARTESIAN_POINT('Ctrl Pts',(-3.58274121447438,-1.30000000000018,
10.7359200632382));
#33320=CARTESIAN_POINT('Ctrl Pts',(-3.55620374541987,-1.18514270861191,
10.767524552013));
#33321=CARTESIAN_POINT('Ctrl Pts',(-3.52792852769938,-1.06847604194518,
10.7853891857851));
#33322=CARTESIAN_POINT('Ctrl Pts',(-3.45859257127325,-0.794772684000847,
10.7949182499019));
#33323=CARTESIAN_POINT('Ctrl Pts',(-3.40573136963309,-0.636309800095194,
10.7497140504956));
#33324=CARTESIAN_POINT('Ctrl Pts',(-3.3375004212098,-0.319434907277158,
10.7207477256613));
#33325=CARTESIAN_POINT('Ctrl Pts',(-3.30384439394133,-0.158333333333332,
10.690485409397));
#33326=CARTESIAN_POINT('Ctrl Pts',(-3.27942269203529,0.158333333333333,
10.7133022639117));
#33327=CARTESIAN_POINT('Ctrl Pts',(-3.28760112792004,0.319434907277165,
10.7672871264616));
#33328=CARTESIAN_POINT('Ctrl Pts',(-3.30823759882109,0.636309800095203,
10.840884912149));
#33329=CARTESIAN_POINT('Ctrl Pts',(-3.33455638238823,0.794772684000836,
10.9099482753614));
#33330=CARTESIAN_POINT('Ctrl Pts',(-3.37125653661945,1.06847604194586,10.9333212751551));
#33331=CARTESIAN_POINT('Ctrl Pts',(-3.38807550314534,1.18514270861327,10.9279007194989));
#33332=CARTESIAN_POINT('Ctrl Pts',(-3.40582729930512,1.3000000000022,10.9069423026308));
#33333=CARTESIAN_POINT('Ctrl Pts',(-3.57558296861516,-1.30000000000236,
10.7121202278766));
#33334=CARTESIAN_POINT('Ctrl Pts',(-3.54899722098252,-1.18514270861389,
10.7382144502947));
#33335=CARTESIAN_POINT('Ctrl Pts',(-3.52050276185225,-1.06847604194697,
10.7521771288085));
#33336=CARTESIAN_POINT('Ctrl Pts',(-3.45026535556835,-0.794772684002182,
10.7564074160735));
#33337=CARTESIAN_POINT('Ctrl Pts',(-3.39573104119172,-0.636309800096262,
10.7133992517982));
#33338=CARTESIAN_POINT('Ctrl Pts',(-3.3270486465882,-0.319434907277695,
10.6845828030105));
#33339=CARTESIAN_POINT('Ctrl Pts',(-3.29427438855773,-0.158333333333598,
10.6555281147055));
#33340=CARTESIAN_POINT('Ctrl Pts',(-3.27041076489765,0.1583333333336,10.6780128576633));
#33341=CARTESIAN_POINT('Ctrl Pts',(-3.27864253380086,0.319434907277705,
10.7301959709333));
#33342=CARTESIAN_POINT('Ctrl Pts',(-3.30009924532343,0.636309800096275,
10.8035010882691));
#33343=CARTESIAN_POINT('Ctrl Pts',(-3.32709168674241,0.794772684002175,
10.8711791666546));
#33344=CARTESIAN_POINT('Ctrl Pts',(-3.36497326618527,1.06847604194766,10.8996552636671));
#33345=CARTESIAN_POINT('Ctrl Pts',(-3.38235194885042,1.18514270861525,10.8978655456807));
#33346=CARTESIAN_POINT('Ctrl Pts',(-3.40071178209068,1.30000000000438,10.8819598624545));
#33347=CARTESIAN_POINT('Ctrl Pts',(-3.56846700829314,-1.30000000000448,
10.6880753023113));
#33348=CARTESIAN_POINT('Ctrl Pts',(-3.5396465007391,-1.18514270861582,10.7101749123656));
#33349=CARTESIAN_POINT('Ctrl Pts',(-3.50966832071176,-1.06847604194871,
10.7211153748007));
#33350=CARTESIAN_POINT('Ctrl Pts',(-3.43773827272932,-0.794772684003476,
10.7206101682778));
#33351=CARTESIAN_POINT('Ctrl Pts',(-3.38488511663496,-0.636309800097297,
10.6775025502549));
#33352=CARTESIAN_POINT('Ctrl Pts',(-3.31672657946322,-0.319434907278215,
10.6481671548942));
#33353=CARTESIAN_POINT('Ctrl Pts',(-3.28399515052784,-0.158333333333855,
10.6208824265012));
#33354=CARTESIAN_POINT('Ctrl Pts',(-3.26072518366511,0.158333333333857,
10.6430059624589));
#33355=CARTESIAN_POINT('Ctrl Pts',(-3.26924648437681,0.319434907278222,
10.6932227713766));
#33356=CARTESIAN_POINT('Ctrl Pts',(-3.29192081554073,0.636309800097307,
10.7659752694701));
#33357=CARTESIAN_POINT('Ctrl Pts',(-3.32006229542947,0.794772684003464,
10.8319547752052));
#33358=CARTESIAN_POINT('Ctrl Pts',(-3.35925865987659,1.06847604194939,10.8654753627169));
#33359=CARTESIAN_POINT('Ctrl Pts',(-3.37715256797164,1.18514270861719,10.8673647356509));
#33360=CARTESIAN_POINT('Ctrl Pts',(-3.39597373036095,1.3000000000065,10.8566336612452));
#33361=CARTESIAN_POINT('Ctrl Pts',(-3.56482293374636,-1.30000000000484,
10.6760625013374));
#33362=CARTESIAN_POINT('Ctrl Pts',(-3.53566894486391,-1.18514270861616,
10.6955880507016));
#33363=CARTESIAN_POINT('Ctrl Pts',(-3.5053946453138,-1.06847604194901,10.7046832736887));
#33364=CARTESIAN_POINT('Ctrl Pts',(-3.43286681524052,-0.794772684003699,
10.7015989177713));
#33365=CARTESIAN_POINT('Ctrl Pts',(-3.3796708582827,-0.636309800097476,
10.6592633358045));
#33366=CARTESIAN_POINT('Ctrl Pts',(-3.31123172933568,-0.319434907278304,
10.6300376279778));
#33367=CARTESIAN_POINT('Ctrl Pts',(-3.27845132813535,-0.1583333333339,10.6036939265839));
#33368=CARTESIAN_POINT('Ctrl Pts',(-3.25546516233841,0.158333333333902,
10.6256432851867));
#33369=CARTESIAN_POINT('Ctrl Pts',(-3.26453005067804,0.319434907278311,
10.6746022809027));
#33370=CARTESIAN_POINT('Ctrl Pts',(-3.28763364240969,0.636309800097486,
10.7471807886859));
#33371=CARTESIAN_POINT('Ctrl Pts',(-3.31555303628374,0.794772684003689,
10.8128030858203));
#33372=CARTESIAN_POINT('Ctrl Pts',(-3.35541107546838,1.0684760419497,10.8488670492249));
#33373=CARTESIAN_POINT('Ctrl Pts',(-3.37373782596862,1.18514270861752,10.8525041026793));
#33374=CARTESIAN_POINT('Ctrl Pts',(-3.39313825869191,1.30000000000687,10.8441674561317));
#33375=CARTESIAN_POINT('Ctrl Pts',(-3.5647656098383,-1.30000000000484,10.6758768710106));
#33376=CARTESIAN_POINT('Ctrl Pts',(-3.53560670555812,-1.18514270861615,
10.6953623028687));
#33377=CARTESIAN_POINT('Ctrl Pts',(-3.50532801058858,-1.06847604194901,
10.704428759195));
#33378=CARTESIAN_POINT('Ctrl Pts',(-3.43279122747106,-0.794772684003698,
10.7013041692597));
#33379=CARTESIAN_POINT('Ctrl Pts',(-3.37959022019577,-0.636309800097475,
10.658980400634));
#33380=CARTESIAN_POINT('Ctrl Pts',(-3.31114632355007,-0.319434907278303,
10.6297566683138));
#33381=CARTESIAN_POINT('Ctrl Pts',(-3.27836400035346,-0.158333333333899,
10.6034283295616));
#33382=CARTESIAN_POINT('Ctrl Pts',(-3.25538212571374,0.158333333333901,
10.6253750534706));
#33383=CARTESIAN_POINT('Ctrl Pts',(-3.26445637979772,0.319434907278311,
10.6743139130905));
#33384=CARTESIAN_POINT('Ctrl Pts',(-3.28756705840575,0.636309800097484,
10.7468894351868));
#33385=CARTESIAN_POINT('Ctrl Pts',(-3.315482936733,0.794772684003688,10.8125062482728));
#33386=CARTESIAN_POINT('Ctrl Pts',(-3.35535126532992,1.06847604194969,10.8486096365886));
#33387=CARTESIAN_POINT('Ctrl Pts',(-3.37368471811786,1.18514270861751,10.8522737991005));
#33388=CARTESIAN_POINT('Ctrl Pts',(-3.39309410151123,1.30000000000686,10.8439743050846));
#33389=CARTESIAN_POINT('Ctrl Pts',(-3.56466570358193,-1.30000000000484,
10.6755517052646));
#33390=CARTESIAN_POINT('Ctrl Pts',(-3.53549792772271,-1.18514270861615,
10.6949671392659));
#33391=CARTESIAN_POINT('Ctrl Pts',(-3.50521135057255,-1.06847604194901,
10.7039833998441));
#33392=CARTESIAN_POINT('Ctrl Pts',(-3.43265864374919,-0.794772684003698,
10.7007885945215));
#33393=CARTESIAN_POINT('Ctrl Pts',(-3.37944873025216,-0.636309800097476,
10.6584855261697));
#33394=CARTESIAN_POINT('Ctrl Pts',(-3.31099685750756,-0.319434907278303,
10.6292650047689));
#33395=CARTESIAN_POINT('Ctrl Pts',(-3.27821203825765,-0.1583333333339,10.6029629733926));
#33396=CARTESIAN_POINT('Ctrl Pts',(-3.25523775215173,0.158333333333901,
10.624905036394));
#33397=CARTESIAN_POINT('Ctrl Pts',(-3.26432762546627,0.319434907278311,
10.6738091758094));
#33398=CARTESIAN_POINT('Ctrl Pts',(-3.28745046379999,0.636309800097485,
10.746379635446));
#33399=CARTESIAN_POINT('Ctrl Pts',(-3.31536045548722,0.794772684003688,
10.8119866746284));
#33400=CARTESIAN_POINT('Ctrl Pts',(-3.35524682273211,1.06847604194969,10.8481590280866));
#33401=CARTESIAN_POINT('Ctrl Pts',(-3.37359199792297,1.18514270861752,10.8518706311386));
#33402=CARTESIAN_POINT('Ctrl Pts',(-3.39301701785986,1.30000000000686,10.8436361657485));
#33403=CARTESIAN_POINT('Ctrl Pts',(-3.56452220822542,-1.30000000000484,
10.6750877402548));
#33404=CARTESIAN_POINT('Ctrl Pts',(-3.53534166513088,-1.18514270861615,
10.6944032219802));
#33405=CARTESIAN_POINT('Ctrl Pts',(-3.50504379632556,-1.06847604194901,
10.7033477814798));
#33406=CARTESIAN_POINT('Ctrl Pts',(-3.43246841240526,-0.794772684003697,
10.7000525982394));
#33407=CARTESIAN_POINT('Ctrl Pts',(-3.3792461880662,-0.636309800097475,
10.6577788260496));
#33408=CARTESIAN_POINT('Ctrl Pts',(-3.31078289800484,-0.319434907278303,
10.6285628970504));
#33409=CARTESIAN_POINT('Ctrl Pts',(-3.27799407242096,-0.158333333333899,
10.6022987392734));
#33410=CARTESIAN_POINT('Ctrl Pts',(-3.2550305779373,0.158333333333901,10.6242341681237));
#33411=CARTESIAN_POINT('Ctrl Pts',(-3.26414294810058,0.319434907278311,
10.673088573858));
#33412=CARTESIAN_POINT('Ctrl Pts',(-3.28728350341888,0.636309800097484,
10.7456515726491));
#33413=CARTESIAN_POINT('Ctrl Pts',(-3.31518555604749,0.794772684003687,
10.811244349333));
#33414=CARTESIAN_POINT('Ctrl Pts',(-3.35509782672543,1.06847604194969,10.8475151463616));
#33415=CARTESIAN_POINT('Ctrl Pts',(-3.37345971013758,1.18514270861751,10.8512945514547));
#33416=CARTESIAN_POINT('Ctrl Pts',(-3.3929069338807,1.30000000000686,10.8431530775728));
#33417=CARTESIAN_POINT('Ctrl Pts',(-3.564349417289,-1.30000000000484,10.674531392229));
#33418=CARTESIAN_POINT('Ctrl Pts',(-3.53515306526229,-1.18514270861615,
10.6937272657619));
#33419=CARTESIAN_POINT('Ctrl Pts',(-3.50484135793382,-1.06847604194901,
10.7025859799768));
#33420=CARTESIAN_POINT('Ctrl Pts',(-3.43223855629568,-0.794772684003697,
10.6991704760268));
#33421=CARTESIAN_POINT('Ctrl Pts',(-3.37900212853287,-0.636309800097474,
10.656931455314));
#33422=CARTESIAN_POINT('Ctrl Pts',(-3.31052558194566,-0.319434907278303,
10.6277207251215));
#33423=CARTESIAN_POINT('Ctrl Pts',(-3.27773238178739,-0.158333333333899,
10.6015017257394));
#33424=CARTESIAN_POINT('Ctrl Pts',(-3.2547818419222,0.158333333333901,10.6234291808475));
#33425=CARTESIAN_POINT('Ctrl Pts',(-3.26392046214312,0.31943490727831,10.6722243902951));
#33426=CARTESIAN_POINT('Ctrl Pts',(-3.28708249045311,0.636309800097484,
10.7447783005775));
#33427=CARTESIAN_POINT('Ctrl Pts',(-3.31497613290306,0.794772684003687,
10.8103532451295));
#33428=CARTESIAN_POINT('Ctrl Pts',(-3.35491970635418,1.06847604194969,10.8467420377067));
#33429=CARTESIAN_POINT('Ctrl Pts',(-3.37330154458274,1.18514270861751,10.8506028685909));
#33430=CARTESIAN_POINT('Ctrl Pts',(-3.39277512814806,1.30000000000686,10.8425731703904));
#33431=CARTESIAN_POINT('Ctrl Pts',(-3.5640021797759,-1.30000000000484,10.6734198538772));
#33432=CARTESIAN_POINT('Ctrl Pts',(-3.53477320726961,-1.18514270861615,
10.6923771850188));
#33433=CARTESIAN_POINT('Ctrl Pts',(-3.50443325568522,-1.068476041949,10.7010645848694));
#33434=CARTESIAN_POINT('Ctrl Pts',(-3.43177531411776,-0.794772684003695,
10.6974086206578));
#33435=CARTESIAN_POINT('Ctrl Pts',(-3.37851196008848,-0.636309800097473,
10.6552380707824));
#33436=CARTESIAN_POINT('Ctrl Pts',(-3.31000971826934,-0.319434907278302,
10.6260371567929));
#33437=CARTESIAN_POINT('Ctrl Pts',(-3.27720815839903,-0.158333333333899,
10.599908210249));
#33438=CARTESIAN_POINT('Ctrl Pts',(-3.25428347088739,0.158333333333901,
10.6218197316737));
#33439=CARTESIAN_POINT('Ctrl Pts',(-3.26347335217478,0.31943490727831,10.6704973405271));
#33440=CARTESIAN_POINT('Ctrl Pts',(-3.28667900751217,0.636309800097482,
10.7430326358703));
#33441=CARTESIAN_POINT('Ctrl Pts',(-3.31455833413199,0.794772684003684,
10.8085703159024));
#33442=CARTESIAN_POINT('Ctrl Pts',(-3.35456499042273,1.06847604194969,10.8451948052891));
#33443=CARTESIAN_POINT('Ctrl Pts',(-3.37298649636271,1.18514270861751,10.8492186495772));
#33444=CARTESIAN_POINT('Ctrl Pts',(-3.39251210912706,1.30000000000686,10.841412953769));
#33445=CARTESIAN_POINT('Ctrl Pts',(-3.56347571232416,-1.30000000000483,
10.6717564062968));
#33446=CARTESIAN_POINT('Ctrl Pts',(-3.53419300891418,-1.18514270861614,
10.6903592176008));
#33447=CARTESIAN_POINT('Ctrl Pts',(-3.50380790798684,-1.06847604194899,
10.6987915422063));
#33448=CARTESIAN_POINT('Ctrl Pts',(-3.43106548752715,-0.794772684003688,
10.6947760400535));
#33449=CARTESIAN_POINT('Ctrl Pts',(-3.37776796299676,-0.636309800097467,
10.652703824103));
#33450=CARTESIAN_POINT('Ctrl Pts',(-3.30923142734901,-0.319434907278299,
10.6235146541448));
#33451=CARTESIAN_POINT('Ctrl Pts',(-3.2764207460507,-0.158333333333898,
10.5975184936668));
#33452=CARTESIAN_POINT('Ctrl Pts',(-3.25353469006426,0.158333333333899,
10.6194061215614));
#33453=CARTESIAN_POINT('Ctrl Pts',(-3.26279455275997,0.319434907278307,
10.6679118021839));
#33454=CARTESIAN_POINT('Ctrl Pts',(-3.28606791379863,0.636309800097477,
10.7404177444664));
#33455=CARTESIAN_POINT('Ctrl Pts',(-3.31393689224648,0.794772684003677,
10.805892423076));
#33456=CARTESIAN_POINT('Ctrl Pts',(-3.35404007894592,1.06847604194968,10.8428692671772));
#33457=CARTESIAN_POINT('Ctrl Pts',(-3.37251994711931,1.1851427086175,10.8471383750334));
#33458=CARTESIAN_POINT('Ctrl Pts',(-3.39212049991335,1.30000000000685,10.8396706850613));
#33459=CARTESIAN_POINT('Ctrl Pts',(-3.56288008463113,-1.30000000000482,
10.6699153100721));
#33460=CARTESIAN_POINT('Ctrl Pts',(-3.53352504187793,-1.18514270861613,
10.688132976957));
#33461=CARTESIAN_POINT('Ctrl Pts',(-3.50308238913506,-1.06847604194898,
10.6962869902133));
#33462=CARTESIAN_POINT('Ctrl Pts',(-3.43024117461551,-0.794772684003681,
10.6918753389307));
#33463=CARTESIAN_POINT('Ctrl Pts',(-3.37692113363069,-0.636309800097462,
10.6499014916574));
#33464=CARTESIAN_POINT('Ctrl Pts',(-3.30835829639661,-0.319434907278296,
10.6207171664895));
#33465=CARTESIAN_POINT('Ctrl Pts',(-3.27554874317051,-0.158333333333896,
10.5948610178512));
#33466=CARTESIAN_POINT('Ctrl Pts',(-3.25270507405461,0.158333333333898,
10.6167222438594));
#33467=CARTESIAN_POINT('Ctrl Pts',(-3.26202237611515,0.319434907278304,
10.66505008052));
#33468=CARTESIAN_POINT('Ctrl Pts',(-3.28537541909464,0.636309800097471,
10.7375206818382));
#33469=CARTESIAN_POINT('Ctrl Pts',(-3.31326193793976,0.794772684003671,
10.8029068995155));
#33470=CARTESIAN_POINT('Ctrl Pts',(-3.35347649267537,1.06847604194967,10.8402726868186));
#33471=CARTESIAN_POINT('Ctrl Pts',(-3.37201781453021,1.18514270861749,10.8448164903824));
#33472=CARTESIAN_POINT('Ctrl Pts',(-3.39169306759087,1.30000000000684,10.8377298327253));
#33473=CARTESIAN_POINT('Ctrl Pts',(-3.56239728410032,-1.30000000000481,
10.6684465924844));
#33474=CARTESIAN_POINT('Ctrl Pts',(-3.53297521638305,-1.18514270861612,
10.6863625247026));
#33475=CARTESIAN_POINT('Ctrl Pts',(-3.50248113498807,-1.06847604194898,
10.6942976370287));
#33476=CARTESIAN_POINT('Ctrl Pts',(-3.42955714059451,-0.794772684003679,
10.6895716433085));
#33477=CARTESIAN_POINT('Ctrl Pts',(-3.37622978260571,-0.63630980009746,
10.647668936555));
#33478=CARTESIAN_POINT('Ctrl Pts',(-3.30765465018317,-0.319434907278295,
10.6184824351893));
#33479=CARTESIAN_POINT('Ctrl Pts',(-3.27485508668908,-0.158333333333896,
10.5927322349785));
#33480=CARTESIAN_POINT('Ctrl Pts',(-3.25204494547751,0.158333333333897,
10.6145724490381));
#33481=CARTESIAN_POINT('Ctrl Pts',(-3.26139275085378,0.319434907278303,
10.662768043132));
#33482=CARTESIAN_POINT('Ctrl Pts',(-3.28481219545305,0.636309800097469,
10.7352087802632));
#33483=CARTESIAN_POINT('Ctrl Pts',(-3.31273351341567,0.794772684003668,
10.8005110532342));
#33484=CARTESIAN_POINT('Ctrl Pts',(-3.35303990765138,1.06847604194967,10.8381862837691));
#33485=CARTESIAN_POINT('Ctrl Pts',(-3.3716278902605,1.18514270861749,10.842951442016));
#33486=CARTESIAN_POINT('Ctrl Pts',(-3.39135671091313,1.30000000000683,10.8361735472162));
#33487=CARTESIAN_POINT('Ctrl Pts',(-3.56166717131598,-1.3000000000048,10.6662473927834));
#33488=CARTESIAN_POINT('Ctrl Pts',(-3.53213539832158,-1.18514270861612,
10.6837171284086));
#33489=CARTESIAN_POINT('Ctrl Pts',(-3.5015587453786,-1.06847604194897,10.6913276776729));
#33490=CARTESIAN_POINT('Ctrl Pts',(-3.4285066785331,-0.794772684003673,
10.6861328761411));
#33491=CARTESIAN_POINT('Ctrl Pts',(-3.37517873510585,-0.636309800097455,
10.644329539887));
#33492=CARTESIAN_POINT('Ctrl Pts',(-3.30659388175246,-0.319434907278293,
10.6151337471993));
#33493=CARTESIAN_POINT('Ctrl Pts',(-3.27381864911049,-0.158333333333895,
10.5895362325923));
#33494=CARTESIAN_POINT('Ctrl Pts',(-3.25105854279058,0.158333333333896,
10.6113449523485));
#33495=CARTESIAN_POINT('Ctrl Pts',(-3.26043674820715,0.319434907278301,
10.6593521508946));
#33496=CARTESIAN_POINT('Ctrl Pts',(-3.28395826579358,0.636309800097465,
10.7317466146758));
#33497=CARTESIAN_POINT('Ctrl Pts',(-3.31195199728272,0.794772684003663,
10.7969101537614));
#33498=CARTESIAN_POINT('Ctrl Pts',(-3.35239889578995,1.06847604194966,10.8350478260744));
#33499=CARTESIAN_POINT('Ctrl Pts',(-3.37105449282202,1.18514270861748,10.8401465257561));
#33500=CARTESIAN_POINT('Ctrl Pts',(-3.3908577232276,1.30000000000682,10.8338355399152));
#33501=CARTESIAN_POINT('Ctrl Pts',(-3.5605509826163,-1.30000000000476,10.6629622113181));
#33502=CARTESIAN_POINT('Ctrl Pts',(-3.53081837342967,-1.18514270861608,
10.6797880844511));
#33503=CARTESIAN_POINT('Ctrl Pts',(-3.50009634366811,-1.06847604194894,
10.6869268691001));
#33504=CARTESIAN_POINT('Ctrl Pts',(-3.42683654953696,-0.794772684003649,
10.6810397774547));
#33505=CARTESIAN_POINT('Ctrl Pts',(-3.37354839289819,-0.636309800097436,
10.6393567271974));
#33506=CARTESIAN_POINT('Ctrl Pts',(-3.30498358068139,-0.319434907278283,
10.610123118836));
#33507=CARTESIAN_POINT('Ctrl Pts',(-3.27228264912268,-0.15833333333389,
10.5847294420948));
#33508=CARTESIAN_POINT('Ctrl Pts',(-3.24959637980222,0.158333333333892,
10.6064911810025));
#33509=CARTESIAN_POINT('Ctrl Pts',(-3.2589585365903,0.319434907278291,10.6542558381739));
#33510=CARTESIAN_POINT('Ctrl Pts',(-3.28264215828697,0.636309800097445,
10.7265755606784));
#33511=CARTESIAN_POINT('Ctrl Pts',(-3.31082405553576,0.794772684003639,
10.7914805646343));
#33512=CARTESIAN_POINT('Ctrl Pts',(-3.3514923734059,1.06847604194963,10.8303051522282));
#33513=CARTESIAN_POINT('Ctrl Pts',(-3.37024002099385,1.18514270861744,10.8359100775422));
#33514=CARTESIAN_POINT('Ctrl Pts',(-3.39013150827335,1.30000000000678,10.8303142027936));
#33515=CARTESIAN_POINT('Ctrl Pts',(-3.55903559501172,-1.30000000000473,
10.6585990137924));
#33516=CARTESIAN_POINT('Ctrl Pts',(-3.52898566602019,-1.18514270861605,
10.6746008966558));
#33517=CARTESIAN_POINT('Ctrl Pts',(-3.49803917570353,-1.06847604194892,
10.6811319700951));
#33518=CARTESIAN_POINT('Ctrl Pts',(-3.42447535623036,-0.79477268400363,
10.6743405918781));
#33519=CARTESIAN_POINT('Ctrl Pts',(-3.37128560137921,-0.636309800097421,
10.6327859803119));
#33520=CARTESIAN_POINT('Ctrl Pts',(-3.30278947088664,-0.319434907278276,
10.6034731326008));
#33521=CARTESIAN_POINT('Ctrl Pts',(-3.27023986261253,-0.158333333333886,
10.5783165335595));
#33522=CARTESIAN_POINT('Ctrl Pts',(-3.24765357747863,0.158333333333888,
10.6000134933769));
#33523=CARTESIAN_POINT('Ctrl Pts',(-3.25691882719003,0.319434907278284,
10.6475029434009));
#33524=CARTESIAN_POINT('Ctrl Pts',(-3.28083024644292,0.63630980009743,10.7197156715094));
#33525=CARTESIAN_POINT('Ctrl Pts',(-3.30935748754829,0.79477268400362,10.7842163758251));
#33526=CARTESIAN_POINT('Ctrl Pts',(-3.35033881509226,1.0684760419496,10.8239457582688));
#33527=CARTESIAN_POINT('Ctrl Pts',(-3.36920131774698,1.18514270861741,10.8302307025121));
#33528=CARTESIAN_POINT('Ctrl Pts',(-3.3891870248704,1.30000000000675,10.8256032134573));
#33529=CARTESIAN_POINT('Ctrl Pts',(-3.55752159162629,-1.30000000000469,
10.6542337760585));
#33530=CARTESIAN_POINT('Ctrl Pts',(-3.52715172501055,-1.18514270861602,
10.6694131300325));
#33531=CARTESIAN_POINT('Ctrl Pts',(-3.49597694911425,-1.06847604194888,
10.6753389254243));
#33532=CARTESIAN_POINT('Ctrl Pts',(-3.42209747884168,-0.794772684003606,
10.6676511267378));
#33533=CARTESIAN_POINT('Ctrl Pts',(-3.368992580335,-0.636309800097402,10.626234723924));
#33534=CARTESIAN_POINT('Ctrl Pts',(-3.30055362425563,-0.319434907278266,
10.5968508024426));
#33535=CARTESIAN_POINT('Ctrl Pts',(-3.26815037522595,-0.158333333333881,
10.5719351062856));
#33536=CARTESIAN_POINT('Ctrl Pts',(-3.24566707198885,0.158333333333883,
10.5935646644834));
#33537=CARTESIAN_POINT('Ctrl Pts',(-3.2548509611682,0.319434907278274,10.6407670490172));
#33538=CARTESIAN_POINT('Ctrl Pts',(-3.27899234172843,0.636309800097411,
10.7128702963079));
#33539=CARTESIAN_POINT('Ctrl Pts',(-3.30784607106761,0.794772684003596,
10.7769787929198));
#33540=CARTESIAN_POINT('Ctrl Pts',(-3.34914925161841,1.06847604194957,10.8176075249763));
#33541=CARTESIAN_POINT('Ctrl Pts',(-3.36813583255034,1.18514270861738,10.8245668295542));
#33542=CARTESIAN_POINT('Ctrl Pts',(-3.38823037798735,1.30000000000671,10.8208987660454));
#33543=CARTESIAN_POINT('Ctrl Pts',(-3.55627990365541,-1.30000000000468,
10.650581842169));
#33544=CARTESIAN_POINT('Ctrl Pts',(-3.52567472551719,-1.185142708616,10.6650532747694));
#33545=CARTESIAN_POINT('Ctrl Pts',(-3.49432538040437,-1.06847604194887,
10.6704633371688));
#33546=CARTESIAN_POINT('Ctrl Pts',(-3.42018294719733,-0.794772684003595,
10.6620280857059));
#33547=CARTESIAN_POINT('Ctrl Pts',(-3.36709213569808,-0.636309800097393,
10.6207672424199));
#33548=CARTESIAN_POINT('Ctrl Pts',(-3.29865407552894,-0.319434907278262,
10.5913565459549));
#33549=CARTESIAN_POINT('Ctrl Pts',(-3.26633175109663,-0.158333333333879,
10.5666693570679));
#33550=CARTESIAN_POINT('Ctrl Pts',(-3.24394125733372,0.158333333333881,
10.5882377662089));
#33551=CARTESIAN_POINT('Ctrl Pts',(-3.2531381412007,0.31943490727827,10.635146342547));
#33552=CARTESIAN_POINT('Ctrl Pts',(-3.27746541146243,0.636309800097403,
10.7071602656532));
#33553=CARTESIAN_POINT('Ctrl Pts',(-3.30648891039559,0.794772684003586,
10.7710069393103));
#33554=CARTESIAN_POINT('Ctrl Pts',(-3.34805987709607,1.06847604194956,10.8123856843356));
#33555=CARTESIAN_POINT('Ctrl Pts',(-3.3671700124198,1.18514270861736,10.8198945045906));
#33556=CARTESIAN_POINT('Ctrl Pts',(-3.38739575193867,1.3000000000067,10.8170008196127));
#33557=CARTESIAN_POINT('Ctrl Pts',(-3.55530544718959,-1.30000000000466,
10.6476469380569));
#33558=CARTESIAN_POINT('Ctrl Pts',(-3.52453845358926,-1.18514270861599,
10.6615332127035));
#33559=CARTESIAN_POINT('Ctrl Pts',(-3.49306443829092,-1.06847604194886,
10.6665199771758));
#33560=CARTESIAN_POINT('Ctrl Pts',(-3.41871980503502,-0.794772684003589,
10.657480751862));
#33561=CARTESIAN_POINT('Ctrl Pts',(-3.36560903961373,-0.636309800097388,
10.6163664598669));
#33562=CARTESIAN_POINT('Ctrl Pts',(-3.29713541830363,-0.319434907278259,
10.5869595650996));
#33563=CARTESIAN_POINT('Ctrl Pts',(-3.26483504926751,-0.158333333333878,
10.5624846541022));
#33564=CARTESIAN_POINT('Ctrl Pts',(-3.24251388738839,0.15833333333388,10.5840077208246));
#33565=CARTESIAN_POINT('Ctrl Pts',(-3.25177237466923,0.319434907278268,
10.6306468149272));
#33566=CARTESIAN_POINT('Ctrl Pts',(-3.27624745090271,0.636309800097398,
10.7025887389857));
#33567=CARTESIAN_POINT('Ctrl Pts',(-3.30535393223191,0.794772684003579,
10.7662588842987));
#33568=CARTESIAN_POINT('Ctrl Pts',(-3.34713655006451,1.06847604194955,10.8082394976319));
#33569=CARTESIAN_POINT('Ctrl Pts',(-3.36635419398821,1.18514270861735,10.8161828028864));
#33570=CARTESIAN_POINT('Ctrl Pts',(-3.38670333477437,1.30000000000668,10.8138975614185));
#33571=CARTESIAN_POINT('Ctrl Pts',(-3.55433797136118,-1.30000000000466,
10.6447070646829));
#33572=CARTESIAN_POINT('Ctrl Pts',(-3.52342067206276,-1.18514270861598,
10.6579998855295));
#33573=CARTESIAN_POINT('Ctrl Pts',(-3.49182717097928,-1.06847604194885,
10.6625595905517));
#33574=CARTESIAN_POINT('Ctrl Pts',(-3.41727770182104,-0.794772684003584,
10.6529181767109));
#33575=CARTESIAN_POINT('Ctrl Pts',(-3.36411925843592,-0.636309800097384,
10.6119703680613));
#33576=CARTESIAN_POINT('Ctrl Pts',(-3.29559467409961,-0.319434907278257,
10.5825779694666));
#33577=CARTESIAN_POINT('Ctrl Pts',(-3.26330933623401,-0.158333333333877,
10.5583195887821));
#33578=CARTESIAN_POINT('Ctrl Pts',(-3.24106629086893,0.158333333333879,
10.579791104));
#33579=CARTESIAN_POINT('Ctrl Pts',(-3.25042046142221,0.319434907278266,
10.626137820413));
#33580=CARTESIAN_POINT('Ctrl Pts',(-3.27503921876234,0.636309800097394,
10.6980097305382));
#33581=CARTESIAN_POINT('Ctrl Pts',(-3.30417980955526,0.794772684003574,
10.7615346745576));
#33582=CARTESIAN_POINT('Ctrl Pts',(-3.34617223155567,1.06847604194954,10.8041184706937));
#33583=CARTESIAN_POINT('Ctrl Pts',(-3.36550607566519,1.18514270861734,10.8124908401636));
#33584=CARTESIAN_POINT('Ctrl Pts',(-3.38599680037276,1.30000000000668,10.8108026316413));
#33585=CARTESIAN_POINT('Ctrl Pts',(-3.54984970514755,-1.30000000000455,
10.6306658122771));
#33586=CARTESIAN_POINT('Ctrl Pts',(-3.51834143663056,-1.18514270861589,
10.6410528143556));
#33587=CARTESIAN_POINT('Ctrl Pts',(-3.48626566849313,-1.06847604194877,
10.6435233970436));
#33588=CARTESIAN_POINT('Ctrl Pts',(-3.41085318970915,-0.794772684003521,
10.6309424248252));
#33589=CARTESIAN_POINT('Ctrl Pts',(-3.35748539912993,-0.636309800097333,
10.5907706537778));
#33590=CARTESIAN_POINT('Ctrl Pts',(-3.28854880426052,-0.319434907278232,
10.5615660112157));
#33591=CARTESIAN_POINT('Ctrl Pts',(-3.25600785230901,-0.158333333333864,
10.5385678190991));
#33592=CARTESIAN_POINT('Ctrl Pts',(-3.23398649691687,0.158333333333866,
10.5599007473991));
#33593=CARTESIAN_POINT('Ctrl Pts',(-3.24388113552723,0.31943490727824,10.6047995313936));
#33594=CARTESIAN_POINT('Ctrl Pts',(-3.26923480939674,0.636309800097343,
10.6763015230462));
#33595=CARTESIAN_POINT('Ctrl Pts',(-3.29863995344783,0.79477268400351,10.7390613151974));
#33596=CARTESIAN_POINT('Ctrl Pts',(-3.34161847429591,1.06847604194946,10.7845180418296));
#33597=CARTESIAN_POINT('Ctrl Pts',(-3.36147233784438,1.18514270861725,10.7949519108724));
#33598=CARTESIAN_POINT('Ctrl Pts',(-3.38257625577727,1.30000000000657,10.7961431163365));
#33599=CARTESIAN_POINT('Ctrl Pts',(-3.54346327544845,-1.30000000000345,
10.6116084872656));
#33600=CARTESIAN_POINT('Ctrl Pts',(-3.51087038822887,-1.18514270861488,
10.6182069030137));
#33601=CARTESIAN_POINT('Ctrl Pts',(-3.47788547855602,-1.06847604194786,
10.6179921149657));
#33602=CARTESIAN_POINT('Ctrl Pts',(-3.40077808831231,-0.794772684002841,
10.6017560478612));
#33603=CARTESIAN_POINT('Ctrl Pts',(-3.34648395165712,-0.636309800096792,
10.5631227662308));
#33604=CARTESIAN_POINT('Ctrl Pts',(-3.27736572352823,-0.319434907277961,
10.5339123302075));
#33605=CARTESIAN_POINT('Ctrl Pts',(-3.24570255877244,-0.15833333333373,
10.5117636373826));
#33606=CARTESIAN_POINT('Ctrl Pts',(-3.22473605365345,0.158333333333732,
10.5323693415874));
#33607=CARTESIAN_POINT('Ctrl Pts',(-3.23555825476826,0.31943490727797,10.5751540299561));
#33608=CARTESIAN_POINT('Ctrl Pts',(-3.26171350265685,0.636309800096803,
10.6462751005081));
#33609=CARTESIAN_POINT('Ctrl Pts',(-3.29042133095542,0.794772684002834,
10.7086999413166));
#33610=CARTESIAN_POINT('Ctrl Pts',(-3.33480204109443,1.06847604194855,10.7580517685289));
#33611=CARTESIAN_POINT('Ctrl Pts',(-3.35562786553996,1.18514270861624,10.7711322840336));
#33612=CARTESIAN_POINT('Ctrl Pts',(-3.37806874947915,1.30000000000547,10.7759307377082));
#33613=CARTESIAN_POINT('Ctrl Pts',(-3.53506496247113,-1.30000000000306,
10.5885155682011));
#33614=CARTESIAN_POINT('Ctrl Pts',(-3.50062776708192,-1.18514270861453,
10.5908138492831));
#33615=CARTESIAN_POINT('Ctrl Pts',(-3.46639685555495,-1.06847604194754,
10.5873798227));
#33616=CARTESIAN_POINT('Ctrl Pts',(-3.38779315904599,-0.79477268400261,
10.5662037568673));
#33617=CARTESIAN_POINT('Ctrl Pts',(-3.33486996497483,-0.636309800096606,
10.5276326062933));
#33618=CARTESIAN_POINT('Ctrl Pts',(-3.26577734696951,-0.319434907277867,
10.4982277618773));
#33619=CARTESIAN_POINT('Ctrl Pts',(-3.23377655240389,-0.158333333333683,
10.4781750219806));
#33620=CARTESIAN_POINT('Ctrl Pts',(-3.21261251753656,0.158333333333685,
10.4989346304306));
#33621=CARTESIAN_POINT('Ctrl Pts',(-3.22291473938703,0.319434907277874,
10.5402309269832));
#33622=CARTESIAN_POINT('Ctrl Pts',(-3.24998655733667,0.636309800096615,
10.6109358314202));
#33623=CARTESIAN_POINT('Ctrl Pts',(-3.28026677895592,0.794772684002601,
10.671291429696));
#33624=CARTESIAN_POINT('Ctrl Pts',(-3.3263996702633,1.06847604194823,10.7254459437499));
#33625=CARTESIAN_POINT('Ctrl Pts',(-3.34797394235853,1.18514270861589,10.7421061125178));
#33626=CARTESIAN_POINT('Ctrl Pts',(-3.37115326729403,1.30000000000509,10.7519849675422));
#33627=CARTESIAN_POINT('Ctrl Pts',(-3.52689650086691,-1.30000000000268,
10.5652540209631));
#33628=CARTESIAN_POINT('Ctrl Pts',(-3.49113723742897,-1.18514270861418,
10.562853485114));
#33629=CARTESIAN_POINT('Ctrl Pts',(-3.45576242609193,-1.06847604194723,
10.5561146433435));
#33630=CARTESIAN_POINT('Ctrl Pts',(-3.3749276964591,-0.794772684002374,
10.5305242161996));
#33631=CARTESIAN_POINT('Ctrl Pts',(-3.32053529474771,-0.636309800096415,
10.4941077758252));
#33632=CARTESIAN_POINT('Ctrl Pts',(-3.25116009621693,-0.31943490727777,
10.4647365721695));
#33633=CARTESIAN_POINT('Ctrl Pts',(-3.22065187264131,-0.158333333333636,
10.4454354717321));
#33634=CARTESIAN_POINT('Ctrl Pts',(-3.20049904729554,0.158333333333637,
10.465470439846));
#33635=CARTESIAN_POINT('Ctrl Pts',(-3.21091965362889,0.319434907277778,
10.5048325382507));
#33636=CARTESIAN_POINT('Ctrl Pts',(-3.2391121737702,0.636309800096424,10.5749605084516));
#33637=CARTESIAN_POINT('Ctrl Pts',(-3.26980391173995,0.794772684002361,
10.6340355202244));
#33638=CARTESIAN_POINT('Ctrl Pts',(-3.31812627927797,1.06847604194791,10.6926922434587));
#33639=CARTESIAN_POINT('Ctrl Pts',(-3.34093984347042,1.18514270861554,10.7125985698184));
#33640=CARTESIAN_POINT('Ctrl Pts',(-3.36565000946822,1.3000000000047,10.7270209004954));
#33641=CARTESIAN_POINT('Ctrl Pts',(-3.51848982050878,-1.30000000000228,
10.5421141081693));
#33642=CARTESIAN_POINT('Ctrl Pts',(-3.4805863296336,-1.18514270861381,10.5356318371647));
#33643=CARTESIAN_POINT('Ctrl Pts',(-3.44368553106901,-1.0684760419469,10.5258764582561));
#33644=CARTESIAN_POINT('Ctrl Pts',(-3.36075372423075,-0.794772684002127,
10.4957780473791));
#33645=CARTESIAN_POINT('Ctrl Pts',(-3.30728683871919,-0.636309800096218,
10.4597379308942));
#33646=CARTESIAN_POINT('Ctrl Pts',(-3.23767528843882,-0.319434907277672,
10.4303589106883));
#33647=CARTESIAN_POINT('Ctrl Pts',(-3.20694464491671,-0.158333333333587,
10.4130789334689));
#33648=CARTESIAN_POINT('Ctrl Pts',(-3.1868156375817,0.158333333333589,10.4330970843297));
#33649=CARTESIAN_POINT('Ctrl Pts',(-3.19711015924159,0.31943490727768,10.4706721108572));
#33650=CARTESIAN_POINT('Ctrl Pts',(-3.22634594109612,0.636309800096228,
10.5402626408123));
#33651=CARTESIAN_POINT('Ctrl Pts',(-3.25813763743538,0.794772684002116,
10.5975581252224));
#33652=CARTESIAN_POINT('Ctrl Pts',(-3.30855188048357,1.06847604194758,10.6607913253926));
#33653=CARTESIAN_POINT('Ctrl Pts',(-3.33241496581671,1.18514270861517,10.6840852949285));
#33654=CARTESIAN_POINT('Ctrl Pts',(-3.35831867869917,1.3000000000043,10.7033019246676));
#33655=CARTESIAN_POINT('Ctrl Pts',(-3.51014479419037,-1.30000000000198,
10.5226552577285));
#33656=CARTESIAN_POINT('Ctrl Pts',(-3.47081330763693,-1.18514270861354,
10.5122336534893));
#33657=CARTESIAN_POINT('Ctrl Pts',(-3.43276073750195,-1.06847604194665,
10.4996794489523));
#33658=CARTESIAN_POINT('Ctrl Pts',(-3.34780624087258,-0.794772684001944,
10.4657499916987));
#33659=CARTESIAN_POINT('Ctrl Pts',(-3.29367302138748,-0.636309800096072,
10.4311638915496));
#33660=CARTESIAN_POINT('Ctrl Pts',(-3.2236579236351,-0.319434907277599,
10.4019302275856));
#33661=CARTESIAN_POINT('Ctrl Pts',(-3.193285751204,-0.15833333333355,10.3860071381036));
#33662=CARTESIAN_POINT('Ctrl Pts',(-3.17425631785229,0.158333333333552,
10.405209097692));
#33663=CARTESIAN_POINT('Ctrl Pts',(-3.18586725480623,0.319434907277607,
10.4401640643241));
#33664=CARTESIAN_POINT('Ctrl Pts',(-3.21657446722625,0.636309800096082,
10.5088571830631));
#33665=CARTESIAN_POINT('Ctrl Pts',(-3.24843254019359,0.794772684001934,
10.5652288826434));
#33666=CARTESIAN_POINT('Ctrl Pts',(-3.30057225868985,1.06847604194734,10.6325503637368));
#33667=CARTESIAN_POINT('Ctrl Pts',(-3.32540393947806,1.1851427086149,10.6587825433198));
#33668=CARTESIAN_POINT('Ctrl Pts',(-3.35249794888434,1.300000000004,10.682105927827));
#33669=CARTESIAN_POINT('Ctrl Pts',(-3.50627111332775,-1.30000000000195,
10.5126758013699));
#33670=CARTESIAN_POINT('Ctrl Pts',(-3.46614340916371,-1.18514270861352,
10.5003491529217));
#33671=CARTESIAN_POINT('Ctrl Pts',(-3.42745785791775,-1.06847604194663,
10.4864410559917));
#33672=CARTESIAN_POINT('Ctrl Pts',(-3.34141815726407,-0.794772684001931,
10.4506571074177));
#33673=CARTESIAN_POINT('Ctrl Pts',(-3.28697220080956,-0.636309800096061,
10.4167873260709));
#33674=CARTESIAN_POINT('Ctrl Pts',(-3.21680479490168,-0.319434907277593,
10.3875900843894));
#33675=CARTESIAN_POINT('Ctrl Pts',(-3.18691486237597,-0.158333333333548,
10.3721194208555));
#33676=CARTESIAN_POINT('Ctrl Pts',(-3.16805993730455,0.158333333333549,
10.3911809611948));
#33677=CARTESIAN_POINT('Ctrl Pts',(-3.17936658980045,0.319434907277601,
10.4255224204891));
#33678=CARTESIAN_POINT('Ctrl Pts',(-3.21057454954685,0.636309800096071,
10.4939351803383));
#33679=CARTESIAN_POINT('Ctrl Pts',(-3.24308445280218,0.79477268400192,10.5493933453868));
#33680=CARTESIAN_POINT('Ctrl Pts',(-3.29631738645729,1.06847604194732,10.618596658197));
#33681=CARTESIAN_POINT('Ctrl Pts',(-3.32168699236818,1.18514270861488,10.6462629950032));
#33682=CARTESIAN_POINT('Ctrl Pts',(-3.34938363968517,1.30000000000397,10.6716401187353));
#33683=CARTESIAN_POINT('Ctrl Pts',(-3.50442220663023,-1.30000000000194,
10.5076132694343));
#33684=CARTESIAN_POINT('Ctrl Pts',(-3.46384552380066,-1.18514270861351,
10.4943747916605));
#33685=CARTESIAN_POINT('Ctrl Pts',(-3.4248217357718,-1.06847604194662,10.4798074269121));
#33686=CARTESIAN_POINT('Ctrl Pts',(-3.33825647638829,-0.794772684001924,
10.4430839053978));
#33687=CARTESIAN_POINT('Ctrl Pts',(-3.28384015432874,-0.636309800096055,
10.4094268857005));
#33688=CARTESIAN_POINT('Ctrl Pts',(-3.21356381239586,-0.319434907277589,
10.3802731839803));
#33689=CARTESIAN_POINT('Ctrl Pts',(-3.1837029538244,-0.158333333333546,
10.3651927772445));
#33690=CARTESIAN_POINT('Ctrl Pts',(-3.16486895641784,0.158333333333548,
10.384237183974));
#33691=CARTESIAN_POINT('Ctrl Pts',(-3.17613062389401,0.319434907277598,
10.4181942985397));
#33692=CARTESIAN_POINT('Ctrl Pts',(-3.20756518565311,0.636309800096065,
10.4864816761086));
#33693=CARTESIAN_POINT('Ctrl Pts',(-3.24022250464605,0.794772684001912,
10.541604280706));
#33694=CARTESIAN_POINT('Ctrl Pts',(-3.29408957437523,1.06847604194731,10.6116856914377));
#33695=CARTESIAN_POINT('Ctrl Pts',(-3.31982231985351,1.18514270861487,10.640003080883));
#33696=CARTESIAN_POINT('Ctrl Pts',(-3.34797075229587,1.30000000000396,10.6663022138399));
#33697=CARTESIAN_POINT('Ctrl Pts',(-3.50332286786843,-1.30000000000194,
10.5047548383451));
#33698=CARTESIAN_POINT('Ctrl Pts',(-3.46249907684773,-1.18514270861351,
10.4909872449872));
#33699=CARTESIAN_POINT('Ctrl Pts',(-3.42328867404982,-1.06847604194662,
10.4760374556843));
#33700=CARTESIAN_POINT('Ctrl Pts',(-3.33643204912433,-0.794772684001923,
10.4387693425693));
#33701=CARTESIAN_POINT('Ctrl Pts',(-3.28202668760804,-0.636309800096055,
10.4052388113571));
#33702=CARTESIAN_POINT('Ctrl Pts',(-3.21169158000919,-0.31943490727759,
10.3761071804382));
#33703=CARTESIAN_POINT('Ctrl Pts',(-3.18185600383943,-0.158333333333546,
10.3612432547402));
#33704=CARTESIAN_POINT('Ctrl Pts',(-3.16303173093386,0.158333333333548,
10.3802790615228));
#33705=CARTESIAN_POINT('Ctrl Pts',(-3.17425209796324,0.319434907277598,
10.4140275193072));
#33706=CARTESIAN_POINT('Ctrl Pts',(-3.20581766920952,0.636309800096064,
10.4822418536827));
#33707=CARTESIAN_POINT('Ctrl Pts',(-3.23858232090324,0.794772684001912,
10.5371560079436));
#33708=CARTESIAN_POINT('Ctrl Pts',(-3.29280828302676,1.06847604194731,10.6077416082037));
#33709=CARTESIAN_POINT('Ctrl Pts',(-3.31874163469961,1.18514270861487,10.6364359889067));
#33710=CARTESIAN_POINT('Ctrl Pts',(-3.34713592831186,1.30000000000396,10.6632708594143));
#33711=CARTESIAN_POINT('Ctrl Pts',(-3.49802816243002,-1.3000000000019,10.4921711193909));
#33712=CARTESIAN_POINT('Ctrl Pts',(-3.45607526139304,-1.18514270861347,
10.4760324866026));
#33713=CARTESIAN_POINT('Ctrl Pts',(-3.41602730485291,-1.06847604194659,
10.4593577238278));
#33714=CARTESIAN_POINT('Ctrl Pts',(-3.32790931654956,-0.7947726840019,10.4195971185223));
#33715=CARTESIAN_POINT('Ctrl Pts',(-3.27368731733683,-0.636309800096035,
10.3865334216883));
#33716=CARTESIAN_POINT('Ctrl Pts',(-3.20313098737036,-0.31943490727758,
10.3574669172447));
#33717=CARTESIAN_POINT('Ctrl Pts',(-3.17331373829767,-0.158333333333541,
10.3436502842482));
#33718=CARTESIAN_POINT('Ctrl Pts',(-3.15458900713016,0.158333333333543,
10.3626037702061));
#33719=CARTESIAN_POINT('Ctrl Pts',(-3.16579131284204,0.319434907277589,
10.3952847176026));
#33720=CARTESIAN_POINT('Ctrl Pts',(-3.19798308378842,0.636309800096045,
10.4631397442888));
#33721=CARTESIAN_POINT('Ctrl Pts',(-3.23113884245982,0.794772684001888,
10.517183788305));
#33722=CARTESIAN_POINT('Ctrl Pts',(-3.28690490196432,1.06847604194728,10.5900916182367));
#33723=CARTESIAN_POINT('Ctrl Pts',(-3.3137062707773,1.18514270861483,10.6205071590004));
#33724=CARTESIAN_POINT('Ctrl Pts',(-3.34316994757983,1.30000000000392,10.6497791424516));
#33725=CARTESIAN_POINT('Ctrl Pts',(-3.48397706310386,-1.30000000000141,
10.4576138699549));
#33726=CARTESIAN_POINT('Ctrl Pts',(-3.43892185456666,-1.18514270861303,
10.4350647117943));
#33727=CARTESIAN_POINT('Ctrl Pts',(-3.39646067472579,-1.06847604194619,
10.4138137881798));
#33728=CARTESIAN_POINT('Ctrl Pts',(-3.30435958018563,-0.7947726840016,10.3677190849106));
#33729=CARTESIAN_POINT('Ctrl Pts',(-3.24962674772453,-0.636309800095795,
10.3367046172998));
#33730=CARTESIAN_POINT('Ctrl Pts',(-3.1781699323947,-0.319434907277458,
10.3080563523622));
#33731=CARTESIAN_POINT('Ctrl Pts',(-3.14881299455345,-0.158333333333481,
10.2967802534541));
#33732=CARTESIAN_POINT('Ctrl Pts',(-3.13084603918494,0.158333333333483,
10.3151362963075));
#33733=CARTESIAN_POINT('Ctrl Pts',(-3.1424211459828,0.319434907277467,10.3445817757753));
#33734=CARTESIAN_POINT('Ctrl Pts',(-3.17690348196985,0.636309800095804,
10.4110001959783));
#33735=CARTESIAN_POINT('Ctrl Pts',(-3.21181232388892,0.794772684001585,
10.4621613398969));
#33736=CARTESIAN_POINT('Ctrl Pts',(-3.27143809948091,1.06847604194687,10.5415995405055));
#33737=CARTESIAN_POINT('Ctrl Pts',(-3.30019347467114,1.18514270861439,10.5769819782888));
#33738=CARTESIAN_POINT('Ctrl Pts',(-3.33189443615046,1.30000000000344,10.6133610002872));
#33739=CARTESIAN_POINT('Ctrl Pts',(-3.46377916361696,-1.30000000000082,
10.4138557361379));
#33740=CARTESIAN_POINT('Ctrl Pts',(-3.41402371948706,-1.18514270861249,
10.3833809953346));
#33741=CARTESIAN_POINT('Ctrl Pts',(-3.36792730141995,-1.0684760419457,10.356495138021));
#33742=CARTESIAN_POINT('Ctrl Pts',(-3.2698884363188,-0.794772684001241,
10.3026744679445));
#33743=CARTESIAN_POINT('Ctrl Pts',(-3.2142860913702,-0.636309800095512,
10.2745877798555));
#33744=CARTESIAN_POINT('Ctrl Pts',(-3.14208095012235,-0.319434907277318,
10.2461465738796));
#33745=CARTESIAN_POINT('Ctrl Pts',(-3.11455340661153,-0.158333333333411,
10.2371914073107));
#33746=CARTESIAN_POINT('Ctrl Pts',(-3.09792221777229,0.158333333333413,
10.2544087077735));
#33747=CARTESIAN_POINT('Ctrl Pts',(-3.10963346579246,0.319434907277324,
10.2798132868226));
#33748=CARTESIAN_POINT('Ctrl Pts',(-3.14630219378336,0.63630980009552,10.3448890266851));
#33749=CARTESIAN_POINT('Ctrl Pts',(-3.18162015994576,0.794772684001235,
10.3936449172902));
#33750=CARTESIAN_POINT('Ctrl Pts',(-3.24699522480645,1.0684760419464,10.4811548570736));
#33751=CARTESIAN_POINT('Ctrl Pts',(-3.27920998334397,1.18514270861386,10.5224088501547));
#33752=CARTESIAN_POINT('Ctrl Pts',(-3.31534105722563,1.30000000000285,10.5670370259473));
#33753=CARTESIAN_POINT('Ctrl Pts',(-3.44488287358291,-1.30000000000062,
10.3765723257512));
#33754=CARTESIAN_POINT('Ctrl Pts',(-3.39066496137285,-1.1851427086123,10.3394879857485));
#33755=CARTESIAN_POINT('Ctrl Pts',(-3.34107969198908,-1.06847604194554,
10.3079609144036));
#33756=CARTESIAN_POINT('Ctrl Pts',(-3.23723013189924,-0.794772684001115,
10.2479654749552));
#33757=CARTESIAN_POINT('Ctrl Pts',(-3.18090985311315,-0.636309800095411,
10.2224572148459));
#33758=CARTESIAN_POINT('Ctrl Pts',(-3.10701733313301,-0.319434907277268,
10.1951055044507));
#33759=CARTESIAN_POINT('Ctrl Pts',(-3.07956989313146,-0.158333333333386,
10.189486269028));
#33760=CARTESIAN_POINT('Ctrl Pts',(-3.06373460659005,0.158333333333388,
10.2059523010134));
#33761=CARTESIAN_POINT('Ctrl Pts',(-3.07606165687102,0.319434907277274,
10.227261115237));
#33762=CARTESIAN_POINT('Ctrl Pts',(-3.116242644995,0.63630980009542,10.2897345264231));
#33763=CARTESIAN_POINT('Ctrl Pts',(-3.15420785454821,0.79477268400111,10.3344921720662));
#33764=CARTESIAN_POINT('Ctrl Pts',(-3.22583655900311,1.06847604194623,10.428013227239));
#33765=CARTESIAN_POINT('Ctrl Pts',(-3.26127444105666,1.18514270861367,10.4742267922661));
#33766=CARTESIAN_POINT('Ctrl Pts',(-3.30114479311019,1.30000000000264,10.5261721228327));
#33767=CARTESIAN_POINT('Ctrl Pts',(-3.43444272475388,-1.30000000000054,
10.3549066020539));
#33768=CARTESIAN_POINT('Ctrl Pts',(-3.37747777932839,-1.18514270861223,
10.3141508035821));
#33769=CARTESIAN_POINT('Ctrl Pts',(-3.32566871721267,-1.06847604194547,
10.2801253752984));
#33770=CARTESIAN_POINT('Ctrl Pts',(-3.21789054123447,-0.794772684001071,
10.2170683307399));
#33771=CARTESIAN_POINT('Ctrl Pts',(-3.16022877986869,-0.636309800095372,
10.19386882768));
#33772=CARTESIAN_POINT('Ctrl Pts',(-3.08551117227782,-0.319434907277247,
10.1670275964095));
#33773=CARTESIAN_POINT('Ctrl Pts',(-3.05948635543789,-0.158333333333376,
10.1621534237937));
#33774=CARTESIAN_POINT('Ctrl Pts',(-3.04426266656423,0.158333333333378,
10.1780338017966));
#33775=CARTESIAN_POINT('Ctrl Pts',(-3.05611868438866,0.319434907277256,
10.1976691980544));
#33776=CARTESIAN_POINT('Ctrl Pts',(-3.09767799919942,0.636309800095382,
10.2591372527431));
#33777=CARTESIAN_POINT('Ctrl Pts',(-3.13673010463398,0.79477268400106,10.3018913725775));
#33778=CARTESIAN_POINT('Ctrl Pts',(-3.2117957519062,1.06847604194616,10.3989965816232));
#33779=CARTESIAN_POINT('Ctrl Pts',(-3.24913105512162,1.18514270861359,10.4480394373749));
#33780=CARTESIAN_POINT('Ctrl Pts',(-3.29130852430455,1.30000000000256,10.5040919019848));
#33781=CARTESIAN_POINT('Ctrl Pts',(-3.4258722715173,-1.30000000000042,10.3393534519172));
#33782=CARTESIAN_POINT('Ctrl Pts',(-3.3668675213799,-1.18514270861212,10.2959381003515));
#33783=CARTESIAN_POINT('Ctrl Pts',(-3.31344654722717,-1.06847604194537,
10.2600789851213));
#33784=CARTESIAN_POINT('Ctrl Pts',(-3.20293304966028,-0.794772684000992,
10.1946936729031));
#33785=CARTESIAN_POINT('Ctrl Pts',(-3.14481525590605,-0.636309800095313,
10.172787671385));
#33786=CARTESIAN_POINT('Ctrl Pts',(-3.06922746540355,-0.319434907277219,
10.1465725101371));
#33787=CARTESIAN_POINT('Ctrl Pts',(-3.04322309875081,-0.158333333333361,
10.1431059236598));
#33788=CARTESIAN_POINT('Ctrl Pts',(-3.02833554978959,0.158333333333363,
10.1586363454208));
#33789=CARTESIAN_POINT('Ctrl Pts',(-3.04050029213829,0.319434907277224,
10.1764674528015));
#33790=CARTESIAN_POINT('Ctrl Pts',(-3.08362867027232,0.636309800095321,
10.2366918210486));
#33791=CARTESIAN_POINT('Ctrl Pts',(-3.12363637801034,0.794772684000988,
10.2778011992827));
#33792=CARTESIAN_POINT('Ctrl Pts',(-3.20185073556315,1.06847604194606,10.377011123269));
#33793=CARTESIAN_POINT('Ctrl Pts',(-3.24090185094023,1.18514270861348,10.427870915147));
#33794=CARTESIAN_POINT('Ctrl Pts',(-3.28514798443724,1.30000000000244,10.4866461988992));
#33795=CARTESIAN_POINT('Ctrl Pts',(-3.41721009436127,-1.30000000000036,
10.3237432942192));
#33796=CARTESIAN_POINT('Ctrl Pts',(-3.35605655066583,-1.18514270861207,
10.2775200347506));
#33797=CARTESIAN_POINT('Ctrl Pts',(-3.30084535509438,-1.06847604194533,
10.2398021730802));
#33798=CARTESIAN_POINT('Ctrl Pts',(-3.18702446129158,-0.794772684000962,
10.1723155376019));
#33799=CARTESIAN_POINT('Ctrl Pts',(-3.12697012194977,-0.636309800095285,
10.15303905683));
#33800=CARTESIAN_POINT('Ctrl Pts',(-3.05144450916497,-0.319434907277203,
10.1265784713633));
#33801=CARTESIAN_POINT('Ctrl Pts',(-3.02869685173172,-0.158333333333355,
10.1216965641621));
#33802=CARTESIAN_POINT('Ctrl Pts',(-3.01462692612418,0.158333333333357,
10.1364364939386));
#33803=CARTESIAN_POINT('Ctrl Pts',(-3.02483723154194,0.319434907277213,
10.1544033900266));
#33804=CARTESIAN_POINT('Ctrl Pts',(-3.06858167687439,0.636309800095296,
10.2142591465703));
#33805=CARTESIAN_POINT('Ctrl Pts',(-3.10986244179941,0.794772684000952,
10.2534454206316));
#33806=CARTESIAN_POINT('Ctrl Pts',(-3.19101517929812,1.06847604194602,10.3551902348169));
#33807=CARTESIAN_POINT('Ctrl Pts',(-3.23167729713891,1.18514270861343,10.4081154683092));
#33808=CARTESIAN_POINT('Ctrl Pts',(-3.27787351976245,1.30000000000239,10.4699243752498));
#33809=CARTESIAN_POINT('Ctrl Pts',(-3.41007224859412,-1.3000000000003,10.3108264414936));
#33810=CARTESIAN_POINT('Ctrl Pts',(-3.34662820042611,-1.18514270861202,
10.2630357435561));
#33811=CARTESIAN_POINT('Ctrl Pts',(-3.28989222434501,-1.06847604194528,
10.2240457564814));
#33812=CARTESIAN_POINT('Ctrl Pts',(-3.17431775807052,-0.794772684000926,
10.1543024890875));
#33813=CARTESIAN_POINT('Ctrl Pts',(-3.11591086660822,-0.636309800095255,
10.1342856641298));
#33814=CARTESIAN_POINT('Ctrl Pts',(-3.04098812630273,-0.319434907277188,
10.1072387673856));
#33815=CARTESIAN_POINT('Ctrl Pts',(-3.01902837233301,-0.158333333333347,
10.1029077311548));
#33816=CARTESIAN_POINT('Ctrl Pts',(-3.00449374065794,0.158333333333349,
10.1180418711654));
#33817=CARTESIAN_POINT('Ctrl Pts',(-3.0127637651021,0.319434907277197,10.1364598249738));
#33818=CARTESIAN_POINT('Ctrl Pts',(-3.05635950237011,0.636309800095265,
10.1964669919186));
#33819=CARTESIAN_POINT('Ctrl Pts',(-3.09844750254128,0.794772684000913,
10.2341642937794));
#33820=CARTESIAN_POINT('Ctrl Pts',(-3.18175214399387,1.06847604194597,10.3378593563706));
#33821=CARTESIAN_POINT('Ctrl Pts',(-3.22367765549952,1.18514270861338,10.3923324889705));
#33822=CARTESIAN_POINT('Ctrl Pts',(-3.27146918596705,1.30000000000232,10.4563930038551));
#33823=CARTESIAN_POINT('Ctrl Pts',(-3.40085406844961,-1.30000000000027,
10.2957145443334));
#33824=CARTESIAN_POINT('Ctrl Pts',(-3.33439270608681,-1.18514270861199,
10.245758638802));
#33825=CARTESIAN_POINT('Ctrl Pts',(-3.2757464998873,-1.06847604194525,10.2048938980597));
#33826=CARTESIAN_POINT('Ctrl Pts',(-3.15831660558689,-0.794772684000905,
10.1314905813258));
#33827=CARTESIAN_POINT('Ctrl Pts',(-3.10274865638003,-0.63630980009524,
10.1096261219701));
#33828=CARTESIAN_POINT('Ctrl Pts',(-3.02931459861233,-0.31943490727718,
10.0809918745011));
#33829=CARTESIAN_POINT('Ctrl Pts',(-3.00853263993761,-0.158333333333343,
10.0772919082541));
#33830=CARTESIAN_POINT('Ctrl Pts',(-2.99406174270539,0.158333333333345,
10.0923384537343));
#33831=CARTESIAN_POINT('Ctrl Pts',(-3.00096348447118,0.319434907277189,
10.1102436642837));
#33832=CARTESIAN_POINT('Ctrl Pts',(-3.04371819322789,0.636309800095249,
10.1712403114327));
#33833=CARTESIAN_POINT('Ctrl Pts',(-3.08435585321636,0.794772684000894,
10.2095531317405));
#33834=CARTESIAN_POINT('Ctrl Pts',(-3.16967607158215,1.06847604194594,10.316836258828));
#33835=CARTESIAN_POINT('Ctrl Pts',(-3.21328275026215,1.18514270861335,10.3734354818652));
#33836=CARTESIAN_POINT('Ctrl Pts',(-3.26356414651715,1.30000000000229,10.440195037455));
#33837=CARTESIAN_POINT('Ctrl Pts',(-3.39465878599097,-1.30000000000019,
10.2853534708596));
#33838=CARTESIAN_POINT('Ctrl Pts',(-3.32511928143436,-1.18514270861191,
10.2348322744866));
#33839=CARTESIAN_POINT('Ctrl Pts',(-3.26484306626976,-1.06847604194518,
10.1931031343358));
#33840=CARTESIAN_POINT('Ctrl Pts',(-3.14699300263423,-0.794772684000851,
10.1170118814196));
#33841=CARTESIAN_POINT('Ctrl Pts',(-3.09695175410121,-0.636309800095197,
10.0915712362322));
#33842=CARTESIAN_POINT('Ctrl Pts',(-3.02637472772942,-0.319434907277159,
10.0609469829604));
#33843=CARTESIAN_POINT('Ctrl Pts',(-3.00611348042902,-0.158333333333332,
10.058191722331));
#33844=CARTESIAN_POINT('Ctrl Pts',(-2.99178541075593,0.158333333333334,
10.0731598884958));
#33845=CARTESIAN_POINT('Ctrl Pts',(-2.99824596807587,0.319434907277167,
10.0901842798419));
#33846=CARTESIAN_POINT('Ctrl Pts',(-3.03856351371756,0.636309800095206,
10.1527214947233));
#33847=CARTESIAN_POINT('Ctrl Pts',(-3.07432779059338,0.79477268400084,10.1936664632184));
#33848=CARTESIAN_POINT('Ctrl Pts',(-3.16003000210956,1.06847604194587,10.3036861053275));
#33849=CARTESIAN_POINT('Ctrl Pts',(-3.2050733914081,1.18514270861327,10.3614091951292));
#33850=CARTESIAN_POINT('Ctrl Pts',(-3.25806285821962,1.30000000000221,10.4292319482927));
#33851=CARTESIAN_POINT('Ctrl Pts',(-3.39267401414631,-1.30000000000019,
10.276983507709));
#33852=CARTESIAN_POINT('Ctrl Pts',(-3.32322027641436,-1.18514270861191,
10.226698532237));
#33853=CARTESIAN_POINT('Ctrl Pts',(-3.26328889377517,-1.06847604194518,
10.1849734474866));
#33854=CARTESIAN_POINT('Ctrl Pts',(-3.1468339558515,-0.794772684000851,
10.1083552146057));
#33855=CARTESIAN_POINT('Ctrl Pts',(-3.09896529592857,-0.636309800095197,
10.0815496804376));
#33856=CARTESIAN_POINT('Ctrl Pts',(-3.02984981618038,-0.319434907277159,
10.0500837393884));
#33857=CARTESIAN_POINT('Ctrl Pts',(-3.00954349196179,-0.158333333333332,
10.0473018664685));
#33858=CARTESIAN_POINT('Ctrl Pts',(-2.99543061314513,0.158333333333334,
10.0621711387216));
#33859=CARTESIAN_POINT('Ctrl Pts',(-3.0023925612396,0.319434907277167,10.078980785313));
#33860=CARTESIAN_POINT('Ctrl Pts',(-3.04119573834857,0.636309800095206,
10.14244843534));
#33861=CARTESIAN_POINT('Ctrl Pts',(-3.0738873794296,0.79477268400084,10.1853620261542));
#33862=CARTESIAN_POINT('Ctrl Pts',(-3.15831522453578,1.06847604194587,10.2958137160522));
#33863=CARTESIAN_POINT('Ctrl Pts',(-3.20327264332997,1.18514270861327,10.3533447434002));
#33864=CARTESIAN_POINT('Ctrl Pts',(-3.25664179513173,1.30000000000221,10.4205963541777));
#33865=CARTESIAN_POINT('Ctrl Pts',(-3.39267401414619,-1.3,10.2769835077089));
#33866=CARTESIAN_POINT('Ctrl Pts',(-3.3232202764143,-1.18514270861178,10.226698532237));
#33867=CARTESIAN_POINT('Ctrl Pts',(-3.26328889377514,-1.06847604194512,
10.1849734474866));
#33868=CARTESIAN_POINT('Ctrl Pts',(-3.1468339558515,-0.794772684000851,
10.1083552146057));
#33869=CARTESIAN_POINT('Ctrl Pts',(-3.09896529592857,-0.636309800095197,
10.0815496804376));
#33870=CARTESIAN_POINT('Ctrl Pts',(-3.02984981618038,-0.319434907277159,
10.0500837393884));
#33871=CARTESIAN_POINT('Ctrl Pts',(-3.00954349196179,-0.158333333333332,
10.0473018664685));
#33872=CARTESIAN_POINT('Ctrl Pts',(-2.99543061314513,0.158333333333334,
10.0621711387217));
#33873=CARTESIAN_POINT('Ctrl Pts',(-3.0023925612396,0.319434907277167,10.078980785313));
#33874=CARTESIAN_POINT('Ctrl Pts',(-3.04119573834858,0.636309800095206,
10.14244843534));
#33875=CARTESIAN_POINT('Ctrl Pts',(-3.0738873794296,0.79477268400084,10.1853620261542));
#33876=CARTESIAN_POINT('Ctrl Pts',(-3.15831522453555,1.06847604194511,10.2958137160519));
#33877=CARTESIAN_POINT('Ctrl Pts',(-3.2032726433294,1.18514270861178,10.3533447433995));
#33878=CARTESIAN_POINT('Ctrl Pts',(-3.25664179513071,1.3,10.4205963541764));
#33879=CARTESIAN_POINT('',(-3.53203864909401,-1.2,10.6680258045906));
#33880=CARTESIAN_POINT('Ctrl Pts',(-3.53203864909401,-1.2,10.6680258045906));
#33881=CARTESIAN_POINT('Ctrl Pts',(-3.52949649314404,-1.21682298576918,
10.6466030151777));
#33882=CARTESIAN_POINT('Ctrl Pts',(-3.52798214088104,-1.23318431453843,
10.624704621099));
#33883=CARTESIAN_POINT('Ctrl Pts',(-3.52274184472548,-1.26590569890439,
10.5830210172903));
#33884=CARTESIAN_POINT('Ctrl Pts',(-3.5205885687882,-1.28162309756721,10.5625446886959));
#33885=CARTESIAN_POINT('Ctrl Pts',(-3.51745747224793,-1.2984297825913,10.5414408389829));
#33886=CARTESIAN_POINT('Ctrl Pts',(-3.51730897053275,-1.29921484486248,
10.5404572435777));
#33887=CARTESIAN_POINT('Ctrl Pts',(-3.51715788243336,-1.30000000000224,
10.5394760711847));
#33888=CARTESIAN_POINT('',(-3.42060206480302,-0.653834841417127,10.7779856782843));
#33889=CARTESIAN_POINT('Ctrl Pts',(-3.42060206482294,-0.653834841416443,
10.7779856783013));
#33890=CARTESIAN_POINT('Ctrl Pts',(-3.43236036060181,-0.717945624492541,
10.7667445905954));
#33891=CARTESIAN_POINT('Ctrl Pts',(-3.44189203683076,-0.763782257331169,
10.757549404514));
#33892=CARTESIAN_POINT('Ctrl Pts',(-3.4790210626449,-0.949542760432358,
10.7213842943359));
#33893=CARTESIAN_POINT('Ctrl Pts',(-3.49909315631117,-1.04876680996024,
10.7015794055091));
#33894=CARTESIAN_POINT('Ctrl Pts',(-3.53203864909401,-1.2,10.6680258045906));
#33895=CARTESIAN_POINT('',(-3.31841464832137,0.653834841531101,10.8729585107657));
#33896=CARTESIAN_POINT('Ctrl Pts',(-3.31841464832137,0.653834841531102,
10.8729585107657));
#33897=CARTESIAN_POINT('Ctrl Pts',(-3.30609938026503,0.575796605817473,
10.8331482966237));
#33898=CARTESIAN_POINT('Ctrl Pts',(-3.29643526076467,0.493919104637004,
10.799577764871));
#33899=CARTESIAN_POINT('Ctrl Pts',(-3.28487506509149,0.338196295579431,
10.7502176157553));
#33900=CARTESIAN_POINT('Ctrl Pts',(-3.28202732600753,0.265710097563185,
10.7325309479634));
#33901=CARTESIAN_POINT('Ctrl Pts',(-3.28242869861854,0.129740215298289,
10.70812432938));
#33902=CARTESIAN_POINT('Ctrl Pts',(-3.28482835999103,0.066640938344181,
10.7001962776734));
#33903=CARTESIAN_POINT('Ctrl Pts',(-3.29434436054939,-0.0595500090171539,
10.6908442069019));
#33904=CARTESIAN_POINT('Ctrl Pts',(-3.30152115228924,-0.122795915650191,
10.6893370787071));
#33905=CARTESIAN_POINT('Ctrl Pts',(-3.32179927220444,-0.260148629827643,
10.6937120240392));
#33906=CARTESIAN_POINT('Ctrl Pts',(-3.33574425320147,-0.333949114798701,
10.7009893453216));
#33907=CARTESIAN_POINT('Ctrl Pts',(-3.37150302708504,-0.491142723769832,
10.728020880275));
#33908=CARTESIAN_POINT('Ctrl Pts',(-3.39445736914294,-0.574254147968246,
10.7496580885196));
#33909=CARTESIAN_POINT('Ctrl Pts',(-3.42060206481036,-0.653834841428803,
10.7779856782448));
#33910=CARTESIAN_POINT('',(-3.37162231815327,1.2,10.8241775541122));
#33911=CARTESIAN_POINT('Ctrl Pts',(-3.37162231815327,1.2,10.8241775541122));
#33912=CARTESIAN_POINT('Ctrl Pts',(-3.36246959501592,1.13404402018397,10.8326924585674));
#33913=CARTESIAN_POINT('Ctrl Pts',(-3.35047549472867,1.03816619550936,10.8437839273622));
#33914=CARTESIAN_POINT('Ctrl Pts',(-3.32701157089733,0.79525632445983,10.8651966335573));
#33915=CARTESIAN_POINT('Ctrl Pts',(-3.32327568128371,0.741437054735132,
10.8685667042857));
#33916=CARTESIAN_POINT('Ctrl Pts',(-3.31841464832137,0.653834841531101,
10.8729585107657));
#33917=CARTESIAN_POINT('Ctrl Pts',(-3.35750281628589,1.30000000000061,10.699953548067));
#33918=CARTESIAN_POINT('Ctrl Pts',(-3.36044168963578,1.28316801238108,10.7204589243298));
#33919=CARTESIAN_POINT('Ctrl Pts',(-3.36254952465714,1.26661750999833,10.7413041016838));
#33920=CARTESIAN_POINT('Ctrl Pts',(-3.36761026216994,1.23437943378003,10.7808733082656));
#33921=CARTESIAN_POINT('Ctrl Pts',(-3.37028225138757,1.21555984826321,10.8041721739107));
#33922=CARTESIAN_POINT('Ctrl Pts',(-3.37162231815327,1.2,10.8241775541122));
#33923=CARTESIAN_POINT('Ctrl Pts',(-3.39267401414619,-1.3,10.2769835077089));
#33924=CARTESIAN_POINT('Ctrl Pts',(-3.32322027641429,-1.18514270861178,
10.226698532237));
#33925=CARTESIAN_POINT('Ctrl Pts',(-3.26328889377514,-1.06847604194512,
10.1849734474866));
#33926=CARTESIAN_POINT('Ctrl Pts',(-3.14683395585151,-0.794772684000851,
10.1083552146057));
#33927=CARTESIAN_POINT('Ctrl Pts',(-3.09896529592857,-0.636309800095197,
10.0815496804376));
#33928=CARTESIAN_POINT('Ctrl Pts',(-3.02984981618038,-0.319434907277159,
10.0500837393884));
#33929=CARTESIAN_POINT('Ctrl Pts',(-3.00954349196179,-0.158333333333332,
10.0473018664685));
#33930=CARTESIAN_POINT('Ctrl Pts',(-2.99543061314513,0.158333333333334,
10.0621711387216));
#33931=CARTESIAN_POINT('Ctrl Pts',(-3.0023925612396,0.319434907277167,10.078980785313));
#33932=CARTESIAN_POINT('Ctrl Pts',(-3.04119573834858,0.636309800095206,
10.14244843534));
#33933=CARTESIAN_POINT('Ctrl Pts',(-3.0738873794296,0.79477268400084,10.1853620261542));
#33934=CARTESIAN_POINT('Ctrl Pts',(-3.15831522453555,1.06847604194511,10.2958137160519));
#33935=CARTESIAN_POINT('Ctrl Pts',(-3.2032726433294,1.18514270861178,10.3533447433995));
#33936=CARTESIAN_POINT('Ctrl Pts',(-3.25664179513071,1.3,10.4205963541764));
#33937=CARTESIAN_POINT('Ctrl Pts',(-3.44290446030743,-1.3,10.2187081994464));
#33938=CARTESIAN_POINT('Ctrl Pts',(-3.37244803687278,-1.18514270861178,
10.1698358549729));
#33939=CARTESIAN_POINT('Ctrl Pts',(-3.31185538302694,-1.06847604194512,
10.129119962649));
#33940=CARTESIAN_POINT('Ctrl Pts',(-3.19466151211464,-0.794772684000851,
10.0539011423529));
#33941=CARTESIAN_POINT('Ctrl Pts',(-3.14738383460686,-0.636309800095197,
10.026688499191));
#33942=CARTESIAN_POINT('Ctrl Pts',(-3.07891484675056,-0.319434907277159,
9.99505906071815));
#33943=CARTESIAN_POINT('Ctrl Pts',(-3.05956220283012,-0.158333333333332,
9.99148223767552));
#33944=CARTESIAN_POINT('Ctrl Pts',(-3.04571607718934,0.158333333333334,
10.0065916955671));
#33945=CARTESIAN_POINT('Ctrl Pts',(-3.05198711671705,0.319434907277167,
10.0244328930108));
#33946=CARTESIAN_POINT('Ctrl Pts',(-3.09069526886232,0.636309800095206,
10.0885605835139));
#33947=CARTESIAN_POINT('Ctrl Pts',(-3.12304380561888,0.79477268400084,10.1321044737573));
#33948=CARTESIAN_POINT('Ctrl Pts',(-3.20878615765139,1.06847604194511,10.2416750001716));
#33949=CARTESIAN_POINT('Ctrl Pts',(-3.25467811874699,1.18514270861178,10.2984428894918));
#33950=CARTESIAN_POINT('Ctrl Pts',(-3.30934735381061,1.3,10.3645496472358));
#33951=CARTESIAN_POINT('Ctrl Pts',(-3.49313490646867,-1.3,10.1604328911839));
#33952=CARTESIAN_POINT('Ctrl Pts',(-3.42167579733126,-1.18514270861178,
10.1129731777087));
#33953=CARTESIAN_POINT('Ctrl Pts',(-3.36042187227873,-1.06847604194512,
10.0732664778114));
#33954=CARTESIAN_POINT('Ctrl Pts',(-3.24248906837778,-0.794772684000851,
9.99944707010019));
#33955=CARTESIAN_POINT('Ctrl Pts',(-3.19580237328515,-0.636309800095197,
9.97182731794448));
#33956=CARTESIAN_POINT('Ctrl Pts',(-3.12797987732075,-0.319434907277159,
9.94003438204794));
#33957=CARTESIAN_POINT('Ctrl Pts',(-3.10958091369845,-0.158333333333332,
9.93566260888258));
#33958=CARTESIAN_POINT('Ctrl Pts',(-3.09600154123355,0.158333333333334,
9.95101225241256));
#33959=CARTESIAN_POINT('Ctrl Pts',(-3.10158167219449,0.319434907277167,
9.96988500070868));
#33960=CARTESIAN_POINT('Ctrl Pts',(-3.14019479937607,0.636309800095206,
10.0346727316879));
#33961=CARTESIAN_POINT('Ctrl Pts',(-3.17220023180817,0.79477268400084,10.0788469213604));
#33962=CARTESIAN_POINT('Ctrl Pts',(-3.25925709076722,1.06847604194511,10.1875362842913));
#33963=CARTESIAN_POINT('Ctrl Pts',(-3.30608359416459,1.18514270861178,10.2435410355842));
#33964=CARTESIAN_POINT('Ctrl Pts',(-3.3620529124905,1.3,10.3085029402952));
#33965=CARTESIAN_POINT('Ctrl Pts',(-3.54336535262991,-1.3,10.1021575829215));
#33966=CARTESIAN_POINT('Ctrl Pts',(-3.47090355778975,-1.18514270861178,
10.0561105004446));
#33967=CARTESIAN_POINT('Ctrl Pts',(-3.40898836153053,-1.06847604194512,
10.0174129929737));
#33968=CARTESIAN_POINT('Ctrl Pts',(-3.29031662464092,-0.794772684000851,
9.94499299784744));
#33969=CARTESIAN_POINT('Ctrl Pts',(-3.24422091196344,-0.636309800095197,
9.91696613669794));
#33970=CARTESIAN_POINT('Ctrl Pts',(-3.17704490789093,-0.319434907277159,
9.88500970337774));
#33971=CARTESIAN_POINT('Ctrl Pts',(-3.15959962456678,-0.158333333333332,
9.87984298008964));
#33972=CARTESIAN_POINT('Ctrl Pts',(-3.14628700527777,0.158333333333334,
9.89543280925802));
#33973=CARTESIAN_POINT('Ctrl Pts',(-3.15117622767193,0.319434907277167,
9.91533710840653));
#33974=CARTESIAN_POINT('Ctrl Pts',(-3.18969432988981,0.636309800095206,
9.98078487986183));
#33975=CARTESIAN_POINT('Ctrl Pts',(-3.22135665799746,0.79477268400084,10.0255893689635));
#33976=CARTESIAN_POINT('Ctrl Pts',(-3.30972802388306,1.06847604194511,10.133397568411));
#33977=CARTESIAN_POINT('Ctrl Pts',(-3.35748906958219,1.18514270861178,10.1886391816766));
#33978=CARTESIAN_POINT('Ctrl Pts',(-3.4147584711704,1.3,10.2524562333546));
#33979=CARTESIAN_POINT('Ctrl Pts',(-3.54336535262991,-1.3,10.1021575829215));
#33980=CARTESIAN_POINT('Ctrl Pts',(-3.47090355778975,-1.18514270861178,
10.0561105004446));
#33981=CARTESIAN_POINT('Ctrl Pts',(-3.40898836153053,-1.06847604194512,
10.0174129929737));
#33982=CARTESIAN_POINT('Ctrl Pts',(-3.29031662464092,-0.794772684000851,
9.94499299784744));
#33983=CARTESIAN_POINT('Ctrl Pts',(-3.24422091196343,-0.636309800095197,
9.91696613669794));
#33984=CARTESIAN_POINT('Ctrl Pts',(-3.17704490789093,-0.319434907277159,
9.88500970337774));
#33985=CARTESIAN_POINT('Ctrl Pts',(-3.15959962456678,-0.158333333333332,
9.87984298008964));
#33986=CARTESIAN_POINT('Ctrl Pts',(-3.14628700527777,0.158333333333334,
9.89543280925802));
#33987=CARTESIAN_POINT('Ctrl Pts',(-3.15117622767194,0.319434907277167,
9.91533710840653));
#33988=CARTESIAN_POINT('Ctrl Pts',(-3.18969432988982,0.636309800095206,
9.98078487986184));
#33989=CARTESIAN_POINT('Ctrl Pts',(-3.22135665799746,0.79477268400084,10.0255893689635));
#33990=CARTESIAN_POINT('Ctrl Pts',(-3.30972802388306,1.06847604194511,10.133397568411));
#33991=CARTESIAN_POINT('Ctrl Pts',(-3.35748906958219,1.18514270861178,10.1886391816766));
#33992=CARTESIAN_POINT('Ctrl Pts',(-3.4147584711704,1.3,10.2524562333546));
#33993=CARTESIAN_POINT('Ctrl Pts',(-3.54336535262998,-1.30000000000011,
10.1021575829215));
#33994=CARTESIAN_POINT('Ctrl Pts',(-3.47090355778979,-1.18514270861186,
10.0561105004446));
#33995=CARTESIAN_POINT('Ctrl Pts',(-3.40898836153054,-1.06847604194515,
10.0174129929738));
#33996=CARTESIAN_POINT('Ctrl Pts',(-3.29031662464092,-0.794772684000851,
9.94499299784743));
#33997=CARTESIAN_POINT('Ctrl Pts',(-3.24422091196343,-0.636309800095196,
9.91696613669794));
#33998=CARTESIAN_POINT('Ctrl Pts',(-3.17704490789093,-0.319434907277159,
9.88500970337773));
#33999=CARTESIAN_POINT('Ctrl Pts',(-3.15959962456677,-0.158333333333332,
9.87984298008964));
#34000=CARTESIAN_POINT('Ctrl Pts',(-3.14628700527777,0.158333333333334,
9.89543280925802));
#34001=CARTESIAN_POINT('Ctrl Pts',(-3.15117622767193,0.319434907277167,
9.91533710840652));
#34002=CARTESIAN_POINT('Ctrl Pts',(-3.18969432988981,0.636309800095206,
9.98078487986183));
#34003=CARTESIAN_POINT('Ctrl Pts',(-3.22135665799746,0.79477268400084,10.0255893689635));
#34004=CARTESIAN_POINT('Ctrl Pts',(-3.30972802388312,1.06847604194529,10.133397568411));
#34005=CARTESIAN_POINT('Ctrl Pts',(-3.35748906958234,1.18514270861213,10.1886391816768));
#34006=CARTESIAN_POINT('Ctrl Pts',(-3.41475847117067,1.30000000000053,10.2524562333549));
#34007=CARTESIAN_POINT('Ctrl Pts',(-3.55210218155249,-1.30000000000011,
10.102668195856));
#34008=CARTESIAN_POINT('Ctrl Pts',(-3.4791120609986,-1.18514270861186,10.0570584190558));
#34009=CARTESIAN_POINT('Ctrl Pts',(-3.41699686806357,-1.06847604194515,
10.0182954880324));
#34010=CARTESIAN_POINT('Ctrl Pts',(-3.29862160460325,-0.794772684000851,
9.94456294632176));
#34011=CARTESIAN_POINT('Ctrl Pts',(-3.25416255203501,-0.636309800095196,
9.91327450453827));
#34012=CARTESIAN_POINT('Ctrl Pts',(-3.18775359145326,-0.319434907277159,
9.87971474158285));
#34013=CARTESIAN_POINT('Ctrl Pts',(-3.17014714932986,-0.158333333333332,
9.8750691092973));
#34014=CARTESIAN_POINT('Ctrl Pts',(-3.15675867145257,0.158333333333334,
9.89088328771536));
#34015=CARTESIAN_POINT('Ctrl Pts',(-3.16161671556929,0.319434907277167,
9.91074553866713));
#34016=CARTESIAN_POINT('Ctrl Pts',(-3.19945051410825,0.636309800095206,
9.97773483059028));
#34017=CARTESIAN_POINT('Ctrl Pts',(-3.22998252758134,0.79477268400084,10.0248426763756));
#34018=CARTESIAN_POINT('Ctrl Pts',(-3.31797563069844,1.06847604194529,10.1340934432942));
#34019=CARTESIAN_POINT('Ctrl Pts',(-3.36577675439403,1.18514270861213,10.1896775761499));
#34020=CARTESIAN_POINT('Ctrl Pts',(-3.42329004791162,1.30000000000053,10.2535552330021));
#34021=CARTESIAN_POINT('Ctrl Pts',(-3.5635999009408,-1.30000000000012,10.1069613837584));
#34022=CARTESIAN_POINT('Ctrl Pts',(-3.49195235234982,-1.18514270861186,
10.0639305254688));
#34023=CARTESIAN_POINT('Ctrl Pts',(-3.4311052249638,-1.06847604194516,10.0264789131465));
#34024=CARTESIAN_POINT('Ctrl Pts',(-3.31548732187626,-0.794772684000854,
9.95284737082135));
#34025=CARTESIAN_POINT('Ctrl Pts',(-3.27312737539359,-0.636309800095199,
9.91645281846877));
#34026=CARTESIAN_POINT('Ctrl Pts',(-3.20798504741422,-0.319434907277159,
9.88032500074145));
#34027=CARTESIAN_POINT('Ctrl Pts',(-3.18944580480551,-0.158333333333333,
9.87534702119606));
#34028=CARTESIAN_POINT('Ctrl Pts',(-3.17599570552034,0.158333333333335,
9.89131075156943));
#34029=CARTESIAN_POINT('Ctrl Pts',(-3.18186432348549,0.319434907277169,
9.91157121719164));
#34030=CARTESIAN_POINT('Ctrl Pts',(-3.21802203393935,0.636309800095209,
9.98160364984369));
#34031=CARTESIAN_POINT('Ctrl Pts',(-3.24556763131071,0.794772684000842,
10.0345895015107));
#34032=CARTESIAN_POINT('Ctrl Pts',(-3.33084003434444,1.06847604194529,10.1437070747227));
#34033=CARTESIAN_POINT('Ctrl Pts',(-3.37760980803081,1.18514270861214,10.1977620137398));
#34034=CARTESIAN_POINT('Ctrl Pts',(-3.43423809178417,1.30000000000053,10.2586389375353));
#34035=CARTESIAN_POINT('Ctrl Pts',(-3.58052453593308,-1.30000000000012,
10.1131512829018));
#34036=CARTESIAN_POINT('Ctrl Pts',(-3.51182111180035,-1.18514270861186,
10.0723212585934));
#34037=CARTESIAN_POINT('Ctrl Pts',(-3.45326554656784,-1.06847604194516,
10.03632181748));
#34038=CARTESIAN_POINT('Ctrl Pts',(-3.34143406101177,-0.794772684000854,
9.96431552037965));
#34039=CARTESIAN_POINT('Ctrl Pts',(-3.29954742189089,-0.6363098000952,9.92639412658323));
#34040=CARTESIAN_POINT('Ctrl Pts',(-3.23531051004868,-0.319434907277161,
9.88931318271086));
#34041=CARTESIAN_POINT('Ctrl Pts',(-3.21611582752958,-0.158333333333333,
9.88302883410783));
#34042=CARTESIAN_POINT('Ctrl Pts',(-3.20259452330713,0.158333333333335,
9.89905411840604));
#34043=CARTESIAN_POINT('Ctrl Pts',(-3.20923276053098,0.319434907277168,
9.92040043925532));
#34044=CARTESIAN_POINT('Ctrl Pts',(-3.2439624010757,0.636309800095209,9.99208593067343));
#34045=CARTESIAN_POINT('Ctrl Pts',(-3.26993455454521,0.794772684000845,
10.0481295568208));
#34046=CARTESIAN_POINT('Ctrl Pts',(-3.35136767971977,1.0684760419453,10.1557832977204));
#34047=CARTESIAN_POINT('Ctrl Pts',(-3.39607665566982,1.18514270861214,10.2081250226386));
#34048=CARTESIAN_POINT('Ctrl Pts',(-3.4502452250765,1.30000000000053,10.2662091570036));
#34049=CARTESIAN_POINT('Ctrl Pts',(-3.59470999228296,-1.30000000000012,
10.1179996604394));
#34050=CARTESIAN_POINT('Ctrl Pts',(-3.52841604334897,-1.18514270861187,
10.0784975008717));
#34051=CARTESIAN_POINT('Ctrl Pts',(-3.47152795348144,-1.06847604194516,
10.0435856794783));
#34052=CARTESIAN_POINT('Ctrl Pts',(-3.36183450154324,-0.794772684000855,
9.97353698745057));
#34053=CARTESIAN_POINT('Ctrl Pts',(-3.31850387428926,-0.636309800095199,
9.93665114702491));
#34054=CARTESIAN_POINT('Ctrl Pts',(-3.25436105612193,-0.31943490727716,
9.89946741885329));
#34055=CARTESIAN_POINT('Ctrl Pts',(-3.23540186323813,-0.158333333333333,
9.89122756687286));
#34056=CARTESIAN_POINT('Ctrl Pts',(-3.22220303021708,0.158333333333335,
9.90677602232352));
#34057=CARTESIAN_POINT('Ctrl Pts',(-3.22944979183797,0.31943490727717,9.92886386820246));
#34058=CARTESIAN_POINT('Ctrl Pts',(-3.26367984413207,0.63630980009521,10.0011823983456));
#34059=CARTESIAN_POINT('Ctrl Pts',(-3.28915985991411,0.794772684000842,
10.0588476958572));
#34060=CARTESIAN_POINT('Ctrl Pts',(-3.36817452647295,1.06847604194529,10.1650030429831));
#34061=CARTESIAN_POINT('Ctrl Pts',(-3.41144891624779,1.18514270861214,10.2159886719713));
#34062=CARTESIAN_POINT('Ctrl Pts',(-3.46379517442606,1.30000000000054,10.2720092136201));
#34063=CARTESIAN_POINT('Ctrl Pts',(-3.60911751064946,-1.30000000000012,
10.1227295726391));
#34064=CARTESIAN_POINT('Ctrl Pts',(-3.54550367467917,-1.18514270861187,
10.0846191774548));
#34065=CARTESIAN_POINT('Ctrl Pts',(-3.49047558704248,-1.06847604194516,
10.0508755280719));
#34066=CARTESIAN_POINT('Ctrl Pts',(-3.38318449249417,-0.794772684000856,
9.98300900396935));
#34067=CARTESIAN_POINT('Ctrl Pts',(-3.33845114784564,-0.636309800095201,
9.94721788326197));
#34068=CARTESIAN_POINT('Ctrl Pts',(-3.2741201089056,-0.319434907277161,
9.91048396957203));
#34069=CARTESIAN_POINT('Ctrl Pts',(-3.25510443899921,-0.158333333333333,
9.9005970671488));
#34070=CARTESIAN_POINT('Ctrl Pts',(-3.2413673604884,0.158333333333335,9.91683651347412));
#34071=CARTESIAN_POINT('Ctrl Pts',(-3.24779972547716,0.319434907277169,
9.94167544852661));
#34072=CARTESIAN_POINT('Ctrl Pts',(-3.28179917085832,0.636309800095211,
10.0141103141042));
#34073=CARTESIAN_POINT('Ctrl Pts',(-3.30913046338384,0.794772684000846,
10.070145021745));
#34074=CARTESIAN_POINT('Ctrl Pts',(-3.38609183274489,1.0684760419453,10.1737301684728));
#34075=CARTESIAN_POINT('Ctrl Pts',(-3.42768849705096,1.18514270861214,10.2233422864552));
#34076=CARTESIAN_POINT('Ctrl Pts',(-3.47756810056647,1.30000000000053,10.2777283506095));
#34077=CARTESIAN_POINT('Ctrl Pts',(-3.62418184228244,-1.30000000000013,
10.1262166523165));
#34078=CARTESIAN_POINT('Ctrl Pts',(-3.56307216446774,-1.18514270861187,
10.0894944243691));
#34079=CARTESIAN_POINT('Ctrl Pts',(-3.50973124244813,-1.06847604194516,
10.0569771634264));
#34080=CARTESIAN_POINT('Ctrl Pts',(-3.40445042178884,-0.794772684000856,
9.99157010057452));
#34081=CARTESIAN_POINT('Ctrl Pts',(-3.35822909918292,-0.636309800095201,
9.95703313191003));
#34082=CARTESIAN_POINT('Ctrl Pts',(-3.29303524674374,-0.319434907277161,
9.92167902532558));
#34083=CARTESIAN_POINT('Ctrl Pts',(-3.27288063940016,-0.158333333333333,
9.91174316405932));
#34084=CARTESIAN_POINT('Ctrl Pts',(-3.25874017194707,0.158333333333336,
9.92847582885122));
#34085=CARTESIAN_POINT('Ctrl Pts',(-3.26576122781523,0.319434907277169,
9.9539858175574));
#34086=CARTESIAN_POINT('Ctrl Pts',(-3.30010095085377,0.636309800095211,
10.0257830146997));
#34087=CARTESIAN_POINT('Ctrl Pts',(-3.32891779836226,0.794772684000847,
10.0807296485886));
#34088=CARTESIAN_POINT('Ctrl Pts',(-3.40377037538339,1.0684760419453,10.1821617920228));
#34089=CARTESIAN_POINT('Ctrl Pts',(-3.44366765324861,1.18514270861214,10.230642064719));
#34090=CARTESIAN_POINT('Ctrl Pts',(-3.49106130194792,1.30000000000053,10.2836963936501));
#34091=CARTESIAN_POINT('Ctrl Pts',(-3.64724297519888,-1.30000000000012,
10.1335969392188));
#34092=CARTESIAN_POINT('Ctrl Pts',(-3.59027824508293,-1.18514270861187,
10.0990538498164));
#34093=CARTESIAN_POINT('Ctrl Pts',(-3.53982856865866,-1.06847604194516,
10.0683339334076));
#34094=CARTESIAN_POINT('Ctrl Pts',(-3.4383308010552,-0.794772684000858,
10.0061970754434));
#34095=CARTESIAN_POINT('Ctrl Pts',(-3.39043018200663,-0.636309800095201,
9.97259895733519));
#34096=CARTESIAN_POINT('Ctrl Pts',(-3.32428145980048,-0.319434907277161,
9.93882474384284));
#34097=CARTESIAN_POINT('Ctrl Pts',(-3.30202986962655,-0.158333333333333,
9.92911371588886));
#34098=CARTESIAN_POINT('Ctrl Pts',(-3.28753271539489,0.158333333333336,
9.94629507157737));
#34099=CARTESIAN_POINT('Ctrl Pts',(-3.29613726709655,0.31943490727717,9.97221235514739));
#34100=CARTESIAN_POINT('Ctrl Pts',(-3.33102470537107,0.636309800095211,
10.0429699617166));
#34101=CARTESIAN_POINT('Ctrl Pts',(-3.36144877189567,0.794772684000847,
10.0970951480506));
#34102=CARTESIAN_POINT('Ctrl Pts',(-3.43280627831961,1.0684760419453,10.1949767111377));
#34103=CARTESIAN_POINT('Ctrl Pts',(-3.47005463965042,1.18514270861214,10.2414003155185));
#34104=CARTESIAN_POINT('Ctrl Pts',(-3.51366334183729,1.30000000000053,10.291878222489));
#34105=CARTESIAN_POINT('Ctrl Pts',(-3.67397691592538,-1.30000000000014,
10.1404382070295));
#34106=CARTESIAN_POINT('Ctrl Pts',(-3.62202609023204,-1.18514270861188,
10.1075758257365));
#34107=CARTESIAN_POINT('Ctrl Pts',(-3.5750265102802,-1.06847604194518,10.0784238599931));
#34108=CARTESIAN_POINT('Ctrl Pts',(-3.47788644651384,-0.794772684000867,
10.0196487894806));
#34109=CARTESIAN_POINT('Ctrl Pts',(-3.42747667068375,-0.63630980009521,
9.98822773199515));
#34110=CARTESIAN_POINT('Ctrl Pts',(-3.36014651860966,-0.319434907277166,
9.95652681394419));
#34111=CARTESIAN_POINT('Ctrl Pts',(-3.33602530341171,-0.158333333333335,
9.94652219551044));
#34112=CARTESIAN_POINT('Ctrl Pts',(-3.32078017859728,0.158333333333338,
9.96469262459665));
#34113=CARTESIAN_POINT('Ctrl Pts',(-3.33018258285647,0.319434907277173,
9.99224309046664));
#34114=CARTESIAN_POINT('Ctrl Pts',(-3.3653874499001,0.636309800095219,10.0622280921016));
#34115=CARTESIAN_POINT('Ctrl Pts',(-3.3983426815493,0.794772684000859,10.1144671820177));
#34116=CARTESIAN_POINT('Ctrl Pts',(-3.46559427745884,1.06847604194531,10.208815312985));
#34117=CARTESIAN_POINT('Ctrl Pts',(-3.4996381254075,1.18514270861215,10.2533737903643));
#34118=CARTESIAN_POINT('Ctrl Pts',(-3.53861509735278,1.30000000000055,10.3016509351699));
#34119=CARTESIAN_POINT('Ctrl Pts',(-3.70101609997424,-1.30000000000014,
10.1467971727461));
#34120=CARTESIAN_POINT('Ctrl Pts',(-3.65404756630734,-1.18514270861189,
10.1157658379245));
#34121=CARTESIAN_POINT('Ctrl Pts',(-3.61053545627869,-1.06847604194518,
10.0882065343632));
#34122=CARTESIAN_POINT('Ctrl Pts',(-3.51799880760425,-0.794772684000871,
10.0325601167053));
#34123=CARTESIAN_POINT('Ctrl Pts',(-3.46577617204281,-0.636309800095214,
10.0022958257452));
#34124=CARTESIAN_POINT('Ctrl Pts',(-3.39714216002861,-0.319434907277169,
9.97288211177708));
#34125=CARTESIAN_POINT('Ctrl Pts',(-3.36997360449769,-0.158333333333336,
9.96426715395719));
#34126=CARTESIAN_POINT('Ctrl Pts',(-3.35430928158604,0.158333333333338,
9.98302909004582));
#34127=CARTESIAN_POINT('Ctrl Pts',(-3.36619456824415,0.319434907277173,
10.0099446275918));
#34128=CARTESIAN_POINT('Ctrl Pts',(-3.40214530271569,0.636309800095221,
10.0785148041599));
#34129=CARTESIAN_POINT('Ctrl Pts',(-3.43676382154103,0.794772684000866,
10.1299492333641));
#34130=CARTESIAN_POINT('Ctrl Pts',(-3.49950020459075,1.06847604194532,10.2211856027531));
#34131=CARTESIAN_POINT('Ctrl Pts',(-3.53019839035192,1.18514270861216,10.2640078435357));
#34132=CARTESIAN_POINT('Ctrl Pts',(-3.56443850626412,1.30000000000055,10.3101594814332));
#34133=CARTESIAN_POINT('Ctrl Pts',(-3.71878759513281,-1.30000000000015,
10.1514335393157));
#34134=CARTESIAN_POINT('Ctrl Pts',(-3.67489198161409,-1.18514270861189,
10.1220295507434));
#34135=CARTESIAN_POINT('Ctrl Pts',(-3.63358998434732,-1.06847604194518,
10.0957168890385));
#34136=CARTESIAN_POINT('Ctrl Pts',(-3.54416588061798,-0.794772684000874,
10.0420709601515));
#34137=CARTESIAN_POINT('Ctrl Pts',(-3.49117463237641,-0.636309800095215,
10.0117948092667));
#34138=CARTESIAN_POINT('Ctrl Pts',(-3.42225724530448,-0.319434907277169,
9.98301045242503));
#34139=CARTESIAN_POINT('Ctrl Pts',(-3.3937754601307,-0.158333333333337,
9.97433581792676));
#34140=CARTESIAN_POINT('Ctrl Pts',(-3.37779065274495,0.158333333333339,
9.99355658156853));
#34141=CARTESIAN_POINT('Ctrl Pts',(-3.3905367988662,0.319434907277174,10.0211696006522));
#34142=CARTESIAN_POINT('Ctrl Pts',(-3.42638674628363,0.636309800095223,
10.0896804548971));
#34143=CARTESIAN_POINT('Ctrl Pts',(-3.46182891275466,0.794772684000866,
10.1410408923148));
#34144=CARTESIAN_POINT('Ctrl Pts',(-3.52141617533198,1.06847604194532,10.23043352704));
#34145=CARTESIAN_POINT('Ctrl Pts',(-3.54990764801574,1.18514270861216,10.2720718272872));
#34146=CARTESIAN_POINT('Ctrl Pts',(-3.58109747533919,1.30000000000056,10.3166536685326));
#34147=CARTESIAN_POINT('Ctrl Pts',(-3.73401038434222,-1.30000000000015,
10.1545818971217));
#34148=CARTESIAN_POINT('Ctrl Pts',(-3.69324257501991,-1.18514270861189,
10.1255598410473));
#34149=CARTESIAN_POINT('Ctrl Pts',(-3.65411138747389,-1.06847604194518,
10.0997261594864));
#34150=CARTESIAN_POINT('Ctrl Pts',(-3.56749143978366,-0.794772684000874,
10.0474109700294));
#34151=CARTESIAN_POINT('Ctrl Pts',(-3.51312199982019,-0.636309800095216,
10.0184536727513));
#34152=CARTESIAN_POINT('Ctrl Pts',(-3.44347872018291,-0.319434907277169,
9.99102543581514));
#34153=CARTESIAN_POINT('Ctrl Pts',(-3.41355347653865,-0.158333333333337,
9.98280749464256));
#34154=CARTESIAN_POINT('Ctrl Pts',(-3.39726080503651,0.158333333333339,
10.0024891622436));
#34155=CARTESIAN_POINT('Ctrl Pts',(-3.41104041731569,0.319434907277174,
10.0302188284627));
#34156=CARTESIAN_POINT('Ctrl Pts',(-3.44719718804243,0.636309800095223,
10.0980833659227));
#34157=CARTESIAN_POINT('Ctrl Pts',(-3.48378843925299,0.794772684000865,
10.1486515677517));
#34158=CARTESIAN_POINT('Ctrl Pts',(-3.54080406639039,1.06847604194532,10.2364196566261));
#34159=CARTESIAN_POINT('Ctrl Pts',(-3.56736250509839,1.18514270861217,10.2772146646551));
#34160=CARTESIAN_POINT('Ctrl Pts',(-3.5957994301638,1.30000000000056,10.3208131271675));
#34161=CARTESIAN_POINT('Ctrl Pts',(-3.74458338262462,-1.30000000000015,
10.1569162443583));
#34162=CARTESIAN_POINT('Ctrl Pts',(-3.70576961061605,-1.18514270861189,
10.1285656394162));
#34163=CARTESIAN_POINT('Ctrl Pts',(-3.6680144134445,-1.06847604194519,10.1033120089907));
#34164=CARTESIAN_POINT('Ctrl Pts',(-3.58323787471761,-0.794772684000877,
10.0521257014175));
#34165=CARTESIAN_POINT('Ctrl Pts',(-3.52812698520538,-0.636309800095216,
10.0236832244191));
#34166=CARTESIAN_POINT('Ctrl Pts',(-3.45819987631133,-0.319434907277169,
9.99683436947552));
#34167=CARTESIAN_POINT('Ctrl Pts',(-3.42748734455854,-0.158333333333337,
9.98859811477711));
#34168=CARTESIAN_POINT('Ctrl Pts',(-3.4111088685937,0.158333333333339,10.0084029104395));
#34169=CARTESIAN_POINT('Ctrl Pts',(-3.42563400563729,0.319434907277174,
10.0361870918687));
#34170=CARTESIAN_POINT('Ctrl Pts',(-3.46181011952091,0.636309800095224,
10.1039001131025));
#34171=CARTESIAN_POINT('Ctrl Pts',(-3.49871339236154,0.794772684000867,
10.1546653062899));
#34172=CARTESIAN_POINT('Ctrl Pts',(-3.55391749921246,1.06847604194532,10.2413119292474));
#34173=CARTESIAN_POINT('Ctrl Pts',(-3.57923030510806,1.18514270861217,10.2813512158437));
#34174=CARTESIAN_POINT('Ctrl Pts',(-3.60596010455725,1.30000000000056,10.3239236765318));
#34175=CARTESIAN_POINT('Ctrl Pts',(-3.75070071224822,-1.30000000000015,
10.158117784076));
#34176=CARTESIAN_POINT('Ctrl Pts',(-3.71293555971019,-1.18514270861189,
10.1302712463608));
#34177=CARTESIAN_POINT('Ctrl Pts',(-3.67592652198007,-1.06847604194519,
10.1054206976937));
#34178=CARTESIAN_POINT('Ctrl Pts',(-3.59217501765742,-0.794772684000877,
10.0549322929838));
#34179=CARTESIAN_POINT('Ctrl Pts',(-3.53672118512614,-0.636309800095217,
10.0266422905552));
#34180=CARTESIAN_POINT('Ctrl Pts',(-3.46669189355701,-0.319434907277169,
10.0000273475389));
#34181=CARTESIAN_POINT('Ctrl Pts',(-3.43560761307563,-0.158333333333337,
9.99166315756603));
#34182=CARTESIAN_POINT('Ctrl Pts',(-3.41913503061073,0.158333333333339,
10.0116063008335));
#34183=CARTESIAN_POINT('Ctrl Pts',(-3.43393288855804,0.319434907277175,
10.0396543473314));
#34184=CARTESIAN_POINT('Ctrl Pts',(-3.47002952133634,0.636309800095224,
10.1074201856546));
#34185=CARTESIAN_POINT('Ctrl Pts',(-3.50714515538911,0.794772684000867,
10.1582504041928));
#34186=CARTESIAN_POINT('Ctrl Pts',(-3.56125634144506,1.06847604194532,10.2443441091965));
#34187=CARTESIAN_POINT('Ctrl Pts',(-3.5858219639986,1.18514270861217,10.2840044287812));
#34188=CARTESIAN_POINT('Ctrl Pts',(-3.61153048167909,1.30000000000056,10.3260582931406));
#34189=CARTESIAN_POINT('Ctrl Pts',(-3.76607211082024,-1.30000000000015,
10.1609742455453));
#34190=CARTESIAN_POINT('Ctrl Pts',(-3.73099751271949,-1.18514270861189,
10.1342611827223));
#34191=CARTESIAN_POINT('Ctrl Pts',(-3.69590262596997,-1.06847604194519,
10.1103306661676));
#34192=CARTESIAN_POINT('Ctrl Pts',(-3.61477954603314,-0.794772684000878,
10.0614746241691));
#34193=CARTESIAN_POINT('Ctrl Pts',(-3.55846721318748,-0.636309800095217,
10.0335856640069));
#34194=CARTESIAN_POINT('Ctrl Pts',(-3.48812651758648,-0.319434907277169,
10.0076608129102));
#34195=CARTESIAN_POINT('Ctrl Pts',(-3.45597529768671,-0.158333333333337,
9.99920817797782));
#34196=CARTESIAN_POINT('Ctrl Pts',(-3.43925943579227,0.158333333333339,
10.0195222842871));
#34197=CARTESIAN_POINT('Ctrl Pts',(-3.45479591099045,0.319434907277175,
10.0481423271903));
#34198=CARTESIAN_POINT('Ctrl Pts',(-3.49088163105331,0.636309800095224,
10.1157443641273));
#34199=CARTESIAN_POINT('Ctrl Pts',(-3.52886328959088,0.794772684000867,
10.1661993892385));
#34200=CARTESIAN_POINT('Ctrl Pts',(-3.58023784918361,1.06847604194532,10.250919595152));
#34201=CARTESIAN_POINT('Ctrl Pts',(-3.60284905222399,1.18514270861217,10.2897719074366));
#34202=CARTESIAN_POINT('Ctrl Pts',(-3.62583331507207,1.30000000000056,10.3308042940587));
#34203=CARTESIAN_POINT('Ctrl Pts',(-3.7915912137151,-1.30000000000016,10.166868855423));
#34204=CARTESIAN_POINT('Ctrl Pts',(-3.76166361794079,-1.1851427086119,10.1410540242383));
#34205=CARTESIAN_POINT('Ctrl Pts',(-3.73019934521846,-1.0684760419452,10.1180149543402));
#34206=CARTESIAN_POINT('Ctrl Pts',(-3.65396054966258,-0.794772684000883,
10.0712026577869));
#34207=CARTESIAN_POINT('Ctrl Pts',(-3.59579091152071,-0.636309800095222,
10.0447592722612));
#34208=CARTESIAN_POINT('Ctrl Pts',(-3.52464131310718,-0.319434907277172,
10.0204798922187));
#34209=CARTESIAN_POINT('Ctrl Pts',(-3.49014293988893,-0.158333333333338,
10.0126931881361));
#34210=CARTESIAN_POINT('Ctrl Pts',(-3.47330320399168,0.15833333333334,10.0331780310056));
#34211=CARTESIAN_POINT('Ctrl Pts',(-3.49118822947503,0.319434907277177,
10.0610441144754));
#34212=CARTESIAN_POINT('Ctrl Pts',(-3.52757536198082,0.636309800095229,
10.1278755444044));
#34213=CARTESIAN_POINT('Ctrl Pts',(-3.56642191385663,0.794772684000873,
10.1786655205029));
#34214=CARTESIAN_POINT('Ctrl Pts',(-3.61303850726719,1.06847604194533,10.2612448037204));
#34215=CARTESIAN_POINT('Ctrl Pts',(-3.63234446820997,1.18514270861218,10.2987099793951));
#34216=CARTESIAN_POINT('Ctrl Pts',(-3.6507777941231,1.30000000000058,10.3378948189035));
#34217=CARTESIAN_POINT('Ctrl Pts',(-3.82904434197742,-1.30000000000017,
10.1725573801911));
#34218=CARTESIAN_POINT('Ctrl Pts',(-3.80603578149659,-1.18514270861191,
10.1485789281661));
#34219=CARTESIAN_POINT('Ctrl Pts',(-3.7794981298758,-1.0684760419452,10.1271271007892));
#34220=CARTESIAN_POINT('Ctrl Pts',(-3.71003793926713,-0.794772684000884,
10.0834060965121));
#34221=CARTESIAN_POINT('Ctrl Pts',(-3.64975703515377,-0.636309800095225,
10.0581463894763));
#34222=CARTESIAN_POINT('Ctrl Pts',(-3.57770260659287,-0.319434907277174,
10.0359093284447));
#34223=CARTESIAN_POINT('Ctrl Pts',(-3.54024857503223,-0.158333333333339,
10.02866262349));
#34224=CARTESIAN_POINT('Ctrl Pts',(-3.52260595669352,0.158333333333341,
10.0504829942974));
#34225=CARTESIAN_POINT('Ctrl Pts',(-3.54225771277102,0.319434907277179,
10.0797339881208));
#34226=CARTESIAN_POINT('Ctrl Pts',(-3.57870060819418,0.636309800095233,
10.1460429455198));
#34227=CARTESIAN_POINT('Ctrl Pts',(-3.62006023327149,0.794772684000877,
10.195179164837));
#34228=CARTESIAN_POINT('Ctrl Pts',(-3.65986116385648,1.06847604194534,10.2748722818108));
#34229=CARTESIAN_POINT('Ctrl Pts',(-3.67422220811065,1.18514270861218,10.3108252288688));
#34230=CARTESIAN_POINT('Ctrl Pts',(-3.68571594853856,1.30000000000058,10.3482349255678));
#34231=CARTESIAN_POINT('Ctrl Pts',(-3.85796273426452,-1.30000000000018,
10.178266574707));
#34232=CARTESIAN_POINT('Ctrl Pts',(-3.84081716435615,-1.18514270861192,
10.1550010588959));
#34233=CARTESIAN_POINT('Ctrl Pts',(-3.81847119538827,-1.06847604194521,
10.134256092061));
#34234=CARTESIAN_POINT('Ctrl Pts',(-3.75483357461295,-0.794772684000895,
10.0921540410251));
#34235=CARTESIAN_POINT('Ctrl Pts',(-3.69289320873997,-0.636309800095232,
10.0678948309938));
#34236=CARTESIAN_POINT('Ctrl Pts',(-3.62016465998514,-0.319434907277177,
10.0472382191901));
#34237=CARTESIAN_POINT('Ctrl Pts',(-3.57998281606451,-0.158333333333341,
10.0410808411431));
#34238=CARTESIAN_POINT('Ctrl Pts',(-3.56213974746018,0.158333333333343,
10.0632503369065));
#34239=CARTESIAN_POINT('Ctrl Pts',(-3.58443579868164,0.319434907277182,
10.0915216009712));
#34240=CARTESIAN_POINT('Ctrl Pts',(-3.62090632733795,0.636309800095239,
10.1574491524359));
#34241=CARTESIAN_POINT('Ctrl Pts',(-3.66277298302753,0.794772684000885,
10.2077161021715));
#34242=CARTESIAN_POINT('Ctrl Pts',(-3.69695770961202,1.06847604194535,10.2855472711458));
#34243=CARTESIAN_POINT('Ctrl Pts',(-3.70754953577959,1.1851427086122,10.3201022877664));
#34244=CARTESIAN_POINT('Ctrl Pts',(-3.71393588664526,1.3000000000006,10.3555220918877));
#34245=CARTESIAN_POINT('Ctrl Pts',(-3.88331383738313,-1.30000000000019,
10.1812451374793));
#34246=CARTESIAN_POINT('Ctrl Pts',(-3.87071504559958,-1.18514270861193,
10.1592808151736));
#34247=CARTESIAN_POINT('Ctrl Pts',(-3.85164934528007,-1.06847604194522,
10.1395770461112));
#34248=CARTESIAN_POINT('Ctrl Pts',(-3.792663911043,-0.794772684000897,10.0992797280657));
#34249=CARTESIAN_POINT('Ctrl Pts',(-3.72966428221427,-0.636309800095233,
10.0752174409862));
#34250=CARTESIAN_POINT('Ctrl Pts',(-3.65656987687846,-0.319434907277177,
10.055565012233));
#34251=CARTESIAN_POINT('Ctrl Pts',(-3.6145153650832,-0.158333333333341,
10.0496759387229));
#34252=CARTESIAN_POINT('Ctrl Pts',(-3.59606894268156,0.158333333333343,
10.0729123621764));
#34253=CARTESIAN_POINT('Ctrl Pts',(-3.61922110816113,0.319434907277183,
10.1026755664624));
#34254=CARTESIAN_POINT('Ctrl Pts',(-3.65567016343661,0.636309800095241,
10.1683599528127));
#34255=CARTESIAN_POINT('Ctrl Pts',(-3.69948766699002,0.794772684000886,
10.2169949438957));
#34256=CARTESIAN_POINT('Ctrl Pts',(-3.72910291164311,1.06847604194535,10.2929745585285));
#34257=CARTESIAN_POINT('Ctrl Pts',(-3.73633364482524,1.1851427086122,10.3266612256361));
#34258=CARTESIAN_POINT('Ctrl Pts',(-3.73797576913212,1.3000000000006,10.3611457999992));
#34259=CARTESIAN_POINT('Ctrl Pts',(-3.90174032585728,-1.3000000000002,10.1844798363048));
#34260=CARTESIAN_POINT('Ctrl Pts',(-3.89300705345891,-1.18514270861193,
10.1626302526796));
#34261=CARTESIAN_POINT('Ctrl Pts',(-3.87667429073231,-1.06847604194522,
10.1431943317848));
#34262=CARTESIAN_POINT('Ctrl Pts',(-3.82138599854488,-0.794772684000903,
10.1038695101342));
#34263=CARTESIAN_POINT('Ctrl Pts',(-3.75686382275297,-0.636309800095237,
10.0813423020077));
#34264=CARTESIAN_POINT('Ctrl Pts',(-3.6835405027242,-0.319434907277179,
10.0623901632465));
#34265=CARTESIAN_POINT('Ctrl Pts',(-3.64041659361247,-0.158333333333342,
10.0560697623108));
#34266=CARTESIAN_POINT('Ctrl Pts',(-3.62215778243213,0.158333333333344,
10.0789889568926));
#34267=CARTESIAN_POINT('Ctrl Pts',(-3.64693561561035,0.319434907277186,
10.1081907696719));
#34268=CARTESIAN_POINT('Ctrl Pts',(-3.68324480396177,0.636309800095246,
10.1739046182766));
#34269=CARTESIAN_POINT('Ctrl Pts',(-3.72711751271952,0.794772684000892,
10.2237230640728));
#34270=CARTESIAN_POINT('Ctrl Pts',(-3.75286406183021,1.06847604194536,10.299088735948));
#34271=CARTESIAN_POINT('Ctrl Pts',(-3.7575711949502,1.1851427086122,10.3321417122785));
#34272=CARTESIAN_POINT('Ctrl Pts',(-3.75584073408384,1.3000000000006,10.3656246581581));
#34273=CARTESIAN_POINT('Ctrl Pts',(-3.92200665684785,-1.3000000000002,10.187442466889));
#34274=CARTESIAN_POINT('Ctrl Pts',(-3.91700851637555,-1.18514270861194,
10.1665604654));
#34275=CARTESIAN_POINT('Ctrl Pts',(-3.9034222469725,-1.06847604194523,10.1478092117938));
#34276=CARTESIAN_POINT('Ctrl Pts',(-3.8521949508482,-0.794772684000906,
10.1094125186521));
#34277=CARTESIAN_POINT('Ctrl Pts',(-3.78730781975507,-0.636309800095239,
10.0861175764946));
#34278=CARTESIAN_POINT('Ctrl Pts',(-3.71374852816862,-0.31943490727718,
10.0678795136089));
#34279=CARTESIAN_POINT('Ctrl Pts',(-3.6686668503439,-0.158333333333343,
10.0626129675919));
#34280=CARTESIAN_POINT('Ctrl Pts',(-3.64980811405989,0.158333333333344,
10.0866279809606));
#34281=CARTESIAN_POINT('Ctrl Pts',(-3.67550669183711,0.319434907277187,
10.1166464057035));
#34282=CARTESIAN_POINT('Ctrl Pts',(-3.71172018671788,0.636309800095247,
10.1823003800064));
#34283=CARTESIAN_POINT('Ctrl Pts',(-3.75686878802455,0.794772684000892,
10.2313091805914));
#34284=CARTESIAN_POINT('Ctrl Pts',(-3.77883878245198,1.06847604194536,10.3052965512782));
#34285=CARTESIAN_POINT('Ctrl Pts',(-3.78084109508027,1.18514270861221,10.3376124724536));
#34286=CARTESIAN_POINT('Ctrl Pts',(-3.77533572381774,1.30000000000061,10.3702179235365));
#34287=CARTESIAN_POINT('Ctrl Pts',(-3.93787421728648,-1.30000000000021,
10.1891442942232));
#34288=CARTESIAN_POINT('Ctrl Pts',(-3.93601570989885,-1.18514270861194,
10.168468189729));
#34289=CARTESIAN_POINT('Ctrl Pts',(-3.92466395193018,-1.06847604194523,
10.1499934640814));
#34290=CARTESIAN_POINT('Ctrl Pts',(-3.87650781215066,-0.794772684000909,
10.1123987774988));
#34291=CARTESIAN_POINT('Ctrl Pts',(-3.81060836194368,-0.636309800095243,
10.0899431628784));
#34292=CARTESIAN_POINT('Ctrl Pts',(-3.73672414330885,-0.319434907277183,
10.0725578565363));
#34293=CARTESIAN_POINT('Ctrl Pts',(-3.69036900847232,-0.158333333333344,
10.0676607019504));
#34294=CARTESIAN_POINT('Ctrl Pts',(-3.67144693011197,0.158333333333346,
10.0918192063));
#34295=CARTESIAN_POINT('Ctrl Pts',(-3.69840825330412,0.31943490727719,10.1215004566747));
#34296=CARTESIAN_POINT('Ctrl Pts',(-3.73471044748741,0.636309800095253,
10.1868206121894));
#34297=CARTESIAN_POINT('Ctrl Pts',(-3.78053057570353,0.794772684000899,
10.2357323241856));
#34298=CARTESIAN_POINT('Ctrl Pts',(-3.79930689286134,1.06847604194537,10.3091734262881));
#34299=CARTESIAN_POINT('Ctrl Pts',(-3.79908419968581,1.18514270861222,10.3411844214108));
#34300=CARTESIAN_POINT('Ctrl Pts',(-3.79051124136824,1.30000000000062,10.373416479817));
#34301=CARTESIAN_POINT('Ctrl Pts',(-3.95042528865478,-1.30000000000021,
10.1907726542255));
#34302=CARTESIAN_POINT('Ctrl Pts',(-3.95098551996914,-1.18514270861195,
10.1704463443776));
#34303=CARTESIAN_POINT('Ctrl Pts',(-3.94138516874209,-1.06847604194524,
10.1522652425601));
#34304=CARTESIAN_POINT('Ctrl Pts',(-3.8957334585757,-0.794772684000912,
10.1152191199419));
#34305=CARTESIAN_POINT('Ctrl Pts',(-3.82935596711379,-0.636309800095244,
10.0927819243377));
#34306=CARTESIAN_POINT('Ctrl Pts',(-3.75524010088347,-0.319434907277182,
10.0760144773478));
#34307=CARTESIAN_POINT('Ctrl Pts',(-3.70764638659068,-0.158333333333344,
10.0718387952671));
#34308=CARTESIAN_POINT('Ctrl Pts',(-3.68855509195389,0.158333333333346,
10.0963248232461));
#34309=CARTESIAN_POINT('Ctrl Pts',(-3.71647280399642,0.31943490727719,10.1258106403559));
#34310=CARTESIAN_POINT('Ctrl Pts',(-3.75289208497874,0.636309800095253,
10.190775716563));
#34311=CARTESIAN_POINT('Ctrl Pts',(-3.79943225862935,0.794772684000899,
10.2392902622796));
#34312=CARTESIAN_POINT('Ctrl Pts',(-3.81571432852043,1.06847604194537,10.3121932875574));
#34313=CARTESIAN_POINT('Ctrl Pts',(-3.8137112109172,1.18514270861222,10.3439650773515));
#34314=CARTESIAN_POINT('Ctrl Pts',(-3.80265707096503,1.30000000000062,10.3759516386202));
#34315=CARTESIAN_POINT('Ctrl Pts',(-3.95998493006225,-1.30000000000021,
10.1916909496914));
#34316=CARTESIAN_POINT('Ctrl Pts',(-3.96246157838396,-1.18514270861195,
10.1714087627593));
#34317=CARTESIAN_POINT('Ctrl Pts',(-3.95421929895579,-1.06847604194524,
10.1533510482225));
#34318=CARTESIAN_POINT('Ctrl Pts',(-3.91041511719802,-0.794772684000914,
10.1167730914459));
#34319=CARTESIAN_POINT('Ctrl Pts',(-3.84334389128597,-0.636309800095247,
10.0950320918671));
#34320=CARTESIAN_POINT('Ctrl Pts',(-3.76905895310044,-0.319434907277184,
10.0787420572256));
#34321=CARTESIAN_POINT('Ctrl Pts',(-3.7208679411399,-0.158333333333345,
10.0744802704328));
#34322=CARTESIAN_POINT('Ctrl Pts',(-3.70166044317268,0.158333333333347,
10.0991912863336));
#34323=CARTESIAN_POINT('Ctrl Pts',(-3.73008710276877,0.319434907277192,
10.1289200681933));
#34324=CARTESIAN_POINT('Ctrl Pts',(-3.7663820228931,0.636309800095256,10.1940047878435));
#34325=CARTESIAN_POINT('Ctrl Pts',(-3.81322425648508,0.794772684000904,
10.242642154839));
#34326=CARTESIAN_POINT('Ctrl Pts',(-3.82766422345967,1.06847604194537,10.3150922134062));
#34327=CARTESIAN_POINT('Ctrl Pts',(-3.824411638536,1.18514270861223,10.3465324873549));
#34328=CARTESIAN_POINT('Ctrl Pts',(-3.81165594203887,1.30000000000063,10.3780520894376));
#34329=CARTESIAN_POINT('Ctrl Pts',(-3.96796056930311,-1.30000000000022,
10.192428239807));
#34330=CARTESIAN_POINT('Ctrl Pts',(-3.97206870982618,-1.18514270861195,
10.1721128975678));
#34331=CARTESIAN_POINT('Ctrl Pts',(-3.96497989930268,-1.06847604194524,
10.1541138410264));
#34332=CARTESIAN_POINT('Ctrl Pts',(-3.92273613202175,-0.794772684000917,
10.1178835030499));
#34333=CARTESIAN_POINT('Ctrl Pts',(-3.85504424735611,-0.636309800095248,
10.0968054295953));
#34334=CARTESIAN_POINT('Ctrl Pts',(-3.78061951838933,-0.319434907277185,
10.0809165143215));
#34335=CARTESIAN_POINT('Ctrl Pts',(-3.7319573146038,-0.158333333333345,
10.0765407935441));
#34336=CARTESIAN_POINT('Ctrl Pts',(-3.71266131128897,0.158333333333347,
10.1014272047489));
#34337=CARTESIAN_POINT('Ctrl Pts',(-3.74150943516619,0.319434907277192,
10.1313609681455));
#34338=CARTESIAN_POINT('Ctrl Pts',(-3.77768487945715,0.636309800095257,
10.1965736463306));
#34339=CARTESIAN_POINT('Ctrl Pts',(-3.82475685902025,0.794772684000905,
10.2453518195525));
#34340=CARTESIAN_POINT('Ctrl Pts',(-3.83763969446987,1.06847604194538,10.3174666274569));
#34341=CARTESIAN_POINT('Ctrl Pts',(-3.83333732055447,1.18514270861223,10.348647953515));
#34342=CARTESIAN_POINT('Ctrl Pts',(-3.81915607061362,1.30000000000063,10.3797947774065));
#34343=CARTESIAN_POINT('Ctrl Pts',(-3.97349722602794,-1.30000000000022,
10.1930368892965));
#34344=CARTESIAN_POINT('Ctrl Pts',(-3.97869435191075,-1.18514270861196,
10.1728056047134));
#34345=CARTESIAN_POINT('Ctrl Pts',(-3.97239076473802,-1.06847604194524,
10.15489249281));
#34346=CARTESIAN_POINT('Ctrl Pts',(-3.93125926947268,-0.794772684000917,
10.1188650634462));
#34347=CARTESIAN_POINT('Ctrl Pts',(-3.86330482897738,-0.636309800095249,
10.0979046517948));
#34348=CARTESIAN_POINT('Ctrl Pts',(-3.78880121328532,-0.319434907277185,
10.0822558040718));
#34349=CARTESIAN_POINT('Ctrl Pts',(-3.73967479280392,-0.158333333333345,
10.0780642463435));
#34350=CARTESIAN_POINT('Ctrl Pts',(-3.72031792819803,0.158333333333347,
10.103075489714));
#34351=CARTESIAN_POINT('Ctrl Pts',(-3.74954897211557,0.319434907277193,
10.1329852943817));
#34352=CARTESIAN_POINT('Ctrl Pts',(-3.78572095843012,0.636309800095258,
10.1981401286174));
#34353=CARTESIAN_POINT('Ctrl Pts',(-3.83304673731638,0.794772684000906,
10.2468510356027));
#34354=CARTESIAN_POINT('Ctrl Pts',(-3.8448011432344,1.06847604194538,10.3188000213527));
#34355=CARTESIAN_POINT('Ctrl Pts',(-3.83971283334336,1.18514270861223,10.349891825942));
#34356=CARTESIAN_POINT('Ctrl Pts',(-3.82444816678303,1.30000000000063,10.3809313851622));
#34357=CARTESIAN_POINT('Ctrl Pts',(-3.97625624878831,-1.30000000000022,
10.1933594053906));
#34358=CARTESIAN_POINT('Ctrl Pts',(-3.98198868097057,-1.18514270861196,
10.1731886222752));
#34359=CARTESIAN_POINT('Ctrl Pts',(-3.97607415657479,-1.06847604194524,
10.1553255933479));
#34360=CARTESIAN_POINT('Ctrl Pts',(-3.93550362236307,-0.794772684000918,
10.1193897968784));
#34361=CARTESIAN_POINT('Ctrl Pts',(-3.86744965977133,-0.636309800095249,
10.0984242956282));
#34362=CARTESIAN_POINT('Ctrl Pts',(-3.79291200164116,-0.319434907277185,
10.0828842209601));
#34363=CARTESIAN_POINT('Ctrl Pts',(-3.74353202195387,-0.158333333333345,
10.0788268713356));
#34364=CARTESIAN_POINT('Ctrl Pts',(-3.72414430417208,0.158333333333347,
10.1039020972553));
#34365=CARTESIAN_POINT('Ctrl Pts',(-3.7535777313355,0.319434907277192,10.1337792027508));
#34366=CARTESIAN_POINT('Ctrl Pts',(-3.78976231043831,0.636309800095258,
10.1988791532386));
#34367=CARTESIAN_POINT('Ctrl Pts',(-3.83723623512286,0.794772684000907,
10.2475182334964));
#34368=CARTESIAN_POINT('Ctrl Pts',(-3.84842102626566,1.06847604194538,10.3193945152741));
#34369=CARTESIAN_POINT('Ctrl Pts',(-3.8429306802829,1.18514270861223,10.3504582082888));
#34370=CARTESIAN_POINT('Ctrl Pts',(-3.82710850666902,1.30000000000063,10.3814730152152));
#34371=CARTESIAN_POINT('Ctrl Pts',(-3.97783126988176,-1.30000000000022,
10.1935466720133));
#34372=CARTESIAN_POINT('Ctrl Pts',(-3.98386793609951,-1.18514270861196,
10.1734137657586));
#34373=CARTESIAN_POINT('Ctrl Pts',(-3.97817508118458,-1.06847604194524,
10.1555806625564));
#34374=CARTESIAN_POINT('Ctrl Pts',(-3.93792590718021,-0.794772684000918,
10.119695631785));
#34375=CARTESIAN_POINT('Ctrl Pts',(-3.8698211572568,-0.636309800095249,
10.0987151648293));
#34376=CARTESIAN_POINT('Ctrl Pts',(-3.79526405358766,-0.319434907277185,
10.083237165949));
#34377=CARTESIAN_POINT('Ctrl Pts',(-3.74573299628995,-0.158333333333345,
10.0792685590858));
#34378=CARTESIAN_POINT('Ctrl Pts',(-3.72632788005725,0.158333333333347,
10.1043800434176));
#34379=CARTESIAN_POINT('Ctrl Pts',(-3.75588220968736,0.319434907277192,
10.1342284153063));
#34380=CARTESIAN_POINT('Ctrl Pts',(-3.79207682014073,0.636309800095258,
10.1992917672285));
#34381=CARTESIAN_POINT('Ctrl Pts',(-3.83963639922207,0.794772684000907,
10.2478883083645));
#34382=CARTESIAN_POINT('Ctrl Pts',(-3.85049411959542,1.06847604194538,10.3197258711542));
#34383=CARTESIAN_POINT('Ctrl Pts',(-3.84477253459402,1.18514270861223,10.3507761541805));
#34384=CARTESIAN_POINT('Ctrl Pts',(-3.82862945975979,1.30000000000063,10.3817809011455));
#34385=CARTESIAN_POINT('Ctrl Pts',(-3.99120834453964,-1.30000000000021,
10.1951589192355));
#34386=CARTESIAN_POINT('Ctrl Pts',(-3.99981622143662,-1.18514270861195,
10.1753762694606));
#34387=CARTESIAN_POINT('Ctrl Pts',(-3.99600223628861,-1.06847604194524,
10.1578071058687));
#34388=CARTESIAN_POINT('Ctrl Pts',(-3.95849418130268,-0.794772684000911,
10.1223324191615));
#34389=CARTESIAN_POINT('Ctrl Pts',(-3.88999698655893,-0.636309800095245,
10.1011441035307));
#34390=CARTESIAN_POINT('Ctrl Pts',(-3.81531447193312,-0.319434907277184,
10.0861154983723));
#34391=CARTESIAN_POINT('Ctrl Pts',(-3.76453674642973,-0.158333333333344,
10.0828314136448));
#34392=CARTESIAN_POINT('Ctrl Pts',(-3.74497949862722,0.158333333333346,
10.108261146524));
#34393=CARTESIAN_POINT('Ctrl Pts',(-3.77549313140824,0.31943490727719,10.1379971254146));
#34394=CARTESIAN_POINT('Ctrl Pts',(-3.81177873263614,0.636309800095254,
10.2027421965092));
#34395=CARTESIAN_POINT('Ctrl Pts',(-3.86014910952305,0.794772684000902,
10.2508212795318));
#34396=CARTESIAN_POINT('Ctrl Pts',(-3.86823541825366,1.06847604194537,10.322318788935));
#34397=CARTESIAN_POINT('Ctrl Pts',(-3.86053734572664,1.18514270861222,10.3532789195567));
#34398=CARTESIAN_POINT('Ctrl Pts',(-3.84164093725037,1.30000000000063,10.3842505582232));
#34399=CARTESIAN_POINT('Ctrl Pts',(-4.01715141436988,-1.30000000000016,
10.1974276921261));
#34400=CARTESIAN_POINT('Ctrl Pts',(-4.03105905169031,-1.18514270861191,
10.1774944457447));
#34401=CARTESIAN_POINT('Ctrl Pts',(-4.03102853929687,-1.0684760419452,10.1600161809904));
#34402=CARTESIAN_POINT('Ctrl Pts',(-3.99875813540771,-0.79477268400089,
10.1253093915692));
#34403=CARTESIAN_POINT('Ctrl Pts',(-3.92860155491193,-0.636309800095222,
10.1056019296984));
#34404=CARTESIAN_POINT('Ctrl Pts',(-3.85350972014637,-0.31943490727717,
10.0918183982673));
#34405=CARTESIAN_POINT('Ctrl Pts',(-3.80085090679698,-0.158333333333339,
10.0888822558709));
#34406=CARTESIAN_POINT('Ctrl Pts',(-3.78103814166869,0.158333333333341,
10.1148544498269));
#34407=CARTESIAN_POINT('Ctrl Pts',(-3.81330939641933,0.319434907277181,
10.1445089974631));
#34408=CARTESIAN_POINT('Ctrl Pts',(-3.8492148680978,0.636309800095232,10.2096760392664));
#34409=CARTESIAN_POINT('Ctrl Pts',(-3.89789606902708,0.79477268400087,10.259034550803));
#34410=CARTESIAN_POINT('Ctrl Pts',(-3.90095428259184,1.06847604194533,10.3294593072443));
#34411=CARTESIAN_POINT('Ctrl Pts',(-3.88994950178544,1.18514270861218,10.3594286553047));
#34412=CARTESIAN_POINT('Ctrl Pts',(-3.86661615283843,1.30000000000058,10.3888830838563));
#34413=CARTESIAN_POINT('Ctrl Pts',(-4.04264117857264,-1.30000000000011,
10.1996888386742));
#34414=CARTESIAN_POINT('Ctrl Pts',(-4.06162921508693,-1.18514270861186,
10.1798435376198));
#34415=CARTESIAN_POINT('Ctrl Pts',(-4.06526201565739,-1.06847604194515,
10.1625501048079));
#34416=CARTESIAN_POINT('Ctrl Pts',(-4.03818084487975,-0.794772684000851,
10.1284941416128));
#34417=CARTESIAN_POINT('Ctrl Pts',(-3.96674475595548,-0.636309800095196,
10.1095386222874));
#34418=CARTESIAN_POINT('Ctrl Pts',(-3.891393048032,-0.319434907277159,10.0967082635573));
#34419=CARTESIAN_POINT('Ctrl Pts',(-3.83684904087863,-0.158333333333332,
10.0942175847262));
#34420=CARTESIAN_POINT('Ctrl Pts',(-3.81670994245091,0.158333333333334,
10.1208905127328));
#34421=CARTESIAN_POINT('Ctrl Pts',(-3.85032449139867,0.319434907277167,
10.1511988953562));
#34422=CARTESIAN_POINT('Ctrl Pts',(-3.88626421184787,0.636309800095206,
10.2160282620725));
#34423=CARTESIAN_POINT('Ctrl Pts',(-3.93674627805647,0.79477268400084,10.2638747589896));
#34424=CARTESIAN_POINT('Ctrl Pts',(-3.93451699612749,1.06847604194529,10.3338269442228));
#34425=CARTESIAN_POINT('Ctrl Pts',(-3.91970579175577,1.18514270861213,10.3638146300663));
#34426=CARTESIAN_POINT('Ctrl Pts',(-3.89104835655634,1.30000000000053,10.3935102927497));
#34427=CARTESIAN_POINT('Ctrl Pts',(-4.05557051525689,-1.30000000000011,
10.2004379798222));
#34428=CARTESIAN_POINT('Ctrl Pts',(-4.07701141444267,-1.18514270861186,
10.1807976562281));
#34429=CARTESIAN_POINT('Ctrl Pts',(-4.08243023812086,-1.06847604194515,
10.1636773708346));
#34430=CARTESIAN_POINT('Ctrl Pts',(-4.05793460522167,-0.794772684000851,
10.1299478790495));
#34431=CARTESIAN_POINT('Ctrl Pts',(-3.98606842200265,-0.636309800095196,
10.1109415465295));
#34432=CARTESIAN_POINT('Ctrl Pts',(-3.91057658300642,-0.319434907277159,
10.0986164293511));
#34433=CARTESIAN_POINT('Ctrl Pts',(-3.85489608531509,-0.158333333333332,
10.0967615839605));
#34434=CARTESIAN_POINT('Ctrl Pts',(-3.83456187378799,0.158333333333334,
10.1238619534744));
#34435=CARTESIAN_POINT('Ctrl Pts',(-3.86905149194718,0.319434907277167,
10.1540957676226));
#34436=CARTESIAN_POINT('Ctrl Pts',(-3.90486897721865,0.636309800095206,
10.2190179716123));
#34437=CARTESIAN_POINT('Ctrl Pts',(-3.95570286248539,0.79477268400084,10.2671282986158));
#34438=CARTESIAN_POINT('Ctrl Pts',(-3.95093219463511,1.06847604194529,10.3366909515195));
#34439=CARTESIAN_POINT('Ctrl Pts',(-3.93440493783799,1.18514270861213,10.3663638202738));
#34440=CARTESIAN_POINT('Ctrl Pts',(-3.90341546958548,1.30000000000053,10.3955984628905));
#34441=CARTESIAN_POINT('',(-3.81817959106573,1.2,10.3502388179897));
#34442=CARTESIAN_POINT('Ctrl Pts',(-3.81817959106573,1.2,10.3502388179897));
#34443=CARTESIAN_POINT('Ctrl Pts',(-3.79661778313311,1.21681395190025,10.3499524248101));
#34444=CARTESIAN_POINT('Ctrl Pts',(-3.7746889739999,1.23316487520676,10.3507417153752));
#34445=CARTESIAN_POINT('Ctrl Pts',(-3.74255521985325,1.25821638180379,10.3500589326249));
#34446=CARTESIAN_POINT('Ctrl Pts',(-3.73195596097856,1.26642443139157,10.3498984954673));
#34447=CARTESIAN_POINT('Ctrl Pts',(-3.71004144468884,1.28334474964523,10.3495995663522));
#34448=CARTESIAN_POINT('Ctrl Pts',(-3.69832282339783,1.29250139325086,10.3492436833369));
#34449=CARTESIAN_POINT('Ctrl Pts',(-3.68879127704346,1.30000000000059,10.3488599388354));
#34450=CARTESIAN_POINT('',(-3.91593537812686,0.653834841369882,10.2278623010254));
#34451=CARTESIAN_POINT('Ctrl Pts',(-3.91593537815288,0.653834841368625,
10.2278623010518));
#34452=CARTESIAN_POINT('Ctrl Pts',(-3.90605735116792,0.717483776812682,
10.2406375568233));
#34453=CARTESIAN_POINT('Ctrl Pts',(-3.89793780545931,0.764248674190916,
10.2510423166789));
#34454=CARTESIAN_POINT('Ctrl Pts',(-3.86587044819959,0.949850976170393,
10.291727520538));
#34455=CARTESIAN_POINT('Ctrl Pts',(-3.84608078280016,1.0589088106385,10.3164217752187));
#34456=CARTESIAN_POINT('Ctrl Pts',(-3.81817959106573,1.2,10.3502388179897));
#34457=CARTESIAN_POINT('',(-3.99970644341025,-0.653834841531101,10.1163073168894));
#34458=CARTESIAN_POINT('Ctrl Pts',(-3.99970644341023,-0.653834841531111,
10.1163073168894));
#34459=CARTESIAN_POINT('Ctrl Pts',(-3.95891593940165,-0.575966355975947,
10.1082384035645));
#34460=CARTESIAN_POINT('Ctrl Pts',(-3.92429340983449,-0.493639798317628,
10.1021623354875));
#34461=CARTESIAN_POINT('Ctrl Pts',(-3.87408237926539,-0.338140650733339,
10.0958281963273));
#34462=CARTESIAN_POINT('Ctrl Pts',(-3.85622336702604,-0.265666408457172,
10.0948144796845));
#34463=CARTESIAN_POINT('Ctrl Pts',(-3.83202394298176,-0.129722242244509,
10.0977329215106));
#34464=CARTESIAN_POINT('Ctrl Pts',(-3.82439528475797,-0.066627635979717,
10.1009429954397));
#34465=CARTESIAN_POINT('Ctrl Pts',(-3.81609773603222,0.0595477087246973,
10.1113738105213));
#34466=CARTESIAN_POINT('Ctrl Pts',(-3.8153544130588,0.122784223523335,10.1186606316291));
#34467=CARTESIAN_POINT('Ctrl Pts',(-3.82182947500263,0.26013995765241,10.1383623818109));
#34468=CARTESIAN_POINT('Ctrl Pts',(-3.83052491254541,0.333957153420333,
10.1514746983359));
#34469=CARTESIAN_POINT('Ctrl Pts',(-3.86115450447686,0.491217719043045,
10.1842373489534));
#34470=CARTESIAN_POINT('Ctrl Pts',(-3.88506933429854,0.574353853455511,
10.2048500775317));
#34471=CARTESIAN_POINT('Ctrl Pts',(-3.91593537807148,0.653834841386436,
10.2278623010425));
#34472=CARTESIAN_POINT('',(-3.95668316628078,-1.2,10.1744173079227));
#34473=CARTESIAN_POINT('Ctrl Pts',(-3.95668316628078,-1.2,10.1744173079227));
#34474=CARTESIAN_POINT('Ctrl Pts',(-3.96492264622143,-1.12750309682141,
10.1634568379533));
#34475=CARTESIAN_POINT('Ctrl Pts',(-3.97439867849545,-1.03220200323701,
10.1507580406354));
#34476=CARTESIAN_POINT('Ctrl Pts',(-3.99268946522797,-0.796459678297759,
10.1259357400627));
#34477=CARTESIAN_POINT('Ctrl Pts',(-3.99590797836092,-0.740048759787163,
10.1215168999278));
#34478=CARTESIAN_POINT('Ctrl Pts',(-3.99970644341023,-0.653834841531099,
10.1163073168894));
#34479=CARTESIAN_POINT('Ctrl Pts',(-3.83170332429324,-1.30000000000002,
10.1733061790875));
#34480=CARTESIAN_POINT('Ctrl Pts',(-3.84079303276221,-1.29262062153828,
10.1736293612034));
#34481=CARTESIAN_POINT('Ctrl Pts',(-3.85131337624757,-1.28398008608649,
10.1741514649677));
#34482=CARTESIAN_POINT('Ctrl Pts',(-3.87298321825068,-1.26674725507027,
10.1742566864986));
#34483=CARTESIAN_POINT('Ctrl Pts',(-3.88398522746645,-1.25800071781436,
10.1742825776218));
#34484=CARTESIAN_POINT('Ctrl Pts',(-3.90782377744779,-1.23869680098493,
10.174873105833));
#34485=CARTESIAN_POINT('Ctrl Pts',(-3.93037425193878,-1.22042603079793,
10.1754216007778));
#34486=CARTESIAN_POINT('Ctrl Pts',(-3.95668316628078,-1.2,10.1744173079227));
#34487=CARTESIAN_POINT('Origin',(0.,1.25,7.2));
#34488=CARTESIAN_POINT('Origin',(0.,1.2,7.2));
#34489=CARTESIAN_POINT('Origin',(0.,0.92691742076555,7.2));
#34490=CARTESIAN_POINT('Origin',(0.,0.653834841531101,7.2));
#34491=CARTESIAN_POINT('Origin',(0.,0.,7.2));
#34492=CARTESIAN_POINT('Origin',(0.,-0.653834841531101,7.2));
#34493=CARTESIAN_POINT('Origin',(0.,-0.926917420765551,7.2));
#34494=CARTESIAN_POINT('Origin',(0.,-1.2,7.2));
#34495=CARTESIAN_POINT('Origin',(0.,-1.25,7.2));
#34496=CARTESIAN_POINT('Ctrl Pts',(-4.24541645780663,-1.30000000000008,
9.92487448592682));
#34497=CARTESIAN_POINT('Ctrl Pts',(-4.2271889327826,-1.18514270861184,9.96338122303863));
#34498=CARTESIAN_POINT('Ctrl Pts',(-4.20407556081819,-1.06847604194514,
9.98826899902922));
#34499=CARTESIAN_POINT('Ctrl Pts',(-4.13939176392353,-0.794772684000851,
10.0143022156962));
#34500=CARTESIAN_POINT('Ctrl Pts',(-4.07792758948489,-0.636309800095197,
9.98082322651161));
#34501=CARTESIAN_POINT('Ctrl Pts',(-4.00511469268244,-0.319434907277159,
9.96682083809129));
#34502=CARTESIAN_POINT('Ctrl Pts',(-3.96570274858467,-0.158333333333333,
9.94336202437368));
#34503=CARTESIAN_POINT('Ctrl Pts',(-3.94621238249364,0.158333333333334,
9.97107548348392));
#34504=CARTESIAN_POINT('Ctrl Pts',(-3.96518266533145,0.319434907277167,
10.0234576048964));
#34505=CARTESIAN_POINT('Ctrl Pts',(-4.00023280952294,0.636309800095206,
10.0914459396341));
#34506=CARTESIAN_POINT('Ctrl Pts',(-4.04051677784849,0.79477268400084,10.1539214617338));
#34507=CARTESIAN_POINT('Ctrl Pts',(-4.08016499765647,1.06847604194587,10.1667952068506));
#34508=CARTESIAN_POINT('Ctrl Pts',(-4.09477284803601,1.18514270861327,10.1563511401463));
#34509=CARTESIAN_POINT('Ctrl Pts',(-4.10682630355149,1.30000000000221,10.1298904394961));
#34510=CARTESIAN_POINT('Ctrl Pts',(-4.24251264986958,-1.30000000000008,
9.91931621425302));
#34511=CARTESIAN_POINT('Ctrl Pts',(-4.22370557786425,-1.18514270861184,
9.95678523527321));
#34512=CARTESIAN_POINT('Ctrl Pts',(-4.20017735680198,-1.06847604194514,
9.98090562176186));
#34513=CARTESIAN_POINT('Ctrl Pts',(-4.13491566055947,-0.794772684000851,
10.0057905236644));
#34514=CARTESIAN_POINT('Ctrl Pts',(-4.07363130379674,-0.636309800095197,
9.97243807038172));
#34515=CARTESIAN_POINT('Ctrl Pts',(-4.00084366736096,-0.319434907277159,
9.95836321152855));
#34516=CARTESIAN_POINT('Ctrl Pts',(-3.96153146947934,-0.158333333333333,
9.93533203941429));
#34517=CARTESIAN_POINT('Ctrl Pts',(-3.94221421727185,0.158333333333334,
9.96288667338731));
#34518=CARTESIAN_POINT('Ctrl Pts',(-3.96131125943563,0.319434907277167,
10.0146301197666));
#34519=CARTESIAN_POINT('Ctrl Pts',(-3.99658000881247,0.636309800095206,
10.0824737541014));
#34520=CARTESIAN_POINT('Ctrl Pts',(-4.03677336078499,0.79477268400084,10.1447526052678));
#34521=CARTESIAN_POINT('Ctrl Pts',(-4.07697631454619,1.06847604194587,10.1588054041015));
#34522=CARTESIAN_POINT('Ctrl Pts',(-4.0919424571672,1.18514270861327,10.1491838891105));
#34523=CARTESIAN_POINT('Ctrl Pts',(-4.10447237339219,1.30000000000221,10.1238579232207));
#34524=CARTESIAN_POINT('Ctrl Pts',(-4.23681986628123,-1.3000000000001,9.9080585135877));
#34525=CARTESIAN_POINT('Ctrl Pts',(-4.21674166253644,-1.18514270861185,
9.94357552431802));
#34526=CARTESIAN_POINT('Ctrl Pts',(-4.19229548072165,-1.06847604194515,
9.96625706117423));
#34527=CARTESIAN_POINT('Ctrl Pts',(-4.1257290071349,-0.794772684000856,
9.98900343636103));
#34528=CARTESIAN_POINT('Ctrl Pts',(-4.06469021042839,-0.636309800095198,
9.95601141287329));
#34529=CARTESIAN_POINT('Ctrl Pts',(-3.99208575376412,-0.319434907277158,
9.94165487404065));
#34530=CARTESIAN_POINT('Ctrl Pts',(-3.95335341894101,-0.158333333333333,
9.91909219744007));
#34531=CARTESIAN_POINT('Ctrl Pts',(-3.93450274268745,0.158333333333335,
9.94620879746131));
#34532=CARTESIAN_POINT('Ctrl Pts',(-3.95367786492859,0.319434907277169,
9.99685790233624));
#34533=CARTESIAN_POINT('Ctrl Pts',(-3.98932401498674,0.636309800095209,
10.0644735326305));
#34534=CARTESIAN_POINT('Ctrl Pts',(-4.02933574586201,0.79477268400084,10.1263541693987));
#34535=CARTESIAN_POINT('Ctrl Pts',(-4.07064867242679,1.06847604194587,10.1427653324373));
#34536=CARTESIAN_POINT('Ctrl Pts',(-4.08633771688935,1.18514270861327,10.1347839656526));
#34537=CARTESIAN_POINT('Ctrl Pts',(-4.09983297069931,1.30000000000221,10.1117174476973));
#34538=CARTESIAN_POINT('Ctrl Pts',(-4.22773027115874,-1.3000000000001,9.89184542464046));
#34539=CARTESIAN_POINT('Ctrl Pts',(-4.20673506497644,-1.18514270861185,
9.92334340244841));
#34540=CARTESIAN_POINT('Ctrl Pts',(-4.18151913362969,-1.06847604194515,
9.94319197628689));
#34541=CARTESIAN_POINT('Ctrl Pts',(-4.11351456830585,-0.794772684000856,
9.96213369892261));
#34542=CARTESIAN_POINT('Ctrl Pts',(-4.05176903880094,-0.636309800095199,
9.93083420913925));
#34543=CARTESIAN_POINT('Ctrl Pts',(-3.97883825081608,-0.319434907277159,
9.91667421944362));
#34544=CARTESIAN_POINT('Ctrl Pts',(-3.94078375282828,-0.158333333333333,
9.89502227718623));
#34545=CARTESIAN_POINT('Ctrl Pts',(-3.92215022335235,0.158333333333335,
9.92194096575744));
#34546=CARTESIAN_POINT('Ctrl Pts',(-3.9409421645071,0.319434907277169,9.9713830921904));
#34547=CARTESIAN_POINT('Ctrl Pts',(-3.97719907804311,0.636309800095209,
10.0385993384994));
#34548=CARTESIAN_POINT('Ctrl Pts',(-4.01782137157219,0.794772684000842,
10.0990389685616));
#34549=CARTESIAN_POINT('Ctrl Pts',(-4.06081173472643,1.06847604194587,10.1190064288439));
#34550=CARTESIAN_POINT('Ctrl Pts',(-4.07741740679809,1.18514270861328,10.1136670291134));
#34551=CARTESIAN_POINT('Ctrl Pts',(-4.09201981568185,1.30000000000221,10.0943450559635));
#34552=CARTESIAN_POINT('Ctrl Pts',(-4.21852308140183,-1.3000000000001,9.8756612747752));
#34553=CARTESIAN_POINT('Ctrl Pts',(-4.19550261185785,-1.18514270861186,
9.90432169235314));
#34554=CARTESIAN_POINT('Ctrl Pts',(-4.16887662610448,-1.06847604194516,
9.9220231565384));
#34555=CARTESIAN_POINT('Ctrl Pts',(-4.09903580877927,-0.79477268400086,
9.93759970530387));
#34556=CARTESIAN_POINT('Ctrl Pts',(-4.03833506779414,-0.636309800095202,
9.9061569634847));
#34557=CARTESIAN_POINT('Ctrl Pts',(-3.96548412441517,-0.319434907277161,
9.89176508749895));
#34558=CARTESIAN_POINT('Ctrl Pts',(-3.927363106507,-0.158333333333334,9.87177971841636));
#34559=CARTESIAN_POINT('Ctrl Pts',(-3.90916433055663,0.158333333333335,
9.89828720877045));
#34560=CARTESIAN_POINT('Ctrl Pts',(-3.92839276445368,0.31943490727717,9.94571238450143));
#34561=CARTESIAN_POINT('Ctrl Pts',(-3.96558734864098,0.636309800095212,
10.0121990485734));
#34562=CARTESIAN_POINT('Ctrl Pts',(-4.00646810712007,0.794772684000845,
10.0715308840212));
#34563=CARTESIAN_POINT('Ctrl Pts',(-4.05119187067628,1.06847604194588,10.0949974551163));
#34564=CARTESIAN_POINT('Ctrl Pts',(-4.06878677662875,1.18514270861328,10.0922306101798));
#34565=CARTESIAN_POINT('Ctrl Pts',(-4.08461732846891,1.30000000000222,10.0765391112017));
#34566=CARTESIAN_POINT('Ctrl Pts',(-4.21277725489613,-1.30000000000011,
9.86437445357206));
#34567=CARTESIAN_POINT('Ctrl Pts',(-4.18871035144018,-1.18514270861186,
9.8908147696321));
#34568=CARTESIAN_POINT('Ctrl Pts',(-4.16129306149929,-1.06847604194516,
9.90692099325134));
#34569=CARTESIAN_POINT('Ctrl Pts',(-4.090213573903,-0.794772684000864,9.92025577098438));
#34570=CARTESIAN_POINT('Ctrl Pts',(-4.02940487828938,-0.636309800095204,
9.8895529233566));
#34571=CARTESIAN_POINT('Ctrl Pts',(-3.95658703201688,-0.319434907277162,
9.87503390675468));
#34572=CARTESIAN_POINT('Ctrl Pts',(-3.91917788307007,-0.158333333333335,
9.85539785270959));
#34573=CARTESIAN_POINT('Ctrl Pts',(-3.90119054960112,0.158333333333336,
9.88170489192799));
#34574=CARTESIAN_POINT('Ctrl Pts',(-3.91999084243052,0.319434907277171,
9.92849828883152));
#34575=CARTESIAN_POINT('Ctrl Pts',(-3.95743578244152,0.636309800095215,
9.99487084286091));
#34576=CARTESIAN_POINT('Ctrl Pts',(-3.99853228417306,0.794772684000848,
10.053411740087));
#34577=CARTESIAN_POINT('Ctrl Pts',(-4.04440238583212,1.06847604194588,10.0792434466343));
#34578=CARTESIAN_POINT('Ctrl Pts',(-4.06267934271888,1.18514270861329,10.0781861728379));
#34579=CARTESIAN_POINT('Ctrl Pts',(-4.07937778913892,1.30000000000222,10.0648900366399));
#34580=CARTESIAN_POINT('Ctrl Pts',(-4.20970628126203,-1.30000000000011,
9.85885446397306));
#34581=CARTESIAN_POINT('Ctrl Pts',(-4.18521300724093,-1.18514270861186,
9.88405188320314));
#34582=CARTESIAN_POINT('Ctrl Pts',(-4.15746191721057,-1.06847604194516,
9.89927317397398));
#34583=CARTESIAN_POINT('Ctrl Pts',(-4.08582514094864,-0.794772684000863,
9.91139054820488));
#34584=CARTESIAN_POINT('Ctrl Pts',(-4.02493162928629,-0.636309800095206,
9.88110165101293));
#34585=CARTESIAN_POINT('Ctrl Pts',(-3.95197514461098,-0.319434907277163,
9.86667820019585));
#34586=CARTESIAN_POINT('Ctrl Pts',(-3.91461123572,-0.158333333333335,9.84754083457005));
#34587=CARTESIAN_POINT('Ctrl Pts',(-3.89674427954975,0.158333333333336,
9.87373343071214));
#34588=CARTESIAN_POINT('Ctrl Pts',(-3.91570877873406,0.319434907277172,
9.91982112826059));
#34589=CARTESIAN_POINT('Ctrl Pts',(-3.95335612966987,0.636309800095216,
9.98605355826342));
#34590=CARTESIAN_POINT('Ctrl Pts',(-3.99429516133064,0.794772684000851,
10.0444522831198));
#34591=CARTESIAN_POINT('Ctrl Pts',(-4.04075765464447,1.06847604194588,10.0714686819131));
#34592=CARTESIAN_POINT('Ctrl Pts',(-4.0594320810401,1.18514270861329,10.0712266075604));
#34593=CARTESIAN_POINT('Ctrl Pts',(-4.07666904208079,1.30000000000222,10.0590480608735));
#34594=CARTESIAN_POINT('Ctrl Pts',(-4.20963545591083,-1.30000000000011,
9.85872702181624));
#34595=CARTESIAN_POINT('Ctrl Pts',(-4.18513223806645,-1.18514270861186,
9.88389587516515));
#34596=CARTESIAN_POINT('Ctrl Pts',(-4.15737337933957,-1.06847604194516,
9.89909681736857));
#34597=CARTESIAN_POINT('Ctrl Pts',(-4.08572368081249,-0.794772684000863,
9.91118616597669));
#34598=CARTESIAN_POINT('Ctrl Pts',(-4.02482827235545,-0.636309800095206,
9.88090674820191));
#34599=CARTESIAN_POINT('Ctrl Pts',(-3.95186872525836,-0.319434907277163,
9.86648535991826));
#34600=CARTESIAN_POINT('Ctrl Pts',(-3.91450611474061,-0.158333333333335,
9.84735924543995));
#34601=CARTESIAN_POINT('Ctrl Pts',(-3.89664190857931,0.158333333333336,
9.87354922796575));
#34602=CARTESIAN_POINT('Ctrl Pts',(-3.91560983625881,0.319434907277172,
9.91962100343749));
#34603=CARTESIAN_POINT('Ctrl Pts',(-3.95326182446619,0.636309800095215,
9.98585023775694));
#34604=CARTESIAN_POINT('Ctrl Pts',(-3.99419753968574,0.79477268400085,10.0442453697909));
#34605=CARTESIAN_POINT('Ctrl Pts',(-4.04067373102421,1.06847604194588,10.0712890816844));
#34606=CARTESIAN_POINT('Ctrl Pts',(-4.05935728940721,1.18514270861329,10.0710658594948));
#34607=CARTESIAN_POINT('Ctrl Pts',(-4.07660658505531,1.30000000000222,10.0589131943051));
#34608=CARTESIAN_POINT('Ctrl Pts',(-4.20956455372579,-1.30000000000011,
9.85859966803531));
#34609=CARTESIAN_POINT('Ctrl Pts',(-4.18505141943581,-1.18514270861186,
9.8837399224243));
#34610=CARTESIAN_POINT('Ctrl Pts',(-4.15728481071699,-1.06847604194516,
9.89892049350013));
#34611=CARTESIAN_POINT('Ctrl Pts',(-4.08562221309949,-0.794772684000863,
9.91098178866697));
#34612=CARTESIAN_POINT('Ctrl Pts',(-4.0247249144713,-0.636309800095206,
9.88071184746151));
#34613=CARTESIAN_POINT('Ctrl Pts',(-3.95176225583807,-0.319434907277163,
9.86629257173117));
#34614=CARTESIAN_POINT('Ctrl Pts',(-3.91440082462096,-0.158333333333335,
9.84717782853973));
#34615=CARTESIAN_POINT('Ctrl Pts',(-3.89653938038487,0.158333333333336,
9.87336518476813));
#34616=CARTESIAN_POINT('Ctrl Pts',(-3.91551088497831,0.319434907277172,
9.9194208877983));
#34617=CARTESIAN_POINT('Ctrl Pts',(-3.95316754834085,0.636309800095215,
9.98564688632071));
#34618=CARTESIAN_POINT('Ctrl Pts',(-3.9940998582532,0.794772684000851,10.0440385122106));
#34619=CARTESIAN_POINT('Ctrl Pts',(-4.04058975015895,1.06847604194588,10.0711095347789));
#34620=CARTESIAN_POINT('Ctrl Pts',(-4.0592824557011,1.18514270861329,10.0709051503023));
#34621=CARTESIAN_POINT('Ctrl Pts',(-4.07654411519959,1.30000000000222,10.0587783387596));
#34622=CARTESIAN_POINT('Ctrl Pts',(-4.20942270138084,-1.30000000000011,
9.85834500849095));
#34623=CARTESIAN_POINT('Ctrl Pts',(-4.18488967018863,-1.18514270861186,
9.88342813329698));
#34624=CARTESIAN_POINT('Ctrl Pts',(-4.15710752302828,-1.06847604194516,
9.89856800290258));
#34625=CARTESIAN_POINT('Ctrl Pts',(-4.08541909741854,-0.794772684000863,
9.91057322175767));
#34626=CARTESIAN_POINT('Ctrl Pts',(-4.02451808128831,-0.636309800095206,
9.88032216363038));
#34627=CARTESIAN_POINT('Ctrl Pts',(-3.95154926822279,-0.319434907277163,
9.86590704002388));
#34628=CARTESIAN_POINT('Ctrl Pts',(-3.91419029087762,-0.158333333333335,
9.84681494278848));
#34629=CARTESIAN_POINT('Ctrl Pts',(-3.89633435929325,0.158333333333336,
9.87299705619156));
#34630=CARTESIAN_POINT('Ctrl Pts',(-3.91531286007442,0.319434907277171,
9.91902077196273));
#34631=CARTESIAN_POINT('Ctrl Pts',(-3.95297888652735,0.636309800095215,
9.98524028740749));
#34632=CARTESIAN_POINT('Ctrl Pts',(-3.99390457240559,0.79477268400085,10.0436247170789));
#34633=CARTESIAN_POINT('Ctrl Pts',(-4.04042189267401,1.06847604194588,10.0707503352224));
#34634=CARTESIAN_POINT('Ctrl Pts',(-4.0591328728242,1.18514270861329,10.070583646189));
#34635=CARTESIAN_POINT('Ctrl Pts',(-4.0764192088169,1.30000000000222,10.058508593131));
#34636=CARTESIAN_POINT('Ctrl Pts',(-4.20911489946616,-1.30000000000011,
9.85779374196368));
#34637=CARTESIAN_POINT('Ctrl Pts',(-4.18453859769891,-1.18514270861186,
9.88275324427473));
#34638=CARTESIAN_POINT('Ctrl Pts',(-4.15672269581207,-1.06847604194516,
9.89780501156095));
#34639=CARTESIAN_POINT('Ctrl Pts',(-4.08497827354528,-0.794772684000863,
9.90968875514491));
#34640=CARTESIAN_POINT('Ctrl Pts',(-4.02406948399971,-0.636309800095206,
9.87947831400066));
#34641=CARTESIAN_POINT('Ctrl Pts',(-3.95108743737665,-0.319434907277163,
9.86507207165953));
#34642=CARTESIAN_POINT('Ctrl Pts',(-3.91373372858721,-0.158333333333335,
9.84602908681854));
#34643=CARTESIAN_POINT('Ctrl Pts',(-3.8958897421842,0.158333333333336,9.87219983137673));
#34644=CARTESIAN_POINT('Ctrl Pts',(-3.9148833111106,0.319434907277172,9.91815432514302));
#34645=CARTESIAN_POINT('Ctrl Pts',(-3.95256980967421,0.636309800095216,
9.98435960611405));
#34646=CARTESIAN_POINT('Ctrl Pts',(-3.99348156089107,0.794772684000851,
10.0427280298469));
#34647=CARTESIAN_POINT('Ctrl Pts',(-4.04005842136669,1.06847604194588,10.0699718320407));
#34648=CARTESIAN_POINT('Ctrl Pts',(-4.05880897032625,1.18514270861329,10.0698868459808));
#34649=CARTESIAN_POINT('Ctrl Pts',(-4.07614867118817,1.30000000000222,10.0579240413735));
#34650=CARTESIAN_POINT('Ctrl Pts',(-4.20863976745657,-1.30000000000011,
9.85694734936963));
#34651=CARTESIAN_POINT('Ctrl Pts',(-4.18399602124621,-1.18514270861186,
9.88171755971258));
#34652=CARTESIAN_POINT('Ctrl Pts',(-4.15612769058842,-1.06847604194516,
9.89663428854023));
#34653=CARTESIAN_POINT('Ctrl Pts',(-4.08429683657899,-0.794772684000863,
9.90833140273091));
#34654=CARTESIAN_POINT('Ctrl Pts',(-4.02337734430711,-0.636309800095206,
9.87818210770303));
#34655=CARTESIAN_POINT('Ctrl Pts',(-3.95037564248984,-0.319434907277163,
9.8637887589159));
#34656=CARTESIAN_POINT('Ctrl Pts',(-3.91303039482342,-0.158333333333335,
9.84482095921614));
#34657=CARTESIAN_POINT('Ctrl Pts',(-3.89520475213598,0.158333333333336,
9.87097421369106));
#34658=CARTESIAN_POINT('Ctrl Pts',(-3.91422042138237,0.319434907277172,
9.91682327553824));
#34659=CARTESIAN_POINT('Ctrl Pts',(-3.95193905333691,0.636309800095215,
9.98300602138339));
#34660=CARTESIAN_POINT('Ctrl Pts',(-3.99283160922943,0.79477268400085,10.0413476062463));
#34661=CARTESIAN_POINT('Ctrl Pts',(-4.03950053014917,1.06847604194588,10.0687727924243));
#34662=CARTESIAN_POINT('Ctrl Pts',(-4.05831175619488,1.18514270861329,10.0688137102661));
#34663=CARTESIAN_POINT('Ctrl Pts',(-4.07573296167402,1.30000000000222,10.0570241990566));
#34664=CARTESIAN_POINT('Ctrl Pts',(-4.20806696965542,-1.30000000000011,
9.85593446970752));
#34665=CARTESIAN_POINT('Ctrl Pts',(-4.18334015744563,-1.18514270861186,
9.88047976421315));
#34666=CARTESIAN_POINT('Ctrl Pts',(-4.15540768083246,-1.06847604194516,
9.89523572728958));
#34667=CARTESIAN_POINT('Ctrl Pts',(-4.08347234592043,-0.794772684000863,
9.90670963996597));
#34668=CARTESIAN_POINT('Ctrl Pts',(-4.02254283004788,-0.636309800095206,
9.87663069019566));
#34669=CARTESIAN_POINT('Ctrl Pts',(-3.94951942063887,-0.319434907277163,
9.86225079315611));
#34670=CARTESIAN_POINT('Ctrl Pts',(-3.91218578056065,-0.158333333333335,
9.84337171740359));
#34671=CARTESIAN_POINT('Ctrl Pts',(-3.89438204868042,0.158333333333336,
9.86950402703382));
#34672=CARTESIAN_POINT('Ctrl Pts',(-3.91342112525749,0.319434907277171,
9.91522966746529));
#34673=CARTESIAN_POINT('Ctrl Pts',(-3.9511794034085,0.636309800095215,9.98138431152671));
#34674=CARTESIAN_POINT('Ctrl Pts',(-3.99205408438125,0.79477268400085,10.0396886129266));
#34675=CARTESIAN_POINT('Ctrl Pts',(-4.03883435040479,1.06847604194588,10.0673306244702));
#34676=CARTESIAN_POINT('Ctrl Pts',(-4.05771784961653,1.18514270861329,10.0675231719302));
#34677=CARTESIAN_POINT('Ctrl Pts',(-4.07523540425804,1.30000000000222,10.0559430642906));
#34678=CARTESIAN_POINT('Ctrl Pts',(-4.20729978356503,-1.30000000000011,
9.85458758065339));
#34679=CARTESIAN_POINT('Ctrl Pts',(-4.18245885715696,-1.18514270861186,
9.87883653400406));
#34680=CARTESIAN_POINT('Ctrl Pts',(-4.15443889534823,-1.06847604194516,
9.89338019829312));
#34681=CARTESIAN_POINT('Ctrl Pts',(-4.08236297045647,-0.794772684000863,
9.90455781298223));
#34682=CARTESIAN_POINT('Ctrl Pts',(-4.02142431303854,-0.636309800095206,
9.87456810921836));
#34683=CARTESIAN_POINT('Ctrl Pts',(-3.9483749932468,-0.319434907277163,
9.8602029025274));
#34684=CARTESIAN_POINT('Ctrl Pts',(-3.9110595018654,-0.158333333333335,
9.84143937715152));
#34685=CARTESIAN_POINT('Ctrl Pts',(-3.89328483770833,0.158333333333336,
9.86754382120249));
#34686=CARTESIAN_POINT('Ctrl Pts',(-3.91234996015436,0.319434907277172,
9.91311004771467));
#34687=CARTESIAN_POINT('Ctrl Pts',(-3.95016254525791,0.636309800095215,
9.97922582794848));
#34688=CARTESIAN_POINT('Ctrl Pts',(-3.99102131770104,0.79477268400085,10.0374726331695));
#34689=CARTESIAN_POINT('Ctrl Pts',(-4.03795128511267,1.06847604194588,10.0654025539362));
#34690=CARTESIAN_POINT('Ctrl Pts',(-4.05693027753792,1.18514270861329,10.0657981457286));
#34691=CARTESIAN_POINT('Ctrl Pts',(-4.07457401842252,1.30000000000222,10.0544995015191));
#34692=CARTESIAN_POINT('Ctrl Pts',(-4.20633388256444,-1.30000000000011,
9.85291111779125));
#34693=CARTESIAN_POINT('Ctrl Pts',(-4.18134193001888,-1.18514270861186,
9.87679856646903));
#34694=CARTESIAN_POINT('Ctrl Pts',(-4.15320771225699,-1.06847604194516,
9.89108205667209));
#34695=CARTESIAN_POINT('Ctrl Pts',(-4.0809527797383,-0.794772684000862,
9.9018927111017));
#34696=CARTESIAN_POINT('Ctrl Pts',(-4.02001288636102,-0.636309800095206,
9.87200356719769));
#34697=CARTESIAN_POINT('Ctrl Pts',(-3.9469391178162,-0.319434907277163,
9.85764827324214));
#34698=CARTESIAN_POINT('Ctrl Pts',(-3.90965405515109,-0.158333333333335,
9.83902122733326));
#34699=CARTESIAN_POINT('Ctrl Pts',(-3.89191535958804,0.158333333333336,
9.86509101628633));
#34700=CARTESIAN_POINT('Ctrl Pts',(-3.91099923026029,0.319434907277171,
9.91047179106491));
#34701=CARTESIAN_POINT('Ctrl Pts',(-3.94888262509831,0.636309800095215,
9.97653623166595));
#34702=CARTESIAN_POINT('Ctrl Pts',(-3.98974110428675,0.79477268400085,10.0346919588768));
#34703=CARTESIAN_POINT('Ctrl Pts',(-4.03686087928501,1.06847604194588,10.062979181776));
#34704=CARTESIAN_POINT('Ctrl Pts',(-4.05595689544923,1.18514270861329,10.0636308936443));
#34705=CARTESIAN_POINT('Ctrl Pts',(-4.07375252314058,1.30000000000222,10.0526898267328));
#34706=CARTESIAN_POINT('Ctrl Pts',(-4.20399595551413,-1.3000000000001,9.8489076789416));
#34707=CARTESIAN_POINT('Ctrl Pts',(-4.17861348591113,-1.18514270861186,
9.87195746698897));
#34708=CARTESIAN_POINT('Ctrl Pts',(-4.15018848428161,-1.06847604194516,
9.88563419569662));
#34709=CARTESIAN_POINT('Ctrl Pts',(-4.07749218647761,-0.794772684000863,
9.89557653288265));
#34710=CARTESIAN_POINT('Ctrl Pts',(-4.01658172222461,-0.636309800095205,
9.86589371255771));
#34711=CARTESIAN_POINT('Ctrl Pts',(-3.94347564908434,-0.319434907277163,
9.85153423006119));
#34712=CARTESIAN_POINT('Ctrl Pts',(-3.90629110283546,-0.158333333333335,
9.83320656333423));
#34713=CARTESIAN_POINT('Ctrl Pts',(-3.88863762367487,0.158333333333336,
9.85919366497471));
#34714=CARTESIAN_POINT('Ctrl Pts',(-3.9077196744278,0.319434907277172,9.90417613627861));
#34715=CARTESIAN_POINT('Ctrl Pts',(-3.94578149555549,0.636309800095215,
9.97010941087807));
#34716=CARTESIAN_POINT('Ctrl Pts',(-3.98670278361234,0.79477268400085,10.02798434251));
#34717=CARTESIAN_POINT('Ctrl Pts',(-4.03428693524991,1.06847604194588,10.0571205549456));
#34718=CARTESIAN_POINT('Ctrl Pts',(-4.05365640950548,1.18514270861328,10.0583942458085));
#34719=CARTESIAN_POINT('Ctrl Pts',(-4.07179794193922,1.30000000000222,10.048329640774));
#34720=CARTESIAN_POINT('Ctrl Pts',(-4.20040784106706,-1.3000000000001,9.84298435754321));
#34721=CARTESIAN_POINT('Ctrl Pts',(-4.1743076309958,-1.18514270861185,9.86491912305311));
#34722=CARTESIAN_POINT('Ctrl Pts',(-4.14536838919967,-1.06847604194516,
9.87776936096711));
#34723=CARTESIAN_POINT('Ctrl Pts',(-4.07195422014435,-0.794772684000861,
9.88646890512968));
#34724=CARTESIAN_POINT('Ctrl Pts',(-4.0112364048357,-0.636309800095204,
9.85693508166246));
#34725=CARTESIAN_POINT('Ctrl Pts',(-3.93821104618483,-0.319434907277162,
9.84243266425045));
#34726=CARTESIAN_POINT('Ctrl Pts',(-3.90131968533194,-0.158333333333334,
9.82440782567619));
#34727=CARTESIAN_POINT('Ctrl Pts',(-3.88379015100995,0.158333333333336,
9.85027179693815));
#34728=CARTESIAN_POINT('Ctrl Pts',(-3.90263894184727,0.31943490727717,9.89488746204669));
#34729=CARTESIAN_POINT('Ctrl Pts',(-3.94100291802066,0.636309800095213,
9.96059237479716));
#34730=CARTESIAN_POINT('Ctrl Pts',(-3.98231865005701,0.794772684000848,
10.017752737638));
#34731=CARTESIAN_POINT('Ctrl Pts',(-4.03063693422305,1.06847604194588,10.0481259924018));
#34732=CARTESIAN_POINT('Ctrl Pts',(-4.05037942106035,1.18514270861328,10.050368943366));
#34733=CARTESIAN_POINT('Ctrl Pts',(-4.06894919988829,1.30000000000222,10.0417073887471));
#34734=CARTESIAN_POINT('Ctrl Pts',(-4.1968256822688,-1.3000000000001,9.83705064195634));
#34735=CARTESIAN_POINT('Ctrl Pts',(-4.1700044681053,-1.18514270861185,9.85787241418812));
#34736=CARTESIAN_POINT('Ctrl Pts',(-4.14054247363241,-1.06847604194516,
9.86990432345096));
#34737=CARTESIAN_POINT('Ctrl Pts',(-4.06637864174727,-0.79477268400086,
9.87739409895908));
#34738=CARTESIAN_POINT('Ctrl Pts',(-4.00580735908187,-0.636309800095204,
9.84805992860588));
#34739=CARTESIAN_POINT('Ctrl Pts',(-3.93282936913909,-0.319434907277162,
9.83345069349348));
#34740=CARTESIAN_POINT('Ctrl Pts',(-3.89622042641662,-0.158333333333334,
9.81574129977556));
#34741=CARTESIAN_POINT('Ctrl Pts',(-3.87882705640936,0.158333333333336,
9.84146716804513));
#34742=CARTESIAN_POINT('Ctrl Pts',(-3.8974936901642,0.319434907277171,9.88565824574615));
#34743=CARTESIAN_POINT('Ctrl Pts',(-3.93616078690375,0.636309800095214,
9.95112968001173));
#34744=CARTESIAN_POINT('Ctrl Pts',(-3.97779854689507,0.794772684000848,
10.0076472985041));
#34745=CARTESIAN_POINT('Ctrl Pts',(-4.02687371345706,1.06847604194588,10.0392359805595));
#34746=CARTESIAN_POINT('Ctrl Pts',(-4.04701803744443,1.18514270861328,10.0424206334433));
#34747=CARTESIAN_POINT('Ctrl Pts',(-4.06606386422855,1.30000000000222,10.035116369225));
#34748=CARTESIAN_POINT('Ctrl Pts',(-4.19448001643774,-1.3000000000001,9.83304924992269));
#34749=CARTESIAN_POINT('Ctrl Pts',(-4.16724072708871,-1.18514270861185,
9.85306085170418));
#34750=CARTESIAN_POINT('Ctrl Pts',(-4.13746434556555,-1.06847604194516,
9.86450992596167));
#34751=CARTESIAN_POINT('Ctrl Pts',(-4.06281375703653,-0.79477268400086,
9.87117842636774));
#34752=CARTESIAN_POINT('Ctrl Pts',(-4.00225118025671,-0.636309800095204,
9.84207406594856));
#34753=CARTESIAN_POINT('Ctrl Pts',(-3.92922046485511,-0.319434907277162,
9.82748327159995));
#34754=CARTESIAN_POINT('Ctrl Pts',(-3.89271235913522,-0.158333333333334,
9.81007549925909));
#34755=CARTESIAN_POINT('Ctrl Pts',(-3.87541122126775,0.158333333333336,
9.83570817700522));
#34756=CARTESIAN_POINT('Ctrl Pts',(-3.89409296887522,0.319434907277171,
9.87947571683529));
#34757=CARTESIAN_POINT('Ctrl Pts',(-3.93295234798587,0.636309800095213,
9.94479740068427));
#34758=CARTESIAN_POINT('Ctrl Pts',(-3.97464088946348,0.794772684000847,
10.001046114713));
#34759=CARTESIAN_POINT('Ctrl Pts',(-4.02421355278176,1.06847604194588,10.0334526591426));
#34760=CARTESIAN_POINT('Ctrl Pts',(-4.04465393193101,1.18514270861328,10.0372384894363));
#34761=CARTESIAN_POINT('Ctrl Pts',(-4.06407652112715,1.30000000000222,10.0307825577209));
#34762=CARTESIAN_POINT('Ctrl Pts',(-4.19292299273677,-1.3000000000001,9.83037415643151));
#34763=CARTESIAN_POINT('Ctrl Pts',(-4.1654137661498,-1.18514270861185,9.8498359998899));
#34764=CARTESIAN_POINT('Ctrl Pts',(-4.13543275923749,-1.06847604194516,
9.86089103928364));
#34765=CARTESIAN_POINT('Ctrl Pts',(-4.06046032856068,-0.79477268400086,
9.86700899267152));
#34766=CARTESIAN_POINT('Ctrl Pts',(-3.99989325823722,-0.636309800095204,
9.83806908637676));
#34767=CARTESIAN_POINT('Ctrl Pts',(-3.92681497328307,-0.319434907277162,
9.82350388919076));
#34768=CARTESIAN_POINT('Ctrl Pts',(-3.89035937021541,-0.158333333333334,
9.80631285247433));
#34769=CARTESIAN_POINT('Ctrl Pts',(-3.87311760228999,0.158333333333336,
9.83188568740066));
#34770=CARTESIAN_POINT('Ctrl Pts',(-3.89182538863478,0.319434907277171,
9.8753541709064));
#34771=CARTESIAN_POINT('Ctrl Pts',(-3.93081421873702,0.636309800095213,
9.94057414790096));
#34772=CARTESIAN_POINT('Ctrl Pts',(-3.97252364569437,0.794772684000847,
9.99665590741682));
#34773=CARTESIAN_POINT('Ctrl Pts',(-4.02242720258882,1.06847604194588,10.0296086204888));
#34774=CARTESIAN_POINT('Ctrl Pts',(-4.04306684180308,1.18514270861328,10.0337936350233));
#34775=CARTESIAN_POINT('Ctrl Pts',(-4.06274471956094,1.30000000000222,10.0278996556217));
#34776=CARTESIAN_POINT('Ctrl Pts',(-4.18867884642207,-1.3000000000001,9.82297686484869));
#34777=CARTESIAN_POINT('Ctrl Pts',(-4.16048043130391,-1.18514270861185,
9.84086892551032));
#34778=CARTESIAN_POINT('Ctrl Pts',(-4.12996650707679,-1.06847604194516,
9.85080774886732));
#34779=CARTESIAN_POINT('Ctrl Pts',(-4.05412394856475,-0.79477268400086,
9.85539484986342));
#34780=CARTESIAN_POINT('Ctrl Pts',(-3.99347745659756,-0.636309800095204,
9.82698000795613));
#34781=CARTESIAN_POINT('Ctrl Pts',(-3.92019730142325,-0.319434907277162,
9.81256084403552));
#34782=CARTESIAN_POINT('Ctrl Pts',(-3.88380645695757,-0.158333333333334,
9.79604955309708));
#34783=CARTESIAN_POINT('Ctrl Pts',(-3.86672209666436,0.158333333333336,
9.82146449407055));
#34784=CARTESIAN_POINT('Ctrl Pts',(-3.88560788011893,0.319434907277171,
9.86400104662747));
#34785=CARTESIAN_POINT('Ctrl Pts',(-3.92494536056161,0.636309800095213,
9.92894543616526));
#34786=CARTESIAN_POINT('Ctrl Pts',(-3.96659069941214,0.794772684000848,
9.98468540910302));
#34787=CARTESIAN_POINT('Ctrl Pts',(-4.0173955002244,1.06847604194588,10.0191495270543));
#34788=CARTESIAN_POINT('Ctrl Pts',(-4.03860173661218,1.18514270861328,10.0244152737678));
#34789=CARTESIAN_POINT('Ctrl Pts',(-4.05902269361942,1.30000000000222,10.0200285275551));
#34790=CARTESIAN_POINT('Ctrl Pts',(-4.18327543477343,-1.3000000000001,9.81355715492352));
#34791=CARTESIAN_POINT('Ctrl Pts',(-4.15419431067351,-1.18514270861185,
9.82945370324904));
#34792=CARTESIAN_POINT('Ctrl Pts',(-4.12300938712133,-1.06847604194515,
9.83796172973357));
#34793=CARTESIAN_POINT('Ctrl Pts',(-4.04610577759482,-0.794772684000857,
9.84054800941627));
#34794=CARTESIAN_POINT('Ctrl Pts',(-3.98547441096753,-0.636309800095203,
9.81267820358621));
#34795=CARTESIAN_POINT('Ctrl Pts',(-3.91194208684675,-0.319434907277162,
9.7984430963628));
#34796=CARTESIAN_POINT('Ctrl Pts',(-3.87555616930008,-0.158333333333334,
9.78288741997211));
#34797=CARTESIAN_POINT('Ctrl Pts',(-3.85858039408216,0.158333333333336,
9.8081980387313));
#34798=CARTESIAN_POINT('Ctrl Pts',(-3.87752872335823,0.319434907277171,
9.84970799273135));
#34799=CARTESIAN_POINT('Ctrl Pts',(-3.91742329559321,0.636309800095213,
9.9141879212094));
#34800=CARTESIAN_POINT('Ctrl Pts',(-3.95944359784781,0.794772684000847,
9.96903623482389));
#34801=CARTESIAN_POINT('Ctrl Pts',(-4.0114028600779,1.06847604194588,10.0054193555547));
#34802=CARTESIAN_POINT('Ctrl Pts',(-4.03323521473105,1.18514270861328,10.0121574872712));
#34803=CARTESIAN_POINT('Ctrl Pts',(-4.05440868469828,1.30000000000222,10.0098848458672));
#34804=CARTESIAN_POINT('Ctrl Pts',(-4.17689145237611,-1.3000000000001,9.80301252814214));
#34805=CARTESIAN_POINT('Ctrl Pts',(-4.1465997387043,-1.18514270861185,9.81684487549646));
#34806=CARTESIAN_POINT('Ctrl Pts',(-4.11450022071243,-1.06847604194516,
9.82387604727132));
#34807=CARTESIAN_POINT('Ctrl Pts',(-4.03616752303527,-0.794772684000861,
9.82440738449327));
#34808=CARTESIAN_POINT('Ctrl Pts',(-3.97545993580296,-0.636309800095203,
9.79726188892626));
#34809=CARTESIAN_POINT('Ctrl Pts',(-3.9018874991181,-0.319434907277162,
9.78296702519706));
#34810=CARTESIAN_POINT('Ctrl Pts',(-3.86605396024536,-0.158333333333334,
9.76791040528507));
#34811=CARTESIAN_POINT('Ctrl Pts',(-3.84946804647695,0.158333333333336,
9.79281292514629));
#34812=CARTESIAN_POINT('Ctrl Pts',(-3.86849596672761,0.31943490727717,9.83315145538546));
#34813=CARTESIAN_POINT('Ctrl Pts',(-3.90873161425928,0.636309800095212,
9.89739816796892));
#34814=CARTESIAN_POINT('Ctrl Pts',(-3.950382362248,0.794772684000848,9.95203175065576));
#34815=CARTESIAN_POINT('Ctrl Pts',(-4.00371999356563,1.06847604194588,9.99054841316902));
#34816=CARTESIAN_POINT('Ctrl Pts',(-4.02649062745679,1.18514270861328,9.99874474446717));
#34817=CARTESIAN_POINT('Ctrl Pts',(-4.04894401099567,1.30000000000222,9.99846497104443));
#34818=CARTESIAN_POINT('Ctrl Pts',(-4.17047928941036,-1.30000000000009,
9.79249304649564));
#34819=CARTESIAN_POINT('Ctrl Pts',(-4.13894720136848,-1.18514270861185,
9.80429279693164));
#34820=CARTESIAN_POINT('Ctrl Pts',(-4.10591112926829,-1.06847604194515,
9.80987067792703));
#34821=CARTESIAN_POINT('Ctrl Pts',(-4.02611668982759,-0.794772684000857,
9.80838293578912));
#34822=CARTESIAN_POINT('Ctrl Pts',(-3.96535321334187,-0.636309800095201,
9.78194278190101));
#34823=CARTESIAN_POINT('Ctrl Pts',(-3.89170712988408,-0.319434907277161,
9.76762399515949));
#34824=CARTESIAN_POINT('Ctrl Pts',(-3.85635262368045,-0.158333333333334,
9.75314386280003));
#34825=CARTESIAN_POINT('Ctrl Pts',(-3.84017053254468,0.158333333333335,
9.77761910141739));
#34826=CARTESIAN_POINT('Ctrl Pts',(-3.85937613224551,0.319434907277171,
9.81667709579077));
#34827=CARTESIAN_POINT('Ctrl Pts',(-3.899992866501,0.636309800095212,9.8806411448506));
#34828=CARTESIAN_POINT('Ctrl Pts',(-3.9412868762951,0.794772684000845,9.93503778605955));
#34829=CARTESIAN_POINT('Ctrl Pts',(-3.9959273914875,1.06847604194587,9.97577138358011));
#34830=CARTESIAN_POINT('Ctrl Pts',(-4.01958056028507,1.18514270861328,9.98548958062305));
#34831=CARTESIAN_POINT('Ctrl Pts',(-4.04323504348396,1.30000000000222,9.98729390967078));
#34832=CARTESIAN_POINT('Ctrl Pts',(-4.1623027602077,-1.30000000000009,9.77952294110834));
#34833=CARTESIAN_POINT('Ctrl Pts',(-4.12916991535113,-1.18514270861185,
9.78883210821292));
#34834=CARTESIAN_POINT('Ctrl Pts',(-4.09501090828536,-1.06847604194515,
9.79253669957329));
#34835=CARTESIAN_POINT('Ctrl Pts',(-4.01372612849118,-0.794772684000858,
9.78814735555604));
#34836=CARTESIAN_POINT('Ctrl Pts',(-3.95376169659582,-0.636309800095203,
9.76163075512583));
#34837=CARTESIAN_POINT('Ctrl Pts',(-3.88005908306621,-0.319434907277162,
9.74724167966076));
#34838=CARTESIAN_POINT('Ctrl Pts',(-3.84471622657658,-0.158333333333334,
9.73414067785112));
#34839=CARTESIAN_POINT('Ctrl Pts',(-3.82837867217028,0.158333333333335,
9.75878967722972));
#34840=CARTESIAN_POINT('Ctrl Pts',(-3.84695230195744,0.319434907277168,
9.79712332573153));
#34841=CARTESIAN_POINT('Ctrl Pts',(-3.88825577889028,0.636309800095211,
9.86053179059021));
#34842=CARTESIAN_POINT('Ctrl Pts',(-3.9307976075957,0.794772684000848,9.91290040708799));
#34843=CARTESIAN_POINT('Ctrl Pts',(-3.98709463873616,1.06847604194588,9.95638684629109));
#34844=CARTESIAN_POINT('Ctrl Pts',(-4.01151951885904,1.18514270861328,9.96835168815166));
#34845=CARTESIAN_POINT('Ctrl Pts',(-4.03600038033461,1.30000000000221,9.97345770367308));
#34846=CARTESIAN_POINT('Ctrl Pts',(-4.15271715219705,-1.30000000000009,
9.76367829885413));
#34847=CARTESIAN_POINT('Ctrl Pts',(-4.11773142355429,-1.18514270861185,
9.76992275657636));
#34848=CARTESIAN_POINT('Ctrl Pts',(-4.08214402329409,-1.06847604194515,
9.77146808850168));
#34849=CARTESIAN_POINT('Ctrl Pts',(-3.99854002765769,-0.794772684000857,
9.764182193744));
#34850=CARTESIAN_POINT('Ctrl Pts',(-3.93818305842922,-0.636309800095199,
9.7390655135235));
#34851=CARTESIAN_POINT('Ctrl Pts',(-3.86437826392957,-0.319434907277159,
9.72463233575177));
#34852=CARTESIAN_POINT('Ctrl Pts',(-3.83016010562027,-0.158333333333333,
9.71196014514568));
#34853=CARTESIAN_POINT('Ctrl Pts',(-3.81435573406753,0.158333333333335,
9.73603306311532));
#34854=CARTESIAN_POINT('Ctrl Pts',(-3.83272201883899,0.319434907277169,
9.77293474300738));
#34855=CARTESIAN_POINT('Ctrl Pts',(-3.87443120456167,0.636309800095209,
9.83608379687782));
#34856=CARTESIAN_POINT('Ctrl Pts',(-3.91637856299569,0.794772684000842,
9.88815189746707));
#34857=CARTESIAN_POINT('Ctrl Pts',(-3.97509502513964,1.06847604194587,9.93448054688383));
#34858=CARTESIAN_POINT('Ctrl Pts',(-4.00117540355945,1.18514270861327,9.94838567794813));
#34859=CARTESIAN_POINT('Ctrl Pts',(-4.02791997959621,1.30000000000221,9.95614198438979));
#34860=CARTESIAN_POINT('Ctrl Pts',(-4.14458288155458,-1.30000000000009,
9.75064115448924));
#34861=CARTESIAN_POINT('Ctrl Pts',(-4.10811453968855,-1.18514270861185,
9.75424928515064));
#34862=CARTESIAN_POINT('Ctrl Pts',(-4.07135896780956,-1.06847604194515,
9.75396300487519));
#34863=CARTESIAN_POINT('Ctrl Pts',(-3.98578268505204,-0.794772684000857,
9.74430477183034));
#34864=CARTESIAN_POINT('Ctrl Pts',(-3.92497542566649,-0.636309800095201,
9.72052245946643));
#34865=CARTESIAN_POINT('Ctrl Pts',(-3.85084161620007,-0.319434907277161,
9.70632290465302));
#34866=CARTESIAN_POINT('Ctrl Pts',(-3.81721658744817,-0.158333333333333,
9.69437078927507));
#34867=CARTESIAN_POINT('Ctrl Pts',(-3.80187495488852,0.158333333333335,
9.71792536556004));
#34868=CARTESIAN_POINT('Ctrl Pts',(-3.82021028003475,0.319434907277167,
9.75343912820627));
#34869=CARTESIAN_POINT('Ctrl Pts',(-3.86298851307109,0.636309800095209,
9.81560325584252));
#34870=CARTESIAN_POINT('Ctrl Pts',(-3.90596293721407,0.794772684000845,
9.86587151787597));
#34871=CARTESIAN_POINT('Ctrl Pts',(-3.96639767861555,1.06847604194587,9.91489479795498));
#34872=CARTESIAN_POINT('Ctrl Pts',(-3.99329518192105,1.18514270861328,9.93100668664934));
#34873=CARTESIAN_POINT('Ctrl Pts',(-4.02093022830713,1.30000000000221,9.94201010258334));
#34874=CARTESIAN_POINT('Ctrl Pts',(-4.13792080370513,-1.30000000000009,
9.7403656665557));
#34875=CARTESIAN_POINT('Ctrl Pts',(-4.09991568165613,-1.18514270861185,
9.7422691668776));
#34876=CARTESIAN_POINT('Ctrl Pts',(-4.06208162057071,-1.06847604194515,
9.74068441285067));
#34877=CARTESIAN_POINT('Ctrl Pts',(-3.97507255583187,-0.794772684000857,
9.72896474865087));
#34878=CARTESIAN_POINT('Ctrl Pts',(-3.91499224411171,-0.636309800095201,
9.70500070162394));
#34879=CARTESIAN_POINT('Ctrl Pts',(-3.84087419871896,-0.31943490727716,
9.69067377855575));
#34880=CARTESIAN_POINT('Ctrl Pts',(-3.80740469694953,-0.158333333333333,
9.67968200748737));
#34881=CARTESIAN_POINT('Ctrl Pts',(-3.79197211150342,0.158333333333335,
9.70333725927779));
#34882=CARTESIAN_POINT('Ctrl Pts',(-3.80990338042646,0.319434907277168,
9.73816695474585));
#34883=CARTESIAN_POINT('Ctrl Pts',(-3.85280155659604,0.636309800095209,
9.80030583152426));
#34884=CARTESIAN_POINT('Ctrl Pts',(-3.89559684856876,0.794772684000844,
9.85012092965609));
#34885=CARTESIAN_POINT('Ctrl Pts',(-3.9576382974083,1.06847604194587,9.90105238271874));
#34886=CARTESIAN_POINT('Ctrl Pts',(-3.98560809415924,1.18514270861328,9.91850102054971));
#34887=CARTESIAN_POINT('Ctrl Pts',(-4.01469224332062,1.30000000000221,9.93135195737708));
#34888=CARTESIAN_POINT('Ctrl Pts',(-4.1278777586158,-1.30000000000009,9.7250220110376));
#34889=CARTESIAN_POINT('Ctrl Pts',(-4.08773437020547,-1.18514270861184,
9.72417262169841));
#34890=CARTESIAN_POINT('Ctrl Pts',(-4.04832068672469,-1.06847604194515,
9.72059219835672));
#34891=CARTESIAN_POINT('Ctrl Pts',(-3.95895295756798,-0.794772684000853,
9.70601146928899));
#34892=CARTESIAN_POINT('Ctrl Pts',(-3.8992301361605,-0.636309800095199,
9.6826078545982));
#34893=CARTESIAN_POINT('Ctrl Pts',(-3.82480580924965,-0.31943490727716,
9.66846543483889));
#34894=CARTESIAN_POINT('Ctrl Pts',(-3.79137440572589,-0.158333333333333,
9.65913160969459));
#34895=CARTESIAN_POINT('Ctrl Pts',(-3.7765073752783,0.158333333333335,9.68215845182108));
#34896=CARTESIAN_POINT('Ctrl Pts',(-3.79520088663898,0.319434907277168,
9.71442671474825));
#34897=CARTESIAN_POINT('Ctrl Pts',(-3.83907909760253,0.636309800095208,
9.77566137492616));
#34898=CARTESIAN_POINT('Ctrl Pts',(-3.88150208085316,0.794772684000841,
9.82497614627297));
#34899=CARTESIAN_POINT('Ctrl Pts',(-3.94580247883527,1.06847604194587,9.87893518081619));
#34900=CARTESIAN_POINT('Ctrl Pts',(-3.97522304931586,1.18514270861327,9.89854771494412));
#34901=CARTESIAN_POINT('Ctrl Pts',(-4.00623093055504,1.30000000000221,9.91441591652541));
#34902=CARTESIAN_POINT('Ctrl Pts',(-4.11635470812674,-1.3000000000001,9.70687190739252));
#34903=CARTESIAN_POINT('Ctrl Pts',(-4.07409459096131,-1.18514270861185,
9.70235142307796));
#34904=CARTESIAN_POINT('Ctrl Pts',(-4.03300344320846,-1.06847604194515,
9.6962394264141));
#34905=CARTESIAN_POINT('Ctrl Pts',(-3.94077522483799,-0.794772684000855,
9.67844277951203));
#34906=CARTESIAN_POINT('Ctrl Pts',(-3.88026343239008,-0.636309800095201,
9.65713349321762));
#34907=CARTESIAN_POINT('Ctrl Pts',(-3.80545909140476,-0.319434907277161,
9.64323923547767));
#34908=CARTESIAN_POINT('Ctrl Pts',(-3.77335449162494,-0.158333333333333,
9.63435059380748));
#34909=CARTESIAN_POINT('Ctrl Pts',(-3.75885308043993,0.158333333333335,
9.65694128325831));
#34910=CARTESIAN_POINT('Ctrl Pts',(-3.77669857829229,0.319434907277168,
9.68815090112606));
#34911=CARTESIAN_POINT('Ctrl Pts',(-3.82147102231926,0.636309800095209,
9.74861015317067));
#34912=CARTESIAN_POINT('Ctrl Pts',(-3.86480586979095,0.794772684000845,
9.7958608588833));
#34913=CARTESIAN_POINT('Ctrl Pts',(-3.93202952355851,1.06847604194587,9.85304439935273));
#34914=CARTESIAN_POINT('Ctrl Pts',(-3.96309385828612,1.18514270861328,9.87524035766234));
#34915=CARTESIAN_POINT('Ctrl Pts',(-3.99612389890713,1.30000000000221,9.89487963847128));
#34916=CARTESIAN_POINT('Ctrl Pts',(-4.10202300360559,-1.30000000000009,
9.68751099507706));
#34917=CARTESIAN_POINT('Ctrl Pts',(-4.05666990056074,-1.18514270861184,
9.67958214782389));
#34918=CARTESIAN_POINT('Ctrl Pts',(-4.01334637963241,-1.06847604194515,
9.67094158349285));
#34919=CARTESIAN_POINT('Ctrl Pts',(-3.91794912015298,-0.794772684000855,
9.64933594252076));
#34920=CARTESIAN_POINT('Ctrl Pts',(-3.85840997143452,-0.636309800095199,
9.62819587095804));
#34921=CARTESIAN_POINT('Ctrl Pts',(-3.78334012526085,-0.31943490727716,
9.6143824976442));
#34922=CARTESIAN_POINT('Ctrl Pts',(-3.75139511139691,-0.158333333333333,
9.60762197008548));
#34923=CARTESIAN_POINT('Ctrl Pts',(-3.73708422400504,0.158333333333335,
9.62997188908506));
#34924=CARTESIAN_POINT('Ctrl Pts',(-3.75477217548896,0.319434907277168,
9.65900825018191));
#34925=CARTESIAN_POINT('Ctrl Pts',(-3.80058213678986,0.636309800095208,
9.71849770600095));
#34926=CARTESIAN_POINT('Ctrl Pts',(-3.84417322803187,0.794772684000842,
9.764189669864));
#34927=CARTESIAN_POINT('Ctrl Pts',(-3.9148570456614,1.06847604194587,9.824923839085));
#34928=CARTESIAN_POINT('Ctrl Pts',(-3.94802895223982,1.18514270861327,9.84983730924623));
#34929=CARTESIAN_POINT('Ctrl Pts',(-3.98377635983831,1.30000000000221,9.8733746781356));
#34930=CARTESIAN_POINT('Ctrl Pts',(-4.09223550484063,-1.30000000000009,
9.67180067703011));
#34931=CARTESIAN_POINT('Ctrl Pts',(-4.04492506092978,-1.18514270861184,
9.66088402866375));
#34932=CARTESIAN_POINT('Ctrl Pts',(-4.00004421825906,-1.06847604194515,
9.65020916578641));
#34933=CARTESIAN_POINT('Ctrl Pts',(-3.90197335821266,-0.794772684000854,
9.62610666988942));
#34934=CARTESIAN_POINT('Ctrl Pts',(-3.84178364041155,-0.636309800095198,
9.60674608144195));
#34935=CARTESIAN_POINT('Ctrl Pts',(-3.76608130219754,-0.319434907277159,
9.59351969773874));
#34936=CARTESIAN_POINT('Ctrl Pts',(-3.73471560689843,-0.158333333333333,
9.58781315447167));
#34937=CARTESIAN_POINT('Ctrl Pts',(-3.72083677057423,0.158333333333335,
9.60964344590414));
#34938=CARTESIAN_POINT('Ctrl Pts',(-3.73860850554392,0.319434907277169,
9.63679929512494));
#34939=CARTESIAN_POINT('Ctrl Pts',(-3.78546038158528,0.636309800095208,
9.69526845063128));
#34940=CARTESIAN_POINT('Ctrl Pts',(-3.82955687974671,0.794772684000841,
9.73947794767306));
#34941=CARTESIAN_POINT('Ctrl Pts',(-3.90259112333981,1.06847604194587,9.80315290720977));
#34942=CARTESIAN_POINT('Ctrl Pts',(-3.93709699733448,1.18514270861327,9.83037577538033));
#34943=CARTESIAN_POINT('Ctrl Pts',(-3.97449492745768,1.30000000000221,9.85725898112772));
#34944=CARTESIAN_POINT('Ctrl Pts',(-4.08088288391462,-1.30000000000009,
9.65800792817637));
#34945=CARTESIAN_POINT('Ctrl Pts',(-4.0310277457008,-1.18514270861184,9.6448068787467));
#34946=CARTESIAN_POINT('Ctrl Pts',(-3.98431745788211,-1.06847604194514,
9.63242188925164));
#34947=CARTESIAN_POINT('Ctrl Pts',(-3.88367258219778,-0.794772684000849,
9.60569534761062));
#34948=CARTESIAN_POINT('Ctrl Pts',(-3.82416264746573,-0.636309800095196,
9.58651222178451));
#34949=CARTESIAN_POINT('Ctrl Pts',(-3.74862535627239,-0.319434907277159,
9.57290001362148));
#34950=CARTESIAN_POINT('Ctrl Pts',(-3.71821062371238,-0.158333333333333,
9.5677937300466));
#34951=CARTESIAN_POINT('Ctrl Pts',(-3.70451747313622,0.158333333333334,
9.58937323654366));
#34952=CARTESIAN_POINT('Ctrl Pts',(-3.72141492809999,0.319434907277168,
9.61578986157383));
#34953=CARTESIAN_POINT('Ctrl Pts',(-3.76870201691248,0.636309800095208,
9.67390624050485));
#34954=CARTESIAN_POINT('Ctrl Pts',(-3.81278249322028,0.79477268400084,9.71712672772544));
#34955=CARTESIAN_POINT('Ctrl Pts',(-3.88891793965976,1.06847604194587,9.78289475248831));
#34956=CARTESIAN_POINT('Ctrl Pts',(-3.92540934858402,1.18514270861327,9.81171155206745));
#34957=CARTESIAN_POINT('Ctrl Pts',(-3.96543595276512,1.30000000000221,9.84087661025131));
#34958=CARTESIAN_POINT('Ctrl Pts',(-4.07272838886402,-1.30000000000009,
9.64488009164317));
#34959=CARTESIAN_POINT('Ctrl Pts',(-4.02104634242638,-1.18514270861184,
9.62941756709542));
#34960=CARTESIAN_POINT('Ctrl Pts',(-3.97289920341682,-1.06847604194515,
9.61550255020163));
#34961=CARTESIAN_POINT('Ctrl Pts',(-3.86983602381723,-0.794772684000853,
9.58693112974593));
#34962=CARTESIAN_POINT('Ctrl Pts',(-3.80992709147984,-0.636309800095198,
9.56908533013396));
#34963=CARTESIAN_POINT('Ctrl Pts',(-3.73373118466259,-0.31943490727716,
9.55613499866793));
#34964=CARTESIAN_POINT('Ctrl Pts',(-3.70354447410378,-0.158333333333333,
9.55222294139156));
#34965=CARTESIAN_POINT('Ctrl Pts',(-3.69014793205364,0.158333333333334,
9.5734258816163));
#34966=CARTESIAN_POINT('Ctrl Pts',(-3.70716886738543,0.319434907277167,
9.59816262664611));
#34967=CARTESIAN_POINT('Ctrl Pts',(-3.75560692722669,0.636309800095207,
9.65507229373653));
#34968=CARTESIAN_POINT('Ctrl Pts',(-3.80062603915456,0.794772684000841,
9.69646175637529));
#34969=CARTESIAN_POINT('Ctrl Pts',(-3.87879994236377,1.06847604194587,9.76458752472658));
#34970=CARTESIAN_POINT('Ctrl Pts',(-3.91632666232639,1.18514270861327,9.79541903485025));
#34971=CARTESIAN_POINT('Ctrl Pts',(-3.95754151618084,1.30000000000221,9.82759293428673));
#34972=CARTESIAN_POINT('Ctrl Pts',(-4.06138621253067,-1.30000000000009,
9.63106202969797));
#34973=CARTESIAN_POINT('Ctrl Pts',(-4.00730211428524,-1.18514270861184,
9.61313433541102));
#34974=CARTESIAN_POINT('Ctrl Pts',(-3.95736582749986,-1.06847604194515,
9.59745646095828));
#34975=CARTESIAN_POINT('Ctrl Pts',(-3.85158528954522,-0.794772684000852,
9.56643496851635));
#34976=CARTESIAN_POINT('Ctrl Pts',(-3.79178142684599,-0.636309800095198,
9.54948273309652));
#34977=CARTESIAN_POINT('Ctrl Pts',(-3.71552477875022,-0.31943490727716,
9.53642279036497));
#34978=CARTESIAN_POINT('Ctrl Pts',(-3.68634494508279,-0.158333333333333,
9.5330333244766));
#34979=CARTESIAN_POINT('Ctrl Pts',(-3.67337150255953,0.158333333333334,
9.55369078341368));
#34980=CARTESIAN_POINT('Ctrl Pts',(-3.68994656139196,0.319434907277167,
9.57716760640096));
#34981=CARTESIAN_POINT('Ctrl Pts',(-3.73902629165065,0.636309800095207,
9.6334665619966));
#34982=CARTESIAN_POINT('Ctrl Pts',(-3.78402389339273,0.794772684000841,
9.67387788185577));
#34983=CARTESIAN_POINT('Ctrl Pts',(-3.86502638086352,1.06847604194587,9.74440089113378));
#34984=CARTESIAN_POINT('Ctrl Pts',(-3.90434124164542,1.18514270861327,9.77704838131755));
#34985=CARTESIAN_POINT('Ctrl Pts',(-3.94790798782096,1.30000000000221,9.81181656410356));
#34986=CARTESIAN_POINT('Ctrl Pts',(-4.04716422159609,-1.30000000000008,
9.61149186781036));
#34987=CARTESIAN_POINT('Ctrl Pts',(-3.9900803286236,-1.18514270861184,9.59001943537044));
#34988=CARTESIAN_POINT('Ctrl Pts',(-3.9378059472672,-1.06847604194515,9.57193282854236));
#34989=CARTESIAN_POINT('Ctrl Pts',(-3.8281526028524,-0.794772684000852,
9.53797108305162));
#34990=CARTESIAN_POINT('Ctrl Pts',(-3.76783820314362,-0.636309800095198,
9.52306019173905));
#34991=CARTESIAN_POINT('Ctrl Pts',(-3.69064922620234,-0.31943490727716,
9.51093114831833));
#34992=CARTESIAN_POINT('Ctrl Pts',(-3.66194871726299,-0.158333333333333,
9.50931618908867));
#34993=CARTESIAN_POINT('Ctrl Pts',(-3.64945527695434,0.158333333333334,
9.52932029129036));
#34994=CARTESIAN_POINT('Ctrl Pts',(-3.66631284837025,0.319434907277167,
9.54995749515016));
#34995=CARTESIAN_POINT('Ctrl Pts',(-3.71672855962466,0.636309800095207,
9.60483342758972));
#34996=CARTESIAN_POINT('Ctrl Pts',(-3.7618242424883,0.794772684000842,9.64385514916113));
#34997=CARTESIAN_POINT('Ctrl Pts',(-3.8465484654073,1.06847604194587,9.71762767022338));
#34998=CARTESIAN_POINT('Ctrl Pts',(-3.88814294340621,1.18514270861327,9.75280796524565));
#34999=CARTESIAN_POINT('Ctrl Pts',(-3.93465792264413,1.30000000000221,9.79123516446356));
#35000=CARTESIAN_POINT('Ctrl Pts',(-4.02999794901952,-1.30000000000008,
9.59094278729835));
#35001=CARTESIAN_POINT('Ctrl Pts',(-3.96900965522733,-1.18514270861183,
9.5661695695801));
#35002=CARTESIAN_POINT('Ctrl Pts',(-3.91382227090955,-1.06847604194514,
9.54574039801195));
#35003=CARTESIAN_POINT('Ctrl Pts',(-3.79972963429092,-0.794772684000849,
9.508580540478));
#35004=CARTESIAN_POINT('Ctrl Pts',(-3.73982716968739,-0.636309800095198,
9.4946692715688));
#35005=CARTESIAN_POINT('Ctrl Pts',(-3.66196688951287,-0.319434907277161,
9.48314438624894));
#35006=CARTESIAN_POINT('Ctrl Pts',(-3.633791005323,-0.158333333333332,9.4836530037158));
#35007=CARTESIAN_POINT('Ctrl Pts',(-3.62157560849388,0.158333333333334,
9.50325490140512));
#35008=CARTESIAN_POINT('Ctrl Pts',(-3.63788921901196,0.319434907277164,
9.52169048774121));
#35009=CARTESIAN_POINT('Ctrl Pts',(-3.6901483289376,0.636309800095204,9.57448270236182));
#35010=CARTESIAN_POINT('Ctrl Pts',(-3.73668867689305,0.794772684000843,
9.61023444256769));
#35011=CARTESIAN_POINT('Ctrl Pts',(-3.82637409362723,1.06847604194587,9.68670843100664));
#35012=CARTESIAN_POINT('Ctrl Pts',(-3.87074606138443,1.18514270861327,9.72449403600665));
#35013=CARTESIAN_POINT('Ctrl Pts',(-3.92066850316669,1.3000000000022,9.76696249005188));
#35014=CARTESIAN_POINT('Ctrl Pts',(-4.01715577671309,-1.30000000000008,
9.57427610753466));
#35015=CARTESIAN_POINT('Ctrl Pts',(-3.95336640312922,-1.18514270861184,
9.54660857832973));
#35016=CARTESIAN_POINT('Ctrl Pts',(-3.89592815820484,-1.06847604194514,
9.52433493947444));
#35017=CARTESIAN_POINT('Ctrl Pts',(-3.77790669969032,-0.794772684000849,
9.48533934364431));
#35018=CARTESIAN_POINT('Ctrl Pts',(-3.71674723482175,-0.636309800095197,
9.47438761560753));
#35019=CARTESIAN_POINT('Ctrl Pts',(-3.63816837785436,-0.319434907277159,
9.46357932395661));
#35020=CARTESIAN_POINT('Ctrl Pts',(-3.61155232655921,-0.158333333333332,
9.46411500242012));
#35021=CARTESIAN_POINT('Ctrl Pts',(-3.59992805160763,0.158333333333334,
9.48285863809054));
#35022=CARTESIAN_POINT('Ctrl Pts',(-3.6157130109624,0.319434907277166,9.49975938519163));
#35023=CARTESIAN_POINT('Ctrl Pts',(-3.66899840014624,0.636309800095205,
9.55140980597997));
#35024=CARTESIAN_POINT('Ctrl Pts',(-3.71596769087412,0.79477268400084,9.58543622672668));
#35025=CARTESIAN_POINT('Ctrl Pts',(-3.80909149309595,1.06847604194587,9.66450059946136));
#35026=CARTESIAN_POINT('Ctrl Pts',(-3.85552438516391,1.18514270861327,9.70442591341075));
#35027=CARTESIAN_POINT('Ctrl Pts',(-3.9080803258948,1.3000000000022,9.75005250397632));
#35028=CARTESIAN_POINT('Ctrl Pts',(-4.01049046738461,-1.30000000000008,
9.56625472662844));
#35029=CARTESIAN_POINT('Ctrl Pts',(-3.94503884995572,-1.18514270861183,
9.53748069470923));
#35030=CARTESIAN_POINT('Ctrl Pts',(-3.88636334134026,-1.06847604194514,
9.514425957823));
#35031=CARTESIAN_POINT('Ctrl Pts',(-3.76646534535823,-0.79477268400085,
9.47437761919877));
#35032=CARTESIAN_POINT('Ctrl Pts',(-3.70553200215322,-0.636309800095198,
9.46373730882956));
#35033=CARTESIAN_POINT('Ctrl Pts',(-3.62662698637735,-0.319434907277161,
9.45326350530048));
#35034=CARTESIAN_POINT('Ctrl Pts',(-3.60013762995176,-0.158333333333332,
9.4547533903638));
#35035=CARTESIAN_POINT('Ctrl Pts',(-3.58856078912183,0.158333333333334,
9.47341021636554));
#35036=CARTESIAN_POINT('Ctrl Pts',(-3.60417149421509,0.319434907277165,
9.48937813042208));
#35037=CARTESIAN_POINT('Ctrl Pts',(-3.65807315704533,0.636309800095205,
9.54029687660626));
#35038=CARTESIAN_POINT('Ctrl Pts',(-3.70532264680744,0.794772684000842,
9.57334189081042));
#35039=CARTESIAN_POINT('Ctrl Pts',(-3.8004913239218,1.06847604194587,9.65331202159248));
#35040=CARTESIAN_POINT('Ctrl Pts',(-3.84814442854337,1.18514270861327,9.69409179552363));
#35041=CARTESIAN_POINT('Ctrl Pts',(-3.90225564381061,1.30000000000221,9.74103523695565));
#35042=CARTESIAN_POINT('Ctrl Pts',(-4.00659335599282,-1.30000000000008,
9.56178696274011));
#35043=CARTESIAN_POINT('Ctrl Pts',(-3.94028249235065,-1.18514270861184,
9.53226304267891));
#35044=CARTESIAN_POINT('Ctrl Pts',(-3.88093929508802,-1.06847604194514,
9.50871543648836));
#35045=CARTESIAN_POINT('Ctrl Pts',(-3.75994134105903,-0.794772684000851,
9.46812223610436));
#35046=CARTESIAN_POINT('Ctrl Pts',(-3.69883896773334,-0.636309800095198,
9.45809388202234));
#35047=CARTESIAN_POINT('Ctrl Pts',(-3.61975297932188,-0.31943490727716,
9.44780401461268));
#35048=CARTESIAN_POINT('Ctrl Pts',(-3.59359330179776,-0.158333333333333,
9.44945850523304));
#35049=CARTESIAN_POINT('Ctrl Pts',(-3.58213377403886,0.158333333333334,
9.46793215917097));
#35050=CARTESIAN_POINT('Ctrl Pts',(-3.59755411097818,0.319434907277166,
9.48349796950585));
#35051=CARTESIAN_POINT('Ctrl Pts',(-3.65183089703969,0.636309800095206,
9.53397032962117));
#35052=CARTESIAN_POINT('Ctrl Pts',(-3.69933866067861,0.794772684000842,
9.56633036465978));
#35053=CARTESIAN_POINT('Ctrl Pts',(-3.7956733638959,1.06847604194587,9.64681194796218));
#35054=CARTESIAN_POINT('Ctrl Pts',(-3.84400078616579,1.18514270861327,9.68810289381018));
#35055=CARTESIAN_POINT('Ctrl Pts',(-3.89895590723521,1.30000000000221,9.73584729023102));
#35056=CARTESIAN_POINT('Ctrl Pts',(-4.00072166766443,-1.30000000000008,
9.555143627305));
#35057=CARTESIAN_POINT('Ctrl Pts',(-3.93325540212071,-1.18514270861184,
9.52435152354733));
#35058=CARTESIAN_POINT('Ctrl Pts',(-3.87297212247522,-1.06847604194514,
9.50000972486456));
#35059=CARTESIAN_POINT('Ctrl Pts',(-3.75029982124167,-0.79477268400085,
9.4586767954494));
#35060=CARTESIAN_POINT('Ctrl Pts',(-3.68854925872017,-0.636309800095198,
9.450112526269));
#35061=CARTESIAN_POINT('Ctrl Pts',(-3.60918410847569,-0.319434907277161,
9.44009345725221));
#35062=CARTESIAN_POINT('Ctrl Pts',(-3.58382081815314,-0.158333333333333,
9.44152662577802));
#35063=CARTESIAN_POINT('Ctrl Pts',(-3.57266363030392,0.158333333333334,
9.45954457671088));
#35064=CARTESIAN_POINT('Ctrl Pts',(-3.58775278672523,0.319434907277166,
9.47460764988021));
#35065=CARTESIAN_POINT('Ctrl Pts',(-3.64259283135499,0.636309800095206,
9.52442759976224));
#35066=CARTESIAN_POINT('Ctrl Pts',(-3.69049519762091,0.794772684000843,
9.55577179754062));
#35067=CARTESIAN_POINT('Ctrl Pts',(-3.78853507143873,1.06847604194587,9.63704397580051));
#35068=CARTESIAN_POINT('Ctrl Pts',(-3.83784386572028,1.18514270861327,9.67911301725969));
#35069=CARTESIAN_POINT('Ctrl Pts',(-3.89402362564286,1.30000000000221,9.72807138564023));
#35070=CARTESIAN_POINT('Ctrl Pts',(-3.99198996060069,-1.30000000000008,
9.54496247330596));
#35071=CARTESIAN_POINT('Ctrl Pts',(-3.92239848053823,-1.18514270861184,
9.51258568427901));
#35072=CARTESIAN_POINT('Ctrl Pts',(-3.86045956466931,-1.06847604194514,
9.48722049547628));
#35073=CARTESIAN_POINT('Ctrl Pts',(-3.73504723235175,-0.794772684000852,
9.44482003423708));
#35074=CARTESIAN_POINT('Ctrl Pts',(-3.67258059959666,-0.636309800095198,
9.43806097931972));
#35075=CARTESIAN_POINT('Ctrl Pts',(-3.59326729399712,-0.31943490727716,
9.42779540032309));
#35076=CARTESIAN_POINT('Ctrl Pts',(-3.56992252153975,-0.158333333333333,
9.42792332139754));
#35077=CARTESIAN_POINT('Ctrl Pts',(-3.55915076488227,0.158333333333334,
9.4453691550592));
#35078=CARTESIAN_POINT('Ctrl Pts',(-3.57280337312768,0.319434907277167,
9.46085721877722));
#35079=CARTESIAN_POINT('Ctrl Pts',(-3.62797633392986,0.636309800095207,
9.51038597519395));
#35080=CARTESIAN_POINT('Ctrl Pts',(-3.67645485979168,0.794772684000843,
9.54018297807693));
#35081=CARTESIAN_POINT('Ctrl Pts',(-3.77705435099628,1.06847604194587,9.62285502829093));
#35082=CARTESIAN_POINT('Ctrl Pts',(-3.8278900846652,1.18514270861327,9.66616756632872));
#35083=CARTESIAN_POINT('Ctrl Pts',(-3.88601575983895,1.30000000000221,9.7170069751679));
#35084=CARTESIAN_POINT('Ctrl Pts',(-3.98223602054929,-1.30000000000008,
9.53389065551683));
#35085=CARTESIAN_POINT('Ctrl Pts',(-3.91009970729482,-1.18514270861184,
9.50037021018406));
#35086=CARTESIAN_POINT('Ctrl Pts',(-3.84640729865907,-1.06847604194515,
9.47403296621852));
#35087=CARTESIAN_POINT('Ctrl Pts',(-3.71877220195439,-0.794772684000855,
9.42978329606333));
#35088=CARTESIAN_POINT('Ctrl Pts',(-3.657624226043,-0.636309800095198,9.42216489294489));
#35089=CARTESIAN_POINT('Ctrl Pts',(-3.57877337913983,-0.31943490727716,
9.41120306132792));
#35090=CARTESIAN_POINT('Ctrl Pts',(-3.55642229010766,-0.158333333333333,
9.41156642016226));
#35091=CARTESIAN_POINT('Ctrl Pts',(-3.54533915517231,0.158333333333334,
9.42940478405905));
#35092=CARTESIAN_POINT('Ctrl Pts',(-3.55719468008065,0.319434907277166,
9.44570670973183));
#35093=CARTESIAN_POINT('Ctrl Pts',(-3.61227313969613,0.636309800095206,
9.49539348245401));
#35094=CARTESIAN_POINT('Ctrl Pts',(-3.66122310062954,0.794772684000842,
9.52357900580051));
#35095=CARTESIAN_POINT('Ctrl Pts',(-3.76434798221053,1.06847604194587,9.60775523228691));
#35096=CARTESIAN_POINT('Ctrl Pts',(-3.81675088661188,1.18514270861327,9.65234746810249));
#35097=CARTESIAN_POINT('Ctrl Pts',(-3.87691775533148,1.30000000000221,9.70509517032415));
#35098=CARTESIAN_POINT('Ctrl Pts',(-3.97422670435764,-1.30000000000008,
9.52527149172315));
#35099=CARTESIAN_POINT('Ctrl Pts',(-3.89993944215733,-1.18514270861184,
9.49074311189192));
#35100=CARTESIAN_POINT('Ctrl Pts',(-3.83481605433959,-1.06847604194514,
9.46345282333785));
#35101=CARTESIAN_POINT('Ctrl Pts',(-3.70553838364206,-0.794772684000852,
9.41712823619988));
#35102=CARTESIAN_POINT('Ctrl Pts',(-3.64587798071845,-0.636309800095197,
9.40803695520255));
#35103=CARTESIAN_POINT('Ctrl Pts',(-3.56772851893399,-0.319434907277159,
9.3959004776643));
#35104=CARTESIAN_POINT('Ctrl Pts',(-3.54619807190222,-0.158333333333333,
9.39649432519919));
#35105=CARTESIAN_POINT('Ctrl Pts',(-3.53514505713312,0.158333333333334,
9.41426901412984));
#35106=CARTESIAN_POINT('Ctrl Pts',(-3.54608006064357,0.319434907277166,
9.43043728191244));
#35107=CARTESIAN_POINT('Ctrl Pts',(-3.60078328750133,0.636309800095205,
9.48084206052464));
#35108=CARTESIAN_POINT('Ctrl Pts',(-3.64893849711766,0.794772684000841,
9.50956420724531));
#35109=CARTESIAN_POINT('Ctrl Pts',(-3.75380923964106,1.06847604194587,9.59573353455122));
#35110=CARTESIAN_POINT('Ctrl Pts',(-3.80754380960878,1.18514270861327,9.64145231986177));
#35111=CARTESIAN_POINT('Ctrl Pts',(-3.86961829094969,1.30000000000221,9.69559038158027));
#35112=CARTESIAN_POINT('Ctrl Pts',(-3.9658917442215,-1.30000000000008,9.51663189767499));
#35113=CARTESIAN_POINT('Ctrl Pts',(-3.88867313305062,-1.18514270861184,
9.4816967127887));
#35114=CARTESIAN_POINT('Ctrl Pts',(-3.82176442120232,-1.06847604194515,
9.45367222838924));
#35115=CARTESIAN_POINT('Ctrl Pts',(-3.69100984171424,-0.794772684000854,
9.40489516375309));
#35116=CARTESIAN_POINT('Ctrl Pts',(-3.63472860148631,-0.636309800095199,
9.39236816688827));
#35117=CARTESIAN_POINT('Ctrl Pts',(-3.55824395824535,-0.31943490727716,
9.37820427155903));
#35118=CARTESIAN_POINT('Ctrl Pts',(-3.53752962997678,-0.158333333333333,
9.3794112337313));
#35119=CARTESIAN_POINT('Ctrl Pts',(-3.52653899124765,0.158333333333334,
9.39711672986148));
#35120=CARTESIAN_POINT('Ctrl Pts',(-3.53661209047723,0.319434907277166,
9.41279812490356));
#35121=CARTESIAN_POINT('Ctrl Pts',(-3.58999787159868,0.636309800095206,
9.46469129414753));
#35122=CARTESIAN_POINT('Ctrl Pts',(-3.63546698501272,0.794772684000843,
9.49566253282961));
#35123=CARTESIAN_POINT('Ctrl Pts',(-3.74183138047937,1.06847604194587,9.58429741893322));
#35124=CARTESIAN_POINT('Ctrl Pts',(-3.79719329321463,1.18514270861327,9.63104264461239));
#35125=CARTESIAN_POINT('Ctrl Pts',(-3.86187591307676,1.30000000000221,9.68616633802254));
#35126=CARTESIAN_POINT('Ctrl Pts',(-3.9607311993876,-1.30000000000008,9.50955037962429));
#35127=CARTESIAN_POINT('Ctrl Pts',(-3.88225168772289,-1.18514270861184,
9.47466234423755));
#35128=CARTESIAN_POINT('Ctrl Pts',(-3.81472938981739,-1.06847604194514,
9.44635463975158));
#35129=CARTESIAN_POINT('Ctrl Pts',(-3.68405272963316,-0.794772684000851,
9.39616006022359));
#35130=CARTESIAN_POINT('Ctrl Pts',(-3.63042937353999,-0.636309800095197,
9.38108392494785));
#35131=CARTESIAN_POINT('Ctrl Pts',(-3.55544568811449,-0.319434907277159,
9.36542695146836));
#35132=CARTESIAN_POINT('Ctrl Pts',(-3.53503780515506,-0.158333333333333,
9.36693889716871));
#35133=CARTESIAN_POINT('Ctrl Pts',(-3.52419820399014,0.158333333333334,
9.38451178833638));
#35134=CARTESIAN_POINT('Ctrl Pts',(-3.53420574803466,0.319434907277167,
9.39971616479935));
#35135=CARTESIAN_POINT('Ctrl Pts',(-3.58621520078905,0.636309800095206,
9.45291262168402));
#35136=CARTESIAN_POINT('Ctrl Pts',(-3.62884548279216,0.79477268400084,9.48638184647067));
#35137=CARTESIAN_POINT('Ctrl Pts',(-3.73516370162499,1.06847604194587,9.57640799112453));
#35138=CARTESIAN_POINT('Ctrl Pts',(-3.79118274870548,1.18514270861327,9.62344798197328));
#35139=CARTESIAN_POINT('Ctrl Pts',(-3.85719962541184,1.30000000000221,9.67855898144743));
#35140=CARTESIAN_POINT('Ctrl Pts',(-3.95827679071521,-1.30000000000008,
9.50436744488838));
#35141=CARTESIAN_POINT('Ctrl Pts',(-3.87988594951763,-1.18514270861184,
9.46962156082299));
#35142=CARTESIAN_POINT('Ctrl Pts',(-3.8125890784605,-1.06847604194514,9.44126870438154));
#35143=CARTESIAN_POINT('Ctrl Pts',(-3.68274913399113,-0.794772684000851,
9.39053710676437));
#35144=CARTESIAN_POINT('Ctrl Pts',(-3.630353335205,-0.636309800095197,9.3742697918532));
#35145=CARTESIAN_POINT('Ctrl Pts',(-3.55620605750903,-0.319434907277159,
9.35786137336722));
#35146=CARTESIAN_POINT('Ctrl Pts',(-3.53576509129249,-0.158333333333333,
9.35936221324764));
#35147=CARTESIAN_POINT('Ctrl Pts',(-3.52505210827391,0.158333333333334,
9.37684078872384));
#35148=CARTESIAN_POINT('Ctrl Pts',(-3.53535684314381,0.319434907277167,
9.39183563380664));
#35149=CARTESIAN_POINT('Ctrl Pts',(-3.58650774416314,0.636309800095206,
9.44584872924291));
#35150=CARTESIAN_POINT('Ctrl Pts',(-3.62740723167583,0.79477268400084,9.48102758076392));
#35151=CARTESIAN_POINT('Ctrl Pts',(-3.73295432340194,1.06847604194587,9.57151210020652));
#35152=CARTESIAN_POINT('Ctrl Pts',(-3.78889068790107,1.18514270861327,9.61843876361845));
#35153=CARTESIAN_POINT('Ctrl Pts',(-3.85507599179614,1.30000000000221,9.67312469475735));
#35154=CARTESIAN_POINT('Ctrl Pts',(-3.95827679071515,-1.3,9.50436744488836));
#35155=CARTESIAN_POINT('Ctrl Pts',(-3.8798859495176,-1.18514270861178,9.46962156082298));
#35156=CARTESIAN_POINT('Ctrl Pts',(-3.81258907846048,-1.06847604194512,
9.44126870438153));
#35157=CARTESIAN_POINT('Ctrl Pts',(-3.68274913399113,-0.794772684000851,
9.39053710676437));
#35158=CARTESIAN_POINT('Ctrl Pts',(-3.630353335205,-0.636309800095197,9.3742697918532));
#35159=CARTESIAN_POINT('Ctrl Pts',(-3.55620605750903,-0.319434907277159,
9.35786137336722));
#35160=CARTESIAN_POINT('Ctrl Pts',(-3.53576509129249,-0.158333333333332,
9.35936221324765));
#35161=CARTESIAN_POINT('Ctrl Pts',(-3.52505210827392,0.158333333333334,
9.37684078872385));
#35162=CARTESIAN_POINT('Ctrl Pts',(-3.53535684314381,0.319434907277167,
9.39183563380664));
#35163=CARTESIAN_POINT('Ctrl Pts',(-3.58650774416314,0.636309800095206,
9.44584872924292));
#35164=CARTESIAN_POINT('Ctrl Pts',(-3.62740723167583,0.79477268400084,9.48102758076392));
#35165=CARTESIAN_POINT('Ctrl Pts',(-3.73295432340165,1.06847604194511,9.57151210020627));
#35166=CARTESIAN_POINT('Ctrl Pts',(-3.78889068790036,1.18514270861178,9.61843876361785));
#35167=CARTESIAN_POINT('Ctrl Pts',(-3.85507599179487,1.3,9.6731246947563));
#35168=CARTESIAN_POINT('',(-4.17593056680875,-1.2,9.85783820071734));
#35169=CARTESIAN_POINT('Ctrl Pts',(-4.17593056680875,-1.2,9.85783820071734));
#35170=CARTESIAN_POINT('Ctrl Pts',(-4.16900460433805,-1.21680656858669,
9.83741928428235));
#35171=CARTESIAN_POINT('Ctrl Pts',(-4.16296024818596,-1.23316317392224,
9.8163387999078));
#35172=CARTESIAN_POINT('Ctrl Pts',(-4.1488048506352,-1.2666702566154,9.77575381663696));
#35173=CARTESIAN_POINT('Ctrl Pts',(-4.14194603049473,-1.28324039240427,
9.75534893186735));
#35174=CARTESIAN_POINT('Ctrl Pts',(-4.13459357261703,-1.30000000000009,
9.73527828635697));
#35175=CARTESIAN_POINT('',(-4.08975874013753,-0.653834841453647,9.98861496935521));
#35176=CARTESIAN_POINT('Ctrl Pts',(-4.0897587401673,-0.653834841446134,
9.98861496933965));
#35177=CARTESIAN_POINT('Ctrl Pts',(-4.09775715954222,-0.709816513138484,
9.97688455624721));
#35178=CARTESIAN_POINT('Ctrl Pts',(-4.10667273452126,-0.767198090793461,
9.96369085870135));
#35179=CARTESIAN_POINT('Ctrl Pts',(-4.13494013389672,-0.949641514625852,
9.92139732810018));
#35180=CARTESIAN_POINT('Ctrl Pts',(-4.15505714074664,-1.07515677647218,
9.89063401872584));
#35181=CARTESIAN_POINT('Ctrl Pts',(-4.17593056680875,-1.2,9.85783820071734));
#35182=CARTESIAN_POINT('',(-4.00955034077224,0.653834841531101,10.1027583545334));
#35183=CARTESIAN_POINT('Ctrl Pts',(-4.00955034077224,0.653834841531109,
10.1027583545334));
#35184=CARTESIAN_POINT('Ctrl Pts',(-3.9892075661712,0.575721283879273,10.0663434637934));
#35185=CARTESIAN_POINT('Ctrl Pts',(-3.97294247893386,0.49370810326247,10.0352117278294));
#35186=CARTESIAN_POINT('Ctrl Pts',(-3.95139645767513,0.338002156994941,
9.98935818625072));
#35187=CARTESIAN_POINT('Ctrl Pts',(-3.94495289412142,0.265532347033553,
9.97263620467793));
#35188=CARTESIAN_POINT('Ctrl Pts',(-3.94026888251158,0.129607443941674,
9.94872120414658));
#35189=CARTESIAN_POINT('Ctrl Pts',(-3.94093793002591,0.0665876566835187,
9.94052695975531));
#35190=CARTESIAN_POINT('Ctrl Pts',(-3.94825596348623,-0.0594622425677186,
9.92946225854297));
#35191=CARTESIAN_POINT('Ctrl Pts',(-3.95493666965847,-0.12262589836043,
9.92651382436694));
#35192=CARTESIAN_POINT('Ctrl Pts',(-3.97559481777179,-0.259989755378361,
9.92666831668788));
#35193=CARTESIAN_POINT('Ctrl Pts',(-3.99070125145753,-0.333867720853484,
9.93096966087476));
#35194=CARTESIAN_POINT('Ctrl Pts',(-4.03134687200918,-0.491609040819702,
9.95017991763267));
#35195=CARTESIAN_POINT('Ctrl Pts',(-4.05860469882518,-0.575043211348306,
9.9665674288075));
#35196=CARTESIAN_POINT('Ctrl Pts',(-4.08975874015232,-0.653834841462508,
9.98861496930265));
#35197=CARTESIAN_POINT('',(-4.05146929769195,1.2,10.0439578987495));
#35198=CARTESIAN_POINT('Ctrl Pts',(-4.05146929769195,1.2,10.0439578987495));
#35199=CARTESIAN_POINT('Ctrl Pts',(-4.04424830449576,1.13358862703007,10.0542448415506));
#35200=CARTESIAN_POINT('Ctrl Pts',(-4.03476005464607,1.03679350577961,10.0676732148766));
#35201=CARTESIAN_POINT('Ctrl Pts',(-4.01423194498588,0.76628625112874,10.0963297482212));
#35202=CARTESIAN_POINT('Ctrl Pts',(-4.01217510060249,0.713687193651155,
10.0991328007027));
#35203=CARTESIAN_POINT('Ctrl Pts',(-4.00955034077224,0.6538348415311,10.1027583545334));
#35204=CARTESIAN_POINT('Ctrl Pts',(-4.01176133534861,1.30000000000221,9.92548545917613));
#35205=CARTESIAN_POINT('Ctrl Pts',(-4.01208413859466,1.29919712732527,9.92643902247361));
#35206=CARTESIAN_POINT('Ctrl Pts',(-4.01241001091402,1.29839310268918,9.92738991408859));
#35207=CARTESIAN_POINT('Ctrl Pts',(-4.01932105646512,1.28166623088641,9.9469745517571));
#35208=CARTESIAN_POINT('Ctrl Pts',(-4.02569239595674,1.26580539078481,9.96573574783945));
#35209=CARTESIAN_POINT('Ctrl Pts',(-4.03644635502667,1.2393255832925,9.99676311150203));
#35210=CARTESIAN_POINT('Ctrl Pts',(-4.04452227242327,1.21971041315455,10.0195479433281));
#35211=CARTESIAN_POINT('Ctrl Pts',(-4.05146929769195,1.2,10.0439578987495));
#35212=CARTESIAN_POINT('Ctrl Pts',(-3.95827679071515,-1.3,9.50436744488836));
#35213=CARTESIAN_POINT('Ctrl Pts',(-3.8798859495176,-1.18514270861178,9.46962156082298));
#35214=CARTESIAN_POINT('Ctrl Pts',(-3.81258907846048,-1.06847604194512,
9.44126870438153));
#35215=CARTESIAN_POINT('Ctrl Pts',(-3.68274913399113,-0.794772684000851,
9.39053710676437));
#35216=CARTESIAN_POINT('Ctrl Pts',(-3.630353335205,-0.636309800095197,9.3742697918532));
#35217=CARTESIAN_POINT('Ctrl Pts',(-3.55620605750903,-0.319434907277159,
9.35786137336722));
#35218=CARTESIAN_POINT('Ctrl Pts',(-3.53576509129249,-0.158333333333332,
9.35936221324765));
#35219=CARTESIAN_POINT('Ctrl Pts',(-3.52505210827391,0.158333333333334,
9.37684078872384));
#35220=CARTESIAN_POINT('Ctrl Pts',(-3.53535684314381,0.319434907277167,
9.39183563380664));
#35221=CARTESIAN_POINT('Ctrl Pts',(-3.58650774416314,0.636309800095206,
9.44584872924291));
#35222=CARTESIAN_POINT('Ctrl Pts',(-3.62740723167583,0.79477268400084,9.48102758076392));
#35223=CARTESIAN_POINT('Ctrl Pts',(-3.73295432340165,1.06847604194511,9.57151210020627));
#35224=CARTESIAN_POINT('Ctrl Pts',(-3.78889068790036,1.18514270861178,9.61843876361785));
#35225=CARTESIAN_POINT('Ctrl Pts',(-3.85507599179487,1.3,9.6731246947563));
#35226=CARTESIAN_POINT('Ctrl Pts',(-3.99529346323778,-1.3,9.43692209493747));
#35227=CARTESIAN_POINT('Ctrl Pts',(-3.91621554992515,-1.18514270861178,
9.40376644257368));
#35228=CARTESIAN_POINT('Ctrl Pts',(-3.84848168092754,-1.06847604194512,
9.37653821129757));
#35229=CARTESIAN_POINT('Ctrl Pts',(-3.7182099051649,-0.794772684000851,
9.32732907854981));
#35230=CARTESIAN_POINT('Ctrl Pts',(-3.66630753169098,-0.636309800095197,
9.31054067879995));
#35231=CARTESIAN_POINT('Ctrl Pts',(-3.59275862546216,-0.319434907277159,
9.29383792247894));
#35232=CARTESIAN_POINT('Ctrl Pts',(-3.57308521991698,-0.158333333333332,
9.29436290252082));
#35233=CARTESIAN_POINT('Ctrl Pts',(-3.56268309827957,0.158333333333334,
9.31202095389912));
#35234=CARTESIAN_POINT('Ctrl Pts',(-3.57252649407444,0.319434907277167,
9.32816845594153));
#35235=CARTESIAN_POINT('Ctrl Pts',(-3.62372167678492,0.636309800095206,
9.38284692518677));
#35236=CARTESIAN_POINT('Ctrl Pts',(-3.66441660424588,0.79477268400084,9.41871363798237));
#35237=CARTESIAN_POINT('Ctrl Pts',(-3.77106627357833,1.06847604194511,9.50806294811988));
#35238=CARTESIAN_POINT('Ctrl Pts',(-3.8277580930697,1.18514270861178,9.55404884763091));
#35239=CARTESIAN_POINT('Ctrl Pts',(-3.89497704195816,1.3,9.60734464101269));
#35240=CARTESIAN_POINT('Ctrl Pts',(-4.0323101357604,-1.3,9.36947674498658));
#35241=CARTESIAN_POINT('Ctrl Pts',(-3.95254515033271,-1.18514270861178,
9.33791132432438));
#35242=CARTESIAN_POINT('Ctrl Pts',(-3.88437428339459,-1.06847604194512,
9.3118077182136));
#35243=CARTESIAN_POINT('Ctrl Pts',(-3.75367067633867,-0.794772684000851,
9.26412105033525));
#35244=CARTESIAN_POINT('Ctrl Pts',(-3.70226172817696,-0.636309800095197,
9.24681156574669));
#35245=CARTESIAN_POINT('Ctrl Pts',(-3.62931119341529,-0.319434907277159,
9.22981447159065));
#35246=CARTESIAN_POINT('Ctrl Pts',(-3.61040534854147,-0.158333333333332,
9.229363591794));
#35247=CARTESIAN_POINT('Ctrl Pts',(-3.60031408828524,0.158333333333334,
9.24720111907439));
#35248=CARTESIAN_POINT('Ctrl Pts',(-3.60969614500508,0.319434907277167,
9.26450127807642));
#35249=CARTESIAN_POINT('Ctrl Pts',(-3.6609356094067,0.636309800095206,9.31984512113063));
#35250=CARTESIAN_POINT('Ctrl Pts',(-3.70142597681592,0.79477268400084,9.35639969520082));
#35251=CARTESIAN_POINT('Ctrl Pts',(-3.80917822375501,1.06847604194511,9.4446137960335));
#35252=CARTESIAN_POINT('Ctrl Pts',(-3.86662549823905,1.18514270861178,9.48965893164399));
#35253=CARTESIAN_POINT('Ctrl Pts',(-3.93487809212145,1.3,9.54156458726908));
#35254=CARTESIAN_POINT('Ctrl Pts',(-4.06932680828303,-1.3,9.30203139503569));
#35255=CARTESIAN_POINT('Ctrl Pts',(-3.98887475074027,-1.18514270861178,
9.27205620607508));
#35256=CARTESIAN_POINT('Ctrl Pts',(-3.92026688586165,-1.06847604194512,
9.24707722512964));
#35257=CARTESIAN_POINT('Ctrl Pts',(-3.78913144751244,-0.794772684000851,
9.20091302212069));
#35258=CARTESIAN_POINT('Ctrl Pts',(-3.73821592466294,-0.636309800095197,
9.18308245269344));
#35259=CARTESIAN_POINT('Ctrl Pts',(-3.66586376136842,-0.319434907277159,
9.16579102070237));
#35260=CARTESIAN_POINT('Ctrl Pts',(-3.64772547716596,-0.158333333333332,
9.16436428106718));
#35261=CARTESIAN_POINT('Ctrl Pts',(-3.6379450782909,0.158333333333334,9.18238128424967));
#35262=CARTESIAN_POINT('Ctrl Pts',(-3.64686579593571,0.319434907277167,
9.20083410021131));
#35263=CARTESIAN_POINT('Ctrl Pts',(-3.69814954202848,0.636309800095206,
9.25684331707449));
#35264=CARTESIAN_POINT('Ctrl Pts',(-3.73843534938597,0.79477268400084,9.29408575241927));
#35265=CARTESIAN_POINT('Ctrl Pts',(-3.84729017393168,1.06847604194511,9.38116464394711));
#35266=CARTESIAN_POINT('Ctrl Pts',(-3.90549290340839,1.18514270861178,9.42526901565705));
#35267=CARTESIAN_POINT('Ctrl Pts',(-3.97477914228474,1.3,9.47578453352548));
#35268=CARTESIAN_POINT('Ctrl Pts',(-4.06932680828303,-1.3,9.30203139503569));
#35269=CARTESIAN_POINT('Ctrl Pts',(-3.98887475074027,-1.18514270861178,
9.27205620607508));
#35270=CARTESIAN_POINT('Ctrl Pts',(-3.92026688586165,-1.06847604194512,
9.24707722512964));
#35271=CARTESIAN_POINT('Ctrl Pts',(-3.78913144751244,-0.794772684000851,
9.20091302212069));
#35272=CARTESIAN_POINT('Ctrl Pts',(-3.73821592466294,-0.636309800095197,
9.18308245269344));
#35273=CARTESIAN_POINT('Ctrl Pts',(-3.66586376136842,-0.319434907277159,
9.16579102070237));
#35274=CARTESIAN_POINT('Ctrl Pts',(-3.64772547716596,-0.158333333333332,
9.16436428106718));
#35275=CARTESIAN_POINT('Ctrl Pts',(-3.6379450782909,0.158333333333334,9.18238128424967));
#35276=CARTESIAN_POINT('Ctrl Pts',(-3.64686579593571,0.319434907277167,
9.20083410021132));
#35277=CARTESIAN_POINT('Ctrl Pts',(-3.69814954202848,0.636309800095206,
9.25684331707449));
#35278=CARTESIAN_POINT('Ctrl Pts',(-3.73843534938597,0.79477268400084,9.29408575241927));
#35279=CARTESIAN_POINT('Ctrl Pts',(-3.84729017393169,1.06847604194511,9.38116464394711));
#35280=CARTESIAN_POINT('Ctrl Pts',(-3.90549290340839,1.18514270861178,9.42526901565705));
#35281=CARTESIAN_POINT('Ctrl Pts',(-3.97477914228474,1.3,9.47578453352548));
#35282=CARTESIAN_POINT('Ctrl Pts',(-4.0693268082841,-1.30000000000154,9.30203139503609));
#35283=CARTESIAN_POINT('Ctrl Pts',(-3.98887475074088,-1.18514270861282,
9.2720562060753));
#35284=CARTESIAN_POINT('Ctrl Pts',(-3.9202668858619,-1.06847604194564,9.24707722512973));
#35285=CARTESIAN_POINT('Ctrl Pts',(-3.78913144751244,-0.794772684000851,
9.20091302212069));
#35286=CARTESIAN_POINT('Ctrl Pts',(-3.73821592466294,-0.636309800095197,
9.18308245269344));
#35287=CARTESIAN_POINT('Ctrl Pts',(-3.66586376136842,-0.319434907277159,
9.16579102070237));
#35288=CARTESIAN_POINT('Ctrl Pts',(-3.64772547716596,-0.158333333333332,
9.16436428106718));
#35289=CARTESIAN_POINT('Ctrl Pts',(-3.6379450782909,0.158333333333334,9.18238128424967));
#35290=CARTESIAN_POINT('Ctrl Pts',(-3.64686579593571,0.319434907277167,
9.20083410021132));
#35291=CARTESIAN_POINT('Ctrl Pts',(-3.69814954202848,0.636309800095206,
9.25684331707449));
#35292=CARTESIAN_POINT('Ctrl Pts',(-3.73843534938597,0.79477268400084,9.29408575241927));
#35293=CARTESIAN_POINT('Ctrl Pts',(-3.84729017393255,1.06847604194727,9.3811646439478));
#35294=CARTESIAN_POINT('Ctrl Pts',(-3.90549290341051,1.18514270861603,9.42526901565866));
#35295=CARTESIAN_POINT('Ctrl Pts',(-3.97477914228853,1.30000000000629,9.47578453352824));
#35296=CARTESIAN_POINT('Ctrl Pts',(-4.07797887893123,-1.30000000000154,
9.30071436097919));
#35297=CARTESIAN_POINT('Ctrl Pts',(-3.9971009618214,-1.18514270861282,9.27127676660931));
#35298=CARTESIAN_POINT('Ctrl Pts',(-3.92828386835242,-1.06847604194564,
9.24627537341984));
#35299=CARTESIAN_POINT('Ctrl Pts',(-3.79716553099689,-0.794772684000851,
9.19876566582649));
#35300=CARTESIAN_POINT('Ctrl Pts',(-3.74717278256212,-0.636309800095197,
9.1774045083569));
#35301=CARTESIAN_POINT('Ctrl Pts',(-3.67523755004237,-0.319434907277159,
9.15838530602086));
#35302=CARTESIAN_POINT('Ctrl Pts',(-3.65704996965851,-0.158333333333332,
9.15750177709801));
#35303=CARTESIAN_POINT('Ctrl Pts',(-3.64724201471915,0.158333333333334,
9.17575399884814));
#35304=CARTESIAN_POINT('Ctrl Pts',(-3.65612349309497,0.319434907277167,
9.1941721677954));
#35305=CARTESIAN_POINT('Ctrl Pts',(-3.70705838931291,0.636309800095206,
9.2518314939406));
#35306=CARTESIAN_POINT('Ctrl Pts',(-3.7467174769052,0.79477268400084,9.29156195772604));
#35307=CARTESIAN_POINT('Ctrl Pts',(-3.85550223127429,1.06847604194727,9.38013053841707));
#35308=CARTESIAN_POINT('Ctrl Pts',(-3.91381537677535,1.18514270861603,9.42456161215902));
#35309=CARTESIAN_POINT('Ctrl Pts',(-3.98335277848303,1.30000000000629,9.47508570285074));
#35310=CARTESIAN_POINT('Ctrl Pts',(-4.09011797873321,-1.30000000000154,
9.30252364569461));
#35311=CARTESIAN_POINT('Ctrl Pts',(-4.01108973039803,-1.18514270861282,
9.27532957844728));
#35312=CARTESIAN_POINT('Ctrl Pts',(-3.94378582323447,-1.06847604194564,
9.25134724675337));
#35313=CARTESIAN_POINT('Ctrl Pts',(-3.81538590713933,-0.794772684000851,
9.2033630145254));
#35314=CARTESIAN_POINT('Ctrl Pts',(-3.76638481191805,-0.636309800095196,
9.17657067845296));
#35315=CARTESIAN_POINT('Ctrl Pts',(-3.69515467615052,-0.319434907277158,
9.15477598516934));
#35316=CARTESIAN_POINT('Ctrl Pts',(-3.67598551438858,-0.158333333333332,
9.15376112563587));
#35317=CARTESIAN_POINT('Ctrl Pts',(-3.6661483823356,0.158333333333334,9.17217245872481));
#35318=CARTESIAN_POINT('Ctrl Pts',(-3.67610124044008,0.319434907277168,
9.19077019887138));
#35319=CARTESIAN_POINT('Ctrl Pts',(-3.72602926377211,0.636309800095206,
9.25175495003996));
#35320=CARTESIAN_POINT('Ctrl Pts',(-3.76398909419763,0.794772684000839,
9.29785643624438));
#35321=CARTESIAN_POINT('Ctrl Pts',(-3.87008466638102,1.06847604194727,9.38686020609118));
#35322=CARTESIAN_POINT('Ctrl Pts',(-3.9270709548608,1.18514270861603,9.43000966829725));
#35323=CARTESIAN_POINT('Ctrl Pts',(-3.99511868985009,1.30000000000629,9.47778215865702));
#35324=CARTESIAN_POINT('Ctrl Pts',(-4.10795972278025,-1.30000000000153,
9.30505955869257));
#35325=CARTESIAN_POINT('Ctrl Pts',(-4.03226889918297,-1.18514270861282,
9.27940612168916));
#35326=CARTESIAN_POINT('Ctrl Pts',(-3.96750844541615,-1.06847604194564,
9.25636778477935));
#35327=CARTESIAN_POINT('Ctrl Pts',(-3.84315018285207,-0.794772684000848,
9.20918602207947));
#35328=CARTESIAN_POINT('Ctrl Pts',(-3.79429460663926,-0.636309800095195,
9.18080176601074));
#35329=CARTESIAN_POINT('Ctrl Pts',(-3.72375195285354,-0.319434907277158,
9.15788647602099));
#35330=CARTESIAN_POINT('Ctrl Pts',(-3.70367005810356,-0.158333333333332,
9.15573000955476));
#35331=CARTESIAN_POINT('Ctrl Pts',(-3.69377607554661,0.158333333333334,
9.17421636327135));
#35332=CARTESIAN_POINT('Ctrl Pts',(-3.70470750896684,0.319434907277167,
9.1937162806825));
#35333=CARTESIAN_POINT('Ctrl Pts',(-3.75358233346997,0.636309800095204,
9.25661495278545));
#35334=CARTESIAN_POINT('Ctrl Pts',(-3.79063880992344,0.794772684000837,
9.30603464088148));
#35335=CARTESIAN_POINT('Ctrl Pts',(-3.89267460720987,1.06847604194727,9.39440474368925));
#35336=CARTESIAN_POINT('Ctrl Pts',(-3.94728891409695,1.18514270861603,9.43630682995842));
#35337=CARTESIAN_POINT('Ctrl Pts',(-4.01235001202426,1.30000000000629,9.48185885942593));
#35338=CARTESIAN_POINT('Ctrl Pts',(-4.12284323460048,-1.30000000000154,
9.30685293138367));
#35339=CARTESIAN_POINT('Ctrl Pts',(-4.049785457782,-1.18514270861282,9.28199742225637));
#35340=CARTESIAN_POINT('Ctrl Pts',(-3.98688228258699,-1.06847604194564,
9.25967626151977));
#35341=CARTESIAN_POINT('Ctrl Pts',(-3.86502252532105,-0.794772684000848,
9.21396476666262));
#35342=CARTESIAN_POINT('Ctrl Pts',(-3.81496983539429,-0.636309800095194,
9.18689354017524));
#35343=CARTESIAN_POINT('Ctrl Pts',(-3.74449789211767,-0.319434907277157,
9.1638580222074));
#35344=CARTESIAN_POINT('Ctrl Pts',(-3.72423974057687,-0.158333333333331,
9.15973969708325));
#35345=CARTESIAN_POINT('Ctrl Pts',(-3.71456204305582,0.158333333333333,
9.17769261665386));
#35346=CARTESIAN_POINT('Ctrl Pts',(-3.72624291205814,0.319434907277165,
9.19779147741451));
#35347=CARTESIAN_POINT('Ctrl Pts',(-3.77476061621474,0.636309800095203,
9.261413403952));
#35348=CARTESIAN_POINT('Ctrl Pts',(-3.81167277195878,0.794772684000836,
9.31252192677137));
#35349=CARTESIAN_POINT('Ctrl Pts',(-3.91103129697726,1.06847604194727,9.39992907820287));
#35350=CARTESIAN_POINT('Ctrl Pts',(-3.96396036050981,1.18514270861603,9.44080281486098));
#35351=CARTESIAN_POINT('Ctrl Pts',(-4.02680986369017,1.30000000000629,9.48471497107627));
#35352=CARTESIAN_POINT('Ctrl Pts',(-4.13791931153452,-1.30000000000153,
9.30848411321606));
#35353=CARTESIAN_POINT('Ctrl Pts',(-4.06777250467259,-1.18514270861282,
9.2844327204044));
#35354=CARTESIAN_POINT('Ctrl Pts',(-4.00693160854003,-1.06847604194564,
9.26286747711773));
#35355=CARTESIAN_POINT('Ctrl Pts',(-3.88787548272047,-0.794772684000849,
9.2187909537687));
#35356=CARTESIAN_POINT('Ctrl Pts',(-3.83667833394984,-0.636309800095196,
9.19308213945078));
#35357=CARTESIAN_POINT('Ctrl Pts',(-3.76611582358144,-0.319434907277159,
9.17052568769673));
#35358=CARTESIAN_POINT('Ctrl Pts',(-3.74545998680562,-0.158333333333332,
9.16480797938058));
#35359=CARTESIAN_POINT('Ctrl Pts',(-3.73539946788037,0.158333333333334,
9.18354871474106));
#35360=CARTESIAN_POINT('Ctrl Pts',(-3.74685571876856,0.319434907277166,
9.20650796240082));
#35361=CARTESIAN_POINT('Ctrl Pts',(-3.79517201785929,0.636309800095204,
9.27029169704709));
#35362=CARTESIAN_POINT('Ctrl Pts',(-3.83355595154219,0.794772684000839,
9.31942042979027));
#35363=CARTESIAN_POINT('Ctrl Pts',(-3.93037163322943,1.06847604194727,9.4047403873389));
#35364=CARTESIAN_POINT('Ctrl Pts',(-3.98137404529088,1.18514270861603,9.44461938474921));
#35365=CARTESIAN_POINT('Ctrl Pts',(-4.04147094818551,1.30000000000629,9.48744553136265));
#35366=CARTESIAN_POINT('Ctrl Pts',(-4.1533794268455,-1.30000000000153,9.30876317496566));
#35367=CARTESIAN_POINT('Ctrl Pts',(-4.085970772055,-1.18514270861282,9.28554892971681));
#35368=CARTESIAN_POINT('Ctrl Pts',(-4.02703523000209,-1.06847604194564,
9.26483245483457));
#35369=CARTESIAN_POINT('Ctrl Pts',(-3.91045692330953,-0.794772684000848,
9.2227436027642));
#35370=CARTESIAN_POINT('Ctrl Pts',(-3.85806507197327,-0.636309800095194,
9.19857085576219));
#35371=CARTESIAN_POINT('Ctrl Pts',(-3.78694551084616,-0.319434907277157,
9.17754337018662));
#35372=CARTESIAN_POINT('Ctrl Pts',(-3.76516544649804,-0.158333333333331,
9.17201447101112));
#35373=CARTESIAN_POINT('Ctrl Pts',(-3.75481287203959,0.158333333333333,
9.19132159300446));
#35374=CARTESIAN_POINT('Ctrl Pts',(-3.76698441355051,0.319434907277164,
9.21481508671862));
#35375=CARTESIAN_POINT('Ctrl Pts',(-3.81550094633685,0.636309800095202,
9.27790442139565));
#35376=CARTESIAN_POINT('Ctrl Pts',(-3.85511179032036,0.794772684000835,
9.32565992050354));
#35377=CARTESIAN_POINT('Ctrl Pts',(-3.94941707868567,1.06847604194727,9.40931224094343));
#35378=CARTESIAN_POINT('Ctrl Pts',(-3.99852187921034,1.18514270861603,9.44843737352206));
#35379=CARTESIAN_POINT('Ctrl Pts',(-4.05591021528127,1.30000000000628,9.49047764878448));
#35380=CARTESIAN_POINT('Ctrl Pts',(-4.17747110574483,-1.30000000000153,
9.31118743640778));
#35381=CARTESIAN_POINT('Ctrl Pts',(-4.11456988829079,-1.18514270861282,
9.28924299342072));
#35382=CARTESIAN_POINT('Ctrl Pts',(-4.05883609878957,-1.06847604194564,
9.26968351006847));
#35383=CARTESIAN_POINT('Ctrl Pts',(-3.94663808794569,-0.79477268400085,
9.23000692452956));
#35384=CARTESIAN_POINT('Ctrl Pts',(-3.89279883435421,-0.636309800095195,
9.20710163656167));
#35385=CARTESIAN_POINT('Ctrl Pts',(-3.82107374744563,-0.319434907277158,
9.18781803868467));
#35386=CARTESIAN_POINT('Ctrl Pts',(-3.79728925346981,-0.158333333333332,
9.18294505239384));
#35387=CARTESIAN_POINT('Ctrl Pts',(-3.78668110903818,0.158333333333334,
9.20276514259551));
#35388=CARTESIAN_POINT('Ctrl Pts',(-3.8004863198785,0.319434907277165,9.22632762165036));
#35389=CARTESIAN_POINT('Ctrl Pts',(-3.84932243521093,0.636309800095203,
9.2882862617491));
#35390=CARTESIAN_POINT('Ctrl Pts',(-3.89033444775097,0.794772684000838,
9.33490442857791));
#35391=CARTESIAN_POINT('Ctrl Pts',(-3.98048279233754,1.06847604194727,9.41581046998228));
#35392=CARTESIAN_POINT('Ctrl Pts',(-4.02656895818941,1.18514270861603,9.45347458012295));
#35393=CARTESIAN_POINT('Ctrl Pts',(-4.0797194118466,1.30000000000628,9.49378157294425));
#35394=CARTESIAN_POINT('Ctrl Pts',(-4.20504288008068,-1.30000000000152,
9.31232210003516));
#35395=CARTESIAN_POINT('Ctrl Pts',(-4.14739578132247,-1.18514270861281,
9.29097859693842));
#35396=CARTESIAN_POINT('Ctrl Pts',(-4.0953629535084,-1.06847604194563,9.27223503249788));
#35397=CARTESIAN_POINT('Ctrl Pts',(-3.98812680113864,-0.794772684000841,
9.23494002741484));
#35398=CARTESIAN_POINT('Ctrl Pts',(-3.93228588504089,-0.636309800095189,
9.21468589554296));
#35399=CARTESIAN_POINT('Ctrl Pts',(-3.8598363508624,-0.319434907277155,
9.19767572904004));
#35400=CARTESIAN_POINT('Ctrl Pts',(-3.83416215730614,-0.15833333333333,
9.19290392150196));
#35401=CARTESIAN_POINT('Ctrl Pts',(-3.8230277047217,0.158333333333332,9.21384776584676));
#35402=CARTESIAN_POINT('Ctrl Pts',(-3.83795207230725,0.319434907277163,
9.23884390516112));
#35403=CARTESIAN_POINT('Ctrl Pts',(-3.88693807156031,0.636309800095198,
9.29998076988301));
#35404=CARTESIAN_POINT('Ctrl Pts',(-3.93003483749848,0.794772684000829,
9.3442254552323));
#35405=CARTESIAN_POINT('Ctrl Pts',(-4.01543246685247,1.06847604194726,9.42252823998472));
#35406=CARTESIAN_POINT('Ctrl Pts',(-4.05799623300798,1.18514270861602,9.45903423613183));
#35407=CARTESIAN_POINT('Ctrl Pts',(-4.10615829586529,1.30000000000628,9.4981518543105));
#35408=CARTESIAN_POINT('Ctrl Pts',(-4.23281323594865,-1.30000000000152,
9.31292054619255));
#35409=CARTESIAN_POINT('Ctrl Pts',(-4.18042031073655,-1.18514270861281,
9.29233208269215));
#35410=CARTESIAN_POINT('Ctrl Pts',(-4.13212992153116,-1.06847604194563,
9.27442120575142));
#35411=CARTESIAN_POINT('Ctrl Pts',(-4.03004714089272,-0.794772684000843,
9.23922925756194));
#35412=CARTESIAN_POINT('Ctrl Pts',(-3.97267347876869,-0.636309800095191,
9.22048356055537));
#35413=CARTESIAN_POINT('Ctrl Pts',(-3.89942412464079,-0.319434907277156,
9.20598169033391));
#35414=CARTESIAN_POINT('Ctrl Pts',(-3.87105812842082,-0.15833333333333,
9.20320269393037));
#35415=CARTESIAN_POINT('Ctrl Pts',(-3.85963656380305,0.158333333333332,
9.22481241000328));
#35416=CARTESIAN_POINT('Ctrl Pts',(-3.87685740408209,0.31943490727716,9.24867162974645));
#35417=CARTESIAN_POINT('Ctrl Pts',(-3.92627882889088,0.636309800095195,
9.30826947423017));
#35418=CARTESIAN_POINT('Ctrl Pts',(-3.97083543862442,0.794772684000832,
9.35138080852935));
#35419=CARTESIAN_POINT('Ctrl Pts',(-4.05116957893062,1.06847604194726,9.42757846509117));
#35420=CARTESIAN_POINT('Ctrl Pts',(-4.09009978676833,1.18514270861602,9.46308177444326));
#35421=CARTESIAN_POINT('Ctrl Pts',(-4.13318652977812,1.30000000000628,9.50110525102292));
#35422=CARTESIAN_POINT('Ctrl Pts',(-4.25116029379157,-1.30000000000152,
9.31376081103458));
#35423=CARTESIAN_POINT('Ctrl Pts',(-4.20211149992213,-1.18514270861281,
9.29412518622882));
#35424=CARTESIAN_POINT('Ctrl Pts',(-4.15624213215879,-1.06847604194563,
9.27697416319944));
#35425=CARTESIAN_POINT('Ctrl Pts',(-4.05761982683721,-0.794772684000842,
9.2430917960976));
#35426=CARTESIAN_POINT('Ctrl Pts',(-3.99949188056049,-0.636309800095188,
9.22449431303707));
#35427=CARTESIAN_POINT('Ctrl Pts',(-3.92609620592482,-0.319434907277154,
9.21066694055706));
#35428=CARTESIAN_POINT('Ctrl Pts',(-3.89643329069856,-0.15833333333333,
9.20810256072842));
#35429=CARTESIAN_POINT('Ctrl Pts',(-3.8847936228239,0.158333333333332,9.23022775344872));
#35430=CARTESIAN_POINT('Ctrl Pts',(-3.90300145842652,0.319434907277162,
9.25459038551016));
#35431=CARTESIAN_POINT('Ctrl Pts',(-3.95231197470889,0.636309800095196,
9.31415113672722));
#35432=CARTESIAN_POINT('Ctrl Pts',(-3.99765893703627,0.794772684000827,
9.35701865505897));
#35433=CARTESIAN_POINT('Ctrl Pts',(-4.07452946440137,1.06847604194726,9.43206753415053));
#35434=CARTESIAN_POINT('Ctrl Pts',(-4.11105502488755,1.18514270861602,9.46687156953381));
#35435=CARTESIAN_POINT('Ctrl Pts',(-4.15083174289697,1.30000000000627,9.50399376137633));
#35436=CARTESIAN_POINT('Ctrl Pts',(-4.26670499109829,-1.30000000000152,
9.31367542306743));
#35437=CARTESIAN_POINT('Ctrl Pts',(-4.22079506822243,-1.18514270861281,
9.29376305362827));
#35438=CARTESIAN_POINT('Ctrl Pts',(-4.17714866477651,-1.06847604194563,
9.2766291896994));
#35439=CARTESIAN_POINT('Ctrl Pts',(-4.08154592408225,-0.794772684000842,
9.24346543997298));
#35440=CARTESIAN_POINT('Ctrl Pts',(-4.02234410608837,-0.636309800095189,
9.22644454060134));
#35441=CARTESIAN_POINT('Ctrl Pts',(-3.94852035825935,-0.319434907277154,
9.21409456825448));
#35442=CARTESIAN_POINT('Ctrl Pts',(-3.91754048734327,-0.15833333333333,
9.21227699640609));
#35443=CARTESIAN_POINT('Ctrl Pts',(-3.90569550186702,0.158333333333332,
9.23491704998506));
#35444=CARTESIAN_POINT('Ctrl Pts',(-3.92493844300946,0.319434907277162,
9.25917897805349));
#35445=CARTESIAN_POINT('Ctrl Pts',(-3.97441470660465,0.636309800095196,
9.31804373083212));
#35446=CARTESIAN_POINT('Ctrl Pts',(-4.02072096957854,0.794772684000828,
9.35989732509025));
#35447=CARTESIAN_POINT('Ctrl Pts',(-4.09473830712847,1.06847604194726,9.43389179977599));
#35448=CARTESIAN_POINT('Ctrl Pts',(-4.1291977435757,1.18514270861602,9.46827286972838));
#35449=CARTESIAN_POINT('Ctrl Pts',(-4.16607725365714,1.30000000000627,9.50500554330687));
#35450=CARTESIAN_POINT('Ctrl Pts',(-4.27753228080596,-1.30000000000152,
9.31376050379798));
#35451=CARTESIAN_POINT('Ctrl Pts',(-4.23367329127038,-1.18514270861281,
9.29409865065746));
#35452=CARTESIAN_POINT('Ctrl Pts',(-4.19149340446467,-1.06847604194563,
9.27724608128728));
#35453=CARTESIAN_POINT('Ctrl Pts',(-4.09792849109564,-0.79477268400084,
9.24480328220206));
#35454=CARTESIAN_POINT('Ctrl Pts',(-4.03810846364677,-0.636309800095188,
9.22844010672574));
#35455=CARTESIAN_POINT('Ctrl Pts',(-3.96412755056454,-0.319434907277154,
9.21671586212742));
#35456=CARTESIAN_POINT('Ctrl Pts',(-3.93237379326356,-0.15833333333333,
9.21504405513902));
#35457=CARTESIAN_POINT('Ctrl Pts',(-3.92047047892969,0.158333333333332,
9.23782238423847));
#35458=CARTESIAN_POINT('Ctrl Pts',(-3.94045398425137,0.319434907277162,
9.261982637299));
#35459=CARTESIAN_POINT('Ctrl Pts',(-3.98991766466715,0.636309800095196,
9.32069516903308));
#35460=CARTESIAN_POINT('Ctrl Pts',(-4.03657008444672,0.794772684000827,
9.36267658603357));
#35461=CARTESIAN_POINT('Ctrl Pts',(-4.10858232727238,1.06847604194726,9.43595073645765));
#35462=CARTESIAN_POINT('Ctrl Pts',(-4.14166623194688,1.18514270861602,9.46985157773273));
#35463=CARTESIAN_POINT('Ctrl Pts',(-4.17666260969292,1.30000000000627,9.50593559563883));
#35464=CARTESIAN_POINT('Ctrl Pts',(-4.28376574468374,-1.30000000000152,
9.31366392579355));
#35465=CARTESIAN_POINT('Ctrl Pts',(-4.24103726129138,-1.18514270861281,
9.29427710274561));
#35466=CARTESIAN_POINT('Ctrl Pts',(-4.19967103402951,-1.06847604194563,
9.2776636701469));
#35467=CARTESIAN_POINT('Ctrl Pts',(-4.10725385794923,-0.794772684000841,
9.24569040409073));
#35468=CARTESIAN_POINT('Ctrl Pts',(-4.04713008303279,-0.636309800095188,
9.22954767265744));
#35469=CARTESIAN_POINT('Ctrl Pts',(-3.97309785341113,-0.319434907277154,
9.21807347310103));
#35470=CARTESIAN_POINT('Ctrl Pts',(-3.94095387220251,-0.15833333333333,
9.21635381743337));
#35471=CARTESIAN_POINT('Ctrl Pts',(-3.92898727114034,0.158333333333332,
9.23928703884165));
#35472=CARTESIAN_POINT('Ctrl Pts',(-3.94929239596999,0.319434907277162,
9.26364869411582));
#35473=CARTESIAN_POINT('Ctrl Pts',(-3.99868931413014,0.636309800095197,
9.32242941227565));
#35474=CARTESIAN_POINT('Ctrl Pts',(-4.04556297752378,0.794772684000828,
9.36443027327445));
#35475=CARTESIAN_POINT('Ctrl Pts',(-4.11639122616648,1.06847604194726,9.43739081622));
#35476=CARTESIAN_POINT('Ctrl Pts',(-4.14866548399181,1.18514270861602,9.47107631964459));
#35477=CARTESIAN_POINT('Ctrl Pts',(-4.18255507525001,1.30000000000627,9.50686541090687));
#35478=CARTESIAN_POINT('Ctrl Pts',(-4.299395134043,-1.30000000000152,9.31326205030675));
#35479=CARTESIAN_POINT('Ctrl Pts',(-4.2595340555938,-1.18514270861281,9.29442455647643));
#35480=CARTESIAN_POINT('Ctrl Pts',(-4.22023142337693,-1.06847604194563,
9.27831309146941));
#35481=CARTESIAN_POINT('Ctrl Pts',(-4.13072460300502,-0.79477268400084,
9.24739005613777));
#35482=CARTESIAN_POINT('Ctrl Pts',(-4.06984446995732,-0.636309800095188,
9.23181809073007));
#35483=CARTESIAN_POINT('Ctrl Pts',(-3.99565112279439,-0.319434907277155,
9.22108363448806));
#35484=CARTESIAN_POINT('Ctrl Pts',(-3.96244514185411,-0.15833333333333,
9.21949927156026));
#35485=CARTESIAN_POINT('Ctrl Pts',(-3.95031771039047,0.158333333333332,
9.24284591715237));
#35486=CARTESIAN_POINT('Ctrl Pts',(-3.97146423549848,0.319434907277161,
9.26761349642659));
#35487=CARTESIAN_POINT('Ctrl Pts',(-4.02081641650737,0.636309800095196,
9.32623628233159));
#35488=CARTESIAN_POINT('Ctrl Pts',(-4.06845915214776,0.794772684000829,
9.36769014467127));
#35489=CARTESIAN_POINT('Ctrl Pts',(-4.13632501846853,1.06847604194726,9.43987618616326));
#35490=CARTESIAN_POINT('Ctrl Pts',(-4.16651958174986,1.18514270861602,9.4731776780092));
#35491=CARTESIAN_POINT('Ctrl Pts',(-4.19753208946014,1.30000000000627,9.50853399909531));
#35492=CARTESIAN_POINT('Ctrl Pts',(-4.32558216921391,-1.30000000000151,
9.31372186269296));
#35493=CARTESIAN_POINT('Ctrl Pts',(-4.29094222329233,-1.1851427086128,9.29469301243295));
#35494=CARTESIAN_POINT('Ctrl Pts',(-4.25537610244751,-1.06847604194562,
9.27869877259595));
#35495=CARTESIAN_POINT('Ctrl Pts',(-4.17107159896477,-0.794772684000835,
9.24875943608465));
#35496=CARTESIAN_POINT('Ctrl Pts',(-4.10867533471152,-0.636309800095184,
9.23498747374347));
#35497=CARTESIAN_POINT('Ctrl Pts',(-4.03403287930407,-0.319434907277152,
9.22603066394919));
#35498=CARTESIAN_POINT('Ctrl Pts',(-3.99866953595907,-0.158333333333329,
9.22558567956006));
#35499=CARTESIAN_POINT('Ctrl Pts',(-3.98645646098271,0.158333333333331,
9.24912504001713));
#35500=CARTESIAN_POINT('Ctrl Pts',(-4.00974347283856,0.319434907277159,
9.27266673277605));
#35501=CARTESIAN_POINT('Ctrl Pts',(-4.05923023725212,0.636309800095192,
9.33047317536098));
#35502=CARTESIAN_POINT('Ctrl Pts',(-4.10778847468005,0.794772684000823,
9.37207515896062));
#35503=CARTESIAN_POINT('Ctrl Pts',(-4.17055531628905,1.06847604194725,9.44315633901884));
#35504=CARTESIAN_POINT('Ctrl Pts',(-4.197228550674,1.18514270861601,9.47578816178047));
#35505=CARTESIAN_POINT('Ctrl Pts',(-4.22340557945179,1.30000000000627,9.51028339827349));
#35506=CARTESIAN_POINT('Ctrl Pts',(-4.36339961556755,-1.30000000000151,
9.31149883582506));
#35507=CARTESIAN_POINT('Ctrl Pts',(-4.33590918874599,-1.1851427086128,9.29282781111208));
#35508=CARTESIAN_POINT('Ctrl Pts',(-4.30549194641469,-1.06847604194562,
9.27736191017708));
#35509=CARTESIAN_POINT('Ctrl Pts',(-4.22846050234616,-0.794772684000833,
9.24903706218436));
#35510=CARTESIAN_POINT('Ctrl Pts',(-4.16424523170537,-0.636309800095181,
9.23686177834877));
#35511=CARTESIAN_POINT('Ctrl Pts',(-4.08914233458117,-0.31943490727715,
9.23009077363859));
#35512=CARTESIAN_POINT('Ctrl Pts',(-4.05100021784028,-0.158333333333329,
9.23078853853655));
#35513=CARTESIAN_POINT('Ctrl Pts',(-4.03827950130655,0.158333333333331,
9.25580113040377));
#35514=CARTESIAN_POINT('Ctrl Pts',(-4.06358260654506,0.319434907277162,
9.28033001254928));
#35515=CARTESIAN_POINT('Ctrl Pts',(-4.11301527834565,0.636309800095193,
9.33761385094508));
#35516=CARTESIAN_POINT('Ctrl Pts',(-4.16368772934163,0.794772684000819,
9.37707595318374));
#35517=CARTESIAN_POINT('Ctrl Pts',(-4.21918785472595,1.06847604194724,9.44675113514984));
#35518=CARTESIAN_POINT('Ctrl Pts',(-4.24070989192469,1.185142708616,9.47893185897244));
#35519=CARTESIAN_POINT('Ctrl Pts',(-4.25973001852536,1.30000000000626,9.51313350206414));
#35520=CARTESIAN_POINT('Ctrl Pts',(-4.39287315342704,-1.3000000000015,9.31107034343129));
#35521=CARTESIAN_POINT('Ctrl Pts',(-4.37126556181242,-1.18514270861279,
9.29187809878067));
#35522=CARTESIAN_POINT('Ctrl Pts',(-4.3450951857209,-1.06847604194561,9.27623236383228));
#35523=CARTESIAN_POINT('Ctrl Pts',(-4.27409543666033,-0.794772684000828,
9.24828073307203));
#35524=CARTESIAN_POINT('Ctrl Pts',(-4.20846511303003,-0.63630980009518,
9.23742862906884));
#35525=CARTESIAN_POINT('Ctrl Pts',(-4.13303144622131,-0.319434907277151,
9.23234354937861));
#35526=CARTESIAN_POINT('Ctrl Pts',(-4.09244763322764,-0.158333333333328,
9.23467408865915));
#35527=CARTESIAN_POINT('Ctrl Pts',(-4.07960349336706,0.15833333333333,9.26006972675397));
#35528=CARTESIAN_POINT('Ctrl Pts',(-4.1072895064877,0.319434907277159,9.2830901745054));
#35529=CARTESIAN_POINT('Ctrl Pts',(-4.15666988679089,0.636309800095189,
9.33999529144816));
#35530=CARTESIAN_POINT('Ctrl Pts',(-4.20807314245923,0.794772684000818,
9.38045854599755));
#35531=CARTESIAN_POINT('Ctrl Pts',(-4.25769277471803,1.06847604194724,9.44948027541786));
#35532=CARTESIAN_POINT('Ctrl Pts',(-4.27523743063318,1.18514270861601,9.48107725233575));
#35533=CARTESIAN_POINT('Ctrl Pts',(-4.288848242247,1.30000000000626,9.5143942570123));
#35534=CARTESIAN_POINT('Ctrl Pts',(-4.41828955691599,-1.3000000000015,9.30871299493204));
#35535=CARTESIAN_POINT('Ctrl Pts',(-4.40139988976438,-1.18514270861279,
9.28984824185018));
#35536=CARTESIAN_POINT('Ctrl Pts',(-4.37865455922241,-1.06847604194561,
9.27453897962996));
#35537=CARTESIAN_POINT('Ctrl Pts',(-4.31258054162962,-0.794772684000826,
9.24738541645785));
#35538=CARTESIAN_POINT('Ctrl Pts',(-4.24595507448116,-0.636309800095179,
9.23694606010339));
#35539=CARTESIAN_POINT('Ctrl Pts',(-4.17037233349577,-0.319434907277151,
9.23291925778407));
#35540=CARTESIAN_POINT('Ctrl Pts',(-4.12801255166076,-0.158333333333328,
9.23590162478777));
#35541=CARTESIAN_POINT('Ctrl Pts',(-4.11480007208656,0.15833333333333,9.26246631800015));
#35542=CARTESIAN_POINT('Ctrl Pts',(-4.14363369407532,0.31943490727716,9.28676807309881));
#35543=CARTESIAN_POINT('Ctrl Pts',(-4.1929425096266,0.63630980009519,9.34343981792205));
#35544=CARTESIAN_POINT('Ctrl Pts',(-4.24591465250796,0.794772684000817,
9.38190123681928));
#35545=CARTESIAN_POINT('Ctrl Pts',(-4.29067970726545,1.06847604194724,9.45006192760711));
#35546=CARTESIAN_POINT('Ctrl Pts',(-4.30475619025655,1.185142708616,9.48150833098788));
#35547=CARTESIAN_POINT('Ctrl Pts',(-4.3135320227428,1.30000000000626,9.51489690030957));
#35548=CARTESIAN_POINT('Ctrl Pts',(-4.43698594830172,-1.3000000000015,9.30804571980993));
#35549=CARTESIAN_POINT('Ctrl Pts',(-4.42390105088262,-1.18514270861279,
9.2884897363668));
#35550=CARTESIAN_POINT('Ctrl Pts',(-4.40388453279908,-1.06847604194561,
9.27287439871892));
#35551=CARTESIAN_POINT('Ctrl Pts',(-4.34162894133467,-0.794772684000827,
9.24590352502531));
#35552=CARTESIAN_POINT('Ctrl Pts',(-4.27383343181233,-0.636309800095178,
9.23728199950697));
#35553=CARTESIAN_POINT('Ctrl Pts',(-4.19817239325749,-0.31943490727715,
9.23398769339868));
#35554=CARTESIAN_POINT('Ctrl Pts',(-4.15467691343505,-0.158333333333328,
9.23677055247689));
#35555=CARTESIAN_POINT('Ctrl Pts',(-4.14158202539205,0.15833333333333,9.26298585791562));
#35556=CARTESIAN_POINT('Ctrl Pts',(-4.17188912877299,0.319434907277159,
9.28640029692033));
#35557=CARTESIAN_POINT('Ctrl Pts',(-4.22106725238384,0.636309800095188,
9.34312997232989));
#35558=CARTESIAN_POINT('Ctrl Pts',(-4.27433933090947,0.794772684000817,
9.38273777429863));
#35559=CARTESIAN_POINT('Ctrl Pts',(-4.31519262141616,1.06847604194724,9.45110238518818));
#35560=CARTESIAN_POINT('Ctrl Pts',(-4.32666894689436,1.185142708616,9.48245364140811));
#35561=CARTESIAN_POINT('Ctrl Pts',(-4.33193772215384,1.30000000000625,9.51556364695209));
#35562=CARTESIAN_POINT('Ctrl Pts',(-4.45742539215227,-1.30000000000149,
9.30672991413338));
#35563=CARTESIAN_POINT('Ctrl Pts',(-4.44819512374719,-1.18514270861278,
9.2873438766223));
#35564=CARTESIAN_POINT('Ctrl Pts',(-4.4310073952158,-1.06847604194561,9.27182726939889));
#35565=CARTESIAN_POINT('Ctrl Pts',(-4.37291697913885,-0.794772684000826,
9.24491996066763));
#35566=CARTESIAN_POINT('Ctrl Pts',(-4.30460489739991,-0.636309800095177,
9.23562325498352));
#35567=CARTESIAN_POINT('Ctrl Pts',(-4.22886151246214,-0.319434907277149,
9.2330764560671));
#35568=CARTESIAN_POINT('Ctrl Pts',(-4.18367015350271,-0.158333333333327,
9.23729721921038));
#35569=CARTESIAN_POINT('Ctrl Pts',(-4.1702162969332,0.158333333333329,9.26470909809492));
#35570=CARTESIAN_POINT('Ctrl Pts',(-4.20159383392492,0.319434907277157,
9.28873078254841));
#35571=CARTESIAN_POINT('Ctrl Pts',(-4.2506659053382,0.636309800095186,9.34542179636802));
#35572=CARTESIAN_POINT('Ctrl Pts',(-4.30501761360352,0.794772684000815,
9.38397247896077));
#35573=CARTESIAN_POINT('Ctrl Pts',(-4.34189032661779,1.06847604194724,9.45177413756467));
#35574=CARTESIAN_POINT('Ctrl Pts',(-4.35056771527077,1.185142708616,9.4829668134292));
#35575=CARTESIAN_POINT('Ctrl Pts',(-4.35196166138135,1.30000000000625,9.51600333944736));
#35576=CARTESIAN_POINT('Ctrl Pts',(-4.47330007032464,-1.30000000000149,
9.30509533005243));
#35577=CARTESIAN_POINT('Ctrl Pts',(-4.46718357161219,-1.18514270861278,
9.28525798096092));
#35578=CARTESIAN_POINT('Ctrl Pts',(-4.45223897087315,-1.06847604194561,
9.26954732156572));
#35579=CARTESIAN_POINT('Ctrl Pts',(-4.39731927177176,-0.794772684000823,
9.24278603419616));
#35580=CARTESIAN_POINT('Ctrl Pts',(-4.32819150206691,-0.636309800095176,
9.23452078395232));
#35581=CARTESIAN_POINT('Ctrl Pts',(-4.25230757573395,-0.319434907277149,
9.23287568972763));
#35582=CARTESIAN_POINT('Ctrl Pts',(-4.20594738799116,-0.158333333333327,
9.23772258646171));
#35583=CARTESIAN_POINT('Ctrl Pts',(-4.19246143001637,0.158333333333329,
9.26528793158875));
#35584=CARTESIAN_POINT('Ctrl Pts',(-4.22500406516011,0.319434907277157,
9.28871710104222));
#35585=CARTESIAN_POINT('Ctrl Pts',(-4.27409350049364,0.636309800095185,
9.34506313089331));
#35586=CARTESIAN_POINT('Ctrl Pts',(-4.32908181488484,0.794772684000814,
9.38337935851737));
#35587=CARTESIAN_POINT('Ctrl Pts',(-4.36271708420564,1.06847604194724,9.45131076833307));
#35588=CARTESIAN_POINT('Ctrl Pts',(-4.36915471491328,1.18514270861599,9.48266781477494));
#35589=CARTESIAN_POINT('Ctrl Pts',(-4.36747051454899,1.30000000000625,9.51597691745595));
#35590=CARTESIAN_POINT('Ctrl Pts',(-4.48591544608392,-1.30000000000149,
9.30407848436835));
#35591=CARTESIAN_POINT('Ctrl Pts',(-4.48223751921892,-1.18514270861278,
9.28408043200416));
#35592=CARTESIAN_POINT('Ctrl Pts',(-4.46906707167276,-1.0684760419456,9.26829286640692));
#35593=CARTESIAN_POINT('Ctrl Pts',(-4.4167110813565,-0.794772684000821,
9.24154749832233));
#35594=CARTESIAN_POINT('Ctrl Pts',(-4.34711954603316,-0.636309800095173,
9.23339966233023));
#35595=CARTESIAN_POINT('Ctrl Pts',(-4.27113748432086,-0.319434907277147,
9.2324071115974));
#35596=CARTESIAN_POINT('Ctrl Pts',(-4.22371578345613,-0.158333333333326,
9.23821726492005));
#35597=CARTESIAN_POINT('Ctrl Pts',(-4.2101324175127,0.158333333333328,9.2661381208997));
#35598=CARTESIAN_POINT('Ctrl Pts',(-4.24356994227013,0.319434907277155,
9.28917716981086));
#35599=CARTESIAN_POINT('Ctrl Pts',(-4.29270008703502,0.636309800095182,
9.34515151932937));
#35600=CARTESIAN_POINT('Ctrl Pts',(-4.34831010011928,0.794772684000811,
9.3829296317695));
#35601=CARTESIAN_POINT('Ctrl Pts',(-4.3793937664007,1.06847604194723,9.45085335887142));
#35602=CARTESIAN_POINT('Ctrl Pts',(-4.38404015954559,1.18514270861599,9.48234661916512));
#35603=CARTESIAN_POINT('Ctrl Pts',(-4.37987797846535,1.30000000000624,9.51593147511192));
#35604=CARTESIAN_POINT('Ctrl Pts',(-4.49545712166529,-1.30000000000149,
9.30298909365531));
#35605=CARTESIAN_POINT('Ctrl Pts',(-4.49366288936686,-1.18514270861278,
9.28263576101769));
#35606=CARTESIAN_POINT('Ctrl Pts',(-4.4818464760129,-1.0684760419456,9.26668653526624));
#35607=CARTESIAN_POINT('Ctrl Pts',(-4.43139495413128,-0.794772684000821,
9.2400150010944));
#35608=CARTESIAN_POINT('Ctrl Pts',(-4.36126958694013,-0.636309800095173,
9.23269240322661));
#35609=CARTESIAN_POINT('Ctrl Pts',(-4.28522139944164,-0.319434907277147,
9.23220200621834));
#35610=CARTESIAN_POINT('Ctrl Pts',(-4.23719754852272,-0.158333333333326,
9.2380521444923));
#35611=CARTESIAN_POINT('Ctrl Pts',(-4.22354730410942,0.158333333333328,
9.26621721072458));
#35612=CARTESIAN_POINT('Ctrl Pts',(-4.25753318963454,0.319434907277155,
9.28938803048818));
#35613=CARTESIAN_POINT('Ctrl Pts',(-4.30656657183381,0.636309800095182,
9.34550524947842));
#35614=CARTESIAN_POINT('Ctrl Pts',(-4.36249756287696,0.794772684000811,
9.38334073259891));
#35615=CARTESIAN_POINT('Ctrl Pts',(-4.39168520889225,1.06847604194723,9.45120441704213));
#35616=CARTESIAN_POINT('Ctrl Pts',(-4.39504051886166,1.18514270861599,9.48263319967326));
#35617=CARTESIAN_POINT('Ctrl Pts',(-4.38911688834923,1.30000000000624,9.5161150905371));
#35618=CARTESIAN_POINT('Ctrl Pts',(-4.50341177882622,-1.30000000000148,
9.30205197134735));
#35619=CARTESIAN_POINT('Ctrl Pts',(-4.50320647280269,-1.18514270861278,
9.28132700338567));
#35620=CARTESIAN_POINT('Ctrl Pts',(-4.49253050120596,-1.0684760419456,9.26519534066278));
#35621=CARTESIAN_POINT('Ctrl Pts',(-4.44367753897328,-0.79477268400082,
9.23853942663408));
#35622=CARTESIAN_POINT('Ctrl Pts',(-4.37308289742706,-0.636309800095173,
9.23199434726505));
#35623=CARTESIAN_POINT('Ctrl Pts',(-4.29698135930824,-0.319434907277147,
9.23192540247938));
#35624=CARTESIAN_POINT('Ctrl Pts',(-4.24847292057746,-0.158333333333326,
9.23776209480255));
#35625=CARTESIAN_POINT('Ctrl Pts',(-4.23477258182423,0.158333333333328,
9.26611709674983));
#35626=CARTESIAN_POINT('Ctrl Pts',(-4.26921336639415,0.319434907277154,
9.28940069847015));
#35627=CARTESIAN_POINT('Ctrl Pts',(-4.31815649596753,0.636309800095181,
9.34566789569745));
#35628=CARTESIAN_POINT('Ctrl Pts',(-4.37434146750644,0.794772684000811,
9.38359338165133));
#35629=CARTESIAN_POINT('Ctrl Pts',(-4.40193631222051,1.06847604194723,9.4514529290796));
#35630=CARTESIAN_POINT('Ctrl Pts',(-4.40421094214181,1.18514270861599,9.48284670770899));
#35631=CARTESIAN_POINT('Ctrl Pts',(-4.39681541619732,1.30000000000624,9.51626038132981));
#35632=CARTESIAN_POINT('Ctrl Pts',(-4.50895399487148,-1.30000000000149,
9.3014961675291));
#35633=CARTESIAN_POINT('Ctrl Pts',(-4.50983134943706,-1.18514270861278,
9.28062700615559));
#35634=CARTESIAN_POINT('Ctrl Pts',(-4.49994130733982,-1.0684760419456,9.26441615343415));
#35635=CARTESIAN_POINT('Ctrl Pts',(-4.45221849129775,-0.79477268400082,
9.23772746555552));
#35636=CARTESIAN_POINT('Ctrl Pts',(-4.38139149177153,-0.636309800095173,
9.23135207715777));
#35637=CARTESIAN_POINT('Ctrl Pts',(-4.3052627002583,-0.319434907277147,
9.23153436528605));
#35638=CARTESIAN_POINT('Ctrl Pts',(-4.25633847738863,-0.158333333333326,
9.23764772076595));
#35639=CARTESIAN_POINT('Ctrl Pts',(-4.24260456385794,0.158333333333328,
9.26613747379966));
#35640=CARTESIAN_POINT('Ctrl Pts',(-4.27741492625282,0.319434907277154,
9.28931800303927));
#35641=CARTESIAN_POINT('Ctrl Pts',(-4.32634264934668,0.636309800095181,
9.34552933216575));
#35642=CARTESIAN_POINT('Ctrl Pts',(-4.38276188423467,0.794772684000811,
9.38333626246547));
#35643=CARTESIAN_POINT('Ctrl Pts',(-4.40921848311906,1.06847604194723,9.45126823561079));
#35644=CARTESIAN_POINT('Ctrl Pts',(-4.41070574048119,1.18514270861599,9.48273786026433));
#35645=CARTESIAN_POINT('Ctrl Pts',(-4.40222817386188,1.30000000000624,9.51627187552419));
#35646=CARTESIAN_POINT('Ctrl Pts',(-4.51171978258121,-1.30000000000148,
9.30123799540998));
#35647=CARTESIAN_POINT('Ctrl Pts',(-4.51313332307936,-1.18514270861277,
9.28031671505525));
#35648=CARTESIAN_POINT('Ctrl Pts',(-4.50363425316894,-1.0684760419456,9.26407395976082));
#35649=CARTESIAN_POINT('Ctrl Pts',(-4.45647918828954,-0.794772684000819,
9.23735827450373));
#35650=CARTESIAN_POINT('Ctrl Pts',(-4.38555378140777,-0.636309800095172,
9.23099860708769));
#35651=CARTESIAN_POINT('Ctrl Pts',(-4.30941430465361,-0.319434907277147,
9.23129437494411));
#35652=CARTESIAN_POINT('Ctrl Pts',(-4.26026996600083,-0.158333333333326,
9.2375917282832));
#35653=CARTESIAN_POINT('Ctrl Pts',(-4.24651917741272,0.158333333333328,
9.2661504769457));
#35654=CARTESIAN_POINT('Ctrl Pts',(-4.2815207054548,0.319434907277154,9.28925693144228));
#35655=CARTESIAN_POINT('Ctrl Pts',(-4.33044933657815,0.636309800095181,
9.34541195362376));
#35656=CARTESIAN_POINT('Ctrl Pts',(-4.38699854464526,0.79477268400081,9.38311782851278));
#35657=CARTESIAN_POINT('Ctrl Pts',(-4.41288286047686,1.06847604194723,9.45109712145016));
#35658=CARTESIAN_POINT('Ctrl Pts',(-4.41397102284211,1.18514270861599,9.48262284024169));
#35659=CARTESIAN_POINT('Ctrl Pts',(-4.40494298635743,1.30000000000624,9.51624856079291));
#35660=CARTESIAN_POINT('Ctrl Pts',(-4.51329932039636,-1.30000000000148,
9.30109370574358));
#35661=CARTESIAN_POINT('Ctrl Pts',(-4.51501832187378,-1.18514270861278,
9.2801462216824));
#35662=CARTESIAN_POINT('Ctrl Pts',(-4.5057422995373,-1.0684760419456,9.26388665087337));
#35663=CARTESIAN_POINT('Ctrl Pts',(-4.45891212772117,-0.794772684000819,
9.23715380701488));
#35664=CARTESIAN_POINT('Ctrl Pts',(-4.38793393240501,-0.636309800095172,
9.2307900577638));
#35665=CARTESIAN_POINT('Ctrl Pts',(-4.31178834187582,-0.319434907277147,
9.23115058609829));
#35666=CARTESIAN_POINT('Ctrl Pts',(-4.26251467800089,-0.158333333333326,
9.23756615242111));
#35667=CARTESIAN_POINT('Ctrl Pts',(-4.24875440944061,0.158333333333328,
9.26616398536437));
#35668=CARTESIAN_POINT('Ctrl Pts',(-4.28386822297713,0.319434907277154,
9.28921720033903));
#35669=CARTESIAN_POINT('Ctrl Pts',(-4.33279905653247,0.636309800095181,
9.3453343395105));
#35670=CARTESIAN_POINT('Ctrl Pts',(-4.3894232030314,0.79477268400081,9.38298079613845));
#35671=CARTESIAN_POINT('Ctrl Pts',(-4.41497954531572,1.06847604194723,9.45099021661041));
#35672=CARTESIAN_POINT('Ctrl Pts',(-4.41583873375347,1.18514270861599,9.48255089471637));
#35673=CARTESIAN_POINT('Ctrl Pts',(-4.40649471700977,1.30000000000624,9.51623349280305));
#35674=CARTESIAN_POINT('Ctrl Pts',(-4.52671929080664,-1.30000000000149,
9.29988940418204));
#35675=CARTESIAN_POINT('Ctrl Pts',(-4.53102612742524,-1.18514270861278,
9.27874990296268));
#35676=CARTESIAN_POINT('Ctrl Pts',(-4.52364278147363,-1.0684760419456,9.26235785230968));
#35677=CARTESIAN_POINT('Ctrl Pts',(-4.47957911494204,-0.794772684000821,
9.23545649661536));
#35678=CARTESIAN_POINT('Ctrl Pts',(-4.4081738110316,-0.636309800095175,
9.22897113594562));
#35679=CARTESIAN_POINT('Ctrl Pts',(-4.33199896083579,-0.319434907277148,
9.22979738586081));
#35680=CARTESIAN_POINT('Ctrl Pts',(-4.28164817918848,-0.158333333333327,
9.23714176846705));
#35681=CARTESIAN_POINT('Ctrl Pts',(-4.26780528345959,0.158333333333329,
9.26608248702132));
#35682=CARTESIAN_POINT('Ctrl Pts',(-4.30383410908715,0.319434907277155,
9.28882617419779));
#35683=CARTESIAN_POINT('Ctrl Pts',(-4.35278778872378,0.636309800095183,
9.34461301233644));
#35684=CARTESIAN_POINT('Ctrl Pts',(-4.4100974176126,0.794772684000813,9.38158476192281));
#35685=CARTESIAN_POINT('Ctrl Pts',(-4.43287220873722,1.06847604194723,9.44983783067013));
#35686=CARTESIAN_POINT('Ctrl Pts',(-4.4317793571628,1.18514270861599,9.48172130387332));
#35687=CARTESIAN_POINT('Ctrl Pts',(-4.41973529082518,1.30000000000624,9.51594402584412));
#35688=CARTESIAN_POINT('Ctrl Pts',(-4.55256722381233,-1.30000000000151,
9.29671431789035));
#35689=CARTESIAN_POINT('Ctrl Pts',(-4.56202663520296,-1.1851427086128,9.27432544232462));
#35690=CARTESIAN_POINT('Ctrl Pts',(-4.55836291693832,-1.06847604194562,
9.25723560809462));
#35691=CARTESIAN_POINT('Ctrl Pts',(-4.51958194004603,-0.794772684000833,
9.2299965177689));
#35692=CARTESIAN_POINT('Ctrl Pts',(-4.44686126006357,-0.636309800095181,
9.22530520419382));
#35693=CARTESIAN_POINT('Ctrl Pts',(-4.37054477627713,-0.319434907277149,
9.22743480805897));
#35694=CARTESIAN_POINT('Ctrl Pts',(-4.31842629925649,-0.158333333333328,
9.23551089484534));
#35695=CARTESIAN_POINT('Ctrl Pts',(-4.30444631564053,0.15833333333333,9.26503516002087));
#35696=CARTESIAN_POINT('Ctrl Pts',(-4.3421776205791,0.319434907277159,9.28733307489918));
#35697=CARTESIAN_POINT('Ctrl Pts',(-4.39084729791894,0.63630980009519,9.34361142133363));
#35698=CARTESIAN_POINT('Ctrl Pts',(-4.44872689766476,0.794772684000818,
9.38177011967397));
#35699=CARTESIAN_POINT('Ctrl Pts',(-4.46636044443875,1.06847604194724,9.45001957626592));
#35700=CARTESIAN_POINT('Ctrl Pts',(-4.46182716187524,1.185142708616,9.48162162355187));
#35701=CARTESIAN_POINT('Ctrl Pts',(-4.445127687737,1.30000000000626,9.51528305725643));
#35702=CARTESIAN_POINT('Ctrl Pts',(-4.57797014782426,-1.30000000000154,
9.29362607769095));
#35703=CARTESIAN_POINT('Ctrl Pts',(-4.59241718008654,-1.18514270861282,
9.27026660930158));
#35704=CARTESIAN_POINT('Ctrl Pts',(-4.59237508839258,-1.06847604194564,
9.25259577777905));
#35705=CARTESIAN_POINT('Ctrl Pts',(-4.55880507328098,-0.794772684000851,
9.22491451109467));
#35706=CARTESIAN_POINT('Ctrl Pts',(-4.48498896022062,-0.636309800095197,
9.22122561337946));
#35707=CARTESIAN_POINT('Ctrl Pts',(-4.40861628632671,-0.319434907277159,
9.22434212977147));
#35708=CARTESIAN_POINT('Ctrl Pts',(-4.35474635534818,-0.158333333333332,
9.23324621499998));
#35709=CARTESIAN_POINT('Ctrl Pts',(-4.34059295810106,0.158333333333334,
9.26352342953991));
#35710=CARTESIAN_POINT('Ctrl Pts',(-4.37977441558119,0.319434907277167,
9.28618064357722));
#35711=CARTESIAN_POINT('Ctrl Pts',(-4.42840755015825,0.636309800095206,
9.34212104504176));
#35712=CARTESIAN_POINT('Ctrl Pts',(-4.48773430817405,0.79477268400084,9.37842616946321));
#35713=CARTESIAN_POINT('Ctrl Pts',(-4.50009761851219,1.06847604194727,9.44731322539085));
#35714=CARTESIAN_POINT('Ctrl Pts',(-4.49184486495908,1.18514270861603,9.47972503089479));
#35715=CARTESIAN_POINT('Ctrl Pts',(-4.46998773891322,1.30000000000629,9.51472998790827));
#35716=CARTESIAN_POINT('Ctrl Pts',(-4.59077270268374,-1.30000000000154,
9.29167068805624));
#35717=CARTESIAN_POINT('Ctrl Pts',(-4.60766161389343,-1.18514270861282,
9.26800173905256));
#35718=CARTESIAN_POINT('Ctrl Pts',(-4.60940251578967,-1.06847604194564,
9.25012893617775));
#35719=CARTESIAN_POINT('Ctrl Pts',(-4.57842941557334,-0.794772684000851,
9.22222944316779));
#35720=CARTESIAN_POINT('Ctrl Pts',(-4.50418204215329,-0.636309800095197,
9.2185802642803));
#35721=CARTESIAN_POINT('Ctrl Pts',(-4.42777734501206,-0.319434907277159,
9.22222011637217));
#35722=CARTESIAN_POINT('Ctrl Pts',(-4.37292795574625,-0.158333333333332,
9.23198243022416));
#35723=CARTESIAN_POINT('Ctrl Pts',(-4.35867257917563,0.158333333333334,
9.26271831194325));
#35724=CARTESIAN_POINT('Ctrl Pts',(-4.39869447984769,0.319434907277167,
9.28512064988622));
#35725=CARTESIAN_POINT('Ctrl Pts',(-4.44722735233343,0.636309800095206,
9.34117727402952));
#35726=CARTESIAN_POINT('Ctrl Pts',(-4.50695309467615,0.79477268400084,9.37766731592182));
#35727=CARTESIAN_POINT('Ctrl Pts',(-4.51674956614754,1.06847604194727,9.44670173557987));
#35728=CARTESIAN_POINT('Ctrl Pts',(-4.50675280587843,1.18514270861603,9.47916239086454));
#35729=CARTESIAN_POINT('Ctrl Pts',(-4.48251875583523,1.30000000000629,9.51420125914098));
#35730=CARTESIAN_POINT('',(-4.38971485813411,1.2,9.48755403526923));
#35731=CARTESIAN_POINT('Ctrl Pts',(-4.38971485813412,1.2,9.48755403526923));
#35732=CARTESIAN_POINT('Ctrl Pts',(-4.36856465842126,1.21681404005281,9.49175671093172));
#35733=CARTESIAN_POINT('Ctrl Pts',(-4.34727912103697,1.23316506853804,9.49708784014508));
#35734=CARTESIAN_POINT('Ctrl Pts',(-4.31570563125357,1.25821670499925,9.50310064771019));
#35735=CARTESIAN_POINT('Ctrl Pts',(-4.30530467128022,1.26642476319251,9.50514734277103));
#35736=CARTESIAN_POINT('Ctrl Pts',(-4.28380750759288,1.28334467201644,9.50941095015061));
#35737=CARTESIAN_POINT('Ctrl Pts',(-4.27227103446103,1.29250131658665,9.51149917491571));
#35738=CARTESIAN_POINT('Ctrl Pts',(-4.26286793819922,1.30000000000626,9.51310547563494));
#35739=CARTESIAN_POINT('',(-4.45989076530874,0.653834841369816,9.34752749950966));
#35740=CARTESIAN_POINT('Ctrl Pts',(-4.45989076533968,0.653834841368558,
9.34752749953006));
#35741=CARTESIAN_POINT('Ctrl Pts',(-4.4528848487179,0.717482614179447,9.36207707938459));
#35742=CARTESIAN_POINT('Ctrl Pts',(-4.44710663293816,0.764240546950704,
9.37394135883623));
#35743=CARTESIAN_POINT('Ctrl Pts',(-4.42419760792246,0.949850583838299,
9.42040738323249));
#35744=CARTESIAN_POINT('Ctrl Pts',(-4.40997428413873,1.05891269470216,9.44867709423153));
#35745=CARTESIAN_POINT('Ctrl Pts',(-4.38971485813412,1.2,9.48755403526923));
#35746=CARTESIAN_POINT('',(-4.51863764645995,-0.653834841531101,9.22099327559368));
#35747=CARTESIAN_POINT('Ctrl Pts',(-4.51863764645995,-0.6538348415311,9.22099327559368));
#35748=CARTESIAN_POINT('Ctrl Pts',(-4.47706062852027,-0.57596586359716,
9.22158151376161));
#35749=CARTESIAN_POINT('Ctrl Pts',(-4.44193143807525,-0.49363919130031,
9.22283656802191));
#35750=CARTESIAN_POINT('Ctrl Pts',(-4.39150077182074,-0.338139586062805,
9.22708011483244));
#35751=CARTESIAN_POINT('Ctrl Pts',(-4.37382131335729,-0.265665248839193,
9.22980161915001));
#35752=CARTESIAN_POINT('Ctrl Pts',(-4.35075762524346,-0.129721413745824,
9.23768769470636));
#35753=CARTESIAN_POINT('Ctrl Pts',(-4.34396312512813,-0.0666272124195298,
9.24241374472171));
#35754=CARTESIAN_POINT('Ctrl Pts',(-4.33801561083273,0.059547323378811,
9.25434173739283));
#35755=CARTESIAN_POINT('Ctrl Pts',(-4.33880352141602,0.12278345398452,9.26162381306405));
#35756=CARTESIAN_POINT('Ctrl Pts',(-4.34923310016955,0.260138689594822,
9.27954883606279));
#35757=CARTESIAN_POINT('Ctrl Pts',(-4.36046457083349,0.333955905815987,
9.29056690922749));
#35758=CARTESIAN_POINT('Ctrl Pts',(-4.39723646550573,0.491216885915717,
9.31624550765387));
#35759=CARTESIAN_POINT('Ctrl Pts',(-4.42491449632406,0.574353373727776,
9.33143546434627));
#35760=CARTESIAN_POINT('Ctrl Pts',(-4.4598907652581,0.653834841386376,9.34752749953792));
#35761=CARTESIAN_POINT('',(-4.48863561636269,-1.2,9.28677988861316));
#35762=CARTESIAN_POINT('Ctrl Pts',(-4.48863561636269,-1.2,9.28677988861316));
#35763=CARTESIAN_POINT('Ctrl Pts',(-4.4944288750257,-1.12734343599548,9.27431866675094));
#35764=CARTESIAN_POINT('Ctrl Pts',(-4.50105363556384,-1.03203660304106,
9.25993526667585));
#35765=CARTESIAN_POINT('Ctrl Pts',(-4.51377570799241,-0.796458044101793,
9.23187056708943));
#35766=CARTESIAN_POINT('Ctrl Pts',(-4.51600510749749,-0.740055726332444,
9.22687923761306));
#35767=CARTESIAN_POINT('Ctrl Pts',(-4.51863764645995,-0.653834841531101,
9.22099327559368));
#35768=CARTESIAN_POINT('Ctrl Pts',(-4.36615556544122,-1.29999999999999,
9.31167837948083));
#35769=CARTESIAN_POINT('Ctrl Pts',(-4.37511427302833,-1.29262032296144,
9.31010442892759));
#35770=CARTESIAN_POINT('Ctrl Pts',(-4.38551309604794,-1.28397999449773,
9.30842771658611));
#35771=CARTESIAN_POINT('Ctrl Pts',(-4.40673157410085,-1.26674695084208,
9.30402510739829));
#35772=CARTESIAN_POINT('Ctrl Pts',(-4.41749867593977,-1.25800032086002,
9.30176293427779));
#35773=CARTESIAN_POINT('Ctrl Pts',(-4.44091918379889,-1.2387128136161,9.29738790117898));
#35774=CARTESIAN_POINT('Ctrl Pts',(-4.46310927593388,-1.22042691903373,
9.29323250571027));
#35775=CARTESIAN_POINT('Ctrl Pts',(-4.48863561636269,-1.2,9.28677988861316));
#35776=CARTESIAN_POINT('Origin',(0.,1.25,7.2));
#35777=CARTESIAN_POINT('Origin',(0.,1.2,7.2));
#35778=CARTESIAN_POINT('Origin',(0.,0.92691742076555,7.2));
#35779=CARTESIAN_POINT('Origin',(0.,0.653834841531101,7.2));
#35780=CARTESIAN_POINT('Origin',(0.,0.,7.2));
#35781=CARTESIAN_POINT('Origin',(0.,-0.653834841531101,7.2));
#35782=CARTESIAN_POINT('Origin',(0.,-0.926917420765551,7.2));
#35783=CARTESIAN_POINT('Origin',(0.,-1.2,7.2));
#35784=CARTESIAN_POINT('Origin',(0.,-1.25,7.2));
#35785=CARTESIAN_POINT('Ctrl Pts',(-4.71917718395474,-1.30000000000184,
8.98265772674134));
#35786=CARTESIAN_POINT('Ctrl Pts',(-4.70935397490598,-1.18514270861303,
9.02411271480684));
#35787=CARTESIAN_POINT('Ctrl Pts',(-4.69192014516097,-1.06847604194575,
9.05326217342547));
#35788=CARTESIAN_POINT('Ctrl Pts',(-4.63406245451663,-0.794772684000851,
9.0921750194286));
#35789=CARTESIAN_POINT('Ctrl Pts',(-4.56698074651016,-0.636309800095196,
9.07220674691498));
#35790=CARTESIAN_POINT('Ctrl Pts',(-4.49284772594841,-0.319434907277159,
9.07364899676464));
#35791=CARTESIAN_POINT('Ctrl Pts',(-4.44941966576432,-0.158333333333332,
9.05889701834648));
#35792=CARTESIAN_POINT('Ctrl Pts',(-4.43611716307696,0.158333333333335,
9.09005714685184));
#35793=CARTESIAN_POINT('Ctrl Pts',(-4.46556375515151,0.319434907277167,
9.13735044965271));
#35794=CARTESIAN_POINT('Ctrl Pts',(-4.51398353922898,0.636309800095206,
9.19656574141201));
#35795=CARTESIAN_POINT('Ctrl Pts',(-4.56637659762912,0.794772684000841,
9.24930051549101));
#35796=CARTESIAN_POINT('Ctrl Pts',(-4.60783501082195,1.06847604194523,9.25364960997122));
#35797=CARTESIAN_POINT('Ctrl Pts',(-4.61995220105506,1.18514270861202,9.24039662831112));
#35798=CARTESIAN_POINT('Ctrl Pts',(-4.6262407706357,1.30000000000035,9.21200810314026));
#35799=CARTESIAN_POINT('Ctrl Pts',(-4.71118521909806,-1.30000000000184,
8.97299157777347));
#35800=CARTESIAN_POINT('Ctrl Pts',(-4.69979673845635,-1.18514270861303,
9.01265747601402));
#35801=CARTESIAN_POINT('Ctrl Pts',(-4.68123224291413,-1.06847604194575,
9.04047819818707));
#35802=CARTESIAN_POINT('Ctrl Pts',(-4.62176651442011,-0.794772684000851,
9.0773849055878));
#35803=CARTESIAN_POINT('Ctrl Pts',(-4.55508919945686,-0.636309800095196,
9.05758940225795));
#35804=CARTESIAN_POINT('Ctrl Pts',(-4.48097546072877,-0.319434907277159,
9.05887937469646));
#35805=CARTESIAN_POINT('Ctrl Pts',(-4.43792035696632,-0.158333333333332,
9.04492251268587));
#35806=CARTESIAN_POINT('Ctrl Pts',(-4.42489047293301,0.158333333333335,
9.07569994753693));
#35807=CARTESIAN_POINT('Ctrl Pts',(-4.45431946765658,0.319434907277167,
9.12169110394353));
#35808=CARTESIAN_POINT('Ctrl Pts',(-4.50310673819832,0.636309800095206,
9.18053241785163));
#35809=CARTESIAN_POINT('Ctrl Pts',(-4.5552407438893,0.794772684000839,9.2329201259259));
#35810=CARTESIAN_POINT('Ctrl Pts',(-4.59827465855662,1.06847604194523,9.23934512618654));
#35811=CARTESIAN_POINT('Ctrl Pts',(-4.61143481041735,1.18514270861202,9.22755231220432));
#35812=CARTESIAN_POINT('Ctrl Pts',(-4.619127327043,1.30000000000036,9.20118553969676));
#35813=CARTESIAN_POINT('Ctrl Pts',(-4.69495064211116,-1.30000000000059,
8.95419085396944));
#35814=CARTESIAN_POINT('Ctrl Pts',(-4.68128463589822,-1.18514270861189,
8.98882994277146));
#35815=CARTESIAN_POINT('Ctrl Pts',(-4.66093855700018,-1.06847604194472,
9.01316614706116));
#35816=CARTESIAN_POINT('Ctrl Pts',(-4.59850274028019,-0.794772684000084,
9.04558592310283));
#35817=CARTESIAN_POINT('Ctrl Pts',(-4.53119122967445,-0.636309800094586,
9.02847825346989));
#35818=CARTESIAN_POINT('Ctrl Pts',(-4.45672260605069,-0.319434907276853,
9.03009305916203));
#35819=CARTESIAN_POINT('Ctrl Pts',(-4.41495444464664,-0.15833333333318,
9.01689174836914));
#35820=CARTESIAN_POINT('Ctrl Pts',(-4.40229456280709,0.158333333333182,
9.04714490931517));
#35821=CARTESIAN_POINT('Ctrl Pts',(-4.43103772959592,0.319434907276858,
9.09147270934599));
#35822=CARTESIAN_POINT('Ctrl Pts',(-4.48046279388933,0.636309800094593,
9.14970250735217));
#35823=CARTESIAN_POINT('Ctrl Pts',(-4.5326729724665,0.794772684000079,9.20051480885182));
#35824=CARTESIAN_POINT('Ctrl Pts',(-4.57885430690899,1.06847604194421,9.21113198619779));
#35825=CARTESIAN_POINT('Ctrl Pts',(-4.59399225125184,1.18514270861088,9.20244350937703));
#35826=CARTESIAN_POINT('Ctrl Pts',(-4.60427795144447,1.29999999999911,9.18047077306761));
#35827=CARTESIAN_POINT('Ctrl Pts',(-4.67856627830505,-1.29999999999933,
8.93502616643288));
#35828=CARTESIAN_POINT('Ctrl Pts',(-4.66121991197996,-1.18514270861074,
8.96689761340208));
#35829=CARTESIAN_POINT('Ctrl Pts',(-4.63827918184726,-1.06847604194369,
8.98905607801689));
#35830=CARTESIAN_POINT('Ctrl Pts',(-4.57235740641933,-0.794772683999317,
9.01780763174861));
#35831=CARTESIAN_POINT('Ctrl Pts',(-4.50654676965981,-0.636309800093967,
8.99992851636126));
#35832=CARTESIAN_POINT('Ctrl Pts',(-4.43234600151776,-0.319434907276541,
9.00085303067297));
#35833=CARTESIAN_POINT('Ctrl Pts',(-4.39134027920529,-0.158333333333026,
8.98925773605429));
#35834=CARTESIAN_POINT('Ctrl Pts',(-4.37907445022117,0.158333333333029,
9.01894067946668));
#35835=CARTESIAN_POINT('Ctrl Pts',(-4.40727167410129,0.31943490727655,9.06135701309618));
#35836=CARTESIAN_POINT('Ctrl Pts',(-4.45759321036425,0.636309800093976,
9.11857629848427));
#35837=CARTESIAN_POINT('Ctrl Pts',(-4.51018664253024,0.794772683999303,
9.16732445132942));
#35838=CARTESIAN_POINT('Ctrl Pts',(-4.5596318477288,1.06847604194317,9.18205049763488));
#35839=CARTESIAN_POINT('Ctrl Pts',(-4.57673844140366,1.18514270860973,9.17654629265128));
#35840=CARTESIAN_POINT('Ctrl Pts',(-4.58954863154836,1.29999999999785,9.15916352289222));
#35841=CARTESIAN_POINT('Ctrl Pts',(-4.6701509419572,-1.29999999999917,8.92533046634025));
#35842=CARTESIAN_POINT('Ctrl Pts',(-4.65142766969827,-1.1851427086106,8.95492352907192));
#35843=CARTESIAN_POINT('Ctrl Pts',(-4.62744617719791,-1.06847604194356,
8.97547310910894));
#35844=CARTESIAN_POINT('Ctrl Pts',(-4.55989659138003,-0.794772683999221,
9.00205449575667));
#35845=CARTESIAN_POINT('Ctrl Pts',(-4.49408411031015,-0.63630980009389,
8.98504509224385));
#35846=CARTESIAN_POINT('Ctrl Pts',(-4.41966049746464,-0.319434907276502,
8.98619857882796));
#35847=CARTESIAN_POINT('Ctrl Pts',(-4.37898964047838,-0.158333333333007,
8.97552017176666));
#35848=CARTESIAN_POINT('Ctrl Pts',(-4.36691509201292,0.15833333333301,9.00492423313939));
#35849=CARTESIAN_POINT('Ctrl Pts',(-4.39510610028442,0.319434907276512,
9.0459240393071));
#35850=CARTESIAN_POINT('Ctrl Pts',(-4.44576029472738,0.6363098000939,9.10279595766359));
#35851=CARTESIAN_POINT('Ctrl Pts',(-4.49799652989938,0.794772683999208,
9.15130408714472));
#35852=CARTESIAN_POINT('Ctrl Pts',(-4.54911845680959,1.06847604194304,9.16813305033091));
#35853=CARTESIAN_POINT('Ctrl Pts',(-4.56735662103664,1.18514270860958,9.16408323843005));
#35854=CARTESIAN_POINT('Ctrl Pts',(-4.58170416158539,1.29999999999769,9.14869898003955));
#35855=CARTESIAN_POINT('Ctrl Pts',(-4.66976691393927,-1.29999999999918,
8.92489233702175));
#35856=CARTESIAN_POINT('Ctrl Pts',(-4.65098084725317,-1.1851427086106,8.95438205260471));
#35857=CARTESIAN_POINT('Ctrl Pts',(-4.62695198669783,-1.06847604194356,
8.97485851129906));
#35858=CARTESIAN_POINT('Ctrl Pts',(-4.55932860920279,-0.794772683999223,
9.00134080067594));
#35859=CARTESIAN_POINT('Ctrl Pts',(-4.49351714732034,-0.636309800093892,
8.98436918385726));
#35860=CARTESIAN_POINT('Ctrl Pts',(-4.41908317169223,-0.319434907276503,
8.98553341344849));
#35861=CARTESIAN_POINT('Ctrl Pts',(-4.37842602012149,-0.158333333333007,
8.9748991022583));
#35862=CARTESIAN_POINT('Ctrl Pts',(-4.36636003466096,0.15833333333301,9.00429066709948));
#35863=CARTESIAN_POINT('Ctrl Pts',(-4.39455172304245,0.319434907276513,
9.04522449790572));
#35864=CARTESIAN_POINT('Ctrl Pts',(-4.44522186243731,0.636309800093902,
9.10207933113157));
#35865=CARTESIAN_POINT('Ctrl Pts',(-4.49744245446759,0.79477268399921,9.1505756752673));
#35866=CARTESIAN_POINT('Ctrl Pts',(-4.54864086351237,1.06847604194304,9.16749987030133));
#35867=CARTESIAN_POINT('Ctrl Pts',(-4.56693044085057,1.18514270860959,9.16351623316231));
#35868=CARTESIAN_POINT('Ctrl Pts',(-4.58134770133951,1.29999999999769,9.14822310195727));
#35869=CARTESIAN_POINT('Ctrl Pts',(-4.66938288464626,-1.29999999999917,
8.92445418124858));
#35870=CARTESIAN_POINT('Ctrl Pts',(-4.65053373614899,-1.1851427086106,8.95384105559867));
#35871=CARTESIAN_POINT('Ctrl Pts',(-4.62645731659445,-1.06847604194356,
8.97424472842433));
#35872=CARTESIAN_POINT('Ctrl Pts',(-4.55875992909808,-0.794772683999222,
9.00062830178755));
#35873=CARTESIAN_POINT('Ctrl Pts',(-4.49294953019207,-0.636309800093891,
8.98369436139404));
#35874=CARTESIAN_POINT('Ctrl Pts',(-4.41850559492078,-0.319434907276503,
8.98486867585451));
#35875=CARTESIAN_POINT('Ctrl Pts',(-4.37786298007624,-0.158333333333007,
8.97427713099188));
#35876=CARTESIAN_POINT('Ctrl Pts',(-4.3658055989932,0.15833333333301,9.00365612250243));
#35877=CARTESIAN_POINT('Ctrl Pts',(-4.39399706732632,0.319434907276513,
9.04452539926505));
#35878=CARTESIAN_POINT('Ctrl Pts',(-4.44468305731729,0.636309800093901,
9.10136330569213));
#35879=CARTESIAN_POINT('Ctrl Pts',(-4.49688870555336,0.794772683999209,
9.14984678924392));
#35880=CARTESIAN_POINT('Ctrl Pts',(-4.5481636859491,1.06847604194304,9.16686606916854));
#35881=CARTESIAN_POINT('Ctrl Pts',(-4.56650460819516,1.18514270860959,9.16294870394952));
#35882=CARTESIAN_POINT('Ctrl Pts',(-4.58099141359925,1.29999999999769,9.14774695785857));
#35883=CARTESIAN_POINT('Ctrl Pts',(-4.66861347039935,-1.29999999999918,
8.92358013837401));
#35884=CARTESIAN_POINT('Ctrl Pts',(-4.64963749040481,-1.1851427086106,8.95276236609815));
#35885=CARTESIAN_POINT('Ctrl Pts',(-4.6254655903302,-1.06847604194356,8.97302101570254));
#35886=CARTESIAN_POINT('Ctrl Pts',(-4.55762005076071,-0.794772683999223,
8.99920729840525));
#35887=CARTESIAN_POINT('Ctrl Pts',(-4.49181298717508,-0.636309800093892,
8.98234672987362));
#35888=CARTESIAN_POINT('Ctrl Pts',(-4.4173495517368,-0.319434907276503,
8.9835404905542));
#35889=CARTESIAN_POINT('Ctrl Pts',(-4.37673580888741,-0.158333333333008,
8.97303479950824));
#35890=CARTESIAN_POINT('Ctrl Pts',(-4.36469554604491,0.15833333333301,9.00238874670316));
#35891=CARTESIAN_POINT('Ctrl Pts',(-4.39288607310709,0.319434907276513,
9.04312964025067));
#35892=CARTESIAN_POINT('Ctrl Pts',(-4.44360440763777,0.636309800093902,
9.09993270284471));
#35893=CARTESIAN_POINT('Ctrl Pts',(-4.49578189097155,0.79477268399921,9.14838786158691));
#35894=CARTESIAN_POINT('Ctrl Pts',(-4.54721036505604,1.06847604194304,9.16559680985666));
#35895=CARTESIAN_POINT('Ctrl Pts',(-4.56565380824756,1.18514270860959,9.16181226444056));
#35896=CARTESIAN_POINT('Ctrl Pts',(-4.5802792138122,1.29999999999769,9.14679405755677));
#35897=CARTESIAN_POINT('Ctrl Pts',(-4.66694146222015,-1.29999999999918,
8.92169446539642));
#35898=CARTESIAN_POINT('Ctrl Pts',(-4.64768643612071,-1.18514270861061,
8.95044021925838));
#35899=CARTESIAN_POINT('Ctrl Pts',(-4.62330517815074,-1.06847604194356,
8.97038867822463));
#35900=CARTESIAN_POINT('Ctrl Pts',(-4.55513697366628,-0.794772683999226,
8.99615009801027));
#35901=CARTESIAN_POINT('Ctrl Pts',(-4.4893423677817,-0.636309800093895,
8.97943975591989));
#35902=CARTESIAN_POINT('Ctrl Pts',(-4.41484050350011,-0.319434907276505,
8.98066927837885));
#35903=CARTESIAN_POINT('Ctrl Pts',(-4.3742927596087,-0.158333333333008,
8.9703440922254));
#35904=CARTESIAN_POINT('Ctrl Pts',(-4.36228947202549,0.158333333333011,
8.99964374619661));
#35905=CARTESIAN_POINT('Ctrl Pts',(-4.39047144214751,0.319434907276514,
9.04011650144985));
#35906=CARTESIAN_POINT('Ctrl Pts',(-4.44126183214889,0.636309800093905,
9.09684112242019));
#35907=CARTESIAN_POINT('Ctrl Pts',(-4.4933884427905,0.794772683999213,9.14521954990681));
#35908=CARTESIAN_POINT('Ctrl Pts',(-4.5451512764238,1.06847604194305,9.16283677826069));
#35909=CARTESIAN_POINT('Ctrl Pts',(-4.56381585087666,1.18514270860959,9.1593415406099));
#35910=CARTESIAN_POINT('Ctrl Pts',(-4.57873878710452,1.2999999999977,9.14472521993657));
#35911=CARTESIAN_POINT('Ctrl Pts',(-4.66383012966025,-1.29999999999921,
8.9182524003141));
#35912=CARTESIAN_POINT('Ctrl Pts',(-4.64403034108178,-1.18514270861063,
8.94624124721707));
#35913=CARTESIAN_POINT('Ctrl Pts',(-4.61924529166989,-1.06847604194358,
8.96564550953633));
#35914=CARTESIAN_POINT('Ctrl Pts',(-4.55046991947324,-0.794772683999241,
8.99064112957451));
#35915=CARTESIAN_POINT('Ctrl Pts',(-4.48473463973545,-0.636309800093906,
8.97414722434077));
#35916=CARTESIAN_POINT('Ctrl Pts',(-4.41018948450046,-0.31943490727651,
8.97539711220255));
#35917=CARTESIAN_POINT('Ctrl Pts',(-4.36979011905288,-0.158333333333011,
8.96536307830696));
#35918=CARTESIAN_POINT('Ctrl Pts',(-4.35785324122113,0.158333333333013,
8.9945642572073));
#35919=CARTESIAN_POINT('Ctrl Pts',(-4.385970225677,0.31943490727652,9.03461780582221));
#35920=CARTESIAN_POINT('Ctrl Pts',(-4.43690458531225,0.636309800093916,
9.0911817256847));
#35921=CARTESIAN_POINT('Ctrl Pts',(-4.48900848213158,0.794772683999227,
9.13931103832431));
#35922=CARTESIAN_POINT('Ctrl Pts',(-4.54139807333501,1.06847604194306,9.15766798960639));
#35923=CARTESIAN_POINT('Ctrl Pts',(-4.56046217222793,1.18514270860961,9.15472013499506));
#35924=CARTESIAN_POINT('Ctrl Pts',(-4.57591285720746,1.29999999999772,9.14087838175445));
#35925=CARTESIAN_POINT('Ctrl Pts',(-4.66068107962505,-1.29999999999924,
8.91486837523097));
#35926=CARTESIAN_POINT('Ctrl Pts',(-4.64027435180129,-1.18514270861066,
8.94220381448194));
#35927=CARTESIAN_POINT('Ctrl Pts',(-4.6150485220739,-1.06847604194361,8.961125420333));
#35928=CARTESIAN_POINT('Ctrl Pts',(-4.54563871953845,-0.794772683999263,
8.98540047676775));
#35929=CARTESIAN_POINT('Ctrl Pts',(-4.48003079702452,-0.636309800093924,
8.96900863205523));
#35930=CARTESIAN_POINT('Ctrl Pts',(-4.40550277551653,-0.319434907276519,
8.97017988484825));
#35931=CARTESIAN_POINT('Ctrl Pts',(-4.36532033989244,-0.158333333333015,
8.9603283847655));
#35932=CARTESIAN_POINT('Ctrl Pts',(-4.35344807657413,0.158333333333018,
8.98943145542105));
#35933=CARTESIAN_POINT('Ctrl Pts',(-4.38139047634244,0.319434907276529,
9.02923464366669));
#35934=CARTESIAN_POINT('Ctrl Pts',(-4.4324846784807,0.636309800093934,9.08561567754849));
#35935=CARTESIAN_POINT('Ctrl Pts',(-4.48470648986488,0.79477268399925,9.13328477364608));
#35936=CARTESIAN_POINT('Ctrl Pts',(-4.53774240678189,1.06847604194309,9.15235208885783));
#35937=CARTESIAN_POINT('Ctrl Pts',(-4.55718993418727,1.18514270860965,9.14997562706888));
#35938=CARTESIAN_POINT('Ctrl Pts',(-4.57312770573906,1.29999999999776,9.13696916924947));
#35939=CARTESIAN_POINT('Ctrl Pts',(-4.65646846761001,-1.29999999999927,
8.91037603753981));
#35940=CARTESIAN_POINT('Ctrl Pts',(-4.6352269128868,-1.18514270861068,8.93688219706871));
#35941=CARTESIAN_POINT('Ctrl Pts',(-4.60939692572218,-1.06847604194363,
8.95518720285638));
#35942=CARTESIAN_POINT('Ctrl Pts',(-4.53912429124843,-0.794772683999279,
8.9785291223523));
#35943=CARTESIAN_POINT('Ctrl Pts',(-4.47370568965768,-0.636309800093937,
8.96224085178219));
#35944=CARTESIAN_POINT('Ctrl Pts',(-4.39921677806005,-0.319434907276526,
8.96328101300153));
#35945=CARTESIAN_POINT('Ctrl Pts',(-4.35934575137206,-0.158333333333019,
8.95363882849874));
#35946=CARTESIAN_POINT('Ctrl Pts',(-4.34755960691698,0.158333333333021,
8.98260930693076));
#35947=CARTESIAN_POINT('Ctrl Pts',(-4.37523520704753,0.319434907276536,
9.02212829560295));
#35948=CARTESIAN_POINT('Ctrl Pts',(-4.42655026919399,0.636309800093947,
9.07825279273653));
#35949=CARTESIAN_POINT('Ctrl Pts',(-4.478975712082,0.794772683999266,9.1252385327736));
#35950=CARTESIAN_POINT('Ctrl Pts',(-4.53288438138959,1.06847604194312,9.14523718484589));
#35951=CARTESIAN_POINT('Ctrl Pts',(-4.55284054409227,1.18514270860967,9.14362704630053));
#35952=CARTESIAN_POINT('Ctrl Pts',(-4.56941780406742,1.29999999999779,9.1317500937508));
#35953=CARTESIAN_POINT('Ctrl Pts',(-4.65173281621968,-1.29999999999929,
8.90531318004771));
#35954=CARTESIAN_POINT('Ctrl Pts',(-4.62955463356647,-1.18514270861071,
8.93088072622139));
#35955=CARTESIAN_POINT('Ctrl Pts',(-4.60304276398764,-1.06847604194366,
8.94849480373194));
#35956=CARTESIAN_POINT('Ctrl Pts',(-4.53178335783007,-0.794772683999295,
8.97081274276759));
#35957=CARTESIAN_POINT('Ctrl Pts',(-4.46654428001928,-0.636309800093951,
8.95469810355981));
#35958=CARTESIAN_POINT('Ctrl Pts',(-4.39208112856424,-0.319434907276533,
8.95562126723687));
#35959=CARTESIAN_POINT('Ctrl Pts',(-4.35255944184997,-0.158333333333022,
8.94621635495254));
#35960=CARTESIAN_POINT('Ctrl Pts',(-4.34088102723102,0.158333333333025,
8.97501821684063));
#35961=CARTESIAN_POINT('Ctrl Pts',(-4.36829040143653,0.319434907276542,
9.01415991626995));
#35962=CARTESIAN_POINT('Ctrl Pts',(-4.41984928194637,0.63630980009396,9.06999969602464));
#35963=CARTESIAN_POINT('Ctrl Pts',(-4.47244306656148,0.794772683999283,
9.11631047386423));
#35964=CARTESIAN_POINT('Ctrl Pts',(-4.52734909122831,1.06847604194314,9.13733324890494));
#35965=CARTESIAN_POINT('Ctrl Pts',(-4.54789985251689,1.1851427086097,9.1365511894133));
#35966=CARTESIAN_POINT('Ctrl Pts',(-4.56523459148449,1.29999999999781,9.12588709008547));
#35967=CARTESIAN_POINT('Ctrl Pts',(-4.64344920784895,-1.29999999999938,
8.89608889763532));
#35968=CARTESIAN_POINT('Ctrl Pts',(-4.61980770460998,-1.18514270861078,
8.91964675638172));
#35969=CARTESIAN_POINT('Ctrl Pts',(-4.59219580800188,-1.06847604194373,
8.93584234783779));
#35970=CARTESIAN_POINT('Ctrl Pts',(-4.51923440013915,-0.794772683999346,
8.95624909376107));
#35971=CARTESIAN_POINT('Ctrl Pts',(-4.45405596235386,-0.636309800093991,
8.94088045270961));
#35972=CARTESIAN_POINT('Ctrl Pts',(-4.37935657175661,-0.319434907276553,
8.94206055169668));
#35973=CARTESIAN_POINT('Ctrl Pts',(-4.34013166891365,-0.158333333333032,
8.93360300549307));
#35974=CARTESIAN_POINT('Ctrl Pts',(-4.32863106798455,0.158333333333035,
8.96212981746688));
#35975=CARTESIAN_POINT('Ctrl Pts',(-4.35601081266152,0.319434907276562,
8.99989490221463));
#35976=CARTESIAN_POINT('Ctrl Pts',(-4.40798614551958,0.636309800094001,
9.05523158141004));
#35977=CARTESIAN_POINT('Ctrl Pts',(-4.46040103921712,0.794772683999334,
9.10105041962622));
#35978=CARTESIAN_POINT('Ctrl Pts',(-4.51703295531289,1.06847604194321,9.12397152635148));
#35979=CARTESIAN_POINT('Ctrl Pts',(-4.5387044942274,1.18514270860977,9.12457455335947));
#35980=CARTESIAN_POINT('Ctrl Pts',(-4.55753371399785,1.29999999999789,9.11585890958479));
#35981=CARTESIAN_POINT('Ctrl Pts',(-4.63312481503961,-1.2999999999996,8.8844851501262));
#35982=CARTESIAN_POINT('Ctrl Pts',(-4.60764312208804,-1.18514270861098,
8.90554365189251));
#35983=CARTESIAN_POINT('Ctrl Pts',(-4.57865309865353,-1.06847604194391,
8.91996761939151));
#35984=CARTESIAN_POINT('Ctrl Pts',(-4.50357539983094,-0.79477268399948,
8.93796276842742));
#35985=CARTESIAN_POINT('Ctrl Pts',(-4.43850715508563,-0.6363098000941,8.92347121376613));
#35986=CARTESIAN_POINT('Ctrl Pts',(-4.36355026845127,-0.319434907276608,
8.92491696466319));
#35987=CARTESIAN_POINT('Ctrl Pts',(-4.32475600711511,-0.158333333333059,
8.9175594843186));
#35988=CARTESIAN_POINT('Ctrl Pts',(-4.31342837560234,0.158333333333061,
8.94582352378791));
#35989=CARTESIAN_POINT('Ctrl Pts',(-4.34057580169344,0.319434907276616,
8.98216733508143));
#35990=CARTESIAN_POINT('Ctrl Pts',(-4.39310931357207,0.636309800094108,
9.03682214176766));
#35991=CARTESIAN_POINT('Ctrl Pts',(-4.44556179129244,0.79477268399947,9.08163575589306));
#35992=CARTESIAN_POINT('Ctrl Pts',(-4.50444501918549,1.06847604194339,9.10677955103585));
#35993=CARTESIAN_POINT('Ctrl Pts',(-4.52752445138544,1.18514270860997,9.10909684800232));
#35994=CARTESIAN_POINT('Ctrl Pts',(-4.54819494826906,1.29999999999812,9.10284762468738));
#35995=CARTESIAN_POINT('Ctrl Pts',(-4.6161315750982,-1.29999999999994,8.866720229488));
#35996=CARTESIAN_POINT('Ctrl Pts',(-4.58734282213314,-1.1851427086113,8.8843813116644));
#35997=CARTESIAN_POINT('Ctrl Pts',(-4.55590757304771,-1.06847604194419,
8.89636879561943));
#35998=CARTESIAN_POINT('Ctrl Pts',(-4.47717192359272,-0.794772683999692,
8.91095513475269));
#35999=CARTESIAN_POINT('Ctrl Pts',(-4.41243224464801,-0.636309800094267,
8.89762029551915));
#36000=CARTESIAN_POINT('Ctrl Pts',(-4.33739806449051,-0.319434907276691,
8.8989196168512));
#36001=CARTESIAN_POINT('Ctrl Pts',(-4.29979269678325,-0.158333333333101,
8.89246819235823));
#36002=CARTESIAN_POINT('Ctrl Pts',(-4.2890368109278,0.158333333333103,8.91979970437644));
#36003=CARTESIAN_POINT('Ctrl Pts',(-4.31586211496023,0.319434907276701,
8.95379793509703));
#36004=CARTESIAN_POINT('Ctrl Pts',(-4.36903657855686,0.636309800094277,
9.00773239700906));
#36005=CARTESIAN_POINT('Ctrl Pts',(-4.42091912841294,0.794772683999679,
9.05187752173051));
#36006=CARTESIAN_POINT('Ctrl Pts',(-4.48321977595797,1.06847604194367,9.08089683226442));
#36007=CARTESIAN_POINT('Ctrl Pts',(-4.5085784892226,1.18514270861028,9.08594630258439));
#36008=CARTESIAN_POINT('Ctrl Pts',(-4.5323282738961,1.29999999999846,9.08348385896562));
#36009=CARTESIAN_POINT('Ctrl Pts',(-4.59925616540522,-1.30000000000032,
8.84868787826823));
#36010=CARTESIAN_POINT('Ctrl Pts',(-4.56715847804536,-1.18514270861164,
8.86295398912095));
#36011=CARTESIAN_POINT('Ctrl Pts',(-4.53330573141733,-1.0684760419445,8.87245513260324));
#36012=CARTESIAN_POINT('Ctrl Pts',(-4.45104457648016,-0.79477268399992,
8.88339664689042));
#36013=CARTESIAN_POINT('Ctrl Pts',(-4.38695875673159,-0.636309800094451,
8.87064203255691));
#36014=CARTESIAN_POINT('Ctrl Pts',(-4.31180285795805,-0.319434907276784,
8.87187236007619));
#36015=CARTESIAN_POINT('Ctrl Pts',(-4.27516556234439,-0.158333333333146,
8.86674567150868));
#36016=CARTESIAN_POINT('Ctrl Pts',(-4.26450690044457,0.158333333333149,
8.8939273071107));
#36017=CARTESIAN_POINT('Ctrl Pts',(-4.29033189167834,0.319434907276792,
8.92664269784874));
#36018=CARTESIAN_POINT('Ctrl Pts',(-4.34408982228034,0.636309800094459,
8.97995023961783));
#36019=CARTESIAN_POINT('Ctrl Pts',(-4.39602601489726,0.794772683999908,
9.02244203897655));
#36020=CARTESIAN_POINT('Ctrl Pts',(-4.46216995079192,1.06847604194398,9.05465827179795));
#36021=CARTESIAN_POINT('Ctrl Pts',(-4.48997068438421,1.18514270861063,9.06217871559226));
#36022=CARTESIAN_POINT('Ctrl Pts',(-4.51694089259435,1.29999999999883,9.06327438972156));
#36023=CARTESIAN_POINT('Ctrl Pts',(-4.58213601648041,-1.30000000000044,
8.83109175807416));
#36024=CARTESIAN_POINT('Ctrl Pts',(-4.54681642970871,-1.18514270861175,
8.84177044112995));
#36025=CARTESIAN_POINT('Ctrl Pts',(-4.5105029459682,-1.0684760419446,8.84883487206191));
#36026=CARTESIAN_POINT('Ctrl Pts',(-4.42431543321399,-0.794772683999997,
8.85680547531458));
#36027=CARTESIAN_POINT('Ctrl Pts',(-4.35985910129541,-0.63630980009451,
8.84647000817917));
#36028=CARTESIAN_POINT('Ctrl Pts',(-4.28438268322261,-0.319434907276813,
8.84796957882561));
#36029=CARTESIAN_POINT('Ctrl Pts',(-4.24924643579066,-0.158333333333161,
8.84319498291508));
#36030=CARTESIAN_POINT('Ctrl Pts',(-4.23918044863051,0.158333333333164,
8.86934531494356));
#36031=CARTESIAN_POINT('Ctrl Pts',(-4.26434527221524,0.319434907276823,
8.90018990350982));
#36032=CARTESIAN_POINT('Ctrl Pts',(-4.31912538055828,0.636309800094519,
8.95212032183667));
#36033=CARTESIAN_POINT('Ctrl Pts',(-4.37148981486424,0.794772683999981,
8.99233910505878));
#36034=CARTESIAN_POINT('Ctrl Pts',(-4.44130624086955,1.06847604194408,9.02805188718885));
#36035=CARTESIAN_POINT('Ctrl Pts',(-4.47132133777115,1.18514270861074,9.03843348444035));
#36036=CARTESIAN_POINT('Ctrl Pts',(-4.50113058771019,1.29999999999895,9.04373793884824));
#36037=CARTESIAN_POINT('Ctrl Pts',(-4.56928530707914,-1.30000000000059,
8.8178345395562));
#36038=CARTESIAN_POINT('Ctrl Pts',(-4.53110597748958,-1.18514270861189,
8.82663583470339));
#36039=CARTESIAN_POINT('Ctrl Pts',(-4.49276685699007,-1.06847604194472,
8.83220890665423));
#36040=CARTESIAN_POINT('Ctrl Pts',(-4.40382666995363,-0.794772684000086,
8.83762597636249));
#36041=CARTESIAN_POINT('Ctrl Pts',(-4.34059639319766,-0.636309800094585,
8.82639912022816));
#36042=CARTESIAN_POINT('Ctrl Pts',(-4.26501625064136,-0.319434907276852,
8.8278652604988));
#36043=CARTESIAN_POINT('Ctrl Pts',(-4.23003147946568,-0.15833333333318,
8.82512789904));
#36044=CARTESIAN_POINT('Ctrl Pts',(-4.21988571051916,0.158333333333182,
8.85142664380134));
#36045=CARTESIAN_POINT('Ctrl Pts',(-4.24464215762767,0.319434907276859,
8.88069629902359));
#36046=CARTESIAN_POINT('Ctrl Pts',(-4.29972425819613,0.636309800094593,
8.93232308575814));
#36047=CARTESIAN_POINT('Ctrl Pts',(-4.35149662840352,0.794772684000076,
8.97226784151546));
#36048=CARTESIAN_POINT('Ctrl Pts',(-4.42431116283579,1.0684760419442,9.01019869496993));
#36049=CARTESIAN_POINT('Ctrl Pts',(-4.45636948654916,1.18514270861088,9.02211217414616));
#36050=CARTESIAN_POINT('Ctrl Pts',(-4.48896742006456,1.2999999999991,9.0295202715148));
#36051=CARTESIAN_POINT('Ctrl Pts',(-4.55583799175337,-1.30000000000069,
8.80577096598503));
#36052=CARTESIAN_POINT('Ctrl Pts',(-4.51528035914532,-1.18514270861198,
8.81177075214429));
#36053=CARTESIAN_POINT('Ctrl Pts',(-4.47510676734569,-1.0684760419448,8.81546891809767));
#36054=CARTESIAN_POINT('Ctrl Pts',(-4.38318494468386,-0.794772684000149,
8.81869521815243));
#36055=CARTESIAN_POINT('Ctrl Pts',(-4.31952068576917,-0.636309800094635,
8.80960689064762));
#36056=CARTESIAN_POINT('Ctrl Pts',(-4.24365109879925,-0.319434907276876,
8.81136459575073));
#36057=CARTESIAN_POINT('Ctrl Pts',(-4.2097125059512,-0.158333333333192,
8.80902096173901));
#36058=CARTESIAN_POINT('Ctrl Pts',(-4.20031047460861,0.158333333333195,
8.83399022560956));
#36059=CARTESIAN_POINT('Ctrl Pts',(-4.22514604427133,0.319434907276886,
8.86080966478229));
#36060=CARTESIAN_POINT('Ctrl Pts',(-4.28125531227806,0.636309800094644,
8.91091769219793));
#36061=CARTESIAN_POINT('Ctrl Pts',(-4.33317146618663,0.794772684000139,
8.94946370267855));
#36062=CARTESIAN_POINT('Ctrl Pts',(-4.40863350682741,1.06847604194429,8.99021278084444));
#36063=CARTESIAN_POINT('Ctrl Pts',(-4.44229150336739,1.18514270861097,9.00438862413133));
#36064=CARTESIAN_POINT('Ctrl Pts',(-4.47694277519813,1.29999999999921,9.01510154466924));
#36065=CARTESIAN_POINT('Ctrl Pts',(-4.54314694081231,-1.30000000000081,
8.79218277495134));
#36066=CARTESIAN_POINT('Ctrl Pts',(-4.49993318296694,-1.18514270861209,
8.79591737570066));
#36067=CARTESIAN_POINT('Ctrl Pts',(-4.45779290816555,-1.0684760419449,8.79800537855424));
#36068=CARTESIAN_POINT('Ctrl Pts',(-4.36292040382263,-0.79477268400022,
8.79902511230956));
#36069=CARTESIAN_POINT('Ctrl Pts',(-4.29959080148349,-0.636309800094691,
8.79067950908064));
#36070=CARTESIAN_POINT('Ctrl Pts',(-4.22346388217673,-0.319434907276905,
8.79268807838411));
#36071=CARTESIAN_POINT('Ctrl Pts',(-4.19031851099241,-0.158333333333206,
8.79123196627607));
#36072=CARTESIAN_POINT('Ctrl Pts',(-4.18082761705046,0.158333333333209,
8.81634013469114));
#36073=CARTESIAN_POINT('Ctrl Pts',(-4.2046155438811,0.319434907276914,8.84267021748946));
#36074=CARTESIAN_POINT('Ctrl Pts',(-4.26113836839254,0.636309800094701,
8.89228222330199));
#36075=CARTESIAN_POINT('Ctrl Pts',(-4.3132448740173,0.794772684000209,8.92922932179509));
#36076=CARTESIAN_POINT('Ctrl Pts',(-4.39195396843211,1.06847604194438,8.97177994644193));
#36077=CARTESIAN_POINT('Ctrl Pts',(-4.42765482463769,1.18514270861108,8.9874919159399));
#36078=CARTESIAN_POINT('Ctrl Pts',(-4.46498628653604,1.29999999999932,9.00049726618224));
#36079=CARTESIAN_POINT('Ctrl Pts',(-4.53154583913819,-1.30000000000086,
8.78285112053937));
#36080=CARTESIAN_POINT('Ctrl Pts',(-4.48607560509566,-1.18514270861213,
8.78475025417892));
#36081=CARTESIAN_POINT('Ctrl Pts',(-4.44228833053133,-1.06847604194494,
8.7854889063467));
#36082=CARTESIAN_POINT('Ctrl Pts',(-4.34501893974323,-0.794772684000252,
8.78451439626788));
#36083=CARTESIAN_POINT('Ctrl Pts',(-4.2821642101198,-0.636309800094717,
8.77641182159235));
#36084=CARTESIAN_POINT('Ctrl Pts',(-4.20592949896746,-0.319434907276918,
8.77841722805452));
#36085=CARTESIAN_POINT('Ctrl Pts',(-4.17329074901145,-0.158333333333213,
8.77798649026425));
#36086=CARTESIAN_POINT('Ctrl Pts',(-4.16401602768526,0.158333333333215,
8.80268342941709));
#36087=CARTESIAN_POINT('Ctrl Pts',(-4.18750489629661,0.319434907276928,
8.82757110874094));
#36088=CARTESIAN_POINT('Ctrl Pts',(-4.24459337785601,0.636309800094728,
8.87636044696449));
#36089=CARTESIAN_POINT('Ctrl Pts',(-4.29665787175149,0.794772684000242,
8.91232952829772));
#36090=CARTESIAN_POINT('Ctrl Pts',(-4.37787154550263,1.06847604194443,8.95672080950009));
#36091=CARTESIAN_POINT('Ctrl Pts',(-4.41516042469046,1.18514270861112,8.97390617246834));
#36092=CARTESIAN_POINT('Ctrl Pts',(-4.45458379296244,1.29999999999938,8.98906155763138));
#36093=CARTESIAN_POINT('Ctrl Pts',(-4.52306413166245,-1.30000000000088,
8.77380443519589));
#36094=CARTESIAN_POINT('Ctrl Pts',(-4.4758111708909,-1.18514270861215,8.77420613643231));
#36095=CARTESIAN_POINT('Ctrl Pts',(-4.43067705000433,-1.06847604194496,
8.77393111173708));
#36096=CARTESIAN_POINT('Ctrl Pts',(-4.33130314571344,-0.794772684000266,
8.77173237739195));
#36097=CARTESIAN_POINT('Ctrl Pts',(-4.26846935116606,-0.636309800094728,
8.76450136718779));
#36098=CARTESIAN_POINT('Ctrl Pts',(-4.19191385220492,-0.319434907276924,
8.76696076118828));
#36099=CARTESIAN_POINT('Ctrl Pts',(-4.15967196114376,-0.158333333333216,
8.76738409871529));
#36100=CARTESIAN_POINT('Ctrl Pts',(-4.15054722647059,0.158333333333218,
8.79179444465084));
#36101=CARTESIAN_POINT('Ctrl Pts',(-4.17383252913904,0.319434907276932,
8.81543206158095));
#36102=CARTESIAN_POINT('Ctrl Pts',(-4.23145909870731,0.636309800094738,
8.86340646993248));
#36103=CARTESIAN_POINT('Ctrl Pts',(-4.28368320628294,0.794772684000255,
8.89827172268338));
#36104=CARTESIAN_POINT('Ctrl Pts',(-4.36682683181974,1.06847604194444,8.94427098979597));
#36105=CARTESIAN_POINT('Ctrl Pts',(-4.40529200932223,1.18514270861114,8.9628014504945));
#36106=CARTESIAN_POINT('Ctrl Pts',(-4.44623256960727,1.2999999999994,8.97995099359933));
#36107=CARTESIAN_POINT('Ctrl Pts',(-4.50966808728432,-1.30000000000095,
8.76156795041173));
#36108=CARTESIAN_POINT('Ctrl Pts',(-4.45978821012882,-1.18514270861221,
8.75962299771254));
#36109=CARTESIAN_POINT('Ctrl Pts',(-4.41268861520961,-1.06847604194501,
8.75771534776358));
#36110=CARTESIAN_POINT('Ctrl Pts',(-4.31030213686421,-0.794772684000305,
8.75339447157283));
#36111=CARTESIAN_POINT('Ctrl Pts',(-4.2475790859924,-0.63630980009476,8.74732930188912));
#36112=CARTESIAN_POINT('Ctrl Pts',(-4.17078494416672,-0.31943490727694,
8.74999343533582));
#36113=CARTESIAN_POINT('Ctrl Pts',(-4.13947211741483,-0.158333333333223,
8.75104020535033));
#36114=CARTESIAN_POINT('Ctrl Pts',(-4.13054071912278,0.158333333333226,
8.77506361269285));
#36115=CARTESIAN_POINT('Ctrl Pts',(-4.15314876472547,0.319434907276948,
8.79754744461613));
#36116=CARTESIAN_POINT('Ctrl Pts',(-4.2112886885093,0.636309800094769,8.84482107130969));
#36117=CARTESIAN_POINT('Ctrl Pts',(-4.26335617522184,0.794772684000296,
8.87866853656956));
#36118=CARTESIAN_POINT('Ctrl Pts',(-4.34975387162024,1.0684760419445,8.92645407663372));
#36119=CARTESIAN_POINT('Ctrl Pts',(-4.39032400174482,1.1851427086112,8.94641808617921));
#36120=CARTESIAN_POINT('Ctrl Pts',(-4.43406590057326,1.29999999999946,8.9656615156052));
#36121=CARTESIAN_POINT('Ctrl Pts',(-4.48972114667131,-1.3000000000011,8.74286441635357));
#36122=CARTESIAN_POINT('Ctrl Pts',(-4.43547883514081,-1.18514270861236,
8.73822466035712));
#36123=CARTESIAN_POINT('Ctrl Pts',(-4.38514975315686,-1.06847604194515,
8.73442121547394));
#36124=CARTESIAN_POINT('Ctrl Pts',(-4.27791984856732,-0.794772684000405,
8.72756654289241));
#36125=CARTESIAN_POINT('Ctrl Pts',(-4.21573214866852,-0.636309800094839,
8.7225529096059));
#36126=CARTESIAN_POINT('Ctrl Pts',(-4.13855575725197,-0.319434907276979,
8.72558877417398));
#36127=CARTESIAN_POINT('Ctrl Pts',(-4.10842119208862,-0.158333333333243,
8.72800182405605));
#36128=CARTESIAN_POINT('Ctrl Pts',(-4.09977236837343,0.158333333333246,
8.75144365581481));
#36129=CARTESIAN_POINT('Ctrl Pts',(-4.12136531014535,0.319434907276988,
8.7721314354358));
#36130=CARTESIAN_POINT('Ctrl Pts',(-4.18070631104924,0.636309800094849,
8.81753949133427));
#36131=CARTESIAN_POINT('Ctrl Pts',(-4.23351725580547,0.794772684000396,
8.84812274771854));
#36132=CARTESIAN_POINT('Ctrl Pts',(-4.32465269180564,1.06847604194463,8.8987984096838));
#36133=CARTESIAN_POINT('Ctrl Pts',(-4.36805402374264,1.18514270861135,8.92146825773577));
#36134=CARTESIAN_POINT('Ctrl Pts',(-4.41540753427286,1.29999999999962,8.94487233749329));
#36135=CARTESIAN_POINT('Ctrl Pts',(-4.46225757065984,-1.30000000000127,
8.71958453597259));
#36136=CARTESIAN_POINT('Ctrl Pts',(-4.4025506934583,-1.18514270861251,8.71060091650708));
#36137=CARTESIAN_POINT('Ctrl Pts',(-4.34809231889145,-1.06847604194528,
8.70388865690302));
#36138=CARTESIAN_POINT('Ctrl Pts',(-4.23440767032736,-0.794772684000507,
8.69362929009866));
#36139=CARTESIAN_POINT('Ctrl Pts',(-4.17214331313643,-0.63630980009492,
8.69166805282642));
#36140=CARTESIAN_POINT('Ctrl Pts',(-4.09424342713997,-0.31943490727702,
8.69563909448733));
#36141=CARTESIAN_POINT('Ctrl Pts',(-4.06586783821613,-0.158333333333263,
8.69949510324146));
#36142=CARTESIAN_POINT('Ctrl Pts',(-4.05786199444834,0.158333333333265,
8.72157248282735));
#36143=CARTESIAN_POINT('Ctrl Pts',(-4.07874176403268,0.319434907277027,
8.73856548687397));
#36144=CARTESIAN_POINT('Ctrl Pts',(-4.13929543967664,0.636309800094928,
8.78206657250136));
#36145=CARTESIAN_POINT('Ctrl Pts',(-4.19139502078103,0.794772684000495,
8.81130446539696));
#36146=CARTESIAN_POINT('Ctrl Pts',(-4.28896174323994,1.06847604194477,8.86567732901192));
#36147=CARTESIAN_POINT('Ctrl Pts',(-4.3365817094158,1.1851427086115,8.89121162387947));
#36148=CARTESIAN_POINT('Ctrl Pts',(-4.38958862281842,1.29999999999979,8.91874421566881));
#36149=CARTESIAN_POINT('Ctrl Pts',(-4.43911310247445,-1.30000000000157,
8.70074230118706));
#36150=CARTESIAN_POINT('Ctrl Pts',(-4.37448267385302,-1.18514270861279,
8.6889702543753));
#36151=CARTESIAN_POINT('Ctrl Pts',(-4.31635227442594,-1.06847604194553,
8.6803703284716));
#36152=CARTESIAN_POINT('Ctrl Pts',(-4.19707579056849,-0.794772684000693,
8.66783101310304));
#36153=CARTESIAN_POINT('Ctrl Pts',(-4.13529783701336,-0.636309800095066,
8.66733511322863));
#36154=CARTESIAN_POINT('Ctrl Pts',(-4.05664387112888,-0.319434907277092,
8.67245999763365));
#36155=CARTESIAN_POINT('Ctrl Pts',(-4.02921254050706,-0.158333333333299,
8.67863830460936));
#36156=CARTESIAN_POINT('Ctrl Pts',(-4.02140348472796,0.158333333333302,
8.70020161040361));
#36157=CARTESIAN_POINT('Ctrl Pts',(-4.04130261769599,0.319434907277102,
8.7147047681238));
#36158=CARTESIAN_POINT('Ctrl Pts',(-4.10348615916234,0.636309800095076,
8.7552990318348));
#36159=CARTESIAN_POINT('Ctrl Pts',(-4.15653007774043,0.794772684000676,
8.7804454628435));
#36160=CARTESIAN_POINT('Ctrl Pts',(-4.26006427161474,1.06847604194501,8.83661089969961));
#36161=CARTESIAN_POINT('Ctrl Pts',(-4.31123720445708,1.18514270861177,8.86439776995298));
#36162=CARTESIAN_POINT('Ctrl Pts',(-4.36876695393351,1.30000000000009,8.89565957397926));
#36163=CARTESIAN_POINT('Ctrl Pts',(-4.42075431675889,-1.30000000000158,
8.68521657502598));
#36164=CARTESIAN_POINT('Ctrl Pts',(-4.35219808770137,-1.18514270861279,
8.6710538738467));
#36165=CARTESIAN_POINT('Ctrl Pts',(-4.29106007738977,-1.06847604194554,
8.66099953632976));
#36166=CARTESIAN_POINT('Ctrl Pts',(-4.16695661226589,-0.794772684000697,
8.64726314723766));
#36167=CARTESIAN_POINT('Ctrl Pts',(-4.10471537309693,-0.636309800095071,
8.64981620211422));
#36168=CARTESIAN_POINT('Ctrl Pts',(-4.02550494520748,-0.319434907277095,
8.65575584817436));
#36169=CARTESIAN_POINT('Ctrl Pts',(-3.99977596517424,-0.158333333333301,
8.6617818347337));
#36170=CARTESIAN_POINT('Ctrl Pts',(-3.99236947390528,0.158333333333303,
8.68238426965024));
#36171=CARTESIAN_POINT('Ctrl Pts',(-4.01124821738469,0.319434907277104,
8.69539919887263));
#36172=CARTESIAN_POINT('Ctrl Pts',(-4.07423910504128,0.63630980009508,8.73460593135742));
#36173=CARTESIAN_POINT('Ctrl Pts',(-4.12728445891231,0.794772684000685,
8.75782848948147));
#36174=CARTESIAN_POINT('Ctrl Pts',(-4.23532127633879,1.06847604194502,8.81604471656162));
#36175=CARTESIAN_POINT('Ctrl Pts',(-4.28935485892354,1.18514270861178,8.84568172449774));
#36176=CARTESIAN_POINT('Ctrl Pts',(-4.35065688898772,1.30000000000009,8.87975609279077));
#36177=CARTESIAN_POINT('Ctrl Pts',(-4.40659708526905,-1.30000000000166,
8.67446878376005));
#36178=CARTESIAN_POINT('Ctrl Pts',(-4.33500103708209,-1.18514270861287,
8.65885991086501));
#36179=CARTESIAN_POINT('Ctrl Pts',(-4.27159398066144,-1.0684760419456,8.64785577527442));
#36180=CARTESIAN_POINT('Ctrl Pts',(-4.1440292049743,-0.794772684000745,
8.6330718850382));
#36181=CARTESIAN_POINT('Ctrl Pts',(-4.0820895603583,-0.63630980009511,8.63655403448564));
#36182=CARTESIAN_POINT('Ctrl Pts',(-4.00237175737431,-0.319434907277115,
8.643356071981));
#36183=CARTESIAN_POINT('Ctrl Pts',(-3.97716150569709,-0.15833333333331,
8.65088312043462));
#36184=CARTESIAN_POINT('Ctrl Pts',(-3.96985075878325,0.158333333333313,
8.67118698661727));
#36185=CARTESIAN_POINT('Ctrl Pts',(-3.98820168570649,0.319434907277123,
8.68254269792091));
#36186=CARTESIAN_POINT('Ctrl Pts',(-4.05210850918212,0.636309800095118,
8.7199928653782));
#36187=CARTESIAN_POINT('Ctrl Pts',(-4.10541687631528,0.794772684000733,
8.74119421122248));
#36188=CARTESIAN_POINT('Ctrl Pts',(-4.21724916319844,1.06847604194508,8.79997976559179));
#36189=CARTESIAN_POINT('Ctrl Pts',(-4.2736200148387,1.18514270861185,8.83055472465665));
#36190=CARTESIAN_POINT('Ctrl Pts',(-4.33795366492212,1.30000000000017,8.86625855451932));
#36191=CARTESIAN_POINT('Ctrl Pts',(-4.39232901724014,-1.3000000000017,8.66375480980727));
#36192=CARTESIAN_POINT('Ctrl Pts',(-4.31766672800015,-1.1851427086129,8.64639229265701));
#36193=CARTESIAN_POINT('Ctrl Pts',(-4.25188946484526,-1.06847604194564,
8.63438908801193));
#36194=CARTESIAN_POINT('Ctrl Pts',(-4.12045701596139,-0.79477268400077,
8.61904036806275));
#36195=CARTESIAN_POINT('Ctrl Pts',(-4.05774099367921,-0.636309800095132,
8.62588706975922));
#36196=CARTESIAN_POINT('Ctrl Pts',(-3.97797184968243,-0.319434907277126,
8.63245483859954));
#36197=CARTESIAN_POINT('Ctrl Pts',(-3.95519739470823,-0.158333333333316,
8.63725925921173));
#36198=CARTESIAN_POINT('Ctrl Pts',(-3.94834123033963,0.158333333333319,
8.65644217709915));
#36199=CARTESIAN_POINT('Ctrl Pts',(-3.96498865647832,0.319434907277135,
8.66867953880038));
#36200=CARTESIAN_POINT('Ctrl Pts',(-4.02930709073509,0.636309800095142,
8.70554733147818));
#36201=CARTESIAN_POINT('Ctrl Pts',(-4.0829650466866,0.794772684000761,8.72454112670396));
#36202=CARTESIAN_POINT('Ctrl Pts',(-4.19848477060446,1.06847604194512,8.78448064229685));
#36203=CARTESIAN_POINT('Ctrl Pts',(-4.25715537491875,1.18514270861189,8.81629550060161));
#36204=CARTESIAN_POINT('Ctrl Pts',(-4.32449237549088,1.30000000000022,8.85397962188891));
#36205=CARTESIAN_POINT('Ctrl Pts',(-4.38055136998851,-1.30000000000175,
8.65486034483293));
#36206=CARTESIAN_POINT('Ctrl Pts',(-4.30314549901928,-1.18514270861294,
8.63701984983662));
#36207=CARTESIAN_POINT('Ctrl Pts',(-4.23545078584017,-1.06847604194568,
8.62448447136143));
#36208=CARTESIAN_POINT('Ctrl Pts',(-4.10149717332144,-0.794772684000798,
8.60778111983862));
#36209=CARTESIAN_POINT('Ctrl Pts',(-4.0400134261722,-0.636309800095152,
8.61321666597366));
#36210=CARTESIAN_POINT('Ctrl Pts',(-3.96056350920759,-0.319434907277135,
8.61898989843895));
#36211=CARTESIAN_POINT('Ctrl Pts',(-3.93872539640991,-0.158333333333321,
8.62400320920415));
#36212=CARTESIAN_POINT('Ctrl Pts',(-3.93159547877079,0.158333333333323,
8.64375728571561));
#36213=CARTESIAN_POINT('Ctrl Pts',(-3.94664076546426,0.319434907277145,
8.65721696059045));
#36214=CARTESIAN_POINT('Ctrl Pts',(-4.01088092238389,0.636309800095162,
8.6942908495018));
#36215=CARTESIAN_POINT('Ctrl Pts',(-4.06467681579459,0.794772684000785,
8.71158207420152));
#36216=CARTESIAN_POINT('Ctrl Pts',(-4.18296403816074,1.06847604194515,8.77241849605042));
#36217=CARTESIAN_POINT('Ctrl Pts',(-4.24342309250851,1.18514270861193,8.80512936980167));
#36218=CARTESIAN_POINT('Ctrl Pts',(-4.31313904561529,1.30000000000026,8.84421728449737));
#36219=CARTESIAN_POINT('Ctrl Pts',(-4.36598120515593,-1.30000000000177,
8.64481132314811));
#36220=CARTESIAN_POINT('Ctrl Pts',(-4.28494496219392,-1.18514270861297,
8.62620935511287));
#36221=CARTESIAN_POINT('Ctrl Pts',(-4.2147464284803,-1.06847604194569,8.61273308884697));
#36222=CARTESIAN_POINT('Ctrl Pts',(-4.07761104887375,-0.794772684000812,
8.59344161433524));
#36223=CARTESIAN_POINT('Ctrl Pts',(-4.01795641242019,-0.636309800095164,
8.5960638488432));
#36224=CARTESIAN_POINT('Ctrl Pts',(-3.93922052986902,-0.319434907277142,
8.59978175807134));
#36225=CARTESIAN_POINT('Ctrl Pts',(-3.91872281830903,-0.158333333333324,
8.60487133018024));
#36226=CARTESIAN_POINT('Ctrl Pts',(-3.91162073886137,0.158333333333326,
8.62450764463315));
#36227=CARTESIAN_POINT('Ctrl Pts',(-3.925211094291,0.319434907277151,8.63805118402258));
#36228=CARTESIAN_POINT('Ctrl Pts',(-3.98908391499714,0.636309800095174,
8.6763744856589));
#36229=CARTESIAN_POINT('Ctrl Pts',(-4.04179842596812,0.7947726840008,8.69483225573699));
#36230=CARTESIAN_POINT('Ctrl Pts',(-4.16338112100733,1.06847604194518,8.75813315058748));
#36231=CARTESIAN_POINT('Ctrl Pts',(-4.22623879415762,1.18514270861196,8.79210358693433));
#36232=CARTESIAN_POINT('Ctrl Pts',(-4.29932549685856,1.30000000000029,8.83264384777654));
#36233=CARTESIAN_POINT('Ctrl Pts',(-4.3561014276295,-1.30000000000184,8.63787852952414));
#36234=CARTESIAN_POINT('Ctrl Pts',(-4.27202510729764,-1.18514270861303,
8.62000938470732));
#36235=CARTESIAN_POINT('Ctrl Pts',(-4.19998727434634,-1.06847604194575,
8.60640446368449));
#36236=CARTESIAN_POINT('Ctrl Pts',(-4.06137678325034,-0.794772684000851,
8.58482558448585));
#36237=CARTESIAN_POINT('Ctrl Pts',(-4.00531418533707,-0.636309800095196,
8.58193800807906));
#36238=CARTESIAN_POINT('Ctrl Pts',(-3.92838285750872,-0.319434907277159,
8.58266762339361));
#36239=CARTESIAN_POINT('Ctrl Pts',(-3.90875262161207,-0.158333333333332,
8.58839155927254));
#36240=CARTESIAN_POINT('Ctrl Pts',(-3.90175138030431,0.158333333333335,
8.60789341044225));
#36241=CARTESIAN_POINT('Ctrl Pts',(-3.91457783688431,0.319434907277167,
8.62081822042886));
#36242=CARTESIAN_POINT('Ctrl Pts',(-3.97684592441674,0.636309800095206,
8.66155018584608));
#36243=CARTESIAN_POINT('Ctrl Pts',(-4.02617203613903,0.794772684000841,
8.68440863390959));
#36244=CARTESIAN_POINT('Ctrl Pts',(-4.14921392208312,1.06847604194523,8.75005834839344));
#36245=CARTESIAN_POINT('Ctrl Pts',(-4.2138412015471,1.18514270861202,8.78447021792653));
#36246=CARTESIAN_POINT('Ctrl Pts',(-4.28983548720103,1.30000000000035,8.82487662815433));
#36247=CARTESIAN_POINT('Ctrl Pts',(-4.35088387761181,-1.30000000000184,
8.63103946714464));
#36248=CARTESIAN_POINT('Ctrl Pts',(-4.26698198886935,-1.18514270861303,
8.61335123634859));
#36249=CARTESIAN_POINT('Ctrl Pts',(-4.19526082558524,-1.06847604194575,
8.59960976409458));
#36250=CARTESIAN_POINT('Ctrl Pts',(-4.05771050318435,-0.794772684000851,
8.5769820159942));
#36251=CARTESIAN_POINT('Ctrl Pts',(-4.00307751336492,-0.636309800095196,
8.57196388006084));
#36252=CARTESIAN_POINT('Ctrl Pts',(-3.9271390295546,-0.319434907277159,
8.57133011076225));
#36253=CARTESIAN_POINT('Ctrl Pts',(-3.90745678965039,-0.158333333333332,
8.5770480695384));
#36254=CARTESIAN_POINT('Ctrl Pts',(-3.90061191119441,0.158333333333335,
8.59637205061778));
#36255=CARTESIAN_POINT('Ctrl Pts',(-3.91380906647831,0.319434907277167,
8.60889674750867));
#36256=CARTESIAN_POINT('Ctrl Pts',(-3.9750721515842,0.636309800095206,8.65109465690008));
#36257=CARTESIAN_POINT('Ctrl Pts',(-4.02239198166674,0.794772684000841,
8.67700128450958));
#36258=CARTESIAN_POINT('Ctrl Pts',(-4.14444540563293,1.06847604194523,8.74356402580408));
#36259=CARTESIAN_POINT('Ctrl Pts',(-4.20891602829553,1.18514270861202,8.77783540490947));
#36260=CARTESIAN_POINT('Ctrl Pts',(-4.28502486891082,1.30000000000035,8.8175656188065));
#36261=CARTESIAN_POINT('Ctrl Pts',(-4.35088387761047,-1.3,8.63103946714436));
#36262=CARTESIAN_POINT('Ctrl Pts',(-4.26698198886859,-1.18514270861178,
8.61335123634844));
#36263=CARTESIAN_POINT('Ctrl Pts',(-4.19526082558493,-1.06847604194512,
8.59960976409452));
#36264=CARTESIAN_POINT('Ctrl Pts',(-4.05771050318435,-0.794772684000851,
8.5769820159942));
#36265=CARTESIAN_POINT('Ctrl Pts',(-4.00307751336492,-0.636309800095197,
8.57196388006084));
#36266=CARTESIAN_POINT('Ctrl Pts',(-3.9271390295546,-0.319434907277159,
8.57133011076224));
#36267=CARTESIAN_POINT('Ctrl Pts',(-3.90745678965039,-0.158333333333332,
8.5770480695384));
#36268=CARTESIAN_POINT('Ctrl Pts',(-3.90061191119441,0.158333333333334,
8.59637205061778));
#36269=CARTESIAN_POINT('Ctrl Pts',(-3.91380906647831,0.319434907277167,
8.60889674750867));
#36270=CARTESIAN_POINT('Ctrl Pts',(-3.9750721515842,0.636309800095206,8.65109465690008));
#36271=CARTESIAN_POINT('Ctrl Pts',(-4.02239198166674,0.79477268400084,8.67700128450958));
#36272=CARTESIAN_POINT('Ctrl Pts',(-4.14444540563287,1.06847604194511,8.74356402580405));
#36273=CARTESIAN_POINT('Ctrl Pts',(-4.20891602829539,1.18514270861178,8.7778354049094));
#36274=CARTESIAN_POINT('Ctrl Pts',(-4.28502486891058,1.3,8.81756561880638));
#36275=CARTESIAN_POINT('',(-4.63723388560792,-1.2,8.93163561125591));
#36276=CARTESIAN_POINT('Ctrl Pts',(-4.63723388560792,-1.2,8.93163561125591));
#36277=CARTESIAN_POINT('Ctrl Pts',(-4.62753389439639,-1.21478802097806,
8.91533912501957));
#36278=CARTESIAN_POINT('Ctrl Pts',(-4.62697861968183,-1.21593888768291,
8.91350422791788));
#36279=CARTESIAN_POINT('Ctrl Pts',(-4.61456982759609,-1.23519182817029,
8.89149335283502));
#36280=CARTESIAN_POINT('Ctrl Pts',(-4.61325995412872,-1.23709049084105,
8.88956307144032));
#36281=CARTESIAN_POINT('Ctrl Pts',(-4.59898272268779,-1.25866691551418,
8.86569698934375));
#36282=CARTESIAN_POINT('Ctrl Pts',(-4.59362321232696,-1.26678758340789,
8.85663230638542));
#36283=CARTESIAN_POINT('Ctrl Pts',(-4.58386363196318,-1.28145275507162,
8.84041978907459));
#36284=CARTESIAN_POINT('Ctrl Pts',(-4.57687058714458,-1.29190031914763,
8.82892890064751));
#36285=CARTESIAN_POINT('Ctrl Pts',(-4.5724258367586,-1.29846636104134,8.82182026882674));
#36286=CARTESIAN_POINT('Ctrl Pts',(-4.57190495076468,-1.29923376230637,
8.82099308234304));
#36287=CARTESIAN_POINT('Ctrl Pts',(-4.57138290900173,-1.30000000000056,
8.82017230542972));
#36288=CARTESIAN_POINT('',(-4.58017336249762,-0.653834841416747,9.07736836268454));
#36289=CARTESIAN_POINT('Ctrl Pts',(-4.5801733625228,-0.653834841416062,
9.07736836269194));
#36290=CARTESIAN_POINT('Ctrl Pts',(-4.58634132012241,-0.717928704880547,
9.06232053528613));
#36291=CARTESIAN_POINT('Ctrl Pts',(-4.59131394979481,-0.763797028297237,
9.05003100375446));
#36292=CARTESIAN_POINT('Ctrl Pts',(-4.61052464146469,-0.949538109615673,
9.00188729361407));
#36293=CARTESIAN_POINT('Ctrl Pts',(-4.62075787424104,-1.04843725126253,
8.97575754875452));
#36294=CARTESIAN_POINT('Ctrl Pts',(-4.63723388560792,-1.2,8.93163561125591));
#36295=CARTESIAN_POINT('',(-4.52544944337419,0.653834841531101,9.20569372922794));
#36296=CARTESIAN_POINT('Ctrl Pts',(-4.52544944337418,0.653834841531102,
9.20569372922795));
#36297=CARTESIAN_POINT('Ctrl Pts',(-4.49800477099097,0.575791366845458,
9.1743322544575));
#36298=CARTESIAN_POINT('Ctrl Pts',(-4.47552136690656,0.493917914177405,
9.14760173032986));
#36299=CARTESIAN_POINT('Ctrl Pts',(-4.44488215025619,0.338198323071554,
9.10721680052762));
#36300=CARTESIAN_POINT('Ctrl Pts',(-4.43508703909453,0.265710276728555,
9.0922158274664));
#36301=CARTESIAN_POINT('Ctrl Pts',(-4.42552808798967,0.129738884446912,
9.06975255594665));
#36302=CARTESIAN_POINT('Ctrl Pts',(-4.4244963582949,0.0666402419227446,
9.06153246854483));
#36303=CARTESIAN_POINT('Ctrl Pts',(-4.42938618481451,-0.0595493706457138,
9.04911769727901));
#36304=CARTESIAN_POINT('Ctrl Pts',(-4.43532950520763,-0.122795525062026,
9.04482175652539));
#36305=CARTESIAN_POINT('Ctrl Pts',(-4.45563401062421,-0.260143259403432,
9.04056858786434));
#36306=CARTESIAN_POINT('Ctrl Pts',(-4.47133340707415,-0.333940698349591,
9.04154200493254));
#36307=CARTESIAN_POINT('Ctrl Pts',(-4.51502088722612,-0.49122835763458,
9.05169607394797));
#36308=CARTESIAN_POINT('Ctrl Pts',(-4.54472679166538,-0.574163474744005,
9.06210644021376));
#36309=CARTESIAN_POINT('Ctrl Pts',(-4.5801733624882,-0.653834841428463,
9.07736836264527));
#36310=CARTESIAN_POINT('',(-4.55421084628694,1.2,9.1395008552621));
#36311=CARTESIAN_POINT('Ctrl Pts',(-4.55421084628694,1.2,9.1395008552621));
#36312=CARTESIAN_POINT('Ctrl Pts',(-4.54938195732035,1.13478776924219,9.15083974095914));
#36313=CARTESIAN_POINT('Ctrl Pts',(-4.54293098542071,1.03871837843732,9.16586603442479));
#36314=CARTESIAN_POINT('Ctrl Pts',(-4.5301428206211,0.795010067313144,9.19511397277935));
#36315=CARTESIAN_POINT('Ctrl Pts',(-4.52811399206583,0.741769803333558,
9.1996817044518));
#36316=CARTESIAN_POINT('Ctrl Pts',(-4.52544944337418,0.653834841531102,
9.20569372922794));
#36317=CARTESIAN_POINT('Ctrl Pts',(-4.49082727704437,1.29999999999907,9.03165781950759));
#36318=CARTESIAN_POINT('Ctrl Pts',(-4.50187711672958,1.28314156068347,9.04920504305177));
#36319=CARTESIAN_POINT('Ctrl Pts',(-4.51232625581989,1.26655442348624,9.06737950428502));
#36320=CARTESIAN_POINT('Ctrl Pts',(-4.53007724292771,1.23873360654381,9.09710440627825));
#36321=CARTESIAN_POINT('Ctrl Pts',(-4.54264069501209,1.21921921678529,9.1176177947092));
#36322=CARTESIAN_POINT('Ctrl Pts',(-4.55421084628694,1.2,9.1395008552621));
#36323=CARTESIAN_POINT('Ctrl Pts',(-4.35088387761047,-1.3,8.63103946714436));
#36324=CARTESIAN_POINT('Ctrl Pts',(-4.26698198886859,-1.18514270861178,
8.61335123634844));
#36325=CARTESIAN_POINT('Ctrl Pts',(-4.19526082558493,-1.06847604194512,
8.59960976409452));
#36326=CARTESIAN_POINT('Ctrl Pts',(-4.05771050318435,-0.794772684000851,
8.5769820159942));
#36327=CARTESIAN_POINT('Ctrl Pts',(-4.00307751336492,-0.636309800095196,
8.57196388006084));
#36328=CARTESIAN_POINT('Ctrl Pts',(-3.9271390295546,-0.319434907277158,
8.57133011076224));
#36329=CARTESIAN_POINT('Ctrl Pts',(-3.90745678965039,-0.158333333333332,
8.57704806953839));
#36330=CARTESIAN_POINT('Ctrl Pts',(-3.90061191119441,0.158333333333335,
8.59637205061778));
#36331=CARTESIAN_POINT('Ctrl Pts',(-3.91380906647831,0.319434907277167,
8.60889674750866));
#36332=CARTESIAN_POINT('Ctrl Pts',(-3.9750721515842,0.636309800095206,8.65109465690008));
#36333=CARTESIAN_POINT('Ctrl Pts',(-4.02239198166674,0.794772684000841,
8.67700128450958));
#36334=CARTESIAN_POINT('Ctrl Pts',(-4.14444540563287,1.06847604194511,8.74356402580405));
#36335=CARTESIAN_POINT('Ctrl Pts',(-4.20891602829539,1.18514270861178,8.7778354049094));
#36336=CARTESIAN_POINT('Ctrl Pts',(-4.28502486891058,1.3,8.81756561880638));
#36337=CARTESIAN_POINT('Ctrl Pts',(-4.37306897027954,-1.3,8.55737176093662));
#36338=CARTESIAN_POINT('Ctrl Pts',(-4.28882565135864,-1.18514270861178,
8.54138186178938));
#36339=CARTESIAN_POINT('Ctrl Pts',(-4.21691086230761,-1.06847604194512,
8.52883129592335));
#36340=CARTESIAN_POINT('Ctrl Pts',(-4.0792546834088,-0.794772684000851,
8.50778252595658));
#36341=CARTESIAN_POINT('Ctrl Pts',(-4.02499599674477,-0.636309800095196,
8.50215210324751));
#36342=CARTESIAN_POINT('Ctrl Pts',(-3.94958161227244,-0.319434907277158,
8.5011060196783));
#36343=CARTESIAN_POINT('Ctrl Pts',(-3.93044726732831,-0.158333333333332,
8.50570985865775));
#36344=CARTESIAN_POINT('Ctrl Pts',(-3.92394377232475,0.158333333333335,
8.52514476194479));
#36345=CARTESIAN_POINT('Ctrl Pts',(-3.93692932075669,0.319434907277167,
8.53889284526232));
#36346=CARTESIAN_POINT('Ctrl Pts',(-3.99837405888618,0.636309800095206,
8.58173238176729));
#36347=CARTESIAN_POINT('Ctrl Pts',(-4.04563681344556,0.794772684000841,
8.6083543696584));
#36348=CARTESIAN_POINT('Ctrl Pts',(-4.16853269776624,1.06847604194511,8.67357746992056));
#36349=CARTESIAN_POINT('Ctrl Pts',(-4.23354667110408,1.18514270861178,8.70677157514888));
#36350=CARTESIAN_POINT('Ctrl Pts',(-4.31037754319865,1.3,8.74492712225608));
#36351=CARTESIAN_POINT('Ctrl Pts',(-4.39525406294861,-1.3,8.48370405472888));
#36352=CARTESIAN_POINT('Ctrl Pts',(-4.3106693138487,-1.18514270861178,8.46941248723032));
#36353=CARTESIAN_POINT('Ctrl Pts',(-4.2385608990303,-1.06847604194512,8.45805282775218));
#36354=CARTESIAN_POINT('Ctrl Pts',(-4.10079886363325,-0.794772684000851,
8.43858303591895));
#36355=CARTESIAN_POINT('Ctrl Pts',(-4.04691448012462,-0.636309800095196,
8.43234032643418));
#36356=CARTESIAN_POINT('Ctrl Pts',(-3.97202419499028,-0.319434907277158,
8.43088192859436));
#36357=CARTESIAN_POINT('Ctrl Pts',(-3.95343774500623,-0.158333333333332,
8.4343716477771));
#36358=CARTESIAN_POINT('Ctrl Pts',(-3.94727563345509,0.158333333333335,
8.4539174732718));
#36359=CARTESIAN_POINT('Ctrl Pts',(-3.96004957503508,0.319434907277167,
8.46888894301597));
#36360=CARTESIAN_POINT('Ctrl Pts',(-4.02167596618816,0.636309800095206,
8.5123701066345));
#36361=CARTESIAN_POINT('Ctrl Pts',(-4.06888164522438,0.794772684000841,
8.53970745480722));
#36362=CARTESIAN_POINT('Ctrl Pts',(-4.19261998989962,1.06847604194511,8.60359091403707));
#36363=CARTESIAN_POINT('Ctrl Pts',(-4.25817731391276,1.18514270861178,8.63570774538835));
#36364=CARTESIAN_POINT('Ctrl Pts',(-4.33573021748671,1.3,8.67228862570577));
#36365=CARTESIAN_POINT('Ctrl Pts',(-4.41743915561768,-1.3,8.41003634852114));
#36366=CARTESIAN_POINT('Ctrl Pts',(-4.33251297633875,-1.18514270861178,
8.39744311267125));
#36367=CARTESIAN_POINT('Ctrl Pts',(-4.26021093575299,-1.06847604194512,
8.38727435958101));
#36368=CARTESIAN_POINT('Ctrl Pts',(-4.12234304385769,-0.794772684000851,
8.36938354588133));
#36369=CARTESIAN_POINT('Ctrl Pts',(-4.06883296350448,-0.636309800095196,
8.36252854962085));
#36370=CARTESIAN_POINT('Ctrl Pts',(-3.99446677770812,-0.319434907277158,
8.36065783751042));
#36371=CARTESIAN_POINT('Ctrl Pts',(-3.97642822268415,-0.158333333333332,
8.36303343689645));
#36372=CARTESIAN_POINT('Ctrl Pts',(-3.97060749458543,0.158333333333335,
8.38269018459881));
#36373=CARTESIAN_POINT('Ctrl Pts',(-3.98316982931346,0.319434907277167,
8.39888504076963));
#36374=CARTESIAN_POINT('Ctrl Pts',(-4.04497787349015,0.636309800095206,
8.44300783150171));
#36375=CARTESIAN_POINT('Ctrl Pts',(-4.0921264770032,0.794772684000841,8.47106053995604));
#36376=CARTESIAN_POINT('Ctrl Pts',(-4.21670728203299,1.06847604194511,8.53360435815359));
#36377=CARTESIAN_POINT('Ctrl Pts',(-4.28280795672145,1.18514270861178,8.56464391562783));
#36378=CARTESIAN_POINT('Ctrl Pts',(-4.36108289177478,1.3,8.59965012915547));
#36379=CARTESIAN_POINT('Ctrl Pts',(-4.41743915561768,-1.3,8.41003634852114));
#36380=CARTESIAN_POINT('Ctrl Pts',(-4.33251297633875,-1.18514270861178,
8.39744311267125));
#36381=CARTESIAN_POINT('Ctrl Pts',(-4.26021093575299,-1.06847604194512,
8.38727435958101));
#36382=CARTESIAN_POINT('Ctrl Pts',(-4.12234304385769,-0.794772684000851,
8.36938354588133));
#36383=CARTESIAN_POINT('Ctrl Pts',(-4.06883296350448,-0.636309800095197,
8.36252854962085));
#36384=CARTESIAN_POINT('Ctrl Pts',(-3.99446677770812,-0.319434907277159,
8.36065783751042));
#36385=CARTESIAN_POINT('Ctrl Pts',(-3.97642822268415,-0.158333333333332,
8.36303343689645));
#36386=CARTESIAN_POINT('Ctrl Pts',(-3.97060749458543,0.158333333333334,
8.38269018459881));
#36387=CARTESIAN_POINT('Ctrl Pts',(-3.98316982931346,0.319434907277167,
8.39888504076963));
#36388=CARTESIAN_POINT('Ctrl Pts',(-4.04497787349014,0.636309800095206,
8.44300783150171));
#36389=CARTESIAN_POINT('Ctrl Pts',(-4.0921264770032,0.79477268400084,8.47106053995604));
#36390=CARTESIAN_POINT('Ctrl Pts',(-4.21670728203298,1.06847604194511,8.53360435815359));
#36391=CARTESIAN_POINT('Ctrl Pts',(-4.28280795672145,1.18514270861178,8.56464391562783));
#36392=CARTESIAN_POINT('Ctrl Pts',(-4.36108289177478,1.3,8.59965012915547));
#36393=CARTESIAN_POINT('Ctrl Pts',(-4.41743915562091,-1.30000000000437,
8.41003634852161));
#36394=CARTESIAN_POINT('Ctrl Pts',(-4.33251297634058,-1.18514270861474,
8.39744311267151));
#36395=CARTESIAN_POINT('Ctrl Pts',(-4.26021093575375,-1.06847604194662,
8.38727435958111));
#36396=CARTESIAN_POINT('Ctrl Pts',(-4.12234304385769,-0.794772684000851,
8.36938354588133));
#36397=CARTESIAN_POINT('Ctrl Pts',(-4.06883296350448,-0.636309800095197,
8.36252854962085));
#36398=CARTESIAN_POINT('Ctrl Pts',(-3.99446677770812,-0.319434907277159,
8.36065783751042));
#36399=CARTESIAN_POINT('Ctrl Pts',(-3.97642822268415,-0.158333333333332,
8.36303343689645));
#36400=CARTESIAN_POINT('Ctrl Pts',(-3.97060749458543,0.158333333333334,
8.38269018459881));
#36401=CARTESIAN_POINT('Ctrl Pts',(-3.98316982931346,0.319434907277167,
8.39888504076963));
#36402=CARTESIAN_POINT('Ctrl Pts',(-4.04497787349015,0.636309800095206,
8.44300783150171));
#36403=CARTESIAN_POINT('Ctrl Pts',(-4.0921264770032,0.79477268400084,8.47106053995604));
#36404=CARTESIAN_POINT('Ctrl Pts',(-4.21670728203318,1.06847604194555,8.53360435815368));
#36405=CARTESIAN_POINT('Ctrl Pts',(-4.28280795672194,1.18514270861264,8.56464391562806));
#36406=CARTESIAN_POINT('Ctrl Pts',(-4.36108289177564,1.30000000000127,8.59965012915586));
#36407=CARTESIAN_POINT('Ctrl Pts',(-4.42289860586574,-1.30000000000437,
8.40797826829483));
#36408=CARTESIAN_POINT('Ctrl Pts',(-4.33776923904344,-1.18514270861474,
8.39579462447261));
#36409=CARTESIAN_POINT('Ctrl Pts',(-4.26532765431604,-1.06847604194662,
8.3856402571071));
#36410=CARTESIAN_POINT('Ctrl Pts',(-4.12728441652869,-0.794772684000851,
8.36686967168899));
#36411=CARTESIAN_POINT('Ctrl Pts',(-4.0738867088757,-0.636309800095197,
8.35758448088744));
#36412=CARTESIAN_POINT('Ctrl Pts',(-3.99955292053485,-0.319434907277159,
8.35452930264375));
#36413=CARTESIAN_POINT('Ctrl Pts',(-3.98155751278828,-0.158333333333332,
8.35726596170137));
#36414=CARTESIAN_POINT('Ctrl Pts',(-3.97575141855083,0.158333333333334,
8.37707991454073));
#36415=CARTESIAN_POINT('Ctrl Pts',(-3.98828336306808,0.319434907277167,
8.39325761631741));
#36416=CARTESIAN_POINT('Ctrl Pts',(-4.05009264080661,0.636309800095206,
8.43850479398448));
#36417=CARTESIAN_POINT('Ctrl Pts',(-4.0971774214965,0.79477268400084,8.46826681004936));
#36418=CARTESIAN_POINT('Ctrl Pts',(-4.2219190164042,1.06847604194555,8.53179176443982));
#36419=CARTESIAN_POINT('Ctrl Pts',(-4.28813697665279,1.18514270861264,8.56302905926473));
#36420=CARTESIAN_POINT('Ctrl Pts',(-4.36657688284595,1.30000000000127,8.59800604999041));
#36421=CARTESIAN_POINT('Ctrl Pts',(-4.43168171124751,-1.30000000000412,
8.40635777334216));
#36422=CARTESIAN_POINT('Ctrl Pts',(-4.34743550989965,-1.18514270861451,
8.39517850942592));
#36423=CARTESIAN_POINT('Ctrl Pts',(-4.27565255026722,-1.06847604194641,
8.38531825593481));
#36424=CARTESIAN_POINT('Ctrl Pts',(-4.13861213501102,-0.794772684000699,
8.36558627578272));
#36425=CARTESIAN_POINT('Ctrl Pts',(-4.08517130083353,-0.636309800095075,
8.35251835237303));
#36426=CARTESIAN_POINT('Ctrl Pts',(-4.01088514461499,-0.319434907277098,
8.34756649540242));
#36427=CARTESIAN_POINT('Ctrl Pts',(-3.99249114174688,-0.158333333333302,
8.35057250956555));
#36428=CARTESIAN_POINT('Ctrl Pts',(-3.98668829928627,0.158333333333304,
8.37058162387864));
#36429=CARTESIAN_POINT('Ctrl Pts',(-3.99965319507378,0.319434907277107,
8.38677599326486));
#36430=CARTESIAN_POINT('Ctrl Pts',(-4.06135810695932,0.636309800095085,
8.43413230172235));
#36431=CARTESIAN_POINT('Ctrl Pts',(-4.10832680843737,0.794772684000687,
8.46757637384159));
#36432=CARTESIAN_POINT('Ctrl Pts',(-4.23206754042395,1.06847604194534,8.53210485181926));
#36433=CARTESIAN_POINT('Ctrl Pts',(-4.29766467805669,1.18514270861241,8.56307409624329));
#36434=CARTESIAN_POINT('Ctrl Pts',(-4.37529617549109,1.30000000000103,8.59708059799053));
#36435=CARTESIAN_POINT('Ctrl Pts',(-4.44386598093114,-1.30000000000411,
8.40580624828163));
#36436=CARTESIAN_POINT('Ctrl Pts',(-4.36209777541527,-1.1851427086145,8.39590606023192));
#36437=CARTESIAN_POINT('Ctrl Pts',(-4.29216674290469,-1.0684760419464,8.38656864163037));
#36438=CARTESIAN_POINT('Ctrl Pts',(-4.15795830581166,-0.794772684000692,
8.36629744672359));
#36439=CARTESIAN_POINT('Ctrl Pts',(-4.1043911877798,-0.636309800095068,
8.34972927827051));
#36440=CARTESIAN_POINT('Ctrl Pts',(-4.0303296578903,-0.319434907277094,
8.34280141108802));
#36441=CARTESIAN_POINT('Ctrl Pts',(-4.01099725901343,-0.158333333333301,
8.34549045978168));
#36442=CARTESIAN_POINT('Ctrl Pts',(-4.00518509494333,0.158333333333303,
8.36559053335744));
#36443=CARTESIAN_POINT('Ctrl Pts',(-4.01915231905867,0.319434907277104,
8.38197995070172));
#36444=CARTESIAN_POINT('Ctrl Pts',(-4.08046440418983,0.636309800095079,
8.43193116150102));
#36445=CARTESIAN_POINT('Ctrl Pts',(-4.12714006947675,0.794772684000679,
8.470189810946));
#36446=CARTESIAN_POINT('Ctrl Pts',(-4.24806959090074,1.06847604194533,8.53526181972456));
#36447=CARTESIAN_POINT('Ctrl Pts',(-4.31192641504674,1.1851427086124,8.5653946542121));
#36448=CARTESIAN_POINT('Ctrl Pts',(-4.3872941543946,1.30000000000101,8.59749306174244));
#36449=CARTESIAN_POINT('Ctrl Pts',(-4.45581389180656,-1.30000000000389,
8.40486348086234));
#36450=CARTESIAN_POINT('Ctrl Pts',(-4.37635417638695,-1.1851427086143,8.39545398101981));
#36451=CARTESIAN_POINT('Ctrl Pts',(-4.30815058881763,-1.06847604194623,
8.386354586336));
#36452=CARTESIAN_POINT('Ctrl Pts',(-4.1765905645673,-0.794772684000559,
8.36604956924188));
#36453=CARTESIAN_POINT('Ctrl Pts',(-4.12289143621399,-0.636309800094961,
8.34852785954195));
#36454=CARTESIAN_POINT('Ctrl Pts',(-4.04911224368695,-0.319434907277039,
8.34084171680965));
#36455=CARTESIAN_POINT('Ctrl Pts',(-4.02906394959355,-0.158333333333274,
8.3429410583932));
#36456=CARTESIAN_POINT('Ctrl Pts',(-4.02322438445646,0.158333333333276,
8.36310480910221));
#36457=CARTESIAN_POINT('Ctrl Pts',(-4.03791161393723,0.319434907277051,
8.37994596770624));
#36458=CARTESIAN_POINT('Ctrl Pts',(-4.09882136162751,0.636309800094973,
8.43119589202976));
#36459=CARTESIAN_POINT('Ctrl Pts',(-4.14540012634608,0.794772684000544,
8.47153457102627));
#36460=CARTESIAN_POINT('Ctrl Pts',(-4.26369021134847,1.06847604194515,8.53677119739374));
#36461=CARTESIAN_POINT('Ctrl Pts',(-4.32588176501405,1.1851427086122,8.56647926923266));
#36462=CARTESIAN_POINT('Ctrl Pts',(-4.39906147762723,1.30000000000079,8.59765689461122));
#36463=CARTESIAN_POINT('Ctrl Pts',(-4.47075640156972,-1.3000000000037,8.40366332508016));
#36464=CARTESIAN_POINT('Ctrl Pts',(-4.39408547423049,-1.18514270861413,
8.39449920403769));
#36465=CARTESIAN_POINT('Ctrl Pts',(-4.32788474088457,-1.06847604194607,
8.38571258744119));
#36466=CARTESIAN_POINT('Ctrl Pts',(-4.19913604612478,-0.794772684000445,
8.36628585613646));
#36467=CARTESIAN_POINT('Ctrl Pts',(-4.14455012992047,-0.63630980009487,
8.35020437312365));
#36468=CARTESIAN_POINT('Ctrl Pts',(-4.07082622887265,-0.319434907276994,
8.34232785746959));
#36469=CARTESIAN_POINT('Ctrl Pts',(-4.05018226442897,-0.158333333333251,
8.34251620036384));
#36470=CARTESIAN_POINT('Ctrl Pts',(-4.04443109382666,0.158333333333253,
8.36216210760339));
#36471=CARTESIAN_POINT('Ctrl Pts',(-4.05996668533522,0.319434907277002,
8.3795672648057));
#36472=CARTESIAN_POINT('Ctrl Pts',(-4.12066653339907,0.636309800094878,
8.43164168452648));
#36473=CARTESIAN_POINT('Ctrl Pts',(-4.16747651626436,0.794772684000431,
8.47359690481767));
#36474=CARTESIAN_POINT('Ctrl Pts',(-4.28289918668377,1.068476041945,8.53841973135357));
#36475=CARTESIAN_POINT('Ctrl Pts',(-4.34319383731295,1.18514270861203,8.56746214337356));
#36476=CARTESIAN_POINT('Ctrl Pts',(-4.4138209413781,1.3000000000006,8.59748756772854));
#36477=CARTESIAN_POINT('Ctrl Pts',(-4.48584345896765,-1.30000000000344,
8.40202163820259));
#36478=CARTESIAN_POINT('Ctrl Pts',(-4.41216396723739,-1.1851427086139,8.39306715726315));
#36479=CARTESIAN_POINT('Ctrl Pts',(-4.34811956953621,-1.06847604194586,
8.3846166180924));
#36480=CARTESIAN_POINT('Ctrl Pts',(-4.22242319351063,-0.794772684000284,
8.36625838838242));
#36481=CARTESIAN_POINT('Ctrl Pts',(-4.16699602803123,-0.636309800094742,
8.35177995975142));
#36482=CARTESIAN_POINT('Ctrl Pts',(-4.09327754286868,-0.31943490727693,
8.34441429358004));
#36483=CARTESIAN_POINT('Ctrl Pts',(-4.07191265586848,-0.158333333333219,
8.34314884305873));
#36484=CARTESIAN_POINT('Ctrl Pts',(-4.06596905594175,0.158333333333221,
8.36356395927886));
#36485=CARTESIAN_POINT('Ctrl Pts',(-4.08191651241254,0.31943490727694,8.38361776836517));
#36486=CARTESIAN_POINT('Ctrl Pts',(-4.14245654330086,0.636309800094752,
8.43588114455287));
#36487=CARTESIAN_POINT('Ctrl Pts',(-4.19024487723722,0.794772684000271,
8.47580430836259));
#36488=CARTESIAN_POINT('Ctrl Pts',(-4.3027596398058,1.06847604194478,8.53915043374496));
#36489=CARTESIAN_POINT('Ctrl Pts',(-4.36098091201217,1.18514270861179,8.56760429441749));
#36490=CARTESIAN_POINT('Ctrl Pts',(-4.42871998479172,1.30000000000034,8.59709182528973));
#36491=CARTESIAN_POINT('Ctrl Pts',(-4.49796178306258,-1.30000000000328,
8.39985529775308));
#36492=CARTESIAN_POINT('Ctrl Pts',(-4.4265716679256,-1.18514270861375,8.39102831551921));
#36493=CARTESIAN_POINT('Ctrl Pts',(-4.3641669090176,-1.06847604194573,8.38286387332469));
#36494=CARTESIAN_POINT('Ctrl Pts',(-4.24075740231498,-0.794772684000189,
8.36553297859603));
#36495=CARTESIAN_POINT('Ctrl Pts',(-4.18466518323386,-0.636309800094665,
8.35239895718667));
#36496=CARTESIAN_POINT('Ctrl Pts',(-4.11077564597456,-0.319434907276892,
8.34628584930232));
#36497=CARTESIAN_POINT('Ctrl Pts',(-4.08858028343262,-0.1583333333332,8.34531114978367));
#36498=CARTESIAN_POINT('Ctrl Pts',(-4.08246237772048,0.158333333333202,
8.36639209712338));
#36499=CARTESIAN_POINT('Ctrl Pts',(-4.09895492167411,0.319434907276901,
8.38716863132232));
#36500=CARTESIAN_POINT('Ctrl Pts',(-4.15953722291765,0.636309800094675,
8.43882757144716));
#36501=CARTESIAN_POINT('Ctrl Pts',(-4.20818172714539,0.794772684000175,
8.4769038044228));
#36502=CARTESIAN_POINT('Ctrl Pts',(-4.31847323885501,1.06847604194465,8.53929490820517));
#36503=CARTESIAN_POINT('Ctrl Pts',(-4.37507204160506,1.18514270861165,8.56754341388116));
#36504=CARTESIAN_POINT('Ctrl Pts',(-4.44052853838925,1.30000000000019,8.59703362822392));
#36505=CARTESIAN_POINT('Ctrl Pts',(-4.51007860939701,-1.30000000000315,
8.3979383522798));
#36506=CARTESIAN_POINT('Ctrl Pts',(-4.44100930532193,-1.18514270861363,
8.38941168788246));
#36507=CARTESIAN_POINT('Ctrl Pts',(-4.38027215191213,-1.06847604194562,
8.38162370178122));
#36508=CARTESIAN_POINT('Ctrl Pts',(-4.25920611198825,-0.794772684000105,
8.36533839054226));
#36509=CARTESIAN_POINT('Ctrl Pts',(-4.20248488562437,-0.636309800094599,
8.35323389895756));
#36510=CARTESIAN_POINT('Ctrl Pts',(-4.12844451407313,-0.319434907276858,
8.34819835713744));
#36511=CARTESIAN_POINT('Ctrl Pts',(-4.10532022283471,-0.158333333333184,
8.34776543894798));
#36512=CARTESIAN_POINT('Ctrl Pts',(-4.0991761536252,0.158333333333186,8.36890156372869));
#36513=CARTESIAN_POINT('Ctrl Pts',(-4.11660188214324,0.319434907276868,
8.3889786766779));
#36514=CARTESIAN_POINT('Ctrl Pts',(-4.17721976246158,0.636309800094609,
8.440105936855));
#36515=CARTESIAN_POINT('Ctrl Pts',(-4.22627658771814,0.794772684000092,
8.47825264716756));
#36516=CARTESIAN_POINT('Ctrl Pts',(-4.33422678212072,1.06847604194454,8.53984899167736));
#36517=CARTESIAN_POINT('Ctrl Pts',(-4.38921285224113,1.18514270861152,8.56761729879319));
#36518=CARTESIAN_POINT('Ctrl Pts',(-4.45245735327389,1.30000000000005,8.596491137856));
#36519=CARTESIAN_POINT('Ctrl Pts',(-4.53106911977121,-1.30000000000305,
8.39593541505668));
#36520=CARTESIAN_POINT('Ctrl Pts',(-4.4660914337767,-1.18514270861354,8.38735736377513));
#36521=CARTESIAN_POINT('Ctrl Pts',(-4.40831205489554,-1.06847604194554,
8.37973152868131));
#36522=CARTESIAN_POINT('Ctrl Pts',(-4.29145966040395,-0.794772684000049,
8.36431413395546));
#36523=CARTESIAN_POINT('Ctrl Pts',(-4.23375442648326,-0.636309800094552,
8.35356438794742));
#36524=CARTESIAN_POINT('Ctrl Pts',(-4.15956532476393,-0.319434907276834,
8.34996167513517));
#36525=CARTESIAN_POINT('Ctrl Pts',(-4.13497148445359,-0.158333333333172,
8.35005035444579));
#36526=CARTESIAN_POINT('Ctrl Pts',(-4.12857804521935,0.158333333333174,
8.37223496440372));
#36527=CARTESIAN_POINT('Ctrl Pts',(-4.14703263166815,0.319434907276844,
8.39362037831457));
#36528=CARTESIAN_POINT('Ctrl Pts',(-4.207681000708,0.636309800094562,8.44385881569951));
#36529=CARTESIAN_POINT('Ctrl Pts',(-4.25809253894196,0.794772684000033,
8.47913032176147));
#36530=CARTESIAN_POINT('Ctrl Pts',(-4.36205133787161,1.06847604194446,8.53907191087305));
#36531=CARTESIAN_POINT('Ctrl Pts',(-4.41416449316683,1.18514270861144,8.56640563709156));
#36532=CARTESIAN_POINT('Ctrl Pts',(-4.47339089175368,1.29999999999995,8.59512659665689));
#36533=CARTESIAN_POINT('Ctrl Pts',(-4.56150565654056,-1.30000000000123,
8.38949940982674));
#36534=CARTESIAN_POINT('Ctrl Pts',(-4.50244338963643,-1.18514270861188,
8.38033582366812));
#36535=CARTESIAN_POINT('Ctrl Pts',(-4.44890849532253,-1.06847604194404,
8.37283373114573));
#36536=CARTESIAN_POINT('Ctrl Pts',(-4.33800151626977,-0.794772683998929,
8.35934077931099));
#36537=CARTESIAN_POINT('Ctrl Pts',(-4.27864161246945,-0.63630980009366,
8.35265240911047));
#36538=CARTESIAN_POINT('Ctrl Pts',(-4.2040464737142,-0.319434907276387,
8.35253483013444));
#36539=CARTESIAN_POINT('Ctrl Pts',(-4.17712750120142,-0.15833333333295,
8.35434255827378));
#36540=CARTESIAN_POINT('Ctrl Pts',(-4.17062388918443,0.158333333332952,
8.37694849962917));
#36541=CARTESIAN_POINT('Ctrl Pts',(-4.19133310937807,0.319434907276396,
8.39654062259916));
#36542=CARTESIAN_POINT('Ctrl Pts',(-4.25208228768441,0.636309800093669,
8.44516159542419));
#36543=CARTESIAN_POINT('Ctrl Pts',(-4.30369303470636,0.794772683998919,
8.47961188578339));
#36544=CARTESIAN_POINT('Ctrl Pts',(-4.4017359065261,1.06847604194297,8.53808733355857));
#36545=CARTESIAN_POINT('Ctrl Pts',(-4.44974244953311,1.18514270860978,8.56478284930283));
#36546=CARTESIAN_POINT('Ctrl Pts',(-4.50331640918273,1.29999999999814,8.59286202617833));
#36547=CARTESIAN_POINT('Ctrl Pts',(-4.59169939732753,-1.30000000000067,
8.3846346623458));
#36548=CARTESIAN_POINT('Ctrl Pts',(-4.53841605520976,-1.18514270861137,
8.37598483604062));
#36549=CARTESIAN_POINT('Ctrl Pts',(-4.48909322327351,-1.06847604194358,
8.36894569229234));
#36550=CARTESIAN_POINT('Ctrl Pts',(-4.38429718531943,-0.794772683998593,
8.35640486098037));
#36551=CARTESIAN_POINT('Ctrl Pts',(-4.32383495195998,-0.636309800093389,
8.34978771198848));
#36552=CARTESIAN_POINT('Ctrl Pts',(-4.24917041175543,-0.319434907276251,
8.35113767529032));
#36553=CARTESIAN_POINT('Ctrl Pts',(-4.2200309626269,-0.158333333332882,
8.35464748725542));
#36554=CARTESIAN_POINT('Ctrl Pts',(-4.21330443794114,0.158333333332884,
8.37837348494326));
#36555=CARTESIAN_POINT('Ctrl Pts',(-4.23586855189251,0.319434907276259,
8.39806561965051));
#36556=CARTESIAN_POINT('Ctrl Pts',(-4.29652368349501,0.636309800093397,
8.44611125949594));
#36557=CARTESIAN_POINT('Ctrl Pts',(-4.34948336474048,0.794772683998581,
8.47911759872889));
#36558=CARTESIAN_POINT('Ctrl Pts',(-4.44149850175252,1.06847604194251,8.53678390432497));
#36559=CARTESIAN_POINT('Ctrl Pts',(-4.48531559698022,1.18514270860927,8.56328821396476));
#36560=CARTESIAN_POINT('Ctrl Pts',(-4.53311984411989,1.29999999999758,8.59133522629897));
#36561=CARTESIAN_POINT('Ctrl Pts',(-4.61597083254814,-1.30000000000025,
8.37961235158112));
#36562=CARTESIAN_POINT('Ctrl Pts',(-4.56749114781657,-1.18514270861098,
8.36964515588487));
#36563=CARTESIAN_POINT('Ctrl Pts',(-4.52164350144129,-1.06847604194323,
8.36197774758551));
#36564=CARTESIAN_POINT('Ctrl Pts',(-4.42180680166536,-0.79477268399833,
8.349577469512));
#36565=CARTESIAN_POINT('Ctrl Pts',(-4.36020003889848,-0.636309800093179,
8.34555660847258));
#36566=CARTESIAN_POINT('Ctrl Pts',(-4.28539468703016,-0.319434907276146,
8.34909085241622));
#36567=CARTESIAN_POINT('Ctrl Pts',(-4.25450152199579,-0.15833333333283,
8.35391668965212));
#36568=CARTESIAN_POINT('Ctrl Pts',(-4.24763644272708,0.158333333332832,
8.37845901604611));
#36569=CARTESIAN_POINT('Ctrl Pts',(-4.27175720512554,0.319434907276154,
8.39781547154599));
#36570=CARTESIAN_POINT('Ctrl Pts',(-4.33239010919754,0.636309800093188,
8.44500554199925));
#36571=CARTESIAN_POINT('Ctrl Pts',(-4.38643587888284,0.794772683998319,
8.4765648173077));
#36572=CARTESIAN_POINT('Ctrl Pts',(-4.47363483284698,1.06847604194216,8.53351665496209));
#36573=CARTESIAN_POINT('Ctrl Pts',(-4.51409770384844,1.18514270860888,8.55991989753419));
#36574=CARTESIAN_POINT('Ctrl Pts',(-4.55727824971992,1.29999999999715,8.58807404243134));
#36575=CARTESIAN_POINT('Ctrl Pts',(-4.63419695389682,-1.29999999999978,
8.37547771778039));
#36576=CARTESIAN_POINT('Ctrl Pts',(-4.58919288393035,-1.18514270861056,
8.3657354368593));
#36577=CARTESIAN_POINT('Ctrl Pts',(-4.54587154765948,-1.06847604194285,
8.35835394360906));
#36578=CARTESIAN_POINT('Ctrl Pts',(-4.44967804593736,-0.794772683998049,
8.34675510933199));
#36579=CARTESIAN_POINT('Ctrl Pts',(-4.38731242984226,-0.636309800092953,
8.34358113784012));
#36580=CARTESIAN_POINT('Ctrl Pts',(-4.3125118722081,-0.319434907276032,
8.3478546023281));
#36581=CARTESIAN_POINT('Ctrl Pts',(-4.28044235230206,-0.158333333332774,
8.35274872547764));
#36582=CARTESIAN_POINT('Ctrl Pts',(-4.27351671455972,0.158333333332776,
8.3775853109577));
#36583=CARTESIAN_POINT('Ctrl Pts',(-4.2987586842706,0.319434907276041,8.39702114369619));
#36584=CARTESIAN_POINT('Ctrl Pts',(-4.35925241921496,0.636309800092963,
8.44436998353798));
#36585=CARTESIAN_POINT('Ctrl Pts',(-4.41391057284775,0.794772683998036,
8.47615970930566));
#36586=CARTESIAN_POINT('Ctrl Pts',(-4.49745258358852,1.06847604194178,8.53285635263349));
#36587=CARTESIAN_POINT('Ctrl Pts',(-4.53542189161,1.18514270860846,8.55903248064369));
#36588=CARTESIAN_POINT('Ctrl Pts',(-4.57519826673979,1.29999999999669,8.58684286058509));
#36589=CARTESIAN_POINT('Ctrl Pts',(-4.65239690742634,-1.29999999999925,
8.37146876966087));
#36590=CARTESIAN_POINT('Ctrl Pts',(-4.61097032453698,-1.18514270861007,
8.36085690229744));
#36591=CARTESIAN_POINT('Ctrl Pts',(-4.57024914788923,-1.06847604194241,
8.3530118089499));
#36592=CARTESIAN_POINT('Ctrl Pts',(-4.47780471312426,-0.794772683997723,
8.34127987537955));
#36593=CARTESIAN_POINT('Ctrl Pts',(-4.41468297213334,-0.63630980009269,
8.33935590736899));
#36594=CARTESIAN_POINT('Ctrl Pts',(-4.33983425300278,-0.319434907275899,
8.34498441267624));
#36595=CARTESIAN_POINT('Ctrl Pts',(-4.30644484530562,-0.158333333332708,
8.35107549269899));
#36596=CARTESIAN_POINT('Ctrl Pts',(-4.2994246769601,0.15833333333271,8.37656059683744));
#36597=CARTESIAN_POINT('Ctrl Pts',(-4.32582229625926,0.319434907275909,
8.39580990391751));
#36598=CARTESIAN_POINT('Ctrl Pts',(-4.38631363002924,0.636309800092699,
8.44238749893344));
#36599=CARTESIAN_POINT('Ctrl Pts',(-4.44184660082066,0.794772683997706,
8.47258005635774));
#36600=CARTESIAN_POINT('Ctrl Pts',(-4.52173596106959,1.06847604194134,8.52901154981768));
#36601=CARTESIAN_POINT('Ctrl Pts',(-4.55715003109018,1.18514270860797,8.55540087922434));
#36602=CARTESIAN_POINT('Ctrl Pts',(-4.59339702727207,1.29999999999615,8.58375243551171));
#36603=CARTESIAN_POINT('Ctrl Pts',(-4.67662765556481,-1.29999999999835,
8.36638064005668));
#36604=CARTESIAN_POINT('Ctrl Pts',(-4.6399265403655,-1.18514270860925,8.35506988887774));
#36605=CARTESIAN_POINT('Ctrl Pts',(-4.60264173680922,-1.06847604194167,
8.34690329443953));
#36606=CARTESIAN_POINT('Ctrl Pts',(-4.51515794492436,-0.794772683997172,
8.33530045862321));
#36607=CARTESIAN_POINT('Ctrl Pts',(-4.45104183914462,-0.63630980009225,
8.33471367558874));
#36608=CARTESIAN_POINT('Ctrl Pts',(-4.37615858752344,-0.319434907275679,
8.34182081472496));
#36609=CARTESIAN_POINT('Ctrl Pts',(-4.3410379233413,-0.158333333332599,
8.34929253009869));
#36610=CARTESIAN_POINT('Ctrl Pts',(-4.33396356331471,0.158333333332601,
8.37509679924112));
#36611=CARTESIAN_POINT('Ctrl Pts',(-4.36205431788642,0.31943490727569,8.39302674220606));
#36612=CARTESIAN_POINT('Ctrl Pts',(-4.42243706520714,0.636309800092261,
8.43930113056221));
#36613=CARTESIAN_POINT('Ctrl Pts',(-4.47875680438225,0.794772683997159,
8.47003111695546));
#36614=CARTESIAN_POINT('Ctrl Pts',(-4.55370323347117,1.0684760419406,8.52660505233009));
#36615=CARTESIAN_POINT('Ctrl Pts',(-4.58574695648383,1.18514270860715,8.55301302704109));
#36616=CARTESIAN_POINT('Ctrl Pts',(-4.61739287039539,1.29999999999525,8.58134021611028));
#36617=CARTESIAN_POINT('Ctrl Pts',(-4.69789919864171,-1.29999999999678,
8.36090082369946));
#36618=CARTESIAN_POINT('Ctrl Pts',(-4.66536018132445,-1.18514270860782,
8.34847304056692));
#36619=CARTESIAN_POINT('Ctrl Pts',(-4.63110015263561,-1.06847604194038,
8.33973082770565));
#36620=CARTESIAN_POINT('Ctrl Pts',(-4.54797675211423,-0.794772683996213,
8.32804897174489));
#36621=CARTESIAN_POINT('Ctrl Pts',(-4.48294097752206,-0.636309800091482,
8.3295239875756));
#36622=CARTESIAN_POINT('Ctrl Pts',(-4.4080743825454,-0.319434907275293,
8.33788201166714));
#36623=CARTESIAN_POINT('Ctrl Pts',(-4.37158871913637,-0.158333333332408,
8.34554546637412));
#36624=CARTESIAN_POINT('Ctrl Pts',(-4.36441939582717,0.15833333333241,8.37203984518833));
#36625=CARTESIAN_POINT('Ctrl Pts',(-4.39371384560967,0.319434907275301,
8.39075278554675));
#36626=CARTESIAN_POINT('Ctrl Pts',(-4.45402163421419,0.63630980009149,8.43660222784233));
#36627=CARTESIAN_POINT('Ctrl Pts',(-4.51138877020508,0.794772683996199,
8.46519550192625));
#36628=CARTESIAN_POINT('Ctrl Pts',(-4.58202224890887,1.06847604193931,8.52184443050647));
#36629=CARTESIAN_POINT('Ctrl Pts',(-4.61105314249528,1.18514270860572,8.54875829622621));
#36630=CARTESIAN_POINT('Ctrl Pts',(-4.63854031396548,1.29999999999368,8.57806480553295));
#36631=CARTESIAN_POINT('Ctrl Pts',(-4.7161409482319,-1.2999999999962,8.35590271413686));
#36632=CARTESIAN_POINT('Ctrl Pts',(-4.68713869592175,-1.1851427086073,8.34279578720867));
#36633=CARTESIAN_POINT('Ctrl Pts',(-4.65546276338965,-1.06847604193991,
8.33362197404163));
#36634=CARTESIAN_POINT('Ctrl Pts',(-4.57610828631184,-0.794772683995863,
8.32151491001579));
#36635=CARTESIAN_POINT('Ctrl Pts',(-4.51045420438319,-0.636309800091202,
8.3230585656632));
#36636=CARTESIAN_POINT('Ctrl Pts',(-4.43556241906787,-0.319434907275153,
8.33283856066987));
#36637=CARTESIAN_POINT('Ctrl Pts',(-4.39766426030354,-0.158333333332338,
8.34294220161402));
#36638=CARTESIAN_POINT('Ctrl Pts',(-4.39039693442986,0.15833333333234,8.37036241559784));
#36639=CARTESIAN_POINT('Ctrl Pts',(-4.42095202386697,0.319434907275162,
8.38797320825141));
#36640=CARTESIAN_POINT('Ctrl Pts',(-4.48119507360353,0.636309800091212,
8.4334469106398));
#36641=CARTESIAN_POINT('Ctrl Pts',(-4.53922661725484,0.79477268399585,8.4618577332553));
#36642=CARTESIAN_POINT('Ctrl Pts',(-4.60615474087746,1.06847604193884,8.51866629487098));
#36643=CARTESIAN_POINT('Ctrl Pts',(-4.6326429935655,1.1851427086052,8.5457569896651));
#36644=CARTESIAN_POINT('Ctrl Pts',(-4.65664879415669,1.29999999999311,8.57534805789455));
#36645=CARTESIAN_POINT('Ctrl Pts',(-4.72823715178914,-1.29999999999609,
8.35339014157118));
#36646=CARTESIAN_POINT('Ctrl Pts',(-4.70157648358082,-1.1851427086072,8.34013566417898));
#36647=CARTESIAN_POINT('Ctrl Pts',(-4.6716106932305,-1.06847604193982,8.33087284428749));
#36648=CARTESIAN_POINT('Ctrl Pts',(-4.59474822955049,-0.794772683995793,
8.31869540467249));
#36649=CARTESIAN_POINT('Ctrl Pts',(-4.52863710511104,-0.636309800091145,
8.32041158642372));
#36650=CARTESIAN_POINT('Ctrl Pts',(-4.45380783327018,-0.319434907275124,
8.33028811432542));
#36651=CARTESIAN_POINT('Ctrl Pts',(-4.41513333680483,-0.158333333332324,
8.34052686594499));
#36652=CARTESIAN_POINT('Ctrl Pts',(-4.40788109043004,0.158333333332326,
8.36780256651529));
#36653=CARTESIAN_POINT('Ctrl Pts',(-4.43925339017667,0.319434907275135,
8.38489298636552));
#36654=CARTESIAN_POINT('Ctrl Pts',(-4.49941210358521,0.636309800091156,
8.4304661802376));
#36655=CARTESIAN_POINT('Ctrl Pts',(-4.55779440082702,0.794772683995778,
8.45954256857753));
#36656=CARTESIAN_POINT('Ctrl Pts',(-4.62223204623287,1.06847604193874,8.51666493827882));
#36657=CARTESIAN_POINT('Ctrl Pts',(-4.64703395571431,1.18514270860509,8.54382151210089));
#36658=CARTESIAN_POINT('Ctrl Pts',(-4.66874510563104,1.29999999999299,8.57340850249371));
#36659=CARTESIAN_POINT('Ctrl Pts',(-4.74340335118311,-1.29999999999471,
8.34928292021594));
#36660=CARTESIAN_POINT('Ctrl Pts',(-4.71975192723288,-1.18514270860593,
8.33452631874549));
#36661=CARTESIAN_POINT('Ctrl Pts',(-4.69197337306874,-1.06847604193868,
8.32439339815895));
#36662=CARTESIAN_POINT('Ctrl Pts',(-4.61826485944567,-0.794772683994948,
8.3116659523263));
#36663=CARTESIAN_POINT('Ctrl Pts',(-4.55150389070566,-0.63630980009047,
8.31530639162805));
#36664=CARTESIAN_POINT('Ctrl Pts',(-4.47666293354192,-0.319434907274786,
8.32657119999817));
#36665=CARTESIAN_POINT('Ctrl Pts',(-4.43694261924442,-0.158333333332156,
8.337662514481));
#36666=CARTESIAN_POINT('Ctrl Pts',(-4.42961852259884,0.158333333332158,
8.3655893801562));
#36667=CARTESIAN_POINT('Ctrl Pts',(-4.46192298299084,0.319434907274794,
8.38263381659107));
#36668=CARTESIAN_POINT('Ctrl Pts',(-4.52203218557171,0.636309800090479,
8.4278285386015));
#36669=CARTESIAN_POINT('Ctrl Pts',(-4.58109824215759,0.794772683994937,
8.45573367388843));
#36670=CARTESIAN_POINT('Ctrl Pts',(-4.64245005899539,1.06847604193761,8.51300720003524));
#36671=CARTESIAN_POINT('Ctrl Pts',(-4.6651086871392,1.18514270860383,8.54052734185137));
#36672=CARTESIAN_POINT('Ctrl Pts',(-4.68386901522655,1.29999999999161,8.57077603820792));
#36673=CARTESIAN_POINT('Ctrl Pts',(-4.76167893245149,-1.29999999999383,
8.34369189625078));
#36674=CARTESIAN_POINT('Ctrl Pts',(-4.74150919494958,-1.18514270860513,
8.32887343937279));
#36675=CARTESIAN_POINT('Ctrl Pts',(-4.7162784389449,-1.06847604193795,8.31869365207076));
#36676=CARTESIAN_POINT('Ctrl Pts',(-4.64629837998445,-0.794772683994407,
8.30589256162683));
#36677=CARTESIAN_POINT('Ctrl Pts',(-4.57891469655928,-0.636309800090037,
8.30930913056515));
#36678=CARTESIAN_POINT('Ctrl Pts',(-4.50415702674796,-0.319434907274568,
8.32100124625156));
#36679=CARTESIAN_POINT('Ctrl Pts',(-4.46324312599945,-0.158333333332048,
8.33279575559108));
#36680=CARTESIAN_POINT('Ctrl Pts',(-4.45585255642742,0.15833333333205,8.36145869754515));
#36681=CARTESIAN_POINT('Ctrl Pts',(-4.48922780131988,0.319434907274574,
8.37907070770448));
#36682=CARTESIAN_POINT('Ctrl Pts',(-4.54923305414967,0.636309800090044,
8.42424832705878));
#36683=CARTESIAN_POINT('Ctrl Pts',(-4.6090698142711,0.794772683994395,8.45098139609059));
#36684=CARTESIAN_POINT('Ctrl Pts',(-4.66671552092437,1.06847604193688,8.50848521847131));
#36685=CARTESIAN_POINT('Ctrl Pts',(-4.68681425050692,1.18514270860302,8.53638505230757));
#36686=CARTESIAN_POINT('Ctrl Pts',(-4.70205901924573,1.29999999999073,8.56729344599807));
#36687=CARTESIAN_POINT('Ctrl Pts',(-4.77982710526041,-1.29999999999232,
8.33905011299784));
#36688=CARTESIAN_POINT('Ctrl Pts',(-4.76326639868391,-1.18514270860376,
8.32231210199745));
#36689=CARTESIAN_POINT('Ctrl Pts',(-4.74065971664241,-1.06847604193671,
8.3110086941711));
#36690=CARTESIAN_POINT('Ctrl Pts',(-4.67446634585838,-0.794772683993484,
8.29745058137394));
#36691=CARTESIAN_POINT('Ctrl Pts',(-4.60627902145023,-0.636309800089299,
8.30355111374383));
#36692=CARTESIAN_POINT('Ctrl Pts',(-4.53157317325735,-0.319434907274198,
8.31633606172721));
#36693=CARTESIAN_POINT('Ctrl Pts',(-4.48949570989188,-0.158333333331864,
8.32826416125297));
#36694=CARTESIAN_POINT('Ctrl Pts',(-4.48213234554617,0.158333333331866,
8.35668177661298));
#36695=CARTESIAN_POINT('Ctrl Pts',(-4.51675009789326,0.319434907274205,
8.37315955889524));
#36696=CARTESIAN_POINT('Ctrl Pts',(-4.57665355432879,0.636309800089306,
8.41828314766454));
#36697=CARTESIAN_POINT('Ctrl Pts',(-4.6370722671515,0.794772683993473,8.44570568631553));
#36698=CARTESIAN_POINT('Ctrl Pts',(-4.69093818547079,1.06847604193564,8.50417913824327));
#36699=CARTESIAN_POINT('Ctrl Pts',(-4.70846533482425,1.18514270860165,8.5325837124655));
#36700=CARTESIAN_POINT('Ctrl Pts',(-4.72020307341969,1.29999999998922,8.56408187022532));
#36701=CARTESIAN_POINT('Ctrl Pts',(-4.79803343217889,-1.29999999999099,
8.33394511610362));
#36702=CARTESIAN_POINT('Ctrl Pts',(-4.7849677374734,-1.18514270860254,8.31688391588858));
#36703=CARTESIAN_POINT('Ctrl Pts',(-4.76492392505446,-1.06847604193562,
8.30527350198988));
#36704=CARTESIAN_POINT('Ctrl Pts',(-4.70249786073047,-0.794772683992672,
8.29104353004542));
#36705=CARTESIAN_POINT('Ctrl Pts',(-4.63374160723767,-0.636309800088648,
8.29620513161596));
#36706=CARTESIAN_POINT('Ctrl Pts',(-4.55911762196679,-0.319434907273871,
8.30950121211404));
#36707=CARTESIAN_POINT('Ctrl Pts',(-4.51578716586765,-0.158333333331702,
8.32306342541251));
#36708=CARTESIAN_POINT('Ctrl Pts',(-4.50832961490194,0.158333333331705,
8.35263978253959));
#36709=CARTESIAN_POINT('Ctrl Pts',(-4.54402552275341,0.319434907273878,
8.36952925941727));
#36710=CARTESIAN_POINT('Ctrl Pts',(-4.60381954438777,0.636309800088656,
8.41469509842377));
#36711=CARTESIAN_POINT('Ctrl Pts',(-4.66500217002981,0.79477268399266,8.44099914592903));
#36712=CARTESIAN_POINT('Ctrl Pts',(-4.71516619093475,1.06847604193455,8.49972033154497));
#36713=CARTESIAN_POINT('Ctrl Pts',(-4.73013805396894,1.18514270860044,8.5284997162424));
#36714=CARTESIAN_POINT('Ctrl Pts',(-4.7383676341477,1.29999999998789,8.56064026021845));
#36715=CARTESIAN_POINT('Ctrl Pts',(-4.81094149750922,-1.29999999998978,
8.32978009402368));
#36716=CARTESIAN_POINT('Ctrl Pts',(-4.80039230401006,-1.18514270860144,
8.31169231381476));
#36717=CARTESIAN_POINT('Ctrl Pts',(-4.7821836182234,-1.06847604193462,8.29946834001264));
#36718=CARTESIAN_POINT('Ctrl Pts',(-4.72242295196123,-0.794772683991931,
8.28477508098243));
#36719=CARTESIAN_POINT('Ctrl Pts',(-4.65316124219068,-0.636309800088055,
8.29111147785697));
#36720=CARTESIAN_POINT('Ctrl Pts',(-4.57857606554552,-0.319434907273573,
8.30524578386532));
#36721=CARTESIAN_POINT('Ctrl Pts',(-4.53438456950182,-0.158333333331555,
8.31951483890184));
#36722=CARTESIAN_POINT('Ctrl Pts',(-4.52692720614846,0.158333333331557,
8.34921452120318));
#36723=CARTESIAN_POINT('Ctrl Pts',(-4.56348734251723,0.31943490727358,8.36538523893045));
#36724=CARTESIAN_POINT('Ctrl Pts',(-4.62323682493845,0.636309800088062,
8.4102395363381));
#36725=CARTESIAN_POINT('Ctrl Pts',(-4.68491217123887,0.794772683991919,
8.43621329058605));
#36726=CARTESIAN_POINT('Ctrl Pts',(-4.73240589414762,1.06847604193355,8.49562341725007));
#36727=CARTESIAN_POINT('Ctrl Pts',(-4.74554246979028,1.18514270859933,8.52494769230183));
#36728=CARTESIAN_POINT('Ctrl Pts',(-4.75125734824424,1.29999999998668,8.5578797999346));
#36729=CARTESIAN_POINT('Ctrl Pts',(-4.81852392502146,-1.29999999998959,
8.32749751318685));
#36730=CARTESIAN_POINT('Ctrl Pts',(-4.80944615872512,-1.18514270860127,
8.30897667740979));
#36731=CARTESIAN_POINT('Ctrl Pts',(-4.79231288165303,-1.06847604193448,
8.29646873585038));
#36732=CARTESIAN_POINT('Ctrl Pts',(-4.73412174272511,-0.79477268399182,
8.2814638771612));
#36733=CARTESIAN_POINT('Ctrl Pts',(-4.66458809103075,-0.636309800087967,
8.2880031704567));
#36734=CARTESIAN_POINT('Ctrl Pts',(-4.59002800238769,-0.319434907273529,
8.30255284095863));
#36735=CARTESIAN_POINT('Ctrl Pts',(-4.54531512979248,-0.158333333331533,
8.31750113977235));
#36736=CARTESIAN_POINT('Ctrl Pts',(-4.53784740212769,0.158333333331535,
8.34739593227855));
#36737=CARTESIAN_POINT('Ctrl Pts',(-4.5749074249398,0.319434907273536,8.36318641560727));
#36738=CARTESIAN_POINT('Ctrl Pts',(-4.63463337044967,0.636309800087975,
8.4078111388242));
#36739=CARTESIAN_POINT('Ctrl Pts',(-4.69661484844976,0.794772683991809,
8.43341649612987));
#36740=CARTESIAN_POINT('Ctrl Pts',(-4.74254482298291,1.0684760419334,8.49317263346162));
#36741=CARTESIAN_POINT('Ctrl Pts',(-4.75460297195919,1.18514270859917,8.52281712210147));
#36742=CARTESIAN_POINT('Ctrl Pts',(-4.75883788580962,1.2999999999865,8.55623988171332));
#36743=CARTESIAN_POINT('Ctrl Pts',(-4.82041977295653,-1.29999999998959,
8.32691849490388));
#36744=CARTESIAN_POINT('Ctrl Pts',(-4.81170975047181,-1.18514270860127,
8.30828675594369));
#36745=CARTESIAN_POINT('Ctrl Pts',(-4.79484522454245,-1.06847604193447,
8.29570698049037));
#36746=CARTESIAN_POINT('Ctrl Pts',(-4.73704626164923,-0.794772683991816,
8.28062642900982));
#36747=CARTESIAN_POINT('Ctrl Pts',(-4.66744427478885,-0.636309800087964,
8.28722884049732));
#36748=CARTESIAN_POINT('Ctrl Pts',(-4.59289080743435,-0.319434907273528,
8.3018811056208));
#36749=CARTESIAN_POINT('Ctrl Pts',(-4.54804875165676,-0.158333333331532,
8.31698349332809));
#36750=CARTESIAN_POINT('Ctrl Pts',(-4.54057832594463,0.158333333331534,
8.3469283166452));
#36751=CARTESIAN_POINT('Ctrl Pts',(-4.57776226683473,0.319434907273535,
8.36263692754277));
#36752=CARTESIAN_POINT('Ctrl Pts',(-4.6374813242383,0.636309800087972,8.40721577472294));
#36753=CARTESIAN_POINT('Ctrl Pts',(-4.69953831741039,0.794772683991806,
8.43273932158352));
#36754=CARTESIAN_POINT('Ctrl Pts',(-4.74507757726615,1.0684760419334,8.49257974884738));
#36755=CARTESIAN_POINT('Ctrl Pts',(-4.75686656169974,1.18514270859916,8.52229970933397));
#36756=CARTESIAN_POINT('Ctrl Pts',(-4.7607322723712,1.29999999998649,8.55583692665094));
#36757=CARTESIAN_POINT('Ctrl Pts',(-4.82269479895944,-1.29999999998956,
8.32621878032447));
#36758=CARTESIAN_POINT('Ctrl Pts',(-4.8144260230379,-1.18514270860124,8.30745082409725));
#36759=CARTESIAN_POINT('Ctrl Pts',(-4.79788395737724,-1.06847604193445,
8.29478338814642));
#36760=CARTESIAN_POINT('Ctrl Pts',(-4.74055552210931,-0.7947726839918,8.27961249923156));
#36761=CARTESIAN_POINT('Ctrl Pts',(-4.67087133177399,-0.636309800087951,
8.28630024690135));
#36762=CARTESIAN_POINT('Ctrl Pts',(-4.59632606869179,-0.319434907273521,
8.30107481000781));
#36763=CARTESIAN_POINT('Ctrl Pts',(-4.55132986051768,-0.158333333331529,
8.3163499578362));
#36764=CARTESIAN_POINT('Ctrl Pts',(-4.54385592295093,0.158333333331531,
8.34635759780241));
#36765=CARTESIAN_POINT('Ctrl Pts',(-4.58118745436961,0.319434907273528,
8.36198104652681));
#36766=CARTESIAN_POINT('Ctrl Pts',(-4.64089736676338,0.636309800087958,
8.40651507099385));
#36767=CARTESIAN_POINT('Ctrl Pts',(-4.70304427261792,0.794772683991789,
8.43194799941686));
#36768=CARTESIAN_POINT('Ctrl Pts',(-4.7481150701394,1.06847604193338,8.49188621570782));
#36769=CARTESIAN_POINT('Ctrl Pts',(-4.75958153919977,1.18514270859914,8.52169207072452));
#36770=CARTESIAN_POINT('Ctrl Pts',(-4.76300499911106,1.29999999998647,8.55535874785532));
#36771=CARTESIAN_POINT('Ctrl Pts',(-4.82724518123329,-1.29999999998947,
8.32480162162588));
#36772=CARTESIAN_POINT('Ctrl Pts',(-4.81985877333475,-1.18514270860116,
8.30575213666847));
#36773=CARTESIAN_POINT('Ctrl Pts',(-4.80396149243278,-1.06847604193437,
8.29290542346446));
#36774=CARTESIAN_POINT('Ctrl Pts',(-4.7475737740772,-0.794772683991742,
8.27755658959772));
#36775=CARTESIAN_POINT('Ctrl Pts',(-4.67772434607518,-0.636309800087904,
8.28444559580218));
#36776=CARTESIAN_POINT('Ctrl Pts',(-4.60319626152197,-0.319434907273498,
8.29946273161348));
#36777=CARTESIAN_POINT('Ctrl Pts',(-4.55789440269426,-0.158333333331517,
8.31504728914924));
#36778=CARTESIAN_POINT('Ctrl Pts',(-4.5504130055163,0.158333333331519,8.34518520592664));
#36779=CARTESIAN_POINT('Ctrl Pts',(-4.58803698786698,0.319434907273504,
8.36067115696744));
#36780=CARTESIAN_POINT('Ctrl Pts',(-4.64772621923239,0.636309800087912,
8.4051431652836));
#36781=CARTESIAN_POINT('Ctrl Pts',(-4.71005075988252,0.794772683991732,
8.43041777479225));
#36782=CARTESIAN_POINT('Ctrl Pts',(-4.75418534119007,1.0684760419333,8.49054555455211));
#36783=CARTESIAN_POINT('Ctrl Pts',(-4.76500790392179,1.18514270859905,8.52051208905625));
#36784=CARTESIAN_POINT('Ctrl Pts',(-4.76754880448457,1.29999999998637,8.55441807016026));
#36785=CARTESIAN_POINT('Ctrl Pts',(-4.83445330411152,-1.29999999998922,
8.3224116128313));
#36786=CARTESIAN_POINT('Ctrl Pts',(-4.82846766580034,-1.18514270860093,
8.30278026328514));
#36787=CARTESIAN_POINT('Ctrl Pts',(-4.8135928108613,-1.06847604193417,8.28958539587345));
#36788=CARTESIAN_POINT('Ctrl Pts',(-4.7586930515559,-0.794772683991593,
8.27397217387284));
#36789=CARTESIAN_POINT('Ctrl Pts',(-4.68856715970435,-0.636309800087784,
8.2815609625007));
#36790=CARTESIAN_POINT('Ctrl Pts',(-4.6140701043017,-0.319434907273438,
8.29697865182959));
#36791=CARTESIAN_POINT('Ctrl Pts',(-4.56830640821597,-0.158333333331488,
8.31272251695755));
#36792=CARTESIAN_POINT('Ctrl Pts',(-4.56081294584385,0.15833333333149,8.34306422751495));
#36793=CARTESIAN_POINT('Ctrl Pts',(-4.59888398565192,0.319434907273445,
8.35854789869529));
#36794=CARTESIAN_POINT('Ctrl Pts',(-4.65852314139286,0.636309800087793,
8.40312972582311));
#36795=CARTESIAN_POINT('Ctrl Pts',(-4.7211081020808,0.794772683991581,8.42837394721402));
#36796=CARTESIAN_POINT('Ctrl Pts',(-4.76376426071759,1.0684760419331,8.4887680229739));
#36797=CARTESIAN_POINT('Ctrl Pts',(-4.77357562396977,1.18514270859883,8.51890352477032));
#36798=CARTESIAN_POINT('Ctrl Pts',(-4.77473407996669,1.29999999998613,8.55303217078774));
#36799=CARTESIAN_POINT('Ctrl Pts',(-4.84090172139479,-1.29999999998864,
8.32022306470272));
#36800=CARTESIAN_POINT('Ctrl Pts',(-4.83617138484706,-1.1851427086004,8.30000540687456));
#36801=CARTESIAN_POINT('Ctrl Pts',(-4.82221247131159,-1.06847604193369,
8.28646006688069));
#36802=CARTESIAN_POINT('Ctrl Pts',(-4.76864472956175,-0.794772683991235,
8.27058201074876));
#36803=CARTESIAN_POINT('Ctrl Pts',(-4.69826634496861,-0.636309800087498,
8.27890451007233));
#36804=CARTESIAN_POINT('Ctrl Pts',(-4.62380013668611,-0.319434907273293,
8.29467661136089));
#36805=CARTESIAN_POINT('Ctrl Pts',(-4.57763211214118,-0.158333333331416,
8.31048006764925));
#36806=CARTESIAN_POINT('Ctrl Pts',(-4.57013078277785,0.158333333331418,
8.3409843725767));
#36807=CARTESIAN_POINT('Ctrl Pts',(-4.60859948159869,0.319434907273301,
8.35648703793527));
#36808=CARTESIAN_POINT('Ctrl Pts',(-4.66818932641239,0.636309800087505,
8.40121676647618));
#36809=CARTESIAN_POINT('Ctrl Pts',(-4.73100056677066,0.794772683991223,
8.42650073147393));
#36810=CARTESIAN_POINT('Ctrl Pts',(-4.7723309702851,1.06847604193262,8.4871754226118));
#36811=CARTESIAN_POINT('Ctrl Pts',(-4.78123739741691,1.1851427085983,8.5174718613016));
#36812=CARTESIAN_POINT('Ctrl Pts',(-4.7811598514415,1.29999999998554,8.55180091310643));
#36813=CARTESIAN_POINT('Ctrl Pts',(-4.84469211502532,-1.29999999998857,
8.31899636837851));
#36814=CARTESIAN_POINT('Ctrl Pts',(-4.84069767541249,-1.18514270860033,
8.29849818618627));
#36815=CARTESIAN_POINT('Ctrl Pts',(-4.82727652100109,-1.06847604193363,
8.28477299775572));
#36816=CARTESIAN_POINT('Ctrl Pts',(-4.77449337242585,-0.794772683991192,
8.26871203728901));
#36817=CARTESIAN_POINT('Ctrl Pts',(-4.70397525490767,-0.636309800087463,
8.27725099678412));
#36818=CARTESIAN_POINT('Ctrl Pts',(-4.62952730006986,-0.319434907273276,
8.29320881981134));
#36819=CARTESIAN_POINT('Ctrl Pts',(-4.58311248005771,-0.158333333331408,
8.3092164002926));
#36820=CARTESIAN_POINT('Ctrl Pts',(-4.57560738480491,0.15833333333141,8.33981920313398));
#36821=CARTESIAN_POINT('Ctrl Pts',(-4.61431686521015,0.319434907273283,
8.3552276973425));
#36822=CARTESIAN_POINT('Ctrl Pts',(-4.67388536473402,0.636309800087471,
8.39994900403055));
#36823=CARTESIAN_POINT('Ctrl Pts',(-4.73683980643477,0.79477268399118,8.42514666196667));
#36824=CARTESIAN_POINT('Ctrl Pts',(-4.77738673633568,1.06847604193256,8.48602790384311));
#36825=CARTESIAN_POINT('Ctrl Pts',(-4.78575576767938,1.18514270859823,8.51647683565076));
#36826=CARTESIAN_POINT('Ctrl Pts',(-4.78494256682449,1.29999999998547,8.55102146553006));
#36827=CARTESIAN_POINT('Ctrl Pts',(-4.84620807955783,-1.29999999998855,
8.31850938759095));
#36828=CARTESIAN_POINT('Ctrl Pts',(-4.84250783269422,-1.18514270860032,
8.29790295896496));
#36829=CARTESIAN_POINT('Ctrl Pts',(-4.82930171446687,-1.06847604193362,
8.28410738306688));
#36830=CARTESIAN_POINT('Ctrl Pts',(-4.77683247499386,-0.794772683991185,
8.26797127525481));
#36831=CARTESIAN_POINT('Ctrl Pts',(-4.70625903418148,-0.636309800087458,
8.27658305038065));
#36832=CARTESIAN_POINT('Ctrl Pts',(-4.63181841837675,-0.319434907273273,
8.29261338980029));
#36833=CARTESIAN_POINT('Ctrl Pts',(-4.58530434898141,-0.158333333331406,
8.30871300401627));
#36834=CARTESIAN_POINT('Ctrl Pts',(-4.57779781922702,0.158333333331408,
8.33935530629564));
#36835=CARTESIAN_POINT('Ctrl Pts',(-4.61660402946877,0.31943490727328,8.35471974975148));
#36836=CARTESIAN_POINT('Ctrl Pts',(-4.67616447814182,0.636309800087465,
8.39943171718987));
#36837=CARTESIAN_POINT('Ctrl Pts',(-4.73917685456128,0.794772683991173,
8.4245876721559));
#36838=CARTESIAN_POINT('Ctrl Pts',(-4.77941016424681,1.06847604193255,8.48555436720518));
#36839=CARTESIAN_POINT('Ctrl Pts',(-4.78756391136092,1.18514270859822,8.51606813087895));
#36840=CARTESIAN_POINT('Ctrl Pts',(-4.78645589661729,1.29999999998546,8.55070543497829));
#36841=CARTESIAN_POINT('Ctrl Pts',(-4.8481026095768,-1.29999999998851,8.31790944516153));
#36842=CARTESIAN_POINT('Ctrl Pts',(-4.84476969930837,-1.18514270860029,
8.29717727121702));
#36843=CARTESIAN_POINT('Ctrl Pts',(-4.83183220576747,-1.06847604193359,
8.28329759320041));
#36844=CARTESIAN_POINT('Ctrl Pts',(-4.77975549880186,-0.79477268399116,
8.26706339679263));
#36845=CARTESIAN_POINT('Ctrl Pts',(-4.70911424471676,-0.636309800087438,
8.27573422660257));
#36846=CARTESIAN_POINT('Ctrl Pts',(-4.63468285954174,-0.319434907273264,
8.29185128022252));
#36847=CARTESIAN_POINT('Ctrl Pts',(-4.58804345446328,-0.158333333331401,
8.30809002830088));
#36848=CARTESIAN_POINT('Ctrl Pts',(-4.58053525050573,0.158333333331403,
8.33878219628126));
#36849=CARTESIAN_POINT('Ctrl Pts',(-4.61946329649243,0.31943490727327,8.35407725721605));
#36850=CARTESIAN_POINT('Ctrl Pts',(-4.67901482319528,0.636309800087446,
8.39876357767907));
#36851=CARTESIAN_POINT('Ctrl Pts',(-4.74210119862822,0.794772683991148,
8.42385020461042));
#36852=CARTESIAN_POINT('Ctrl Pts',(-4.78194200703895,1.06847604193252,8.4849296291328));
#36853=CARTESIAN_POINT('Ctrl Pts',(-4.7898259182097,1.18514270859818,8.51553301549614));
#36854=CARTESIAN_POINT('Ctrl Pts',(-4.78834813083761,1.29999999998542,8.55030076856277));
#36855=CARTESIAN_POINT('Ctrl Pts',(-4.84980725425054,-1.29999999998848,
8.31737761465617));
#36856=CARTESIAN_POINT('Ctrl Pts',(-4.84680454639138,-1.18514270860025,
8.2965412065861));
#36857=CARTESIAN_POINT('Ctrl Pts',(-4.83410864630962,-1.06847604193356,
8.28258937106431));
#36858=CARTESIAN_POINT('Ctrl Pts',(-4.78238536416429,-0.794772683991136,
8.26626257979442));
#36859=CARTESIAN_POINT('Ctrl Pts',(-4.71168437486339,-0.636309800087419,
8.2749562061174));
#36860=CARTESIAN_POINT('Ctrl Pts',(-4.63726141895635,-0.319434907273254,
8.29114666110038));
#36861=CARTESIAN_POINT('Ctrl Pts',(-4.59050809948508,-0.158333333331397,
8.30753196390599));
#36862=CARTESIAN_POINT('Ctrl Pts',(-4.58299851718329,0.158333333331399,
8.33826944875672));
#36863=CARTESIAN_POINT('Ctrl Pts',(-4.62203700163914,0.319434907273261,
8.35349010881316));
#36864=CARTESIAN_POINT('Ctrl Pts',(-4.68158156410424,0.636309800087427,
8.39814067012216));
#36865=CARTESIAN_POINT('Ctrl Pts',(-4.74473605054966,0.794772683991125,
8.42314821811786));
#36866=CARTESIAN_POINT('Ctrl Pts',(-4.78422322584727,1.06847604193248,8.48433441417299));
#36867=CARTESIAN_POINT('Ctrl Pts',(-4.79186363629283,1.18514270859815,8.51502642501498));
#36868=CARTESIAN_POINT('Ctrl Pts',(-4.79005192214164,1.29999999998538,8.54992520959865));
#36869=CARTESIAN_POINT('Ctrl Pts',(-4.85094353887164,-1.29999999998846,
8.3170253307956));
#36870=CARTESIAN_POINT('Ctrl Pts',(-4.8481608384203,-1.18514270860024,8.29612198038685));
#36871=CARTESIAN_POINT('Ctrl Pts',(-4.83562594699106,-1.06847604193355,
8.28212298961925));
#36872=CARTESIAN_POINT('Ctrl Pts',(-4.7841383281153,-0.79477268399113,8.26573297244118));
#36873=CARTESIAN_POINT('Ctrl Pts',(-4.71339791183896,-0.636309800087413,
8.27443280912155));
#36874=CARTESIAN_POINT('Ctrl Pts',(-4.63898064804253,-0.319434907273251,
8.29067036055618));
#36875=CARTESIAN_POINT('Ctrl Pts',(-4.59215110952092,-0.158333333331395,
8.30715890120654));
#36876=CARTESIAN_POINT('Ctrl Pts',(-4.58464065380343,0.158333333331397,
8.33792673389281));
#36877=CARTESIAN_POINT('Ctrl Pts',(-4.62375294779913,0.319434907273258,
8.35309509327714));
#36878=CARTESIAN_POINT('Ctrl Pts',(-4.68329316798326,0.636309800087421,
8.39771843549319));
#36879=CARTESIAN_POINT('Ctrl Pts',(-4.74649349899409,0.794772683991118,
8.42266833267474));
#36880=CARTESIAN_POINT('Ctrl Pts',(-4.78574485520293,1.06847604193248,8.48392703633881));
#36881=CARTESIAN_POINT('Ctrl Pts',(-4.79322277563256,1.18514270859814,8.5146802882616));
#36882=CARTESIAN_POINT('Ctrl Pts',(-4.79118815879509,1.29999999998537,8.54967016914964));
#36883=CARTESIAN_POINT('Ctrl Pts',(-4.85151165403496,-1.29999999998846,
8.31684956349615));
#36884=CARTESIAN_POINT('Ctrl Pts',(-4.84883893538057,-1.18514270860024,
8.29591313944484));
#36885=CARTESIAN_POINT('Ctrl Pts',(-4.83638453913278,-1.06847604193355,
8.28189070955156));
#36886=CARTESIAN_POINT('Ctrl Pts',(-4.78501476024864,-0.794772683991129,
8.26546880096556));
#36887=CARTESIAN_POINT('Ctrl Pts',(-4.71425469626629,-0.636309800087412,
8.27417029196364));
#36888=CARTESIAN_POINT('Ctrl Pts',(-4.6398402970313,-0.319434907273251,
8.29043100080685));
#36889=CARTESIAN_POINT('Ctrl Pts',(-4.59297261469187,-0.158333333331395,
8.30697189695609));
#36890=CARTESIAN_POINT('Ctrl Pts',(-4.58546173106472,0.158333333331397,
8.33775491528288));
#36891=CARTESIAN_POINT('Ctrl Pts',(-4.62461094888219,0.319434907273258,
8.35289685748205));
#36892=CARTESIAN_POINT('Ctrl Pts',(-4.68414904630666,0.63630980008742,8.39750607192482));
#36893=CARTESIAN_POINT('Ctrl Pts',(-4.74737237762247,0.794772683991117,
8.42242623561674));
#36894=CARTESIAN_POINT('Ctrl Pts',(-4.78650581916945,1.06847604193247,8.48372139404888));
#36895=CARTESIAN_POINT('Ctrl Pts',(-4.79390247131605,1.18514270859814,8.51450562532234));
#36896=CARTESIAN_POINT('Ctrl Pts',(-4.79175635880045,1.29999999998537,8.54954168499341));
#36897=CARTESIAN_POINT('Ctrl Pts',(-4.85198506445694,-1.29999999998846,
8.31670332061117));
#36898=CARTESIAN_POINT('Ctrl Pts',(-4.84940397997935,-1.18514270860023,
8.29573963809466));
#36899=CARTESIAN_POINT('Ctrl Pts',(-4.83701665562309,-1.06847604193354,
8.28169778118904));
#36900=CARTESIAN_POINT('Ctrl Pts',(-4.78574508243343,-0.794772683991124,
8.26524908454092));
#36901=CARTESIAN_POINT('Ctrl Pts',(-4.71496869699086,-0.636309800087409,
8.2739508205106));
#36902=CARTESIAN_POINT('Ctrl Pts',(-4.64055669627058,-0.319434907273249,
8.29023058588678));
#36903=CARTESIAN_POINT('Ctrl Pts',(-4.59365719512019,-0.158333333331394,
8.3068157981148));
#36904=CARTESIAN_POINT('Ctrl Pts',(-4.58614596134621,0.158333333331396,
8.33761149946187));
#36905=CARTESIAN_POINT('Ctrl Pts',(-4.62532597163485,0.319434907273256,
8.35273109638902));
#36906=CARTESIAN_POINT('Ctrl Pts',(-4.68486233467704,0.636309800087417,
8.39732817014555));
#36907=CARTESIAN_POINT('Ctrl Pts',(-4.74810487786108,0.794772683991113,
8.42222305832064));
#36908=CARTESIAN_POINT('Ctrl Pts',(-4.78714005540755,1.06847604193247,8.4835487297326));
#36909=CARTESIAN_POINT('Ctrl Pts',(-4.79446897067439,1.18514270859813,8.51435899761028));
#36910=CARTESIAN_POINT('Ctrl Pts',(-4.79222991924408,1.29999999998536,8.54943392255144));
#36911=CARTESIAN_POINT('Ctrl Pts',(-4.85231643937463,-1.29999999998846,
8.31660108815661));
#36912=CARTESIAN_POINT('Ctrl Pts',(-4.84979949165294,-1.18514270860024,
8.29561841335129));
#36913=CARTESIAN_POINT('Ctrl Pts',(-4.83745911474827,-1.06847604193354,
8.28156297720895));
#36914=CARTESIAN_POINT('Ctrl Pts',(-4.78625628883194,-0.794772683991127,
8.26509541504073));
#36915=CARTESIAN_POINT('Ctrl Pts',(-4.71546849695651,-0.636309800087411,
8.27379696214256));
#36916=CARTESIAN_POINT('Ctrl Pts',(-4.64105818945796,-0.31943490727325,
8.29008982354754));
#36917=CARTESIAN_POINT('Ctrl Pts',(-4.59413642176686,-0.158333333331395,
8.30670599098071));
#36918=CARTESIAN_POINT('Ctrl Pts',(-4.58662494660489,0.158333333331397,
8.33751055346706));
#36919=CARTESIAN_POINT('Ctrl Pts',(-4.62582649875683,0.319434907273257,
8.35261471713071));
#36920=CARTESIAN_POINT('Ctrl Pts',(-4.68536166131313,0.636309800087419,
8.39720317678635));
#36921=CARTESIAN_POINT('Ctrl Pts',(-4.74861769015291,0.794772683991115,
8.42207989545944));
#36922=CARTESIAN_POINT('Ctrl Pts',(-4.78758408758185,1.06847604193247,8.48342696453893));
#36923=CARTESIAN_POINT('Ctrl Pts',(-4.79486558149654,1.18514270859813,8.51425558722074));
#36924=CARTESIAN_POINT('Ctrl Pts',(-4.79256145972622,1.29999999998536,8.54935795951273));
#36925=CARTESIAN_POINT('Ctrl Pts',(-4.85250579798908,-1.29999999998845,
8.31654263126025));
#36926=CARTESIAN_POINT('Ctrl Pts',(-4.85002549762174,-1.18514270860023,
8.29554916044781));
#36927=CARTESIAN_POINT('Ctrl Pts',(-4.83771194672594,-1.06847604193354,
8.28148599004196));
#36928=CARTESIAN_POINT('Ctrl Pts',(-4.7865484049838,-0.794772683991122,
8.265007633418));
#36929=CARTESIAN_POINT('Ctrl Pts',(-4.71575410397166,-0.636309800087407,
8.27370884675981));
#36930=CARTESIAN_POINT('Ctrl Pts',(-4.64134475800369,-0.319434907273248,
8.29000928574408));
#36931=CARTESIAN_POINT('Ctrl Pts',(-4.59441024648493,-0.158333333331394,
8.30664352448534));
#36932=CARTESIAN_POINT('Ctrl Pts',(-4.58689863389259,0.158333333331396,
8.33745318337796));
#36933=CARTESIAN_POINT('Ctrl Pts',(-4.62611251846933,0.319434907273255,
8.35254818476237));
#36934=CARTESIAN_POINT('Ctrl Pts',(-4.6856469976215,0.636309800087415,8.39713168181365));
#36935=CARTESIAN_POINT('Ctrl Pts',(-4.74891071436139,0.79477268399111,8.42199827809077));
#36936=CARTESIAN_POINT('Ctrl Pts',(-4.78783780671656,1.06847604193247,8.48335758804548));
#36937=CARTESIAN_POINT('Ctrl Pts',(-4.79509220458799,1.18514270859813,8.51419666155191));
#36938=CARTESIAN_POINT('Ctrl Pts',(-4.7927509044412,1.29999999998536,8.54931463687183));
#36939=CARTESIAN_POINT('Ctrl Pts',(-4.86471868730759,-1.29999999998952,
8.31278254654165));
#36940=CARTESIAN_POINT('Ctrl Pts',(-4.86460208837969,-1.1851427086012,8.29108942207398));
#36941=CARTESIAN_POINT('Ctrl Pts',(-4.85401881867296,-1.06847604193441,
8.27652499052704));
#36942=CARTESIAN_POINT('Ctrl Pts',(-4.80538924512544,-0.794772683991774,
8.25934694678619));
#36943=CARTESIAN_POINT('Ctrl Pts',(-4.7341748410259,-0.636309800087929,
8.2680389006263));
#36944=CARTESIAN_POINT('Ctrl Pts',(-4.65982891346145,-0.319434907273511,
8.28480552536));
#36945=CARTESIAN_POINT('Ctrl Pts',(-4.61207524473024,-0.158333333331524,
8.3025546175784));
#36946=CARTESIAN_POINT('Ctrl Pts',(-4.60455487191363,0.158333333331526,
8.33368824322348));
#36947=CARTESIAN_POINT('Ctrl Pts',(-4.64456077521837,0.319434907273517,
8.34824442195183));
#36948=CARTESIAN_POINT('Ctrl Pts',(-4.70405142721366,0.636309800087937,
8.39250819384349));
#36949=CARTESIAN_POINT('Ctrl Pts',(-4.76781486087401,0.794772683991763,
8.41666929233755));
#36950=CARTESIAN_POINT('Ctrl Pts',(-4.80420730546169,1.06847604193334,8.47881786275056));
#36951=CARTESIAN_POINT('Ctrl Pts',(-4.80971358233116,1.1851427085991,8.51034101279893));
#36952=CARTESIAN_POINT('Ctrl Pts',(-4.80497319528103,1.29999999998642,8.5464854995953));
#36953=CARTESIAN_POINT('Ctrl Pts',(-4.88296319426862,-1.29999999999803,
8.30623816835216));
#36954=CARTESIAN_POINT('Ctrl Pts',(-4.88638185991351,-1.18514270860896,
8.28290786847773));
#36955=CARTESIAN_POINT('Ctrl Pts',(-4.87838251735454,-1.06847604194141,
8.26729920094536));
#36956=CARTESIAN_POINT('Ctrl Pts',(-4.83352455266495,-0.794772683996978,
8.24907857185986));
#36957=CARTESIAN_POINT('Ctrl Pts',(-4.76163519605766,-0.636309800092096,
8.2591829394193));
#36958=CARTESIAN_POINT('Ctrl Pts',(-4.68739480387011,-0.319434907275602,
8.27685037539968));
#36959=CARTESIAN_POINT('Ctrl Pts',(-4.63849073644685,-0.158333333332561,
8.29527453260398));
#36960=CARTESIAN_POINT('Ctrl Pts',(-4.63095498045046,0.158333333332563,
8.32700558912046));
#36961=CARTESIAN_POINT('Ctrl Pts',(-4.67210354006842,0.319434907275611,
8.34128797459167));
#36962=CARTESIAN_POINT('Ctrl Pts',(-4.73144175849589,0.636309800092106,
8.3862674209549));
#36963=CARTESIAN_POINT('Ctrl Pts',(-4.79576457762992,0.794772683996967,
8.41158971382161));
#36964=CARTESIAN_POINT('Ctrl Pts',(-4.82846153604461,1.06847604194034,8.47426058233221));
#36965=CARTESIAN_POINT('Ctrl Pts',(-4.83146067933456,1.18514270860686,8.50582862891778));
#36966=CARTESIAN_POINT('Ctrl Pts',(-4.82330566415844,1.29999999999493,8.54183682529518));
#36967=CARTESIAN_POINT('Ctrl Pts',(-4.90715283621587,-1.3,8.29842404846038));
#36968=CARTESIAN_POINT('Ctrl Pts',(-4.9152638301882,-1.18514270861076,8.27298278446696));
#36969=CARTESIAN_POINT('Ctrl Pts',(-4.91069673261394,-1.06847604194303,
8.25599416747618));
#36970=CARTESIAN_POINT('Ctrl Pts',(-4.87085689585679,-0.794772683998181,
8.23627436918876));
#36971=CARTESIAN_POINT('Ctrl Pts',(-4.79810158493444,-0.636309800093057,
8.24784641680822));
#36972=CARTESIAN_POINT('Ctrl Pts',(-4.7239959857142,-0.319434907276084,
8.26668557716251));
#36973=CARTESIAN_POINT('Ctrl Pts',(-4.67351228603286,-0.1583333333328,8.28656988747768));
#36974=CARTESIAN_POINT('Ctrl Pts',(-4.66597277435144,0.158333333332802,
8.31875211991404));
#36975=CARTESIAN_POINT('Ctrl Pts',(-4.70866985933996,0.319434907276095,
8.33222208436452));
#36976=CARTESIAN_POINT('Ctrl Pts',(-4.76792134717021,0.636309800093068,
8.37654844845054));
#36977=CARTESIAN_POINT('Ctrl Pts',(-4.83327179504176,0.794772683998166,
8.39999714139346));
#36978=CARTESIAN_POINT('Ctrl Pts',(-4.86090739952758,1.06847604194195,8.46469604840318));
#36979=CARTESIAN_POINT('Ctrl Pts',(-4.86040992141996,1.18514270860865,8.49801701093837));
#36980=CARTESIAN_POINT('Ctrl Pts',(-4.84745253602286,1.2999999999969,8.53665317649499));
#36981=CARTESIAN_POINT('Ctrl Pts',(-4.91927797405485,-1.30000000000437,
8.29377458052673));
#36982=CARTESIAN_POINT('Ctrl Pts',(-4.92971468412874,-1.18514270861474,
8.26751665921141));
#36983=CARTESIAN_POINT('Ctrl Pts',(-4.92685055912788,-1.06847604194662,
8.24995659760688));
#36984=CARTESIAN_POINT('Ctrl Pts',(-4.8895062675643,-0.794772684000851,
8.22948313835506));
#36985=CARTESIAN_POINT('Ctrl Pts',(-4.81632945957884,-0.636309800095197,
8.24128634225486));
#36986=CARTESIAN_POINT('Ctrl Pts',(-4.74231241411425,-0.319434907277159,
8.26047280583125));
#36987=CARTESIAN_POINT('Ctrl Pts',(-4.69108112428619,-0.158333333333332,
8.28090406141698));
#36988=CARTESIAN_POINT('Ctrl Pts',(-4.683529805314,0.158333333333334,8.31369722637576));
#36989=CARTESIAN_POINT('Ctrl Pts',(-4.72695029650717,0.319434907277167,
8.32750102064963));
#36990=CARTESIAN_POINT('Ctrl Pts',(-4.78611439032821,0.636309800095206,
8.37217485718424));
#36991=CARTESIAN_POINT('Ctrl Pts',(-4.85190733217758,0.79477268400084,8.3954008624989));
#36992=CARTESIAN_POINT('Ctrl Pts',(-4.87708284447686,1.06847604194555,8.46055100386331));
#36993=CARTESIAN_POINT('Ctrl Pts',(-4.87490135690222,1.18514270861264,8.49417556843746));
#36994=CARTESIAN_POINT('Ctrl Pts',(-4.85964083532324,1.30000000000127,8.53322361543972));
#36995=CARTESIAN_POINT('Ctrl Pts',(-4.92533609403178,-1.30000000000437,
8.29148735027311));
#36996=CARTESIAN_POINT('Ctrl Pts',(-4.93693489080363,-1.18514270861474,
8.26482422250723));
#36997=CARTESIAN_POINT('Ctrl Pts',(-4.93492178515129,-1.06847604194662,
8.24698002939983));
#36998=CARTESIAN_POINT('Ctrl Pts',(-4.89882489072262,-0.794772684000851,
8.22612987688622));
#36999=CARTESIAN_POINT('Ctrl Pts',(-4.82544129359841,-0.636309800095197,
8.23799733825931));
#37000=CARTESIAN_POINT('Ctrl Pts',(-4.75146299020767,-0.319434907277159,
8.25744308061905));
#37001=CARTESIAN_POINT('Ctrl Pts',(-4.69984189087486,-0.158333333333332,
8.27839589375356));
#37002=CARTESIAN_POINT('Ctrl Pts',(-4.69228837762174,0.158333333333334,
8.31142398215957));
#37003=CARTESIAN_POINT('Ctrl Pts',(-4.73609341170092,0.319434907277167,
8.32501575423084));
#37004=CARTESIAN_POINT('Ctrl Pts',(-4.79522055198673,0.636309800095206,
8.36975685506309));
#37005=CARTESIAN_POINT('Ctrl Pts',(-4.86122784986915,0.79477268400084,8.39303182191491));
#37006=CARTESIAN_POINT('Ctrl Pts',(-4.88516330785013,1.06847604194555,8.4585208729234));
#37007=CARTESIAN_POINT('Ctrl Pts',(-4.88213395050331,1.18514270861264,8.49235062833803));
#37008=CARTESIAN_POINT('Ctrl Pts',(-4.86571446294582,1.30000000000127,8.53166235559416));
#37009=CARTESIAN_POINT('',(-4.76940701573779,1.2,8.5248610184586));
#37010=CARTESIAN_POINT('Ctrl Pts',(-4.76940701573779,1.2,8.5248610184586));
#37011=CARTESIAN_POINT('Ctrl Pts',(-4.74959775132473,1.21680199780992,8.53339667265294));
#37012=CARTESIAN_POINT('Ctrl Pts',(-4.72988508062029,1.23316175714919,8.54300746795801));
#37013=CARTESIAN_POINT('Ctrl Pts',(-4.70624255731438,1.25313382902886,8.552991453738));
#37014=CARTESIAN_POINT('Ctrl Pts',(-4.68241322188002,1.2731048455244,8.56362856372702));
#37015=CARTESIAN_POINT('Ctrl Pts',(-4.6525154957812,1.29841093120771,8.57550588696848));
#37016=CARTESIAN_POINT('Ctrl Pts',(-4.6515830528172,1.29920026509202,8.57587556280998));
#37017=CARTESIAN_POINT('Ctrl Pts',(-4.65063820841642,1.29999999999331,8.5762500697483));
#37018=CARTESIAN_POINT('',(-4.80892752946133,0.653834841327865,8.37333542346878));
#37019=CARTESIAN_POINT('Ctrl Pts',(-4.80892752948835,0.653834841312438,
8.37333542353798));
#37020=CARTESIAN_POINT('Ctrl Pts',(-4.80542009361191,0.712175033180002,
8.3877106862342));
#37021=CARTESIAN_POINT('Ctrl Pts',(-4.80171376700822,0.767439432116428,
8.40262161143459));
#37022=CARTESIAN_POINT('Ctrl Pts',(-4.79380687348683,0.881523157784702,
8.43376581863121));
#37023=CARTESIAN_POINT('Ctrl Pts',(-4.78991228436266,0.939238214520343,
8.44883908268581));
#37024=CARTESIAN_POINT('Ctrl Pts',(-4.78300534853591,1.03041410836302,8.47492136578765));
#37025=CARTESIAN_POINT('Ctrl Pts',(-4.7816957916988,1.04693620269592,8.47990356864517));
#37026=CARTESIAN_POINT('Ctrl Pts',(-4.77434691931254,1.13963387115676,8.50699986195079));
#37027=CARTESIAN_POINT('Ctrl Pts',(-4.77208504469432,1.16791763773685,8.51522030149607));
#37028=CARTESIAN_POINT('Ctrl Pts',(-4.76940701573779,1.2,8.5248610184586));
#37029=CARTESIAN_POINT('',(-4.84008270153025,-0.653834841531101,8.23735213035285));
#37030=CARTESIAN_POINT('Ctrl Pts',(-4.84008270153025,-0.653834841531099,
8.23735213035285));
#37031=CARTESIAN_POINT('Ctrl Pts',(-4.79943687647267,-0.575774454259114,
8.24659452518038));
#37032=CARTESIAN_POINT('Ctrl Pts',(-4.76540108947681,-0.493710702847288,
8.25532385189694));
#37033=CARTESIAN_POINT('Ctrl Pts',(-4.71692660388303,-0.338121740996384,
8.27001974097562));
#37034=CARTESIAN_POINT('Ctrl Pts',(-4.70018760001661,-0.265673667041442,
8.27641839251951));
#37035=CARTESIAN_POINT('Ctrl Pts',(-4.67924730487146,-0.129742825061959,
8.28899804955198));
#37036=CARTESIAN_POINT('Ctrl Pts',(-4.67358921948777,-0.066665686974624,
8.29501142948854));
#37037=CARTESIAN_POINT('Ctrl Pts',(-4.67025713110064,0.0595066342539753,
8.30787286844477));
#37038=CARTESIAN_POINT('Ctrl Pts',(-4.67254530496467,0.122729721736906,
8.31479683851603));
#37039=CARTESIAN_POINT('Ctrl Pts',(-4.68651536486654,0.260113581388072,
8.32999321016995));
#37040=CARTESIAN_POINT('Ctrl Pts',(-4.69982530968251,0.333986144077667,
8.33833894741233));
#37041=CARTESIAN_POINT('Ctrl Pts',(-4.74125637880943,0.491528819855043,
8.35566552490392));
#37042=CARTESIAN_POINT('Ctrl Pts',(-4.771640731347,0.574924749423742,8.364924270098));
#37043=CARTESIAN_POINT('Ctrl Pts',(-4.80892752938989,0.65383484135055,8.37333542357261));
#37044=CARTESIAN_POINT('',(-4.82442585316259,-1.2,8.3078877142276));
#37045=CARTESIAN_POINT('Ctrl Pts',(-4.82442585316259,-1.2,8.3078877142276));
#37046=CARTESIAN_POINT('Ctrl Pts',(-4.82689451181185,-1.14179354867607,
8.29713765313641));
#37047=CARTESIAN_POINT('Ctrl Pts',(-4.8307416685721,-1.0415419554568,8.28018439951763));
#37048=CARTESIAN_POINT('Ctrl Pts',(-4.83823646441324,-0.774556440178833,
8.24604982293182));
#37049=CARTESIAN_POINT('Ctrl Pts',(-4.83902226279081,-0.721499503691961,
8.24229993066929));
#37050=CARTESIAN_POINT('Ctrl Pts',(-4.84008270153025,-0.653834841531101,
8.23735213035285));
#37051=CARTESIAN_POINT('Ctrl Pts',(-4.70981757142094,-1.29999999999641,
8.35763484915121));
#37052=CARTESIAN_POINT('Ctrl Pts',(-4.71097463231061,-1.29899465260559,
8.35713934673585));
#37053=CARTESIAN_POINT('Ctrl Pts',(-4.71213258962288,-1.29798697378795,
8.35664921501205));
#37054=CARTESIAN_POINT('Ctrl Pts',(-4.73158341462519,-1.28099071752189,
8.34869701228178));
#37055=CARTESIAN_POINT('Ctrl Pts',(-4.74981785750062,-1.26509988311611,
8.34088437013692));
#37056=CARTESIAN_POINT('Ctrl Pts',(-4.77997485499785,-1.23871758437594,
8.3280932555352));
#37057=CARTESIAN_POINT('Ctrl Pts',(-4.80250841816378,-1.21895688910026,
8.31863107643311));
#37058=CARTESIAN_POINT('Ctrl Pts',(-4.82442585316259,-1.2,8.3078877142276));
#37059=CARTESIAN_POINT('Origin',(0.,1.25,7.2));
#37060=CARTESIAN_POINT('Origin',(0.,1.2,7.2));
#37061=CARTESIAN_POINT('Origin',(0.,0.92691742076555,7.2));
#37062=CARTESIAN_POINT('Origin',(0.,0.653834841531101,7.2));
#37063=CARTESIAN_POINT('Origin',(0.,0.,7.2));
#37064=CARTESIAN_POINT('Origin',(0.,-0.653834841531101,7.2));
#37065=CARTESIAN_POINT('Origin',(0.,-0.926917420765551,7.2));
#37066=CARTESIAN_POINT('Origin',(0.,-1.2,7.2));
#37067=CARTESIAN_POINT('Origin',(0.,-1.25,7.2));
#37068=CARTESIAN_POINT('Ctrl Pts',(-4.98668722203916,-1.30000000000015,
7.96253027075762));
#37069=CARTESIAN_POINT('Ctrl Pts',(-4.98569765033805,-1.18514270861188,
8.00512172787461));
#37070=CARTESIAN_POINT('Ctrl Pts',(-4.97470530482919,-1.06847604194517,
8.03725889790462));
#37071=CARTESIAN_POINT('Ctrl Pts',(-4.92620237914858,-0.794772684000851,
8.08735069514887));
#37072=CARTESIAN_POINT('Ctrl Pts',(-4.85643493010791,-0.636309800095197,
8.08176584863345));
#37073=CARTESIAN_POINT('Ctrl Pts',(-4.78422175451511,-0.319434907277159,
8.09858970351398));
#37074=CARTESIAN_POINT('Ctrl Pts',(-4.73867559286569,-0.158333333333332,
8.09318929263998));
#37075=CARTESIAN_POINT('Ctrl Pts',(-4.73214233678195,0.158333333333335,
8.1264342434019));
#37076=CARTESIAN_POINT('Ctrl Pts',(-4.77077828071914,0.319434907277167,
8.1665717833203));
#37077=CARTESIAN_POINT('Ctrl Pts',(-4.83045152777451,0.636309800095207,
8.21442603970484));
#37078=CARTESIAN_POINT('Ctrl Pts',(-4.89266384818737,0.794772684000841,
8.25511530308637));
#37079=CARTESIAN_POINT('Ctrl Pts',(-4.93412052316908,1.06847604194528,8.25074967063201));
#37080=CARTESIAN_POINT('Ctrl Pts',(-4.9432174738979,1.18514270861211,8.23526699290927));
#37081=CARTESIAN_POINT('Ctrl Pts',(-4.94346631687715,1.30000000000049,8.20619135799067));
#37082=CARTESIAN_POINT('Ctrl Pts',(-4.97686019541383,-1.30000000000015,
7.95473697326264));
#37083=CARTESIAN_POINT('Ctrl Pts',(-4.97396758436907,-1.18514270861188,
7.99590387472333));
#37084=CARTESIAN_POINT('Ctrl Pts',(-4.9615930209824,-1.06847604194517,8.02697642302472));
#37085=CARTESIAN_POINT('Ctrl Pts',(-4.9111000972684,-0.794772684000851,
8.07544025047651));
#37086=CARTESIAN_POINT('Ctrl Pts',(-4.84176412504578,-0.636309800095197,
8.06994031968232));
#37087=CARTESIAN_POINT('Ctrl Pts',(-4.76953814967826,-0.319434907277159,
8.08661121585988));
#37088=CARTESIAN_POINT('Ctrl Pts',(-4.72452210845454,-0.158333333333332,
8.08191100419208));
#37089=CARTESIAN_POINT('Ctrl Pts',(-4.71817594716844,0.158333333333335,
8.11472494346892));
#37090=CARTESIAN_POINT('Ctrl Pts',(-4.75652394684048,0.319434907277167,
8.15359245071089));
#37091=CARTESIAN_POINT('Ctrl Pts',(-4.81647889553182,0.636309800095207,
8.2010044968254));
#37092=CARTESIAN_POINT('Ctrl Pts',(-4.87836566507891,0.794772684000841,
8.2414081385139));
#37093=CARTESIAN_POINT('Ctrl Pts',(-4.92179501812863,1.06847604194528,8.23874548314256));
#37094=CARTESIAN_POINT('Ctrl Pts',(-4.93221572520194,1.18514270861211,8.22447422101514));
#37095=CARTESIAN_POINT('Ctrl Pts',(-4.93425818162945,1.30000000000049,8.19708426160946));
#37096=CARTESIAN_POINT('Ctrl Pts',(-4.95707257542365,-1.3000000000004,7.93971797339418));
#37097=CARTESIAN_POINT('Ctrl Pts',(-4.95090720637166,-1.18514270861211,
7.9764403553286));
#37098=CARTESIAN_POINT('Ctrl Pts',(-4.93606540805145,-1.06847604194537,
8.00447473012978));
#37099=CARTESIAN_POINT('Ctrl Pts',(-4.88173359751691,-0.794772684001005,
8.04916870967032));
#37100=CARTESIAN_POINT('Ctrl Pts',(-4.81233385660756,-0.636309800095321,
8.04643608415275));
#37101=CARTESIAN_POINT('Ctrl Pts',(-4.73982846661425,-0.319434907277221,
8.06349820095983));
#37102=CARTESIAN_POINT('Ctrl Pts',(-4.69623080845726,-0.158333333333363,
8.05926321453546));
#37103=CARTESIAN_POINT('Ctrl Pts',(-4.69013837127611,0.158333333333365,
8.09148533256226));
#37104=CARTESIAN_POINT('Ctrl Pts',(-4.72746932272836,0.319434907277228,
8.12886904361067));
#37105=CARTESIAN_POINT('Ctrl Pts',(-4.78791983132539,0.636309800095329,
8.17555363023394));
#37106=CARTESIAN_POINT('Ctrl Pts',(-4.84954939611665,0.794772684000997,
8.21441230389292));
#37107=CARTESIAN_POINT('Ctrl Pts',(-4.89693206221802,1.06847604194549,8.21518779027577));
#37108=CARTESIAN_POINT('Ctrl Pts',(-4.9099356983377,1.18514270861234,8.20353394339688));
#37109=CARTESIAN_POINT('Ctrl Pts',(-4.91543277012257,1.30000000000074,8.17989057031857));
#37110=CARTESIAN_POINT('Ctrl Pts',(-4.93706273410424,-1.30000000000065,
7.92437433149745));
#37111=CARTESIAN_POINT('Ctrl Pts',(-4.92672246011735,-1.18514270861234,
7.9591527062714));
#37112=CARTESIAN_POINT('Ctrl Pts',(-4.9088900170747,-1.06847604194558,7.98559559832303));
#37113=CARTESIAN_POINT('Ctrl Pts',(-4.85038509695605,-0.79477268400116,
8.0274273362486));
#37114=CARTESIAN_POINT('Ctrl Pts',(-4.78229038223289,-0.636309800095441,
8.02363556847094));
#37115=CARTESIAN_POINT('Ctrl Pts',(-4.70990346987882,-0.319434907277281,
8.03996699510912));
#37116=CARTESIAN_POINT('Ctrl Pts',(-4.66738796843898,-0.158333333333393,
8.03713816760568));
#37117=CARTESIAN_POINT('Ctrl Pts',(-4.66156310125004,0.158333333333395,
8.06871883459887));
#37118=CARTESIAN_POINT('Ctrl Pts',(-4.69796211219866,0.31943490727729,8.10434728984312));
#37119=CARTESIAN_POINT('Ctrl Pts',(-4.7590782051624,0.636309800095451,8.14986047271179));
#37120=CARTESIAN_POINT('Ctrl Pts',(-4.82064942303686,0.794772684001145,
8.18663205747421));
#37121=CARTESIAN_POINT('Ctrl Pts',(-4.87208201945832,1.06847604194569,8.19073989913263));
#37122=CARTESIAN_POINT('Ctrl Pts',(-4.88767626585109,1.18514270861257,8.18178352934301));
#37123=CARTESIAN_POINT('Ctrl Pts',(-4.89660149341129,1.30000000000099,8.16209265732034));
#37124=CARTESIAN_POINT('Ctrl Pts',(-4.92681556703292,-1.30000000000068,
7.91663963991158));
#37125=CARTESIAN_POINT('Ctrl Pts',(-4.91465480283025,-1.18514270861237,
7.94947552149818));
#37126=CARTESIAN_POINT('Ctrl Pts',(-4.89546982950633,-1.06847604194561,
7.97456102308863));
#37127=CARTESIAN_POINT('Ctrl Pts',(-4.83492137492904,-0.794772684001177,
8.01460862185063));
#37128=CARTESIAN_POINT('Ctrl Pts',(-4.76700538266001,-0.636309800095456,
8.01166877733264));
#37129=CARTESIAN_POINT('Ctrl Pts',(-4.69444812518406,-0.319434907277288,
8.02827046106348));
#37130=CARTESIAN_POINT('Ctrl Pts',(-4.65245112947184,-0.158333333333397,
8.02626803251437));
#37131=CARTESIAN_POINT('Ctrl Pts',(-4.64675546908366,0.158333333333399,
8.05753591142075));
#37132=CARTESIAN_POINT('Ctrl Pts',(-4.68285379896454,0.319434907277297,
8.09178027156682));
#37133=CARTESIAN_POINT('Ctrl Pts',(-4.74422291380177,0.636309800095465,
8.13688493060965));
#37134=CARTESIAN_POINT('Ctrl Pts',(-4.80539436748246,0.794772684001164,
8.17349735392384));
#37135=CARTESIAN_POINT('Ctrl Pts',(-4.85890464595191,1.06847604194571,8.17931255377106));
#37136=CARTESIAN_POINT('Ctrl Pts',(-4.87590847415212,1.18514270861259,8.17154257504764));
#37137=CARTESIAN_POINT('Ctrl Pts',(-4.88675351375432,1.30000000000102,8.15348543306134));
#37138=CARTESIAN_POINT('Ctrl Pts',(-4.92634883800722,-1.30000000000068,
7.91629093381771));
#37139=CARTESIAN_POINT('Ctrl Pts',(-4.91410516658122,-1.18514270861237,
7.94903877767638));
#37140=CARTESIAN_POINT('Ctrl Pts',(-4.89485865912818,-1.0684760419456,7.9740626005799));
#37141=CARTESIAN_POINT('Ctrl Pts',(-4.83421742452598,-0.794772684001177,
8.01402860389416));
#37142=CARTESIAN_POINT('Ctrl Pts',(-4.7663102877219,-0.636309800095456,
8.01112550257999));
#37143=CARTESIAN_POINT('Ctrl Pts',(-4.69374512410901,-0.319434907277288,
8.02773985836219));
#37144=CARTESIAN_POINT('Ctrl Pts',(-4.6517706931809,-0.158333333333396,
8.02577773664887));
#37145=CARTESIAN_POINT('Ctrl Pts',(-4.6460808087952,0.158333333333399,8.05703161637855));
#37146=CARTESIAN_POINT('Ctrl Pts',(-4.68216609320299,0.319434907277297,
8.09121128549913));
#37147=CARTESIAN_POINT('Ctrl Pts',(-4.74354725462836,0.636309800095465,
8.1362959106994));
#37148=CARTESIAN_POINT('Ctrl Pts',(-4.80470095934226,0.794772684001163,
8.1729000489884));
#37149=CARTESIAN_POINT('Ctrl Pts',(-4.85830584169813,1.06847604194571,8.17879251565979));
#37150=CARTESIAN_POINT('Ctrl Pts',(-4.87537371287317,1.18514270861259,8.17107659024682));
#37151=CARTESIAN_POINT('Ctrl Pts',(-4.88630588790803,1.30000000000102,8.15309410893623));
#37152=CARTESIAN_POINT('Ctrl Pts',(-4.92588209917281,-1.30000000000068,
7.91594220576637));
#37153=CARTESIAN_POINT('Ctrl Pts',(-4.91355533436984,-1.18514270861237,
7.94860259453505));
#37154=CARTESIAN_POINT('Ctrl Pts',(-4.89424716922786,-1.0684760419456,7.97356512423356));
#37155=CARTESIAN_POINT('Ctrl Pts',(-4.83351301375721,-0.794772684001177,
8.01344996717057));
#37156=CARTESIAN_POINT('Ctrl Pts',(-4.76561475713913,-0.636309800095456,
8.0105834766292));
#37157=CARTESIAN_POINT('Ctrl Pts',(-4.69304195822735,-0.319434907277288,
8.02720973951435));
#37158=CARTESIAN_POINT('Ctrl Pts',(-4.65109065207363,-0.158333333333397,
8.02528638895818));
#37159=CARTESIAN_POINT('Ctrl Pts',(-4.64540657107658,0.158333333333399,
8.05652617740995));
#37160=CARTESIAN_POINT('Ctrl Pts',(-4.68147820223513,0.319434907277297,
8.09064279235515));
#37161=CARTESIAN_POINT('Ctrl Pts',(-4.74287134831426,0.636309800095465,
8.13570756737513));
#37162=CARTESIAN_POINT('Ctrl Pts',(-4.80400777628441,0.794772684001164,
8.17230219840906));
#37163=CARTESIAN_POINT('Ctrl Pts',(-4.85770732971282,1.06847604194571,8.17827174263832));
#37164=CARTESIAN_POINT('Ctrl Pts',(-4.87483920216915,1.18514270861259,8.17060996610002));
#37165=CARTESIAN_POINT('Ctrl Pts',(-4.8858584001672,1.30000000000102,8.15270241851999));
#37166=CARTESIAN_POINT('Ctrl Pts',(-4.92494779478317,-1.30000000000068,
7.91524717629567));
#37167=CARTESIAN_POINT('Ctrl Pts',(-4.91245445453818,-1.18514270861237,
7.94773366183714));
#37168=CARTESIAN_POINT('Ctrl Pts',(-4.89302276215951,-1.0684760419456,7.97257413225111));
#37169=CARTESIAN_POINT('Ctrl Pts',(-4.83210268402666,-0.794772684001177,
8.01229676370186));
#37170=CARTESIAN_POINT('Ctrl Pts',(-4.76422290354184,-0.636309800095456,
8.00950146958473));
#37171=CARTESIAN_POINT('Ctrl Pts',(-4.69163503655158,-0.319434907277288,
8.02615091416697));
#37172=CARTESIAN_POINT('Ctrl Pts',(-4.64972978259324,-0.158333333333396,
8.02430564665363));
#37173=CARTESIAN_POINT('Ctrl Pts',(-4.6440572383016,0.158333333333399,8.05551738278739));
#37174=CARTESIAN_POINT('Ctrl Pts',(-4.68010131535152,0.319434907277297,
8.08950845780255));
#37175=CARTESIAN_POINT('Ctrl Pts',(-4.74151884911486,0.636309800095465,
8.13453243628381));
#37176=CARTESIAN_POINT('Ctrl Pts',(-4.80262176161668,0.794772684001163,
8.17110541371026));
#37177=CARTESIAN_POINT('Ctrl Pts',(-4.8565108926544,1.06847604194571,8.17722855690648));
#37178=CARTESIAN_POINT('Ctrl Pts',(-4.87377067854012,1.18514270861259,8.16967533570393));
#37179=CARTESIAN_POINT('Ctrl Pts',(-4.88496364227441,1.30000000000102,8.15191841149398));
#37180=CARTESIAN_POINT('Ctrl Pts',(-4.9229201203918,-1.30000000000068,7.91375075345988));
#37181=CARTESIAN_POINT('Ctrl Pts',(-4.91006283010197,-1.18514270861237,
7.94586907183033));
#37182=CARTESIAN_POINT('Ctrl Pts',(-4.89036171580574,-1.0684760419456,7.97045009443501));
#37183=CARTESIAN_POINT('Ctrl Pts',(-4.82903759802996,-0.794772684001176,
8.00982451301876));
#37184=CARTESIAN_POINT('Ctrl Pts',(-4.76120153532038,-0.636309800095455,
8.00717269005564));
#37185=CARTESIAN_POINT('Ctrl Pts',(-4.68858380635237,-0.319434907277288,
8.02386427242913));
#37186=CARTESIAN_POINT('Ctrl Pts',(-4.64678096711319,-0.158333333333396,
8.02218093374858));
#37187=CARTESIAN_POINT('Ctrl Pts',(-4.64113331134503,0.158333333333399,
8.05333183005413));
#37188=CARTESIAN_POINT('Ctrl Pts',(-4.67711279962206,0.319434907277297,
8.08706365877751));
#37189=CARTESIAN_POINT('Ctrl Pts',(-4.73858453889471,0.636309800095464,
8.13199587542556));
#37190=CARTESIAN_POINT('Ctrl Pts',(-4.79962230512729,0.794772684001163,
8.16850293988758));
#37191=CARTESIAN_POINT('Ctrl Pts',(-4.85392337802701,1.06847604194571,8.17495592741023));
#37192=CARTESIAN_POINT('Ctrl Pts',(-4.8714595015132,1.18514270861259,8.16764000235142));
#37193=CARTESIAN_POINT('Ctrl Pts',(-4.88302682608031,1.30000000000102,8.150214893042));
#37194=CARTESIAN_POINT('Ctrl Pts',(-4.91853551063343,-1.30000000000067,
7.91057496125883));
#37195=CARTESIAN_POINT('Ctrl Pts',(-4.90487437231569,-1.18514270861236,
7.94195741056749));
#37196=CARTESIAN_POINT('Ctrl Pts',(-4.88458126831889,-1.0684760419456,7.96601291574697));
#37197=CARTESIAN_POINT('Ctrl Pts',(-4.82237897102587,-0.794772684001172,
8.00465923831033));
#37198=CARTESIAN_POINT('Ctrl Pts',(-4.75466130079436,-0.636309800095453,
8.0022453434556));
#37199=CARTESIAN_POINT('Ctrl Pts',(-4.68199751600308,-0.319434907277287,
8.01897522261329));
#37200=CARTESIAN_POINT('Ctrl Pts',(-4.64043299418673,-0.158333333333396,
8.01759269083693));
#37201=CARTESIAN_POINT('Ctrl Pts',(-4.63483723281784,0.158333333333398,
8.04861522386223));
#37202=CARTESIAN_POINT('Ctrl Pts',(-4.67064341031251,0.319434907277295,
8.08187764026623));
#37203=CARTESIAN_POINT('Ctrl Pts',(-4.73224020187204,0.636309800095462,
8.12659206370196));
#37204=CARTESIAN_POINT('Ctrl Pts',(-4.79318824006026,0.794772684001161,
8.16282900060846));
#37205=CARTESIAN_POINT('Ctrl Pts',(-4.84838418783909,1.06847604194571,8.16997350796069));
#37206=CARTESIAN_POINT('Ctrl Pts',(-4.86650983018688,1.18514270861259,8.16318320752625));
#37207=CARTESIAN_POINT('Ctrl Pts',(-4.87886883430042,1.30000000000101,8.14651001415467));
#37208=CARTESIAN_POINT('Ctrl Pts',(-4.91221750856866,-1.30000000000066,
7.90618028712686));
#37209=CARTESIAN_POINT('Ctrl Pts',(-4.89732171538367,-1.18514270861235,
7.93676277428599));
#37210=CARTESIAN_POINT('Ctrl Pts',(-4.87613173456936,-1.06847604194559,
7.96021652033425));
#37211=CARTESIAN_POINT('Ctrl Pts',(-4.81263780727549,-0.794772684001163,
7.99793054754568));
#37212=CARTESIAN_POINT('Ctrl Pts',(-4.74518442134474,-0.636309800095445,
7.99557610459018));
#37213=CARTESIAN_POINT('Ctrl Pts',(-4.6725406087231,-0.319434907277283,
8.01211698986252));
#37214=CARTESIAN_POINT('Ctrl Pts',(-4.63141471593923,-0.158333333333394,
8.01089761866659));
#37215=CARTESIAN_POINT('Ctrl Pts',(-4.62588971921968,0.158333333333396,
8.04173769180815));
#37216=CARTESIAN_POINT('Ctrl Pts',(-4.66128991219664,0.319434907277292,
8.07474335059151));
#37217=CARTESIAN_POINT('Ctrl Pts',(-4.72308852205137,0.636309800095455,
8.11909410305302));
#37218=CARTESIAN_POINT('Ctrl Pts',(-4.78411408326621,0.79477268400115,8.15442691127934));
#37219=CARTESIAN_POINT('Ctrl Pts',(-4.84061394483196,1.06847604194569,8.16249551717092));
#37220=CARTESIAN_POINT('Ctrl Pts',(-4.85955619075815,1.18514270861257,8.15652027226193));
#37221=CARTESIAN_POINT('Ctrl Pts',(-4.87298398606488,1.300000000001,8.14107718192479));
#37222=CARTESIAN_POINT('Ctrl Pts',(-4.90590397924942,-1.30000000000065,
7.90176328971422));
#37223=CARTESIAN_POINT('Ctrl Pts',(-4.88977578450812,-1.18514270861234,
7.93153530673559));
#37224=CARTESIAN_POINT('Ctrl Pts',(-4.86768692716434,-1.06847604194558,
7.95439047087062));
#37225=CARTESIAN_POINT('Ctrl Pts',(-4.80288692480121,-0.794772684001158,
7.99121115830334));
#37226=CARTESIAN_POINT('Ctrl Pts',(-4.73567112619427,-0.636309800095442,
7.98899675141701));
#37227=CARTESIAN_POINT('Ctrl Pts',(-4.66302451807155,-0.319434907277281,
8.00541558753617));
#37228=CARTESIAN_POINT('Ctrl Pts',(-4.62232442101259,-0.158333333333393,
8.00439907906812));
#37229=CARTESIAN_POINT('Ctrl Pts',(-4.61687292524796,0.158333333333395,
8.03504454203713));
#37230=CARTESIAN_POINT('Ctrl Pts',(-4.65189635062452,0.31943490727729,8.06770186423874));
#37231=CARTESIAN_POINT('Ctrl Pts',(-4.71389732152674,0.636309800095451,
8.11167817180113));
#37232=CARTESIAN_POINT('Ctrl Pts',(-4.77496018471075,0.794772684001146,
8.14621029392679));
#37233=CARTESIAN_POINT('Ctrl Pts',(-4.83277887881808,1.06847604194569,8.15516634666519));
#37234=CARTESIAN_POINT('Ctrl Pts',(-4.85255522845339,1.18514270861256,8.14996319804911));
#37235=CARTESIAN_POINT('Ctrl Pts',(-4.86708035743869,1.30000000000099,8.13568015744095));
#37236=CARTESIAN_POINT('Ctrl Pts',(-4.90087799425075,-1.30000000000065,
7.89815843086838));
#37237=CARTESIAN_POINT('Ctrl Pts',(-4.88380456050229,-1.18514270861234,
7.9271602890803));
#37238=CARTESIAN_POINT('Ctrl Pts',(-4.86101812269967,-1.06847604194558,
7.94947168469374));
#37239=CARTESIAN_POINT('Ctrl Pts',(-4.79517871071664,-0.794772684001156,
7.98555916491523));
#37240=CARTESIAN_POINT('Ctrl Pts',(-4.72808987790012,-0.636309800095441,
7.98364475480844));
#37241=CARTESIAN_POINT('Ctrl Pts',(-4.65538329456378,-0.319434907277281,
8.00013082479717));
#37242=CARTESIAN_POINT('Ctrl Pts',(-4.61496515703839,-0.158333333333393,
7.99943824782273));
#37243=CARTESIAN_POINT('Ctrl Pts',(-4.60957871500424,0.158333333333395,
8.02991066345015));
#37244=CARTESIAN_POINT('Ctrl Pts',(-4.64440612757375,0.319434907277289,
8.06200266067117));
#37245=CARTESIAN_POINT('Ctrl Pts',(-4.70655702592597,0.63630980009545,8.10569846556605));
#37246=CARTESIAN_POINT('Ctrl Pts',(-4.76751286578663,0.794772684001145,
8.13993353417728));
#37247=CARTESIAN_POINT('Ctrl Pts',(-4.82637845774924,1.06847604194569,8.14962346925743));
#37248=CARTESIAN_POINT('Ctrl Pts',(-4.84684451433475,1.18514270861256,8.14498504018903));
#37249=CARTESIAN_POINT('Ctrl Pts',(-4.8622958939303,1.30000000000099,8.1315137682035));
#37250=CARTESIAN_POINT('Ctrl Pts',(-4.88837681016349,-1.30000000000063,
7.88895028194231));
#37251=CARTESIAN_POINT('Ctrl Pts',(-4.86900693933979,-1.18514270861232,
7.91582915034754));
#37252=CARTESIAN_POINT('Ctrl Pts',(-4.84451742320507,-1.06847604194556,
7.93665969675292));
#37253=CARTESIAN_POINT('Ctrl Pts',(-4.77611433697291,-0.794772684001145,
7.97080959230356));
#37254=CARTESIAN_POINT('Ctrl Pts',(-4.70929268250738,-0.636309800095433,
7.96979288413007));
#37255=CARTESIAN_POINT('Ctrl Pts',(-4.6363516185457,-0.319434907277277,
7.98669439873285));
#37256=CARTESIAN_POINT('Ctrl Pts',(-4.59652414874773,-0.158333333333391,
7.98714544677113));
#37257=CARTESIAN_POINT('Ctrl Pts',(-4.59125935571234,0.158333333333393,
8.01730741108527));
#37258=CARTESIAN_POINT('Ctrl Pts',(-4.62566171926125,0.319434907277285,
8.04780317230802));
#37259=CARTESIAN_POINT('Ctrl Pts',(-4.68820532536085,0.636309800095442,
8.09074073463353));
#37260=CARTESIAN_POINT('Ctrl Pts',(-4.74887696505617,0.794772684001136,
8.12426276571075));
#37261=CARTESIAN_POINT('Ctrl Pts',(-4.8103702126134,1.06847604194567,8.1357578335284));
#37262=CARTESIAN_POINT('Ctrl Pts',(-4.83256879930426,1.18514270861255,8.13251177472534));
#37263=CARTESIAN_POINT('Ctrl Pts',(-4.85034782436782,1.30000000000097,8.1210438681952));
#37264=CARTESIAN_POINT('Ctrl Pts',(-4.86688257452678,-1.30000000000049,
7.87399374566793));
#37265=CARTESIAN_POINT('Ctrl Pts',(-4.84340178599782,-1.18514270861219,
7.897854654973));
#37266=CARTESIAN_POINT('Ctrl Pts',(-4.81588313053963,-1.06847604194544,
7.91655196948616));
#37267=CARTESIAN_POINT('Ctrl Pts',(-4.742981250964,-0.794772684001054,7.94781756945355));
#37268=CARTESIAN_POINT('Ctrl Pts',(-4.67671488697888,-0.63630980009536,
7.94806267967043));
#37269=CARTESIAN_POINT('Ctrl Pts',(-4.60360265705701,-0.31943490727724,
7.96500904542826));
#37270=CARTESIAN_POINT('Ctrl Pts',(-4.56511770040999,-0.158333333333372,
7.96640620775939));
#37271=CARTESIAN_POINT('Ctrl Pts',(-4.56022059376211,0.158333333333375,
7.99554457965105));
#37272=CARTESIAN_POINT('Ctrl Pts',(-4.59380357309349,0.319434907277248,
8.02358096865707));
#37273=CARTESIAN_POINT('Ctrl Pts',(-4.65695067057653,0.636309800095368,
8.0653861091333));
#37274=CARTESIAN_POINT('Ctrl Pts',(-4.71707246892219,0.794772684001043,
8.0978669334104));
#37275=CARTESIAN_POINT('Ctrl Pts',(-4.78294691811059,1.06847604194555,8.11268991939168));
#37276=CARTESIAN_POINT('Ctrl Pts',(-4.80805404966436,1.18514270861242,8.1119314974408));
#37277=CARTESIAN_POINT('Ctrl Pts',(-4.82975370460714,1.30000000000083,8.1039983321535));
#37278=CARTESIAN_POINT('Ctrl Pts',(-4.84151828404587,-1.30000000000042,
7.85646916935349));
#37279=CARTESIAN_POINT('Ctrl Pts',(-4.81307876780055,-1.18514270861214,
7.87712509595763));
#37280=CARTESIAN_POINT('Ctrl Pts',(-4.78193549602595,-1.06847604194539,
7.89347420359149));
#37281=CARTESIAN_POINT('Ctrl Pts',(-4.70374209187939,-0.794772684001021,
7.92129429945595));
#37282=CARTESIAN_POINT('Ctrl Pts',(-4.63841532094869,-0.636309800095332,
7.92211268173844));
#37283=CARTESIAN_POINT('Ctrl Pts',(-4.56516336664136,-0.319434907277226,
7.93892324566879));
#37284=CARTESIAN_POINT('Ctrl Pts',(-4.52826122899799,-0.158333333333366,
7.94152088547465));
#37285=CARTESIAN_POINT('Ctrl Pts',(-4.52349391948293,0.158333333333368,
7.97030284749727));
#37286=CARTESIAN_POINT('Ctrl Pts',(-4.55556801363061,0.319434907277235,
7.99690404660842));
#37287=CARTESIAN_POINT('Ctrl Pts',(-4.61923301245898,0.636309800095341,
8.03787111873039));
#37288=CARTESIAN_POINT('Ctrl Pts',(-4.6788605164949,0.79477268400101,8.06865183019706));
#37289=CARTESIAN_POINT('Ctrl Pts',(-4.75023795639241,1.06847604194551,8.08646674481053));
#37290=CARTESIAN_POINT('Ctrl Pts',(-4.77898396544915,1.18514270861236,8.0880753688951));
#37291=CARTESIAN_POINT('Ctrl Pts',(-4.80557933462579,1.30000000000077,8.08358120063571));
#37292=CARTESIAN_POINT('Ctrl Pts',(-4.82112874987559,-1.30000000000039,
7.84277001524222));
#37293=CARTESIAN_POINT('Ctrl Pts',(-4.78880172461059,-1.1851427086121,7.8605584606925));
#37294=CARTESIAN_POINT('Ctrl Pts',(-4.7547519322164,-1.06847604194537,7.87501539674751));
#37295=CARTESIAN_POINT('Ctrl Pts',(-4.67211016344138,-0.794772684000998,
7.90071735796543));
#37296=CARTESIAN_POINT('Ctrl Pts',(-4.60692508051203,-0.636309800095313,
7.90397466208613));
#37297=CARTESIAN_POINT('Ctrl Pts',(-4.53340717249417,-0.319434907277217,
7.92114127676621));
#37298=CARTESIAN_POINT('Ctrl Pts',(-4.49803145325506,-0.158333333333361,
7.92381830623259));
#37299=CARTESIAN_POINT('Ctrl Pts',(-4.49361450863589,0.158333333333363,
7.95151283923301));
#37300=CARTESIAN_POINT('Ctrl Pts',(-4.52463871769815,0.319434907277226,
7.97646143477411));
#37301=CARTESIAN_POINT('Ctrl Pts',(-4.58902634230981,0.636309800095323,
8.01584695036339));
#37302=CARTESIAN_POINT('Ctrl Pts',(-4.64863712159789,0.794772684000986,
8.04422098867795));
#37303=CARTESIAN_POINT('Ctrl Pts',(-4.72434480941012,1.06847604194547,8.06466009624927));
#37304=CARTESIAN_POINT('Ctrl Pts',(-4.75585078787386,1.18514270861233,8.06860628573794));
#37305=CARTESIAN_POINT('Ctrl Pts',(-4.78609169199371,1.30000000000073,8.0676513323912));
#37306=CARTESIAN_POINT('Ctrl Pts',(-4.80579794746511,-1.30000000000037,
7.83248813918676));
#37307=CARTESIAN_POINT('Ctrl Pts',(-4.77028007162946,-1.18514270861208,
7.84904374373791));
#37308=CARTESIAN_POINT('Ctrl Pts',(-4.73393636878789,-1.06847604194535,
7.86246982037874));
#37309=CARTESIAN_POINT('Ctrl Pts',(-4.64806731910125,-0.794772684000984,
7.88625690776372));
#37310=CARTESIAN_POINT('Ctrl Pts',(-4.58389442940921,-0.636309800095303,
7.8883926499238));
#37311=CARTESIAN_POINT('Ctrl Pts',(-4.51027105908399,-0.319434907277212,
7.90553912776898));
#37312=CARTESIAN_POINT('Ctrl Pts',(-4.47547361646124,-0.158333333333358,
7.91015777895858));
#37313=CARTESIAN_POINT('Ctrl Pts',(-4.47101506047161,0.158333333333361,
7.93799763499912));
#37314=CARTESIAN_POINT('Ctrl Pts',(-4.50131739459165,0.31943490727722,7.96147710343081));
#37315=CARTESIAN_POINT('Ctrl Pts',(-4.56593346222998,0.636309800095312,
8.00051234348569));
#37316=CARTESIAN_POINT('Ctrl Pts',(-4.6248930339895,0.794772684000973,8.02878061626448));
#37317=CARTESIAN_POINT('Ctrl Pts',(-4.70399233636378,1.06847604194546,8.0507728789089));
#37318=CARTESIAN_POINT('Ctrl Pts',(-4.73781730149281,1.18514270861231,8.05578862073716));
#37319=CARTESIAN_POINT('Ctrl Pts',(-4.77122807467102,1.30000000000071,8.05630046878855));
#37320=CARTESIAN_POINT('Ctrl Pts',(-4.79013869260304,-1.30000000000035,
7.82347634664023));
#37321=CARTESIAN_POINT('Ctrl Pts',(-4.75171347795003,-1.18514270861206,
7.837781748419));
#37322=CARTESIAN_POINT('Ctrl Pts',(-4.7131865700244,-1.06847604194533,7.84975228894376));
#37323=CARTESIAN_POINT('Ctrl Pts',(-4.62394677363127,-0.794772684000971,
7.87201263567021));
#37324=CARTESIAN_POINT('Ctrl Pts',(-4.5597935968354,-0.636309800095291,
7.87633136950941));
#37325=CARTESIAN_POINT('Ctrl Pts',(-4.48594654724452,-0.319434907277205,
7.89382691479891));
#37326=CARTESIAN_POINT('Ctrl Pts',(-4.45225272357408,-0.158333333333356,
7.89861844168121));
#37327=CARTESIAN_POINT('Ctrl Pts',(-4.44824328709278,0.158333333333358,
7.92500913485026));
#37328=CARTESIAN_POINT('Ctrl Pts',(-4.47811132969497,0.319434907277216,
7.94608132457026));
#37329=CARTESIAN_POINT('Ctrl Pts',(-4.54341735300971,0.636309800095302,
7.98341513439605));
#37330=CARTESIAN_POINT('Ctrl Pts',(-4.6022310012356,0.794772684000958,8.01027478191746));
#37331=CARTESIAN_POINT('Ctrl Pts',(-4.68450819501405,1.06847604194544,8.03446676261853));
#37332=CARTESIAN_POINT('Ctrl Pts',(-4.72036882450999,1.18514270861228,8.04136088759017));
#37333=CARTESIAN_POINT('Ctrl Pts',(-4.75647533498565,1.30000000000068,8.04467732548917));
#37334=CARTESIAN_POINT('Ctrl Pts',(-4.77489914987303,-1.30000000000033,
7.81282546636895));
#37335=CARTESIAN_POINT('Ctrl Pts',(-4.73340430295669,-1.18514270861205,
7.82546882596531));
#37336=CARTESIAN_POINT('Ctrl Pts',(-4.69261841482826,-1.06847604194531,
7.83627450334434));
#37337=CARTESIAN_POINT('Ctrl Pts',(-4.6000326906894,-0.794772684000959,
7.85699236620913));
#37338=CARTESIAN_POINT('Ctrl Pts',(-4.53636034458574,-0.636309800095283,
7.86197068256707));
#37339=CARTESIAN_POINT('Ctrl Pts',(-4.46231435141602,-0.319434907277201,
7.87976329549689));
#37340=CARTESIAN_POINT('Ctrl Pts',(-4.4295828439994,-0.158333333333353,
7.8852526458423));
#37341=CARTESIAN_POINT('Ctrl Pts',(-4.42551665113566,0.158333333333356,
7.91179396725503));
#37342=CARTESIAN_POINT('Ctrl Pts',(-4.45425909385832,0.319434907277209,
7.93260279656291));
#37343=CARTESIAN_POINT('Ctrl Pts',(-4.51986544041176,0.636309800095291,
7.96936820656945));
#37344=CARTESIAN_POINT('Ctrl Pts',(-4.57852879619251,0.794772684000948,
7.99463506736218));
#37345=CARTESIAN_POINT('Ctrl Pts',(-4.66435698263534,1.06847604194542,8.01991355514737));
#37346=CARTESIAN_POINT('Ctrl Pts',(-4.7025363183252,1.18514270861227,8.02788276798637));
#37347=CARTESIAN_POINT('Ctrl Pts',(-4.74174314804155,1.30000000000067,8.03287907296246));
#37348=CARTESIAN_POINT('Ctrl Pts',(-4.76161182290268,-1.30000000000032,
7.80610825536315));
#37349=CARTESIAN_POINT('Ctrl Pts',(-4.71752842160646,-1.18514270861204,
7.81742462867045));
#37350=CARTESIAN_POINT('Ctrl Pts',(-4.67485111019541,-1.06847604194531,
7.82725239943781));
#37351=CARTESIAN_POINT('Ctrl Pts',(-4.57950633219105,-0.794772684000953,
7.84651754628806));
#37352=CARTESIAN_POINT('Ctrl Pts',(-4.51634868295189,-0.636309800095279,
7.85163572302273));
#37353=CARTESIAN_POINT('Ctrl Pts',(-4.44219644796232,-0.3194349072772,7.86944813166365));
#37354=CARTESIAN_POINT('Ctrl Pts',(-4.41017374720179,-0.158333333333352,
7.87583513286652));
#37355=CARTESIAN_POINT('Ctrl Pts',(-4.40623331788559,0.158333333333355,
7.90192986702047));
#37356=CARTESIAN_POINT('Ctrl Pts',(-4.43438298209535,0.319434907277207,
7.92139088711657));
#37357=CARTESIAN_POINT('Ctrl Pts',(-4.50037157207737,0.636309800095287,
7.95723410938572));
#37358=CARTESIAN_POINT('Ctrl Pts',(-4.5587905780062,0.794772684000944,7.9815530285965));
#37359=CARTESIAN_POINT('Ctrl Pts',(-4.64745198274385,1.06847604194542,8.00810940448882));
#37360=CARTESIAN_POINT('Ctrl Pts',(-4.68749140106699,1.18514270861226,8.01718845533252));
#37361=CARTESIAN_POINT('Ctrl Pts',(-4.72919200083113,1.30000000000066,8.02385128590684));
#37362=CARTESIAN_POINT('Ctrl Pts',(-4.751434470258,-1.30000000000032,7.79902289403952));
#37363=CARTESIAN_POINT('Ctrl Pts',(-4.70529589232437,-1.18514270861203,
7.80924536461335));
#37364=CARTESIAN_POINT('Ctrl Pts',(-4.66109034485469,-1.0684760419453,7.81836178493761));
#37365=CARTESIAN_POINT('Ctrl Pts',(-4.56343237398343,-0.794772684000951,
7.83686734227923));
#37366=CARTESIAN_POINT('Ctrl Pts',(-4.50047624693983,-0.636309800095276,
7.84283414873083));
#37367=CARTESIAN_POINT('Ctrl Pts',(-4.4261047074392,-0.319434907277198,
7.86115706837341));
#37368=CARTESIAN_POINT('Ctrl Pts',(-4.39464806145917,-0.158333333333352,
7.86829614150567));
#37369=CARTESIAN_POINT('Ctrl Pts',(-4.39079493705768,0.158333333333354,
7.894078837855));
#37370=CARTESIAN_POINT('Ctrl Pts',(-4.41848568860533,0.319434907277207,
7.91235912758977));
#37371=CARTESIAN_POINT('Ctrl Pts',(-4.48483100996797,0.636309800095286,
7.9472937881376));
#37372=CARTESIAN_POINT('Ctrl Pts',(-4.54317603144512,0.79477268400094,7.97050145391679));
#37373=CARTESIAN_POINT('Ctrl Pts',(-4.63405963255871,1.06847604194541,7.9982291981047));
#37374=CARTESIAN_POINT('Ctrl Pts',(-4.67552950583216,1.18514270861226,8.00837888207417));
#37375=CARTESIAN_POINT('Ctrl Pts',(-4.71912910902628,1.30000000000066,8.01667593696833));
#37376=CARTESIAN_POINT('Ctrl Pts',(-4.73578719298179,-1.3000000000003,7.78983839804538));
#37377=CARTESIAN_POINT('Ctrl Pts',(-4.68659125419676,-1.18514270861203,
7.7983113785018));
#37378=CARTESIAN_POINT('Ctrl Pts',(-4.64012373839081,-1.0684760419453,7.80623938864637));
#37379=CARTESIAN_POINT('Ctrl Pts',(-4.53907768398521,-0.794772684000947,
7.82329568763203));
#37380=CARTESIAN_POINT('Ctrl Pts',(-4.47647185678535,-0.636309800095271,
7.83038096282361));
#37381=CARTESIAN_POINT('Ctrl Pts',(-4.40190948645908,-0.319434907277195,
7.84895368410313));
#37382=CARTESIAN_POINT('Ctrl Pts',(-4.37149167166539,-0.15833333333335,
7.85650826084508));
#37383=CARTESIAN_POINT('Ctrl Pts',(-4.36774732594694,0.158333333333353,
7.88187198112008));
#37384=CARTESIAN_POINT('Ctrl Pts',(-4.39453562043689,0.319434907277204,
7.89916475334937));
#37385=CARTESIAN_POINT('Ctrl Pts',(-4.46123713703452,0.63630980009528,7.93330791518739));
#37386=CARTESIAN_POINT('Ctrl Pts',(-4.5192165770096,0.794772684000933,7.95555481439467));
#37387=CARTESIAN_POINT('Ctrl Pts',(-4.61365511815839,1.0684760419454,7.98435171132209));
#37388=CARTESIAN_POINT('Ctrl Pts',(-4.65748255750737,1.18514270861225,7.99546447667734));
#37389=CARTESIAN_POINT('Ctrl Pts',(-4.70425849103481,1.30000000000064,8.00522489773817));
#37390=CARTESIAN_POINT('Ctrl Pts',(-4.71238759485044,-1.30000000000028,
7.77568997553473));
#37391=CARTESIAN_POINT('Ctrl Pts',(-4.65836428021862,-1.185142708612,7.78243366970776));
#37392=CARTESIAN_POINT('Ctrl Pts',(-4.6083436035125,-1.06847604194527,7.78917874543528));
#37393=CARTESIAN_POINT('Ctrl Pts',(-4.50203272805262,-0.794772684000925,
7.80476441138087));
#37394=CARTESIAN_POINT('Ctrl Pts',(-4.4401680936263,-0.63630980009526,7.81276995314513));
#37395=CARTESIAN_POINT('Ctrl Pts',(-4.36530930032411,-0.319434907277191,
7.83178520154449));
#37396=CARTESIAN_POINT('Ctrl Pts',(-4.33632940633184,-0.158333333333348,
7.84042764005913));
#37397=CARTESIAN_POINT('Ctrl Pts',(-4.33274105297626,0.15833333333335,7.86516233735358));
#37398=CARTESIAN_POINT('Ctrl Pts',(-4.35816294414213,0.319434907277198,
7.88090940365321));
#37399=CARTESIAN_POINT('Ctrl Pts',(-4.42565069818634,0.636309800095269,
7.91298008491273));
#37400=CARTESIAN_POINT('Ctrl Pts',(-4.48367624716704,0.794772684000921,
7.93188635609983));
#37401=CARTESIAN_POINT('Ctrl Pts',(-4.58335118562598,1.06847604194539,7.96252186347471));
#37402=CARTESIAN_POINT('Ctrl Pts',(-4.63051192582729,1.18514270861223,7.97568900065146));
#37403=CARTESIAN_POINT('Ctrl Pts',(-4.68168781869149,1.30000000000062,7.98876229901981));
#37404=CARTESIAN_POINT('Ctrl Pts',(-4.68068425748576,-1.30000000000025,
7.75862761062044));
#37405=CARTESIAN_POINT('Ctrl Pts',(-4.62041273591367,-1.18514270861197,
7.76225791249285));
#37406=CARTESIAN_POINT('Ctrl Pts',(-4.56574818199531,-1.06847604194525,
7.76701611525181));
#37407=CARTESIAN_POINT('Ctrl Pts',(-4.45241534378754,-0.794772684000912,
7.78061419218393));
#37408=CARTESIAN_POINT('Ctrl Pts',(-4.39110918291877,-0.636309800095245,
7.7916246561428));
#37409=CARTESIAN_POINT('Ctrl Pts',(-4.31573727102646,-0.319434907277182,
7.81170467698355));
#37410=CARTESIAN_POINT('Ctrl Pts',(-4.2887792412685,-0.158333333333344,
7.82138929851315));
#37411=CARTESIAN_POINT('Ctrl Pts',(-4.28553660227673,0.158333333333346,
7.84465438395679));
#37412=CARTESIAN_POINT('Ctrl Pts',(-4.3094926211426,0.319434907277191,7.85693583601697));
#37413=CARTESIAN_POINT('Ctrl Pts',(-4.37776936877316,0.636309800095255,
7.88689111269756));
#37414=CARTESIAN_POINT('Ctrl Pts',(-4.43481700835146,0.794772684000901,
7.90463604211364));
#37415=CARTESIAN_POINT('Ctrl Pts',(-4.54155275115623,1.06847604194536,7.93754731631996));
#37416=CARTESIAN_POINT('Ctrl Pts',(-4.59343691227159,1.1851427086122,7.95263540923971));
#37417=CARTESIAN_POINT('Ctrl Pts',(-4.65100328639117,1.30000000000059,7.96856552395818));
#37418=CARTESIAN_POINT('Ctrl Pts',(-4.65412859982384,-1.3000000000002,7.74500676190758));
#37419=CARTESIAN_POINT('Ctrl Pts',(-4.58846168458542,-1.18514270861193,
7.74693192997448));
#37420=CARTESIAN_POINT('Ctrl Pts',(-4.52981289644311,-1.06847604194521,
7.75060684134227));
#37421=CARTESIAN_POINT('Ctrl Pts',(-4.41053574074808,-0.794772684000884,
7.76313887882534));
#37422=CARTESIAN_POINT('Ctrl Pts',(-4.35000766089167,-0.636309800095221,
7.77548844878813));
#37423=CARTESIAN_POINT('Ctrl Pts',(-4.27413821844525,-0.31943490727717,
7.79685341886066));
#37424=CARTESIAN_POINT('Ctrl Pts',(-4.24858903766098,-0.158333333333338,
7.80860652078929));
#37425=CARTESIAN_POINT('Ctrl Pts',(-4.2454329537061,0.158333333333341,7.83132513803103));
#37426=CARTESIAN_POINT('Ctrl Pts',(-4.26791211437986,0.319434907277179,
7.84137487601959));
#37427=CARTESIAN_POINT('Ctrl Pts',(-4.33717753520158,0.636309800095231,
7.86815146594569));
#37428=CARTESIAN_POINT('Ctrl Pts',(-4.39429388038338,0.794772684000871,
7.88171031687834));
#37429=CARTESIAN_POINT('Ctrl Pts',(-4.50724165666521,1.06847604194532,7.91512818724497));
#37430=CARTESIAN_POINT('Ctrl Pts',(-4.56307192346659,1.18514270861215,7.93167421003735));
#37431=CARTESIAN_POINT('Ctrl Pts',(-4.62584154984451,1.30000000000054,7.95030089779451));
#37432=CARTESIAN_POINT('Ctrl Pts',(-4.63294304514757,-1.3000000000002,7.73363723320236));
#37433=CARTESIAN_POINT('Ctrl Pts',(-4.56293910323236,-1.18514270861193,
7.73404012696683));
#37434=CARTESIAN_POINT('Ctrl Pts',(-4.50104605242609,-1.06847604194521,
7.73691769506999));
#37435=CARTESIAN_POINT('Ctrl Pts',(-4.37679850444107,-0.794772684000881,
7.74928244582305));
#37436=CARTESIAN_POINT('Ctrl Pts',(-4.31645108600974,-0.636309800095221,
7.76471095515052));
#37437=CARTESIAN_POINT('Ctrl Pts',(-4.24020673369042,-0.319434907277171,
7.78698860707724));
#37438=CARTESIAN_POINT('Ctrl Pts',(-4.21629109567086,-0.158333333333338,
7.7982385847441));
#37439=CARTESIAN_POINT('Ctrl Pts',(-4.21332902939037,0.15833333333334,7.81993355065792));
#37440=CARTESIAN_POINT('Ctrl Pts',(-4.23450068448092,0.319434907277178,
7.82873972143735));
#37441=CARTESIAN_POINT('Ctrl Pts',(-4.30426730097828,0.63630980009523,7.85399130617029));
#37442=CARTESIAN_POINT('Ctrl Pts',(-4.36098494754636,0.794772684000871,
7.86566832729003));
#37443=CARTESIAN_POINT('Ctrl Pts',(-4.47876340129364,1.06847604194532,7.90015581847597));
#37444=CARTESIAN_POINT('Ctrl Pts',(-4.53777653582107,1.18514270861215,7.91791658710113));
#37445=CARTESIAN_POINT('Ctrl Pts',(-4.60482087637055,1.30000000000054,7.93850976730455));
#37446=CARTESIAN_POINT('Ctrl Pts',(-4.6168608328518,-1.30000000000018,7.72606704168878));
#37447=CARTESIAN_POINT('Ctrl Pts',(-4.54358307191281,-1.18514270861192,
7.72568677646031));
#37448=CARTESIAN_POINT('Ctrl Pts',(-4.47927319496849,-1.0684760419452,7.72810685793159));
#37449=CARTESIAN_POINT('Ctrl Pts',(-4.35142212012702,-0.794772684000877,
7.7401670913497));
#37450=CARTESIAN_POINT('Ctrl Pts',(-4.29156209657586,-0.636309800095215,
7.75644417809687));
#37451=CARTESIAN_POINT('Ctrl Pts',(-4.21500073541837,-0.319434907277167,
7.77967099750095));
#37452=CARTESIAN_POINT('Ctrl Pts',(-4.19190516024014,-0.158333333333336,
7.79227950123383));
#37453=CARTESIAN_POINT('Ctrl Pts',(-4.18897493925662,0.158333333333339,
7.81366169079514));
#37454=CARTESIAN_POINT('Ctrl Pts',(-4.209285431662,0.319434907277175,7.82095446965029));
#37455=CARTESIAN_POINT('Ctrl Pts',(-4.27958250757412,0.636309800095223,
7.84429813168956));
#37456=CARTESIAN_POINT('Ctrl Pts',(-4.33613614571148,0.794772684000864,
7.85394641256676));
#37457=CARTESIAN_POINT('Ctrl Pts',(-4.45774599007139,1.06847604194531,7.88820003389546));
#37458=CARTESIAN_POINT('Ctrl Pts',(-4.51924087753763,1.18514270861214,7.90639059637782));
#37459=CARTESIAN_POINT('Ctrl Pts',(-4.58959025693552,1.30000000000053,7.92794459789109));
#37460=CARTESIAN_POINT('Ctrl Pts',(-4.60067713755899,-1.30000000000017,
7.71855328487674));
#37461=CARTESIAN_POINT('Ctrl Pts',(-4.52403569735226,-1.18514270861191,
7.71709481226507));
#37462=CARTESIAN_POINT('Ctrl Pts',(-4.45719976387259,-1.06847604194519,
7.71903031071803));
#37463=CARTESIAN_POINT('Ctrl Pts',(-4.32544806917629,-0.794772684000868,
7.73134245146043));
#37464=CARTESIAN_POINT('Ctrl Pts',(-4.26552769529275,-0.636309800095211,
7.75107352021072));
#37465=CARTESIAN_POINT('Ctrl Pts',(-4.18886738502932,-0.319434907277166,
7.77408197784996));
#37466=CARTESIAN_POINT('Ctrl Pts',(-4.16758864112992,-0.158333333333336,
7.78351981943754));
#37467=CARTESIAN_POINT('Ctrl Pts',(-4.16487016749168,0.158333333333338,
7.80371054916999));
#37468=CARTESIAN_POINT('Ctrl Pts',(-4.183697750681,0.319434907277175,7.81221977204047));
#37469=CARTESIAN_POINT('Ctrl Pts',(-4.25427622869244,0.636309800095221,
7.8349085617001));
#37470=CARTESIAN_POINT('Ctrl Pts',(-4.3107122638051,0.79477268400086,7.84232650600807));
#37471=CARTESIAN_POINT('Ctrl Pts',(-4.43616916091367,1.0684760419453,7.87694127733603));
#37472=CARTESIAN_POINT('Ctrl Pts',(-4.50017163882838,1.18514270861213,7.89586553247259));
#37473=CARTESIAN_POINT('Ctrl Pts',(-4.57387095253565,1.30000000000052,7.9187305908415));
#37474=CARTESIAN_POINT('Ctrl Pts',(-4.58730781279972,-1.30000000000017,
7.71230138859931));
#37475=CARTESIAN_POINT('Ctrl Pts',(-4.50788362503931,-1.1851427086119,7.71094533350715));
#37476=CARTESIAN_POINT('Ctrl Pts',(-4.4390616358845,-1.06847604194518,7.71275877394741));
#37477=CARTESIAN_POINT('Ctrl Pts',(-4.3045622728866,-0.794772684000865,
7.72427035287721));
#37478=CARTESIAN_POINT('Ctrl Pts',(-4.24555331669918,-0.636309800095205,
7.74236664972257));
#37479=CARTESIAN_POINT('Ctrl Pts',(-4.16904001114168,-0.319434907277162,
7.76453178614663));
#37480=CARTESIAN_POINT('Ctrl Pts',(-4.14872086860415,-0.158333333333334,
7.7739781792026));
#37481=CARTESIAN_POINT('Ctrl Pts',(-4.14585353447854,0.158333333333337,
7.79478399944369));
#37482=CARTESIAN_POINT('Ctrl Pts',(-4.16336823012039,0.319434907277172,
7.80482177380069));
#37483=CARTESIAN_POINT('Ctrl Pts',(-4.23391288575959,0.636309800095215,
7.82772870678767));
#37484=CARTESIAN_POINT('Ctrl Pts',(-4.29012932459028,0.794772684000851,
7.83345416959625));
#37485=CARTESIAN_POINT('Ctrl Pts',(-4.41847992247652,1.06847604194529,7.86836987702009));
#37486=CARTESIAN_POINT('Ctrl Pts',(-4.48441830653494,1.18514270861212,7.8877977601388));
#37487=CARTESIAN_POINT('Ctrl Pts',(-4.56073685668519,1.30000000000051,7.91153981038689));
#37488=CARTESIAN_POINT('Ctrl Pts',(-4.57096682812091,-1.30000000000016,
7.70550102152383));
#37489=CARTESIAN_POINT('Ctrl Pts',(-4.48783339483817,-1.1851427086119,7.7041546867954));
#37490=CARTESIAN_POINT('Ctrl Pts',(-4.41636673485974,-1.06847604194518,
7.7055682845817));
#37491=CARTESIAN_POINT('Ctrl Pts',(-4.27821703371616,-0.79477268400086,
7.71520997448892));
#37492=CARTESIAN_POINT('Ctrl Pts',(-4.22041201886117,-0.636309800095203,
7.73017506044892));
#37493=CARTESIAN_POINT('Ctrl Pts',(-4.1441697959739,-0.319434907277162,
7.75018142748202));
#37494=CARTESIAN_POINT('Ctrl Pts',(-4.12517779033268,-0.158333333333334,
7.75942312339014));
#37495=CARTESIAN_POINT('Ctrl Pts',(-4.12231328988027,0.158333333333336,
7.78010768802387));
#37496=CARTESIAN_POINT('Ctrl Pts',(-4.13842233140064,0.31943490727717,7.79052990985211));
#37497=CARTESIAN_POINT('Ctrl Pts',(-4.2088673822804,0.636309800095213,7.81473549588073));
#37498=CARTESIAN_POINT('Ctrl Pts',(-4.26426830305468,0.794772684000848,
7.82182773003922));
#37499=CARTESIAN_POINT('Ctrl Pts',(-4.39635488621716,1.06847604194529,7.85846836579053));
#37500=CARTESIAN_POINT('Ctrl Pts',(-4.46490150414816,1.18514270861212,7.8786290559999));
#37501=CARTESIAN_POINT('Ctrl Pts',(-4.54481935244935,1.30000000000051,7.90309006287123));
#37502=CARTESIAN_POINT('Ctrl Pts',(-4.55986191625154,-1.30000000000015,
7.70077302060858));
#37503=CARTESIAN_POINT('Ctrl Pts',(-4.47390766112863,-1.18514270861188,
7.70077480939679));
#37504=CARTESIAN_POINT('Ctrl Pts',(-4.40061540553237,-1.06847604194517,
7.70244469619189));
#37505=CARTESIAN_POINT('Ctrl Pts',(-4.26054738497045,-0.794772684000851,
7.71015610884605));
#37506=CARTESIAN_POINT('Ctrl Pts',(-4.20510952843759,-0.636309800095197,
7.7189877024356));
#37507=CARTESIAN_POINT('Ctrl Pts',(-4.13001103025471,-0.319434907277159,
7.73569629635065));
#37508=CARTESIAN_POINT('Ctrl Pts',(-4.11199983529727,-0.158333333333332,
7.74537650603382));
#37509=CARTESIAN_POINT('Ctrl Pts',(-4.1092062507607,0.158333333333335,7.76590783488345));
#37510=CARTESIAN_POINT('Ctrl Pts',(-4.12443963758816,0.319434907277167,
7.77588343648702));
#37511=CARTESIAN_POINT('Ctrl Pts',(-4.19381566981051,0.636309800095207,
7.80277904737017));
#37512=CARTESIAN_POINT('Ctrl Pts',(-4.24681642623153,0.794772684000841,
7.81488250821034));
#37513=CARTESIAN_POINT('Ctrl Pts',(-4.38081889489758,1.06847604194528,7.85351577237354));
#37514=CARTESIAN_POINT('Ctrl Pts',(-4.45118854322609,1.18514270861211,7.87373889304781));
#37515=CARTESIAN_POINT('Ctrl Pts',(-4.53392313647837,1.30000000000049,7.8974622258436));
#37516=CARTESIAN_POINT('Ctrl Pts',(-4.55333646119712,-1.30000000000015,
7.69516819779691));
#37517=CARTESIAN_POINT('Ctrl Pts',(-4.46759044005481,-1.18514270861188,
7.69531068083379));
#37518=CARTESIAN_POINT('Ctrl Pts',(-4.39457954353638,-1.06847604194517,
7.69678116104379));
#37519=CARTESIAN_POINT('Ctrl Pts',(-4.25533045233313,-0.794772684000851,
7.70324620363229));
#37520=CARTESIAN_POINT('Ctrl Pts',(-4.20084799529369,-0.636309800095197,
7.7096965632967));
#37521=CARTESIAN_POINT('Ctrl Pts',(-4.1264371815048,-0.319434907277159,
7.724865141945));
#37522=CARTESIAN_POINT('Ctrl Pts',(-4.1083738762426,-0.158333333333332,
7.73455031738056));
#37523=CARTESIAN_POINT('Ctrl Pts',(-4.10569625638313,0.158333333333335,
7.75487515336321));
#37524=CARTESIAN_POINT('Ctrl Pts',(-4.12120905306815,0.319434907277167,
7.76438231270788));
#37525=CARTESIAN_POINT('Ctrl Pts',(-4.18990683146856,0.636309800095207,
7.792920784926));
#37526=CARTESIAN_POINT('Ctrl Pts',(-4.24157890048061,0.794772684000841,
7.80842294468367));
#37527=CARTESIAN_POINT('Ctrl Pts',(-4.37480433638251,1.06847604194528,7.84815479663225));
#37528=CARTESIAN_POINT('Ctrl Pts',(-4.44499154163424,1.18514270861211,7.86827306771218));
#37529=CARTESIAN_POINT('Ctrl Pts',(-4.52769759742464,1.30000000000049,7.89131116337371));
#37530=CARTESIAN_POINT('Ctrl Pts',(-4.55333646119701,-1.3,7.69516819779691));
#37531=CARTESIAN_POINT('Ctrl Pts',(-4.46759044005475,-1.18514270861178,
7.69531068083379));
#37532=CARTESIAN_POINT('Ctrl Pts',(-4.39457954353636,-1.06847604194512,
7.69678116104379));
#37533=CARTESIAN_POINT('Ctrl Pts',(-4.25533045233314,-0.794772684000851,
7.70324620363229));
#37534=CARTESIAN_POINT('Ctrl Pts',(-4.20084799529369,-0.636309800095197,
7.7096965632967));
#37535=CARTESIAN_POINT('Ctrl Pts',(-4.1264371815048,-0.319434907277159,
7.724865141945));
#37536=CARTESIAN_POINT('Ctrl Pts',(-4.1083738762426,-0.158333333333332,
7.73455031738056));
#37537=CARTESIAN_POINT('Ctrl Pts',(-4.10569625638312,0.158333333333334,
7.7548751533632));
#37538=CARTESIAN_POINT('Ctrl Pts',(-4.12120905306815,0.319434907277167,
7.76438231270788));
#37539=CARTESIAN_POINT('Ctrl Pts',(-4.18990683146856,0.636309800095206,
7.792920784926));
#37540=CARTESIAN_POINT('Ctrl Pts',(-4.24157890048061,0.79477268400084,7.80842294468366));
#37541=CARTESIAN_POINT('Ctrl Pts',(-4.37480433638243,1.06847604194511,7.84815479663222));
#37542=CARTESIAN_POINT('Ctrl Pts',(-4.44499154163404,1.18514270861178,7.86827306771212));
#37543=CARTESIAN_POINT('Ctrl Pts',(-4.52769759742429,1.3,7.89131116337361));
#37544=CARTESIAN_POINT('',(-4.8959285873767,-1.2,7.92964598765946));
#37545=CARTESIAN_POINT('Ctrl Pts',(-4.8959285873767,-1.2,7.92964598765946));
#37546=CARTESIAN_POINT('Ctrl Pts',(-4.88128614180205,-1.21682133722576,
7.91377904453193));
#37547=CARTESIAN_POINT('Ctrl Pts',(-4.86705709202731,-1.23328464930557,
7.89716046450904));
#37548=CARTESIAN_POINT('Ctrl Pts',(-4.82891600865078,-1.27679348086419,
7.85588891014176));
#37549=CARTESIAN_POINT('Ctrl Pts',(-4.81667637007595,-1.29060520248064,
7.84294482434472));
#37550=CARTESIAN_POINT('Ctrl Pts',(-4.80971615050746,-1.29844967893122,
7.83574479480255));
#37551=CARTESIAN_POINT('Ctrl Pts',(-4.8090271842101,-1.29922545708331,7.83503667156741));
#37552=CARTESIAN_POINT('Ctrl Pts',(-4.80833847418889,-1.30000000000037,
7.83433517767123));
#37553=CARTESIAN_POINT('',(-4.8704124160437,-0.653834841416788,8.08407177162779));
#37554=CARTESIAN_POINT('Ctrl Pts',(-4.87041241606985,-0.653834841416102,
8.08407177162979));
#37555=CARTESIAN_POINT('Ctrl Pts',(-4.87331744329784,-0.717939165694387,
8.06806777610109));
#37556=CARTESIAN_POINT('Ctrl Pts',(-4.87562719338777,-0.763825235527143,
8.05500749471629));
#37557=CARTESIAN_POINT('Ctrl Pts',(-4.88440882003114,-0.949536215866272,
8.00391931523675));
#37558=CARTESIAN_POINT('Ctrl Pts',(-4.88885629259023,-1.04568967639883,
7.9771011245465));
#37559=CARTESIAN_POINT('Ctrl Pts',(-4.8959285873767,-1.2,7.92964598765946));
#37560=CARTESIAN_POINT('',(-4.84356468978495,0.653834841531101,8.22097066356893));
#37561=CARTESIAN_POINT('Ctrl Pts',(-4.84356468978495,0.653834841531099,
8.22097066356893));
#37562=CARTESIAN_POINT('Ctrl Pts',(-4.81020009414171,0.575793149317761,
8.19600115080956));
#37563=CARTESIAN_POINT('Ctrl Pts',(-4.78265018138025,0.493919053872489,
8.1745279229996));
#37564=CARTESIAN_POINT('Ctrl Pts',(-4.74428415111832,0.338198890099698,
8.14139392359785));
#37565=CARTESIAN_POINT('Ctrl Pts',(-4.731584258065,0.265711321162047,8.12875730458245));
#37566=CARTESIAN_POINT('Ctrl Pts',(-4.71756354556536,0.129739858083149,
8.10877297973432));
#37567=CARTESIAN_POINT('Ctrl Pts',(-4.71484516590534,0.0666407666263151,
8.10094744092773));
#37568=CARTESIAN_POINT('Ctrl Pts',(-4.71704691134613,-0.0595497741256923,
8.08778747206704));
#37569=CARTESIAN_POINT('Ctrl Pts',(-4.72196721471519,-0.12279612842464,
8.08234971685884));
#37570=CARTESIAN_POINT('Ctrl Pts',(-4.74094387627607,-0.260145569197153,
8.0739688976417));
#37571=CARTESIAN_POINT('Ctrl Pts',(-4.75650261542264,-0.333943518744006,
8.07165826059291));
#37572=CARTESIAN_POINT('Ctrl Pts',(-4.80134670116416,-0.491230496872132,
8.07250778651032));
#37573=CARTESIAN_POINT('Ctrl Pts',(-4.83256715599814,-0.574163160314909,
8.07651308744752));
#37574=CARTESIAN_POINT('Ctrl Pts',(-4.87041241602633,-0.653834841428499,
8.08407177159134));
#37575=CARTESIAN_POINT('',(-4.85793966858526,1.2,8.15022217211857));
#37576=CARTESIAN_POINT('Ctrl Pts',(-4.85793966858526,1.2,8.15022217211857));
#37577=CARTESIAN_POINT('Ctrl Pts',(-4.85558604305792,1.13519300442415,8.16225490630404));
#37578=CARTESIAN_POINT('Ctrl Pts',(-4.85238400598773,1.03885769118231,8.17837680110599));
#37579=CARTESIAN_POINT('Ctrl Pts',(-4.84595734033846,0.795132005601969,
8.20963889291911));
#37580=CARTESIAN_POINT('Ctrl Pts',(-4.84491963285573,0.74167848084335,8.21454270765557));
#37581=CARTESIAN_POINT('Ctrl Pts',(-4.84356468978495,0.653834841531102,
8.22097066356893));
#37582=CARTESIAN_POINT('Ctrl Pts',(-4.77350315750449,1.30000000000006,8.05800210098462));
#37583=CARTESIAN_POINT('Ctrl Pts',(-4.78796292235706,1.28314221689022,8.07284648759814));
#37584=CARTESIAN_POINT('Ctrl Pts',(-4.80201716658242,1.26652079478402,8.08834475124509));
#37585=CARTESIAN_POINT('Ctrl Pts',(-4.83622047073047,1.22603540792557,8.12558944398319));
#37586=CARTESIAN_POINT('Ctrl Pts',(-4.84546925287898,1.21510518302868,8.13528868680846));
#37587=CARTESIAN_POINT('Ctrl Pts',(-4.85793966858526,1.2,8.15022217211857));
#37588=CARTESIAN_POINT('Ctrl Pts',(-4.55333646119701,-1.3,7.69516819779691));
#37589=CARTESIAN_POINT('Ctrl Pts',(-4.46759044005475,-1.18514270861178,
7.69531068083379));
#37590=CARTESIAN_POINT('Ctrl Pts',(-4.39457954353636,-1.06847604194512,
7.69678116104379));
#37591=CARTESIAN_POINT('Ctrl Pts',(-4.25533045233313,-0.794772684000851,
7.70324620363229));
#37592=CARTESIAN_POINT('Ctrl Pts',(-4.20084799529369,-0.636309800095196,
7.7096965632967));
#37593=CARTESIAN_POINT('Ctrl Pts',(-4.1264371815048,-0.319434907277159,
7.724865141945));
#37594=CARTESIAN_POINT('Ctrl Pts',(-4.1083738762426,-0.158333333333332,
7.73455031738055));
#37595=CARTESIAN_POINT('Ctrl Pts',(-4.10569625638313,0.158333333333334,
7.7548751533632));
#37596=CARTESIAN_POINT('Ctrl Pts',(-4.12120905306814,0.319434907277167,
7.76438231270788));
#37597=CARTESIAN_POINT('Ctrl Pts',(-4.18990683146856,0.636309800095206,
7.792920784926));
#37598=CARTESIAN_POINT('Ctrl Pts',(-4.24157890048061,0.79477268400084,7.80842294468366));
#37599=CARTESIAN_POINT('Ctrl Pts',(-4.37480433638243,1.06847604194511,7.84815479663222));
#37600=CARTESIAN_POINT('Ctrl Pts',(-4.44499154163404,1.18514270861178,7.86827306771212));
#37601=CARTESIAN_POINT('Ctrl Pts',(-4.52769759742429,1.3,7.89131116337361));
#37602=CARTESIAN_POINT('Ctrl Pts',(-4.559720379007,-1.3,7.61849776759047));
#37603=CARTESIAN_POINT('Ctrl Pts',(-4.47399349175896,-1.18514270861178,
7.62037245698057));
#37604=CARTESIAN_POINT('Ctrl Pts',(-4.40104080402149,-1.06847604194512,
7.62304807647726));
#37605=CARTESIAN_POINT('Ctrl Pts',(-4.26201645755201,-0.794772684000851,
7.63107960154223));
#37606=CARTESIAN_POINT('Ctrl Pts',(-4.20777282266716,-0.636309800095196,
7.63685323236411));
#37607=CARTESIAN_POINT('Ctrl Pts',(-4.13378893043113,-0.319434907277159,
7.65150954041835));
#37608=CARTESIAN_POINT('Ctrl Pts',(-4.11602990877888,-0.158333333333332,
7.65999102848028));
#37609=CARTESIAN_POINT('Ctrl Pts',(-4.11370927434805,0.158333333333334,
7.68035338514341));
#37610=CARTESIAN_POINT('Ctrl Pts',(-4.12926944463902,0.319434907277167,
7.69110119252446));
#37611=CARTESIAN_POINT('Ctrl Pts',(-4.19827830828669,0.636309800095206,
7.72022950297699));
#37612=CARTESIAN_POINT('Ctrl Pts',(-4.25004328077839,0.79477268400084,7.73644325734629));
#37613=CARTESIAN_POINT('Ctrl Pts',(-4.38381424022261,1.06847604194511,7.77468958527649));
#37614=CARTESIAN_POINT('Ctrl Pts',(-4.45430894480039,1.18514270861178,7.79364115454063));
#37615=CARTESIAN_POINT('Ctrl Pts',(-4.53739386231511,1.3,7.81498887487403));
#37616=CARTESIAN_POINT('Ctrl Pts',(-4.56610429681699,-1.3,7.54182733738403));
#37617=CARTESIAN_POINT('Ctrl Pts',(-4.48039654346318,-1.18514270861178,
7.54543423312735));
#37618=CARTESIAN_POINT('Ctrl Pts',(-4.40750206450663,-1.06847604194512,
7.54931499191074));
#37619=CARTESIAN_POINT('Ctrl Pts',(-4.26870246277088,-0.794772684000851,
7.55891299945218));
#37620=CARTESIAN_POINT('Ctrl Pts',(-4.21469765004064,-0.636309800095196,
7.56400990143152));
#37621=CARTESIAN_POINT('Ctrl Pts',(-4.14114067935745,-0.319434907277159,
7.57815393889169));
#37622=CARTESIAN_POINT('Ctrl Pts',(-4.12368594131515,-0.158333333333332,
7.58543173958001));
#37623=CARTESIAN_POINT('Ctrl Pts',(-4.12172229231298,0.158333333333334,
7.60583161692362));
#37624=CARTESIAN_POINT('Ctrl Pts',(-4.1373298362099,0.319434907277167,7.61782007234104));
#37625=CARTESIAN_POINT('Ctrl Pts',(-4.20664978510482,0.636309800095206,
7.64753822102798));
#37626=CARTESIAN_POINT('Ctrl Pts',(-4.25850766107617,0.79477268400084,7.66446357000892));
#37627=CARTESIAN_POINT('Ctrl Pts',(-4.39282414406279,1.06847604194511,7.70122437392077));
#37628=CARTESIAN_POINT('Ctrl Pts',(-4.46362634796674,1.18514270861178,7.71900924136913));
#37629=CARTESIAN_POINT('Ctrl Pts',(-4.54709012720593,1.3,7.73866658637446));
#37630=CARTESIAN_POINT('Ctrl Pts',(-4.57248821462698,-1.3,7.46515690717759));
#37631=CARTESIAN_POINT('Ctrl Pts',(-4.48679959516739,-1.18514270861178,
7.47049600927413));
#37632=CARTESIAN_POINT('Ctrl Pts',(-4.41396332499176,-1.06847604194512,
7.47558190734421));
#37633=CARTESIAN_POINT('Ctrl Pts',(-4.27538846798975,-0.794772684000851,
7.48674639736213));
#37634=CARTESIAN_POINT('Ctrl Pts',(-4.22162247741411,-0.636309800095196,
7.49116657049893));
#37635=CARTESIAN_POINT('Ctrl Pts',(-4.14849242828377,-0.319434907277159,
7.50479833736504));
#37636=CARTESIAN_POINT('Ctrl Pts',(-4.13134197385143,-0.158333333333332,
7.51087245067974));
#37637=CARTESIAN_POINT('Ctrl Pts',(-4.12973531027791,0.158333333333334,
7.53130984870382));
#37638=CARTESIAN_POINT('Ctrl Pts',(-4.14539022778078,0.319434907277167,
7.54453895215762));
#37639=CARTESIAN_POINT('Ctrl Pts',(-4.21502126192296,0.636309800095206,
7.57484693907897));
#37640=CARTESIAN_POINT('Ctrl Pts',(-4.26697204137396,0.79477268400084,7.59248388267156));
#37641=CARTESIAN_POINT('Ctrl Pts',(-4.40183404790297,1.06847604194511,7.62775916256504));
#37642=CARTESIAN_POINT('Ctrl Pts',(-4.47294375113309,1.18514270861178,7.64437732819764));
#37643=CARTESIAN_POINT('Ctrl Pts',(-4.55678639209675,1.3,7.66234429787488));
#37644=CARTESIAN_POINT('Ctrl Pts',(-4.57248821462698,-1.3,7.4651569071776));
#37645=CARTESIAN_POINT('Ctrl Pts',(-4.48679959516739,-1.18514270861178,
7.47049600927413));
#37646=CARTESIAN_POINT('Ctrl Pts',(-4.41396332499177,-1.06847604194512,
7.47558190734422));
#37647=CARTESIAN_POINT('Ctrl Pts',(-4.27538846798975,-0.794772684000851,
7.48674639736213));
#37648=CARTESIAN_POINT('Ctrl Pts',(-4.22162247741411,-0.636309800095197,
7.49116657049893));
#37649=CARTESIAN_POINT('Ctrl Pts',(-4.14849242828377,-0.319434907277159,
7.50479833736504));
#37650=CARTESIAN_POINT('Ctrl Pts',(-4.13134197385143,-0.158333333333332,
7.51087245067974));
#37651=CARTESIAN_POINT('Ctrl Pts',(-4.12973531027791,0.158333333333334,
7.53130984870382));
#37652=CARTESIAN_POINT('Ctrl Pts',(-4.14539022778078,0.319434907277167,
7.54453895215762));
#37653=CARTESIAN_POINT('Ctrl Pts',(-4.21502126192295,0.636309800095206,
7.57484693907897));
#37654=CARTESIAN_POINT('Ctrl Pts',(-4.26697204137395,0.79477268400084,7.59248388267156));
#37655=CARTESIAN_POINT('Ctrl Pts',(-4.40183404790297,1.06847604194511,7.62775916256504));
#37656=CARTESIAN_POINT('Ctrl Pts',(-4.47294375113309,1.18514270861178,7.64437732819763));
#37657=CARTESIAN_POINT('Ctrl Pts',(-4.55678639209675,1.3,7.66234429787488));
#37658=CARTESIAN_POINT('Ctrl Pts',(-4.5724882146272,-1.3000000000003,7.46515690717758));
#37659=CARTESIAN_POINT('Ctrl Pts',(-4.48679959516751,-1.18514270861198,
7.47049600927413));
#37660=CARTESIAN_POINT('Ctrl Pts',(-4.41396332499182,-1.06847604194522,
7.47558190734421));
#37661=CARTESIAN_POINT('Ctrl Pts',(-4.27538846798975,-0.794772684000851,
7.48674639736213));
#37662=CARTESIAN_POINT('Ctrl Pts',(-4.22162247741412,-0.636309800095197,
7.49116657049894));
#37663=CARTESIAN_POINT('Ctrl Pts',(-4.14849242828378,-0.319434907277159,
7.50479833736504));
#37664=CARTESIAN_POINT('Ctrl Pts',(-4.13134197385143,-0.158333333333332,
7.51087245067974));
#37665=CARTESIAN_POINT('Ctrl Pts',(-4.12973531027791,0.158333333333334,
7.53130984870382));
#37666=CARTESIAN_POINT('Ctrl Pts',(-4.14539022778078,0.319434907277167,
7.54453895215762));
#37667=CARTESIAN_POINT('Ctrl Pts',(-4.21502126192296,0.636309800095206,
7.57484693907897));
#37668=CARTESIAN_POINT('Ctrl Pts',(-4.26697204137396,0.79477268400084,7.59248388267156));
#37669=CARTESIAN_POINT('Ctrl Pts',(-4.40183404790331,1.06847604194578,7.62775916256513));
#37670=CARTESIAN_POINT('Ctrl Pts',(-4.47294375113389,1.1851427086131,7.64437732819782));
#37671=CARTESIAN_POINT('Ctrl Pts',(-4.55678639209818,1.30000000000195,7.66234429787519));
#37672=CARTESIAN_POINT('Ctrl Pts',(-4.57985658845494,-1.3000000000003,7.46043462252666));
#37673=CARTESIAN_POINT('Ctrl Pts',(-4.49399758634183,-1.18514270861198,
7.46643805441031));
#37674=CARTESIAN_POINT('Ctrl Pts',(-4.42096106045728,-1.06847604194522,
7.47158857881112));
#37675=CARTESIAN_POINT('Ctrl Pts',(-4.28185455997266,-0.794772684000851,
7.48151693362695));
#37676=CARTESIAN_POINT('Ctrl Pts',(-4.22749554624361,-0.636309800095197,
7.48233642792713));
#37677=CARTESIAN_POINT('Ctrl Pts',(-4.1540436348186,-0.319434907277159,
7.49422021701903));
#37678=CARTESIAN_POINT('Ctrl Pts',(-4.13706908978531,-0.158333333333332,
7.50081062857585));
#37679=CARTESIAN_POINT('Ctrl Pts',(-4.13553292450502,0.158333333333334,
7.52147411751504));
#37680=CARTESIAN_POINT('Ctrl Pts',(-4.1511379029416,0.319434907277167,7.53468752939477));
#37681=CARTESIAN_POINT('Ctrl Pts',(-4.2211214067753,0.636309800095206,7.56664485618235));
#37682=CARTESIAN_POINT('Ctrl Pts',(-4.27351162156741,0.79477268400084,7.58680963674882));
#37683=CARTESIAN_POINT('Ctrl Pts',(-4.40891552697358,1.06847604194578,7.62347431551885));
#37684=CARTESIAN_POINT('Ctrl Pts',(-4.48025898194793,1.1851427086131,7.64034602806548));
#37685=CARTESIAN_POINT('Ctrl Pts',(-4.56433455845528,1.30000000000195,7.65821867227938));
#37686=CARTESIAN_POINT('Ctrl Pts',(-4.59168342474784,-1.3000000000003,7.45718163914688));
#37687=CARTESIAN_POINT('Ctrl Pts',(-4.50842397388543,-1.18514270861199,
7.46447754241301));
#37688=CARTESIAN_POINT('Ctrl Pts',(-4.43718225163949,-1.06847604194522,
7.46993969508268));
#37689=CARTESIAN_POINT('Ctrl Pts',(-4.30036297863612,-0.794772684000854,
7.47832202973116));
#37690=CARTESIAN_POINT('Ctrl Pts',(-4.24470116695618,-0.636309800095197,
7.47377977131766));
#37691=CARTESIAN_POINT('Ctrl Pts',(-4.17076364579087,-0.319434907277159,
7.48282880263746));
#37692=CARTESIAN_POINT('Ctrl Pts',(-4.15283946666577,-0.158333333333333,
7.48967182383003));
#37693=CARTESIAN_POINT('Ctrl Pts',(-4.15133977222458,0.158333333333335,
7.51049912633798));
#37694=CARTESIAN_POINT('Ctrl Pts',(-4.16799329782777,0.319434907277169,
7.52348646991815));
#37695=CARTESIAN_POINT('Ctrl Pts',(-4.23840950953686,0.636309800095208,
7.55889184457618));
#37696=CARTESIAN_POINT('Ctrl Pts',(-4.29184104268107,0.794772684000841,
7.58552360736601));
#37697=CARTESIAN_POINT('Ctrl Pts',(-4.42496865500282,1.06847604194578,7.62366725460812));
#37698=CARTESIAN_POINT('Ctrl Pts',(-4.49458045110704,1.1851427086131,7.63990830968531));
#37699=CARTESIAN_POINT('Ctrl Pts',(-4.57617803280542,1.30000000000195,7.65587944830994));
#37700=CARTESIAN_POINT('Ctrl Pts',(-4.60901429870398,-1.3000000000003,7.45223840664109));
#37701=CARTESIAN_POINT('Ctrl Pts',(-4.5294315556627,-1.18514270861199,7.45959212322105));
#37702=CARTESIAN_POINT('Ctrl Pts',(-4.46089813449078,-1.06847604194522,
7.46488779903224));
#37703=CARTESIAN_POINT('Ctrl Pts',(-4.32809836544721,-0.794772684000851,
7.4723673836669));
#37704=CARTESIAN_POINT('Ctrl Pts',(-4.27192130062999,-0.636309800095196,
7.46631175328514));
#37705=CARTESIAN_POINT('Ctrl Pts',(-4.19815527265973,-0.319434907277159,
7.47405317109067));
#37706=CARTESIAN_POINT('Ctrl Pts',(-4.17893181023939,-0.158333333333332,
7.48021929441616));
#37707=CARTESIAN_POINT('Ctrl Pts',(-4.17741037262064,0.158333333333334,
7.50112354255511));
#37708=CARTESIAN_POINT('Ctrl Pts',(-4.19532546267363,0.319434907277167,
7.51451242989938));
#37709=CARTESIAN_POINT('Ctrl Pts',(-4.26555843318573,0.636309800095207,
7.55209975997349));
#37710=CARTESIAN_POINT('Ctrl Pts',(-4.31951500434467,0.794772684000839,
7.58217353749801));
#37711=CARTESIAN_POINT('Ctrl Pts',(-4.44867563298358,1.06847604194578,7.62139264277946));
#37712=CARTESIAN_POINT('Ctrl Pts',(-4.51561269110254,1.1851427086131,7.63745204139131));
#37713=CARTESIAN_POINT('Ctrl Pts',(-4.59357795707547,1.30000000000195,7.65259434114969));
#37714=CARTESIAN_POINT('Ctrl Pts',(-4.62334264925501,-1.3000000000003,7.44788165467971));
#37715=CARTESIAN_POINT('Ctrl Pts',(-4.54648329086464,-1.18514270861199,
7.45486630178287));
#37716=CARTESIAN_POINT('Ctrl Pts',(-4.47993360321558,-1.06847604194522,
7.46004142012346));
#37717=CARTESIAN_POINT('Ctrl Pts',(-4.35000791338186,-0.794772684000852,
7.4678166053326));
#37718=CARTESIAN_POINT('Ctrl Pts',(-4.29327346583404,-0.636309800095197,
7.46345145619193));
#37719=CARTESIAN_POINT('Ctrl Pts',(-4.21952367814165,-0.319434907277158,
7.47104479061018));
#37720=CARTESIAN_POINT('Ctrl Pts',(-4.1993445185557,-0.158333333333332,
7.47546103682555));
#37721=CARTESIAN_POINT('Ctrl Pts',(-4.19780196954188,0.158333333333334,
7.4958375256331));
#37722=CARTESIAN_POINT('Ctrl Pts',(-4.21663888113668,0.319434907277167,
7.50960329513933));
#37723=CARTESIAN_POINT('Ctrl Pts',(-4.2868386087941,0.636309800095206,7.5479853849349));
#37724=CARTESIAN_POINT('Ctrl Pts',(-4.34135241776995,0.794772684000839,
7.57948276964698));
#37725=CARTESIAN_POINT('Ctrl Pts',(-4.46768129760591,1.06847604194578,7.61888367845877));
#37726=CARTESIAN_POINT('Ctrl Pts',(-4.53266397770261,1.1851427086131,7.63470681844777));
#37727=CARTESIAN_POINT('Ctrl Pts',(-4.60794624676118,1.30000000000195,7.64929790494865));
#37728=CARTESIAN_POINT('Ctrl Pts',(-4.63777744145311,-1.3000000000003,7.44317884815643));
#37729=CARTESIAN_POINT('Ctrl Pts',(-4.56391391198511,-1.18514270861199,
7.44976250583294));
#37730=CARTESIAN_POINT('Ctrl Pts',(-4.49956220640914,-1.06847604194522,
7.4548250227973));
#37731=CARTESIAN_POINT('Ctrl Pts',(-4.37287110903858,-0.794772684000854,
7.46300631038979));
#37732=CARTESIAN_POINT('Ctrl Pts',(-4.31564116562494,-0.6363098000952,7.46034801937047));
#37733=CARTESIAN_POINT('Ctrl Pts',(-4.24200059940824,-0.31943490727716,
7.46841071460317));
#37734=CARTESIAN_POINT('Ctrl Pts',(-4.22080120062564,-0.158333333333333,
7.47153692196261));
#37735=CARTESIAN_POINT('Ctrl Pts',(-4.21922987515411,0.158333333333335,
7.49270076255547));
#37736=CARTESIAN_POINT('Ctrl Pts',(-4.23903267766996,0.319434907277168,
7.50897530883289));
#37737=CARTESIAN_POINT('Ctrl Pts',(-4.30911665623112,0.636309800095208,
7.54761311422366));
#37738=CARTESIAN_POINT('Ctrl Pts',(-4.36416991095692,0.794772684000843,
7.57699568476728));
#37739=CARTESIAN_POINT('Ctrl Pts',(-4.48732042833463,1.06847604194579,7.6155579202634));
#37740=CARTESIAN_POINT('Ctrl Pts',(-4.55013396214836,1.1851427086131,7.63121868568088));
#37741=CARTESIAN_POINT('Ctrl Pts',(-4.62245373397926,1.30000000000196,7.64584805364117));
#37742=CARTESIAN_POINT('Ctrl Pts',(-4.64917211308598,-1.30000000000031,
7.43850439917717));
#37743=CARTESIAN_POINT('Ctrl Pts',(-4.57756288722408,-1.18514270861199,
7.4447173982654));
#37744=CARTESIAN_POINT('Ctrl Pts',(-4.51486638728743,-1.06847604194522,
7.44971239799422));
#37745=CARTESIAN_POINT('Ctrl Pts',(-4.39061510991401,-0.794772684000856,
7.45843802443385));
#37746=CARTESIAN_POINT('Ctrl Pts',(-4.33301937306072,-0.6363098000952,7.45730186698481));
#37747=CARTESIAN_POINT('Ctrl Pts',(-4.25947297944506,-0.31943490727716,
7.4666540550818));
#37748=CARTESIAN_POINT('Ctrl Pts',(-4.23752467864517,-0.158333333333333,
7.47022849234999));
#37749=CARTESIAN_POINT('Ctrl Pts',(-4.23592101691603,0.158333333333335,
7.49206462085004));
#37750=CARTESIAN_POINT('Ctrl Pts',(-4.25640297863503,0.319434907277167,
7.50890472369068));
#37751=CARTESIAN_POINT('Ctrl Pts',(-4.32640311242899,0.636309800095208,
7.54692683029001));
#37752=CARTESIAN_POINT('Ctrl Pts',(-4.38190950729608,0.794772684000843,
7.57433453652904));
#37753=CARTESIAN_POINT('Ctrl Pts',(-4.50269748611023,1.06847604194578,7.61241799452743));
#37754=CARTESIAN_POINT('Ctrl Pts',(-4.56388830615953,1.1851427086131,7.62821040288113));
#37755=CARTESIAN_POINT('Ctrl Pts',(-4.63398530586503,1.30000000000196,7.64331030175218));
#37756=CARTESIAN_POINT('Ctrl Pts',(-4.6606296739892,-1.30000000000031,7.43416986317279));
#37757=CARTESIAN_POINT('Ctrl Pts',(-4.5913570163761,-1.18514270861199,7.44023858076217));
#37758=CARTESIAN_POINT('Ctrl Pts',(-4.53037198922488,-1.06847604194522,
7.44527262176997));
#37759=CARTESIAN_POINT('Ctrl Pts',(-4.40863046079444,-0.794772684000856,
7.45451195366465));
#37760=CARTESIAN_POINT('Ctrl Pts',(-4.3506248344246,-0.636309800095199,
7.45437946766052));
#37761=CARTESIAN_POINT('Ctrl Pts',(-4.27715204799888,-0.319434907277159,
7.46475922721751));
#37762=CARTESIAN_POINT('Ctrl Pts',(-4.254410018565,-0.158333333333333,7.46907130623477));
#37763=CARTESIAN_POINT('Ctrl Pts',(-4.25279259453082,0.158333333333335,
7.49098722395584));
#37764=CARTESIAN_POINT('Ctrl Pts',(-4.27404173721797,0.319434907277167,
7.50699230592871));
#37765=CARTESIAN_POINT('Ctrl Pts',(-4.34396627385687,0.636309800095207,
7.54451024511768));
#37766=CARTESIAN_POINT('Ctrl Pts',(-4.39989096848589,0.794772684000842,
7.57188784901723));
#37767=CARTESIAN_POINT('Ctrl Pts',(-4.5182235149054,1.06847604194578,7.60968824867482));
#37768=CARTESIAN_POINT('Ctrl Pts',(-4.57773690077526,1.1851427086131,7.62535146933581));
#37769=CARTESIAN_POINT('Ctrl Pts',(-4.6455418978228,1.30000000000196,7.64031551828881));
#37770=CARTESIAN_POINT('Ctrl Pts',(-4.68072279072018,-1.30000000000031,
7.42759731688899));
#37771=CARTESIAN_POINT('Ctrl Pts',(-4.61541911481721,-1.18514270861199,
7.43260381853245));
#37772=CARTESIAN_POINT('Ctrl Pts',(-4.557348277575,-1.06847604194523,7.43712245705713));
#37773=CARTESIAN_POINT('Ctrl Pts',(-4.43990233074511,-0.794772684000857,
7.44643435459863));
#37774=CARTESIAN_POINT('Ctrl Pts',(-4.38125332982614,-0.636309800095201,
7.44835440903243));
#37775=CARTESIAN_POINT('Ctrl Pts',(-4.30794495913783,-0.319434907277161,
7.46039562465073));
#37776=CARTESIAN_POINT('Ctrl Pts',(-4.28386650027582,-0.158333333333333,
7.4654873767949));
#37777=CARTESIAN_POINT('Ctrl Pts',(-4.28222139972213,0.158333333333335,
7.48835864464172));
#37778=CARTESIAN_POINT('Ctrl Pts',(-4.30474728282048,0.319434907277169,
7.50515701844512));
#37779=CARTESIAN_POINT('Ctrl Pts',(-4.37451623579684,0.63630980009521,7.54170144404907));
#37780=CARTESIAN_POINT('Ctrl Pts',(-4.43116658239244,0.794772684000845,
7.56616428453284));
#37781=CARTESIAN_POINT('Ctrl Pts',(-4.54525640247321,1.06847604194579,7.60313466934228));
#37782=CARTESIAN_POINT('Ctrl Pts',(-4.60187326939733,1.1851427086131,7.61891801345069));
#37783=CARTESIAN_POINT('Ctrl Pts',(-4.66572174757695,1.30000000000196,7.63448159197121));
#37784=CARTESIAN_POINT('Ctrl Pts',(-4.72058200346455,-1.30000000000031,
7.41055955717715));
#37785=CARTESIAN_POINT('Ctrl Pts',(-4.66328542491091,-1.18514270861199,
7.41376769125186));
#37786=CARTESIAN_POINT('Ctrl Pts',(-4.61110369976158,-1.06847604194523,
7.41757424322289));
#37787=CARTESIAN_POINT('Ctrl Pts',(-4.50236981033514,-0.794772684000858,
7.42775060482769));
#37788=CARTESIAN_POINT('Ctrl Pts',(-4.44249347992462,-0.636309800095199,
7.43416823300931));
#37789=CARTESIAN_POINT('Ctrl Pts',(-4.36958159441681,-0.319434907277159,
7.4502898228441));
#37790=CARTESIAN_POINT('Ctrl Pts',(-4.3428278760223,-0.158333333333332,
7.4582033613571));
#37791=CARTESIAN_POINT('Ctrl Pts',(-4.34115514161927,0.158333333333334,
7.48189348506881));
#37792=CARTESIAN_POINT('Ctrl Pts',(-4.36625935696994,0.319434907277166,
7.49638018296511));
#37793=CARTESIAN_POINT('Ctrl Pts',(-4.43571668233373,0.636309800095206,
7.53114107694557));
#37794=CARTESIAN_POINT('Ctrl Pts',(-4.4937939437635,0.794772684000839,7.55400281128164));
#37795=CARTESIAN_POINT('Ctrl Pts',(-4.59936624074172,1.06847604194579,7.59088089537082));
#37796=CARTESIAN_POINT('Ctrl Pts',(-4.65017390543712,1.18514270861311,7.60709116052329));
#37797=CARTESIAN_POINT('Ctrl Pts',(-4.70609089930505,1.30000000000197,7.62354853469364));
#37798=CARTESIAN_POINT('Ctrl Pts',(-4.75619240536058,-1.30000000000032,
7.39667294505808));
#37799=CARTESIAN_POINT('Ctrl Pts',(-4.70590917649517,-1.18514270861201,
7.39755866929844));
#37800=CARTESIAN_POINT('Ctrl Pts',(-4.65888186664025,-1.06847604194524,
7.39990867579963));
#37801=CARTESIAN_POINT('Ctrl Pts',(-4.55776119735292,-0.79477268400087,
7.40872044588576));
#37802=CARTESIAN_POINT('Ctrl Pts',(-4.49674677444273,-0.636309800095208,
7.41685452571745));
#37803=CARTESIAN_POINT('Ctrl Pts',(-4.42422834751872,-0.319434907277163,
7.4353232018333));
#37804=CARTESIAN_POINT('Ctrl Pts',(-4.39525391132892,-0.158333333333335,
7.4460826510108));
#37805=CARTESIAN_POINT('Ctrl Pts',(-4.39362598481891,0.158333333333337,
7.47138174563145));
#37806=CARTESIAN_POINT('Ctrl Pts',(-4.4209867281482,0.319434907277172,7.48549553851834));
#37807=CARTESIAN_POINT('Ctrl Pts',(-4.49016019306676,0.636309800095216,
7.51942672754422));
#37808=CARTESIAN_POINT('Ctrl Pts',(-4.54948882348156,0.794772684000852,
7.53987197370938));
#37809=CARTESIAN_POINT('Ctrl Pts',(-4.64749609348585,1.0684760419458,7.57715869939665));
#37810=CARTESIAN_POINT('Ctrl Pts',(-4.69314798885547,1.18514270861312,7.59418710374468));
#37811=CARTESIAN_POINT('Ctrl Pts',(-4.742028063937,1.30000000000198,7.61210387050001));
#37812=CARTESIAN_POINT('Ctrl Pts',(-4.78159245634849,-1.30000000000032,
7.38452953948181));
#37813=CARTESIAN_POINT('Ctrl Pts',(-4.73640400144256,-1.18514270861201,
7.38403131096895));
#37814=CARTESIAN_POINT('Ctrl Pts',(-4.69312438118273,-1.06847604194524,
7.38559077565983));
#37815=CARTESIAN_POINT('Ctrl Pts',(-4.59754959021777,-0.794772684000866,
7.39394713400638));
#37816=CARTESIAN_POINT('Ctrl Pts',(-4.53574283459765,-0.636309800095209,
7.40389616287617));
#37817=CARTESIAN_POINT('Ctrl Pts',(-4.46351035596197,-0.319434907277165,
7.4237879980083));
#37818=CARTESIAN_POINT('Ctrl Pts',(-4.43288546941762,-0.158333333333335,
7.43553357003229));
#37819=CARTESIAN_POINT('Ctrl Pts',(-4.43128483385098,0.158333333333337,
7.46145478870264));
#37820=CARTESIAN_POINT('Ctrl Pts',(-4.46030592709637,0.319434907277171,
7.47529081311309));
#37821=CARTESIAN_POINT('Ctrl Pts',(-4.52928445840577,0.636309800095217,
7.5088904200637));
#37822=CARTESIAN_POINT('Ctrl Pts',(-4.58948824265808,0.794772684000855,
7.52806622772443));
#37823=CARTESIAN_POINT('Ctrl Pts',(-4.682065906496,1.0684760419458,7.56631566101118));
#37824=CARTESIAN_POINT('Ctrl Pts',(-4.72402097248571,1.18514270861312,7.58425210078832));
#37825=CARTESIAN_POINT('Ctrl Pts',(-4.76785766413012,1.30000000000198,7.6035682179539));
#37826=CARTESIAN_POINT('Ctrl Pts',(-4.78724263544867,-1.30000000000032,
7.38189848275631));
#37827=CARTESIAN_POINT('Ctrl Pts',(-4.74317456636349,-1.185142708612,7.38098582392651));
#37828=CARTESIAN_POINT('Ctrl Pts',(-4.70071991070143,-1.06847604194524,
7.38229294656453));
#37829=CARTESIAN_POINT('Ctrl Pts',(-4.60636847086696,-0.794772684000865,
7.39044080060378));
#37830=CARTESIAN_POINT('Ctrl Pts',(-4.54439171706508,-0.636309800095209,
7.40079181135806));
#37831=CARTESIAN_POINT('Ctrl Pts',(-4.4722304122187,-0.319434907277165,
7.42106915937384));
#37832=CARTESIAN_POINT('Ctrl Pts',(-4.44125148812159,-0.158333333333335,
7.43321918233995));
#37833=CARTESIAN_POINT('Ctrl Pts',(-4.43965915366256,0.158333333333337,
7.45929086929445));
#37834=CARTESIAN_POINT('Ctrl Pts',(-4.46904138652334,0.319434907277172,
7.47294053951429));
#37835=CARTESIAN_POINT('Ctrl Pts',(-4.53796809517026,0.636309800095217,
7.50632337232342));
#37836=CARTESIAN_POINT('Ctrl Pts',(-4.59835652138401,0.794772684000854,
7.52505510834564));
#37837=CARTESIAN_POINT('Ctrl Pts',(-4.68972657257818,1.0684760419458,7.56350553669529));
#37838=CARTESIAN_POINT('Ctrl Pts',(-4.73086219664383,1.18514270861312,7.58168090727336));
#37839=CARTESIAN_POINT('Ctrl Pts',(-4.77358273520712,1.30000000000198,7.60138788272565));
#37840=CARTESIAN_POINT('Ctrl Pts',(-4.79573463031585,-1.30000000000032,
7.37812243727755));
#37841=CARTESIAN_POINT('Ctrl Pts',(-4.75332696102845,-1.18514270861201,
7.3764183801566));
#37842=CARTESIAN_POINT('Ctrl Pts',(-4.71209659401335,-1.06847604194524,
7.37723615010075));
#37843=CARTESIAN_POINT('Ctrl Pts',(-4.61956600186943,-0.794772684000868,
7.38495128727626));
#37844=CARTESIAN_POINT('Ctrl Pts',(-4.55735067689832,-0.636309800095211,
7.39603127227243));
#37845=CARTESIAN_POINT('Ctrl Pts',(-4.48530329615657,-0.319434907277166,
7.41696807003476));
#37846=CARTESIAN_POINT('Ctrl Pts',(-4.45379954175104,-0.158333333333336,
7.42983981676956));
#37847=CARTESIAN_POINT('Ctrl Pts',(-4.45221924396623,0.158333333333337,
7.4561124445076));
#37848=CARTESIAN_POINT('Ctrl Pts',(-4.4821330754945,0.319434907277172,7.46929534312405));
#37849=CARTESIAN_POINT('Ctrl Pts',(-4.55098110905412,0.636309800095218,
7.50231801079879));
#37850=CARTESIAN_POINT('Ctrl Pts',(-4.61165683769535,0.794772684000857,
7.52057094572087));
#37851=CARTESIAN_POINT('Ctrl Pts',(-4.70121335968738,1.0684760419458,7.55924305725064));
#37852=CARTESIAN_POINT('Ctrl Pts',(-4.74111652794842,1.18514270861312,7.57769178830973));
#37853=CARTESIAN_POINT('Ctrl Pts',(-4.78215716449621,1.30000000000198,7.5978495262896));
#37854=CARTESIAN_POINT('Ctrl Pts',(-4.80424392564089,-1.30000000000032,
7.37453487689565));
#37855=CARTESIAN_POINT('Ctrl Pts',(-4.7634901105747,-1.18514270861201,7.37200723460166));
#37856=CARTESIAN_POINT('Ctrl Pts',(-4.72347848273184,-1.06847604194524,
7.37230262570058));
#37857=CARTESIAN_POINT('Ctrl Pts',(-4.6327582190761,-0.794772684000867,
7.3795068101154));
#37858=CARTESIAN_POINT('Ctrl Pts',(-4.57029597217174,-0.636309800095211,
7.39121525105204));
#37859=CARTESIAN_POINT('Ctrl Pts',(-4.49836555817877,-0.319434907277166,
7.41282614349591));
#37860=CARTESIAN_POINT('Ctrl Pts',(-4.46634941917561,-0.158333333333335,
7.42649666961214));
#37861=CARTESIAN_POINT('Ctrl Pts',(-4.4647946338716,0.158333333333337,7.45314212589848));
#37862=CARTESIAN_POINT('Ctrl Pts',(-4.49524481309089,0.319434907277172,
7.46597526879084));
#37863=CARTESIAN_POINT('Ctrl Pts',(-4.56403100297875,0.636309800095218,
7.49892806274145));
#37864=CARTESIAN_POINT('Ctrl Pts',(-4.62501250401097,0.794772684000857,
7.51697123685178));
#37865=CARTESIAN_POINT('Ctrl Pts',(-4.71276269964325,1.0684760419458,7.55606737412409));
#37866=CARTESIAN_POINT('Ctrl Pts',(-4.75143286611581,1.18514270861312,7.5748406813716));
#37867=CARTESIAN_POINT('Ctrl Pts',(-4.79078939083679,1.30000000000198,7.59546402669605));
#37868=CARTESIAN_POINT('Ctrl Pts',(-4.82116392366532,-1.30000000000033,
7.36648906419669));
#37869=CARTESIAN_POINT('Ctrl Pts',(-4.78379435131418,-1.18514270861201,
7.36295501392018));
#37870=CARTESIAN_POINT('Ctrl Pts',(-4.74627296491281,-1.06847604194524,
7.36265612615519));
#37871=CARTESIAN_POINT('Ctrl Pts',(-4.65924033537166,-0.794772684000869,
7.36943950821944));
#37872=CARTESIAN_POINT('Ctrl Pts',(-4.59626304788614,-0.636309800095212,
7.38238506314081));
#37873=CARTESIAN_POINT('Ctrl Pts',(-4.52451696391414,-0.319434907277167,
7.40479741221343));
#37874=CARTESIAN_POINT('Ctrl Pts',(-4.49139649387496,-0.158333333333336,
7.41909656029638));
#37875=CARTESIAN_POINT('Ctrl Pts',(-4.48982928135806,0.158333333333338,
7.44571920738321));
#37876=CARTESIAN_POINT('Ctrl Pts',(-4.52133173317534,0.319434907277174,
7.45760023335444));
#37877=CARTESIAN_POINT('Ctrl Pts',(-4.58998900565639,0.636309800095222,
7.49031758521192));
#37878=CARTESIAN_POINT('Ctrl Pts',(-4.65161473512541,0.79477268400086,7.50833480079011));
#37879=CARTESIAN_POINT('Ctrl Pts',(-4.73577439163365,1.06847604194581,7.54844247985107));
#37880=CARTESIAN_POINT('Ctrl Pts',(-4.77198716776143,1.18514270861313,7.56790475507659));
#37881=CARTESIAN_POINT('Ctrl Pts',(-4.80798312313707,1.30000000000198,7.58946817739808));
#37882=CARTESIAN_POINT('Ctrl Pts',(-4.84216943247133,-1.30000000000034,
7.35556326655833));
#37883=CARTESIAN_POINT('Ctrl Pts',(-4.8088626711365,-1.18514270861203,7.34958957289585));
#37884=CARTESIAN_POINT('Ctrl Pts',(-4.77434749389395,-1.06847604194526,
7.34775870979043));
#37885=CARTESIAN_POINT('Ctrl Pts',(-4.69181884723649,-0.794772684000882,
7.35309981711123));
#37886=CARTESIAN_POINT('Ctrl Pts',(-4.62831370858818,-0.63630980009522,
7.36800584919602));
#37887=CARTESIAN_POINT('Ctrl Pts',(-4.55695114658674,-0.31943490727717,
7.39253573421515));
#37888=CARTESIAN_POINT('Ctrl Pts',(-4.52260959946483,-0.158333333333338,
7.40901668765982));
#37889=CARTESIAN_POINT('Ctrl Pts',(-4.52119448799517,0.15833333333334,7.43731905635201));
#37890=CARTESIAN_POINT('Ctrl Pts',(-4.55412793237604,0.31943490727718,7.44965249956768));
#37891=CARTESIAN_POINT('Ctrl Pts',(-4.62259373792968,0.63630980009523,7.48172953763251));
#37892=CARTESIAN_POINT('Ctrl Pts',(-4.68477221076676,0.794772684000869,
7.49662215096969));
#37893=CARTESIAN_POINT('Ctrl Pts',(-4.76439994582661,1.06847604194582,7.53744782378967));
#37894=CARTESIAN_POINT('Ctrl Pts',(-4.79756444748894,1.18514270861314,7.55804906096945));
#37895=CARTESIAN_POINT('Ctrl Pts',(-4.82942555480448,1.300000000002,7.58157961430544));
#37896=CARTESIAN_POINT('Ctrl Pts',(-4.86471527153658,-1.30000000000035,
7.34509153261728));
#37897=CARTESIAN_POINT('Ctrl Pts',(-4.83589630809817,-1.18514270861203,
7.33769155048644));
#37898=CARTESIAN_POINT('Ctrl Pts',(-4.80466872282125,-1.06847604194526,
7.33485296909692));
#37899=CARTESIAN_POINT('Ctrl Pts',(-4.72696235548441,-0.794772684000882,
7.3388330264484));
#37900=CARTESIAN_POINT('Ctrl Pts',(-4.66262689024078,-0.636309800095225,
7.3539602446291));
#37901=CARTESIAN_POINT('Ctrl Pts',(-4.5914984942633,-0.319434907277175,
7.37925740599487));
#37902=CARTESIAN_POINT('Ctrl Pts',(-4.55583447616005,-0.158333333333339,
7.3977301527819));
#37903=CARTESIAN_POINT('Ctrl Pts',(-4.55442495747738,0.158333333333341,
7.42603311863638));
#37904=CARTESIAN_POINT('Ctrl Pts',(-4.5886487993213,0.31943490727718,7.4360003318052));
#37905=CARTESIAN_POINT('Ctrl Pts',(-4.6569685545072,0.636309800095233,7.46807522688327));
#37906=CARTESIAN_POINT('Ctrl Pts',(-4.72014068304638,0.794772684000876,
7.48454481489632));
#37907=CARTESIAN_POINT('Ctrl Pts',(-4.79503056754589,1.06847604194583,7.52706756803765));
#37908=CARTESIAN_POINT('Ctrl Pts',(-4.82492219359691,1.18514270861315,7.54847119076495));
#37909=CARTESIAN_POINT('Ctrl Pts',(-4.85228838964271,1.30000000000201,7.57287191200792));
#37910=CARTESIAN_POINT('Ctrl Pts',(-4.88704394490281,-1.30000000000036,
7.33321427224023));
#37911=CARTESIAN_POINT('Ctrl Pts',(-4.86253353208781,-1.18514270861205,
7.32318476000548));
#37912=CARTESIAN_POINT('Ctrl Pts',(-4.83449612414015,-1.06847604194527,
7.31868392688339));
#37913=CARTESIAN_POINT('Ctrl Pts',(-4.76157603858742,-0.794772684000892,
7.32105845674154));
#37914=CARTESIAN_POINT('Ctrl Pts',(-4.69671678765166,-0.636309800095229,
7.3384858027196));
#37915=CARTESIAN_POINT('Ctrl Pts',(-4.62596803169993,-0.319434907277175,
7.36547258104057));
#37916=CARTESIAN_POINT('Ctrl Pts',(-4.58893586763949,-0.158333333333341,
7.38531685764692));
#37917=CARTESIAN_POINT('Ctrl Pts',(-4.58765224720057,0.158333333333343,
7.41480981799401));
#37918=CARTESIAN_POINT('Ctrl Pts',(-4.62340111677445,0.319434907277185,
7.42516619984583));
#37919=CARTESIAN_POINT('Ctrl Pts',(-4.69153456637431,0.636309800095241,
7.45681292809196));
#37920=CARTESIAN_POINT('Ctrl Pts',(-4.75533149080953,0.794772684000879,
7.47071865145091));
#37921=CARTESIAN_POINT('Ctrl Pts',(-4.82542784121493,1.06847604194583,7.51433058353202));
#37922=CARTESIAN_POINT('Ctrl Pts',(-4.85208582812171,1.18514270861316,7.53698574062284));
#37923=CARTESIAN_POINT('Ctrl Pts',(-4.87505968917045,1.30000000000202,7.56341806538787));
#37924=CARTESIAN_POINT('Ctrl Pts',(-4.90657768141063,-1.30000000000039,
7.32290090103421));
#37925=CARTESIAN_POINT('Ctrl Pts',(-4.88587644251424,-1.18514270861207,
7.31093727223514));
#37926=CARTESIAN_POINT('Ctrl Pts',(-4.86065279659967,-1.06847604194529,
7.30519616613079));
#37927=CARTESIAN_POINT('Ctrl Pts',(-4.79193346364755,-0.794772684000907,
7.30630833476157));
#37928=CARTESIAN_POINT('Ctrl Pts',(-4.726589320251,-0.636309800095241,7.32552593661041));
#37929=CARTESIAN_POINT('Ctrl Pts',(-4.6560830739072,-0.319434907277181,
7.35320238465496));
#37930=CARTESIAN_POINT('Ctrl Pts',(-4.61775946080383,-0.158333333333344,
7.37345657161974));
#37931=CARTESIAN_POINT('Ctrl Pts',(-4.6164647011132,0.158333333333345,7.40279181157517));
#37932=CARTESIAN_POINT('Ctrl Pts',(-4.65342039867833,0.31943490727719,7.41204353265549));
#37933=CARTESIAN_POINT('Ctrl Pts',(-4.72143832595232,0.636309800095251,
7.44377321758268));
#37934=CARTESIAN_POINT('Ctrl Pts',(-4.78602682992026,0.794772684000895,
7.45807417436264));
#37935=CARTESIAN_POINT('Ctrl Pts',(-4.85202756920001,1.06847604194585,7.50353636787379));
#37936=CARTESIAN_POINT('Ctrl Pts',(-4.87586835858379,1.18514270861318,7.52731501341855));
#37937=CARTESIAN_POINT('Ctrl Pts',(-4.89498066288547,1.30000000000204,7.55519340547731));
#37938=CARTESIAN_POINT('Ctrl Pts',(-4.92893700457517,-1.3000000000004,7.31156188893225));
#37939=CARTESIAN_POINT('Ctrl Pts',(-4.91258729373097,-1.18514270861208,
7.29737510222025));
#37940=CARTESIAN_POINT('Ctrl Pts',(-4.89055620351791,-1.06847604194531,
7.2900570681081));
#37941=CARTESIAN_POINT('Ctrl Pts',(-4.82653485492317,-0.794772684000918,
7.28901913793627));
#37942=CARTESIAN_POINT('Ctrl Pts',(-4.76039738489715,-0.63630980009525,
7.30861852477781));
#37943=CARTESIAN_POINT('Ctrl Pts',(-4.69019280711872,-0.319434907277186,
7.33729173276116));
#37944=CARTESIAN_POINT('Ctrl Pts',(-4.6506343999844,-0.158333333333346,
7.35966435741067));
#37945=CARTESIAN_POINT('Ctrl Pts',(-4.64949257205487,0.158333333333348,
7.39016580818862));
#37946=CARTESIAN_POINT('Ctrl Pts',(-4.68790778944678,0.319434907277195,
7.39912505243672));
#37947=CARTESIAN_POINT('Ctrl Pts',(-4.75578931986187,0.636309800095261,
7.43088960159304));
#37948=CARTESIAN_POINT('Ctrl Pts',(-4.82112875195722,0.794772684000907,
7.44406967143752));
#37949=CARTESIAN_POINT('Ctrl Pts',(-4.88239462582399,1.06847604194587,7.49108475371676));
#37950=CARTESIAN_POINT('Ctrl Pts',(-4.90301066772921,1.1851427086132,7.51609182245864));
#37951=CARTESIAN_POINT('Ctrl Pts',(-4.91772302486701,1.30000000000206,7.54575487290414));
#37952=CARTESIAN_POINT('Ctrl Pts',(-4.94276812717222,-1.30000000000042,
7.30353165417581));
#37953=CARTESIAN_POINT('Ctrl Pts',(-4.92910617557147,-1.1851427086121,7.28785768897104));
#37954=CARTESIAN_POINT('Ctrl Pts',(-4.90905961567349,-1.06847604194532,
7.27955583815619));
#37955=CARTESIAN_POINT('Ctrl Pts',(-4.84799832960546,-0.79477268400093,
7.27740796102146));
#37956=CARTESIAN_POINT('Ctrl Pts',(-4.78148095270192,-0.636309800095261,
7.29792502713165));
#37957=CARTESIAN_POINT('Ctrl Pts',(-4.71150402741766,-0.319434907277192,
7.32741460625986));
#37958=CARTESIAN_POINT('Ctrl Pts',(-4.67115338279767,-0.158333333333349,
7.35096105844497));
#37959=CARTESIAN_POINT('Ctrl Pts',(-4.67005823101757,0.15833333333335,7.38172799267763));
#37960=CARTESIAN_POINT('Ctrl Pts',(-4.70930946320504,0.319434907277199,
7.38981036950598));
#37961=CARTESIAN_POINT('Ctrl Pts',(-4.77706432180903,0.636309800095271,
7.42123520250692));
#37962=CARTESIAN_POINT('Ctrl Pts',(-4.84286804636516,0.794772684000922,
7.43373837818253));
#37963=CARTESIAN_POINT('Ctrl Pts',(-4.90122283435496,1.06847604194589,7.48211551282895));
#37964=CARTESIAN_POINT('Ctrl Pts',(-4.91985996547775,1.18514270861322,7.50817717942918));
#37965=CARTESIAN_POINT('Ctrl Pts',(-4.93187460226044,1.30000000000208,7.53935984359063));
#37966=CARTESIAN_POINT('Ctrl Pts',(-4.9538826414882,-1.30000000000043,7.29750420865769));
#37967=CARTESIAN_POINT('Ctrl Pts',(-4.94237897545242,-1.1851427086121,7.28065982526099));
#37968=CARTESIAN_POINT('Ctrl Pts',(-4.9239198168277,-1.06847604194533,7.27154899581461));
#37969=CARTESIAN_POINT('Ctrl Pts',(-4.86520688834062,-0.794772684000932,
7.26836721389572));
#37970=CARTESIAN_POINT('Ctrl Pts',(-4.79832348941349,-0.636309800095262,
7.28924975962404));
#37971=CARTESIAN_POINT('Ctrl Pts',(-4.72852281268025,-0.319434907277192,
7.3193741434352));
#37972=CARTESIAN_POINT('Ctrl Pts',(-4.68758819801886,-0.158333333333349,
7.3441861406594));
#37973=CARTESIAN_POINT('Ctrl Pts',(-4.68654436898808,0.158333333333351,
7.37528164155598));
#37974=CARTESIAN_POINT('Ctrl Pts',(-4.72645104332334,0.3194349072772,7.38261274912261));
#37975=CARTESIAN_POINT('Ctrl Pts',(-4.79409315133171,0.636309800095272,
7.41369376798486));
#37976=CARTESIAN_POINT('Ctrl Pts',(-4.86025356328873,0.794772684000922,
7.42552056445429));
#37977=CARTESIAN_POINT('Ctrl Pts',(-4.91627584311807,1.06847604194589,7.47494594133525));
#37978=CARTESIAN_POINT('Ctrl Pts',(-4.93333146029785,1.18514270861322,7.50185755652872));
#37979=CARTESIAN_POINT('Ctrl Pts',(-4.94319272554928,1.30000000000208,7.53428637265453));
#37980=CARTESIAN_POINT('Ctrl Pts',(-4.96215724239579,-1.30000000000043,
7.29262963018817));
#37981=CARTESIAN_POINT('Ctrl Pts',(-4.95223365671038,-1.18514270861211,
7.2747178533983));
#37982=CARTESIAN_POINT('Ctrl Pts',(-4.93494771744396,-1.06847604194533,
7.26492096827301));
#37983=CARTESIAN_POINT('Ctrl Pts',(-4.87800523009233,-0.794772684000934,
7.26103522689715));
#37984=CARTESIAN_POINT('Ctrl Pts',(-4.81096227090518,-0.636309800095264,
7.28284066593449));
#37985=CARTESIAN_POINT('Ctrl Pts',(-4.74130390136971,-0.319434907277193,
7.31344134352605));
#37986=CARTESIAN_POINT('Ctrl Pts',(-4.69983863963916,-0.158333333333349,
7.33855502594921));
#37987=CARTESIAN_POINT('Ctrl Pts',(-4.69883417799421,0.158333333333351,
7.36991044588953));
#37988=CARTESIAN_POINT('Ctrl Pts',(-4.73929568703575,0.3194349072772,7.37714562001663));
#37989=CARTESIAN_POINT('Ctrl Pts',(-4.8069065964319,0.636309800095273,7.40839011633368));
#37990=CARTESIAN_POINT('Ctrl Pts',(-4.87338113727392,0.794772684000924,
7.42011569025137));
#37991=CARTESIAN_POINT('Ctrl Pts',(-4.92764623373385,1.06847604194589,7.47025282760673));
#37992=CARTESIAN_POINT('Ctrl Pts',(-4.94349629326561,1.18514270861322,7.49763280042375));
#37993=CARTESIAN_POINT('Ctrl Pts',(-4.95170706279155,1.30000000000209,7.53069023706064));
#37994=CARTESIAN_POINT('Ctrl Pts',(-4.96904374222928,-1.30000000000044,
7.28854505812584));
#37995=CARTESIAN_POINT('Ctrl Pts',(-4.96042052541168,-1.18514270861211,
7.26964689949081));
#37996=CARTESIAN_POINT('Ctrl Pts',(-4.94410226763909,-1.06847604194533,
7.2592195633072));
#37997=CARTESIAN_POINT('Ctrl Pts',(-4.88862674373442,-0.794772684000939,
7.2546996251866));
#37998=CARTESIAN_POINT('Ctrl Pts',(-4.82147221694671,-0.636309800095268,
7.27741426685326));
#37999=CARTESIAN_POINT('Ctrl Pts',(-4.75193604936788,-0.319434907277195,
7.30841654884995));
#38000=CARTESIAN_POINT('Ctrl Pts',(-4.71002121431227,-0.15833333333335,
7.3337009050263));
#38001=CARTESIAN_POINT('Ctrl Pts',(-4.70904729083083,0.158333333333352,
7.36524202054646));
#38002=CARTESIAN_POINT('Ctrl Pts',(-4.74996964632282,0.319434907277201,
7.37239217961628));
#38003=CARTESIAN_POINT('Ctrl Pts',(-4.81755979929811,0.636309800095276,
7.4038170879835));
#38004=CARTESIAN_POINT('Ctrl Pts',(-4.8843054138207,0.794772684000929,7.41554223504929));
#38005=CARTESIAN_POINT('Ctrl Pts',(-4.93711398704773,1.0684760419459,7.46632498981442));
#38006=CARTESIAN_POINT('Ctrl Pts',(-4.95196218304734,1.18514270861323,7.49410887472559));
#38007=CARTESIAN_POINT('Ctrl Pts',(-4.95879970044698,1.30000000000209,7.52769467169654));
#38008=CARTESIAN_POINT('Ctrl Pts',(-4.97388099006215,-1.30000000000044,
7.28578416877527));
#38009=CARTESIAN_POINT('Ctrl Pts',(-4.96618885844481,-1.18514270861211,
7.26631812393833));
#38010=CARTESIAN_POINT('Ctrl Pts',(-4.95055672722461,-1.06847604194533,
7.25550099325927));
#38011=CARTESIAN_POINT('Ctrl Pts',(-4.89610038943475,-0.79477268400094,
7.25049197934511));
#38012=CARTESIAN_POINT('Ctrl Pts',(-4.82880131880616,-0.636309800095269,
7.27344835749128));
#38013=CARTESIAN_POINT('Ctrl Pts',(-4.75934190858374,-0.319434907277196,
7.30468767637323));
#38014=CARTESIAN_POINT('Ctrl Pts',(-4.71715983708938,-0.15833333333335,
7.33039352380046));
#38015=CARTESIAN_POINT('Ctrl Pts',(-4.71621018252856,0.158333333333352,
7.36207232505676));
#38016=CARTESIAN_POINT('Ctrl Pts',(-4.75742869369747,0.319434907277202,
7.36898193694131));
#38017=CARTESIAN_POINT('Ctrl Pts',(-4.82498205099828,0.636309800095277,
7.40036215025163));
#38018=CARTESIAN_POINT('Ctrl Pts',(-4.89189296390852,0.794772684000931,
7.41187977881973));
#38019=CARTESIAN_POINT('Ctrl Pts',(-4.94369104604812,1.0684760419459,7.4631905316123));
#38020=CARTESIAN_POINT('Ctrl Pts',(-4.95785081403603,1.18514270861323,7.49136397433223));
#38021=CARTESIAN_POINT('Ctrl Pts',(-4.96374887956164,1.3000000000021,7.52550033613888));
#38022=CARTESIAN_POINT('Ctrl Pts',(-4.97630270097834,-1.30000000000044,
7.2844238033571));
#38023=CARTESIAN_POINT('Ctrl Pts',(-4.96907918430619,-1.18514270861211,
7.26469184565172));
#38024=CARTESIAN_POINT('Ctrl Pts',(-4.95379125816367,-1.06847604194533,
7.2536865197006));
#38025=CARTESIAN_POINT('Ctrl Pts',(-4.89984269127916,-0.794772684000939,
7.24842228025466));
#38026=CARTESIAN_POINT('Ctrl Pts',(-4.83246023827133,-0.636309800095268,
7.27143376544033));
#38027=CARTESIAN_POINT('Ctrl Pts',(-4.76303744189354,-0.319434907277195,
7.3027823689946));
#38028=CARTESIAN_POINT('Ctrl Pts',(-4.72072944001479,-0.15833333333335,
7.32874778853514));
#38029=CARTESIAN_POINT('Ctrl Pts',(-4.71979232494156,0.158333333333352,
7.3604957560239));
#38030=CARTESIAN_POINT('Ctrl Pts',(-4.76115473178469,0.319434907277202,
7.36725593780331));
#38031=CARTESIAN_POINT('Ctrl Pts',(-4.82868596530568,0.636309800095277,
7.39858428837193));
#38032=CARTESIAN_POINT('Ctrl Pts',(-4.89567510113326,0.79477268400093,7.40996091959273));
#38033=CARTESIAN_POINT('Ctrl Pts',(-4.94696966254457,1.0684760419459,7.46154837310563));
#38034=CARTESIAN_POINT('Ctrl Pts',(-4.96078757083251,1.18514270861323,7.48993503887023));
#38035=CARTESIAN_POINT('Ctrl Pts',(-4.96621987242418,1.3000000000021,7.52437807327715));
#38036=CARTESIAN_POINT('Ctrl Pts',(-4.97751398613919,-1.30000000000044,
7.28374645930059));
#38037=CARTESIAN_POINT('Ctrl Pts',(-4.97052541992915,-1.18514270861211,
7.26388559369294));
#38038=CARTESIAN_POINT('Ctrl Pts',(-4.95540983892336,-1.06847604194533,
7.25278776428831));
#38039=CARTESIAN_POINT('Ctrl Pts',(-4.90171479295647,-0.794772684000939,
7.24739392491884));
#38040=CARTESIAN_POINT('Ctrl Pts',(-4.83428843862465,-0.636309800095268,
7.27041965738315));
#38041=CARTESIAN_POINT('Ctrl Pts',(-4.76488342798957,-0.319434907277195,
7.30181978514875));
#38042=CARTESIAN_POINT('Ctrl Pts',(-4.72251363369622,-0.15833333333335,
7.32792219164892));
#38043=CARTESIAN_POINT('Ctrl Pts',(-4.72158292793032,0.158333333333352,
7.35970515916855));
#38044=CARTESIAN_POINT('Ctrl Pts',(-4.76301691052441,0.319434907277202,
7.36638801246319));
#38045=CARTESIAN_POINT('Ctrl Pts',(-4.83053654094601,0.636309800095277,
7.39768590388837));
#38046=CARTESIAN_POINT('Ctrl Pts',(-4.89756383643552,0.79477268400093,7.40898434675011));
#38047=CARTESIAN_POINT('Ctrl Pts',(-4.94860690981511,1.0684760419459,7.4607117121741));
#38048=CARTESIAN_POINT('Ctrl Pts',(-4.96225430443568,1.18514270861323,7.48920795008445));
#38049=CARTESIAN_POINT('Ctrl Pts',(-4.96745443854299,1.3000000000021,7.52380956610082));
#38050=CARTESIAN_POINT('Ctrl Pts',(-4.97820627814295,-1.30000000000044,
7.28336032475575));
#38051=CARTESIAN_POINT('Ctrl Pts',(-4.971352034479,-1.18514270861211,7.26342613826192));
#38052=CARTESIAN_POINT('Ctrl Pts',(-4.95633495359243,-1.06847604194533,
7.25227550350771));
#38053=CARTESIAN_POINT('Ctrl Pts',(-4.90278470563348,-0.794772684000939,
7.24680706821067));
#38054=CARTESIAN_POINT('Ctrl Pts',(-4.83533294408251,-0.636309800095269,
7.26983886751155));
#38055=CARTESIAN_POINT('Ctrl Pts',(-4.76593808327655,-0.319434907277196,
7.3012684086979));
#38056=CARTESIAN_POINT('Ctrl Pts',(-4.7235333012043,-0.15833333333335,7.32745135262338));
#38057=CARTESIAN_POINT('Ctrl Pts',(-4.72260623327306,0.158333333333352,
7.35925411712625));
#38058=CARTESIAN_POINT('Ctrl Pts',(-4.76408083964513,0.319434907277202,
7.36589081709313));
#38059=CARTESIAN_POINT('Ctrl Pts',(-4.83159366012784,0.636309800095277,
7.39716990722543));
#38060=CARTESIAN_POINT('Ctrl Pts',(-4.89864264437605,0.79477268400093,7.40842250430178));
#38061=CARTESIAN_POINT('Ctrl Pts',(-4.94954210729726,1.0684760419459,7.4602306906211));
#38062=CARTESIAN_POINT('Ctrl Pts',(-4.96309216930703,1.18514270861323,7.48879047475649));
#38063=CARTESIAN_POINT('Ctrl Pts',(-4.96815980183889,1.3000000000021,7.52348419885205));
#38064=CARTESIAN_POINT('Ctrl Pts',(-4.98962759657728,-1.30000000000043,
7.27698199631737));
#38065=CARTESIAN_POINT('Ctrl Pts',(-4.98499149296135,-1.18514270861211,
7.25585362164017));
#38066=CARTESIAN_POINT('Ctrl Pts',(-4.97160014405788,-1.06847604194533,
7.24383836076752));
#38067=CARTESIAN_POINT('Ctrl Pts',(-4.92043708106566,-0.794772684000933,
7.23713382046774));
#38068=CARTESIAN_POINT('Ctrl Pts',(-4.85255964742921,-0.636309800095263,
7.26023174618339));
#38069=CARTESIAN_POINT('Ctrl Pts',(-4.7833269824838,-0.319434907277192,
7.29211112083101));
#38070=CARTESIAN_POINT('Ctrl Pts',(-4.74034072307501,-0.158333333333349,
7.3195841684387));
#38071=CARTESIAN_POINT('Ctrl Pts',(-4.73947577782764,0.158333333333351,
7.35172297496417));
#38072=CARTESIAN_POINT('Ctrl Pts',(-4.78163015967787,0.319434907277199,
7.35766431892539));
#38073=CARTESIAN_POINT('Ctrl Pts',(-4.84903363693141,0.636309800095271,
7.38865110421101));
#38074=CARTESIAN_POINT('Ctrl Pts',(-4.91643593658566,0.794772684000923,
7.39912063634426));
#38075=CARTESIAN_POINT('Ctrl Pts',(-4.96496492619457,1.06847604194589,7.45224044167948));
#38076=CARTESIAN_POINT('Ctrl Pts',(-4.97690899657539,1.18514270861322,7.48183781444401));
#38077=CARTESIAN_POINT('Ctrl Pts',(-4.97979073591155,1.30000000000209,7.51803896452616));
#38078=CARTESIAN_POINT('Ctrl Pts',(-5.0117800089259,-1.30000000000032,7.26370701698165));
#38079=CARTESIAN_POINT('Ctrl Pts',(-5.01130040405251,-1.185142708612,7.2393276982123));
#38080=CARTESIAN_POINT('Ctrl Pts',(-5.0009945786159,-1.06847604194524,7.22516638093642));
#38081=CARTESIAN_POINT('Ctrl Pts',(-4.95448552495434,-0.794772684000867,
7.21605653262139));
#38082=CARTESIAN_POINT('Ctrl Pts',(-4.88617347564889,-0.636309800095205,
7.24152150033735));
#38083=CARTESIAN_POINT('Ctrl Pts',(-4.81733005758418,-0.319434907277162,
7.27456911590342));
#38084=CARTESIAN_POINT('Ctrl Pts',(-4.77299395413638,-0.158333333333335,
7.30310726673854));
#38085=CARTESIAN_POINT('Ctrl Pts',(-4.77222903565246,0.158333333333337,
7.33575692848211));
#38086=CARTESIAN_POINT('Ctrl Pts',(-4.81576663729055,0.319434907277174,
7.3407686493571));
#38087=CARTESIAN_POINT('Ctrl Pts',(-4.88312037829608,0.636309800095217,
7.3723923810245));
#38088=CARTESIAN_POINT('Ctrl Pts',(-4.95152038481361,0.79477268400085,7.38373983305775));
#38089=CARTESIAN_POINT('Ctrl Pts',(-4.99539107681839,1.06847604194579,7.43891897026865));
#38090=CARTESIAN_POINT('Ctrl Pts',(-5.00410392158195,1.18514270861311,7.46962788899476));
#38091=CARTESIAN_POINT('Ctrl Pts',(-5.0025396141095,1.30000000000196,7.50716072253685));
#38092=CARTESIAN_POINT('Ctrl Pts',(-5.03373827646427,-1.3000000000003,7.25059438324909));
#38093=CARTESIAN_POINT('Ctrl Pts',(-5.03743514540706,-1.18514270861198,
7.22337830960446));
#38094=CARTESIAN_POINT('Ctrl Pts',(-5.03020931803739,-1.06847604194522,
7.20725232196869));
#38095=CARTESIAN_POINT('Ctrl Pts',(-4.98828259773198,-0.794772684000851,
7.19561838178191));
#38096=CARTESIAN_POINT('Ctrl Pts',(-4.91934781307156,-0.636309800095197,
7.22227212406156));
#38097=CARTESIAN_POINT('Ctrl Pts',(-4.85084550516312,-0.319434907277159,
7.25618276845748));
#38098=CARTESIAN_POINT('Ctrl Pts',(-4.80525449214961,-0.158333333333332,
7.28622792996134));
#38099=CARTESIAN_POINT('Ctrl Pts',(-4.80463957298795,0.158333333333334,
7.31964424705875));
#38100=CARTESIAN_POINT('Ctrl Pts',(-4.84964913467177,0.319434907277167,
7.32440610753906));
#38101=CARTESIAN_POINT('Ctrl Pts',(-4.9168307249596,0.636309800095206,7.35572932929558));
#38102=CARTESIAN_POINT('Ctrl Pts',(-4.98579503969523,0.79477268400084,7.36476534440009));
#38103=CARTESIAN_POINT('Ctrl Pts',(-5.02510837557522,1.06847604194578,7.42266819008859));
#38104=CARTESIAN_POINT('Ctrl Pts',(-5.03075217902048,1.1851427086131,7.4556345450565));
#38105=CARTESIAN_POINT('Ctrl Pts',(-5.02502249951117,1.30000000000195,7.49650325860557));
#38106=CARTESIAN_POINT('Ctrl Pts',(-5.04463866368648,-1.3000000000003,7.24360077774404));
#38107=CARTESIAN_POINT('Ctrl Pts',(-5.05044042294363,-1.18514270861198,
7.21510877784411));
#38108=CARTESIAN_POINT('Ctrl Pts',(-5.04476129211947,-1.06847604194522,
7.19807307136938));
#38109=CARTESIAN_POINT('Ctrl Pts',(-5.00511821097741,-0.794772684000851,
7.18518351106726));
#38110=CARTESIAN_POINT('Ctrl Pts',(-4.93580560547694,-0.636309800095197,
7.21204894769254));
#38111=CARTESIAN_POINT('Ctrl Pts',(-4.86748690268216,-0.319434907277159,
7.246450708068));
#38112=CARTESIAN_POINT('Ctrl Pts',(-4.82135018302871,-0.158333333333332,
7.2776782820083));
#38113=CARTESIAN_POINT('Ctrl Pts',(-4.82082865786803,0.158333333333334,
7.31155509115153));
#38114=CARTESIAN_POINT('Ctrl Pts',(-4.86650233516519,0.319434907277167,
7.31574227169103));
#38115=CARTESIAN_POINT('Ctrl Pts',(-4.93363960349709,0.636309800095206,
7.34721244841426));
#38116=CARTESIAN_POINT('Ctrl Pts',(-5.00304362126359,0.79477268400084,7.35625511248847));
#38117=CARTESIAN_POINT('Ctrl Pts',(-5.0400719713854,1.06847604194578,7.41533660906748));
#38118=CARTESIAN_POINT('Ctrl Pts',(-5.04414241441304,1.1851427086131,7.44905694196787));
#38119=CARTESIAN_POINT('Ctrl Pts',(-5.03625509973612,1.30000000000195,7.49092341708471));
#38120=CARTESIAN_POINT('',(-4.94063702204203,1.2,7.50431203792771));
#38121=CARTESIAN_POINT('Ctrl Pts',(-4.94063702204203,1.2,7.50431203792771));
#38122=CARTESIAN_POINT('Ctrl Pts',(-4.91512883127448,1.22435101060601,7.52235013201384));
#38123=CARTESIAN_POINT('Ctrl Pts',(-4.89401189434821,1.24430028798091,7.53844339299767));
#38124=CARTESIAN_POINT('Ctrl Pts',(-4.87220163471289,1.26499468132268,7.55373639813777));
#38125=CARTESIAN_POINT('Ctrl Pts',(-4.85380470391158,1.28236518345201,7.56693408695334));
#38126=CARTESIAN_POINT('Ctrl Pts',(-4.83514000569712,1.30000000019026,7.57936937601991));
#38127=CARTESIAN_POINT('',(-4.94779107628249,0.653834841367462,7.34786299432383));
#38128=CARTESIAN_POINT('Ctrl Pts',(-4.94779107631959,0.653834841366186,
7.34786299432997));
#38129=CARTESIAN_POINT('Ctrl Pts',(-4.9473084793979,0.717511353896306,7.36401165108777));
#38130=CARTESIAN_POINT('Ctrl Pts',(-4.94685377491289,0.764335173772842,
7.37724395261881));
#38131=CARTESIAN_POINT('Ctrl Pts',(-4.94482488289273,0.949838615028042,
7.42900031049909));
#38132=CARTESIAN_POINT('Ctrl Pts',(-4.94338416731764,1.05638952303416,7.45971095101033));
#38133=CARTESIAN_POINT('Ctrl Pts',(-4.94063702204202,1.2,7.50431203792771));
#38134=CARTESIAN_POINT('',(-4.94999291725008,-0.653834841531101,7.20837371924779));
#38135=CARTESIAN_POINT('Ctrl Pts',(-4.94999291725008,-0.653834841531101,
7.20837371924779));
#38136=CARTESIAN_POINT('Ctrl Pts',(-4.91226480228564,-0.575997064012115,
7.22581500711208));
#38137=CARTESIAN_POINT('Ctrl Pts',(-4.88066561057669,-0.493634399437435,
7.2412633377142));
#38138=CARTESIAN_POINT('Ctrl Pts',(-4.83631871381536,-0.338121115118327,
7.26566636353398));
#38139=CARTESIAN_POINT('Ctrl Pts',(-4.8212754954691,-0.265647609368857,
7.27534782958795));
#38140=CARTESIAN_POINT('Ctrl Pts',(-4.8034158492223,-0.129707195798598,
7.291927539413));
#38141=CARTESIAN_POINT('Ctrl Pts',(-4.79913204414778,-0.0666204750968713,
7.29900275589153));
#38142=CARTESIAN_POINT('Ctrl Pts',(-4.79855019295222,0.0595404098440564,
7.31231675611242));
#38143=CARTESIAN_POINT('Ctrl Pts',(-4.80223085851993,0.122767112688131,
7.31865112195024));
#38144=CARTESIAN_POINT('Ctrl Pts',(-4.81904696654134,0.260121328322853,
7.33078741696058));
#38145=CARTESIAN_POINT('Ctrl Pts',(-4.83378857283769,0.333940747791096,
7.33628126340755));
#38146=CARTESIAN_POINT('Ctrl Pts',(-4.87782538116292,0.491202933844601,
7.3447735102832));
#38147=CARTESIAN_POINT('Ctrl Pts',(-4.90928838065488,0.57434292395841,7.34738832882229));
#38148=CARTESIAN_POINT('Ctrl Pts',(-4.94779107624722,0.653834841384265,
7.34786299437092));
#38149=CARTESIAN_POINT('',(-4.94934469642006,-1.2,7.28054238647221));
#38150=CARTESIAN_POINT('Ctrl Pts',(-4.94934469642006,-1.2,7.28054238647221));
#38151=CARTESIAN_POINT('Ctrl Pts',(-4.94953491045765,-1.13825277839996,
7.26885369832488));
#38152=CARTESIAN_POINT('Ctrl Pts',(-4.94976307128066,-1.0401741657608,7.25196470745215));
#38153=CARTESIAN_POINT('Ctrl Pts',(-4.94997841213571,-0.793744901850011,
7.21979027555859));
#38154=CARTESIAN_POINT('Ctrl Pts',(-4.9499822550052,-0.738116445717161,
7.21467653823378));
#38155=CARTESIAN_POINT('Ctrl Pts',(-4.94999291725008,-0.653834841531101,
7.20837371924779));
#38156=CARTESIAN_POINT('Ctrl Pts',(-4.84757993445122,-1.30000000000002,
7.35319523199426));
#38157=CARTESIAN_POINT('Ctrl Pts',(-4.86540775027189,-1.28255817374891,
7.34125683870561));
#38158=CARTESIAN_POINT('Ctrl Pts',(-4.88292260055616,-1.26540481326165,
7.32844907968304));
#38159=CARTESIAN_POINT('Ctrl Pts',(-4.90992288706715,-1.2388585038152,7.30960616899799));
#38160=CARTESIAN_POINT('Ctrl Pts',(-4.9301532007377,-1.21894383345738,7.29560714691683));
#38161=CARTESIAN_POINT('Ctrl Pts',(-4.94934469642006,-1.2,7.28054238647221));
#38162=CARTESIAN_POINT('Origin',(0.,1.25,7.2));
#38163=CARTESIAN_POINT('Origin',(0.,1.2,7.2));
#38164=CARTESIAN_POINT('Origin',(0.,0.92691742076555,7.2));
#38165=CARTESIAN_POINT('Origin',(0.,0.653834841531101,7.2));
#38166=CARTESIAN_POINT('Origin',(0.,0.,7.2));
#38167=CARTESIAN_POINT('Origin',(0.,-0.653834841531101,7.2));
#38168=CARTESIAN_POINT('Origin',(0.,-0.926917420765551,7.2));
#38169=CARTESIAN_POINT('Origin',(0.,-1.2,7.2));
#38170=CARTESIAN_POINT('Origin',(0.,-1.25,7.2));
#38171=CARTESIAN_POINT('Ctrl Pts',(-5.03625509974048,-1.30000000000007,
6.90907658291501));
#38172=CARTESIAN_POINT('Ctrl Pts',(-5.04414241441886,-1.18514270861183,
6.9509430580313));
#38173=CARTESIAN_POINT('Ctrl Pts',(-5.04007197139197,-1.06847604194514,
6.98466339093132));
#38174=CARTESIAN_POINT('Ctrl Pts',(-5.00304362127007,-0.794772684000851,
7.04374488751009));
#38175=CARTESIAN_POINT('Ctrl Pts',(-4.93363960349964,-0.636309800095197,
7.05278755158465));
#38176=CARTESIAN_POINT('Ctrl Pts',(-4.86650233516645,-0.319434907277159,
7.08425772830795));
#38177=CARTESIAN_POINT('Ctrl Pts',(-4.82082865787051,-0.158333333333332,
7.08844490884737));
#38178=CARTESIAN_POINT('Ctrl Pts',(-4.82135018303128,0.158333333333334,
7.12232171799055));
#38179=CARTESIAN_POINT('Ctrl Pts',(-4.86748690268523,0.319434907277167,
7.15354929193078));
#38180=CARTESIAN_POINT('Ctrl Pts',(-4.93580560547817,0.636309800095206,
7.18795105230634));
#38181=CARTESIAN_POINT('Ctrl Pts',(-5.00511821097388,0.79477268400084,7.21481648893188));
#38182=CARTESIAN_POINT('Ctrl Pts',(-5.04476129211656,1.06847604194523,7.20192692862984));
#38183=CARTESIAN_POINT('Ctrl Pts',(-5.05044042294223,1.18514270861202,7.18489122215511));
#38184=CARTESIAN_POINT('Ctrl Pts',(-5.04463866368783,1.30000000000036,7.15639922225512));
#38185=CARTESIAN_POINT('Ctrl Pts',(-5.02502249956532,-1.30000000000007,
6.90349674138989));
#38186=CARTESIAN_POINT('Ctrl Pts',(-5.03075217910045,-1.18514270861183,
6.9443654549365));
#38187=CARTESIAN_POINT('Ctrl Pts',(-5.02510837566902,-1.06847604194514,
6.97733180990305));
#38188=CARTESIAN_POINT('Ctrl Pts',(-4.98579503979314,-0.794772684000855,
7.0352346555911));
#38189=CARTESIAN_POINT('Ctrl Pts',(-4.91683072500823,-0.636309800095199,
7.04427067069983));
#38190=CARTESIAN_POINT('Ctrl Pts',(-4.84964913470357,-0.31943490727716,
7.07559389245761));
#38191=CARTESIAN_POINT('Ctrl Pts',(-4.80463957303102,-0.158333333333333,
7.08035575293656));
#38192=CARTESIAN_POINT('Ctrl Pts',(-4.80525449219259,0.158333333333334,
7.11377207003401));
#38193=CARTESIAN_POINT('Ctrl Pts',(-4.85084550521327,0.319434907277166,
7.14381723153794));
#38194=CARTESIAN_POINT('Ctrl Pts',(-4.91934781310062,0.636309800095206,
7.17772787593541));
#38195=CARTESIAN_POINT('Ctrl Pts',(-4.98828259770892,0.794772684000844,
7.20438161821817));
#38196=CARTESIAN_POINT('Ctrl Pts',(-5.0302093180156,1.06847604194524,7.19274767803144));
#38197=CARTESIAN_POINT('Ctrl Pts',(-5.03743514539829,1.18514270861202,7.17662169039496));
#38198=CARTESIAN_POINT('Ctrl Pts',(-5.033738276481,1.30000000000036,7.14940561674885));
#38199=CARTESIAN_POINT('Ctrl Pts',(-5.0025359559224,-1.30000000000008,6.89289909745494));
#38200=CARTESIAN_POINT('Ctrl Pts',(-5.00410024125434,-1.18514270861184,
6.93044802472378));
#38201=CARTESIAN_POINT('Ctrl Pts',(-4.99538814623125,-1.06847604194515,
6.96116325404221));
#38202=CARTESIAN_POINT('Ctrl Pts',(-4.95152096947629,-0.794772684000856,
7.0163343689863));
#38203=CARTESIAN_POINT('Ctrl Pts',(-4.88312761342581,-0.636309800095201,
7.02762863210533));
#38204=CARTESIAN_POINT('Ctrl Pts',(-4.81577644945599,-0.319434907277162,
7.05924000300318));
#38205=CARTESIAN_POINT('Ctrl Pts',(-4.77223713746572,-0.158333333333333,
7.0642756873531));
#38206=CARTESIAN_POINT('Ctrl Pts',(-4.77299933894179,0.158333333333335,
7.09693713865633));
#38207=CARTESIAN_POINT('Ctrl Pts',(-4.81732684919991,0.319434907277168,
7.12550935560819));
#38208=CARTESIAN_POINT('Ctrl Pts',(-4.88617760910314,0.636309800095209,
7.15849915881206));
#38209=CARTESIAN_POINT('Ctrl Pts',(-4.9545167272229,0.794772684000848,7.18380586237005));
#38210=CARTESIAN_POINT('Ctrl Pts',(-5.00102376613031,1.06847604194524,7.17468790825758));
#38211=CARTESIAN_POINT('Ctrl Pts',(-5.01132229374821,1.18514270861203,7.16055774337157));
#38212=CARTESIAN_POINT('Ctrl Pts',(-5.01178817509663,1.30000000000037,7.13624423808135));
#38213=CARTESIAN_POINT('Ctrl Pts',(-4.97960716003471,-1.30000000000009,
6.88198377980277));
#38214=CARTESIAN_POINT('Ctrl Pts',(-4.97669041571901,-1.18514270861184,
6.91815440719478));
#38215=CARTESIAN_POINT('Ctrl Pts',(-4.96472125689941,-1.06847604194515,
6.94772734858306));
#38216=CARTESIAN_POINT('Ctrl Pts',(-4.91615721717078,-0.794772684000857,
7.00080478470547));
#38217=CARTESIAN_POINT('Ctrl Pts',(-4.84876949114567,-0.636309800095199,
7.0112284788478));
#38218=CARTESIAN_POINT('Ctrl Pts',(-4.78135960772631,-0.319434907277159,
7.04227252440624));
#38219=CARTESIAN_POINT('Ctrl Pts',(-4.7391933891993,-0.158333333333333,
7.04842067117444));
#38220=CARTESIAN_POINT('Ctrl Pts',(-4.74006716269824,0.158333333333335,
7.08049671518586));
#38221=CARTESIAN_POINT('Ctrl Pts',(-4.78307750678514,0.319434907277169,
7.10767563488256));
#38222=CARTESIAN_POINT('Ctrl Pts',(-4.85232759462526,0.636309800095209,
7.1394199387625));
#38223=CARTESIAN_POINT('Ctrl Pts',(-4.920192231045,0.794772684000842,7.16256630016529));
#38224=CARTESIAN_POINT('Ctrl Pts',(-4.97138753900633,1.06847604194524,7.1558995652819));
#38225=CARTESIAN_POINT('Ctrl Pts',(-4.98480071031427,1.18514270861203,7.14391294224171));
#38226=CARTESIAN_POINT('Ctrl Pts',(-4.98946650108681,1.30000000000037,7.1228254786655));
#38227=CARTESIAN_POINT('Ctrl Pts',(-4.96762885674604,-1.30000000000009,
6.87633742376048));
#38228=CARTESIAN_POINT('Ctrl Pts',(-4.96246510401137,-1.18514270861184,
6.91091779260864));
#38229=CARTESIAN_POINT('Ctrl Pts',(-4.94884396706527,-1.06847604194515,
6.93940240086729));
#38230=CARTESIAN_POINT('Ctrl Pts',(-4.89783816639833,-0.794772684000859,
6.99112511785659));
#38231=CARTESIAN_POINT('Ctrl Pts',(-4.83080275526198,-0.636309800095201,
7.00243958032192));
#38232=CARTESIAN_POINT('Ctrl Pts',(-4.76327970162913,-0.31943490727716,
7.03379293971568));
#38233=CARTESIAN_POINT('Ctrl Pts',(-4.72182353139671,-0.158333333333333,
7.04059690457321));
#38234=CARTESIAN_POINT('Ctrl Pts',(-4.72276118318227,0.158333333333335,
7.07232672526039));
#38235=CARTESIAN_POINT('Ctrl Pts',(-4.76516503248846,0.319434907277169,
7.09821999675232));
#38236=CARTESIAN_POINT('Ctrl Pts',(-4.83457759043127,0.63630980009521,7.12952744142756));
#38237=CARTESIAN_POINT('Ctrl Pts',(-4.9020024724805,0.794772684000845,7.15261167039543));
#38238=CARTESIAN_POINT('Ctrl Pts',(-4.95565656440269,1.06847604194524,7.14722264546846));
#38239=CARTESIAN_POINT('Ctrl Pts',(-4.97074493751111,1.18514270861203,7.1361257633454));
#38240=CARTESIAN_POINT('Ctrl Pts',(-4.97769681541484,1.30000000000037,7.11626470830709));
#38241=CARTESIAN_POINT('Ctrl Pts',(-4.96621745329077,-1.30000000000009,
6.87569216528662));
#38242=CARTESIAN_POINT('Ctrl Pts',(-4.96078822827751,-1.18514270861184,
6.91009158941893));
#38243=CARTESIAN_POINT('Ctrl Pts',(-4.94697216315507,-1.06847604194515,
6.93845087341062));
#38244=CARTESIAN_POINT('Ctrl Pts',(-4.89567901039405,-0.794772684000858,
6.99001256063605));
#38245=CARTESIAN_POINT('Ctrl Pts',(-4.82868781665214,-0.636309800095201,
7.00141242393467));
#38246=CARTESIAN_POINT('Ctrl Pts',(-4.76115128673114,-0.31943490727716,
7.03280189955936));
#38247=CARTESIAN_POINT('Ctrl Pts',(-4.71977594578805,-0.158333333333333,
7.03970082655641));
#38248=CARTESIAN_POINT('Ctrl Pts',(-4.72072083981947,0.158333333333335,
7.07139106428865));
#38249=CARTESIAN_POINT('Ctrl Pts',(-4.76305477630722,0.319434907277169,
7.09712274218798));
#38250=CARTESIAN_POINT('Ctrl Pts',(-4.83248807833971,0.63630980009521,7.12836853884634));
#38251=CARTESIAN_POINT('Ctrl Pts',(-4.89986290428982,0.794772684000845,
7.15143598900548));
#38252=CARTESIAN_POINT('Ctrl Pts',(-4.95380679298674,1.06847604194524,7.1461950032419));
#38253=CARTESIAN_POINT('Ctrl Pts',(-4.96909210626636,1.18514270861203,7.13520415984025));
#38254=CARTESIAN_POINT('Ctrl Pts',(-4.97631242222678,1.30000000000037,7.11549110157635));
#38255=CARTESIAN_POINT('Ctrl Pts',(-4.96374656696363,-1.30000000000009,
6.87456873959149));
#38256=CARTESIAN_POINT('Ctrl Pts',(-4.95785143305027,-1.18514270861184,
6.90866323031204));
#38257=CARTESIAN_POINT('Ctrl Pts',(-4.94369341141674,-1.06847604194515,
6.93681044950405));
#38258=CARTESIAN_POINT('Ctrl Pts',(-4.89189662552214,-0.794772684000858,
6.98809676969094));
#38259=CARTESIAN_POINT('Ctrl Pts',(-4.82498350845845,-0.636309800095202,
6.99963802448331));
#38260=CARTESIAN_POINT('Ctrl Pts',(-4.7574253787244,-0.31943490727716,7.03107568321695));
#38261=CARTESIAN_POINT('Ctrl Pts',(-4.71619510299612,-0.158333333333333,
7.03811616881096));
#38262=CARTESIAN_POINT('Ctrl Pts',(-4.71715260925729,0.158333333333335,
7.06973664888779));
#38263=CARTESIAN_POINT('Ctrl Pts',(-4.75935940748507,0.319434907277169,
7.09521663791622));
#38264=CARTESIAN_POINT('Ctrl Pts',(-4.82882917382214,0.63630980009521,7.12635439626132));
#38265=CARTESIAN_POINT('Ctrl Pts',(-4.89612151873647,0.794772684000845,
7.14936169526838));
#38266=CARTESIAN_POINT('Ctrl Pts',(-4.95057326325068,1.06847604194524,7.14437500161006));
#38267=CARTESIAN_POINT('Ctrl Pts',(-4.96620267682485,1.18514270861203,7.13357260010592));
#38268=CARTESIAN_POINT('Ctrl Pts',(-4.97389136140897,1.30000000000037,7.11412635200712));
#38269=CARTESIAN_POINT('Ctrl Pts',(-4.95879846811985,-1.30000000000009,
6.87236883666737));
#38270=CARTESIAN_POINT('Ctrl Pts',(-4.95196564729062,-1.18514270861184,
6.90589852110311));
#38271=CARTESIAN_POINT('Ctrl Pts',(-4.93712024036981,-1.06847604194515,
6.93364785801924));
#38272=CARTESIAN_POINT('Ctrl Pts',(-4.88431370378531,-0.794772684000859,
6.98440061840653));
#38273=CARTESIAN_POINT('Ctrl Pts',(-4.81756427071818,-0.636309800095202,
6.99616354044533));
#38274=CARTESIAN_POINT('Ctrl Pts',(-4.74996685995357,-0.31943490727716,
7.02766556635525));
#38275=CARTESIAN_POINT('Ctrl Pts',(-4.70902907192969,-0.158333333333333,
7.03497395089354));
#38276=CARTESIAN_POINT('Ctrl Pts',(-4.71001081751719,0.158333333333335,
7.06645747723653));
#38277=CARTESIAN_POINT('Ctrl Pts',(-4.75195523949809,0.319434907277169,
7.09148194038527));
#38278=CARTESIAN_POINT('Ctrl Pts',(-4.82150169951971,0.636309800095211,
7.12237958432224));
#38279=CARTESIAN_POINT('Ctrl Pts',(-4.88864476872158,0.794772684000845,
7.14517114864296));
#38280=CARTESIAN_POINT('Ctrl Pts',(-4.94411462370513,1.06847604194524,7.14068026114152));
#38281=CARTESIAN_POINT('Ctrl Pts',(-4.96043038643738,1.18514270861203,7.13026730503555));
#38282=CARTESIAN_POINT('Ctrl Pts',(-4.96905106704017,1.30000000000037,7.1113853316192));
#38283=CARTESIAN_POINT('Ctrl Pts',(-4.94886166525784,-1.30000000000009,
6.86822927322511));
#38284=CARTESIAN_POINT('Ctrl Pts',(-4.94009736845648,-1.18514270861184,
6.9010906915426));
#38285=CARTESIAN_POINT('Ctrl Pts',(-4.92384423109776,-1.06847604194515,
6.92831526656563));
#38286=CARTESIAN_POINT('Ctrl Pts',(-4.86899551254524,-0.794772684000858,
6.97818724546956));
#38287=CARTESIAN_POINT('Ctrl Pts',(-4.80263500910927,-0.636309800095202,
6.98986967448523));
#38288=CARTESIAN_POINT('Ctrl Pts',(-4.73502168478157,-0.319434907277161,
7.0210190415513));
#38289=CARTESIAN_POINT('Ctrl Pts',(-4.69474707272955,-0.158333333333333,
7.02832071879295));
#38290=CARTESIAN_POINT('Ctrl Pts',(-4.6957719818575,0.158333333333335,7.05953614177902));
#38291=CARTESIAN_POINT('Ctrl Pts',(-4.737061776107,0.319434907277169,7.08448458166602));
#38292=CARTESIAN_POINT('Ctrl Pts',(-4.80678257958942,0.63630980009521,7.11481118616956));
#38293=CARTESIAN_POINT('Ctrl Pts',(-4.87380031009546,0.794772684000846,
7.13616060747813));
#38294=CARTESIAN_POINT('Ctrl Pts',(-4.93132886568866,1.06847604194524,7.13252271691075));
#38295=CARTESIAN_POINT('Ctrl Pts',(-4.94899630268446,1.18514270861203,7.12300334849857));
#38296=CARTESIAN_POINT('Ctrl Pts',(-4.95942919660282,1.30000000000037,7.10553931970368));
#38297=CARTESIAN_POINT('Ctrl Pts',(-4.93470246489923,-1.30000000000008,
6.86201249896371));
#38298=CARTESIAN_POINT('Ctrl Pts',(-4.92322980335383,-1.18514270861184,
6.89348640190275));
#38299=CARTESIAN_POINT('Ctrl Pts',(-4.9049905596083,-1.06847604194515,6.91974778539996));
#38300=CARTESIAN_POINT('Ctrl Pts',(-4.84722209927548,-0.79477268400086,
6.96837487217873));
#38301=CARTESIAN_POINT('Ctrl Pts',(-4.78132833125217,-0.636309800095202,
6.98071090897872));
#38302=CARTESIAN_POINT('Ctrl Pts',(-4.71359913861764,-0.31943490727716,
7.0120951323827));
#38303=CARTESIAN_POINT('Ctrl Pts',(-4.6741726937007,-0.158333333333333,
7.02012386392998));
#38304=CARTESIAN_POINT('Ctrl Pts',(-4.67526623655484,0.158333333333335,
7.0508886474674));
#38305=CARTESIAN_POINT('Ctrl Pts',(-4.71579254504536,0.319434907277169,
7.07448489895168));
#38306=CARTESIAN_POINT('Ctrl Pts',(-4.78573633088569,0.63630980009521,7.10401416004235));
#38307=CARTESIAN_POINT('Ctrl Pts',(-4.85233696677326,0.794772684000844,
7.12467923821773));
#38308=CARTESIAN_POINT('Ctrl Pts',(-4.9127987545522,1.06847604194524,7.12232311099618));
#38309=CARTESIAN_POINT('Ctrl Pts',(-4.93244088128556,1.18514270861203,7.11385258528136));
#38310=CARTESIAN_POINT('Ctrl Pts',(-4.9455534671528,1.30000000000038,7.0979314140228));
#38311=CARTESIAN_POINT('Ctrl Pts',(-4.91772347406777,-1.30000000000008,
6.85432821639611));
#38312=CARTESIAN_POINT('Ctrl Pts',(-4.90302035506022,-1.18514270861184,
6.88390141473553));
#38313=CARTESIAN_POINT('Ctrl Pts',(-4.88240980055113,-1.06847604194515,
6.9088562755197));
#38314=CARTESIAN_POINT('Ctrl Pts',(-4.82114793872087,-0.794772684000859,
6.95583771248602));
#38315=CARTESIAN_POINT('Ctrl Pts',(-4.75579823557382,-0.6363098000952,6.96911855277399));
#38316=CARTESIAN_POINT('Ctrl Pts',(-4.6879078771988,-0.319434907277159,
7.00099100397379));
#38317=CARTESIAN_POINT('Ctrl Pts',(-4.64947742668345,-0.158333333333333,
7.01012824404134));
#38318=CARTESIAN_POINT('Ctrl Pts',(-4.65063053921603,0.158333333333335,
7.04053799216907));
#38319=CARTESIAN_POINT('Ctrl Pts',(-4.69022144677078,0.319434907277169,
7.06258925454765));
#38320=CARTESIAN_POINT('Ctrl Pts',(-4.76044565211625,0.636309800095209,
7.09107300423509));
#38321=CARTESIAN_POINT('Ctrl Pts',(-4.82658895705298,0.794772684000842,
7.11064697678831));
#38322=CARTESIAN_POINT('Ctrl Pts',(-4.8905994758702,1.06847604194524,7.10965725427226));
#38323=CARTESIAN_POINT('Ctrl Pts',(-4.91262041978007,1.18514270861203,7.10239436821986));
#38324=CARTESIAN_POINT('Ctrl Pts',(-4.92895452582728,1.30000000000037,7.08829701031943));
#38325=CARTESIAN_POINT('Ctrl Pts',(-4.89497550322615,-1.30000000000008,
6.84496254364098));
#38326=CARTESIAN_POINT('Ctrl Pts',(-4.87586793808774,-1.18514270861184,
6.87279864480645));
#38327=CARTESIAN_POINT('Ctrl Pts',(-4.85203155425065,-1.06847604194515,
6.89653623853556));
#38328=CARTESIAN_POINT('Ctrl Pts',(-4.78604022194376,-0.79477268400086,
6.94190645665755));
#38329=CARTESIAN_POINT('Ctrl Pts',(-4.7214628557846,-0.636309800095199,
6.95607542401912));
#38330=CARTESIAN_POINT('Ctrl Pts',(-4.65344063474061,-0.319434907277158,
6.98787198691369));
#38331=CARTESIAN_POINT('Ctrl Pts',(-4.61646069367224,-0.158333333333333,
6.99742355686582));
#38332=CARTESIAN_POINT('Ctrl Pts',(-4.61775673603919,0.158333333333334,
7.02675962258274));
#38333=CARTESIAN_POINT('Ctrl Pts',(-4.65610228950268,0.319434907277168,
7.04675694704748));
#38334=CARTESIAN_POINT('Ctrl Pts',(-4.72662274639178,0.636309800095207,
7.07428232101385));
#38335=CARTESIAN_POINT('Ctrl Pts',(-4.79197838832543,0.794772684000841,
7.0934352899));
#38336=CARTESIAN_POINT('Ctrl Pts',(-4.86068659839513,1.06847604194524,7.09459518377703));
#38337=CARTESIAN_POINT('Ctrl Pts',(-4.88589934228688,1.18514270861202,7.08891273185031));
#38338=CARTESIAN_POINT('Ctrl Pts',(-4.90658359182129,1.30000000000037,7.07704575291581));
#38339=CARTESIAN_POINT('Ctrl Pts',(-4.87221950826238,-1.30000000000007,
6.8354655065749));
#38340=CARTESIAN_POINT('Ctrl Pts',(-4.84871244991834,-1.18514270861184,
6.86149155824746));
#38341=CARTESIAN_POINT('Ctrl Pts',(-4.821658861283,-1.06847604194515,6.88390778160632));
#38342=CARTESIAN_POINT('Ctrl Pts',(-4.75096646502965,-0.794772684000856,
6.9273543163671));
#38343=CARTESIAN_POINT('Ctrl Pts',(-4.68721690445203,-0.636309800095198,
6.94185272432912));
#38344=CARTESIAN_POINT('Ctrl Pts',(-4.61905429626832,-0.319434907277158,
6.9736595223705));
#38345=CARTESIAN_POINT('Ctrl Pts',(-4.58349758943882,-0.158333333333333,
6.98404901772125));
#38346=CARTESIAN_POINT('Ctrl Pts',(-4.58482508549164,0.158333333333334,
7.01316526577346));
#38347=CARTESIAN_POINT('Ctrl Pts',(-4.62173850853168,0.319434907277168,
7.03232083572209));
#38348=CARTESIAN_POINT('Ctrl Pts',(-4.69254561123477,0.636309800095207,
7.05894826866698));
#38349=CARTESIAN_POINT('Ctrl Pts',(-4.75729511476953,0.794772684000841,
7.07645282720016));
#38350=CARTESIAN_POINT('Ctrl Pts',(-4.83080559532184,1.06847604194524,7.07903999007789));
#38351=CARTESIAN_POINT('Ctrl Pts',(-4.85924414270016,1.18514270861202,7.07469855911161));
#38352=CARTESIAN_POINT('Ctrl Pts',(-4.88430127425747,1.30000000000037,7.06489581023311));
#38353=CARTESIAN_POINT('Ctrl Pts',(-4.84942653756722,-1.30000000000008,
6.82625073361417));
#38354=CARTESIAN_POINT('Ctrl Pts',(-4.82151151621238,-1.18514270861184,
6.85040399206725));
#38355=CARTESIAN_POINT('Ctrl Pts',(-4.79121791804108,-1.06847604194515,
6.87162818259571));
#38356=CARTESIAN_POINT('Ctrl Pts',(-4.71573865777315,-0.794772684000856,
6.91389357573726));
#38357=CARTESIAN_POINT('Ctrl Pts',(-4.65266532438613,-0.636309800095195,
6.9303891365972));
#38358=CARTESIAN_POINT('Ctrl Pts',(-4.58432389488618,-0.319434907277155,
6.96252779418703));
#38359=CARTESIAN_POINT('Ctrl Pts',(-4.55026914228413,-0.158333333333332,
6.97279224916784));
#38360=CARTESIAN_POINT('Ctrl Pts',(-4.55169485151761,0.158333333333334,
7.00096988169182));
#38361=CARTESIAN_POINT('Ctrl Pts',(-4.58721478137616,0.319434907277168,
7.01896552662565));
#38362=CARTESIAN_POINT('Ctrl Pts',(-4.65837988440915,0.636309800095205,
7.04405469749339));
#38363=CARTESIAN_POINT('Ctrl Pts',(-4.72260078732687,0.794772684000835,
7.05922726431916));
#38364=CARTESIAN_POINT('Ctrl Pts',(-4.80090120822937,1.06847604194523,7.06339013240831));
#38365=CARTESIAN_POINT('Ctrl Pts',(-4.8325353964471,1.18514270861202,7.06068270166945));
#38366=CARTESIAN_POINT('Ctrl Pts',(-4.8619104219904,1.30000000000036,7.05346588884542));
#38367=CARTESIAN_POINT('Ctrl Pts',(-4.82657019046039,-1.30000000000008,
6.81740338407784));
#38368=CARTESIAN_POINT('Ctrl Pts',(-4.79416905836716,-1.18514270861184,
6.84057624086466));
#38369=CARTESIAN_POINT('Ctrl Pts',(-4.76060377570003,-1.06847604194515,
6.86098284638132));
#38370=CARTESIAN_POINT('Ctrl Pts',(-4.68037183731389,-0.79477268400086,
6.90173559363148));
#38371=CARTESIAN_POINT('Ctrl Pts',(-4.61824100496772,-0.636309800095199,
6.91727506454465));
#38372=CARTESIAN_POINT('Ctrl Pts',(-4.54974399512114,-0.319434907277158,
6.94956855491332));
#38373=CARTESIAN_POINT('Ctrl Pts',(-4.51700107538385,-0.158333333333333,
6.96198316429634));
#38374=CARTESIAN_POINT('Ctrl Pts',(-4.51846353819816,0.158333333333335,
6.98983189669192));
#38375=CARTESIAN_POINT('Ctrl Pts',(-4.55269701870694,0.319434907277169,
7.00542864644343));
#38376=CARTESIAN_POINT('Ctrl Pts',(-4.6241157264898,0.636309800095208,7.02952975983155));
#38377=CARTESIAN_POINT('Ctrl Pts',(-4.68749595868162,0.794772684000841,
7.04459296382786));
#38378=CARTESIAN_POINT('Ctrl Pts',(-4.77061014902644,1.06847604194523,7.05019540129841));
#38379=CARTESIAN_POINT('Ctrl Pts',(-4.80552645837556,1.18514270861202,7.04854708152255));
#38380=CARTESIAN_POINT('Ctrl Pts',(-4.83938202375779,1.30000000000036,7.0428253543806));
#38381=CARTESIAN_POINT('Ctrl Pts',(-4.79795229094086,-1.30000000000008,
6.807426875264));
#38382=CARTESIAN_POINT('Ctrl Pts',(-4.76002338322289,-1.18514270861183,
6.82818459790646));
#38383=CARTESIAN_POINT('Ctrl Pts',(-4.7223931560717,-1.06847604194514,6.8470950796854));
#38384=CARTESIAN_POINT('Ctrl Pts',(-4.63614981531142,-0.79477268400085,
6.88651457968965));
#38385=CARTESIAN_POINT('Ctrl Pts',(-4.57484916985655,-0.636309800095196,
6.90505395334045));
#38386=CARTESIAN_POINT('Ctrl Pts',(-4.50612552655079,-0.319434907277158,
6.93778081866204));
#38387=CARTESIAN_POINT('Ctrl Pts',(-4.47528358705089,-0.158333333333332,
6.94965909012082));
#38388=CARTESIAN_POINT('Ctrl Pts',(-4.47686718908055,0.158333333333334,
6.97607866248283));
#38389=CARTESIAN_POINT('Ctrl Pts',(-4.50933783153711,0.319434907277168,
6.99019693242906));
#38390=CARTESIAN_POINT('Ctrl Pts',(-4.58119529081328,0.636309800095206,
7.01214651733671));
#38391=CARTESIAN_POINT('Ctrl Pts',(-4.64387276186949,0.794772684000838,
7.02437494544686));
#38392=CARTESIAN_POINT('Ctrl Pts',(-4.73305776181358,1.06847604194523,7.03126602506554));
#38393=CARTESIAN_POINT('Ctrl Pts',(-4.77203210410964,1.18514270861202,7.03122247186028));
#38394=CARTESIAN_POINT('Ctrl Pts',(-4.81137590685587,1.30000000000036,7.02815247242249));
#38395=CARTESIAN_POINT('Ctrl Pts',(-4.77218237162956,-1.30000000000007,
6.79773450848216));
#38396=CARTESIAN_POINT('Ctrl Pts',(-4.7292024132972,-1.18514270861183,6.81729430755761));
#38397=CARTESIAN_POINT('Ctrl Pts',(-4.68787751090051,-1.06847604194515,
6.83535570779021));
#38398=CARTESIAN_POINT('Ctrl Pts',(-4.59623222964992,-0.794772684000858,
6.8736195544176));
#38399=CARTESIAN_POINT('Ctrl Pts',(-4.5359023188134,-0.6363098000952,6.8921746025984));
#38400=CARTESIAN_POINT('Ctrl Pts',(-4.46695698337517,-0.31943490727716,
6.92582470962968));
#38401=CARTESIAN_POINT('Ctrl Pts',(-4.43763614628022,-0.158333333333333,
6.94014570092824));
#38402=CARTESIAN_POINT('Ctrl Pts',(-4.43921533843528,0.158333333333335,
6.96643125277066));
#38403=CARTESIAN_POINT('Ctrl Pts',(-4.47011307856436,0.319434907277169,
6.97826785795477));
#38404=CARTESIAN_POINT('Ctrl Pts',(-4.54227977749132,0.636309800095209,
6.99842016325866));
#38405=CARTESIAN_POINT('Ctrl Pts',(-4.60419731222694,0.794772684000845,
7.00872952970313));
#38406=CARTESIAN_POINT('Ctrl Pts',(-4.69883926674906,1.06847604194524,7.01688503767645));
#38407=CARTESIAN_POINT('Ctrl Pts',(-4.74149462807118,1.18514270861202,7.01821760615924));
#38408=CARTESIAN_POINT('Ctrl Pts',(-4.78583835543282,1.30000000000036,7.01735252591453));
#38409=CARTESIAN_POINT('Ctrl Pts',(-4.75492703857426,-1.30000000000007,
6.79270521874686));
#38410=CARTESIAN_POINT('Ctrl Pts',(-4.70857931792514,-1.18514270861183,
6.81137871632538));
#38411=CARTESIAN_POINT('Ctrl Pts',(-4.6647859738728,-1.06847604194514,6.82886797362648));
#38412=CARTESIAN_POINT('Ctrl Pts',(-4.56951570922326,-0.794772684000854,
6.86653582475861));
#38413=CARTESIAN_POINT('Ctrl Pts',(-4.50976391569166,-0.6363098000952,6.88605516832133));
#38414=CARTESIAN_POINT('Ctrl Pts',(-4.44070375128662,-0.319434907277161,
6.91966119238193));
#38415=CARTESIAN_POINT('Ctrl Pts',(-4.41252091761176,-0.158333333333333,
6.93363240105524));
#38416=CARTESIAN_POINT('Ctrl Pts',(-4.41412987613798,0.158333333333335,
6.95928252399892));
#38417=CARTESIAN_POINT('Ctrl Pts',(-4.44391739568318,0.319434907277169,
6.97063151666728));
#38418=CARTESIAN_POINT('Ctrl Pts',(-4.51626359584969,0.636309800095209,
6.98994497272097));
#38419=CARTESIAN_POINT('Ctrl Pts',(-4.57762680043773,0.794772684000846,
6.99927890139707));
#38420=CARTESIAN_POINT('Ctrl Pts',(-4.67597917764199,1.06847604194524,7.00761371103398));
#38421=CARTESIAN_POINT('Ctrl Pts',(-4.72114777053477,1.18514270861202,7.00933571455169));
#38422=CARTESIAN_POINT('Ctrl Pts',(-4.76891185654332,1.30000000000036,7.00917189133044));
#38423=CARTESIAN_POINT('Ctrl Pts',(-4.74343177047671,-1.30000000000007,
6.78894839353199));
#38424=CARTESIAN_POINT('Ctrl Pts',(-4.69481076451741,-1.18514270861183,
6.80749338476164));
#38425=CARTESIAN_POINT('Ctrl Pts',(-4.64935536677492,-1.06847604194514,
6.82487435084292));
#38426=CARTESIAN_POINT('Ctrl Pts',(-4.55165749292722,-0.794772684000855,
6.86233872858587));
#38427=CARTESIAN_POINT('Ctrl Pts',(-4.49233964697176,-0.636309800095201,
6.88170146657958));
#38428=CARTESIAN_POINT('Ctrl Pts',(-4.42320138459244,-0.319434907277162,
6.9153662578531));
#38429=CARTESIAN_POINT('Ctrl Pts',(-4.39574455555068,-0.158333333333333,
6.92977938387961));
#38430=CARTESIAN_POINT('Ctrl Pts',(-4.39735399981225,0.158333333333335,
6.9552783179463));
#38431=CARTESIAN_POINT('Ctrl Pts',(-4.42639564879919,0.319434907277168,
6.96618433558605));
#38432=CARTESIAN_POINT('Ctrl Pts',(-4.49886239121498,0.636309800095209,
6.9848252571226));
#38433=CARTESIAN_POINT('Ctrl Pts',(-4.55987835731215,0.794772684000848,
6.99323036807503));
#38434=CARTESIAN_POINT('Ctrl Pts',(-4.66069740339173,1.06847604194524,7.00172678604837));
#38435=CARTESIAN_POINT('Ctrl Pts',(-4.70753252772009,1.18514270861203,7.00380117594681));
#38436=CARTESIAN_POINT('Ctrl Pts',(-4.75756194704279,1.30000000000037,7.00427217122634));
#38437=CARTESIAN_POINT('Ctrl Pts',(-4.72910106576438,-1.30000000000007,
6.78356480038481));
#38438=CARTESIAN_POINT('Ctrl Pts',(-4.67768109823327,-1.18514270861183,
6.8012358307048));
#38439=CARTESIAN_POINT('Ctrl Pts',(-4.6301699403561,-1.06847604194514,6.81813955457351));
#38440=CARTESIAN_POINT('Ctrl Pts',(-4.52943979334055,-0.794772684000856,
6.85541790688697));
#38441=CARTESIAN_POINT('Ctrl Pts',(-4.47057871361804,-0.6363098000952,6.87621956871056));
#38442=CARTESIAN_POINT('Ctrl Pts',(-4.40130529644547,-0.319434907277161,
6.91065660584509));
#38443=CARTESIAN_POINT('Ctrl Pts',(-4.37475075817477,-0.158333333333333,
6.92560315869304));
#38444=CARTESIAN_POINT('Ctrl Pts',(-4.37638344582047,0.158333333333335,
6.95053393682423));
#38445=CARTESIAN_POINT('Ctrl Pts',(-4.40453061134416,0.319434907277167,
6.96016363706222));
#38446=CARTESIAN_POINT('Ctrl Pts',(-4.47721129582908,0.636309800095208,
6.97723094189587));
#38447=CARTESIAN_POINT('Ctrl Pts',(-4.53789275173436,0.794772684000846,
6.98372009914652));
#38448=CARTESIAN_POINT('Ctrl Pts',(-4.64175773806367,1.06847604194524,6.99279885795604));
#38449=CARTESIAN_POINT('Ctrl Pts',(-4.69062602097088,1.18514270861203,6.99578117483915));
#38450=CARTESIAN_POINT('Ctrl Pts',(-4.74340328278039,1.30000000000037,6.9978159503179));
#38451=CARTESIAN_POINT('Ctrl Pts',(-4.71179979755842,-1.30000000000008,
6.77906526523393));
#38452=CARTESIAN_POINT('Ctrl Pts',(-4.65698137257456,-1.18514270861184,
6.79625865703069));
#38453=CARTESIAN_POINT('Ctrl Pts',(-4.60698344750808,-1.06847604194515,
6.81284466530486));
#38454=CARTESIAN_POINT('Ctrl Pts',(-4.5026145577007,-0.794772684000858,
6.84975848499391));
#38455=CARTESIAN_POINT('Ctrl Pts',(-4.44437945897796,-0.636309800095201,
6.87100152702682));
#38456=CARTESIAN_POINT('Ctrl Pts',(-4.37499166711687,-0.319434907277161,
6.90537712317566));
#38457=CARTESIAN_POINT('Ctrl Pts',(-4.34954854042974,-0.158333333333333,
6.92025735903156));
#38458=CARTESIAN_POINT('Ctrl Pts',(-4.35119141508047,0.158333333333335,
6.9446473087528));
#38459=CARTESIAN_POINT('Ctrl Pts',(-4.37823623949102,0.319434907277168,
6.95359905506214));
#38460=CARTESIAN_POINT('Ctrl Pts',(-4.4510543231609,0.636309800095209,6.97004057009735));
#38461=CARTESIAN_POINT('Ctrl Pts',(-4.51110163934993,0.794772684000847,
6.9761295594491));
#38462=CARTESIAN_POINT('Ctrl Pts',(-4.6186674384589,1.06847604194524,6.98542356437354));
#38463=CARTESIAN_POINT('Ctrl Pts',(-4.67006233573082,1.18514270861203,6.98868602561221));
#38464=CARTESIAN_POINT('Ctrl Pts',(-4.72629088154604,1.30000000000037,6.99118791773457));
#38465=CARTESIAN_POINT('Ctrl Pts',(-4.68591920074664,-1.30000000000007,
6.77087890474239));
#38466=CARTESIAN_POINT('Ctrl Pts',(-4.62604476318184,-1.18514270861183,
6.78691107828377));
#38467=CARTESIAN_POINT('Ctrl Pts',(-4.57233919319432,-1.06847604194514,
6.80288228225904));
#38468=CARTESIAN_POINT('Ctrl Pts',(-4.46251990094192,-0.79477268400085,
6.83963810657568));
#38469=CARTESIAN_POINT('Ctrl Pts',(-4.40516259399858,-0.636309800095198,
6.86266250192134));
#38470=CARTESIAN_POINT('Ctrl Pts',(-4.33554669631685,-0.319434907277161,
6.89871450375448));
#38471=CARTESIAN_POINT('Ctrl Pts',(-4.31171910011351,-0.158333333333333,
6.91563912927993));
#38472=CARTESIAN_POINT('Ctrl Pts',(-4.31336797283825,0.158333333333335,
6.93926032019774));
#38473=CARTESIAN_POINT('Ctrl Pts',(-4.33877696382717,0.319434907277167,
6.94516708872193));
#38474=CARTESIAN_POINT('Ctrl Pts',(-4.41188894422988,0.636309800095207,
6.9588385113594));
#38475=CARTESIAN_POINT('Ctrl Pts',(-4.47115905367224,0.794772684000845,
6.96281269084457));
#38476=CARTESIAN_POINT('Ctrl Pts',(-4.58426559796726,1.06847604194524,6.9722078167419));
#38477=CARTESIAN_POINT('Ctrl Pts',(-4.63940110944556,1.18514270861202,6.97622079803382));
#38478=CARTESIAN_POINT('Ctrl Pts',(-4.70071250038734,1.30000000000036,6.98017995874043));
#38479=CARTESIAN_POINT('Ctrl Pts',(-4.65706796695331,-1.30000000000007,
6.76297007363097));
#38480=CARTESIAN_POINT('Ctrl Pts',(-4.59150651464294,-1.18514270861183,
6.77828368661244));
#38481=CARTESIAN_POINT('Ctrl Pts',(-4.53363602969887,-1.06847604194514,
6.79401380628528));
#38482=CARTESIAN_POINT('Ctrl Pts',(-4.41771130571616,-0.794772684000849,
6.83131574330816));
#38483=CARTESIAN_POINT('Ctrl Pts',(-4.36137897286265,-0.636309800095198,
6.8570983207674));
#38484=CARTESIAN_POINT('Ctrl Pts',(-4.29154387441274,-0.319434907277161,
6.89377932179117));
#38485=CARTESIAN_POINT('Ctrl Pts',(-4.26956906956148,-0.158333333333333,
6.90966130373019));
#38486=CARTESIAN_POINT('Ctrl Pts',(-4.27120100423192,0.158333333333335,
6.93208761653411));
#38487=CARTESIAN_POINT('Ctrl Pts',(-4.29469526007313,0.319434907277168,
6.93739989461276));
#38488=CARTESIAN_POINT('Ctrl Pts',(-4.36808361310165,0.636309800095208,
6.94890928083732));
#38489=CARTESIAN_POINT('Ctrl Pts',(-4.42648405296358,0.794772684000843,
6.9496565215753));
#38490=CARTESIAN_POINT('Ctrl Pts',(-4.54578080039787,1.06847604194524,6.95909532760112));
#38491=CARTESIAN_POINT('Ctrl Pts',(-4.60510078398202,1.18514270861202,6.96397715982235));
#38492=CARTESIAN_POINT('Ctrl Pts',(-4.67210160956614,1.30000000000037,6.96965511487846));
#38493=CARTESIAN_POINT('Ctrl Pts',(-4.62824128498163,-1.30000000000007,
6.75514249224118));
#38494=CARTESIAN_POINT('Ctrl Pts',(-4.55705822919735,-1.18514270861183,
6.76997343913831));
#38495=CARTESIAN_POINT('Ctrl Pts',(-4.4950748534049,-1.06847604194514,6.78568042640955));
#38496=CARTESIAN_POINT('Ctrl Pts',(-4.37313395676334,-0.794772684000853,
6.82399053769364));
#38497=CARTESIAN_POINT('Ctrl Pts',(-4.31785205317386,-0.636309800095198,
6.85232071213997));
#38498=CARTESIAN_POINT('Ctrl Pts',(-4.24781120390648,-0.31943490727716,
6.89089241386308));
#38499=CARTESIAN_POINT('Ctrl Pts',(-4.22765878228674,-0.158333333333333,
6.90794909635979));
#38500=CARTESIAN_POINT('Ctrl Pts',(-4.22924496873314,0.158333333333335,
6.92951718428705));
#38501=CARTESIAN_POINT('Ctrl Pts',(-4.25082855928738,0.319434907277167,
6.93243445575821));
#38502=CARTESIAN_POINT('Ctrl Pts',(-4.32441611564697,0.636309800095207,
6.94104253228292));
#38503=CARTESIAN_POINT('Ctrl Pts',(-4.38182613959396,0.794772684000843,
6.93932195929744));
#38504=CARTESIAN_POINT('Ctrl Pts',(-4.50726340370541,1.06847604194524,6.94785703943639));
#38505=CARTESIAN_POINT('Ctrl Pts',(-4.57076648303345,1.18514270861202,6.95291462731048));
#38506=CARTESIAN_POINT('Ctrl Pts',(-4.64347549796437,1.30000000000036,6.95933528312239));
#38507=CARTESIAN_POINT('Ctrl Pts',(-4.60795779379676,-1.30000000000007,
6.75077046400054));
#38508=CARTESIAN_POINT('Ctrl Pts',(-4.532697496001,-1.18514270861183,6.76528337471195));
#38509=CARTESIAN_POINT('Ctrl Pts',(-4.46773218910147,-1.06847604194514,
6.78106969840869));
#38510=CARTESIAN_POINT('Ctrl Pts',(-4.3414328223746,-0.79477268400085,6.82048110293289));
#38511=CARTESIAN_POINT('Ctrl Pts',(-4.28692863454769,-0.636309800095197,
6.85217463225275));
#38512=CARTESIAN_POINT('Ctrl Pts',(-4.2167292513552,-0.319434907277159,
6.89061321103449));
#38513=CARTESIAN_POINT('Ctrl Pts',(-4.19787125500864,-0.158333333333333,
6.90432318701196));
#38514=CARTESIAN_POINT('Ctrl Pts',(-4.19940827209993,0.158333333333334,
6.924653254063));
#38515=CARTESIAN_POINT('Ctrl Pts',(-4.21959643664148,0.319434907277168,
6.92904737099824));
#38516=CARTESIAN_POINT('Ctrl Pts',(-4.29334794928819,0.636309800095208,
6.93655382403039));
#38517=CARTESIAN_POINT('Ctrl Pts',(-4.35009169193594,0.794772684000841,
6.93208263408248));
#38518=CARTESIAN_POINT('Ctrl Pts',(-4.47999547157628,1.06847604194523,6.93981305401699));
#38519=CARTESIAN_POINT('Ctrl Pts',(-4.5465288739018,1.18514270861202,6.94498811462777));
#38520=CARTESIAN_POINT('Ctrl Pts',(-4.62336514575594,1.30000000000036,6.95199202349996));
#38521=CARTESIAN_POINT('Ctrl Pts',(-4.59357758309325,-1.30000000000007,
6.74732625969349));
#38522=CARTESIAN_POINT('Ctrl Pts',(-4.51560674585504,-1.18514270861183,
6.76249095077157));
#38523=CARTESIAN_POINT('Ctrl Pts',(-4.44866546053796,-1.06847604194514,
6.77856704318338));
#38524=CARTESIAN_POINT('Ctrl Pts',(-4.31949817128937,-0.794772684000852,
6.81781155207203));
#38525=CARTESIAN_POINT('Ctrl Pts',(-4.26554133800437,-0.636309800095197,
6.84789782529569));
#38526=CARTESIAN_POINT('Ctrl Pts',(-4.1953076385941,-0.319434907277159,
6.88545957404936));
#38527=CARTESIAN_POINT('Ctrl Pts',(-4.17739534454885,-0.158333333333333,
6.89877049130274));
#38528=CARTESIAN_POINT('Ctrl Pts',(-4.1789158924004,0.158333333333334,6.91968195652444));
#38529=CARTESIAN_POINT('Ctrl Pts',(-4.19813604853114,0.319434907277168,
6.9259209804531));
#38530=CARTESIAN_POINT('Ctrl Pts',(-4.27190022002353,0.636309800095207,
6.93372770711639));
#38531=CARTESIAN_POINT('Ctrl Pts',(-4.32807553656376,0.794772684000841,
6.92770471093727));
#38532=CARTESIAN_POINT('Ctrl Pts',(-4.46087871138807,1.06847604194523,6.93522051755055));
#38533=CARTESIAN_POINT('Ctrl Pts',(-4.52941487992161,1.18514270861202,6.94052705783577));
#38534=CARTESIAN_POINT('Ctrl Pts',(-4.60900164344984,1.30000000000036,6.94788682421141));
#38535=CARTESIAN_POINT('Ctrl Pts',(-4.57618074025569,-1.30000000000007,
6.74410801342415));
#38536=CARTESIAN_POINT('Ctrl Pts',(-4.4945865145068,-1.18514270861183,6.76006832332152));
#38537=CARTESIAN_POINT('Ctrl Pts',(-4.42497743498526,-1.06847604194514,
6.77630653423347));
#38538=CARTESIAN_POINT('Ctrl Pts',(-4.29185462144734,-0.794772684000851,
6.8144620568206));
#38539=CARTESIAN_POINT('Ctrl Pts',(-4.23842533221008,-0.636309800095197,
6.84114616167115));
#38540=CARTESIAN_POINT('Ctrl Pts',(-4.1680089369724,-0.319434907277159,
6.87655595092038));
#38541=CARTESIAN_POINT('Ctrl Pts',(-4.15135127738475,-0.158333333333332,
6.88950117056474));
#38542=CARTESIAN_POINT('Ctrl Pts',(-4.15284929561901,0.158333333333334,
6.91031986218473));
#38543=CARTESIAN_POINT('Ctrl Pts',(-4.17077447432536,0.319434907277167,
6.91718425800275));
#38544=CARTESIAN_POINT('Ctrl Pts',(-4.24471173494722,0.636309800095206,
6.92623606006507));
#38545=CARTESIAN_POINT('Ctrl Pts',(-4.30037517936425,0.79477268400084,6.92167986871433));
#38546=CARTESIAN_POINT('Ctrl Pts',(-4.43719031458343,1.06847604194523,6.93006454131363));
#38547=CARTESIAN_POINT('Ctrl Pts',(-4.50842904308767,1.18514270861202,6.93553065253984));
#38548=CARTESIAN_POINT('Ctrl Pts',(-4.59168429756014,1.30000000000036,6.94283346090678));
#38549=CARTESIAN_POINT('Ctrl Pts',(-4.5643345584895,-1.30000000000007,6.74178132771715));
#38550=CARTESIAN_POINT('Ctrl Pts',(-4.48025898197815,-1.18514270861183,
6.75965397193162));
#38551=CARTESIAN_POINT('Ctrl Pts',(-4.40891552700136,-1.06847604194514,
6.7765256844786));
#38552=CARTESIAN_POINT('Ctrl Pts',(-4.2735116215927,-0.794772684000851,
6.81319036324906));
#38553=CARTESIAN_POINT('Ctrl Pts',(-4.22112140679107,-0.636309800095197,
6.83335514381641));
#38554=CARTESIAN_POINT('Ctrl Pts',(-4.15113790298685,-0.319434907277159,
6.86531247060112));
#38555=CARTESIAN_POINT('Ctrl Pts',(-4.13553292461561,-0.158333333333332,
6.87852588247456));
#38556=CARTESIAN_POINT('Ctrl Pts',(-4.13706908989958,0.158333333333334,
6.89918937141314));
#38557=CARTESIAN_POINT('Ctrl Pts',(-4.15404363487221,0.319434907277167,
6.90577978297536));
#38558=CARTESIAN_POINT('Ctrl Pts',(-4.22749554627324,0.636309800095206,
6.91766357206941));
#38559=CARTESIAN_POINT('Ctrl Pts',(-4.2818545600116,0.79477268400084,6.91848306636869));
#38560=CARTESIAN_POINT('Ctrl Pts',(-4.42096106050366,1.06847604194523,6.92841142118433));
#38561=CARTESIAN_POINT('Ctrl Pts',(-4.49399758639363,1.18514270861202,6.93356194558498));
#38562=CARTESIAN_POINT('Ctrl Pts',(-4.57985658851437,1.30000000000036,6.9395653774684));
#38563=CARTESIAN_POINT('Ctrl Pts',(-4.5567863920968,-1.30000000000007,6.7376557021251));
#38564=CARTESIAN_POINT('Ctrl Pts',(-4.47294375113312,-1.18514270861183,
6.75562267180235));
#38565=CARTESIAN_POINT('Ctrl Pts',(-4.40183404790299,-1.06847604194514,
6.77224083743495));
#38566=CARTESIAN_POINT('Ctrl Pts',(-4.26697204137396,-0.794772684000851,
6.80751611732843));
#38567=CARTESIAN_POINT('Ctrl Pts',(-4.21502126192295,-0.636309800095197,
6.82515306092102));
#38568=CARTESIAN_POINT('Ctrl Pts',(-4.14539022778077,-0.319434907277159,
6.85546104784237));
#38569=CARTESIAN_POINT('Ctrl Pts',(-4.12973531027791,-0.158333333333332,
6.86869015129617));
#38570=CARTESIAN_POINT('Ctrl Pts',(-4.13134197385142,0.158333333333334,
6.88912754932025));
#38571=CARTESIAN_POINT('Ctrl Pts',(-4.14849242828377,0.319434907277167,
6.89520166263495));
#38572=CARTESIAN_POINT('Ctrl Pts',(-4.22162247741411,0.636309800095206,
6.90883342950105));
#38573=CARTESIAN_POINT('Ctrl Pts',(-4.27538846798974,0.79477268400084,6.91325360263786));
#38574=CARTESIAN_POINT('Ctrl Pts',(-4.41396332499183,1.06847604194523,6.92441809265578));
#38575=CARTESIAN_POINT('Ctrl Pts',(-4.48679959516754,1.18514270861202,6.92950399072587));
#38576=CARTESIAN_POINT('Ctrl Pts',(-4.57248821462725,1.30000000000036,6.93484309282242));
#38577=CARTESIAN_POINT('Ctrl Pts',(-4.55678639209675,-1.3,6.73765570212511));
#38578=CARTESIAN_POINT('Ctrl Pts',(-4.47294375113309,-1.18514270861178,
6.75562267180236));
#38579=CARTESIAN_POINT('Ctrl Pts',(-4.40183404790298,-1.06847604194512,
6.77224083743496));
#38580=CARTESIAN_POINT('Ctrl Pts',(-4.26697204137396,-0.794772684000851,
6.80751611732844));
#38581=CARTESIAN_POINT('Ctrl Pts',(-4.21502126192295,-0.636309800095197,
6.82515306092103));
#38582=CARTESIAN_POINT('Ctrl Pts',(-4.14539022778078,-0.319434907277159,
6.85546104784238));
#38583=CARTESIAN_POINT('Ctrl Pts',(-4.12973531027791,-0.158333333333332,
6.86869015129617));
#38584=CARTESIAN_POINT('Ctrl Pts',(-4.13134197385143,0.158333333333334,
6.88912754932026));
#38585=CARTESIAN_POINT('Ctrl Pts',(-4.14849242828378,0.319434907277167,
6.89520166263495));
#38586=CARTESIAN_POINT('Ctrl Pts',(-4.22162247741411,0.636309800095206,
6.90883342950106));
#38587=CARTESIAN_POINT('Ctrl Pts',(-4.27538846798974,0.79477268400084,6.91325360263787));
#38588=CARTESIAN_POINT('Ctrl Pts',(-4.41396332499177,1.06847604194511,6.92441809265578));
#38589=CARTESIAN_POINT('Ctrl Pts',(-4.48679959516739,1.18514270861178,6.92950399072586));
#38590=CARTESIAN_POINT('Ctrl Pts',(-4.57248821462698,1.3,6.9348430928224));
#38591=CARTESIAN_POINT('',(-4.94063975534853,-1.2,6.89573234172909));
#38592=CARTESIAN_POINT('Ctrl Pts',(-4.94063975534853,-1.2,6.89573234172909));
#38593=CARTESIAN_POINT('Ctrl Pts',(-4.92830831155243,-1.21176551971707,
6.88690492025552));
#38594=CARTESIAN_POINT('Ctrl Pts',(-4.90579448474807,-1.23313228472086,
6.86991968472727));
#38595=CARTESIAN_POINT('Ctrl Pts',(-4.8691048329432,-1.26793264545523,6.84416995488295));
#38596=CARTESIAN_POINT('Ctrl Pts',(-4.852984802018,-1.28315106047734,6.83266786163372));
#38597=CARTESIAN_POINT('Ctrl Pts',(-4.83515073493498,-1.29999999995714,
6.82076739212789));
#38598=CARTESIAN_POINT('',(-4.9477910762941,-0.653834841369964,7.0521370060455));
#38599=CARTESIAN_POINT('Ctrl Pts',(-4.94779107633063,-0.653834841368707,
7.05213700603945));
#38600=CARTESIAN_POINT('Ctrl Pts',(-4.94731006149294,-0.717303034099604,
7.03604128893171));
#38601=CARTESIAN_POINT('Ctrl Pts',(-4.94685048132318,-0.764700269087877,
7.0226840845037));
#38602=CARTESIAN_POINT('Ctrl Pts',(-4.94483149264608,-0.949624416438056,
6.97114271915527));
#38603=CARTESIAN_POINT('Ctrl Pts',(-4.94334706810035,-1.0588111413964,6.93969316585301));
#38604=CARTESIAN_POINT('Ctrl Pts',(-4.94063975534853,-1.2,6.89573234172909));
#38605=CARTESIAN_POINT('',(-4.94999291725008,0.653834841531101,7.19162628075116));
#38606=CARTESIAN_POINT('Ctrl Pts',(-4.94999291725008,0.6538348415311,7.19162628075116));
#38607=CARTESIAN_POINT('Ctrl Pts',(-4.912250011592,0.575966548977897,7.17417815530401));
#38608=CARTESIAN_POINT('Ctrl Pts',(-4.88066509636651,0.493631594836088,
7.15874248042179));
#38609=CARTESIAN_POINT('Ctrl Pts',(-4.83632007966695,0.338125780962295,
7.13435355557771));
#38610=CARTESIAN_POINT('Ctrl Pts',(-4.82127653986155,0.265650240170082,
7.12467671828353));
#38611=CARTESIAN_POINT('Ctrl Pts',(-4.80341641242718,0.129710677149378,
7.10809226524267));
#38612=CARTESIAN_POINT('Ctrl Pts',(-4.79913228443917,0.0666218126861097,
7.10101164196315));
#38613=CARTESIAN_POINT('Ctrl Pts',(-4.79855056169654,-0.0595420532764043,
7.08769654216656));
#38614=CARTESIAN_POINT('Ctrl Pts',(-4.80223161155448,-0.122773043896495,
7.0813645288135));
#38615=CARTESIAN_POINT('Ctrl Pts',(-4.81904790002624,-0.260121668515325,
7.06922912756428));
#38616=CARTESIAN_POINT('Ctrl Pts',(-4.83378878852566,-0.333938915625325,
7.06372946172096));
#38617=CARTESIAN_POINT('Ctrl Pts',(-4.87782632754073,-0.491207904091508,
7.05522789406418));
#38618=CARTESIAN_POINT('Ctrl Pts',(-4.90929274037476,-0.574351920194419,
7.05261169456229));
#38619=CARTESIAN_POINT('Ctrl Pts',(-4.94779107625937,-0.653834841386509,
7.05213700599913));
#38620=CARTESIAN_POINT('',(-4.94934251834154,1.2,7.11932388124965));
#38621=CARTESIAN_POINT('Ctrl Pts',(-4.94934251834154,1.2,7.11932388124965));
#38622=CARTESIAN_POINT('Ctrl Pts',(-4.94955640842995,1.13010588871483,7.13244567398384));
#38623=CARTESIAN_POINT('Ctrl Pts',(-4.94975019917868,1.05323215079269,7.14617609376067));
#38624=CARTESIAN_POINT('Ctrl Pts',(-4.94997545250846,0.796441226852581,
7.17972746337783));
#38625=CARTESIAN_POINT('Ctrl Pts',(-4.94998203701647,0.739839576001175,
7.18519460114659));
#38626=CARTESIAN_POINT('Ctrl Pts',(-4.94999291725008,0.653834841531101,
7.19162628075116));
#38627=CARTESIAN_POINT('Ctrl Pts',(-4.84757460734146,1.3,7.04663629419473));
#38628=CARTESIAN_POINT('Ctrl Pts',(-4.8653921765581,1.28256957351368,7.05859758341152));
#38629=CARTESIAN_POINT('Ctrl Pts',(-4.88292805709936,1.26539376702234,7.07133403262219));
#38630=CARTESIAN_POINT('Ctrl Pts',(-4.91697372090008,1.2319240199412,7.09520398665546));
#38631=CARTESIAN_POINT('Ctrl Pts',(-4.93329979248523,1.21583846690231,7.10692202008179));
#38632=CARTESIAN_POINT('Ctrl Pts',(-4.94934251834154,1.2,7.11932388124965));
#38633=CARTESIAN_POINT('Ctrl Pts',(-4.55678639209675,-1.3,6.73765570212511));
#38634=CARTESIAN_POINT('Ctrl Pts',(-4.47294375113309,-1.18514270861178,
6.75562267180236));
#38635=CARTESIAN_POINT('Ctrl Pts',(-4.40183404790297,-1.06847604194512,
6.77224083743496));
#38636=CARTESIAN_POINT('Ctrl Pts',(-4.26697204137396,-0.794772684000851,
6.80751611732844));
#38637=CARTESIAN_POINT('Ctrl Pts',(-4.21502126192295,-0.636309800095197,
6.82515306092102));
#38638=CARTESIAN_POINT('Ctrl Pts',(-4.14539022778077,-0.319434907277159,
6.85546104784237));
#38639=CARTESIAN_POINT('Ctrl Pts',(-4.12973531027791,-0.158333333333332,
6.86869015129617));
#38640=CARTESIAN_POINT('Ctrl Pts',(-4.13134197385143,0.158333333333334,
6.88912754932025));
#38641=CARTESIAN_POINT('Ctrl Pts',(-4.14849242828378,0.319434907277167,
6.89520166263495));
#38642=CARTESIAN_POINT('Ctrl Pts',(-4.22162247741411,0.636309800095206,
6.90883342950106));
#38643=CARTESIAN_POINT('Ctrl Pts',(-4.27538846798974,0.79477268400084,6.91325360263786));
#38644=CARTESIAN_POINT('Ctrl Pts',(-4.41396332499176,1.06847604194511,6.92441809265578));
#38645=CARTESIAN_POINT('Ctrl Pts',(-4.48679959516739,1.18514270861178,6.92950399072586));
#38646=CARTESIAN_POINT('Ctrl Pts',(-4.57248821462698,1.3,6.9348430928224));
#38647=CARTESIAN_POINT('Ctrl Pts',(-4.54709012720593,-1.3,6.66133341362554));
#38648=CARTESIAN_POINT('Ctrl Pts',(-4.46362634796674,-1.18514270861178,
6.68099075863086));
#38649=CARTESIAN_POINT('Ctrl Pts',(-4.39282414406279,-1.06847604194512,
6.69877562607923));
#38650=CARTESIAN_POINT('Ctrl Pts',(-4.25850766107618,-0.794772684000851,
6.73553642999107));
#38651=CARTESIAN_POINT('Ctrl Pts',(-4.20664978510482,-0.636309800095197,
6.75246177897201));
#38652=CARTESIAN_POINT('Ctrl Pts',(-4.1373298362099,-0.319434907277159,
6.78217992765895));
#38653=CARTESIAN_POINT('Ctrl Pts',(-4.12172229231298,-0.158333333333332,
6.79416838307638));
#38654=CARTESIAN_POINT('Ctrl Pts',(-4.12368594131515,0.158333333333334,
6.81456826041998));
#38655=CARTESIAN_POINT('Ctrl Pts',(-4.14114067935745,0.319434907277167,
6.8218460611083));
#38656=CARTESIAN_POINT('Ctrl Pts',(-4.21469765004064,0.636309800095206,
6.83599009856847));
#38657=CARTESIAN_POINT('Ctrl Pts',(-4.26870246277087,0.79477268400084,6.84108700054781));
#38658=CARTESIAN_POINT('Ctrl Pts',(-4.40750206450663,1.06847604194511,6.85068500808925));
#38659=CARTESIAN_POINT('Ctrl Pts',(-4.48039654346317,1.18514270861178,6.85456576687264));
#38660=CARTESIAN_POINT('Ctrl Pts',(-4.56610429681699,1.3,6.85817266261596));
#38661=CARTESIAN_POINT('Ctrl Pts',(-4.53739386231511,-1.3,6.58501112512596));
#38662=CARTESIAN_POINT('Ctrl Pts',(-4.45430894480039,-1.18514270861178,
6.60635884545937));
#38663=CARTESIAN_POINT('Ctrl Pts',(-4.38381424022261,-1.06847604194512,
6.6253104147235));
#38664=CARTESIAN_POINT('Ctrl Pts',(-4.2500432807784,-0.794772684000851,
6.6635567426537));
#38665=CARTESIAN_POINT('Ctrl Pts',(-4.19827830828669,-0.636309800095197,
6.67977049702301));
#38666=CARTESIAN_POINT('Ctrl Pts',(-4.12926944463902,-0.319434907277159,
6.70889880747553));
#38667=CARTESIAN_POINT('Ctrl Pts',(-4.11370927434805,-0.158333333333332,
6.71964661485658));
#38668=CARTESIAN_POINT('Ctrl Pts',(-4.11602990877888,0.158333333333334,
6.74000897151971));
#38669=CARTESIAN_POINT('Ctrl Pts',(-4.13378893043113,0.319434907277167,
6.74849045958165));
#38670=CARTESIAN_POINT('Ctrl Pts',(-4.20777282266716,0.636309800095206,
6.76314676763588));
#38671=CARTESIAN_POINT('Ctrl Pts',(-4.262016457552,0.79477268400084,6.76892039845776));
#38672=CARTESIAN_POINT('Ctrl Pts',(-4.40104080402149,1.06847604194511,6.77695192352273));
#38673=CARTESIAN_POINT('Ctrl Pts',(-4.47399349175896,1.18514270861178,6.77962754301942));
#38674=CARTESIAN_POINT('Ctrl Pts',(-4.559720379007,1.3,6.78150223240952));
#38675=CARTESIAN_POINT('Ctrl Pts',(-4.52769759742428,-1.3,6.50868883662639));
#38676=CARTESIAN_POINT('Ctrl Pts',(-4.44499154163403,-1.18514270861178,
6.53172693228787));
#38677=CARTESIAN_POINT('Ctrl Pts',(-4.37480433638243,-1.06847604194512,
6.55184520336777));
#38678=CARTESIAN_POINT('Ctrl Pts',(-4.24157890048062,-0.794772684000851,
6.59157705531633));
#38679=CARTESIAN_POINT('Ctrl Pts',(-4.18990683146856,-0.636309800095197,
6.607079215074));
#38680=CARTESIAN_POINT('Ctrl Pts',(-4.12120905306814,-0.319434907277159,
6.63561768729211));
#38681=CARTESIAN_POINT('Ctrl Pts',(-4.10569625638312,-0.158333333333332,
6.64512484663679));
#38682=CARTESIAN_POINT('Ctrl Pts',(-4.1083738762426,0.158333333333334,6.66544968261944));
#38683=CARTESIAN_POINT('Ctrl Pts',(-4.1264371815048,0.319434907277167,6.67513485805499));
#38684=CARTESIAN_POINT('Ctrl Pts',(-4.20084799529369,0.636309800095206,
6.6903034367033));
#38685=CARTESIAN_POINT('Ctrl Pts',(-4.25533045233312,0.79477268400084,6.6967537963677));
#38686=CARTESIAN_POINT('Ctrl Pts',(-4.39457954353636,1.06847604194511,6.70321883895621));
#38687=CARTESIAN_POINT('Ctrl Pts',(-4.46759044005475,1.18514270861178,6.7046893191662));
#38688=CARTESIAN_POINT('Ctrl Pts',(-4.55333646119701,1.3,6.70483180220308));
#38689=CARTESIAN_POINT('Ctrl Pts',(-4.52769759742429,-1.3,6.50868883662639));
#38690=CARTESIAN_POINT('Ctrl Pts',(-4.44499154163404,-1.18514270861178,
6.53172693228787));
#38691=CARTESIAN_POINT('Ctrl Pts',(-4.37480433638243,-1.06847604194512,
6.55184520336777));
#38692=CARTESIAN_POINT('Ctrl Pts',(-4.24157890048062,-0.794772684000851,
6.59157705531633));
#38693=CARTESIAN_POINT('Ctrl Pts',(-4.18990683146856,-0.636309800095197,
6.607079215074));
#38694=CARTESIAN_POINT('Ctrl Pts',(-4.12120905306814,-0.319434907277159,
6.63561768729212));
#38695=CARTESIAN_POINT('Ctrl Pts',(-4.10569625638312,-0.158333333333332,
6.64512484663679));
#38696=CARTESIAN_POINT('Ctrl Pts',(-4.1083738762426,0.158333333333334,6.66544968261944));
#38697=CARTESIAN_POINT('Ctrl Pts',(-4.1264371815048,0.319434907277167,6.675134858055));
#38698=CARTESIAN_POINT('Ctrl Pts',(-4.20084799529369,0.636309800095206,
6.6903034367033));
#38699=CARTESIAN_POINT('Ctrl Pts',(-4.25533045233312,0.79477268400084,6.69675379636771));
#38700=CARTESIAN_POINT('Ctrl Pts',(-4.39457954353635,1.06847604194511,6.70321883895621));
#38701=CARTESIAN_POINT('Ctrl Pts',(-4.46759044005475,1.18514270861178,6.7046893191662));
#38702=CARTESIAN_POINT('Ctrl Pts',(-4.55333646119701,1.3,6.70483180220308));
#38703=CARTESIAN_POINT('Ctrl Pts',(-4.52769759742576,-1.30000000000204,
6.50868883662598));
#38704=CARTESIAN_POINT('Ctrl Pts',(-4.44499154163487,-1.18514270861317,
6.53172693228763));
#38705=CARTESIAN_POINT('Ctrl Pts',(-4.37480433638277,-1.06847604194582,
6.55184520336767));
#38706=CARTESIAN_POINT('Ctrl Pts',(-4.24157890048062,-0.794772684000851,
6.59157705531633));
#38707=CARTESIAN_POINT('Ctrl Pts',(-4.18990683146856,-0.636309800095197,
6.607079215074));
#38708=CARTESIAN_POINT('Ctrl Pts',(-4.12120905306814,-0.319434907277159,
6.63561768729212));
#38709=CARTESIAN_POINT('Ctrl Pts',(-4.10569625638313,-0.158333333333332,
6.64512484663679));
#38710=CARTESIAN_POINT('Ctrl Pts',(-4.10837387624261,0.158333333333334,
6.66544968261944));
#38711=CARTESIAN_POINT('Ctrl Pts',(-4.1264371815048,0.319434907277167,6.675134858055));
#38712=CARTESIAN_POINT('Ctrl Pts',(-4.20084799529369,0.636309800095206,
6.6903034367033));
#38713=CARTESIAN_POINT('Ctrl Pts',(-4.25533045233312,0.79477268400084,6.69675379636771));
#38714=CARTESIAN_POINT('Ctrl Pts',(-4.39457954353638,1.06847604194515,6.70321883895621));
#38715=CARTESIAN_POINT('Ctrl Pts',(-4.4675904400548,1.18514270861186,6.70468931916621));
#38716=CARTESIAN_POINT('Ctrl Pts',(-4.55333646119711,1.30000000000013,6.70483180220308));
#38717=CARTESIAN_POINT('Ctrl Pts',(-4.5339231364204,-1.30000000000204,6.50253777416358));
#38718=CARTESIAN_POINT('Ctrl Pts',(-4.45118854317515,-1.18514270861317,
6.52626110695818));
#38719=CARTESIAN_POINT('Ctrl Pts',(-4.3808188948516,-1.06847604194582,6.54648422763159));
#38720=CARTESIAN_POINT('Ctrl Pts',(-4.24681642619259,-0.794772684000851,
6.58511749179351));
#38721=CARTESIAN_POINT('Ctrl Pts',(-4.19381566978082,-0.636309800095197,
6.59722095263262));
#38722=CARTESIAN_POINT('Ctrl Pts',(-4.12443963753454,-0.319434907277159,
6.62411656351865));
#38723=CARTESIAN_POINT('Ctrl Pts',(-4.10920625064663,-0.158333333333332,
6.63409216512955));
#38724=CARTESIAN_POINT('Ctrl Pts',(-4.11199983518693,0.158333333333334,
6.65462349397901));
#38725=CARTESIAN_POINT('Ctrl Pts',(-4.13001103020958,0.319434907277167,
6.66430370365475));
#38726=CARTESIAN_POINT('Ctrl Pts',(-4.20510952842189,0.636309800095206,
6.68101229756646));
#38727=CARTESIAN_POINT('Ctrl Pts',(-4.26054738494527,0.79477268400084,6.68984389115715));
#38728=CARTESIAN_POINT('Ctrl Pts',(-4.40061540550435,1.06847604194515,6.69755530381139));
#38729=CARTESIAN_POINT('Ctrl Pts',(-4.47390766109767,1.18514270861186,6.69922519060665));
#38730=CARTESIAN_POINT('Ctrl Pts',(-4.55986191621595,1.30000000000013,6.69922697939514));
#38731=CARTESIAN_POINT('Ctrl Pts',(-4.5448135895363,-1.30000000000205,6.49689772508368));
#38732=CARTESIAN_POINT('Ctrl Pts',(-4.46489006285245,-1.18514270861317,
6.52135155288484));
#38733=CARTESIAN_POINT('Ctrl Pts',(-4.39633993528005,-1.06847604194582,
6.54150917877332));
#38734=CARTESIAN_POINT('Ctrl Pts',(-4.2642502543703,-0.794772684000855,
6.57815224122436));
#38735=CARTESIAN_POINT('Ctrl Pts',(-4.20885493857128,-0.636309800095198,
6.5852607203308));
#38736=CARTESIAN_POINT('Ctrl Pts',(-4.13841391482442,-0.319434907277159,
6.60948142826875));
#38737=CARTESIAN_POINT('Ctrl Pts',(-4.12230889881553,-0.158333333333333,
6.61991362476384));
#38738=CARTESIAN_POINT('Ctrl Pts',(-4.12517372525979,0.158333333333335,
6.64060379659608));
#38739=CARTESIAN_POINT('Ctrl Pts',(-4.14416327229731,0.319434907277169,
6.64985058645173));
#38740=CARTESIAN_POINT('Ctrl Pts',(-4.22039960441716,0.636309800095208,
6.66983398081229));
#38741=CARTESIAN_POINT('Ctrl Pts',(-4.27819317135791,0.794772684000841,
6.68474632087806));
#38742=CARTESIAN_POINT('Ctrl Pts',(-4.41634586929662,1.06847604194516,6.69438203741767));
#38743=CARTESIAN_POINT('Ctrl Pts',(-4.48781729178234,1.18514270861187,6.69580424692545));
#38744=CARTESIAN_POINT('Ctrl Pts',(-4.57095895287809,1.30000000000013,6.69447772128951));
#38745=CARTESIAN_POINT('Ctrl Pts',(-4.56073742191317,-1.30000000000205,
6.48845909030144));
#38746=CARTESIAN_POINT('Ctrl Pts',(-4.48442192180763,-1.18514270861317,
6.51220615399741));
#38747=CARTESIAN_POINT('Ctrl Pts',(-4.41848591804469,-1.06847604194582,
6.53163817724403));
#38748=CARTESIAN_POINT('Ctrl Pts',(-4.29013927186283,-0.794772684000854,
6.56656143164765));
#38749=CARTESIAN_POINT('Ctrl Pts',(-4.23392409411188,-0.636309800095199,
6.57229155951987));
#38750=CARTESIAN_POINT('Ctrl Pts',(-4.16337899081417,-0.319434907277161,
6.59519730954064));
#38751=CARTESIAN_POINT('Ctrl Pts',(-4.14586384459553,-0.158333333333333,
6.60524152164129));
#38752=CARTESIAN_POINT('Ctrl Pts',(-4.14872383855016,0.158333333333335,
6.62601326414715));
#38753=CARTESIAN_POINT('Ctrl Pts',(-4.16903064643432,0.319434907277169,
6.63539167526));
#38754=CARTESIAN_POINT('Ctrl Pts',(-4.24554053944403,0.636309800095209,
6.65754452796728));
#38755=CARTESIAN_POINT('Ctrl Pts',(-4.30456094488862,0.794772684000844,
6.67570553640629));
#38756=CARTESIAN_POINT('Ctrl Pts',(-4.43905798432154,1.06847604194516,6.68721928376245));
#38757=CARTESIAN_POINT('Ctrl Pts',(-4.50787657003776,1.18514270861187,6.68902278901192));
#38758=CARTESIAN_POINT('Ctrl Pts',(-4.58729495670616,1.30000000000014,6.68764592490677));
#38759=CARTESIAN_POINT('Ctrl Pts',(-4.57384637688119,-1.30000000000206,
6.48122083117096));
#38760=CARTESIAN_POINT('Ctrl Pts',(-4.5001190698821,-1.18514270861318,6.50404878417318));
#38761=CARTESIAN_POINT('Ctrl Pts',(-4.43609853906568,-1.06847604194583,
6.52295418356865));
#38762=CARTESIAN_POINT('Ctrl Pts',(-4.31062290043274,-0.794772684000857,
6.55756755464857));
#38763=CARTESIAN_POINT('Ctrl Pts',(-4.25420802456576,-0.636309800095198,
6.56504532209082));
#38764=CARTESIAN_POINT('Ctrl Pts',(-4.18364678301027,-0.319434907277158,
6.58779809546497));
#38765=CARTESIAN_POINT('Ctrl Pts',(-4.16483643709211,-0.158333333333333,
6.59633856424103));
#38766=CARTESIAN_POINT('Ctrl Pts',(-4.16756733952373,0.158333333333335,
6.61660382348019));
#38767=CARTESIAN_POINT('Ctrl Pts',(-4.18885460237251,0.319434907277171,
6.6261653388731));
#38768=CARTESIAN_POINT('Ctrl Pts',(-4.26549584572766,0.636309800095211,
6.64909787497906));
#38769=CARTESIAN_POINT('Ctrl Pts',(-4.32535183742634,0.79477268400084,6.66851424753936));
#38770=CARTESIAN_POINT('Ctrl Pts',(-4.45711939879762,1.06847604194516,6.68079853180302));
#38771=CARTESIAN_POINT('Ctrl Pts',(-4.52398008152087,1.18514270861187,6.68278444915833));
#38772=CARTESIAN_POINT('Ctrl Pts',(-4.60066415211911,1.30000000000014,6.68143887238882));
#38773=CARTESIAN_POINT('Ctrl Pts',(-4.58698656110146,-1.30000000000206,
6.47361713730369));
#38774=CARTESIAN_POINT('Ctrl Pts',(-4.51610414428804,-1.18514270861318,
6.49542637411433));
#38775=CARTESIAN_POINT('Ctrl Pts',(-4.4542087767042,-1.06847604194583,6.51376238589569));
#38776=CARTESIAN_POINT('Ctrl Pts',(-4.33197997703341,-0.794772684000859,
6.54809839658323));
#38777=CARTESIAN_POINT('Ctrl Pts',(-4.27543672620479,-0.636309800095201,
6.55735169090154));
#38778=CARTESIAN_POINT('Ctrl Pts',(-4.20508111331027,-0.31943490727716,
6.58054420274352));
#38779=CARTESIAN_POINT('Ctrl Pts',(-4.18500629610171,-0.158333333333334,
6.58803931713282));
#38780=CARTESIAN_POINT('Ctrl Pts',(-4.18787298644458,0.158333333333336,
6.60908156055377));
#38781=CARTESIAN_POINT('Ctrl Pts',(-4.21062555247697,0.319434907277171,
6.62089441202161));
#38782=CARTESIAN_POINT('Ctrl Pts',(-4.2872052674614,0.636309800095212,6.64409603346161));
#38783=CARTESIAN_POINT('Ctrl Pts',(-4.34714661054135,0.794772684000845,
6.66132220693935));
#38784=CARTESIAN_POINT('Ctrl Pts',(-4.4756319386759,1.06847604194516,6.67344753163792));
#38785=CARTESIAN_POINT('Ctrl Pts',(-4.54033845160057,1.18514270861187,6.67572832282236));
#38786=CARTESIAN_POINT('Ctrl Pts',(-4.61413493975109,1.30000000000014,6.6750413014168));
#38787=CARTESIAN_POINT('Ctrl Pts',(-4.59716171915453,-1.30000000000206,
6.46668272213426));
#38788=CARTESIAN_POINT('Ctrl Pts',(-4.52841185704875,-1.18514270861318,
6.48767753331008));
#38789=CARTESIAN_POINT('Ctrl Pts',(-4.46812366280871,-1.06847604194583,
6.50561171696502));
#38790=CARTESIAN_POINT('Ctrl Pts',(-4.34839401902338,-0.79477268400086,
6.5399726070793));
#38791=CARTESIAN_POINT('Ctrl Pts',(-4.29179822741274,-0.636309800095201,
6.55075275265294));
#38792=CARTESIAN_POINT('Ctrl Pts',(-4.22179938955352,-0.31943490727716,
6.57517535074014));
#38793=CARTESIAN_POINT('Ctrl Pts',(-4.20108843781605,-0.158333333333334,
6.58327406446806));
#38794=CARTESIAN_POINT('Ctrl Pts',(-4.20406498716468,0.158333333333336,
6.60498790748946));
#38795=CARTESIAN_POINT('Ctrl Pts',(-4.22760153990135,0.319434907277171,
6.61722407555977));
#38796=CARTESIAN_POINT('Ctrl Pts',(-4.30397086538426,0.636309800095213,
6.63983985698167));
#38797=CARTESIAN_POINT('Ctrl Pts',(-4.36393959524977,0.794772684000845,
6.65501862934024));
#38798=CARTESIAN_POINT('Ctrl Pts',(-4.49001682200018,1.06847604194516,6.66717258273725));
#38799=CARTESIAN_POINT('Ctrl Pts',(-4.55316604490403,1.18514270861187,6.66992754548968));
#38800=CARTESIAN_POINT('Ctrl Pts',(-4.62489033087317,1.30000000000014,6.67017647491734));
#38801=CARTESIAN_POINT('Ctrl Pts',(-4.6074622528922,-1.30000000000206,6.4600435350283));
#38802=CARTESIAN_POINT('Ctrl Pts',(-4.54095552050019,-1.18514270861318,
6.48037531005611));
#38803=CARTESIAN_POINT('Ctrl Pts',(-4.48234277686481,-1.06847604194583,
6.49797291440743));
#38804=CARTESIAN_POINT('Ctrl Pts',(-4.36517230684305,-0.794772684000862,
6.53231041961595));
#38805=CARTESIAN_POINT('Ctrl Pts',(-4.3084061450825,-0.636309800095201,
6.54422769854724));
#38806=CARTESIAN_POINT('Ctrl Pts',(-4.23870137528444,-0.31943490727716,
6.56966697083763));
#38807=CARTESIAN_POINT('Ctrl Pts',(-4.21736580827584,-0.158333333333334,
6.5786460731632));
#38808=CARTESIAN_POINT('Ctrl Pts',(-4.22034314131664,0.158333333333336,
6.60043051355548));
#38809=CARTESIAN_POINT('Ctrl Pts',(-4.24445058191402,0.319434907277172,
6.61166749200678));
#38810=CARTESIAN_POINT('Ctrl Pts',(-4.32063847085125,0.636309800095213,
6.63379619187466));
#38811=CARTESIAN_POINT('Ctrl Pts',(-4.38101305593257,0.794772684000846,
6.64887344683999));
#38812=CARTESIAN_POINT('Ctrl Pts',(-4.50462812710003,1.06847604194516,6.66125269831112));
#38813=CARTESIAN_POINT('Ctrl Pts',(-4.56610840349878,1.18514270861187,6.66422266738462));
#38814=CARTESIAN_POINT('Ctrl Pts',(-4.6355605723777,1.30000000000014,6.66480408626625));
#38815=CARTESIAN_POINT('Ctrl Pts',(-4.62576982567855,-1.30000000000206,
6.44950879919769));
#38816=CARTESIAN_POINT('Ctrl Pts',(-4.56297469544779,-1.18514270861318,
6.46813363441796));
#38817=CARTESIAN_POINT('Ctrl Pts',(-4.50713158452972,-1.06847604194583,
6.48470193121604));
#38818=CARTESIAN_POINT('Ctrl Pts',(-4.39418338229227,-0.794772684000863,
6.51822699613158));
#38819=CARTESIAN_POINT('Ctrl Pts',(-4.33711557690431,-0.636309800095203,
6.53196081109196));
#38820=CARTESIAN_POINT('Ctrl Pts',(-4.26788192627813,-0.319434907277161,
6.55887662222457));
#38821=CARTESIAN_POINT('Ctrl Pts',(-4.24541656673626,-0.158333333333334,
6.56894597707075));
#38822=CARTESIAN_POINT('Ctrl Pts',(-4.24857776470334,0.158333333333336,
6.59172388317241));
#38823=CARTESIAN_POINT('Ctrl Pts',(-4.27412252605687,0.319434907277173,
6.6035729289362));
#38824=CARTESIAN_POINT('Ctrl Pts',(-4.34996192220723,0.636309800095215,
6.62480482326914));
#38825=CARTESIAN_POINT('Ctrl Pts',(-4.41041420828552,0.794772684000848,
6.63676577957294));
#38826=CARTESIAN_POINT('Ctrl Pts',(-4.52971866708554,1.06847604194516,6.64925831825317));
#38827=CARTESIAN_POINT('Ctrl Pts',(-4.58840297499466,1.18514270861187,6.65299604768975));
#38828=CARTESIAN_POINT('Ctrl Pts',(-4.65412911126427,1.30000000000014,6.65506394946243));
#38829=CARTESIAN_POINT('Ctrl Pts',(-4.65102959463181,-1.30000000000207,
6.43149214232983));
#38830=CARTESIAN_POINT('Ctrl Pts',(-4.59342345447021,-1.18514270861319,
6.44725725954069));
#38831=CARTESIAN_POINT('Ctrl Pts',(-4.54151473414863,-1.06847604194584,
6.46223724960806));
#38832=CARTESIAN_POINT('Ctrl Pts',(-4.43475738549757,-0.794772684000863,
6.49503022263472));
#38833=CARTESIAN_POINT('Ctrl Pts',(-4.37775267111089,-0.636309800095206,
6.5129043391861));
#38834=CARTESIAN_POINT('Ctrl Pts',(-4.30949729821618,-0.319434907277163,
6.54291781500037));
#38835=CARTESIAN_POINT('Ctrl Pts',(-4.28555768686207,-0.158333333333335,
6.55527121133622));
#38836=CARTESIAN_POINT('Ctrl Pts',(-4.28879291291088,0.158333333333337,
6.57850141380386));
#38837=CARTESIAN_POINT('Ctrl Pts',(-4.31572986483542,0.319434907277173,
6.58808755367647));
#38838=CARTESIAN_POINT('Ctrl Pts',(-4.39105971583867,0.636309800095217,
6.60802132189756));
#38839=CARTESIAN_POINT('Ctrl Pts',(-4.45231395200949,0.794772684000851,
6.61885578366433));
#38840=CARTESIAN_POINT('Ctrl Pts',(-4.56563152943194,1.06847604194517,6.63244916713826));
#38841=CARTESIAN_POINT('Ctrl Pts',(-4.62030035672222,1.18514270861188,6.63725293761837));
#38842=CARTESIAN_POINT('Ctrl Pts',(-4.68058703086667,1.30000000000015,6.64097640655724));
#38843=CARTESIAN_POINT('Ctrl Pts',(-4.67660141836003,-1.30000000000208,
6.41469238425056));
#38844=CARTESIAN_POINT('Ctrl Pts',(-4.6244180160509,-1.1851427086132,6.42841838267233));
#38845=CARTESIAN_POINT('Ctrl Pts',(-4.57650422860925,-1.06847604194585,
6.44201135867463));
#38846=CARTESIAN_POINT('Ctrl Pts',(-4.47567745897646,-0.794772684000876,
6.47310654410536));
#38847=CARTESIAN_POINT('Ctrl Pts',(-4.41774861709085,-0.636309800095216,
6.49162551861622));
#38848=CARTESIAN_POINT('Ctrl Pts',(-4.35007866327408,-0.319434907277168,
6.52318622767854));
#38849=CARTESIAN_POINT('Ctrl Pts',(-4.32485665302354,-0.158333333333337,
6.53819614711616));
#38850=CARTESIAN_POINT('Ctrl Pts',(-4.32837761003057,0.158333333333339,
6.56267337539902));
#38851=CARTESIAN_POINT('Ctrl Pts',(-4.35705261249353,0.319434907277178,
6.57163732124803));
#38852=CARTESIAN_POINT('Ctrl Pts',(-4.43203294160927,0.636309800095227,
6.59096027795895));
#38853=CARTESIAN_POINT('Ctrl Pts',(-4.49385171345939,0.794772684000865,
6.59960001635686));
#38854=CARTESIAN_POINT('Ctrl Pts',(-4.60132980001507,1.06847604194518,6.61482716747228));
#38855=CARTESIAN_POINT('Ctrl Pts',(-4.65210969249407,1.1851427086119,6.6211845265236));
#38856=CARTESIAN_POINT('Ctrl Pts',(-4.70714619623773,1.30000000000016,6.62730797512994));
#38857=CARTESIAN_POINT('Ctrl Pts',(-4.69671938666277,-1.30000000000209,
6.40019410542714));
#38858=CARTESIAN_POINT('Ctrl Pts',(-4.64842311742148,-1.1851427086132,6.41087046079619));
#38859=CARTESIAN_POINT('Ctrl Pts',(-4.6034504998882,-1.06847604194585,6.42254637528841));
#38860=CARTESIAN_POINT('Ctrl Pts',(-4.5072330569851,-0.794772684000877,
6.45182925505966));
#38861=CARTESIAN_POINT('Ctrl Pts',(-4.44928913645816,-0.636309800095218,
6.47312960657745));
#38862=CARTESIAN_POINT('Ctrl Pts',(-4.38234940217106,-0.31943490727717,
6.50664610297841));
#38863=CARTESIAN_POINT('Ctrl Pts',(-4.35602518955894,-0.158333333333338,
6.52343144267528));
#38864=CARTESIAN_POINT('Ctrl Pts',(-4.35973297066254,0.15833333333334,6.54864062035165));
#38865=CARTESIAN_POINT('Ctrl Pts',(-4.38969701810412,0.319434907277179,
6.55667724125419));
#38866=CARTESIAN_POINT('Ctrl Pts',(-4.46432763719829,0.636309800095229,
6.57529875796418));
#38867=CARTESIAN_POINT('Ctrl Pts',(-4.52658608900722,0.794772684000869,
6.58231619209787));
#38868=CARTESIAN_POINT('Ctrl Pts',(-4.62938916242825,1.06847604194519,6.59890314423408));
#38869=CARTESIAN_POINT('Ctrl Pts',(-4.67706492192611,1.1851427086119,6.60653296645766));
#38870=CARTESIAN_POINT('Ctrl Pts',(-4.72791679966716,1.30000000000016,6.61461273393221));
#38871=CARTESIAN_POINT('Ctrl Pts',(-4.70923780805004,-1.3000000000021,6.39102177259869));
#38872=CARTESIAN_POINT('Ctrl Pts',(-4.6635969880334,-1.18514270861322,6.40051570703614));
#38873=CARTESIAN_POINT('Ctrl Pts',(-4.62060190244937,-1.06847604194587,
6.41144232091127));
#38874=CARTESIAN_POINT('Ctrl Pts',(-4.52738682942984,-0.794772684000888,
6.43999476093189));
#38875=CARTESIAN_POINT('Ctrl Pts',(-4.46920699193414,-0.636309800095222,
6.46234118216104));
#38876=CARTESIAN_POINT('Ctrl Pts',(-4.4025623868709,-0.31943490727717,6.49655685460303));
#38877=CARTESIAN_POINT('Ctrl Pts',(-4.37541513495486,-0.158333333333339,
6.51397711161568));
#38878=CARTESIAN_POINT('Ctrl Pts',(-4.37917902611795,0.158333333333341,
6.53943833931756));
#38879=CARTESIAN_POINT('Ctrl Pts',(-4.40997661151049,0.319434907277181,
6.54698729143357));
#38880=CARTESIAN_POINT('Ctrl Pts',(-4.48451930069498,0.636309800095233,
6.56563651295819));
#38881=CARTESIAN_POINT('Ctrl Pts',(-4.5473088792165,0.794772684000871,6.57257058558995));
#38882=CARTESIAN_POINT('Ctrl Pts',(-4.6472204427376,1.0684760419452,6.59009146329908));
#38883=CARTESIAN_POINT('Ctrl Pts',(-4.69291326935205,1.18514270861191,6.59834469554946));
#38884=CARTESIAN_POINT('Ctrl Pts',(-4.74105090882094,1.30000000000018,6.60726702130246));
#38885=CARTESIAN_POINT('Ctrl Pts',(-4.71915423907025,-1.3000000000021,6.38338868641404));
#38886=CARTESIAN_POINT('Ctrl Pts',(-4.67558438284768,-1.18514270861322,
6.39176024939273));
#38887=CARTESIAN_POINT('Ctrl Pts',(-4.6341320352647,-1.06847604194586,6.4019526285067));
#38888=CARTESIAN_POINT('Ctrl Pts',(-4.54326068839814,-0.794772684000886,
6.4297055127638));
#38889=CARTESIAN_POINT('Ctrl Pts',(-4.48488407740131,-0.636309800095222,
6.45283233370657));
#38890=CARTESIAN_POINT('Ctrl Pts',(-4.4185044797531,-0.319434907277171,
6.48765999012121));
#38891=CARTESIAN_POINT('Ctrl Pts',(-4.39077257383743,-0.158333333333339,
6.50579668879949));
#38892=CARTESIAN_POINT('Ctrl Pts',(-4.39462161644564,0.158333333333341,
6.53157765106085));
#38893=CARTESIAN_POINT('Ctrl Pts',(-4.42611643536731,0.31943490727718,6.5388660264981));
#38894=CARTESIAN_POINT('Ctrl Pts',(-4.50051169546631,0.636309800095232,
6.55727725244718));
#38895=CARTESIAN_POINT('Ctrl Pts',(-4.56348191940118,0.794772684000872,
6.56327773993498));
#38896=CARTESIAN_POINT('Ctrl Pts',(-4.66113327163995,1.0684760419452,6.5817654056829));
#38897=CARTESIAN_POINT('Ctrl Pts',(-4.70532941426806,1.18514270861191,6.59085487148191));
#38898=CARTESIAN_POINT('Ctrl Pts',(-4.75145204747931,1.30000000000018,6.60103117761319));
#38899=CARTESIAN_POINT('Ctrl Pts',(-4.72667488592144,-1.3000000000021,6.37792955793686));
#38900=CARTESIAN_POINT('Ctrl Pts',(-4.68456043694553,-1.18514270861322,
6.38516989090598));
#38901=CARTESIAN_POINT('Ctrl Pts',(-4.64420101572682,-1.06847604194587,
6.39462061151743));
#38902=CARTESIAN_POINT('Ctrl Pts',(-4.55501714404858,-0.79477268400089,
6.42156010438024));
#38903=CARTESIAN_POINT('Ctrl Pts',(-4.49655799527695,-0.636309800095224,
6.44544341871139));
#38904=CARTESIAN_POINT('Ctrl Pts',(-4.43043350640925,-0.319434907277171,
6.48091370749242));
#38905=CARTESIAN_POINT('Ctrl Pts',(-4.40235455693084,-0.158333333333339,
6.4999227553353));
#38906=CARTESIAN_POINT('Ctrl Pts',(-4.40625515181025,0.158333333333341,
6.52588892814653));
#38907=CARTESIAN_POINT('Ctrl Pts',(-4.43815605035426,0.319434907277181,
6.53254907422115));
#38908=CARTESIAN_POINT('Ctrl Pts',(-4.51238596599926,0.636309800095234,
6.55057493445345));
#38909=CARTESIAN_POINT('Ctrl Pts',(-4.57552966840074,0.794772684000873,
6.55601893442645));
#38910=CARTESIAN_POINT('Ctrl Pts',(-4.67145177573476,1.0684760419452,6.57509412671058));
#38911=CARTESIAN_POINT('Ctrl Pts',(-4.71450117951397,1.18514270861191,6.58471346725663));
#38912=CARTESIAN_POINT('Ctrl Pts',(-4.75907886107186,1.30000000000018,6.59569520441448));
#38913=CARTESIAN_POINT('Ctrl Pts',(-4.734255397592,-1.3000000000021,6.37265708709577));
#38914=CARTESIAN_POINT('Ctrl Pts',(-4.69358239480132,-1.18514270861322,
6.37873089092264));
#38915=CARTESIAN_POINT('Ctrl Pts',(-4.65430406422572,-1.06847604194587,
6.38740850709591));
#38916=CARTESIAN_POINT('Ctrl Pts',(-4.56678523481327,-0.79477268400089,
6.41347086381832));
#38917=CARTESIAN_POINT('Ctrl Pts',(-4.50823028163824,-0.636309800095224,
6.43806485257171));
#38918=CARTESIAN_POINT('Ctrl Pts',(-4.44235847902296,-0.319434907277172,
6.47416472709407));
#38919=CARTESIAN_POINT('Ctrl Pts',(-4.41392972446464,-0.158333333333339,
6.49401963091343));
#38920=CARTESIAN_POINT('Ctrl Pts',(-4.41792639169605,0.158333333333341,
6.52032614564209));
#38921=CARTESIAN_POINT('Ctrl Pts',(-4.4502860278473,0.319434907277181,6.52655417793902));
#38922=CARTESIAN_POINT('Ctrl Pts',(-4.52443275445227,0.636309800095234,
6.54449419332223));
#38923=CARTESIAN_POINT('Ctrl Pts',(-4.58781814377579,0.794772684000874,
6.54962033414097));
#38924=CARTESIAN_POINT('Ctrl Pts',(-4.68204912169694,1.0684760419452,6.56943868959626));
#38925=CARTESIAN_POINT('Ctrl Pts',(-4.7239553147106,1.18514270861191,6.57961360926114));
#38926=CARTESIAN_POINT('Ctrl Pts',(-4.7669786019977,1.30000000000018,6.59138481685674));
#38927=CARTESIAN_POINT('Ctrl Pts',(-4.74915526276146,-1.30000000000211,
6.36133152319297));
#38928=CARTESIAN_POINT('Ctrl Pts',(-4.71159373872046,-1.18514270861323,
6.36574451713122));
#38929=CARTESIAN_POINT('Ctrl Pts',(-4.67463144480465,-1.06847604194587,
6.37333227298729));
#38930=CARTESIAN_POINT('Ctrl Pts',(-4.59062549304262,-0.794772684000893,
6.39819584207924));
#38931=CARTESIAN_POINT('Ctrl Pts',(-4.53177671566121,-0.636309800095225,
6.42396941101353));
#38932=CARTESIAN_POINT('Ctrl Pts',(-4.46626236278133,-0.319434907277171,
6.46085697245643));
#38933=CARTESIAN_POINT('Ctrl Pts',(-4.43694193193331,-0.158333333333339,
6.48174434943689));
#38934=CARTESIAN_POINT('Ctrl Pts',(-4.44094155352027,0.158333333333341,
6.50809496769723));
#38935=CARTESIAN_POINT('Ctrl Pts',(-4.47410752652201,0.319434907277183,
6.51308535134564));
#38936=CARTESIAN_POINT('Ctrl Pts',(-4.54808266930368,0.636309800095236,
6.53083527893999));
#38937=CARTESIAN_POINT('Ctrl Pts',(-4.61211578504224,0.794772684000874,
6.53588389196195));
#38938=CARTESIAN_POINT('Ctrl Pts',(-4.70304571945319,1.0684760419452,6.55744846867296));
#38939=CARTESIAN_POINT('Ctrl Pts',(-4.7426871346182,1.18514270861191,6.56879771750923));
#38940=CARTESIAN_POINT('Ctrl Pts',(-4.78260976562786,1.30000000000019,6.58216170896991));
#38941=CARTESIAN_POINT('Ctrl Pts',(-4.76634878519204,-1.30000000000213,
6.3476858866717));
#38942=CARTESIAN_POINT('Ctrl Pts',(-4.73196573478673,-1.18514270861324,
6.34892138513482));
#38943=CARTESIAN_POINT('Ctrl Pts',(-4.69742228238918,-1.06847604194589,
6.35444763451218));
#38944=CARTESIAN_POINT('Ctrl Pts',(-4.61724943626669,-0.794772684000906,
6.37712686906987));
#38945=CARTESIAN_POINT('Ctrl Pts',(-4.5584804369824,-0.636309800095237,
6.4053238999801));
#38946=CARTESIAN_POINT('Ctrl Pts',(-4.49366541735373,-0.319434907277178,
6.44387353912698));
#38947=CARTESIAN_POINT('Ctrl Pts',(-4.46342250085206,-0.158333333333343,
6.46628358235333));
#38948=CARTESIAN_POINT('Ctrl Pts',(-4.46777277979179,0.158333333333345,
6.49379687313776));
#38949=CARTESIAN_POINT('Ctrl Pts',(-4.50235376958148,0.31943490727719,6.49900342147022));
#38950=CARTESIAN_POINT('Ctrl Pts',(-4.57605485621362,0.636309800095249,
6.516285958389));
#38951=CARTESIAN_POINT('Ctrl Pts',(-4.64005443781643,0.79477268400089,6.51856964778118));
#38952=CARTESIAN_POINT('Ctrl Pts',(-4.72702626445182,1.06847604194522,6.54178838191889));
#38953=CARTESIAN_POINT('Ctrl Pts',(-4.76411617897703,1.18514270861194,6.55480108031344));
#38954=CARTESIAN_POINT('Ctrl Pts',(-4.80064912690079,1.30000000000021,6.57077594743321));
#38955=CARTESIAN_POINT('Ctrl Pts',(-4.78351752825162,-1.30000000000214,
6.33396408287167));
#38956=CARTESIAN_POINT('Ctrl Pts',(-4.75275769233394,-1.18514270861325,
6.333286827875));
#38957=CARTESIAN_POINT('Ctrl Pts',(-4.72086801148614,-1.0684760419459,6.33742145422915));
#38958=CARTESIAN_POINT('Ctrl Pts',(-4.64458630140589,-0.794772684000911,
6.35808967677029));
#38959=CARTESIAN_POINT('Ctrl Pts',(-4.58500979039674,-0.636309800095242,
6.38620665294528));
#38960=CARTESIAN_POINT('Ctrl Pts',(-4.52064386708827,-0.31943490727718,
6.42570464158484));
#38961=CARTESIAN_POINT('Ctrl Pts',(-4.48987871233452,-0.158333333333344,
6.45081921693384));
#38962=CARTESIAN_POINT('Ctrl Pts',(-4.49440306962352,0.158333333333346,
6.47885211931188));
#38963=CARTESIAN_POINT('Ctrl Pts',(-4.52972330413681,0.319434907277192,
6.48200646357875));
#38964=CARTESIAN_POINT('Ctrl Pts',(-4.60324243801808,0.636309800095253,
6.49912872852762));
#38965=CARTESIAN_POINT('Ctrl Pts',(-4.66814302376787,0.794772684000896,
6.50182552231488));
#38966=CARTESIAN_POINT('Ctrl Pts',(-4.75129428421296,1.06847604194523,6.52712794414452));
#38967=CARTESIAN_POINT('Ctrl Pts',(-4.78573195602785,1.18514270861195,6.54143715833394));
#38968=CARTESIAN_POINT('Ctrl Pts',(-4.81861420006882,1.30000000000022,6.55910310584988));
#38969=CARTESIAN_POINT('Ctrl Pts',(-4.79351020449058,-1.30000000000214,
6.32669361767881));
#38970=CARTESIAN_POINT('Ctrl Pts',(-4.76463717974963,-1.18514270861326,
6.32440463555332));
#38971=CARTESIAN_POINT('Ctrl Pts',(-4.73416404442742,-1.0684760419459,6.32746190834394));
#38972=CARTESIAN_POINT('Ctrl Pts',(-4.66006843015977,-0.794772684000913,
6.34687573846635));
#38973=CARTESIAN_POINT('Ctrl Pts',(-4.6004453570215,-0.636309800095244,
6.37614473661813));
#38974=CARTESIAN_POINT('Ctrl Pts',(-4.53628448794618,-0.319434907277182,
6.41599063572804));
#38975=CARTESIAN_POINT('Ctrl Pts',(-4.50480502257955,-0.158333333333344,
6.44136201860304));
#38976=CARTESIAN_POINT('Ctrl Pts',(-4.50932945420639,0.158333333333346,
6.46940381619497));
#38977=CARTESIAN_POINT('Ctrl Pts',(-4.54529505697776,0.319434907277193,
6.47212900611573));
#38978=CARTESIAN_POINT('Ctrl Pts',(-4.6187498700802,0.636309800095256,6.48929065647793));
#38979=CARTESIAN_POINT('Ctrl Pts',(-4.68404496334481,0.794772684000899,
6.49180109369998));
#38980=CARTESIAN_POINT('Ctrl Pts',(-4.7650418024707,1.06847604194523,6.51838131827057));
#38981=CARTESIAN_POINT('Ctrl Pts',(-4.798002140494,1.18514270861195,6.53355737900788));
#38982=CARTESIAN_POINT('Ctrl Pts',(-4.82886228611167,1.30000000000022,6.55240390616028));
#38983=CARTESIAN_POINT('Ctrl Pts',(-4.80309023084405,-1.30000000000215,
6.31826901427401));
#38984=CARTESIAN_POINT('Ctrl Pts',(-4.77600203615311,-1.18514270861327,
6.3141225697839));
#38985=CARTESIAN_POINT('Ctrl Pts',(-4.74688787067909,-1.06847604194591,
6.31596191332453));
#38986=CARTESIAN_POINT('Ctrl Pts',(-4.67494792636251,-0.794772684000919,
6.33403953266657));
#38987=CARTESIAN_POINT('Ctrl Pts',(-4.61534329009613,-0.636309800095249,
6.36454325354339));
#38988=CARTESIAN_POINT('Ctrl Pts',(-4.55164121933099,-0.319434907277184,
6.40545613306711));
#38989=CARTESIAN_POINT('Ctrl Pts',(-4.51977914903012,-0.158333333333345,
6.4320952154525));
#38990=CARTESIAN_POINT('Ctrl Pts',(-4.52453026698855,0.158333333333347,
6.46083045310235));
#38991=CARTESIAN_POINT('Ctrl Pts',(-4.56119231513724,0.319434907277194,
6.46330528331013));
#38992=CARTESIAN_POINT('Ctrl Pts',(-4.63447254701522,0.636309800095259,
6.48015268027933));
#38993=CARTESIAN_POINT('Ctrl Pts',(-4.69980372445602,0.794772684000905,
6.48133545414669));
#38994=CARTESIAN_POINT('Ctrl Pts',(-4.77856328943643,1.06847604194524,6.50892485024042));
#38995=CARTESIAN_POINT('Ctrl Pts',(-4.81007267890541,1.18514270861196,6.52504888586614));
#38996=CARTESIAN_POINT('Ctrl Pts',(-4.83899936049287,1.30000000000023,6.5453545298365));
#38997=CARTESIAN_POINT('Ctrl Pts',(-4.8151634792988,-1.30000000000216,6.30798701144558));
#38998=CARTESIAN_POINT('Ctrl Pts',(-4.79067658130991,-1.18514270861328,
6.30253576501484));
#38999=CARTESIAN_POINT('Ctrl Pts',(-4.76347243022552,-1.06847604194592,
6.30343865451421));
#39000=CARTESIAN_POINT('Ctrl Pts',(-4.6943480008138,-0.794772684000923,
6.32020383501925));
#39001=CARTESIAN_POINT('Ctrl Pts',(-4.63428503062086,-0.636309800095255,
6.35100853932324));
#39002=CARTESIAN_POINT('Ctrl Pts',(-4.5707634552206,-0.319434907277188,
6.39213218953601));
#39003=CARTESIAN_POINT('Ctrl Pts',(-4.53812729072339,-0.158333333333347,
6.41940644321399));
#39004=CARTESIAN_POINT('Ctrl Pts',(-4.54300525495016,0.158333333333349,
6.44850906375524));
#39005=CARTESIAN_POINT('Ctrl Pts',(-4.58063982343268,0.319434907277196,
6.45094237657877));
#39006=CARTESIAN_POINT('Ctrl Pts',(-4.65385213362159,0.636309800095264,
6.46786643758685));
#39007=CARTESIAN_POINT('Ctrl Pts',(-4.71946179757621,0.794772684000914,
6.46817393771025));
#39008=CARTESIAN_POINT('Ctrl Pts',(-4.79551793645857,1.06847604194525,6.49731744769436));
#39009=CARTESIAN_POINT('Ctrl Pts',(-4.82521431329873,1.18514270861197,6.51461888169237));
#39010=CARTESIAN_POINT('Ctrl Pts',(-4.85168518261458,1.30000000000024,6.53660660408975));
#39011=CARTESIAN_POINT('Ctrl Pts',(-4.83477143778585,-1.3000000000022,6.29251624496656));
#39012=CARTESIAN_POINT('Ctrl Pts',(-4.81377366445927,-1.18514270861331,
6.28313357612478));
#39013=CARTESIAN_POINT('Ctrl Pts',(-4.78922108492948,-1.06847604194595,
6.28142252691672));
#39014=CARTESIAN_POINT('Ctrl Pts',(-4.72428740102317,-0.794772684000946,
6.295192637008));
#39015=CARTESIAN_POINT('Ctrl Pts',(-4.66435349403994,-0.63630980009527,
6.32877289855501));
#39016=CARTESIAN_POINT('Ctrl Pts',(-4.60144303786872,-0.319434907277194,
6.37109892073663));
#39017=CARTESIAN_POINT('Ctrl Pts',(-4.56763172782983,-0.15833333333335,
6.39963149870782));
#39018=CARTESIAN_POINT('Ctrl Pts',(-4.5725564222523,0.158333333333352,6.42885247543347));
#39019=CARTESIAN_POINT('Ctrl Pts',(-4.61122651902749,0.319434907277203,
6.42965623035112));
#39020=CARTESIAN_POINT('Ctrl Pts',(-4.68430247235875,0.636309800095278,
6.44661626158103));
#39021=CARTESIAN_POINT('Ctrl Pts',(-4.75085363649386,0.794772684000929,
6.44701279901738));
#39022=CARTESIAN_POINT('Ctrl Pts',(-4.82274353785692,1.06847604194528,6.47910808759719));
#39023=CARTESIAN_POINT('Ctrl Pts',(-4.84954953792693,1.185142708612,6.49831652994811));
#39024=CARTESIAN_POINT('Ctrl Pts',(-4.87204306355026,1.30000000000028,6.52284055347141));
#39025=CARTESIAN_POINT('Ctrl Pts',(-4.85153310217081,-1.30000000000223,
6.27786966763461));
#39026=CARTESIAN_POINT('Ctrl Pts',(-4.83402424918511,-1.18514270861334,
6.26630098670574));
#39027=CARTESIAN_POINT('Ctrl Pts',(-4.81201988519055,-1.06847604194598,
6.26297025167625));
#39028=CARTESIAN_POINT('Ctrl Pts',(-4.75079987265101,-0.79477268400097,
6.27430689046979));
#39029=CARTESIAN_POINT('Ctrl Pts',(-4.69003131232683,-0.63630980009529,
6.30770515699895));
#39030=CARTESIAN_POINT('Ctrl Pts',(-4.62751857539782,-0.319434907277205,
6.35069569126754));
#39031=CARTESIAN_POINT('Ctrl Pts',(-4.59310018206488,-0.158333333333355,
6.38142770799137));
#39032=CARTESIAN_POINT('Ctrl Pts',(-4.59840815265766,0.158333333333357,
6.41171884616477));
#39033=CARTESIAN_POINT('Ctrl Pts',(-4.63832885544279,0.319434907277214,
6.41216717778079));
#39034=CARTESIAN_POINT('Ctrl Pts',(-4.711257692019,0.636309800095299,6.42906625385325));
#39035=CARTESIAN_POINT('Ctrl Pts',(-4.77808303811375,0.794772684000955,
6.42788358715442));
#39036=CARTESIAN_POINT('Ctrl Pts',(-4.84621721564676,1.06847604194531,6.46219989217757));
#39037=CARTESIAN_POINT('Ctrl Pts',(-4.87053159509923,1.18514270861204,6.48317159004119));
#39038=CARTESIAN_POINT('Ctrl Pts',(-4.88966759317023,1.30000000000032,6.51026072886833));
#39039=CARTESIAN_POINT('Ctrl Pts',(-4.86590096980636,-1.30000000000225,
6.26540695232221));
#39040=CARTESIAN_POINT('Ctrl Pts',(-4.85112756911822,-1.18514270861336,
6.25127678148908));
#39041=CARTESIAN_POINT('Ctrl Pts',(-4.83116921414428,-1.06847604194599,
6.24618503207826));
#39042=CARTESIAN_POINT('Ctrl Pts',(-4.77308313985265,-0.794772684000978,
6.2553026339538));
#39043=CARTESIAN_POINT('Ctrl Pts',(-4.7120659869826,-0.636309800095298,
6.28980887743881));
#39044=CARTESIAN_POINT('Ctrl Pts',(-4.65004983253428,-0.31943490727721,
6.33377644641802));
#39045=CARTESIAN_POINT('Ctrl Pts',(-4.61510964605151,-0.158333333333357,
6.36639155506332));
#39046=CARTESIAN_POINT('Ctrl Pts',(-4.62053313323579,0.158333333333359,
6.39696545018637));
#39047=CARTESIAN_POINT('Ctrl Pts',(-4.66110704130425,0.319434907277217,
6.39587846474762));
#39048=CARTESIAN_POINT('Ctrl Pts',(-4.7337422163046,0.636309800095307,6.41224402484117));
#39049=CARTESIAN_POINT('Ctrl Pts',(-4.80092708373685,0.794772684000967,
6.41010148174191));
#39050=CARTESIAN_POINT('Ctrl Pts',(-4.86600560625236,1.06847604194532,6.44680209804103));
#39051=CARTESIAN_POINT('Ctrl Pts',(-4.88828350587341,1.18514270861205,6.46957015367528));
#39052=CARTESIAN_POINT('Ctrl Pts',(-4.90466922411546,1.30000000000034,6.49921992803975));
#39053=CARTESIAN_POINT('Ctrl Pts',(-4.87299453743658,-1.30000000000226,
6.25895256639751));
#39054=CARTESIAN_POINT('Ctrl Pts',(-4.85955957430163,-1.18514270861336,
6.24348838571595));
#39055=CARTESIAN_POINT('Ctrl Pts',(-4.84061301095117,-1.06847604194599,
6.23749936438882));
#39056=CARTESIAN_POINT('Ctrl Pts',(-4.78410976027508,-0.794772684000981,
6.24555304063138));
#39057=CARTESIAN_POINT('Ctrl Pts',(-4.72308912485098,-0.636309800095299,
6.28089123849204));
#39058=CARTESIAN_POINT('Ctrl Pts',(-4.66130212304377,-0.31943490727721,
6.32527212826392));
#39059=CARTESIAN_POINT('Ctrl Pts',(-4.62591888048782,-0.158333333333358,
6.35832773529538));
#39060=CARTESIAN_POINT('Ctrl Pts',(-4.63144916783238,0.15833333333336,6.38918989253));
#39061=CARTESIAN_POINT('Ctrl Pts',(-4.67256321428421,0.319434907277219,
6.38794731218294));
#39062=CARTESIAN_POINT('Ctrl Pts',(-4.74520657544105,0.636309800095309,
6.40449356194456));
#39063=CARTESIAN_POINT('Ctrl Pts',(-4.81266614593729,0.794772684000968,
6.40215115436439));
#39064=CARTESIAN_POINT('Ctrl Pts',(-4.87616496143012,1.06847604194533,6.43988664395963));
#39065=CARTESIAN_POINT('Ctrl Pts',(-4.89735697851544,1.18514270861205,6.4633515401264));
#39066=CARTESIAN_POINT('Ctrl Pts',(-4.91225472832225,1.30000000000034,6.49394703725185));
#39067=CARTESIAN_POINT('Ctrl Pts',(-4.87887450905704,-1.30000000000227,
6.25350829485688));
#39068=CARTESIAN_POINT('Ctrl Pts',(-4.86649867966928,-1.18514270861337,
6.23678922594398));
#39069=CARTESIAN_POINT('Ctrl Pts',(-4.84836392564263,-1.068476041946,6.22997309568147));
#39070=CARTESIAN_POINT('Ctrl Pts',(-4.7931647480114,-0.794772684000989,
6.23710424057133));
#39071=CARTESIAN_POINT('Ctrl Pts',(-4.73224393961161,-0.636309800095306,
6.2734062904428));
#39072=CARTESIAN_POINT('Ctrl Pts',(-4.67066449497868,-0.319434907277213,
6.31816582250651));
#39073=CARTESIAN_POINT('Ctrl Pts',(-4.63487003306998,-0.158333333333359,
6.35146409740365));
#39074=CARTESIAN_POINT('Ctrl Pts',(-4.64046203740145,0.158333333333361,
6.38248190288132));
#39075=CARTESIAN_POINT('Ctrl Pts',(-4.6820015236105,0.319434907277222,6.38103682856874));
#39076=CARTESIAN_POINT('Ctrl Pts',(-4.75465978777017,0.636309800095315,
6.39775669322459));
#39077=CARTESIAN_POINT('Ctrl Pts',(-4.82238897181522,0.794772684000976,
6.39537091488647));
#39078=CARTESIAN_POINT('Ctrl Pts',(-4.88460180587223,1.06847604194534,6.43405409518991));
#39079=CARTESIAN_POINT('Ctrl Pts',(-4.90490010156291,1.18514270861207,6.45812920302176));
#39080=CARTESIAN_POINT('Ctrl Pts',(-4.91856706229369,1.30000000000035,6.4895349032852));
#39081=CARTESIAN_POINT('Ctrl Pts',(-4.88303349416408,-1.30000000000227,
6.24980581282697));
#39082=CARTESIAN_POINT('Ctrl Pts',(-4.87145190564438,-1.18514270861337,
6.23234183502179));
#39083=CARTESIAN_POINT('Ctrl Pts',(-4.8539079585843,-1.06847604194601,6.22500365239295));
#39084=CARTESIAN_POINT('Ctrl Pts',(-4.79960369022706,-0.794772684000991,
6.23144359503765));
#39085=CARTESIAN_POINT('Ctrl Pts',(-4.73858754855097,-0.636309800095307,
6.26800085290985));
#39086=CARTESIAN_POINT('Ctrl Pts',(-4.67713136339042,-0.319434907277214,
6.31297344610454));
#39087=CARTESIAN_POINT('Ctrl Pts',(-4.64116430483494,-0.15833333333336,
6.34674272239031));
#39088=CARTESIAN_POINT('Ctrl Pts',(-4.64681024934969,0.158333333333362,
6.3778948753898));
#39089=CARTESIAN_POINT('Ctrl Pts',(-4.68859166985004,0.319434907277222,
6.37615982618997));
#39090=CARTESIAN_POINT('Ctrl Pts',(-4.76120518328696,0.636309800095316,
6.3928452042231));
#39091=CARTESIAN_POINT('Ctrl Pts',(-4.82905128233515,0.794772684000978,
6.39021706347285));
#39092=CARTESIAN_POINT('Ctrl Pts',(-4.89038451800035,1.06847604194534,6.42962388239991));
#39093=CARTESIAN_POINT('Ctrl Pts',(-4.91009005518737,1.18514270861207,6.45422208087761));
#39094=CARTESIAN_POINT('Ctrl Pts',(-4.92295224446233,1.30000000000035,6.48636072608605));
#39095=CARTESIAN_POINT('Ctrl Pts',(-4.88511906029955,-1.30000000000227,
6.24797069807145));
#39096=CARTESIAN_POINT('Ctrl Pts',(-4.87394015206932,-1.18514270861337,
6.23014816124439));
#39097=CARTESIAN_POINT('Ctrl Pts',(-4.85669357019099,-1.06847604194601,
6.22255385660423));
#39098=CARTESIAN_POINT('Ctrl Pts',(-4.8028329759242,-0.794772684000991,
6.22863875615257));
#39099=CARTESIAN_POINT('Ctrl Pts',(-4.74174774993459,-0.636309800095307,
6.26526985332957));
#39100=CARTESIAN_POINT('Ctrl Pts',(-4.68035044328705,-0.319434907277214,
6.31034259500331));
#39101=CARTESIAN_POINT('Ctrl Pts',(-4.64431401494797,-0.15833333333336,
6.34439156977969));
#39102=CARTESIAN_POINT('Ctrl Pts',(-4.64998628638108,0.158333333333362,
6.37560784920097));
#39103=CARTESIAN_POINT('Ctrl Pts',(-4.69187679406689,0.319434907277223,
6.37369499021199));
#39104=CARTESIAN_POINT('Ctrl Pts',(-4.76445777957717,0.636309800095317,
6.39033392162532));
#39105=CARTESIAN_POINT('Ctrl Pts',(-4.83235154908065,0.794772684000978,
6.38755292826981));
#39106=CARTESIAN_POINT('Ctrl Pts',(-4.89325001331377,1.06847604194534,6.42733573848687));
#39107=CARTESIAN_POINT('Ctrl Pts',(-4.91266555316545,1.18514270861207,6.45221377491437));
#39108=CARTESIAN_POINT('Ctrl Pts',(-4.92513594421278,1.30000000000035,6.48474934332482));
#39109=CARTESIAN_POINT('Ctrl Pts',(-4.88616316227367,-1.30000000000227,
6.24705661024912));
#39110=CARTESIAN_POINT('Ctrl Pts',(-4.87518733634367,-1.18514270861337,
6.2290593099747));
#39111=CARTESIAN_POINT('Ctrl Pts',(-4.858090127115,-1.06847604194601,6.22133875711569));
#39112=CARTESIAN_POINT('Ctrl Pts',(-4.80445053351347,-0.794772684000991,
6.22724407790598));
#39113=CARTESIAN_POINT('Ctrl Pts',(-4.74332517984475,-0.636309800095307,
6.26389783228499));
#39114=CARTESIAN_POINT('Ctrl Pts',(-4.68195577762773,-0.319434907277214,
6.30901673411741));
#39115=CARTESIAN_POINT('Ctrl Pts',(-4.64588712997815,-0.15833333333336,
6.34321187867584));
#39116=CARTESIAN_POINT('Ctrl Pts',(-4.65157298490524,0.158333333333362,
6.37446118104646));
#39117=CARTESIAN_POINT('Ctrl Pts',(-4.69351785246644,0.319434907277223,
6.37245896529304));
#39118=CARTESIAN_POINT('Ctrl Pts',(-4.76608117200806,0.636309800095317,
6.38907054326162));
#39119=CARTESIAN_POINT('Ctrl Pts',(-4.83399558226774,0.794772684000978,
6.38620392993072));
#39120=CARTESIAN_POINT('Ctrl Pts',(-4.89467711682258,1.06847604194534,6.42617579067426));
#39121=CARTESIAN_POINT('Ctrl Pts',(-4.91394871474128,1.18514270861207,6.45119662852342));
#39122=CARTESIAN_POINT('Ctrl Pts',(-4.92622512274235,1.30000000000035,6.48393596680926));
#39123=CARTESIAN_POINT('Ctrl Pts',(-4.88675992689258,-1.30000000000227,
6.2465346801272));
#39124=CARTESIAN_POINT('Ctrl Pts',(-4.87590019523263,-1.18514270861337,
6.22843761554879));
#39125=CARTESIAN_POINT('Ctrl Pts',(-4.85888833846411,-1.06847604194601,
6.22064489604193));
#39126=CARTESIAN_POINT('Ctrl Pts',(-4.80537490638943,-0.794772684000991,
6.22644725354528));
#39127=CARTESIAN_POINT('Ctrl Pts',(-4.74422603700827,-0.636309800095308,
6.26311241974435));
#39128=CARTESIAN_POINT('Ctrl Pts',(-4.68287294129434,-0.319434907277214,
6.30825867370313));
#39129=CARTESIAN_POINT('Ctrl Pts',(-4.64678722961753,-0.15833333333336,
6.34254095850511));
#39130=CARTESIAN_POINT('Ctrl Pts',(-4.6524807662358,0.158333333333362,6.37380888393949));
#39131=CARTESIAN_POINT('Ctrl Pts',(-4.69445524493705,0.319434907277223,
6.37175166515498));
#39132=CARTESIAN_POINT('Ctrl Pts',(-4.76700799451387,0.636309800095317,
6.38834629748932));
#39133=CARTESIAN_POINT('Ctrl Pts',(-4.8349346515849,0.794772684000978,6.3854318888518));
#39134=CARTESIAN_POINT('Ctrl Pts',(-4.89549252003682,1.06847604194534,6.42551268428735));
#39135=CARTESIAN_POINT('Ctrl Pts',(-4.91468201642996,1.18514270861207,6.45061562505171));
#39136=CARTESIAN_POINT('Ctrl Pts',(-4.92684775185358,1.30000000000035,6.48347201537625));
#39137=CARTESIAN_POINT('Ctrl Pts',(-4.89661012634148,-1.30000000000225,
6.23793284476157));
#39138=CARTESIAN_POINT('Ctrl Pts',(-4.88767323528789,-1.18514270861336,
6.21821005201528));
#39139=CARTESIAN_POINT('Ctrl Pts',(-4.87207220842793,-1.06847604194599,
6.20923437608288));
#39140=CARTESIAN_POINT('Ctrl Pts',(-4.82063522853835,-0.794772684000981,
6.21332675889466));
#39141=CARTESIAN_POINT('Ctrl Pts',(-4.75908214733113,-0.636309800095299,
6.25014073779938));
#39142=CARTESIAN_POINT('Ctrl Pts',(-4.69797005826219,-0.31943490727721,
6.29566381090703));
#39143=CARTESIAN_POINT('Ctrl Pts',(-4.66156496293845,-0.158333333333358,
6.33127953794985));
#39144=CARTESIAN_POINT('Ctrl Pts',(-4.66738833257477,0.15833333333336,6.36286126460822));
#39145=CARTESIAN_POINT('Ctrl Pts',(-4.70990593945366,0.319434907277218,
6.36004321413319));
#39146=CARTESIAN_POINT('Ctrl Pts',(-4.7822908519055,0.636309800095308,6.37637304185465));
#39147=CARTESIAN_POINT('Ctrl Pts',(-4.85037588380938,0.794772684000967,
6.37255171433152));
#39148=CARTESIAN_POINT('Ctrl Pts',(-4.90888799196061,1.06847604194532,6.41440829010348));
#39149=CARTESIAN_POINT('Ctrl Pts',(-4.92672720751677,1.18514270861205,6.44087330209631));
#39150=CARTESIAN_POINT('Ctrl Pts',(-4.9370779150977,1.30000000000034,6.47568516536931));
#39151=CARTESIAN_POINT('Ctrl Pts',(-4.91551434023808,-1.30000000000215,
6.22032402652648));
#39152=CARTESIAN_POINT('Ctrl Pts',(-4.90999433762571,-1.18514270861327,
6.19661715740314));
#39153=CARTESIAN_POINT('Ctrl Pts',(-4.89697781727854,-1.06847604194591,
6.18492582636369));
#39154=CARTESIAN_POINT('Ctrl Pts',(-4.84958859569011,-0.79477268400092,
6.18567480949371));
#39155=CARTESIAN_POINT('Ctrl Pts',(-4.78801610962174,-0.636309800095251,
6.22466937483527));
#39156=CARTESIAN_POINT('Ctrl Pts',(-4.72754050454037,-0.319434907277186,
6.2712911094235));
#39157=CARTESIAN_POINT('Ctrl Pts',(-4.69013335396713,-0.158333333333346,
6.30849393952512));
#39158=CARTESIAN_POINT('Ctrl Pts',(-4.69618212274349,0.158333333333348,
6.34061055348662));
#39159=CARTESIAN_POINT('Ctrl Pts',(-4.73980871380282,0.319434907277193,
6.33645276090364));
#39160=CARTESIAN_POINT('Ctrl Pts',(-4.81225757937188,0.63630980009526,6.35335912454488));
#39161=CARTESIAN_POINT('Ctrl Pts',(-4.88150378801858,0.794772684000909,
6.35018783882674));
#39162=CARTESIAN_POINT('Ctrl Pts',(-4.9358861614365,1.06847604194524,6.39503939976606));
#39163=CARTESIAN_POINT('Ctrl Pts',(-4.95079638343893,1.18514270861196,6.42327726850731));
#39164=CARTESIAN_POINT('Ctrl Pts',(-4.9570767130567,1.30000000000024,6.4603384271733));
#39165=CARTESIAN_POINT('Ctrl Pts',(-4.93425818161267,-1.30000000000204,
6.20291573839235));
#39166=CARTESIAN_POINT('Ctrl Pts',(-4.93221572521049,-1.18514270861317,
6.17552577898254));
#39167=CARTESIAN_POINT('Ctrl Pts',(-4.92179501815007,-1.06847604194582,
6.161254516853));
#39168=CARTESIAN_POINT('Ctrl Pts',(-4.87836566510148,-0.794772684000851,
6.15859186148136));
#39169=CARTESIAN_POINT('Ctrl Pts',(-4.81647889550275,-0.636309800095197,
6.19899550317773));
#39170=CARTESIAN_POINT('Ctrl Pts',(-4.75652394679047,-0.319434907277159,
6.2464075492951));
#39171=CARTESIAN_POINT('Ctrl Pts',(-4.71817594712549,-0.158333333333332,
6.28527505653548));
#39172=CARTESIAN_POINT('Ctrl Pts',(-4.72452210841149,0.158333333333334,
6.31808899581228));
#39173=CARTESIAN_POINT('Ctrl Pts',(-4.76953814964646,0.319434907277167,
6.31338878414349));
#39174=CARTESIAN_POINT('Ctrl Pts',(-4.84176412499723,0.636309800095206,
6.33005968032332));
#39175=CARTESIAN_POINT('Ctrl Pts',(-4.91110009717082,0.79477268400084,6.32455974953522));
#39176=CARTESIAN_POINT('Ctrl Pts',(-4.96159302088883,1.06847604194515,6.37302357698648));
#39177=CARTESIAN_POINT('Ctrl Pts',(-4.97396758428929,1.18514270861186,6.40409612528611));
#39178=CARTESIAN_POINT('Ctrl Pts',(-4.9768601953599,1.30000000000013,6.44526302674352));
#39179=CARTESIAN_POINT('Ctrl Pts',(-4.94346631687566,-1.30000000000204,
6.19380864200921));
#39180=CARTESIAN_POINT('Ctrl Pts',(-4.94321747389919,-1.18514270861317,
6.16473300708982));
#39181=CARTESIAN_POINT('Ctrl Pts',(-4.93412052317185,-1.06847604194582,
6.14925032936665));
#39182=CARTESIAN_POINT('Ctrl Pts',(-4.89266384819064,-0.794772684000851,
6.14488469691208));
#39183=CARTESIAN_POINT('Ctrl Pts',(-4.83045152777307,-0.636309800095197,
6.18557396029434));
#39184=CARTESIAN_POINT('Ctrl Pts',(-4.77077828071587,-0.319434907277159,
6.23342821667916));
#39185=CARTESIAN_POINT('Ctrl Pts',(-4.73214233677919,-0.158333333333332,
6.27356575659754));
#39186=CARTESIAN_POINT('Ctrl Pts',(-4.73867559286303,0.158333333333334,
6.30681070735946));
#39187=CARTESIAN_POINT('Ctrl Pts',(-4.78422175451366,0.319434907277167,
6.3014102964853));
#39188=CARTESIAN_POINT('Ctrl Pts',(-4.85643493010519,0.636309800095206,
6.31823415136601));
#39189=CARTESIAN_POINT('Ctrl Pts',(-4.92620237914194,0.79477268400084,6.31264930485107));
#39190=CARTESIAN_POINT('Ctrl Pts',(-4.97470530482241,1.06847604194515,6.36274110209546));
#39191=CARTESIAN_POINT('Ctrl Pts',(-4.98569765033206,1.18514270861186,6.39487827212544));
#39192=CARTESIAN_POINT('Ctrl Pts',(-4.98668722203483,1.30000000000013,6.43746972924232));
#39193=CARTESIAN_POINT('',(-4.89594487155746,1.2,6.47046328764746));
#39194=CARTESIAN_POINT('Ctrl Pts',(-4.89594487155747,1.2,6.47046328764746));
#39195=CARTESIAN_POINT('Ctrl Pts',(-4.88130603224287,1.21680975658284,6.48627790618805));
#39196=CARTESIAN_POINT('Ctrl Pts',(-4.86723316699216,1.23314745186375,6.50310393971268));
#39197=CARTESIAN_POINT('Ctrl Pts',(-4.8493590579957,1.253505911239,6.52222463180939));
#39198=CARTESIAN_POINT('Ctrl Pts',(-4.84243698897397,1.26137686198304,6.52950748511096));
#39199=CARTESIAN_POINT('Ctrl Pts',(-4.82345328747211,1.28297787599002,6.55019123736902));
#39200=CARTESIAN_POINT('Ctrl Pts',(-4.81590450479927,1.29149306134563,6.55797296612504));
#39201=CARTESIAN_POINT('Ctrl Pts',(-4.80835019126374,1.30000000000021,6.56575364551941));
#39202=CARTESIAN_POINT('',(-4.87041241531834,0.65383484136893,6.3159282244369));
#39203=CARTESIAN_POINT('Ctrl Pts',(-4.87041241535557,0.653834841367665,
6.31592822443521));
#39204=CARTESIAN_POINT('Ctrl Pts',(-4.87329288427579,0.717401826164069,
6.33179692647823));
#39205=CARTESIAN_POINT('Ctrl Pts',(-4.87557695120327,0.763838048869181,
6.3447039736521));
#39206=CARTESIAN_POINT('Ctrl Pts',(-4.88436973136448,0.94985745749883,6.39584548840163));
#39207=CARTESIAN_POINT('Ctrl Pts',(-4.88949053569551,1.05909846488692,6.42714802739034));
#39208=CARTESIAN_POINT('Ctrl Pts',(-4.89594487155747,1.2,6.47046328764746));
#39209=CARTESIAN_POINT('',(-4.84356468978474,-0.653834841531101,6.17902933643005));
#39210=CARTESIAN_POINT('Ctrl Pts',(-4.84356468978474,-0.653834841531102,
6.17902933643005));
#39211=CARTESIAN_POINT('Ctrl Pts',(-4.81028140400316,-0.575983337726512,
6.2039379982198));
#39212=CARTESIAN_POINT('Ctrl Pts',(-4.78259022663897,-0.493640408079208,
6.22559809788892));
#39213=CARTESIAN_POINT('Ctrl Pts',(-4.74428627662278,-0.338139747975588,
6.25868215812499));
#39214=CARTESIAN_POINT('Ctrl Pts',(-4.73158448822581,-0.265664659145223,
6.27128401929845));
#39215=CARTESIAN_POINT('Ctrl Pts',(-4.71756195934014,-0.129719176923065,
6.29122561025372));
#39216=CARTESIAN_POINT('Ctrl Pts',(-4.71484294667695,-0.0666270999531989,
6.2990415867733));
#39217=CARTESIAN_POINT('Ctrl Pts',(-4.71704250209496,0.0595442011092,6.3121886496183));
#39218=CARTESIAN_POINT('Ctrl Pts',(-4.72196055121145,0.122778981188862,
6.31761996529194));
#39219=CARTESIAN_POINT('Ctrl Pts',(-4.74093392508663,0.260130875799006,
6.32599484684145));
#39220=CARTESIAN_POINT('Ctrl Pts',(-4.75649502802252,0.333944555596331,
6.32830536516641));
#39221=CARTESIAN_POINT('Ctrl Pts',(-4.80133474624554,0.491207260125491,
6.32745516422823));
#39222=CARTESIAN_POINT('Ctrl Pts',(-4.83265655726508,0.574351676991665,
6.32346821745691));
#39223=CARTESIAN_POINT('Ctrl Pts',(-4.87041241529386,0.653834841385582,
6.31592822448981));
#39224=CARTESIAN_POINT('',(-4.85793751499296,-1.2,6.24976681786834));
#39225=CARTESIAN_POINT('Ctrl Pts',(-4.85793751499296,-1.2,6.24976681786834));
#39226=CARTESIAN_POINT('Ctrl Pts',(-4.85542006159989,-1.13062235224762,
6.23689668082158));
#39227=CARTESIAN_POINT('Ctrl Pts',(-4.85227594825653,-1.03539419544579,
6.22109841849004));
#39228=CARTESIAN_POINT('Ctrl Pts',(-4.84600629457664,-0.796367988442622,
6.19059863057003));
#39229=CARTESIAN_POINT('Ctrl Pts',(-4.84488934637906,-0.739714948888321,
6.1853136109301));
#39230=CARTESIAN_POINT('Ctrl Pts',(-4.84356468978474,-0.653834841531101,
6.17902933643005));
#39231=CARTESIAN_POINT('Ctrl Pts',(-4.7734976991615,-1.30000000000002,6.34196753202476));
#39232=CARTESIAN_POINT('Ctrl Pts',(-4.78796623709172,-1.28305027811014,
6.32665270521319));
#39233=CARTESIAN_POINT('Ctrl Pts',(-4.80233849726868,-1.26612557264441,
6.31121947396146));
#39234=CARTESIAN_POINT('Ctrl Pts',(-4.82382646364986,-1.24074712529506,
6.28813340180523));
#39235=CARTESIAN_POINT('Ctrl Pts',(-4.83211932393341,-1.23088984123249,
6.27897567894286));
#39236=CARTESIAN_POINT('Ctrl Pts',(-4.84513604156342,-1.21538971859288,
6.26453695584227));
#39237=CARTESIAN_POINT('Ctrl Pts',(-4.8521670910965,-1.20698331563184,6.25664413364353));
#39238=CARTESIAN_POINT('Ctrl Pts',(-4.85793751499296,-1.2,6.24976681786834));
#39239=CARTESIAN_POINT('Origin',(0.,1.25,7.2));
#39240=CARTESIAN_POINT('Origin',(0.,1.2,7.2));
#39241=CARTESIAN_POINT('Origin',(0.,0.92691742076555,7.2));
#39242=CARTESIAN_POINT('Origin',(0.,0.653834841531101,7.2));
#39243=CARTESIAN_POINT('Origin',(0.,0.,7.2));
#39244=CARTESIAN_POINT('Origin',(0.,-0.653834841531101,7.2));
#39245=CARTESIAN_POINT('Origin',(0.,-0.926917420765551,7.2));
#39246=CARTESIAN_POINT('Origin',(0.,-1.2,7.2));
#39247=CARTESIAN_POINT('Origin',(0.,-1.25,7.2));
#39248=CARTESIAN_POINT('Ctrl Pts',(-4.86571446294974,-1.30000000000134,
5.868337644404));
#39249=CARTESIAN_POINT('Ctrl Pts',(-4.8821339505088,-1.18514270861269,5.90764937165957));
#39250=CARTESIAN_POINT('Ctrl Pts',(-4.88516330785636,-1.06847604194558,
5.94147912707392));
#39251=CARTESIAN_POINT('Ctrl Pts',(-4.86122784987519,-0.794772684000851,
6.00696817808235));
#39252=CARTESIAN_POINT('Ctrl Pts',(-4.795220551989,-0.636309800095197,6.03024314493531));
#39253=CARTESIAN_POINT('Ctrl Pts',(-4.73609341170194,-0.319434907277159,
6.07498424576792));
#39254=CARTESIAN_POINT('Ctrl Pts',(-4.69228837762394,-0.158333333333332,
6.08857601783884));
#39255=CARTESIAN_POINT('Ctrl Pts',(-4.69984189087714,0.158333333333334,
6.12160410624479));
#39256=CARTESIAN_POINT('Ctrl Pts',(-4.75146299021043,0.319434907277167,
6.14255691937913));
#39257=CARTESIAN_POINT('Ctrl Pts',(-4.82544129359938,0.636309800095206,
6.16200266173935));
#39258=CARTESIAN_POINT('Ctrl Pts',(-4.89882489071899,0.79477268400084,6.17387012311368));
#39259=CARTESIAN_POINT('Ctrl Pts',(-4.9349217851481,1.06847604194518,6.15301997060013));
#39260=CARTESIAN_POINT('Ctrl Pts',(-4.93693489080205,1.18514270861192,6.13517577749273));
#39261=CARTESIAN_POINT('Ctrl Pts',(-4.92533609403335,1.30000000000022,6.10851264972677));
#39262=CARTESIAN_POINT('Ctrl Pts',(-4.85356720775247,-1.30000000000134,
5.86521512469838));
#39263=CARTESIAN_POINT('Ctrl Pts',(-4.86766876337791,-1.18514270861269,
5.90399949143929));
#39264=CARTESIAN_POINT('Ctrl Pts',(-4.86900238119369,-1.06847604194558,
5.93741886516899));
#39265=CARTESIAN_POINT('Ctrl Pts',(-4.84258681457997,-0.794772684000851,
6.00223009688818));
#39266=CARTESIAN_POINT('Ctrl Pts',(-4.77700822871633,-0.636309800095197,
6.02540714067998));
#39267=CARTESIAN_POINT('Ctrl Pts',(-4.71780718134386,-0.319434907277159,
6.07001371292168));
#39268=CARTESIAN_POINT('Ctrl Pts',(-4.67477123304744,-0.158333333333332,
6.08402952939453));
#39269=CARTESIAN_POINT('Ctrl Pts',(-4.6823203577386,0.158333333333334,6.11658777090616));
#39270=CARTESIAN_POINT('Ctrl Pts',(-4.73316183806893,0.319434907277167,
6.13649746894165));
#39271=CARTESIAN_POINT('Ctrl Pts',(-4.80721762558705,0.636309800095206,
6.15542465374059));
#39272=CARTESIAN_POINT('Ctrl Pts',(-4.88018764438342,0.79477268400084,6.16716360018097));
#39273=CARTESIAN_POINT('Ctrl Pts',(-4.91877933308293,1.06847604194518,6.14706683419082));
#39274=CARTESIAN_POINT('Ctrl Pts',(-4.92249447744502,1.18514270861192,6.12979090408604));
#39275=CARTESIAN_POINT('Ctrl Pts',(-4.91321985409419,1.30000000000022,6.10393818921505));
#39276=CARTESIAN_POINT('Ctrl Pts',(-4.82938120791274,-1.30000000000253,
5.8595404167699));
#39277=CARTESIAN_POINT('Ctrl Pts',(-4.83868584525243,-1.18514270861378,
5.89560518362874));
#39278=CARTESIAN_POINT('Ctrl Pts',(-4.8365301203178,-1.06847604194656,5.92725947612256));
#39279=CARTESIAN_POINT('Ctrl Pts',(-4.80507423497627,-0.794772684001587,
5.99019814610711));
#39280=CARTESIAN_POINT('Ctrl Pts',(-4.74056097052128,-0.636309800095781,
6.01592842036806));
#39281=CARTESIAN_POINT('Ctrl Pts',(-4.68126449885463,-0.31943490727745,
6.06100334291516));
#39282=CARTESIAN_POINT('Ctrl Pts',(-4.63971683522099,-0.158333333333478,
6.07486407107751));
#39283=CARTESIAN_POINT('Ctrl Pts',(-4.64725684719242,0.15833333333348,6.10676535616951));
#39284=CARTESIAN_POINT('Ctrl Pts',(-4.69656249034137,0.319434907277462,
6.12571209947254));
#39285=CARTESIAN_POINT('Ctrl Pts',(-4.77077343930226,0.636309800095791,
6.14377196129411));
#39286=CARTESIAN_POINT('Ctrl Pts',(-4.84287989741261,0.794772684001569,
6.15422858003056));
#39287=CARTESIAN_POINT('Ctrl Pts',(-4.88648202335048,1.06847604194616,6.13566971188501));
#39288=CARTESIAN_POINT('Ctrl Pts',(-4.89362191156687,1.18514270861301,6.11973294382499));
#39289=CARTESIAN_POINT('Ctrl Pts',(-4.88902794329912,1.30000000000141,6.09589285405133));
#39290=CARTESIAN_POINT('Ctrl Pts',(-4.80495569332938,-1.30000000000374,
5.85368628458532));
#39291=CARTESIAN_POINT('Ctrl Pts',(-4.80967406261113,-1.18514270861488,
5.88968235144291));
#39292=CARTESIAN_POINT('Ctrl Pts',(-4.80415227688878,-1.06847604194755,
5.92110637924295));
#39293=CARTESIAN_POINT('Ctrl Pts',(-4.76773904064537,-0.794772684002323,
5.98313984495985));
#39294=CARTESIAN_POINT('Ctrl Pts',(-4.70398214416904,-0.636309800096376,
6.00737539224725));
#39295=CARTESIAN_POINT('Ctrl Pts',(-4.64449817003754,-0.31943490727775,
6.05173515931923));
#39296=CARTESIAN_POINT('Ctrl Pts',(-4.60450849084288,-0.158333333333626,
6.06643614477618));
#39297=CARTESIAN_POINT('Ctrl Pts',(-4.6120319495031,0.158333333333627,6.09763340854605));
#39298=CARTESIAN_POINT('Ctrl Pts',(-4.65977508101751,0.31943490727776,6.11534010784939));
#39299=CARTESIAN_POINT('Ctrl Pts',(-4.73411531820855,0.636309800096385,
6.1320613803948));
#39300=CARTESIAN_POINT('Ctrl Pts',(-4.80532269523504,0.794772684002312,
6.14066184138635));
#39301=CARTESIAN_POINT('Ctrl Pts',(-4.8539609032049,1.06847604194716,6.12349932855702));
#39302=CARTESIAN_POINT('Ctrl Pts',(-4.86455173919657,1.18514270861412,6.10896728959689));
#39303=CARTESIAN_POINT('Ctrl Pts',(-4.86467973317292,1.30000000000263,6.08733222754667));
#39304=CARTESIAN_POINT('Ctrl Pts',(-4.79263759311852,-1.3000000000039,5.85082946845672));
#39305=CARTESIAN_POINT('Ctrl Pts',(-4.79494039025008,-1.18514270861502,
5.88581163158155));
#39306=CARTESIAN_POINT('Ctrl Pts',(-4.78765825739138,-1.06847604194768,
5.91655896413454));
#39307=CARTESIAN_POINT('Ctrl Pts',(-4.74869196796596,-0.794772684002417,
5.97780814751876));
#39308=CARTESIAN_POINT('Ctrl Pts',(-4.68543647819062,-0.63630980009645,
6.00273352707067));
#39309=CARTESIAN_POINT('Ctrl Pts',(-4.62590743407482,-0.319434907277788,
6.04740201192308));
#39310=CARTESIAN_POINT('Ctrl Pts',(-4.58671565461658,-0.158333333333644,
6.06263789863126));
#39311=CARTESIAN_POINT('Ctrl Pts',(-4.59423006993087,0.158333333333646,
6.09350046461607));
#39312=CARTESIAN_POINT('Ctrl Pts',(-4.64114799628483,0.319434907277798,
6.11008166880538));
#39313=CARTESIAN_POINT('Ctrl Pts',(-4.7155520813538,0.636309800096461,6.12633371016645));
#39314=CARTESIAN_POINT('Ctrl Pts',(-4.78633595217113,0.794772684002406,
6.13495132958802));
#39315=CARTESIAN_POINT('Ctrl Pts',(-4.83752743384807,1.06847604194729,6.11849378740315));
#39316=CARTESIAN_POINT('Ctrl Pts',(-4.84986177812713,1.18514270861426,6.10446522757005));
#39317=CARTESIAN_POINT('Ctrl Pts',(-4.85237157109861,1.30000000000278,6.08353196810363));
#39318=CARTESIAN_POINT('Ctrl Pts',(-4.79235345691312,-1.3000000000039,5.85076475170828));
#39319=CARTESIAN_POINT('Ctrl Pts',(-4.79460046688034,-1.18514270861502,
5.88572335809722));
#39320=CARTESIAN_POINT('Ctrl Pts',(-4.78727767678747,-1.06847604194768,
5.91645491529231));
#39321=CARTESIAN_POINT('Ctrl Pts',(-4.7482524141831,-0.794772684002416,
5.97768563098373));
#39322=CARTESIAN_POINT('Ctrl Pts',(-4.68500846948588,-0.636309800096449,
6.00262629599803));
#39323=CARTESIAN_POINT('Ctrl Pts',(-4.62547840464194,-0.319434907277788,
6.04730232452214));
#39324=CARTESIAN_POINT('Ctrl Pts',(-4.58630512781722,-0.158333333333644,
6.06255206409805));
#39325=CARTESIAN_POINT('Ctrl Pts',(-4.59381933770018,0.158333333333646,
6.0934070741634));
#39326=CARTESIAN_POINT('Ctrl Pts',(-4.64071814564975,0.319434907277797,
6.1099612324191));
#39327=CARTESIAN_POINT('Ctrl Pts',(-4.7151236688301,0.63630980009646,6.1262018217059));
#39328=CARTESIAN_POINT('Ctrl Pts',(-4.78589776844809,0.794772684002405,
6.13481967784126));
#39329=CARTESIAN_POINT('Ctrl Pts',(-4.83714817867047,1.06847604194729,6.11837827953156));
#39330=CARTESIAN_POINT('Ctrl Pts',(-4.84952276532352,1.18514270861426,6.10436134959035));
#39331=CARTESIAN_POINT('Ctrl Pts',(-4.85208753505921,1.30000000000278,6.08344436182233));
#39332=CARTESIAN_POINT('Ctrl Pts',(-4.79206929192536,-1.3000000000039,5.85069980751958));
#39333=CARTESIAN_POINT('Ctrl Pts',(-4.79426054278171,-1.18514270861502,
5.88563507380463));
#39334=CARTESIAN_POINT('Ctrl Pts',(-4.78689711474143,-1.06847604194768,
5.91635100912804));
#39335=CARTESIAN_POINT('Ctrl Pts',(-4.74781290326158,-0.794772684002417,
5.97756346583113));
#39336=CARTESIAN_POINT('Ctrl Pts',(-4.68458049645332,-0.63630980009645,
6.00251948238273));
#39337=CARTESIAN_POINT('Ctrl Pts',(-4.62504939046843,-0.319434907277788,
6.04720275100294));
#39338=CARTESIAN_POINT('Ctrl Pts',(-4.58589457293348,-0.158333333333644,
6.06246562381856));
#39339=CARTESIAN_POINT('Ctrl Pts',(-4.5934085730634,0.158333333333646,6.09331300309073));
#39340=CARTESIAN_POINT('Ctrl Pts',(-4.64028830282297,0.319434907277797,
6.10984075513259));
#39341=CARTESIAN_POINT('Ctrl Pts',(-4.71469527329583,0.63630980009646,6.12607005366339));
#39342=CARTESIAN_POINT('Ctrl Pts',(-4.78545958296302,0.794772684002405,
6.13468785029002));
#39343=CARTESIAN_POINT('Ctrl Pts',(-4.83676891622233,1.06847604194729,6.11826256621009));
#39344=CARTESIAN_POINT('Ctrl Pts',(-4.84918374438527,1.18514270861426,6.10425728837294));
#39345=CARTESIAN_POINT('Ctrl Pts',(-4.85180349154136,1.30000000000278,6.08335662956008));
#39346=CARTESIAN_POINT('Ctrl Pts',(-4.79150104411294,-1.30000000000389,
5.85057075286265));
#39347=CARTESIAN_POINT('Ctrl Pts',(-4.7935807724207,-1.18514270861502,5.8854594671761));
#39348=CARTESIAN_POINT('Ctrl Pts',(-4.78613606158058,-1.06847604194768,
5.91614420454618));
#39349=CARTESIAN_POINT('Ctrl Pts',(-4.74693393044161,-0.794772684002416,
5.97732005858974));
#39350=CARTESIAN_POINT('Ctrl Pts',(-4.68372456524032,-0.636309800096449,
6.00230625476568));
#39351=CARTESIAN_POINT('Ctrl Pts',(-4.62419136920195,-0.319434907277788,
6.04700400909723));
#39352=CARTESIAN_POINT('Ctrl Pts',(-4.58507349960888,-0.158333333333644,
6.06229365668962));
#39353=CARTESIAN_POINT('Ctrl Pts',(-4.59258707820112,0.158333333333646,
6.09312584206709));
#39354=CARTESIAN_POINT('Ctrl Pts',(-4.6394286323444,0.319434907277797,6.10960059291445));
#39355=CARTESIAN_POINT('Ctrl Pts',(-4.71383847627133,0.63630980009646,6.12580692931946));
#39356=CARTESIAN_POINT('Ctrl Pts',(-4.7845831842747,0.794772684002405,6.13442406850582));
#39357=CARTESIAN_POINT('Ctrl Pts',(-4.83601036310554,1.06847604194729,6.1180308641712));
#39358=CARTESIAN_POINT('Ctrl Pts',(-4.84850568027476,1.18514270861426,6.10404893558892));
#39359=CARTESIAN_POINT('Ctrl Pts',(-4.85123539446212,1.30000000000278,6.08318108915274));
#39360=CARTESIAN_POINT('Ctrl Pts',(-4.79064879748123,-1.30000000000389,
5.85037865044717));
#39361=CARTESIAN_POINT('Ctrl Pts',(-4.79256131938749,-1.18514270861502,
5.88519857264719));
#39362=CARTESIAN_POINT('Ctrl Pts',(-4.78499472665041,-1.06847604194768,
5.91583711764781));
#39363=CARTESIAN_POINT('Ctrl Pts',(-4.74561573261963,-0.794772684002415,
5.97695846800678));
#39364=CARTESIAN_POINT('Ctrl Pts',(-4.6824408103457,-0.636309800096449,
6.00198863703091));
#39365=CARTESIAN_POINT('Ctrl Pts',(-4.62290439564666,-0.319434907277787,
6.04670719585982));
#39366=CARTESIAN_POINT('Ctrl Pts',(-4.58384189752997,-0.158333333333644,
6.06203623124653));
#39367=CARTESIAN_POINT('Ctrl Pts',(-4.59135482701311,0.158333333333646,
6.09284559935395));
#39368=CARTESIAN_POINT('Ctrl Pts',(-4.63813918883291,0.319434907277797,
6.10924228682364));
#39369=CARTESIAN_POINT('Ctrl Pts',(-4.71255331597794,0.636309800096459,
6.12541364383744));
#39370=CARTESIAN_POINT('Ctrl Pts',(-4.78326850781132,0.794772684002404,
6.13402741690736));
#39371=CARTESIAN_POINT('Ctrl Pts',(-4.83487243796819,1.06847604194729,6.11768186589438));
#39372=CARTESIAN_POINT('Ctrl Pts',(-4.84748850226198,1.18514270861426,6.10373517179134));
#39373=CARTESIAN_POINT('Ctrl Pts',(-4.85038320159871,1.30000000000278,6.08291716695642));
#39374=CARTESIAN_POINT('Ctrl Pts',(-4.78970212769114,-1.30000000000389,
5.85016849536932));
#39375=CARTESIAN_POINT('Ctrl Pts',(-4.79142904799313,-1.18514270861502,
5.8849144498525));
#39376=CARTESIAN_POINT('Ctrl Pts',(-4.78372712974911,-1.06847604194768,
5.91550308170812));
#39377=CARTESIAN_POINT('Ctrl Pts',(-4.74415165456808,-0.794772684002414,
5.9765646935901));
#39378=CARTESIAN_POINT('Ctrl Pts',(-4.68101470387775,-0.636309800096448,
6.00164031176));
#39379=CARTESIAN_POINT('Ctrl Pts',(-4.62147451839339,-0.319434907277787,
6.04637982868371));
#39380=CARTESIAN_POINT('Ctrl Pts',(-4.58247344360906,-0.158333333333644,
6.06175115231738));
#39381=CARTESIAN_POINT('Ctrl Pts',(-4.58998562257767,0.158333333333646,
6.0925352710236));
#39382=CARTESIAN_POINT('Ctrl Pts',(-4.63670660217091,0.319434907277796,
6.10884861201663));
#39383=CARTESIAN_POINT('Ctrl Pts',(-4.71112543273955,0.636309800096458,
6.1249797811688));
#39384=CARTESIAN_POINT('Ctrl Pts',(-4.78180756889426,0.794772684002403,
6.133583938481));
#39385=CARTESIAN_POINT('Ctrl Pts',(-4.83360785935252,1.06847604194728,6.11729033614163));
#39386=CARTESIAN_POINT('Ctrl Pts',(-4.84635812346542,1.18514270861425,6.10338341028972));
#39387=CARTESIAN_POINT('Ctrl Pts',(-4.84943622534175,1.30000000000278,6.08262245530113));
#39388=CARTESIAN_POINT('Ctrl Pts',(-4.78894492917833,-1.30000000000389,
5.85000225316197));
#39389=CARTESIAN_POINT('Ctrl Pts',(-4.79052351881161,-1.18514270861502,
5.88469093422728));
#39390=CARTESIAN_POINT('Ctrl Pts',(-4.78271342462246,-1.06847604194768,
5.91524073943617));
#39391=CARTESIAN_POINT('Ctrl Pts',(-4.74298080681207,-0.794772684002414,
5.97625526972861));
#39392=CARTESIAN_POINT('Ctrl Pts',(-4.67987401751868,-0.636309800096447,
6.00136483869678));
#39393=CARTESIAN_POINT('Ctrl Pts',(-4.6203306644492,-0.319434907277787,
6.04611937197189));
#39394=CARTESIAN_POINT('Ctrl Pts',(-4.58137862503731,-0.158333333333644,
6.06152297641083));
#39395=CARTESIAN_POINT('Ctrl Pts',(-4.58889018478066,0.158333333333646,
6.0922869758967));
#39396=CARTESIAN_POINT('Ctrl Pts',(-4.63556060966728,0.319434907277796,
6.10853657817495));
#39397=CARTESIAN_POINT('Ctrl Pts',(-4.70998317996087,0.636309800096458,
6.1246348456659));
#39398=CARTESIAN_POINT('Ctrl Pts',(-4.78063868238186,0.794772684002403,
6.13322692900062));
#39399=CARTESIAN_POINT('Ctrl Pts',(-4.83259604193094,1.06847604194728,6.11697421639103));
#39400=CARTESIAN_POINT('Ctrl Pts',(-4.84545369240368,1.18514270861425,6.10309959311482));
#39401=CARTESIAN_POINT('Ctrl Pts',(-4.84867857761027,1.30000000000278,6.08238554362872));
#39402=CARTESIAN_POINT('Ctrl Pts',(-4.78705216995794,-1.30000000000389,
5.84958985324092));
#39403=CARTESIAN_POINT('Ctrl Pts',(-4.78826023810035,-1.18514270861501,
5.88413897274494));
#39404=CARTESIAN_POINT('Ctrl Pts',(-4.78017987927369,-1.06847604194767,
5.91459382625139));
#39405=CARTESIAN_POINT('Ctrl Pts',(-4.74005450947193,-0.794772684002412,
5.97549205681426));
#39406=CARTESIAN_POINT('Ctrl Pts',(-4.67702271654217,-0.636309800096446,
6.00068204622885));
#39407=CARTESIAN_POINT('Ctrl Pts',(-4.61747116261762,-0.319434907277786,
6.04547075761471));
#39408=CARTESIAN_POINT('Ctrl Pts',(-4.5786415099605,-0.158333333333643,
6.06095195063578));
#39409=CARTESIAN_POINT('Ctrl Pts',(-4.58615148454829,0.158333333333645,
6.09166571508387));
#39410=CARTESIAN_POINT('Ctrl Pts',(-4.63269580912546,0.319434907277795,
6.1077614980812));
#39411=CARTESIAN_POINT('Ctrl Pts',(-4.70712768682217,0.636309800096456,
6.12377621359621));
#39412=CARTESIAN_POINT('Ctrl Pts',(-4.77771625631815,0.7947726840024,6.13233008846881));
#39413=CARTESIAN_POINT('Ctrl Pts',(-4.83006624206924,1.06847604194728,6.11617846264734));
#39414=CARTESIAN_POINT('Ctrl Pts',(-4.84319239988727,1.18514270861425,6.10238553916046));
#39415=CARTESIAN_POINT('Ctrl Pts',(-4.84678434644982,1.30000000000277,6.0817911325281));
#39416=CARTESIAN_POINT('Ctrl Pts',(-4.78232267396703,-1.30000000000387,
5.84859386619855));
#39417=CARTESIAN_POINT('Ctrl Pts',(-4.78260808356488,-1.18514270861499,
5.88283739808244));
#39418=CARTESIAN_POINT('Ctrl Pts',(-4.77385415910733,-1.06847604194765,
5.91308020204031));
#39419=CARTESIAN_POINT('Ctrl Pts',(-4.73274817241335,-0.794772684002398,
5.97370464738306));
#39420=CARTESIAN_POINT('Ctrl Pts',(-4.66989905139225,-0.636309800096434,
5.99904293743694));
#39421=CARTESIAN_POINT('Ctrl Pts',(-4.61032360362397,-0.31943490727778,
6.04387655671116));
#39422=CARTESIAN_POINT('Ctrl Pts',(-4.57179738839238,-0.158333333333641,
6.05951301291473));
#39423=CARTESIAN_POINT('Ctrl Pts',(-4.57930300663517,0.158333333333642,
6.09010245591926));
#39424=CARTESIAN_POINT('Ctrl Pts',(-4.6255356682504,0.31943490727779,6.10588183844076));
#39425=CARTESIAN_POINT('Ctrl Pts',(-4.69999044749396,0.636309800096445,
6.12167340347345));
#39426=CARTESIAN_POINT('Ctrl Pts',(-4.77040755918437,0.794772684002386,
6.13003584639514));
#39427=CARTESIAN_POINT('Ctrl Pts',(-4.82373861375105,1.06847604194726,6.11412346862001));
#39428=CARTESIAN_POINT('Ctrl Pts',(-4.83753655289709,1.18514270861423,6.10054603239835));
#39429=CARTESIAN_POINT('Ctrl Pts',(-4.84204739377757,1.30000000000275,6.08027903868217));
#39430=CARTESIAN_POINT('Ctrl Pts',(-4.77627501138971,-1.30000000000379,
5.84743290715711));
#39431=CARTESIAN_POINT('Ctrl Pts',(-4.77539694113463,-1.18514270861493,
5.88148413234476));
#39432=CARTESIAN_POINT('Ctrl Pts',(-4.76579122721606,-1.06847604194759,
5.91157346660426));
#39433=CARTESIAN_POINT('Ctrl Pts',(-4.72343750362598,-0.794772684002353,
5.9719330874767));
#39434=CARTESIAN_POINT('Ctrl Pts',(-4.66080161735695,-0.636309800096398,
5.99723877747126));
#39435=CARTESIAN_POINT('Ctrl Pts',(-4.60118031170647,-0.319434907277762,
6.04193925472643));
#39436=CARTESIAN_POINT('Ctrl Pts',(-4.56302917655413,-0.158333333333632,
6.05756656837047));
#39437=CARTESIAN_POINT('Ctrl Pts',(-4.57052736738655,0.158333333333633,
6.0880007030458));
#39438=CARTESIAN_POINT('Ctrl Pts',(-4.6163784835927,0.319434907277771,6.10370721172841));
#39439=CARTESIAN_POINT('Ctrl Pts',(-4.69086203192954,0.636309800096409,
6.11916627651037));
#39440=CARTESIAN_POINT('Ctrl Pts',(-4.76104209380644,0.794772684002341,
6.12685833128135));
#39441=CARTESIAN_POINT('Ctrl Pts',(-4.81562672710523,1.0684760419472,6.11119753499256));
#39442=CARTESIAN_POINT('Ctrl Pts',(-4.83028658473183,1.18514270861416,6.09794745392577));
#39443=CARTESIAN_POINT('Ctrl Pts',(-4.83597863478999,1.30000000000268,6.07822627021593));
#39444=CARTESIAN_POINT('Ctrl Pts',(-4.77022543175637,-1.30000000000376,
5.84627362658672));
#39445=CARTESIAN_POINT('Ctrl Pts',(-4.7681845197533,-1.1851427086149,5.88014847704338));
#39446=CARTESIAN_POINT('Ctrl Pts',(-4.75772785182655,-1.06847604194757,
5.91009960050316));
#39447=CARTESIAN_POINT('Ctrl Pts',(-4.71412877731664,-0.794772684002333,
5.97022809309519));
#39448=CARTESIAN_POINT('Ctrl Pts',(-4.6517090215279,-0.636309800096382,
5.99552776578552));
#39449=CARTESIAN_POINT('Ctrl Pts',(-4.59204348242412,-0.319434907277754,
6.0401111535088));
#39450=CARTESIAN_POINT('Ctrl Pts',(-4.55426759534573,-0.158333333333628,
6.05572325434686));
#39451=CARTESIAN_POINT('Ctrl Pts',(-4.56175638576926,0.15833333333363,6.08599115135827));
#39452=CARTESIAN_POINT('Ctrl Pts',(-4.6072219529283,0.319434907277763,6.10160387512772));
#39453=CARTESIAN_POINT('Ctrl Pts',(-4.68173242114704,0.636309800096393,
6.11672482164359));
#39454=CARTESIAN_POINT('Ctrl Pts',(-4.75167730793368,0.794772684002322,
6.12377701094137));
#39455=CARTESIAN_POINT('Ctrl Pts',(-4.80751491300795,1.06847604194717,6.10834343885876));
#39456=CARTESIAN_POINT('Ctrl Pts',(-4.82303611146367,1.18514270861413,6.09539943328269));
#39457=CARTESIAN_POINT('Ctrl Pts',(-4.82990847812561,1.30000000000264,6.0761920436149));
#39458=CARTESIAN_POINT('Ctrl Pts',(-4.76568523200038,-1.30000000000375,
5.84537209489026));
#39459=CARTESIAN_POINT('Ctrl Pts',(-4.76276723985793,-1.18514270861489,
5.87906444452569));
#39460=CARTESIAN_POINT('Ctrl Pts',(-4.75166970878787,-1.06847604194756,
5.90888582986161));
#39461=CARTESIAN_POINT('Ctrl Pts',(-4.70713582072867,-0.794772684002326,
5.96883649381953));
#39462=CARTESIAN_POINT('Ctrl Pts',(-4.64488596516521,-0.636309800096377,
5.99421317981936));
#39463=CARTESIAN_POINT('Ctrl Pts',(-4.58519342042272,-0.319434907277752,
6.03878281966128));
#39464=CARTESIAN_POINT('Ctrl Pts',(-4.54770428969278,-0.158333333333626,
6.05445557738353));
#39465=CARTESIAN_POINT('Ctrl Pts',(-4.55518551943629,0.158333333333628,
6.08459347174527));
#39466=CARTESIAN_POINT('Ctrl Pts',(-4.60035336788503,0.319434907277761,
6.10001436535062));
#39467=CARTESIAN_POINT('Ctrl Pts',(-4.67488237016258,0.636309800096388,
6.11488663820045));
#39468=CARTESIAN_POINT('Ctrl Pts',(-4.74465663872414,0.794772684002315,
6.12160101488735));
#39469=CARTESIAN_POINT('Ctrl Pts',(-4.8014344625704,1.06847604194717,6.10634068048414));
#39470=CARTESIAN_POINT('Ctrl Pts',(-4.81760103124188,1.18514270861412,6.09359999685794));
#39471=CARTESIAN_POINT('Ctrl Pts',(-4.82535715246749,1.30000000000263,6.07472426291758));
#39472=CARTESIAN_POINT('Ctrl Pts',(-4.76114118660295,-1.30000000000373,
5.8444295275307));
#39473=CARTESIAN_POINT('Ctrl Pts',(-4.75734057622045,-1.18514270861487,
5.87788182555618));
#39474=CARTESIAN_POINT('Ctrl Pts',(-4.74559912821443,-1.06847604194755,
5.90754235702996));
#39475=CARTESIAN_POINT('Ctrl Pts',(-4.7001291109825,-0.794772684002317,
5.96730437902859));
#39476=CARTESIAN_POINT('Ctrl Pts',(-4.63805715956591,-0.63630980009637,
5.99284271864704));
#39477=CARTESIAN_POINT('Ctrl Pts',(-4.57834408708591,-0.319434907277748,
6.03747567657016));
#39478=CARTESIAN_POINT('Ctrl Pts',(-4.5411474242754,-0.158333333333624,
6.05328516135936));
#39479=CARTESIAN_POINT('Ctrl Pts',(-4.5486211589217,0.158333333333626,6.08329216744718));
#39480=CARTESIAN_POINT('Ctrl Pts',(-4.59348320110659,0.319434907277756,
6.09840197555842));
#39481=CARTESIAN_POINT('Ctrl Pts',(-4.66802936642217,0.636309800096379,
6.11303286590956));
#39482=CARTESIAN_POINT('Ctrl Pts',(-4.73763869169212,0.794772684002305,
6.11955205859386));
#39483=CARTESIAN_POINT('Ctrl Pts',(-4.79535698540585,1.06847604194715,6.10446706721648));
#39484=CARTESIAN_POINT('Ctrl Pts',(-4.81216812185674,1.18514270861411,6.09190266428265));
#39485=CARTESIAN_POINT('Ctrl Pts',(-4.82080628408339,1.30000000000262,6.07330359222823));
#39486=CARTESIAN_POINT('Ctrl Pts',(-4.75204633607105,-1.3000000000037,5.84247157674721));
#39487=CARTESIAN_POINT('Ctrl Pts',(-4.74647043807593,-1.18514270861484,
5.87533933711595));
#39488=CARTESIAN_POINT('Ctrl Pts',(-4.73343521713089,-1.06847604194752,
5.90461737006026));
#39489=CARTESIAN_POINT('Ctrl Pts',(-4.68608872081418,-0.794772684002296,
5.96396249473901));
#39490=CARTESIAN_POINT('Ctrl Pts',(-4.62438259342724,-0.636309800096353,
5.9899294806832));
#39491=CARTESIAN_POINT('Ctrl Pts',(-4.56464098529988,-0.319434907277739,
6.03483539724006));
#39492=CARTESIAN_POINT('Ctrl Pts',(-4.52804496558433,-0.15833333333362,
6.05110941818164));
#39493=CARTESIAN_POINT('Ctrl Pts',(-4.53550641380118,0.158333333333622,
6.08088277914227));
#39494=CARTESIAN_POINT('Ctrl Pts',(-4.57974262825361,0.319434907277748,
6.09517289227285));
#39495=CARTESIAN_POINT('Ctrl Pts',(-4.65431857536549,0.636309800096363,
6.109302420349));
#39496=CARTESIAN_POINT('Ctrl Pts',(-4.72360073491046,0.794772684002285,
6.11557128000159));
#39497=CARTESIAN_POINT('Ctrl Pts',(-4.78320294093358,1.06847604194713,6.10086986779172));
#39498=CARTESIAN_POINT('Ctrl Pts',(-4.80130507524539,1.18514270861408,6.08865415566601));
#39499=CARTESIAN_POINT('Ctrl Pts',(-4.81170975736097,1.30000000000258,6.07058642801923));
#39500=CARTESIAN_POINT('Ctrl Pts',(-4.73839544802899,-1.30000000000347,
5.83951983631493));
#39501=CARTESIAN_POINT('Ctrl Pts',(-4.7301586668395,-1.18514270861464,5.87155305687854));
#39502=CARTESIAN_POINT('Ctrl Pts',(-4.7151830138948,-1.06847604194733,5.90027308429101));
#39503=CARTESIAN_POINT('Ctrl Pts',(-4.6650181178623,-0.794772684002159,
5.95896795405434));
#39504=CARTESIAN_POINT('Ctrl Pts',(-4.60385010015465,-0.636309800096243,
5.98546376809877));
#39505=CARTESIAN_POINT('Ctrl Pts',(-4.5440599408242,-0.319434907277684,
6.0306795094364));
#39506=CARTESIAN_POINT('Ctrl Pts',(-4.50836163191022,-0.158333333333593,
6.04753069331569));
#39507=CARTESIAN_POINT('Ctrl Pts',(-4.51581263521795,0.158333333333595,
6.07704719623594));
#39508=CARTESIAN_POINT('Ctrl Pts',(-4.55913169821868,0.319434907277693,
6.09048284576324));
#39509=CARTESIAN_POINT('Ctrl Pts',(-4.63375324468253,0.636309800096253,
6.10382098788036));
#39510=CARTESIAN_POINT('Ctrl Pts',(-4.70252536720865,0.794772684002148,
6.10926268214505));
#39511=CARTESIAN_POINT('Ctrl Pts',(-4.76494233919913,1.06847604194694,6.09498933287893));
#39512=CARTESIAN_POINT('Ctrl Pts',(-4.78497737290546,1.18514270861387,6.08329204250012));
#39513=CARTESIAN_POINT('Ctrl Pts',(-4.79802944592016,1.30000000000236,6.06607586576008));
#39514=CARTESIAN_POINT('Ctrl Pts',(-4.71419853039106,-1.30000000000326,
5.83508745077068));
#39515=CARTESIAN_POINT('Ctrl Pts',(-4.70128641819185,-1.18514270861444,
5.86629312556564));
#39516=CARTESIAN_POINT('Ctrl Pts',(-4.68289983264278,-1.06847604194715,
5.89447943720253));
#39517=CARTESIAN_POINT('Ctrl Pts',(-4.62777601319786,-0.794772684002022,
5.95262012281929));
#39518=CARTESIAN_POINT('Ctrl Pts',(-4.56756758295101,-0.636309800096134,
5.98001645391371));
#39519=CARTESIAN_POINT('Ctrl Pts',(-4.50763426831788,-0.319434907277629,
6.02520090889999));
#39520=CARTESIAN_POINT('Ctrl Pts',(-4.4734303023097,-0.158333333333566,
6.04204654909383));
#39521=CARTESIAN_POINT('Ctrl Pts',(-4.48078676006398,0.158333333333568,
6.07036303417538));
#39522=CARTESIAN_POINT('Ctrl Pts',(-4.52244787459498,0.319434907277638,
6.08189554315551));
#39523=CARTESIAN_POINT('Ctrl Pts',(-4.59716066414553,0.636309800096144,
6.09426412410944));
#39524=CARTESIAN_POINT('Ctrl Pts',(-4.66509691199277,0.794772684002011,
6.099765775605));
#39525=CARTESIAN_POINT('Ctrl Pts',(-4.73255426551456,1.06847604194676,6.08658695557659));
#39526=CARTESIAN_POINT('Ctrl Pts',(-4.75603454243535,1.18514270861367,6.07568871813639));
#39527=CARTESIAN_POINT('Ctrl Pts',(-4.77379530747862,1.30000000000213,6.05959686612286));
#39528=CARTESIAN_POINT('Ctrl Pts',(-4.6899767271724,-1.30000000000266,5.83061257312496));
#39529=CARTESIAN_POINT('Ctrl Pts',(-4.67239628145367,-1.18514270861389,
5.86104763341269));
#39530=CARTESIAN_POINT('Ctrl Pts',(-4.65059129853361,-1.06847604194666,
5.88862683954874));
#39531=CARTESIAN_POINT('Ctrl Pts',(-4.59045789986563,-0.794772684001657,
5.94574272852212));
#39532=CARTESIAN_POINT('Ctrl Pts',(-4.53107781153004,-0.636309800095843,
5.97283638745076));
#39533=CARTESIAN_POINT('Ctrl Pts',(-4.47099998458852,-0.319434907277484,
6.01798611679661));
#39534=CARTESIAN_POINT('Ctrl Pts',(-4.43838210287182,-0.158333333333493,
6.03554697854391));
#39535=CARTESIAN_POINT('Ctrl Pts',(-4.44575286345258,0.158333333333495,
6.06394314232543));
#39536=CARTESIAN_POINT('Ctrl Pts',(-4.48587786612484,0.319434907277491,
6.07537408568716));
#39537=CARTESIAN_POINT('Ctrl Pts',(-4.56069164539184,0.636309800095852,
6.08685201887608));
#39538=CARTESIAN_POINT('Ctrl Pts',(-4.62764863713308,0.794772684001649,
6.09033053580248));
#39539=CARTESIAN_POINT('Ctrl Pts',(-4.70010066093033,1.06847604194627,6.07757917622409));
#39540=CARTESIAN_POINT('Ctrl Pts',(-4.72702320461142,1.18514270861313,6.06744101183158));
#39541=CARTESIAN_POINT('Ctrl Pts',(-4.74950649548384,1.30000000000154,6.05268427412358));
#39542=CARTESIAN_POINT('Ctrl Pts',(-4.66877735037765,-1.30000000000264,
5.82675327965573));
#39543=CARTESIAN_POINT('Ctrl Pts',(-4.64706603325485,-1.18514270861388,
5.85625566876312));
#39544=CARTESIAN_POINT('Ctrl Pts',(-4.62226555204477,-1.06847604194665,
5.88336993160839));
#39545=CARTESIAN_POINT('Ctrl Pts',(-4.5578348921036,-0.794772684001648,
5.94049225356201));
#39546=CARTESIAN_POINT('Ctrl Pts',(-4.49946257054952,-0.636309800095834,
5.96973893422419));
#39547=CARTESIAN_POINT('Ctrl Pts',(-4.43931596611307,-0.319434907277479,
6.01540532493937));
#39548=CARTESIAN_POINT('Ctrl Pts',(-4.40795888236539,-0.158333333333491,
6.03257214071144));
#39549=CARTESIAN_POINT('Ctrl Pts',(-4.4152014829334,0.158333333333493,6.05973785294993));
#39550=CARTESIAN_POINT('Ctrl Pts',(-4.45384676217341,0.319434907277487,
6.0697156635662));
#39551=CARTESIAN_POINT('Ctrl Pts',(-4.52865314890444,0.636309800095844,
6.07942682304315));
#39552=CARTESIAN_POINT('Ctrl Pts',(-4.59476100455357,0.794772684001637,
6.08114178701595));
#39553=CARTESIAN_POINT('Ctrl Pts',(-4.67161008343351,1.06847604194625,6.0689607630618));
#39554=CARTESIAN_POINT('Ctrl Pts',(-4.7015700288836,1.18514270861311,6.05971218530979));
#39555=CARTESIAN_POINT('Ctrl Pts',(-4.72822480107566,1.30000000000152,6.04648774372412));
#39556=CARTESIAN_POINT('Ctrl Pts',(-4.65668899582123,-1.30000000000259,
5.82486454122853));
#39557=CARTESIAN_POINT('Ctrl Pts',(-4.63268492611192,-1.18514270861383,
5.85438347155262));
#39558=CARTESIAN_POINT('Ctrl Pts',(-4.60619833147062,-1.0684760419466,5.88143057604729));
#39559=CARTESIAN_POINT('Ctrl Pts',(-4.53927387000397,-0.794772684001615,
5.93820438603154));
#39560=CARTESIAN_POINT('Ctrl Pts',(-4.48123986180072,-0.636309800095808,
5.96667396749507));
#39561=CARTESIAN_POINT('Ctrl Pts',(-4.42100907641847,-0.319434907277466,
6.01224361017099));
#39562=CARTESIAN_POINT('Ctrl Pts',(-4.39048085176486,-0.158333333333485,
6.03003588512597));
#39563=CARTESIAN_POINT('Ctrl Pts',(-4.39774247939571,0.158333333333486,
6.05739059266253));
#39564=CARTESIAN_POINT('Ctrl Pts',(-4.43560985984673,0.319434907277474,
6.06724398831812));
#39565=CARTESIAN_POINT('Ctrl Pts',(-4.51047413856541,0.636309800095818,
6.07680124445811));
#39566=CARTESIAN_POINT('Ctrl Pts',(-4.57611344914273,0.794772684001604,
6.07816850227793));
#39567=CARTESIAN_POINT('Ctrl Pts',(-4.65545714136725,1.06847604194621,6.06609450796775));
#39568=CARTESIAN_POINT('Ctrl Pts',(-4.68713161746142,1.18514270861306,6.0569985637333));
#39569=CARTESIAN_POINT('Ctrl Pts',(-4.71613562525932,1.30000000000147,6.04403306001569));
#39570=CARTESIAN_POINT('Ctrl Pts',(-4.6385500391079,-1.30000000000254,5.82194913720228));
#39571=CARTESIAN_POINT('Ctrl Pts',(-4.6110649246645,-1.18514270861378,5.85117482972643));
#39572=CARTESIAN_POINT('Ctrl Pts',(-4.58203703282286,-1.06847604194656,
5.87804672524838));
#39573=CARTESIAN_POINT('Ctrl Pts',(-4.51141267123745,-0.794772684001582,
5.93468843765767));
#39574=CARTESIAN_POINT('Ctrl Pts',(-4.45405337867724,-0.636309800095782,
5.96342119536517));
#39575=CARTESIAN_POINT('Ctrl Pts',(-4.39376005396835,-0.319434907277453,
6.00937354447557));
#39576=CARTESIAN_POINT('Ctrl Pts',(-4.36448053136045,-0.158333333333478,
6.02816349840518));
#39577=CARTESIAN_POINT('Ctrl Pts',(-4.37165158819181,0.15833333333348,6.05464897920957));
#39578=CARTESIAN_POINT('Ctrl Pts',(-4.40812695127766,0.319434907277462,
6.06222289700424));
#39579=CARTESIAN_POINT('Ctrl Pts',(-4.48297671991519,0.636309800095792,
6.07046727421452));
#39580=CARTESIAN_POINT('Ctrl Pts',(-4.54799913250792,0.794772684001572,
6.07183807993206));
#39581=CARTESIAN_POINT('Ctrl Pts',(-4.63110244925331,1.06847604194617,6.06010258324103));
#39582=CARTESIAN_POINT('Ctrl Pts',(-4.66535361882063,1.18514270861302,6.05135680623418));
#39583=CARTESIAN_POINT('Ctrl Pts',(-4.69788361141755,1.30000000000142,6.03894511389501));
#39584=CARTESIAN_POINT('Ctrl Pts',(-4.61140095727358,-1.30000000000236,
5.81803205131993));
#39585=CARTESIAN_POINT('Ctrl Pts',(-4.57863767876715,-1.18514270861362,
5.84646339489592));
#39586=CARTESIAN_POINT('Ctrl Pts',(-4.54577035281995,-1.06847604194641,
5.87290621620585));
#39587=CARTESIAN_POINT('Ctrl Pts',(-4.46959988439323,-0.794772684001473,
5.92940053906282));
#39588=CARTESIAN_POINT('Ctrl Pts',(-4.41342115796732,-0.636309800095694,
5.95967386773921));
#39589=CARTESIAN_POINT('Ctrl Pts',(-4.35300585333055,-0.319434907277409,
6.00596677714269));
#39590=CARTESIAN_POINT('Ctrl Pts',(-4.32536175684254,-0.158333333333456,
6.02435308394741));
#39591=CARTESIAN_POINT('Ctrl Pts',(-4.33244618099113,0.158333333333458,
6.05024947851058));
#39592=CARTESIAN_POINT('Ctrl Pts',(-4.36716577455457,0.319434907277417,
6.05764609854191));
#39593=CARTESIAN_POINT('Ctrl Pts',(-4.44202972489185,0.636309800095704,
6.06433340585152));
#39594=CARTESIAN_POINT('Ctrl Pts',(-4.50585104292808,0.794772684001463,
6.06303841157629));
#39595=CARTESIAN_POINT('Ctrl Pts',(-4.59453487650259,1.06847604194602,6.05120416246776));
#39596=CARTESIAN_POINT('Ctrl Pts',(-4.63266259593145,1.18514270861285,6.04306544885702));
#39597=CARTESIAN_POINT('Ctrl Pts',(-4.67053008929466,1.30000000000123,6.03191062957247));
#39598=CARTESIAN_POINT('Ctrl Pts',(-4.57222382486624,-1.30000000000223,
5.8129401407569));
#39599=CARTESIAN_POINT('Ctrl Pts',(-4.53192410469008,-1.1851427086135,5.84097066369169));
#39600=CARTESIAN_POINT('Ctrl Pts',(-4.49355515363301,-1.06847604194631,
5.86719880429505));
#39601=CARTESIAN_POINT('Ctrl Pts',(-4.40937566392314,-0.794772684001394,
5.92362719225931));
#39602=CARTESIAN_POINT('Ctrl Pts',(-4.35463820992037,-0.636309800095632,
5.95423463035154));
#39603=CARTESIAN_POINT('Ctrl Pts',(-4.29413126263758,-0.319434907277378,
6.0016073619271));
#39604=CARTESIAN_POINT('Ctrl Pts',(-4.26923747674129,-0.158333333333441,
6.02208737503148));
#39605=CARTESIAN_POINT('Ctrl Pts',(-4.27623577636103,0.158333333333443,
6.04740990767795));
#39606=CARTESIAN_POINT('Ctrl Pts',(-4.30810217356727,0.319434907277386,
6.05218580897125));
#39607=CARTESIAN_POINT('Ctrl Pts',(-4.3829164785186,0.636309800095641,6.05652894968977));
#39608=CARTESIAN_POINT('Ctrl Pts',(-4.44517956069008,0.794772684001385,
6.05363371707215));
#39609=CARTESIAN_POINT('Ctrl Pts',(-4.54192034046459,1.06847604194591,6.04156167104665));
#39610=CARTESIAN_POINT('Ctrl Pts',(-4.5856176637484,1.18514270861273,6.03381010284268));
#39611=CARTESIAN_POINT('Ctrl Pts',(-4.6311368113508,1.30000000000111,6.02353250784577));
#39612=CARTESIAN_POINT('Ctrl Pts',(-4.5421776312674,-1.30000000000179,5.80967119057722));
#39613=CARTESIAN_POINT('Ctrl Pts',(-4.49613780399504,-1.1851427086131,5.83764276311977));
#39614=CARTESIAN_POINT('Ctrl Pts',(-4.45360293348106,-1.06847604194595,
5.86403841702219));
#39615=CARTESIAN_POINT('Ctrl Pts',(-4.36343602479835,-0.794772684001127,
5.92137697064901));
#39616=CARTESIAN_POINT('Ctrl Pts',(-4.31006770585718,-0.636309800095419,
5.95391965294267));
#39617=CARTESIAN_POINT('Ctrl Pts',(-4.24945538152908,-0.31943490727727,
6.00180978892079));
#39618=CARTESIAN_POINT('Ctrl Pts',(-4.22634870087955,-0.158333333333388,
6.02163654041449));
#39619=CARTESIAN_POINT('Ctrl Pts',(-4.23313585212819,0.15833333333339,6.0457016352853));
#39620=CARTESIAN_POINT('Ctrl Pts',(-4.262919571444,0.319434907277279,6.04960166635644));
#39621=CARTESIAN_POINT('Ctrl Pts',(-4.3375811255764,0.636309800095428,6.0514195136938));
#39622=CARTESIAN_POINT('Ctrl Pts',(-4.39840987105965,0.794772684001118,
6.04525831064287));
#39623=CARTESIAN_POINT('Ctrl Pts',(-4.50126981575944,1.06847604194556,6.03256320433072));
#39624=CARTESIAN_POINT('Ctrl Pts',(-4.54925728061249,1.18514270861234,6.02528851544578));
#39625=CARTESIAN_POINT('Ctrl Pts',(-4.60070795159461,1.30000000000067,6.01623437879837));
#39626=CARTESIAN_POINT('Ctrl Pts',(-4.51828305614685,-1.3000000000018,5.80812478043957));
#39627=CARTESIAN_POINT('Ctrl Pts',(-4.46765585165983,-1.18514270861311,
5.83630343387209));
#39628=CARTESIAN_POINT('Ctrl Pts',(-4.42177977482573,-1.06847604194595,
5.86293272402902));
#39629=CARTESIAN_POINT('Ctrl Pts',(-4.32677291519949,-0.794772684001131,
5.92087237234703));
#39630=CARTESIAN_POINT('Ctrl Pts',(-4.27437894207358,-0.636309800095424,
5.95403163528976));
#39631=CARTESIAN_POINT('Ctrl Pts',(-4.21367516448227,-0.319434907277274,
6.0023185425716));
#39632=CARTESIAN_POINT('Ctrl Pts',(-4.19210250856307,-0.158333333333389,
6.02234076606613));
#39633=CARTESIAN_POINT('Ctrl Pts',(-4.19876223512815,0.158333333333391,
6.04576448034503));
#39634=CARTESIAN_POINT('Ctrl Pts',(-4.22682600268163,0.319434907277282,
6.04858357395717));
#39635=CARTESIAN_POINT('Ctrl Pts',(-4.30143862024318,0.636309800095434,
6.04919538720387));
#39636=CARTESIAN_POINT('Ctrl Pts',(-4.36130680882284,0.794772684001125,
6.04243070845557));
#39637=CARTESIAN_POINT('Ctrl Pts',(-4.46906310127177,1.06847604194557,6.02904686633574));
#39638=CARTESIAN_POINT('Ctrl Pts',(-4.52043980609259,1.18514270861235,6.02155875226917));
#39639=CARTESIAN_POINT('Ctrl Pts',(-4.57654950949723,1.30000000000068,6.01237589346949));
#39640=CARTESIAN_POINT('Ctrl Pts',(-4.49429427127325,-1.3000000000017,5.80593985674212));
#39641=CARTESIAN_POINT('Ctrl Pts',(-4.4390616583647,-1.18514270861302,5.83405670837316));
#39642=CARTESIAN_POINT('Ctrl Pts',(-4.38985170429192,-1.06847604194588,
5.86084339263343));
#39643=CARTESIAN_POINT('Ctrl Pts',(-4.29008041270584,-0.794772684001074,
5.91965303920681));
#39644=CARTESIAN_POINT('Ctrl Pts',(-4.23877689554809,-0.636309800095377,
5.95419134348704));
#39645=CARTESIAN_POINT('Ctrl Pts',(-4.17817840066915,-0.31943490727725,
6.00392523034156));
#39646=CARTESIAN_POINT('Ctrl Pts',(-4.15837916125798,-0.158333333333377,
6.02535045698314));
#39647=CARTESIAN_POINT('Ctrl Pts',(-4.16489595666514,0.158333333333379,
6.04806704337612));
#39648=CARTESIAN_POINT('Ctrl Pts',(-4.19097706891447,0.319434907277256,
6.04857621955896));
#39649=CARTESIAN_POINT('Ctrl Pts',(-4.26532832717098,0.636309800095385,
6.04670763514851));
#39650=CARTESIAN_POINT('Ctrl Pts',(-4.32412599322238,0.794772684001067,
6.03822236852455));
#39651=CARTESIAN_POINT('Ctrl Pts',(-4.43670851265054,1.06847604194549,6.02385186523617));
#39652=CARTESIAN_POINT('Ctrl Pts',(-4.49147101150986,1.18514270861226,6.01629863735659));
#39653=CARTESIAN_POINT('Ctrl Pts',(-4.55226320816154,1.30000000000058,6.00741263999135));
#39654=CARTESIAN_POINT('Ctrl Pts',(-4.46442169461097,-1.30000000000149,
5.80418837180094));
#39655=CARTESIAN_POINT('Ctrl Pts',(-4.40347215655026,-1.18514270861283,
5.83279771823915));
#39656=CARTESIAN_POINT('Ctrl Pts',(-4.35013355197629,-1.0684760419457,5.86021766874858));
#39657=CARTESIAN_POINT('Ctrl Pts',(-4.24449348397574,-0.794772684000947,
5.92081549723424));
#39658=CARTESIAN_POINT('Ctrl Pts',(-4.19475469538735,-0.636309800095274,
5.95776264589176));
#39659=CARTESIAN_POINT('Ctrl Pts',(-4.13407346496599,-0.319434907277198,
6.00817306579063));
#39660=CARTESIAN_POINT('Ctrl Pts',(-4.11588361177796,-0.158333333333352,
6.02827899548824));
#39661=CARTESIAN_POINT('Ctrl Pts',(-4.12214305822338,0.158333333333354,
6.04987688497436));
#39662=CARTESIAN_POINT('Ctrl Pts',(-4.14622564528697,0.319434907277206,
6.05018319061237));
#39663=CARTESIAN_POINT('Ctrl Pts',(-4.22040388452318,0.636309800095284,
6.0461812086317));
#39664=CARTESIAN_POINT('Ctrl Pts',(-4.27768379963794,0.794772684000937,
6.03476888272922));
#39665=CARTESIAN_POINT('Ctrl Pts',(-4.39634270097453,1.06847604194531,6.0192033469583));
#39666=CARTESIAN_POINT('Ctrl Pts',(-4.45538559999196,1.18514270861207,6.01164888581944));
#39667=CARTESIAN_POINT('Ctrl Pts',(-4.52210835638382,1.30000000000038,6.003277707217));
#39668=CARTESIAN_POINT('Ctrl Pts',(-4.43460530968309,-1.30000000000149,
5.80256316172534));
#39669=CARTESIAN_POINT('Ctrl Pts',(-4.36805904278203,-1.18514270861283,
5.8318690467023));
#39670=CARTESIAN_POINT('Ctrl Pts',(-4.31069443391872,-1.0684760419457,5.86012150415013));
#39671=CARTESIAN_POINT('Ctrl Pts',(-4.19938217854564,-0.794772684000941,
5.92295670440955));
#39672=CARTESIAN_POINT('Ctrl Pts',(-4.15120156772676,-0.63630980009527,
5.96218462274267));
#39673=CARTESIAN_POINT('Ctrl Pts',(-4.09071095778597,-0.319434907277196,
6.01447543869057));
#39674=CARTESIAN_POINT('Ctrl Pts',(-4.07454410674807,-0.15833333333335,
6.03532811783394));
#39675=CARTESIAN_POINT('Ctrl Pts',(-4.08057825519952,0.158333333333352,
6.0560835465697));
#39676=CARTESIAN_POINT('Ctrl Pts',(-4.10229506552196,0.319434907277203,
6.05445287108395));
#39677=CARTESIAN_POINT('Ctrl Pts',(-4.17606305985547,0.636309800095278,
6.04756284550421));
#39678=CARTESIAN_POINT('Ctrl Pts',(-4.23185985371759,0.794772684000934,
6.03393132239186));
#39679=CARTESIAN_POINT('Ctrl Pts',(-4.35633249000634,1.06847604194531,6.01618889847783));
#39680=CARTESIAN_POINT('Ctrl Pts',(-4.41950097569454,1.18514270861206,6.00792908300874));
#39681=CARTESIAN_POINT('Ctrl Pts',(-4.49195835498728,1.30000000000037,5.99908948996133));
#39682=CARTESIAN_POINT('Ctrl Pts',(-4.41385708995499,-1.30000000000142,
5.80251373423967));
#39683=CARTESIAN_POINT('Ctrl Pts',(-4.34325629992991,-1.18514270861277,
5.83235874410777));
#39684=CARTESIAN_POINT('Ctrl Pts',(-4.28299099688123,-1.06847604194565,
5.86130912435199));
#39685=CARTESIAN_POINT('Ctrl Pts',(-4.16764313332899,-0.794772684000904,
5.9261235208185));
#39686=CARTESIAN_POINT('Ctrl Pts',(-4.12092017336752,-0.63630980009524,
5.96846324925116));
#39687=CARTESIAN_POINT('Ctrl Pts',(-4.06024674814721,-0.319434907277181,
6.02065767248337));
#39688=CARTESIAN_POINT('Ctrl Pts',(-4.04465236031601,-0.158333333333343,
6.03798273283064));
#39689=CARTESIAN_POINT('Ctrl Pts',(-4.05038226546884,0.158333333333345,
6.05754542838412));
#39690=CARTESIAN_POINT('Ctrl Pts',(-4.07104113219228,0.319434907277188,
6.05764658780402));
#39691=CARTESIAN_POINT('Ctrl Pts',(-4.14474138702257,0.636309800095249,
6.04965181419876));
#39692=CARTESIAN_POINT('Ctrl Pts',(-4.19931517653417,0.794772684000895,
6.03347707935452));
#39693=CARTESIAN_POINT('Ctrl Pts',(-4.32799069168609,1.06847604194526,6.01402650668398));
#39694=CARTESIAN_POINT('Ctrl Pts',(-4.39414832245677,1.185142708612,6.00525411630719));
#39695=CARTESIAN_POINT('Ctrl Pts',(-4.47076472138661,1.3000000000003,5.99612876774794));
#39696=CARTESIAN_POINT('Ctrl Pts',(-4.39907707321258,-1.3000000000014,5.80214342814134));
#39697=CARTESIAN_POINT('Ctrl Pts',(-4.32596135091668,-1.18514270861275,
5.83318873155966));
#39698=CARTESIAN_POINT('Ctrl Pts',(-4.26382414376078,-1.06847604194563,
5.86283274193729));
#39699=CARTESIAN_POINT('Ctrl Pts',(-4.14563733094301,-0.794772684000892,
5.9280790689217));
#39700=CARTESIAN_POINT('Ctrl Pts',(-4.09911568145707,-0.636309800095228,
5.96873290910518));
#39701=CARTESIAN_POINT('Ctrl Pts',(-4.03822628354595,-0.319434907277174,
6.02007589595103));
#39702=CARTESIAN_POINT('Ctrl Pts',(-4.02347322566431,-0.15833333333334,
6.03681301517062));
#39703=CARTESIAN_POINT('Ctrl Pts',(-4.02930776445731,0.158333333333342,
6.05694737783173));
#39704=CARTESIAN_POINT('Ctrl Pts',(-4.04940391664942,0.319434907277182,
6.05905497389403));
#39705=CARTESIAN_POINT('Ctrl Pts',(-4.12317888700689,0.636309800095237,
6.05135115292042));
#39706=CARTESIAN_POINT('Ctrl Pts',(-4.17687402913407,0.794772684000879,
6.03377636155464));
#39707=CARTESIAN_POINT('Ctrl Pts',(-4.30833967460458,1.06847604194524,6.01351250464339));
#39708=CARTESIAN_POINT('Ctrl Pts',(-4.37648281330616,1.18514270861198,6.00445204719333));
#39709=CARTESIAN_POINT('Ctrl Pts',(-4.45586248406738,1.30000000000029,5.99510260510017));
#39710=CARTESIAN_POINT('Ctrl Pts',(-4.38139208292461,-1.30000000000138,
5.80261733027026));
#39711=CARTESIAN_POINT('Ctrl Pts',(-4.3048977109199,-1.18514270861273,5.83519453478588));
#39712=CARTESIAN_POINT('Ctrl Pts',(-4.24018476782454,-1.06847604194561,
5.86555166982907));
#39713=CARTESIAN_POINT('Ctrl Pts',(-4.11790238114195,-0.794772684000877,
5.93055392009809));
#39714=CARTESIAN_POINT('Ctrl Pts',(-4.0711888923754,-0.636309800095217,
5.96776653449272));
#39715=CARTESIAN_POINT('Ctrl Pts',(-4.00967332532343,-0.319434907277169,
6.017042557179));
#39716=CARTESIAN_POINT('Ctrl Pts',(-3.99607174541107,-0.158333333333337,
6.03316436429983));
#39717=CARTESIAN_POINT('Ctrl Pts',(-4.00186520345239,0.158333333333339,
6.05321439144484));
#39718=CARTESIAN_POINT('Ctrl Pts',(-4.02082482242209,0.319434907277176,
6.05620237179938));
#39719=CARTESIAN_POINT('Ctrl Pts',(-4.0950281634806,0.636309800095226,6.04968201126514));
#39720=CARTESIAN_POINT('Ctrl Pts',(-4.14852774059524,0.794772684000865,
6.03365040706671));
#39721=CARTESIAN_POINT('Ctrl Pts',(-4.28409830645338,1.06847604194522,6.01340395768109));
#39722=CARTESIAN_POINT('Ctrl Pts',(-4.3549180638185,1.18514270861197,6.00393822894615));
#39723=CARTESIAN_POINT('Ctrl Pts',(-4.43787410397329,1.30000000000027,5.99377070921041));
#39724=CARTESIAN_POINT('Ctrl Pts',(-4.36932387841515,-1.30000000000134,
5.80281598958122));
#39725=CARTESIAN_POINT('Ctrl Pts',(-4.29080148664791,-1.18514270861269,
5.83777836890749));
#39726=CARTESIAN_POINT('Ctrl Pts',(-4.22452488361665,-1.06847604194558,
5.86911453240873));
#39727=CARTESIAN_POINT('Ctrl Pts',(-4.09970289376746,-0.794772684000851,
5.93313005489667));
#39728=CARTESIAN_POINT('Ctrl Pts',(-4.05265002448005,-0.636309800095197,
5.96374672476965));
#39729=CARTESIAN_POINT('Ctrl Pts',(-3.99084012998884,-0.319434907277159,
6.00955609589528));
#39730=CARTESIAN_POINT('Ctrl Pts',(-3.97832338063956,-0.158333333333332,
6.02572522045514));
#39731=CARTESIAN_POINT('Ctrl Pts',(-3.98412215794982,0.158333333333334,
6.04561777586163));
#39732=CARTESIAN_POINT('Ctrl Pts',(-4.00209599199945,0.319434907277167,
6.04853496477295));
#39733=CARTESIAN_POINT('Ctrl Pts',(-4.07641358158954,0.636309800095206,
6.04488755346973));
#39734=CARTESIAN_POINT('Ctrl Pts',(-4.12975510290133,0.79477268400084,6.03438726539486));
#39735=CARTESIAN_POINT('Ctrl Pts',(-4.26788601364085,1.06847604194518,6.01517679411596));
#39736=CARTESIAN_POINT('Ctrl Pts',(-4.34039737044277,1.18514270861192,6.00502961961175));
#39737=CARTESIAN_POINT('Ctrl Pts',(-4.42562833104214,1.30000000000022,5.99305077180184));
#39738=CARTESIAN_POINT('Ctrl Pts',(-4.36108289177568,-1.30000000000134,
5.80034987084412));
#39739=CARTESIAN_POINT('Ctrl Pts',(-4.28280795672196,-1.18514270861269,
5.83535608437193));
#39740=CARTESIAN_POINT('Ctrl Pts',(-4.21670728203319,-1.06847604194558,
5.86639564184631));
#39741=CARTESIAN_POINT('Ctrl Pts',(-4.09212647700321,-0.794772684000851,
5.92893946004396));
#39742=CARTESIAN_POINT('Ctrl Pts',(-4.04497787349015,-0.636309800095197,
5.95699216849829));
#39743=CARTESIAN_POINT('Ctrl Pts',(-3.98316982931346,-0.319434907277159,
6.00111495923036));
#39744=CARTESIAN_POINT('Ctrl Pts',(-3.97060749458543,-0.158333333333332,
6.01730981540119));
#39745=CARTESIAN_POINT('Ctrl Pts',(-3.97642822268415,0.158333333333334,
6.03696656310354));
#39746=CARTESIAN_POINT('Ctrl Pts',(-3.99446677770813,0.319434907277167,
6.03934216248958));
#39747=CARTESIAN_POINT('Ctrl Pts',(-4.06883296350448,0.636309800095206,
6.03747145037915));
#39748=CARTESIAN_POINT('Ctrl Pts',(-4.12234304385768,0.79477268400084,6.03061645411867));
#39749=CARTESIAN_POINT('Ctrl Pts',(-4.26021093575302,1.06847604194518,6.01272564041898));
#39750=CARTESIAN_POINT('Ctrl Pts',(-4.33251297633884,1.18514270861192,6.00255688732873));
#39751=CARTESIAN_POINT('Ctrl Pts',(-4.41743915561784,1.30000000000022,5.98996365147884));
#39752=CARTESIAN_POINT('Ctrl Pts',(-4.36108289177477,-1.3,5.80034987084453));
#39753=CARTESIAN_POINT('Ctrl Pts',(-4.28280795672145,-1.18514270861178,
5.83535608437217));
#39754=CARTESIAN_POINT('Ctrl Pts',(-4.21670728203298,-1.06847604194512,
5.86639564184641));
#39755=CARTESIAN_POINT('Ctrl Pts',(-4.09212647700321,-0.794772684000851,
5.92893946004396));
#39756=CARTESIAN_POINT('Ctrl Pts',(-4.04497787349015,-0.636309800095197,
5.95699216849829));
#39757=CARTESIAN_POINT('Ctrl Pts',(-3.98316982931346,-0.319434907277159,
6.00111495923036));
#39758=CARTESIAN_POINT('Ctrl Pts',(-3.97060749458543,-0.158333333333332,
6.01730981540119));
#39759=CARTESIAN_POINT('Ctrl Pts',(-3.97642822268415,0.158333333333334,
6.03696656310354));
#39760=CARTESIAN_POINT('Ctrl Pts',(-3.99446677770813,0.319434907277167,
6.03934216248958));
#39761=CARTESIAN_POINT('Ctrl Pts',(-4.06883296350448,0.636309800095206,
6.03747145037915));
#39762=CARTESIAN_POINT('Ctrl Pts',(-4.12234304385768,0.79477268400084,6.03061645411867));
#39763=CARTESIAN_POINT('Ctrl Pts',(-4.26021093575299,1.06847604194511,6.01272564041899));
#39764=CARTESIAN_POINT('Ctrl Pts',(-4.33251297633875,1.18514270861178,6.00255688732874));
#39765=CARTESIAN_POINT('Ctrl Pts',(-4.41743915561768,1.3,5.98996365147886));
#39766=CARTESIAN_POINT('',(-4.76943094974079,-1.2,5.8752251452965));
#39767=CARTESIAN_POINT('Ctrl Pts',(-4.76943094974079,-1.2,5.8752251452965));
#39768=CARTESIAN_POINT('Ctrl Pts',(-4.75137040040528,-1.21532879594667,
5.8674796759455));
#39769=CARTESIAN_POINT('Ctrl Pts',(-4.75128192428144,-1.21526382380562,
5.86695113090664));
#39770=CARTESIAN_POINT('Ctrl Pts',(-4.72841491494507,-1.23443202165904,
5.85651346558973));
#39771=CARTESIAN_POINT('Ctrl Pts',(-4.72629960582589,-1.2362463555996,5.85568195490476));
#39772=CARTESIAN_POINT('Ctrl Pts',(-4.69026521558868,-1.26666727514779,
5.84039241832176));
#39773=CARTESIAN_POINT('Ctrl Pts',(-4.67050837960332,-1.28326560327169,
5.83192379066369));
#39774=CARTESIAN_POINT('Ctrl Pts',(-4.65068316839847,-1.30000000000257,
5.82390186863356));
#39775=CARTESIAN_POINT('',(-4.80892752421831,-0.653834841417905,6.02666455497168));
#39776=CARTESIAN_POINT('Ctrl Pts',(-4.80892752424277,-0.653834841417227,
6.02666455496296));
#39777=CARTESIAN_POINT('Ctrl Pts',(-4.80506824066303,-0.718001778396551,
6.01084724107461));
#39778=CARTESIAN_POINT('Ctrl Pts',(-4.80187412133315,-0.763814897456566,
5.99800871203435));
#39779=CARTESIAN_POINT('Ctrl Pts',(-4.78912428622677,-0.949547840785904,
5.9477928208045));
#39780=CARTESIAN_POINT('Ctrl Pts',(-4.78201437664528,-1.04870126019181,
5.92052777579179));
#39781=CARTESIAN_POINT('Ctrl Pts',(-4.76943094974079,-1.2,5.8752251452965));
#39782=CARTESIAN_POINT('',(-4.84008270153004,0.653834841531101,6.16264786964614));
#39783=CARTESIAN_POINT('Ctrl Pts',(-4.84008270153004,0.653834841531101,
6.16264786964614));
#39784=CARTESIAN_POINT('Ctrl Pts',(-4.79944689285444,0.575793690744437,
6.15340775242001));
#39785=CARTESIAN_POINT('Ctrl Pts',(-4.76554165986554,0.493915978123552,
6.14498973164795));
#39786=CARTESIAN_POINT('Ctrl Pts',(-4.71701543835946,0.338192716619548,
6.13032379860722));
#39787=CARTESIAN_POINT('Ctrl Pts',(-4.70027540041615,0.265706975690616,
6.12394954385036));
#39788=CARTESIAN_POINT('Ctrl Pts',(-4.679340251876,0.129738926799289,6.11140069271612));
#39789=CARTESIAN_POINT('Ctrl Pts',(-4.67367418869134,0.0666398175577108,
6.10535820904037));
#39790=CARTESIAN_POINT('Ctrl Pts',(-4.67033333649289,-0.0595502776848976,
6.09244197012475));
#39791=CARTESIAN_POINT('Ctrl Pts',(-4.67261687834793,-0.122795537269838,
6.08547477710846));
#39792=CARTESIAN_POINT('Ctrl Pts',(-4.68654559054128,-0.260150036719889,
6.07010358967871));
#39793=CARTESIAN_POINT('Ctrl Pts',(-4.69982117916003,-0.333952578847895,
6.06166611745586));
#39794=CARTESIAN_POINT('Ctrl Pts',(-4.7411101764999,-0.491147154103011,
6.0442087836093));
#39795=CARTESIAN_POINT('Ctrl Pts',(-4.77132361579784,-0.574255930628569,
6.03514257932434));
#39796=CARTESIAN_POINT('Ctrl Pts',(-4.80892752418791,-0.653834841429502,
6.02666455494571));
#39797=CARTESIAN_POINT('',(-4.82444443480448,1.2,6.09219320480325));
#39798=CARTESIAN_POINT('Ctrl Pts',(-4.82444443480448,1.2,6.09219320480325));
#39799=CARTESIAN_POINT('Ctrl Pts',(-4.82723947618274,1.13403856392639,6.10436547336207));
#39800=CARTESIAN_POINT('Ctrl Pts',(-4.83083759668361,1.03830672751198,6.1202516992187));
#39801=CARTESIAN_POINT('Ctrl Pts',(-4.83765957916731,0.795125399809678,
6.15132335450788));
#39802=CARTESIAN_POINT('Ctrl Pts',(-4.83870912604018,0.741480188480013,
6.15623903433055));
#39803=CARTESIAN_POINT('Ctrl Pts',(-4.84008270153004,0.653834841531101,
6.16264786964614));
#39804=CARTESIAN_POINT('Ctrl Pts',(-4.70979325221221,1.30000000000036,6.04226621306413));
#39805=CARTESIAN_POINT('Ctrl Pts',(-4.72229378593043,1.28915014241713,6.04766738572323));
#39806=CARTESIAN_POINT('Ctrl Pts',(-4.72828552194237,1.28375313994558,6.04947303494543));
#39807=CARTESIAN_POINT('Ctrl Pts',(-4.75229651621339,1.26293974657568,6.06020423652264));
#39808=CARTESIAN_POINT('Ctrl Pts',(-4.75719339679975,1.25866690039675,6.06233008665453));
#39809=CARTESIAN_POINT('Ctrl Pts',(-4.77865120550695,1.23990130702929,6.07145421674264));
#39810=CARTESIAN_POINT('Ctrl Pts',(-4.80287991746654,1.21864618379946,6.08159730856588));
#39811=CARTESIAN_POINT('Ctrl Pts',(-4.82444443480448,1.2,6.09219320480325));
#39812=CARTESIAN_POINT('Ctrl Pts',(-4.36108289177477,-1.3,5.80034987084453));
#39813=CARTESIAN_POINT('Ctrl Pts',(-4.28280795672145,-1.18514270861178,
5.83535608437217));
#39814=CARTESIAN_POINT('Ctrl Pts',(-4.21670728203298,-1.06847604194512,
5.86639564184641));
#39815=CARTESIAN_POINT('Ctrl Pts',(-4.09212647700321,-0.794772684000851,
5.92893946004396));
#39816=CARTESIAN_POINT('Ctrl Pts',(-4.04497787349015,-0.636309800095197,
5.95699216849828));
#39817=CARTESIAN_POINT('Ctrl Pts',(-3.98316982931346,-0.319434907277159,
6.00111495923036));
#39818=CARTESIAN_POINT('Ctrl Pts',(-3.97060749458542,-0.158333333333333,
6.01730981540119));
#39819=CARTESIAN_POINT('Ctrl Pts',(-3.97642822268415,0.158333333333334,
6.03696656310354));
#39820=CARTESIAN_POINT('Ctrl Pts',(-3.99446677770813,0.319434907277167,
6.03934216248957));
#39821=CARTESIAN_POINT('Ctrl Pts',(-4.06883296350447,0.636309800095206,
6.03747145037914));
#39822=CARTESIAN_POINT('Ctrl Pts',(-4.12234304385768,0.79477268400084,6.03061645411867));
#39823=CARTESIAN_POINT('Ctrl Pts',(-4.26021093575298,1.06847604194511,6.01272564041899));
#39824=CARTESIAN_POINT('Ctrl Pts',(-4.33251297633875,1.18514270861178,6.00255688732874));
#39825=CARTESIAN_POINT('Ctrl Pts',(-4.41743915561768,1.3,5.98996365147886));
#39826=CARTESIAN_POINT('Ctrl Pts',(-4.33573021748671,-1.3,5.72771137429423));
#39827=CARTESIAN_POINT('Ctrl Pts',(-4.25817731391276,-1.18514270861178,
5.76429225461164));
#39828=CARTESIAN_POINT('Ctrl Pts',(-4.19261998989961,-1.06847604194512,
5.79640908596292));
#39829=CARTESIAN_POINT('Ctrl Pts',(-4.06888164522439,-0.794772684000851,
5.86029254519278));
#39830=CARTESIAN_POINT('Ctrl Pts',(-4.02167596618816,-0.636309800095197,
5.88762989336549));
#39831=CARTESIAN_POINT('Ctrl Pts',(-3.96004957503507,-0.319434907277159,
5.93111105698402));
#39832=CARTESIAN_POINT('Ctrl Pts',(-3.94727563345509,-0.158333333333333,
5.9460825267282));
#39833=CARTESIAN_POINT('Ctrl Pts',(-3.95343774500623,0.158333333333334,
5.96562835222289));
#39834=CARTESIAN_POINT('Ctrl Pts',(-3.97202419499028,0.319434907277167,
5.96911807140563));
#39835=CARTESIAN_POINT('Ctrl Pts',(-4.04691448012462,0.636309800095206,
5.96765967356581));
#39836=CARTESIAN_POINT('Ctrl Pts',(-4.10079886363323,0.79477268400084,5.96141696408104));
#39837=CARTESIAN_POINT('Ctrl Pts',(-4.2385608990303,1.06847604194511,5.94194717224782));
#39838=CARTESIAN_POINT('Ctrl Pts',(-4.3106693138487,1.18514270861178,5.93058751276968));
#39839=CARTESIAN_POINT('Ctrl Pts',(-4.39525406294861,1.3,5.91629594527112));
#39840=CARTESIAN_POINT('Ctrl Pts',(-4.31037754319864,-1.3,5.65507287774392));
#39841=CARTESIAN_POINT('Ctrl Pts',(-4.23354667110408,-1.18514270861178,
5.69322842485112));
#39842=CARTESIAN_POINT('Ctrl Pts',(-4.16853269776624,-1.06847604194512,
5.72642253007944));
#39843=CARTESIAN_POINT('Ctrl Pts',(-4.04563681344557,-0.794772684000851,
5.79164563034159));
#39844=CARTESIAN_POINT('Ctrl Pts',(-3.99837405888618,-0.636309800095197,
5.81826761823271));
#39845=CARTESIAN_POINT('Ctrl Pts',(-3.93692932075669,-0.319434907277159,
5.86110715473768));
#39846=CARTESIAN_POINT('Ctrl Pts',(-3.92394377232475,-0.158333333333333,
5.87485523805521));
#39847=CARTESIAN_POINT('Ctrl Pts',(-3.9304472673283,0.158333333333334,5.89429014134224));
#39848=CARTESIAN_POINT('Ctrl Pts',(-3.94958161227244,0.319434907277167,
5.89889398032169));
#39849=CARTESIAN_POINT('Ctrl Pts',(-4.02499599674477,0.636309800095206,
5.89784789675249));
#39850=CARTESIAN_POINT('Ctrl Pts',(-4.07925468340879,0.79477268400084,5.89221747404342));
#39851=CARTESIAN_POINT('Ctrl Pts',(-4.21691086230761,1.06847604194511,5.87116870407665));
#39852=CARTESIAN_POINT('Ctrl Pts',(-4.28882565135864,1.18514270861178,5.85861813821062));
#39853=CARTESIAN_POINT('Ctrl Pts',(-4.37306897027954,1.3,5.84262823906338));
#39854=CARTESIAN_POINT('Ctrl Pts',(-4.28502486891058,-1.3,5.58243438119362));
#39855=CARTESIAN_POINT('Ctrl Pts',(-4.20891602829539,-1.18514270861178,
5.62216459509059));
#39856=CARTESIAN_POINT('Ctrl Pts',(-4.14444540563287,-1.06847604194512,
5.65643597419595));
#39857=CARTESIAN_POINT('Ctrl Pts',(-4.02239198166675,-0.794772684000851,
5.72299871549041));
#39858=CARTESIAN_POINT('Ctrl Pts',(-3.9750721515842,-0.636309800095197,
5.74890534309992));
#39859=CARTESIAN_POINT('Ctrl Pts',(-3.91380906647831,-0.319434907277159,
5.79110325249133));
#39860=CARTESIAN_POINT('Ctrl Pts',(-3.90061191119441,-0.158333333333333,
5.80362794938222));
#39861=CARTESIAN_POINT('Ctrl Pts',(-3.90745678965038,0.158333333333334,
5.8229519304616));
#39862=CARTESIAN_POINT('Ctrl Pts',(-3.9271390295546,0.319434907277167,5.82866988923775));
#39863=CARTESIAN_POINT('Ctrl Pts',(-4.00307751336492,0.636309800095206,
5.82803611993916));
#39864=CARTESIAN_POINT('Ctrl Pts',(-4.05771050318434,0.79477268400084,5.82301798400579));
#39865=CARTESIAN_POINT('Ctrl Pts',(-4.19526082558492,1.06847604194511,5.80039023590548));
#39866=CARTESIAN_POINT('Ctrl Pts',(-4.26698198886859,1.18514270861178,5.78664876365156));
#39867=CARTESIAN_POINT('Ctrl Pts',(-4.35088387761047,1.3,5.76896053285564));
#39868=CARTESIAN_POINT('Ctrl Pts',(-4.28502486891058,-1.3,5.58243438119362));
#39869=CARTESIAN_POINT('Ctrl Pts',(-4.20891602829539,-1.18514270861178,
5.62216459509059));
#39870=CARTESIAN_POINT('Ctrl Pts',(-4.14444540563287,-1.06847604194512,
5.65643597419595));
#39871=CARTESIAN_POINT('Ctrl Pts',(-4.02239198166675,-0.794772684000851,
5.72299871549041));
#39872=CARTESIAN_POINT('Ctrl Pts',(-3.9750721515842,-0.636309800095197,
5.74890534309992));
#39873=CARTESIAN_POINT('Ctrl Pts',(-3.91380906647831,-0.319434907277159,
5.79110325249133));
#39874=CARTESIAN_POINT('Ctrl Pts',(-3.90061191119441,-0.158333333333332,
5.80362794938222));
#39875=CARTESIAN_POINT('Ctrl Pts',(-3.90745678965039,0.158333333333334,
5.8229519304616));
#39876=CARTESIAN_POINT('Ctrl Pts',(-3.9271390295546,0.319434907277167,5.82866988923776));
#39877=CARTESIAN_POINT('Ctrl Pts',(-4.00307751336492,0.636309800095206,
5.82803611993916));
#39878=CARTESIAN_POINT('Ctrl Pts',(-4.05771050318434,0.79477268400084,5.82301798400579));
#39879=CARTESIAN_POINT('Ctrl Pts',(-4.19526082558492,1.06847604194511,5.80039023590548));
#39880=CARTESIAN_POINT('Ctrl Pts',(-4.26698198886859,1.18514270861178,5.78664876365156));
#39881=CARTESIAN_POINT('Ctrl Pts',(-4.35088387761047,1.3,5.76896053285564));
#39882=CARTESIAN_POINT('Ctrl Pts',(-4.28502486891571,-1.30000000000774,
5.58243438119094));
#39883=CARTESIAN_POINT('Ctrl Pts',(-4.20891602829829,-1.18514270861703,
5.62216459508905));
#39884=CARTESIAN_POINT('Ctrl Pts',(-4.14444540563406,-1.06847604194778,
5.6564359741953));
#39885=CARTESIAN_POINT('Ctrl Pts',(-4.02239198166675,-0.794772684000851,
5.72299871549041));
#39886=CARTESIAN_POINT('Ctrl Pts',(-3.9750721515842,-0.636309800095197,
5.74890534309992));
#39887=CARTESIAN_POINT('Ctrl Pts',(-3.91380906647831,-0.319434907277159,
5.79110325249133));
#39888=CARTESIAN_POINT('Ctrl Pts',(-3.90061191119441,-0.158333333333332,
5.80362794938222));
#39889=CARTESIAN_POINT('Ctrl Pts',(-3.90745678965039,0.158333333333335,
5.8229519304616));
#39890=CARTESIAN_POINT('Ctrl Pts',(-3.9271390295546,0.319434907277167,5.82866988923776));
#39891=CARTESIAN_POINT('Ctrl Pts',(-4.00307751336492,0.636309800095206,
5.82803611993916));
#39892=CARTESIAN_POINT('Ctrl Pts',(-4.05771050318434,0.79477268400084,5.8230179840058));
#39893=CARTESIAN_POINT('Ctrl Pts',(-4.19526082558604,1.06847604194732,5.8003902359053));
#39894=CARTESIAN_POINT('Ctrl Pts',(-4.26698198887127,1.18514270861614,5.78664876365104));
#39895=CARTESIAN_POINT('Ctrl Pts',(-4.35088387761518,1.30000000000644,5.76896053285465));
#39896=CARTESIAN_POINT('Ctrl Pts',(-4.28983548714971,-1.30000000000774,
5.57512337186273));
#39897=CARTESIAN_POINT('Ctrl Pts',(-4.21384120150069,-1.18514270861703,
5.61552978208877));
#39898=CARTESIAN_POINT('Ctrl Pts',(-4.14921392204009,-1.06847604194778,
5.64994165162069));
#39899=CARTESIAN_POINT('Ctrl Pts',(-4.0261720361017,-0.794772684000851,
5.7155913661023));
#39900=CARTESIAN_POINT('Ctrl Pts',(-3.97684592438828,-0.636309800095197,
5.73844981416284));
#39901=CARTESIAN_POINT('Ctrl Pts',(-3.91457783683304,-0.319434907277159,
5.77918177958783));
#39902=CARTESIAN_POINT('Ctrl Pts',(-3.9017513801954,-0.158333333333332,
5.79210658959415));
#39903=CARTESIAN_POINT('Ctrl Pts',(-3.90875262150678,0.158333333333335,
5.81160844076292));
#39904=CARTESIAN_POINT('Ctrl Pts',(-3.9283828574657,0.319434907277167,5.81733237662104));
#39905=CARTESIAN_POINT('Ctrl Pts',(-4.00531418532216,0.636309800095206,
5.81806199192622));
#39906=CARTESIAN_POINT('Ctrl Pts',(-4.06137678322638,0.79477268400084,5.81517441552251));
#39907=CARTESIAN_POINT('Ctrl Pts',(-4.19998727432042,1.06847604194732,5.79359553632442));
#39908=CARTESIAN_POINT('Ctrl Pts',(-4.27202510727,1.18514270861614,5.77999061530212));
#39909=CARTESIAN_POINT('Ctrl Pts',(-4.35610142759883,1.30000000000644,5.76212147048619));
#39910=CARTESIAN_POINT('Ctrl Pts',(-4.29926460392529,-1.3000000000078,5.56730754667784));
#39911=CARTESIAN_POINT('Ctrl Pts',(-4.22610897742813,-1.18514270861708,
5.60781633231694));
#39912=CARTESIAN_POINT('Ctrl Pts',(-4.1632069654871,-1.06847604194782,5.64177322539493));
#39913=CARTESIAN_POINT('Ctrl Pts',(-4.04157863525366,-0.794772684000886,
5.70508425893971));
#39914=CARTESIAN_POINT('Ctrl Pts',(-3.98891499615366,-0.636309800095225,
5.72360628567257));
#39915=CARTESIAN_POINT('Ctrl Pts',(-3.92508927153551,-0.319434907277173,
5.76200735853348));
#39916=CARTESIAN_POINT('Ctrl Pts',(-3.91155422483044,-0.158333333333339,
5.77560738379245));
#39917=CARTESIAN_POINT('Ctrl Pts',(-3.91868087788676,0.158333333333341,
5.79530051439071));
#39918=CARTESIAN_POINT('Ctrl Pts',(-3.9391737882875,0.31943490727718,5.80045397900698));
#39919=CARTESIAN_POINT('Ctrl Pts',(-4.01785980381973,0.636309800095233,
5.80408037571868));
#39920=CARTESIAN_POINT('Ctrl Pts',(-4.07738162668686,0.794772684000876,
5.80643110136374));
#39921=CARTESIAN_POINT('Ctrl Pts',(-4.21455464773777,1.06847604194737,5.78710873781506));
#39922=CARTESIAN_POINT('Ctrl Pts',(-4.28480848471052,1.18514270861619,5.77367406491117));
#39923=CARTESIAN_POINT('Ctrl Pts',(-4.36593904060384,1.3000000000065,5.75516865431955));
#39924=CARTESIAN_POINT('Ctrl Pts',(-4.31087898980036,-1.3000000000078,5.55775119234527));
#39925=CARTESIAN_POINT('Ctrl Pts',(-4.24062896799711,-1.18514270861708,
5.59707972499315));
#39926=CARTESIAN_POINT('Ctrl Pts',(-4.17978777933664,-1.06847604194783,
5.6299959312519));
#39927=CARTESIAN_POINT('Ctrl Pts',(-4.0609687490848,-0.794772684000887,
5.69122519583298));
#39928=CARTESIAN_POINT('Ctrl Pts',(-4.00733049135218,-0.636309800095225,
5.70868832752417));
#39929=CARTESIAN_POINT('Ctrl Pts',(-3.94313274773527,-0.319434907277173,
5.74594287877534));
#39930=CARTESIAN_POINT('Ctrl Pts',(-3.92831311803112,-0.158333333333339,
5.75941308314454));
#39931=CARTESIAN_POINT('Ctrl Pts',(-3.93542313374035,0.158333333333342,
5.77910883389326));
#39932=CARTESIAN_POINT('Ctrl Pts',(-3.95702358944834,0.319434907277181,
5.78405811617581));
#39933=CARTESIAN_POINT('Ctrl Pts',(-4.0363744588543,0.636309800095234,5.78952204913013));
#39934=CARTESIAN_POINT('Ctrl Pts',(-4.09763070495285,0.794772684000876,
5.79465216253709));
#39935=CARTESIAN_POINT('Ctrl Pts',(-4.23209270204518,1.06847604194737,5.77753302310594));
#39936=CARTESIAN_POINT('Ctrl Pts',(-4.30017341612242,1.18514270861619,5.76481597001355));
#39937=CARTESIAN_POINT('Ctrl Pts',(-4.37813122804306,1.3000000000065,5.74679210496196));
#39938=CARTESIAN_POINT('Ctrl Pts',(-4.31756355120264,-1.30000000000782,
5.55178320730319));
#39939=CARTESIAN_POINT('Ctrl Pts',(-4.24867237672523,-1.1851427086171,5.59025076843429));
#39940=CARTESIAN_POINT('Ctrl Pts',(-4.18884808425587,-1.06847604194784,
5.62257789921357));
#39941=CARTESIAN_POINT('Ctrl Pts',(-4.07158831210657,-0.794772684000899,
5.68307441583173));
#39942=CARTESIAN_POINT('Ctrl Pts',(-4.01794799809661,-0.636309800095235,
5.70116577658724));
#39943=CARTESIAN_POINT('Ctrl Pts',(-3.95376926507575,-0.319434907277177,
5.7383041614915));
#39944=CARTESIAN_POINT('Ctrl Pts',(-3.93818730491617,-0.158333333333341,
5.75138323538562));
#39945=CARTESIAN_POINT('Ctrl Pts',(-3.94525424323687,0.158333333333344,
5.77101756308156));
#39946=CARTESIAN_POINT('Ctrl Pts',(-3.96745835523679,0.319434907277185,
5.77606932698987));
#39947=CARTESIAN_POINT('Ctrl Pts',(-4.04693793081532,0.636309800095243,
5.78198715454197));
#39948=CARTESIAN_POINT('Ctrl Pts',(-4.1086577796612,0.794772684000887,5.78746954738944));
#39949=CARTESIAN_POINT('Ctrl Pts',(-4.24166935314431,1.06847604194739,5.77125294812262));
#39950=CARTESIAN_POINT('Ctrl Pts',(-4.30870002787006,1.18514270861621,5.75901208534449));
#39951=CARTESIAN_POINT('Ctrl Pts',(-4.38518559572466,1.30000000000652,5.74154992472669));
#39952=CARTESIAN_POINT('Ctrl Pts',(-4.3267322227737,-1.30000000000783,5.5439628437342));
#39953=CARTESIAN_POINT('Ctrl Pts',(-4.25987806407973,-1.1851427086171,5.58127837497687));
#39954=CARTESIAN_POINT('Ctrl Pts',(-4.20158070045236,-1.06847604194785,
5.61286286081461));
#39955=CARTESIAN_POINT('Ctrl Pts',(-4.08667003651182,-0.794772684000902,
5.67258948017672));
#39956=CARTESIAN_POINT('Ctrl Pts',(-4.0330896730832,-0.636309800095237,
5.69197918867089));
#39957=CARTESIAN_POINT('Ctrl Pts',(-3.96886713289172,-0.319434907277179,
5.72899314540867));
#39958=CARTESIAN_POINT('Ctrl Pts',(-3.95196301927249,-0.158333333333342,
5.74113914727316));
#39959=CARTESIAN_POINT('Ctrl Pts',(-3.95891563445526,0.158333333333344,
5.76055677660053));
#39960=CARTESIAN_POINT('Ctrl Pts',(-3.98210843439915,0.319434907277186,
5.76585285006701));
#39961=CARTESIAN_POINT('Ctrl Pts',(-4.06184532639253,0.636309800095245,
5.77241526739943));
#39962=CARTESIAN_POINT('Ctrl Pts',(-4.12436285483472,0.794772684000891,
5.77854795651227));
#39963=CARTESIAN_POINT('Ctrl Pts',(-4.25514280214883,1.06847604194739,5.76328404203811));
#39964=CARTESIAN_POINT('Ctrl Pts',(-4.32053563777679,1.18514270861621,5.75147540083709));
#39965=CARTESIAN_POINT('Ctrl Pts',(-4.39471151571447,1.30000000000652,5.73446530142721));
#39966=CARTESIAN_POINT('Ctrl Pts',(-4.33567044487952,-1.30000000000787,
5.53578209593916));
#39967=CARTESIAN_POINT('Ctrl Pts',(-4.27076977516179,-1.18514270861714,
5.57178751878452));
#39968=CARTESIAN_POINT('Ctrl Pts',(-4.21397255168303,-1.06847604194788,
5.60255450794955));
#39969=CARTESIAN_POINT('Ctrl Pts',(-4.10148018510381,-0.794772684000929,
5.66153057808851));
#39970=CARTESIAN_POINT('Ctrl Pts',(-4.04815945570574,-0.636309800095257,
5.68240275508685));
#39971=CARTESIAN_POINT('Ctrl Pts',(-3.98422899902913,-0.319434907277188,
5.71981566023146));
#39972=CARTESIAN_POINT('Ctrl Pts',(-3.96623137841746,-0.158333333333347,
5.73140454462874));
#39973=CARTESIAN_POINT('Ctrl Pts',(-3.973463674695,0.158333333333349,5.75150962599252));
#39974=CARTESIAN_POINT('Ctrl Pts',(-3.99819974918407,0.319434907277196,
5.75849050162669));
#39975=CARTESIAN_POINT('Ctrl Pts',(-4.07786779404668,0.636309800095265,
5.76515753861331));
#39976=CARTESIAN_POINT('Ctrl Pts',(-4.13987208619196,0.794772684000913,
5.76911726872872));
#39977=CARTESIAN_POINT('Ctrl Pts',(-4.2681142673931,1.06847604194743,5.75422153983162));
#39978=CARTESIAN_POINT('Ctrl Pts',(-4.33195611341596,1.18514270861625,5.74306496903181));
#39979=CARTESIAN_POINT('Ctrl Pts',(-4.40412851706027,1.30000000000657,5.72719963653066));
#39980=CARTESIAN_POINT('Ctrl Pts',(-4.34632504743441,-1.30000000000789,
5.52463757271305));
#39981=CARTESIAN_POINT('Ctrl Pts',(-4.28387476894886,-1.18514270861716,
5.55912000438341));
#39982=CARTESIAN_POINT('Ctrl Pts',(-4.2289766621989,-1.0684760419479,5.58899711003865));
#39983=CARTESIAN_POINT('Ctrl Pts',(-4.11959808079522,-0.794772684000939,
5.64737997660876));
#39984=CARTESIAN_POINT('Ctrl Pts',(-4.06659446385943,-0.636309800095266,
5.67013156883144));
#39985=CARTESIAN_POINT('Ctrl Pts',(-4.00340218462963,-0.319434907277194,
5.70893556077439));
#39986=CARTESIAN_POINT('Ctrl Pts',(-3.98476119738918,-0.158333333333349,
5.72143444261475));
#39987=CARTESIAN_POINT('Ctrl Pts',(-3.99225312203943,0.158333333333352,
5.74221562590154));
#39988=CARTESIAN_POINT('Ctrl Pts',(-4.01797378492831,0.319434907277202,
5.7492518394961));
#39989=CARTESIAN_POINT('Ctrl Pts',(-4.09726629676795,0.636309800095276,
5.7553158128464));
#39990=CARTESIAN_POINT('Ctrl Pts',(-4.15896884281014,0.794772684000927,
5.75719602556793));
#39991=CARTESIAN_POINT('Ctrl Pts',(-4.28425709447938,1.06847604194744,5.7430159451123));
#39992=CARTESIAN_POINT('Ctrl Pts',(-4.34626539680437,1.18514270861627,5.73279018820648));
#39993=CARTESIAN_POINT('Ctrl Pts',(-4.41604935969341,1.30000000000659,5.71847670580035));
#39994=CARTESIAN_POINT('Ctrl Pts',(-4.35515498779441,-1.30000000000792,
5.51626230029215));
#39995=CARTESIAN_POINT('Ctrl Pts',(-4.29473922787703,-1.18514270861719,
5.54960135559851));
#39996=CARTESIAN_POINT('Ctrl Pts',(-4.24138370795419,-1.06847604194792,
5.57875750051019));
#39997=CARTESIAN_POINT('Ctrl Pts',(-4.13443234998209,-0.794772684000958,
5.63645066812221));
#39998=CARTESIAN_POINT('Ctrl Pts',(-4.08141479981886,-0.636309800095282,
5.6601675095401));
#39999=CARTESIAN_POINT('Ctrl Pts',(-4.01868156676103,-0.319434907277201,
5.69981192468275));
#40000=CARTESIAN_POINT('Ctrl Pts',(-3.99964611770337,-0.158333333333353,
5.71335837626925));
#40001=CARTESIAN_POINT('Ctrl Pts',(-4.00716314167774,0.158333333333356,
5.7342185271067));
#40002=CARTESIAN_POINT('Ctrl Pts',(-4.03324584237705,0.319434907277211,
5.74017555382292));
#40003=CARTESIAN_POINT('Ctrl Pts',(-4.11224760444397,0.636309800095291,
5.745785208225));
#40004=CARTESIAN_POINT('Ctrl Pts',(-4.1742891549149,0.794772684000945,5.74743434259157));
#40005=CARTESIAN_POINT('Ctrl Pts',(-4.29720630175374,1.06847604194747,5.73397154115603));
#40006=CARTESIAN_POINT('Ctrl Pts',(-4.35762891092206,1.1851427086163,5.7243040306088));
#40007=CARTESIAN_POINT('Ctrl Pts',(-4.42526785092076,1.30000000000662,5.71079655740988));
#40008=CARTESIAN_POINT('Ctrl Pts',(-4.37078301240193,-1.30000000000792,
5.50197740006034));
#40009=CARTESIAN_POINT('Ctrl Pts',(-4.3135809809026,-1.18514270861719,5.53274415335154));
#40010=CARTESIAN_POINT('Ctrl Pts',(-4.26268519101727,-1.06847604194793,
5.56023868567198));
#40011=CARTESIAN_POINT('Ctrl Pts',(-4.15967441440321,-0.794772684000964,
5.61619707054585));
#40012=CARTESIAN_POINT('Ctrl Pts',(-4.10683439689708,-0.636309800095286,
5.64192240980302));
#40013=CARTESIAN_POINT('Ctrl Pts',(-4.0449049345007,-0.319434907277203,
5.68296884230057));
#40014=CARTESIAN_POINT('Ctrl Pts',(-4.02497298992508,-0.158333333333354,
5.69777784326964));
#40015=CARTESIAN_POINT('Ctrl Pts',(-4.03289635293786,0.158333333333357,
5.71961533094095));
#40016=CARTESIAN_POINT('Ctrl Pts',(-4.06054091444927,0.319434907277212,
5.72594583243566));
#40017=CARTESIAN_POINT('Ctrl Pts',(-4.13903897138624,0.636309800095295,
5.73080253558442));
#40018=CARTESIAN_POINT('Ctrl Pts',(-4.20050281014632,0.794772684000951,
5.72935414887066));
#40019=CARTESIAN_POINT('Ctrl Pts',(-4.31925042598414,1.06847604194747,5.71696518890184));
#40020=CARTESIAN_POINT('Ctrl Pts',(-4.37711181961818,1.1851427086163,5.70867492566776));
#40021=CARTESIAN_POINT('Ctrl Pts',(-4.44143316402236,1.30000000000662,5.69745712091394));
#40022=CARTESIAN_POINT('Ctrl Pts',(-4.38954914692239,-1.30000000000818,
5.48121690616089));
#40023=CARTESIAN_POINT('Ctrl Pts',(-4.33633023486684,-1.18514270861742,
5.50842819923269));
#40024=CARTESIAN_POINT('Ctrl Pts',(-4.28857783106944,-1.06847604194813,
5.53376290222766));
#40025=CARTESIAN_POINT('Ctrl Pts',(-4.19088895311055,-0.794772684001115,
5.58795583584731));
#40026=CARTESIAN_POINT('Ctrl Pts',(-4.13896358606072,-0.636309800095409,
5.6174474536141));
#40027=CARTESIAN_POINT('Ctrl Pts',(-4.07860037207344,-0.319434907277266,
5.66128044194837));
#40028=CARTESIAN_POINT('Ctrl Pts',(-4.05796819861899,-0.158333333333385,
5.67873539850413));
#40029=CARTESIAN_POINT('Ctrl Pts',(-4.06601837690713,0.158333333333388,
5.70088706633193));
#40030=CARTESIAN_POINT('Ctrl Pts',(-4.09423437574826,0.319434907277274,
5.70444375388613));
#40031=CARTESIAN_POINT('Ctrl Pts',(-4.17194515055815,0.636309800095419,
5.70805426417284));
#40032=CARTESIAN_POINT('Ctrl Pts',(-4.2339664774439,0.794772684001107,5.70565218510332));
#40033=CARTESIAN_POINT('Ctrl Pts',(-4.34764865863211,1.06847604194768,5.6953488246972));
#40034=CARTESIAN_POINT('Ctrl Pts',(-4.40217130686692,1.18514270861653,5.68872907315249));
#40035=CARTESIAN_POINT('Ctrl Pts',(-4.46200779943961,1.30000000000688,5.67994951300579));
#40036=CARTESIAN_POINT('Ctrl Pts',(-4.41112472456861,-1.30000000000823,
5.45954571059543));
#40037=CARTESIAN_POINT('Ctrl Pts',(-4.36286900737893,-1.18514270861747,
5.48375018514035));
#40038=CARTESIAN_POINT('Ctrl Pts',(-4.31878817648165,-1.06847604194818,
5.50696965207528));
#40039=CARTESIAN_POINT('Ctrl Pts',(-4.22659746128865,-0.794772684001152,
5.55833570110362));
#40040=CARTESIAN_POINT('Ctrl Pts',(-4.17384714641575,-0.636309800095435,
5.58858728418216));
#40041=CARTESIAN_POINT('Ctrl Pts',(-4.114288708503,-0.319434907277277,5.63364822804344));
#40042=CARTESIAN_POINT('Ctrl Pts',(-4.09283227419875,-0.158333333333391,
5.65372521525302));
#40043=CARTESIAN_POINT('Ctrl Pts',(-4.10136977087594,0.158333333333394,
5.67693826559168));
#40044=CARTESIAN_POINT('Ctrl Pts',(-4.131191075948,0.319434907277288,5.67959205301889));
#40045=CARTESIAN_POINT('Ctrl Pts',(-4.20849140641991,0.636309800095445,
5.68279678218203));
#40046=CARTESIAN_POINT('Ctrl Pts',(-4.27071111802872,0.794772684001137,
5.67832433183507));
#40047=CARTESIAN_POINT('Ctrl Pts',(-4.37903721967095,1.06847604194772,5.67089337405542));
#40048=CARTESIAN_POINT('Ctrl Pts',(-4.43006377787937,1.18514270861658,5.66659176928105));
#40049=CARTESIAN_POINT('Ctrl Pts',(-4.48522653877245,1.30000000000693,5.66120514601103));
#40050=CARTESIAN_POINT('Ctrl Pts',(-4.42782422204453,-1.30000000000832,
5.4412447319148));
#40051=CARTESIAN_POINT('Ctrl Pts',(-4.38266614769295,-1.18514270861755,
5.46153999931372));
#40052=CARTESIAN_POINT('Ctrl Pts',(-4.34101741910968,-1.06847604194825,
5.48219429268874));
#40053=CARTESIAN_POINT('Ctrl Pts',(-4.25290781505086,-0.794772684001202,
5.53073926408937));
#40054=CARTESIAN_POINT('Ctrl Pts',(-4.20075795765716,-0.636309800095476,
5.56376099319447));
#40055=CARTESIAN_POINT('Ctrl Pts',(-4.1423804942734,-0.319434907277298,
5.61069120909608));
#40056=CARTESIAN_POINT('Ctrl Pts',(-4.12030187944122,-0.158333333333401,
5.63290628434515));
#40057=CARTESIAN_POINT('Ctrl Pts',(-4.12921724313909,0.158333333333404,
5.6568772790265));
#40058=CARTESIAN_POINT('Ctrl Pts',(-4.16008957882327,0.319434907277307,
5.65831943327165));
#40059=CARTESIAN_POINT('Ctrl Pts',(-4.23687477385054,0.636309800095485,
5.66085552466139));
#40060=CARTESIAN_POINT('Ctrl Pts',(-4.29913716795114,0.794772684001187,
5.65460753171467));
#40061=CARTESIAN_POINT('Ctrl Pts',(-4.40315349469226,1.06847604194779,5.64944089018014));
#40062=CARTESIAN_POINT('Ctrl Pts',(-4.45140790386964,1.18514270861666,5.64702901501569));
#40063=CARTESIAN_POINT('Ctrl Pts',(-4.50289190856247,1.30000000000702,5.64444171236415));
#40064=CARTESIAN_POINT('Ctrl Pts',(-4.44012243042177,-1.30000000000835,
5.42715703615215));
#40065=CARTESIAN_POINT('Ctrl Pts',(-4.39791645627916,-1.18514270861758,
5.44560341256595));
#40066=CARTESIAN_POINT('Ctrl Pts',(-4.3584859041896,-1.06847604194827,5.4650139957485));
#40067=CARTESIAN_POINT('Ctrl Pts',(-4.2738052209727,-0.79477268400122,5.51208383649821));
#40068=CARTESIAN_POINT('Ctrl Pts',(-4.22154640570247,-0.636309800095492,
5.54625319252759));
#40069=CARTESIAN_POINT('Ctrl Pts',(-4.16359851535671,-0.319434907277307,
5.59376442404522));
#40070=CARTESIAN_POINT('Ctrl Pts',(-4.14058799071849,-0.158333333333405,
5.61669015058547));
#40071=CARTESIAN_POINT('Ctrl Pts',(-4.14960969582907,0.158333333333408,
5.64090260438518));
#40072=CARTESIAN_POINT('Ctrl Pts',(-4.18143139561612,0.319434907277314,
5.64174134575178));
#40073=CARTESIAN_POINT('Ctrl Pts',(-4.25818468406121,0.6363098000955,5.64446165427731));
#40074=CARTESIAN_POINT('Ctrl Pts',(-4.32107128058956,0.794772684001208,
5.63802446775025));
#40075=CARTESIAN_POINT('Ctrl Pts',(-4.42196963571851,1.06847604194782,5.6347801551929));
#40076=CARTESIAN_POINT('Ctrl Pts',(-4.46806959498563,1.18514270861669,5.6336423111258));
#40077=CARTESIAN_POINT('Ctrl Pts',(-4.51659435423661,1.30000000000705,5.63277096568406));
#40078=CARTESIAN_POINT('Ctrl Pts',(-4.454645622087,-1.30000000000857,5.41105919281565));
#40079=CARTESIAN_POINT('Ctrl Pts',(-4.41514556095973,-1.18514270861778,
5.42611614972381));
#40080=CARTESIAN_POINT('Ctrl Pts',(-4.37779927083417,-1.06847604194846,
5.44322501577103));
#40081=CARTESIAN_POINT('Ctrl Pts',(-4.2964975114198,-0.794772684001356,
5.48749023955076));
#40082=CARTESIAN_POINT('Ctrl Pts',(-4.24439282465342,-0.636309800095601,
5.52336511487347));
#40083=CARTESIAN_POINT('Ctrl Pts',(-4.18738209157449,-0.319434907277362,
5.57228049978856));
#40084=CARTESIAN_POINT('Ctrl Pts',(-4.16403365829309,-0.158333333333432,
5.59739153873146));
#40085=CARTESIAN_POINT('Ctrl Pts',(-4.17349511325057,0.158333333333435,
5.62243620194746));
#40086=CARTESIAN_POINT('Ctrl Pts',(-4.20630986171008,0.319434907277368,
5.62237239062541));
#40087=CARTESIAN_POINT('Ctrl Pts',(-4.28258299737053,0.636309800095608,
5.62446595789768));
#40088=CARTESIAN_POINT('Ctrl Pts',(-4.34520753220417,0.794772684001345,
5.61593402713908));
#40089=CARTESIAN_POINT('Ctrl Pts',(-4.44251263710464,1.068476041948,5.61501368822388));
#40090=CARTESIAN_POINT('Ctrl Pts',(-4.48636413798361,1.18514270861689,5.61586237792014));
#40091=CARTESIAN_POINT('Ctrl Pts',(-4.53194736533916,1.30000000000727,5.61795813792712));
#40092=CARTESIAN_POINT('Ctrl Pts',(-4.47094525801616,-1.30000000000866,
5.39216627151158));
#40093=CARTESIAN_POINT('Ctrl Pts',(-4.43513973486294,-1.18514270861787,
5.40435163061268));
#40094=CARTESIAN_POINT('Ctrl Pts',(-4.40057535245081,-1.06847604194854,
5.41950137458678));
#40095=CARTESIAN_POINT('Ctrl Pts',(-4.3235919979,-0.794772684001415,5.4613486359422));
#40096=CARTESIAN_POINT('Ctrl Pts',(-4.27136350000773,-0.636309800095647,
5.4987471794917));
#40097=CARTESIAN_POINT('Ctrl Pts',(-4.21498556763763,-0.319434907277384,
5.5485128165621));
#40098=CARTESIAN_POINT('Ctrl Pts',(-4.19074131770077,-0.158333333333444,
5.57519316288732));
#40099=CARTESIAN_POINT('Ctrl Pts',(-4.20011017939256,0.158333333333446,
5.60009571229502));
#40100=CARTESIAN_POINT('Ctrl Pts',(-4.23345365297838,0.319434907277392,
5.59784807793541));
#40101=CARTESIAN_POINT('Ctrl Pts',(-4.30946451531293,0.636309800095655,
5.59976416600554));
#40102=CARTESIAN_POINT('Ctrl Pts',(-4.37321473773036,0.794772684001403,
5.5915238680523));
#40103=CARTESIAN_POINT('Ctrl Pts',(-4.46666130211471,1.06847604194808,5.59371528518928));
#40104=CARTESIAN_POINT('Ctrl Pts',(-4.50780006940397,1.18514270861698,5.59655722660272));
#40105=CARTESIAN_POINT('Ctrl Pts',(-4.54962804879656,1.30000000000736,5.60129252615098));
#40106=CARTESIAN_POINT('Ctrl Pts',(-4.48493632988914,-1.30000000000885,
5.3752561709007));
#40107=CARTESIAN_POINT('Ctrl Pts',(-4.45163533037209,-1.18514270861804,
5.38375827085221));
#40108=CARTESIAN_POINT('Ctrl Pts',(-4.41904162193305,-1.06847604194869,
5.39643844392018));
#40109=CARTESIAN_POINT('Ctrl Pts',(-4.34537761897406,-0.794772684001532,
5.43538436508636));
#40110=CARTESIAN_POINT('Ctrl Pts',(-4.2936880621305,-0.63630980009574,5.4750722726532));
#40111=CARTESIAN_POINT('Ctrl Pts',(-4.23824685917295,-0.319434907277431,
5.52615416822502));
#40112=CARTESIAN_POINT('Ctrl Pts',(-4.21330023661494,-0.158333333333467,
5.55430405446636));
#40113=CARTESIAN_POINT('Ctrl Pts',(-4.22318318569591,0.15833333333347,5.5801473341821));
#40114=CARTESIAN_POINT('Ctrl Pts',(-4.25796450582175,0.319434907277439,
5.57783932223402));
#40115=CARTESIAN_POINT('Ctrl Pts',(-4.33363484931934,0.636309800095748,
5.57940118940962));
#40116=CARTESIAN_POINT('Ctrl Pts',(-4.39684005390025,0.794772684001519,
5.56856823598866));
#40117=CARTESIAN_POINT('Ctrl Pts',(-4.48678914178438,1.06847604194824,5.57325856522636));
#40118=CARTESIAN_POINT('Ctrl Pts',(-4.52578314351235,1.18514270861715,5.5782710410378));
#40119=CARTESIAN_POINT('Ctrl Pts',(-4.56483551976503,1.30000000000755,5.58626572292747));
#40120=CARTESIAN_POINT('Ctrl Pts',(-4.498861949539,-1.30000000000899,5.35823247550946));
#40121=CARTESIAN_POINT('Ctrl Pts',(-4.46872355137842,-1.18514270861816,
5.36413287876654));
#40122=CARTESIAN_POINT('Ctrl Pts',(-4.43844643707928,-1.0684760419488,5.37491459924435));
#40123=CARTESIAN_POINT('Ctrl Pts',(-4.36817978410308,-0.794772684001614,
5.41109934970751));
#40124=CARTESIAN_POINT('Ctrl Pts',(-4.31565423214811,-0.636309800095808,
5.45083387039926));
#40125=CARTESIAN_POINT('Ctrl Pts',(-4.26086656492057,-0.319434907277466,
5.50278614645565));
#40126=CARTESIAN_POINT('Ctrl Pts',(-4.23599756233597,-0.158333333333484,
5.53373892058108));
#40127=CARTESIAN_POINT('Ctrl Pts',(-4.24621739610398,0.158333333333486,
5.56016007790502));
#40128=CARTESIAN_POINT('Ctrl Pts',(-4.28138354171649,0.319434907277472,
5.55584724853662));
#40129=CARTESIAN_POINT('Ctrl Pts',(-4.35683080108103,0.636309800095816,
5.55726731331466));
#40130=CARTESIAN_POINT('Ctrl Pts',(-4.42087067157835,0.794772684001605,
5.54641067168685));
#40131=CARTESIAN_POINT('Ctrl Pts',(-4.50748336180335,1.06847604194835,5.55387732613153));
#40132=CARTESIAN_POINT('Ctrl Pts',(-4.54415828630143,1.18514270861728,5.56072168072238));
#40133=CARTESIAN_POINT('Ctrl Pts',(-4.58001671101529,1.30000000000769,5.57117835186175));
#40134=CARTESIAN_POINT('Ctrl Pts',(-4.50921253636227,-1.30000000000911,
5.34679556586098));
#40135=CARTESIAN_POINT('Ctrl Pts',(-4.48076316876939,-1.18514270861827,
5.349916494865));
#40136=CARTESIAN_POINT('Ctrl Pts',(-4.45182716951738,-1.0684760419489,5.35883438517782));
#40137=CARTESIAN_POINT('Ctrl Pts',(-4.38385500613636,-0.794772684001686,
5.39282863611934));
#40138=CARTESIAN_POINT('Ctrl Pts',(-4.33190247816714,-0.636309800095865,
5.43450303805174));
#40139=CARTESIAN_POINT('Ctrl Pts',(-4.27758201208292,-0.319434907277494,
5.48702683718887));
#40140=CARTESIAN_POINT('Ctrl Pts',(-4.2518822176191,-0.158333333333498,
5.51844686361384));
#40141=CARTESIAN_POINT('Ctrl Pts',(-4.26207950271066,0.158333333333501,
5.5448406589144));
#40142=CARTESIAN_POINT('Ctrl Pts',(-4.2978562169275,0.319434907277501,5.53972878797136));
#40143=CARTESIAN_POINT('Ctrl Pts',(-4.37319299404238,0.636309800095873,
5.5411416915894));
#40144=CARTESIAN_POINT('Ctrl Pts',(-4.43766183316473,0.794772684001676,
5.52993599454729));
#40145=CARTESIAN_POINT('Ctrl Pts',(-4.52197796054513,1.06847604194845,5.53953275053415));
#40146=CARTESIAN_POINT('Ctrl Pts',(-4.55708058779137,1.18514270861738,5.54783679540291));
#40147=CARTESIAN_POINT('Ctrl Pts',(-4.59078851496094,1.30000000000781,5.56029080506853));
#40148=CARTESIAN_POINT('Ctrl Pts',(-4.52241367989135,-1.30000000000923,
5.32864709204046));
#40149=CARTESIAN_POINT('Ctrl Pts',(-4.49688183956528,-1.18514270861838,
5.32880335169503));
#40150=CARTESIAN_POINT('Ctrl Pts',(-4.47013069643415,-1.068476041949,5.33562922502868));
#40151=CARTESIAN_POINT('Ctrl Pts',(-4.40551337085382,-0.79477268400176,
5.36680649979061));
#40152=CARTESIAN_POINT('Ctrl Pts',(-4.35319518859154,-0.636309800095925,
5.4092594635518));
#40153=CARTESIAN_POINT('Ctrl Pts',(-4.29965614971638,-0.319434907277525,
5.46280526156545));
#40154=CARTESIAN_POINT('Ctrl Pts',(-4.27369098735892,-0.158333333333513,
5.49637428780528));
#40155=CARTESIAN_POINT('Ctrl Pts',(-4.28457445362594,0.158333333333516,
5.52393599581938));
#40156=CARTESIAN_POINT('Ctrl Pts',(-4.32174434070853,0.319434907277532,
5.51863165635827));
#40157=CARTESIAN_POINT('Ctrl Pts',(-4.39679783638627,0.636309800095934,
5.51979515593311));
#40158=CARTESIAN_POINT('Ctrl Pts',(-4.46077305529313,0.794772684001752,
5.50620273685446));
#40159=CARTESIAN_POINT('Ctrl Pts',(-4.54163194195897,1.06847604194855,5.51835365242479));
#40160=CARTESIAN_POINT('Ctrl Pts',(-4.57460044398954,1.18514270861749,5.5288139654911));
#40161=CARTESIAN_POINT('Ctrl Pts',(-4.6055366321297,1.30000000000793,5.54447491050905));
#40162=CARTESIAN_POINT('Ctrl Pts',(-4.53447732780698,-1.30000000000958,
5.31438497829742));
#40163=CARTESIAN_POINT('Ctrl Pts',(-4.5109825104172,-1.1851427086187,5.31125524905197));
#40164=CARTESIAN_POINT('Ctrl Pts',(-4.48584115885595,-1.06847604194929,
5.31586434062888));
#40165=CARTESIAN_POINT('Ctrl Pts',(-4.42395578391596,-0.794772684001975,
5.3443904884623));
#40166=CARTESIAN_POINT('Ctrl Pts',(-4.3723175462256,-0.636309800096095,
5.3891184329957));
#40167=CARTESIAN_POINT('Ctrl Pts',(-4.3192080190876,-0.319434907277609,
5.44310463691538));
#40168=CARTESIAN_POINT('Ctrl Pts',(-4.29212052481273,-0.158333333333556,
5.47701836007896));
#40169=CARTESIAN_POINT('Ctrl Pts',(-4.30275876461167,0.158333333333558,
5.50415463885691));
#40170=CARTESIAN_POINT('Ctrl Pts',(-4.34035579478986,0.319434907277619,
5.4973432969903));
#40171=CARTESIAN_POINT('Ctrl Pts',(-4.41539681098799,0.636309800096105,
5.49870078579237));
#40172=CARTESIAN_POINT('Ctrl Pts',(-4.48040915743014,0.794772684001963,
5.48561753045718));
#40173=CARTESIAN_POINT('Ctrl Pts',(-4.55881635333106,1.06847604194883,5.50084039405422));
#40174=CARTESIAN_POINT('Ctrl Pts',(-4.58998346201326,1.18514270861781,5.51318899988961));
#40175=CARTESIAN_POINT('Ctrl Pts',(-4.61837810954473,1.30000000000827,5.53129679797183));
#40176=CARTESIAN_POINT('Ctrl Pts',(-4.54622410918883,-1.30000000000978,
5.29959293032457));
#40177=CARTESIAN_POINT('Ctrl Pts',(-4.52519371057589,-1.18514270861888,
5.2938693065141));
#40178=CARTESIAN_POINT('Ctrl Pts',(-4.50184469080349,-1.06847604194945,
5.29656112542672));
#40179=CARTESIAN_POINT('Ctrl Pts',(-4.44254730545769,-0.794772684002097,
5.32222112180498));
#40180=CARTESIAN_POINT('Ctrl Pts',(-4.39012972240138,-0.636309800096193,
5.36688731062942));
#40181=CARTESIAN_POINT('Ctrl Pts',(-4.33751850654955,-0.319434907277658,
5.4214535408028));
#40182=CARTESIAN_POINT('Ctrl Pts',(-4.31045165556893,-0.15833333333358,
5.45756077992719));
#40183=CARTESIAN_POINT('Ctrl Pts',(-4.3216903872547,0.158333333333582,5.48568594651191));
#40184=CARTESIAN_POINT('Ctrl Pts',(-4.36028283544304,0.319434907277667,
5.47837482130748));
#40185=CARTESIAN_POINT('Ctrl Pts',(-4.43520221411006,0.636309800096202,
5.47973085897586));
#40186=CARTESIAN_POINT('Ctrl Pts',(-4.50017575770871,0.794772684002084,
5.46528736391715));
#40187=CARTESIAN_POINT('Ctrl Pts',(-4.57575016523733,1.068476041949,5.48291347614234));
#40188=CARTESIAN_POINT('Ctrl Pts',(-4.60508669366304,1.18514270861799,5.49709595582559));
#40189=CARTESIAN_POINT('Ctrl Pts',(-4.63104638980275,1.30000000000848,5.51783122432156));
#40190=CARTESIAN_POINT('Ctrl Pts',(-4.55380108281785,-1.30000000000987,
5.28935232644525));
#40191=CARTESIAN_POINT('Ctrl Pts',(-4.53424726420921,-1.18514270861897,
5.28165515201659));
#40192=CARTESIAN_POINT('Ctrl Pts',(-4.51202417591417,-1.06847604194953,
5.28297086445777));
#40193=CARTESIAN_POINT('Ctrl Pts',(-4.45451784927862,-0.794772684002154,
5.30683199509513));
#40194=CARTESIAN_POINT('Ctrl Pts',(-4.40211975238928,-0.636309800096239,
5.35229014717835));
#40195=CARTESIAN_POINT('Ctrl Pts',(-4.34991373095064,-0.319434907277682,
5.4073364560695));
#40196=CARTESIAN_POINT('Ctrl Pts',(-4.32259149247327,-0.158333333333591,
5.44446771120178));
#40197=CARTESIAN_POINT('Ctrl Pts',(-4.33397838104054,0.158333333333594,
5.47282131878555));
#40198=CARTESIAN_POINT('Ctrl Pts',(-4.37298997785036,0.31943490727769,5.46475274151342));
#40199=CARTESIAN_POINT('Ctrl Pts',(-4.44777416228423,0.636309800096248,
5.46601636464469));
#40200=CARTESIAN_POINT('Ctrl Pts',(-4.51290991151956,0.794772684002143,
5.45099755336283));
#40201=CARTESIAN_POINT('Ctrl Pts',(-4.58676884931904,1.06847604194907,5.47051963942771));
#40202=CARTESIAN_POINT('Ctrl Pts',(-4.61496684428607,1.18514270861808,5.48606125940474));
#40203=CARTESIAN_POINT('Ctrl Pts',(-4.63939203678979,1.30000000000857,5.50869411166581));
#40204=CARTESIAN_POINT('Ctrl Pts',(-4.55954363766313,-1.30000000000996,
5.28177408463877));
#40205=CARTESIAN_POINT('Ctrl Pts',(-4.54105222045902,-1.18514270861904,
5.27252120535695));
#40206=CARTESIAN_POINT('Ctrl Pts',(-4.51964064255725,-1.0684760419496,5.27275048042195));
#40207=CARTESIAN_POINT('Ctrl Pts',(-4.46342945884563,-0.794772684002204,
5.29518582512782));
#40208=CARTESIAN_POINT('Ctrl Pts',(-4.41102636495706,-0.636309800096279,
5.34121416803767));
#40209=CARTESIAN_POINT('Ctrl Pts',(-4.35917783714701,-0.319434907277702,
5.39671080243483));
#40210=CARTESIAN_POINT('Ctrl Pts',(-4.33181650747883,-0.158333333333601,
5.4348563220188));
#40211=CARTESIAN_POINT('Ctrl Pts',(-4.34330364603402,0.158333333333604,
5.46336204431361));
#40212=CARTESIAN_POINT('Ctrl Pts',(-4.38248057779019,0.31943490727771,5.4544820666224));
#40213=CARTESIAN_POINT('Ctrl Pts',(-4.45705852316959,0.636309800096288,
5.45550183824744));
#40214=CARTESIAN_POINT('Ctrl Pts',(-4.52224796629623,0.794772684002193,
5.43993533592643));
#40215=CARTESIAN_POINT('Ctrl Pts',(-4.59484958762752,1.06847604194914,5.46092555646331));
#40216=CARTESIAN_POINT('Ctrl Pts',(-4.62223636980904,1.18514270861815,5.47755649337426));
#40217=CARTESIAN_POINT('Ctrl Pts',(-4.64558338245264,1.30000000000865,5.50173247848997));
#40218=CARTESIAN_POINT('Ctrl Pts',(-4.56528629909216,-1.30000000001002,
5.27419824733449));
#40219=CARTESIAN_POINT('Ctrl Pts',(-4.54793752677531,-1.1851427086191,5.26352024146501));
#40220=CARTESIAN_POINT('Ctrl Pts',(-4.52738073179939,-1.06847604194965,
5.26273417553866));
#40221=CARTESIAN_POINT('Ctrl Pts',(-4.47247924892776,-0.794772684002245,
5.28377056614099));
#40222=CARTESIAN_POINT('Ctrl Pts',(-4.41992575934956,-0.636309800096313,
5.33013966639362));
#40223=CARTESIAN_POINT('Ctrl Pts',(-4.36837877093283,-0.31943490727772,
5.38599536878684));
#40224=CARTESIAN_POINT('Ctrl Pts',(-4.34097756808678,-0.15833333333361,
5.42514489833329));
#40225=CARTESIAN_POINT('Ctrl Pts',(-4.35260577087264,0.158333333333612,
5.45386967431965));
#40226=CARTESIAN_POINT('Ctrl Pts',(-4.39203663865104,0.319434907277726,
5.44433054874481));
#40227=CARTESIAN_POINT('Ctrl Pts',(-4.46645168939803,0.636309800096322,
5.44518118634463));
#40228=CARTESIAN_POINT('Ctrl Pts',(-4.53168185947985,0.794772684002236,
5.42904743639257));
#40229=CARTESIAN_POINT('Ctrl Pts',(-4.60300086052549,1.0684760419492,5.45146138928091));
#40230=CARTESIAN_POINT('Ctrl Pts',(-4.62955813691869,1.18514270861822,5.46914905507073));
#40231=CARTESIAN_POINT('Ctrl Pts',(-4.65180133678155,1.30000000000872,5.49482221696372));
#40232=CARTESIAN_POINT('Ctrl Pts',(-4.56948242172079,-1.30000000001006,
5.26835641752427));
#40233=CARTESIAN_POINT('Ctrl Pts',(-4.55288253832511,-1.18514270861914,
5.25645103233099));
#40234=CARTESIAN_POINT('Ctrl Pts',(-4.53291476005948,-1.06847604194968,
5.25482746551733));
#40235=CARTESIAN_POINT('Ctrl Pts',(-4.47900468683155,-0.794772684002266,
5.27482975871175));
#40236=CARTESIAN_POINT('Ctrl Pts',(-4.42662566433208,-0.636309800096331,
5.3218843316876));
#40237=CARTESIAN_POINT('Ctrl Pts',(-4.37532764569018,-0.319434907277728,
5.37803351666651));
#40238=CARTESIAN_POINT('Ctrl Pts',(-4.34766886857733,-0.158333333333614,
5.4175747831348));
#40239=CARTESIAN_POINT('Ctrl Pts',(-4.3594022483002,0.158333333333617,5.4464640643126));
#40240=CARTESIAN_POINT('Ctrl Pts',(-4.39916950767834,0.319434907277735,
5.43666623015078));
#40241=CARTESIAN_POINT('Ctrl Pts',(-4.47360351911369,0.636309800096339,
5.43762258648556));
#40242=CARTESIAN_POINT('Ctrl Pts',(-4.53901285539156,0.794772684002258,
5.42131440253097));
#40243=CARTESIAN_POINT('Ctrl Pts',(-4.60934782008004,1.06847604194923,5.44475704572301));
#40244=CARTESIAN_POINT('Ctrl Pts',(-4.63522574210525,1.18514270861825,5.46313998662896));
#40245=CARTESIAN_POINT('Ctrl Pts',(-4.65653618610901,1.30000000000876,5.48975841683847));
#40246=CARTESIAN_POINT('Ctrl Pts',(-4.57226309969796,-1.30000000001008,
5.26443910125368));
#40247=CARTESIAN_POINT('Ctrl Pts',(-4.55614439737282,-1.18514270861916,
5.25168907646359));
#40248=CARTESIAN_POINT('Ctrl Pts',(-4.53655907295875,-1.0684760419497,5.24949230992485));
#40249=CARTESIAN_POINT('Ctrl Pts',(-4.48330446501139,-0.794772684002281,
5.26879747749121));
#40250=CARTESIAN_POINT('Ctrl Pts',(-4.4310764076616,-0.636309800096343,
5.31636164782972));
#40251=CARTESIAN_POINT('Ctrl Pts',(-4.37994355381527,-0.319434907277734,
5.37270246234844));
#40252=CARTESIAN_POINT('Ctrl Pts',(-4.35208463527993,-0.158333333333617,
5.41245690758916));
#40253=CARTESIAN_POINT('Ctrl Pts',(-4.36388315554926,0.158333333333619,
5.44144657099326));
#40254=CARTESIAN_POINT('Ctrl Pts',(-4.40388525801494,0.319434907277741,
5.43149382375963));
#40255=CARTESIAN_POINT('Ctrl Pts',(-4.47834879306739,0.63630980009635,5.4325488102522));
#40256=CARTESIAN_POINT('Ctrl Pts',(-4.54389890576145,0.794772684002272,
5.41616089186566));
#40257=CARTESIAN_POINT('Ctrl Pts',(-4.61358662515068,1.06847604194925,5.44030332760959));
#40258=CARTESIAN_POINT('Ctrl Pts',(-4.63901156673434,1.18514270861827,5.45914904729804));
#40259=CARTESIAN_POINT('Ctrl Pts',(-4.65969621836226,1.30000000000878,5.48639012080671));
#40260=CARTESIAN_POINT('Ctrl Pts',(-4.5741188519777,-1.30000000001009,5.26183096309819));
#40261=CARTESIAN_POINT('Ctrl Pts',(-4.55832262344367,-1.18514270861917,
5.24852040473667));
#40262=CARTESIAN_POINT('Ctrl Pts',(-4.53899243564442,-1.06847604194971,
5.24594177814312));
#40263=CARTESIAN_POINT('Ctrl Pts',(-4.48617168196922,-0.794772684002287,
5.26477754415892));
#40264=CARTESIAN_POINT('Ctrl Pts',(-4.434033615713,-0.636309800096347,5.31266555574856));
#40265=CARTESIAN_POINT('Ctrl Pts',(-4.38300947242625,-0.319434907277736,
5.36913184462045));
#40266=CARTESIAN_POINT('Ctrl Pts',(-4.35502611025119,-0.158333333333618,
5.40904168442021));
#40267=CARTESIAN_POINT('Ctrl Pts',(-4.36686780005815,0.15833333333362,5.43809739240082));
#40268=CARTESIAN_POINT('Ctrl Pts',(-4.40701985920357,0.319434907277743,
5.42803103189341));
#40269=CARTESIAN_POINT('Ctrl Pts',(-4.4814985819506,0.636309800096354,5.42914449465699));
#40270=CARTESIAN_POINT('Ctrl Pts',(-4.54713803730562,0.794772684002278,
5.41269591781254));
#40271=CARTESIAN_POINT('Ctrl Pts',(-4.61639854019045,1.06847604194926,5.43731193015391));
#40272=CARTESIAN_POINT('Ctrl Pts',(-4.64152561010396,1.18514270861828,5.45647294845647));
#40273=CARTESIAN_POINT('Ctrl Pts',(-4.66179944458639,1.30000000000879,5.48413962543206));
#40274=CARTESIAN_POINT('Ctrl Pts',(-4.57644778804015,-1.30000000001011,
5.25858548016582));
#40275=CARTESIAN_POINT('Ctrl Pts',(-4.56106380680746,-1.18514270861919,
5.24458808378279));
#40276=CARTESIAN_POINT('Ctrl Pts',(-4.54205553892619,-1.06847604194973,
5.24153671058873));
#40277=CARTESIAN_POINT('Ctrl Pts',(-4.48976981033586,-0.794772684002301,
5.25977493139605));
#40278=CARTESIAN_POINT('Ctrl Pts',(-4.43770668269,-0.636309800096359,5.30801150492459));
#40279=CARTESIAN_POINT('Ctrl Pts',(-4.38681366613632,-0.319434907277742,
5.36462748309272));
#40280=CARTESIAN_POINT('Ctrl Pts',(-4.35870442655486,-0.158333333333621,
5.40477642123583));
#40281=CARTESIAN_POINT('Ctrl Pts',(-4.37059989637588,0.158333333333623,
5.43391337566916));
#40282=CARTESIAN_POINT('Ctrl Pts',(-4.41091950780841,0.319434907277749,
5.42367376371536));
#40283=CARTESIAN_POINT('Ctrl Pts',(-4.48540130712376,0.636309800096367,
5.42483439814329));
#40284=CARTESIAN_POINT('Ctrl Pts',(-4.55113497936443,0.794772684002292,
5.40828071637679));
#40285=CARTESIAN_POINT('Ctrl Pts',(-4.61987196733546,1.06847604194928,5.43350599349821));
#40286=CARTESIAN_POINT('Ctrl Pts',(-4.64463852227565,1.1851427086183,5.45308067856541));
#40287=CARTESIAN_POINT('Ctrl Pts',(-4.6644179370195,1.30000000000881,5.48131096092248));
#40288=CARTESIAN_POINT('Ctrl Pts',(-4.57856707538984,-1.30000000001014,
5.25570001012011));
#40289=CARTESIAN_POINT('Ctrl Pts',(-4.56357914844702,-1.18514270861921,
5.24112202841535));
#40290=CARTESIAN_POINT('Ctrl Pts',(-4.54487067682979,-1.06847604194975,
5.23766032289636));
#40291=CARTESIAN_POINT('Ctrl Pts',(-4.49305516228741,-0.794772684002316,
5.25534391242805));
#40292=CARTESIAN_POINT('Ctrl Pts',(-4.44097465579337,-0.636309800096371,
5.30376671552586));
#40293=CARTESIAN_POINT('Ctrl Pts',(-4.39018970784945,-0.319434907277748,
5.36050340088851));
#40294=CARTESIAN_POINT('Ctrl Pts',(-4.36203206360161,-0.158333333333624,
5.40096741366718));
#40295=CARTESIAN_POINT('Ctrl Pts',(-4.37397750911205,0.158333333333626,
5.43017854321455));
#40296=CARTESIAN_POINT('Ctrl Pts',(-4.41440851291143,0.319434907277755,
5.41972070094411));
#40297=CARTESIAN_POINT('Ctrl Pts',(-4.48885753596838,0.636309800096378,
5.42086554200589));
#40298=CARTESIAN_POINT('Ctrl Pts',(-4.55463482495819,0.794772684002307,
5.4041480378201));
#40299=CARTESIAN_POINT('Ctrl Pts',(-4.62291649322507,1.0684760419493,5.4299478453989));
#40300=CARTESIAN_POINT('Ctrl Pts',(-4.64738044212327,1.18514270861832,5.44993113752389));
#40301=CARTESIAN_POINT('Ctrl Pts',(-4.6667517358118,1.30000000000884,5.47872994104999));
#40302=CARTESIAN_POINT('Ctrl Pts',(-4.57998763858014,-1.30000000001015,
5.25378819732745));
#40303=CARTESIAN_POINT('Ctrl Pts',(-4.56527256586436,-1.18514270861922,
5.23883649972994));
#40304=CARTESIAN_POINT('Ctrl Pts',(-4.54676749277986,-1.06847604194975,
5.23510661561415));
#40305=CARTESIAN_POINT('Ctrl Pts',(-4.49526141298941,-0.79477268400232,
5.25241447120459));
#40306=CARTESIAN_POINT('Ctrl Pts',(-4.44313980655772,-0.636309800096374,
5.30091693696236));
#40307=CARTESIAN_POINT('Ctrl Pts',(-4.39242242526843,-0.31943490727775,
5.35772759265388));
#40308=CARTESIAN_POINT('Ctrl Pts',(-4.36425314259276,-0.158333333333625,
5.39843341442863));
#40309=CARTESIAN_POINT('Ctrl Pts',(-4.37623252610293,0.158333333333627,
5.42769446121915));
#40310=CARTESIAN_POINT('Ctrl Pts',(-4.41672627203826,0.319434907277756,
5.41707285569079));
#40311=CARTESIAN_POINT('Ctrl Pts',(-4.49114189239036,0.636309800096382,
5.41818810853485));
#40312=CARTESIAN_POINT('Ctrl Pts',(-4.55693359486649,0.794772684002312,
5.40133680343764));
#40313=CARTESIAN_POINT('Ctrl Pts',(-4.62491658247708,1.0684760419493,5.42752749481234));
#40314=CARTESIAN_POINT('Ctrl Pts',(-4.64918596137114,1.18514270861833,5.44779498551626));
#40315=CARTESIAN_POINT('Ctrl Pts',(-4.66829740284029,1.30000000000884,5.4769929870886));
#40316=CARTESIAN_POINT('Ctrl Pts',(-4.58069913722931,-1.30000000001015,
5.25283418642123));
#40317=CARTESIAN_POINT('Ctrl Pts',(-4.56612184637048,-1.18514270861922,
5.23769769344442));
#40318=CARTESIAN_POINT('Ctrl Pts',(-4.54771899138673,-1.06847604194975,
5.23383451727211));
#40319=CARTESIAN_POINT('Ctrl Pts',(-4.49636689646632,-0.79477268400232,
5.25095342452577));
#40320=CARTESIAN_POINT('Ctrl Pts',(-4.44422005583735,-0.636309800096374,
5.29948864824094));
#40321=CARTESIAN_POINT('Ctrl Pts',(-4.39353557103492,-0.31943490727775,
5.35633497402513));
#40322=CARTESIAN_POINT('Ctrl Pts',(-4.36536345533378,-0.158333333333625,
5.39716628380688));
#40323=CARTESIAN_POINT('Ctrl Pts',(-4.37735990023755,0.158333333333627,
5.42645234708054));
#40324=CARTESIAN_POINT('Ctrl Pts',(-4.41788351356185,0.319434907277757,
5.41574646919451));
#40325=CARTESIAN_POINT('Ctrl Pts',(-4.4922806760358,0.636309800096382,5.41684401218561));
#40326=CARTESIAN_POINT('Ctrl Pts',(-4.55807708845598,0.794772684002312,
5.39992163775985));
#40327=CARTESIAN_POINT('Ctrl Pts',(-4.62591147829473,1.0684760419493,5.42630893740137));
#40328=CARTESIAN_POINT('Ctrl Pts',(-4.65008471562182,1.18514270861833,5.44672038689974));
#40329=CARTESIAN_POINT('Ctrl Pts',(-4.66906819642635,1.30000000000884,5.47612120162733));
#40330=CARTESIAN_POINT('Ctrl Pts',(-4.58129282510572,-1.30000000001015,
5.25204039785036));
#40331=CARTESIAN_POINT('Ctrl Pts',(-4.5668312977909,-1.18514270861922,5.23675135951165));
#40332=CARTESIAN_POINT('Ctrl Pts',(-4.54851397789909,-1.06847604194976,
5.23277765717448));
#40333=CARTESIAN_POINT('Ctrl Pts',(-4.49728965238091,-0.794772684002322,
5.24973829962777));
#40334=CARTESIAN_POINT('Ctrl Pts',(-4.44511843149432,-0.636309800096376,
5.29829575089737));
#40335=CARTESIAN_POINT('Ctrl Pts',(-4.3944607273938,-0.319434907277751,
5.35517085551875));
#40336=CARTESIAN_POINT('Ctrl Pts',(-4.36628839287869,-0.158333333333625,
5.39611001880934));
#40337=CARTESIAN_POINT('Ctrl Pts',(-4.37829914571928,0.158333333333628,
5.42541700288283));
#40338=CARTESIAN_POINT('Ctrl Pts',(-4.41884657258655,0.319434907277757,
5.41463918881924));
#40339=CARTESIAN_POINT('Ctrl Pts',(-4.49322718206872,0.636309800096384,
5.41572002028131));
#40340=CARTESIAN_POINT('Ctrl Pts',(-4.55902592254007,0.794772684002315,
5.39873574736935));
#40341=CARTESIAN_POINT('Ctrl Pts',(-4.62673696750234,1.0684760419493,5.42528763006261));
#40342=CARTESIAN_POINT('Ctrl Pts',(-4.65083083054437,1.18514270861833,5.44582024270707));
#40343=CARTESIAN_POINT('Ctrl Pts',(-4.66970895420543,1.30000000000885,5.47539214182216));
#40344=CARTESIAN_POINT('Ctrl Pts',(-4.58170873549506,-1.30000000001015,
5.25148528385598));
#40345=CARTESIAN_POINT('Ctrl Pts',(-4.56732852626551,-1.18514270861922,
5.23608990939209));
#40346=CARTESIAN_POINT('Ctrl Pts',(-4.54907116358769,-1.06847604194975,
5.23203897466044));
#40347=CARTESIAN_POINT('Ctrl Pts',(-4.4979360033423,-0.794772684002322,
5.24888843027225));
#40348=CARTESIAN_POINT('Ctrl Pts',(-4.44574659464001,-0.636309800096376,
5.2974597341343));
#40349=CARTESIAN_POINT('Ctrl Pts',(-4.39510719845474,-0.319434907277751,
5.35435430888612));
#40350=CARTESIAN_POINT('Ctrl Pts',(-4.36693505035454,-0.158333333333625,
5.39536947651554));
#40351=CARTESIAN_POINT('Ctrl Pts',(-4.37895582240997,0.158333333333628,
5.42469108545479));
#40352=CARTESIAN_POINT('Ctrl Pts',(-4.41951997902849,0.319434907277757,
5.41386300497789));
#40353=CARTESIAN_POINT('Ctrl Pts',(-4.49388864042137,0.636309800096383,
5.41493151960541));
#40354=CARTESIAN_POINT('Ctrl Pts',(-4.55968810386129,0.794772684002314,
5.39790242646855));
#40355=CARTESIAN_POINT('Ctrl Pts',(-4.62731296829461,1.0684760419493,5.42456973425715));
#40356=CARTESIAN_POINT('Ctrl Pts',(-4.65135158615395,1.18514270861833,5.4451876535451));
#40357=CARTESIAN_POINT('Ctrl Pts',(-4.67015652380732,1.30000000000885,5.47488020270033));
#40358=CARTESIAN_POINT('Ctrl Pts',(-4.5819463590888,-1.30000000001015,5.25116801734297));
#40359=CARTESIAN_POINT('Ctrl Pts',(-4.56761274025231,-1.18514270861922,
5.23571206996149));
#40360=CARTESIAN_POINT('Ctrl Pts',(-4.54938969344282,-1.06847604194976,
5.23161708847656));
#40361=CARTESIAN_POINT('Ctrl Pts',(-4.49830545311051,-0.794772684002324,
5.24840296602242));
#40362=CARTESIAN_POINT('Ctrl Pts',(-4.44610524235701,-0.636309800096377,
5.29698156640216));
#40363=CARTESIAN_POINT('Ctrl Pts',(-4.39547634965677,-0.319434907277752,
5.35388733063218));
#40364=CARTESIAN_POINT('Ctrl Pts',(-4.36730476756172,-0.158333333333626,
5.39494662952139));
#40365=CARTESIAN_POINT('Ctrl Pts',(-4.37933130144857,0.158333333333628,
5.4242766377249));
#40366=CARTESIAN_POINT('Ctrl Pts',(-4.41990464680665,0.319434907277758,
5.41341924517007));
#40367=CARTESIAN_POINT('Ctrl Pts',(-4.49426640787336,0.636309800096385,
5.4144806021061));
#40368=CARTESIAN_POINT('Ctrl Pts',(-4.56006650367745,0.794772684002316,
5.39742624635705));
#40369=CARTESIAN_POINT('Ctrl Pts',(-4.62764213807441,1.06847604194931,5.42415953464588));
#40370=CARTESIAN_POINT('Ctrl Pts',(-4.65164916232392,1.18514270861834,5.44482615986139));
#40371=CARTESIAN_POINT('Ctrl Pts',(-4.67041222261625,1.30000000000885,5.47458756035798));
#40372=CARTESIAN_POINT('Ctrl Pts',(-4.5896776835703,-1.30000000000998,5.24087078904587));
#40373=CARTESIAN_POINT('Ctrl Pts',(-4.57685555325251,-1.18514270861906,
5.22344232441515));
#40374=CARTESIAN_POINT('Ctrl Pts',(-4.55974551517167,-1.06847604194961,
5.21791249958274));
#40375=CARTESIAN_POINT('Ctrl Pts',(-4.51031197962849,-0.794772684002216,
5.2326257362309));
#40376=CARTESIAN_POINT('Ctrl Pts',(-4.45776460123848,-0.636309800096291,
5.28144707494063));
#40377=CARTESIAN_POINT('Ctrl Pts',(-4.40746454541298,-0.319434907277709,
5.33869713889282));
#40378=CARTESIAN_POINT('Ctrl Pts',(-4.37928687943884,-0.158333333333604,
5.38115302849488));
#40379=CARTESIAN_POINT('Ctrl Pts',(-4.39149847991096,0.158333333333606,
5.41075297103868));
#40380=CARTESIAN_POINT('Ctrl Pts',(-4.43239750422643,0.319434907277714,
5.39898567727831));
#40381=CARTESIAN_POINT('Ctrl Pts',(-4.50653337087347,0.636309800096298,
5.39981105663908));
#40382=CARTESIAN_POINT('Ctrl Pts',(-4.57232169147551,0.794772684002208,
5.38188329400092));
#40383=CARTESIAN_POINT('Ctrl Pts',(-4.63829918072036,1.06847604194916,5.41076288483102));
#40384=CARTESIAN_POINT('Ctrl Pts',(-4.66128704727822,1.18514270861817,5.4330242182846));
#40385=CARTESIAN_POINT('Ctrl Pts',(-4.67870357000646,1.30000000000867,5.46504598041558));
#40386=CARTESIAN_POINT('Ctrl Pts',(-4.60062712095472,-1.30000000000845,
5.22482344032791));
#40387=CARTESIAN_POINT('Ctrl Pts',(-4.58971953854938,-1.18514270861767,
5.20400024324085));
#40388=CARTESIAN_POINT('Ctrl Pts',(-4.57409395527427,-1.06847604194836,
5.19610612076081));
#40389=CARTESIAN_POINT('Ctrl Pts',(-4.52709620618016,-0.794772684001287,
5.20773786741273));
#40390=CARTESIAN_POINT('Ctrl Pts',(-4.47476552804312,-0.636309800095545,
5.25800147984835));
#40391=CARTESIAN_POINT('Ctrl Pts',(-4.4251161255172,-0.319434907277333,
5.31597655950532));
#40392=CARTESIAN_POINT('Ctrl Pts',(-4.39653103096014,-0.158333333333419,
5.35985818511565));
#40393=CARTESIAN_POINT('Ctrl Pts',(-4.40909476686169,0.158333333333421,
5.38997142220023));
#40394=CARTESIAN_POINT('Ctrl Pts',(-4.45065571899694,0.319434907277343,
5.37714567020242));
#40395=CARTESIAN_POINT('Ctrl Pts',(-4.52505708475374,0.636309800095555,
5.37858900352638));
#40396=CARTESIAN_POINT('Ctrl Pts',(-4.59201094519908,0.794772684001275,
5.36131287512466));
#40397=CARTESIAN_POINT('Ctrl Pts',(-4.65531542587047,1.06847604194791,5.39282328721827));
#40398=CARTESIAN_POINT('Ctrl Pts',(-4.6763049397076,1.18514270861679,5.41661523283239));
#40399=CARTESIAN_POINT('Ctrl Pts',(-4.6908818033611,1.30000000000715,5.45055943424102));
#40400=CARTESIAN_POINT('Ctrl Pts',(-4.61560427125043,-1.30000000000843,
5.20428584956671));
#40401=CARTESIAN_POINT('Ctrl Pts',(-4.60721582813338,-1.18514270861765,
5.17894198652733));
#40402=CARTESIAN_POINT('Ctrl Pts',(-4.59353793472172,-1.06847604194834,
5.16788666297074));
#40403=CARTESIAN_POINT('Ctrl Pts',(-4.54971957635672,-0.794772684001272,
5.17535603856278));
#40404=CARTESIAN_POINT('Ctrl Pts',(-4.49766388251748,-0.636309800095534,
5.22748590960429));
#40405=CARTESIAN_POINT('Ctrl Pts',(-4.44877749627254,-0.319434907277328,
5.28627334674993));
#40406=CARTESIAN_POINT('Ctrl Pts',(-4.41960624761064,-0.158333333333416,
5.33200674040388));
#40407=CARTESIAN_POINT('Ctrl Pts',(-4.43242015699473,0.158333333333418,
5.36246973164054));
#40408=CARTESIAN_POINT('Ctrl Pts',(-4.47489349638911,0.319434907277335,
5.34829149709891));
#40409=CARTESIAN_POINT('Ctrl Pts',(-4.54888650316088,0.636309800095542,
5.34933031237017));
#40410=CARTESIAN_POINT('Ctrl Pts',(-4.61553439221572,0.794772684001263,
5.32988210434617));
#40411=CARTESIAN_POINT('Ctrl Pts',(-4.6759182053292,1.06847604194789,5.36597580363968));
#40412=CARTESIAN_POINT('Ctrl Pts',(-4.69509996469825,1.18514270861676,5.39322292659584));
#40413=CARTESIAN_POINT('Ctrl Pts',(-4.70732556818005,1.30000000000713,5.4320935474872));
#40414=CARTESIAN_POINT('Ctrl Pts',(-4.62268404883095,-1.30000000000774,
5.19340317858565));
#40415=CARTESIAN_POINT('Ctrl Pts',(-4.61569350574113,-1.18514270861703,
5.16602552974015));
#40416=CARTESIAN_POINT('Ctrl Pts',(-4.60305483470086,-1.06847604194778,
5.15350263191577));
#40417=CARTESIAN_POINT('Ctrl Pts',(-4.56080867077122,-0.794772684000851,
5.15888967928581));
#40418=CARTESIAN_POINT('Ctrl Pts',(-4.50854513869897,-0.636309800095197,
5.2114509203725));
#40419=CARTESIAN_POINT('Ctrl Pts',(-4.45994161137855,-0.319434907277159,
5.2704792232101));
#40420=CARTESIAN_POINT('Ctrl Pts',(-4.43050381798302,-0.158333333333332,
5.31712145281223));
#40421=CARTESIAN_POINT('Ctrl Pts',(-4.44367001134335,0.158333333333335,
5.34809023449043));
#40422=CARTESIAN_POINT('Ctrl Pts',(-4.48691159332261,0.319434907277167,
5.33373581427421));
#40423=CARTESIAN_POINT('Ctrl Pts',(-4.56103497295898,0.636309800095206,
5.33510192542139));
#40424=CARTESIAN_POINT('Ctrl Pts',(-4.62791448441862,0.79477268400084,5.31522003750839));
#40425=CARTESIAN_POINT('Ctrl Pts',(-4.68657619398998,1.06847604194732,5.35312981420995));
#40426=CARTESIAN_POINT('Ctrl Pts',(-4.70457535664068,1.18514270861614,5.38161490460393));
#40427=CARTESIAN_POINT('Ctrl Pts',(-4.71518120149896,1.30000000000644,5.42217534775329));
#40428=CARTESIAN_POINT('Ctrl Pts',(-4.62624077063454,-1.30000000000774,
5.18799189686137));
#40429=CARTESIAN_POINT('Ctrl Pts',(-4.61995220105655,-1.18514270861703,
5.15960337168817));
#40430=CARTESIAN_POINT('Ctrl Pts',(-4.60783501082469,-1.06847604194778,
5.14635039002685));
#40431=CARTESIAN_POINT('Ctrl Pts',(-4.566376597632,-0.794772684000851,5.15069948450678));
#40432=CARTESIAN_POINT('Ctrl Pts',(-4.5139835392274,-0.636309800095197,
5.20343425858748));
#40433=CARTESIAN_POINT('Ctrl Pts',(-4.46556375514821,-0.319434907277159,
5.26264955034744));
#40434=CARTESIAN_POINT('Ctrl Pts',(-4.43611716307415,-0.158333333333332,
5.30994285314818));
#40435=CARTESIAN_POINT('Ctrl Pts',(-4.44941966576161,0.158333333333335,
5.34110298165354));
#40436=CARTESIAN_POINT('Ctrl Pts',(-4.49284772594685,0.319434907277167,
5.32635100323495));
#40437=CARTESIAN_POINT('Ctrl Pts',(-4.56698074650739,0.636309800095206,
5.32779325308506));
#40438=CARTESIAN_POINT('Ctrl Pts',(-4.63406245451013,0.79477268400084,5.30782498057273));
#40439=CARTESIAN_POINT('Ctrl Pts',(-4.69192014515469,1.06847604194732,5.34673782657625));
#40440=CARTESIAN_POINT('Ctrl Pts',(-4.70935397490061,1.18514270861614,5.37588728519524));
#40441=CARTESIAN_POINT('Ctrl Pts',(-4.71917718395088,1.30000000000644,5.41734227326118));
#40442=CARTESIAN_POINT('',(-4.63725024984735,1.2,5.46840821199375));
#40443=CARTESIAN_POINT('Ctrl Pts',(-4.63725024984735,1.2,5.46840821199376));
#40444=CARTESIAN_POINT('Ctrl Pts',(-4.62623288747658,1.21680927464258,5.48695510237328));
#40445=CARTESIAN_POINT('Ctrl Pts',(-4.61595325414295,1.23316098172227,5.50634587166694));
#40446=CARTESIAN_POINT('Ctrl Pts',(-4.59367983320334,1.26666762025062,5.54312911943321));
#40447=CARTESIAN_POINT('Ctrl Pts',(-4.58868040342263,1.27448084893935,5.55224217132525));
#40448=CARTESIAN_POINT('Ctrl Pts',(-4.57136452279491,1.30000000000761,5.5797758180862));
#40449=CARTESIAN_POINT('',(-4.58017335384877,0.653834841338402,5.32263161625288));
#40450=CARTESIAN_POINT('Ctrl Pts',(-4.58017335390807,0.653834841323774,
5.3226316162909));
#40451=CARTESIAN_POINT('Ctrl Pts',(-4.58566039843636,0.710876435607271,
5.33601823521891));
#40452=CARTESIAN_POINT('Ctrl Pts',(-4.59154716380413,0.767442498216031,
5.3505545328843));
#40453=CARTESIAN_POINT('Ctrl Pts',(-4.60348776625804,0.881812809428854,
5.38047657158293));
#40454=CARTESIAN_POINT('Ctrl Pts',(-4.60916965496843,0.939315063510303,
5.39489255928413));
#40455=CARTESIAN_POINT('Ctrl Pts',(-4.61960617994113,1.03703221706045,5.42184408062769));
#40456=CARTESIAN_POINT('Ctrl Pts',(-4.62007222621881,1.04047637892618,5.42298882183644));
#40457=CARTESIAN_POINT('Ctrl Pts',(-4.63064770978488,1.13868342304201,5.45079102623296));
#40458=CARTESIAN_POINT('Ctrl Pts',(-4.63355571084997,1.16612797337853,5.45851413533704));
#40459=CARTESIAN_POINT('Ctrl Pts',(-4.63725024984735,1.2,5.46840821199376));
#40460=CARTESIAN_POINT('',(-4.52544944337377,-0.653834841531101,5.19430627077111));
#40461=CARTESIAN_POINT('Ctrl Pts',(-4.52544944337376,-0.653834841531102,
5.19430627077111));
#40462=CARTESIAN_POINT('Ctrl Pts',(-4.49798587443275,-0.575737631362572,
5.22568933893298));
#40463=CARTESIAN_POINT('Ctrl Pts',(-4.47558879617822,-0.493703172347255,
5.25273934756678));
#40464=CARTESIAN_POINT('Ctrl Pts',(-4.44500736577266,-0.338082431543929,
5.29312978320453));
#40465=CARTESIAN_POINT('Ctrl Pts',(-4.43523489250357,-0.265627281829756,
5.30816486560134));
#40466=CARTESIAN_POINT('Ctrl Pts',(-4.42569301093367,-0.129696671635448,
5.33064595190667));
#40467=CARTESIAN_POINT('Ctrl Pts',(-4.42464816556244,-0.066641443281186,
5.33882442907362));
#40468=CARTESIAN_POINT('Ctrl Pts',(-4.42950987352535,0.0594827545774232,
5.35118240948938));
#40469=CARTESIAN_POINT('Ctrl Pts',(-4.43543101216695,0.122684205165005,
5.35544646033219));
#40470=CARTESIAN_POINT('Ctrl Pts',(-4.4556613000911,0.260063037905712,5.35953858680526));
#40471=CARTESIAN_POINT('Ctrl Pts',(-4.47132565790492,0.333932211455017,
5.35845298339707));
#40472=CARTESIAN_POINT('Ctrl Pts',(-4.51502626842882,0.491503249588507,
5.348104651279));
#40473=CARTESIAN_POINT('Ctrl Pts',(-4.54505774438011,0.574911307367796,
5.33774599738179));
#40474=CARTESIAN_POINT('Ctrl Pts',(-4.58017335385184,0.653834841359911,
5.32263161637234));
#40475=CARTESIAN_POINT('',(-4.55425078118152,-1.2,5.26059291996045));
#40476=CARTESIAN_POINT('Ctrl Pts',(-4.55425078118152,-1.2,5.26059291996045));
#40477=CARTESIAN_POINT('Ctrl Pts',(-4.54944661068513,-1.13516581515213,
5.24931143219995));
#40478=CARTESIAN_POINT('Ctrl Pts',(-4.54291543586199,-1.03784493433457,
5.23409938464372));
#40479=CARTESIAN_POINT('Ctrl Pts',(-4.52921603512606,-0.776832222371542,
5.20276554770155));
#40480=CARTESIAN_POINT('Ctrl Pts',(-4.52760510110744,-0.724975474669047,
5.19917008419827));
#40481=CARTESIAN_POINT('Ctrl Pts',(-4.52544944337376,-0.653834841531101,
5.19430627077111));
#40482=CARTESIAN_POINT('Ctrl Pts',(-4.49074887227402,-1.30000000000891,
5.36814996080924));
#40483=CARTESIAN_POINT('Ctrl Pts',(-4.50169806910935,-1.28307064772788,
5.35016963244304));
#40484=CARTESIAN_POINT('Ctrl Pts',(-4.51244888709795,-1.26620626769394,
5.33200719241798));
#40485=CARTESIAN_POINT('Ctrl Pts',(-4.53220866142032,-1.23557956131176,
5.29981330135354));
#40486=CARTESIAN_POINT('Ctrl Pts',(-4.54172259503861,-1.22080224198256,
5.28426747325981));
#40487=CARTESIAN_POINT('Ctrl Pts',(-4.55425078118152,-1.2,5.26059291996044));
#40488=CARTESIAN_POINT('Origin',(0.,1.25,7.2));
#40489=CARTESIAN_POINT('Origin',(0.,1.2,7.2));
#40490=CARTESIAN_POINT('Origin',(0.,0.92691742076555,7.2));
#40491=CARTESIAN_POINT('Origin',(0.,0.653834841531101,7.2));
#40492=CARTESIAN_POINT('Origin',(0.,0.,7.2));
#40493=CARTESIAN_POINT('Origin',(0.,-0.653834841531101,7.2));
#40494=CARTESIAN_POINT('Origin',(0.,-0.926917420765551,7.2));
#40495=CARTESIAN_POINT('Origin',(0.,-1.2,7.2));
#40496=CARTESIAN_POINT('Origin',(0.,-1.25,7.2));
#40497=CARTESIAN_POINT('Ctrl Pts',(-4.48251875583975,-1.30000000000134,
4.88579874085794));
#40498=CARTESIAN_POINT('Ctrl Pts',(-4.50675280588359,-1.18514270861269,
4.92083760913291));
#40499=CARTESIAN_POINT('Ctrl Pts',(-4.51674956615302,-1.06847604194558,
4.95329826441664));
#40500=CARTESIAN_POINT('Ctrl Pts',(-4.50695309468148,-0.794772684000851,
5.02233268407423));
#40501=CARTESIAN_POINT('Ctrl Pts',(-4.44722735233531,-0.636309800095196,
5.05882272596845));
#40502=CARTESIAN_POINT('Ctrl Pts',(-4.39869447984843,-0.319434907277159,
5.11487935011235));
#40503=CARTESIAN_POINT('Ctrl Pts',(-4.35867257917745,-0.158333333333332,
5.13728168805474));
#40504=CARTESIAN_POINT('Ctrl Pts',(-4.37292795574814,0.158333333333335,
5.16801756977376));
#40505=CARTESIAN_POINT('Ctrl Pts',(-4.42777734501438,0.319434907277167,
5.17777988362547));
#40506=CARTESIAN_POINT('Ctrl Pts',(-4.50418204215396,0.636309800095206,
5.18141973571819));
#40507=CARTESIAN_POINT('Ctrl Pts',(-4.57842941556978,0.79477268400084,5.17777055683287));
#40508=CARTESIAN_POINT('Ctrl Pts',(-4.60940251578666,1.06847604194529,5.14987106382276));
#40509=CARTESIAN_POINT('Ctrl Pts',(-4.60766161389184,1.18514270861212,5.1319982609474));
#40510=CARTESIAN_POINT('Ctrl Pts',(-4.59077270268479,1.30000000000051,5.10832931194267));
#40511=CARTESIAN_POINT('Ctrl Pts',(-4.4699877389614,-1.30000000000134,4.88527001206655));
#40512=CARTESIAN_POINT('Ctrl Pts',(-4.49184486502941,-1.18514270861269,
4.9202749690669));
#40513=CARTESIAN_POINT('Ctrl Pts',(-4.50009761859441,-1.06847604194558,
4.95268677456364));
#40514=CARTESIAN_POINT('Ctrl Pts',(-4.48773430825989,-0.794772684000851,
5.02157383048891));
#40515=CARTESIAN_POINT('Ctrl Pts',(-4.42840755020082,-0.636309800095196,
5.05787895493427));
#40516=CARTESIAN_POINT('Ctrl Pts',(-4.37977441560886,-0.319434907277159,
5.11381935640681));
#40517=CARTESIAN_POINT('Ctrl Pts',(-4.34059295813843,-0.158333333333332,
5.13647657043832));
#40518=CARTESIAN_POINT('Ctrl Pts',(-4.35474635538549,0.158333333333335,
5.16675378497832));
#40519=CARTESIAN_POINT('Ctrl Pts',(-4.40861628637067,0.319434907277167,
5.17565787020395));
#40520=CARTESIAN_POINT('Ctrl Pts',(-4.48498896024595,0.636309800095206,
5.17877438660596));
#40521=CARTESIAN_POINT('Ctrl Pts',(-4.55880507325988,0.79477268400084,5.17508548891478));
#40522=CARTESIAN_POINT('Ctrl Pts',(-4.5923750883726,1.06847604194529,5.14740422222997));
#40523=CARTESIAN_POINT('Ctrl Pts',(-4.59241718007822,1.18514270861212,5.12973339070156));
#40524=CARTESIAN_POINT('Ctrl Pts',(-4.57797014783881,1.30000000000051,5.10637392230058));
#40525=CARTESIAN_POINT('Ctrl Pts',(-4.44513420311915,-1.30000000000135,
4.884733481637));
#40526=CARTESIAN_POINT('Ctrl Pts',(-4.46183589072991,-1.1851427086127,4.91840088906111));
#40527=CARTESIAN_POINT('Ctrl Pts',(-4.46637007123737,-1.06847604194559,
4.95000485425187));
#40528=CARTESIAN_POINT('Ctrl Pts',(-4.44873555975923,-0.794772684000863,
5.01824937184472));
#40529=CARTESIAN_POINT('Ctrl Pts',(-4.39084884309672,-0.636309800095208,
5.05638495800233));
#40530=CARTESIAN_POINT('Ctrl Pts',(-4.34217768828529,-0.319434907277166,
5.11265667084935));
#40531=CARTESIAN_POINT('Ctrl Pts',(-4.30445024732938,-0.158333333333335,
5.13496435846389));
#40532=CARTESIAN_POINT('Ctrl Pts',(-4.31843105932074,0.158333333333337,
5.16449168967078));
#40533=CARTESIAN_POINT('Ctrl Pts',(-4.37054787014169,0.319434907277172,
5.17256490560895));
#40534=CARTESIAN_POINT('Ctrl Pts',(-4.44686472935605,0.636309800095217,
5.17469957498278));
#40535=CARTESIAN_POINT('Ctrl Pts',(-4.51958918518332,0.794772684000857,
5.17002379850672));
#40536=CARTESIAN_POINT('Ctrl Pts',(-4.55836725083314,1.06847604194531,5.14277837197072));
#40537=CARTESIAN_POINT('Ctrl Pts',(-4.56202829741646,1.18514270861214,5.12568088174935));
#40538=CARTESIAN_POINT('Ctrl Pts',(-4.55256480283223,1.30000000000053,5.1032794369115));
#40539=CARTESIAN_POINT('Ctrl Pts',(-4.41974762070072,-1.30000000000138,
4.88408701534507));
#40540=CARTESIAN_POINT('Ctrl Pts',(-4.43179506545039,-1.18514270861273,
4.918318362789));
#40541=CARTESIAN_POINT('Ctrl Pts',(-4.43288914505467,-1.06847604194561,
4.95020390402413));
#40542=CARTESIAN_POINT('Ctrl Pts',(-4.41011222311145,-0.794772684000876,
5.0184466013386));
#40543=CARTESIAN_POINT('Ctrl Pts',(-4.35279015042126,-0.636309800095215,
5.05537792340058));
#40544=CARTESIAN_POINT('Ctrl Pts',(-4.30383441342919,-0.319434907277168,
5.11115473037836));
#40545=CARTESIAN_POINT('Ctrl Pts',(-4.26781347477672,-0.158333333333337,
5.13391900831901));
#40546=CARTESIAN_POINT('Ctrl Pts',(-4.28165805458559,0.158333333333339,
5.16286598935209));
#40547=CARTESIAN_POINT('Ctrl Pts',(-4.33200506651174,0.319434907277176,
5.17020279615525));
#40548=CARTESIAN_POINT('Ctrl Pts',(-4.40818044821254,0.636309800095224,
5.17103807912951));
#40549=CARTESIAN_POINT('Ctrl Pts',(-4.4795930281415,0.794772684000863,5.16458266721689));
#40550=CARTESIAN_POINT('Ctrl Pts',(-4.52365135936066,1.06847604194532,5.13766996221811));
#40551=CARTESIAN_POINT('Ctrl Pts',(-4.53102975534213,1.18514270861216,5.12126379080107));
#40552=CARTESIAN_POINT('Ctrl Pts',(-4.52671532824235,1.30000000000055,5.10010096074699));
#40553=CARTESIAN_POINT('Ctrl Pts',(-4.40650823227987,-1.30000000000138,
4.88380066054156));
#40554=CARTESIAN_POINT('Ctrl Pts',(-4.4158561187712,-1.18514270861273,4.91749327588164));
#40555=CARTESIAN_POINT('Ctrl Pts',(-4.41499837703178,-1.06847604194561,
4.94905656639272));
#40556=CARTESIAN_POINT('Ctrl Pts',(-4.38943977918113,-0.794772684000877,
5.01705491536285));
#40557=CARTESIAN_POINT('Ctrl Pts',(-4.33280187742144,-0.636309800095216,
5.0546567043112));
#40558=CARTESIAN_POINT('Ctrl Pts',(-4.28386852637352,-0.319434907277168,
5.11076200910592));
#40559=CARTESIAN_POINT('Ctrl Pts',(-4.24876292279781,-0.158333333333337,
5.13383636233795));
#40560=CARTESIAN_POINT('Ctrl Pts',(-4.26252502549056,0.158333333333339,
5.16244103234912));
#40561=CARTESIAN_POINT('Ctrl Pts',(-4.31179509598092,0.319434907277178,
5.16885016149766));
#40562=CARTESIAN_POINT('Ctrl Pts',(-4.38794127236082,0.636309800095226,
5.16922043239121));
#40563=CARTESIAN_POINT('Ctrl Pts',(-4.45892689575222,0.794772684000865,
5.16288729977276));
#40564=CARTESIAN_POINT('Ctrl Pts',(-4.50575118631774,1.06847604194532,5.13614182005032));
#40565=CARTESIAN_POINT('Ctrl Pts',(-4.51502186722484,1.18514270861216,5.11986708838312));
#40566=CARTESIAN_POINT('Ctrl Pts',(-4.5132947286642,1.30000000000055,5.09889475220289));
#40567=CARTESIAN_POINT('Ctrl Pts',(-4.4049564025435,-1.30000000000138,4.88378526077544));
#40568=CARTESIAN_POINT('Ctrl Pts',(-4.41398817097975,-1.18514270861273,
4.9174205499076));
#40569=CARTESIAN_POINT('Ctrl Pts',(-4.41290137938959,-1.06847604194561,
4.94894863383354));
#40570=CARTESIAN_POINT('Ctrl Pts',(-4.38701477553246,-0.794772684000877,
5.01691674930255));
#40571=CARTESIAN_POINT('Ctrl Pts',(-4.33045200394104,-0.636309800095216,
5.05457857089677));
#40572=CARTESIAN_POINT('Ctrl Pts',(-4.28152103228337,-0.319434907277168,
5.11072235315133));
#40573=CARTESIAN_POINT('Ctrl Pts',(-4.24652789605534,-0.158333333333337,
5.13385058759899));
#40574=CARTESIAN_POINT('Ctrl Pts',(-4.26028051529038,0.158333333333339,
5.16241615203963));
#40575=CARTESIAN_POINT('Ctrl Pts',(-4.30942099036749,0.319434907277178,
5.16870609135895));
#40576=CARTESIAN_POINT('Ctrl Pts',(-4.38556104175245,0.636309800095226,
5.16901160327323));
#40577=CARTESIAN_POINT('Ctrl Pts',(-4.45649411099206,0.794772684000865,
5.16268349828159));
#40578=CARTESIAN_POINT('Ctrl Pts',(-4.50364335604791,1.06847604194532,5.13595538713736));
#40579=CARTESIAN_POINT('Ctrl Pts',(-4.51313708026413,1.18514270861216,5.11969742432234));
#40580=CARTESIAN_POINT('Ctrl Pts',(-4.5117153675636,1.30000000000055,5.09875110763252));
#40581=CARTESIAN_POINT('Ctrl Pts',(-4.40224219033075,-1.30000000000138,
4.88376394744154));
#40582=CARTESIAN_POINT('Ctrl Pts',(-4.41072430196735,-1.18514270861273,
4.91731017602045));
#40583=CARTESIAN_POINT('Ctrl Pts',(-4.40923886277722,-1.06847604194561,
4.9487836208545));
#40584=CARTESIAN_POINT('Ctrl Pts',(-4.38278016467548,-0.794772684000877,
5.01670502955251));
#40585=CARTESIAN_POINT('Ctrl Pts',(-4.32634622956166,-0.636309800095216,
5.05446426311587));
#40586=CARTESIAN_POINT('Ctrl Pts',(-4.27741512031746,-0.319434907277168,
5.11066084001742));
#40587=CARTESIAN_POINT('Ctrl Pts',(-4.2426120790421,-0.158333333333337,
5.13385937190239));
#40588=CARTESIAN_POINT('Ctrl Pts',(-4.2563478462777,0.158333333333339,5.1623560768868));
#40589=CARTESIAN_POINT('Ctrl Pts',(-4.305269806891,0.319434907277178,5.16846781015905));
#40590=CARTESIAN_POINT('Ctrl Pts',(-4.38139923174149,0.636309800095227,
5.16865980598617));
#40591=CARTESIAN_POINT('Ctrl Pts',(-4.45223248915185,0.794772684000865,
5.16231031191246));
#40592=CARTESIAN_POINT('Ctrl Pts',(-4.49994911871515,1.06847604194532,5.13560794980462));
#40593=CARTESIAN_POINT('Ctrl Pts',(-4.50983384256683,1.18514270861216,5.11938217847402));
#40594=CARTESIAN_POINT('Ctrl Pts',(-4.50894852940762,1.30000000000055,5.09848909894929));
#40595=CARTESIAN_POINT('Ctrl Pts',(-4.39682707636092,-1.30000000000137,
4.88376677553948));
#40596=CARTESIAN_POINT('Ctrl Pts',(-4.4042228376766,-1.18514270861272,4.91717843866259));
#40597=CARTESIAN_POINT('Ctrl Pts',(-4.40194760492648,-1.06847604194561,
4.94856799844571));
#40598=CARTESIAN_POINT('Ctrl Pts',(-4.37434943114728,-0.794772684000875,
5.01641269776876));
#40599=CARTESIAN_POINT('Ctrl Pts',(-4.31815519215306,-0.636309800095215,
5.05430786254906));
#40600=CARTESIAN_POINT('Ctrl Pts',(-4.2692143702594,-0.319434907277168,
5.11057919803083));
#40601=CARTESIAN_POINT('Ctrl Pts',(-4.23478747864304,-0.158333333333337,
5.13390345071257));
#40602=CARTESIAN_POINT('Ctrl Pts',(-4.24848968363826,0.158333333333339,
5.16226517782403));
#40603=CARTESIAN_POINT('Ctrl Pts',(-4.29698668137947,0.319434907277177,
5.16806751836705));
#40604=CARTESIAN_POINT('Ctrl Pts',(-4.3730885201456,0.636309800095226,5.16800900169859));
#40605=CARTESIAN_POINT('Ctrl Pts',(-4.44369767060591,0.794772684000865,
5.1615231738282));
#40606=CARTESIAN_POINT('Ctrl Pts',(-4.49254607107023,1.06847604194532,5.13485966923599));
#40607=CARTESIAN_POINT('Ctrl Pts',(-4.50321621625043,1.18514270861216,5.11871051274717));
#40608=CARTESIAN_POINT('Ctrl Pts',(-4.50341184406145,1.30000000000055,5.09795384292729));
#40609=CARTESIAN_POINT('Ctrl Pts',(-4.38606558456593,-1.30000000000137,
4.8840266581289));
#40610=CARTESIAN_POINT('Ctrl Pts',(-4.39142503744879,-1.18514270861272,
4.9176134919098));
#40611=CARTESIAN_POINT('Ctrl Pts',(-4.38765033200399,-1.06847604194561,
4.94909627641851));
#40612=CARTESIAN_POINT('Ctrl Pts',(-4.35782827428032,-0.794772684000875,
5.01696703201057));
#40613=CARTESIAN_POINT('Ctrl Pts',(-4.30195661046983,-0.636309800095214,
5.0546304847714));
#40614=CARTESIAN_POINT('Ctrl Pts',(-4.25285778594573,-0.319434907277167,
5.11058605655013));
#40615=CARTESIAN_POINT('Ctrl Pts',(-4.21903395867086,-0.158333333333337,
5.13363428064143));
#40616=CARTESIAN_POINT('Ctrl Pts',(-4.23266654153631,0.158333333333339,
5.1617335078417));
#40617=CARTESIAN_POINT('Ctrl Pts',(-4.28053461320322,0.319434907277177,
5.16773276128116));
#40618=CARTESIAN_POINT('Ctrl Pts',(-4.35656350255669,0.636309800095225,
5.16708177445095));
#40619=CARTESIAN_POINT('Ctrl Pts',(-4.42647160968918,0.794772684000862,
5.15932956521396));
#40620=CARTESIAN_POINT('Ctrl Pts',(-4.4775477256098,1.06847604194531,5.13260801730426));
#40621=CARTESIAN_POINT('Ctrl Pts',(-4.4898161662824,1.18514270861216,5.1167254228346));
#40622=CARTESIAN_POINT('Ctrl Pts',(-4.49224408960217,1.30000000000055,5.09652700185447));
#40623=CARTESIAN_POINT('Ctrl Pts',(-4.37060167768334,-1.30000000000137,
4.88410602866374));
#40624=CARTESIAN_POINT('Ctrl Pts',(-4.37292250382272,-1.18514270861271,
4.91752711815292));
#40625=CARTESIAN_POINT('Ctrl Pts',(-4.36694158973788,-1.0684760419456,4.94893796562093));
#40626=CARTESIAN_POINT('Ctrl Pts',(-4.33394580104886,-0.794772684000867,
5.01685924577397));
#40627=CARTESIAN_POINT('Ctrl Pts',(-4.27876641146177,-0.636309800095212,
5.05493001675094));
#40628=CARTESIAN_POINT('Ctrl Pts',(-4.22965716001968,-0.319434907277167,
5.11114702069444));
#40629=CARTESIAN_POINT('Ctrl Pts',(-4.19690370361186,-0.158333333333336,
5.134513836664));
#40630=CARTESIAN_POINT('Ctrl Pts',(-4.21041567571181,0.158333333333339,
5.16217342131387));
#40631=CARTESIAN_POINT('Ctrl Pts',(-4.25703639618286,0.319434907277176,
5.16724835790094));
#40632=CARTESIAN_POINT('Ctrl Pts',(-4.33294485775093,0.636309800095223,
5.16577871662493));
#40633=CARTESIAN_POINT('Ctrl Pts',(-4.40219369493682,0.794772684000861,
5.15757132101997));
#40634=CARTESIAN_POINT('Ctrl Pts',(-4.45647104436528,1.06847604194531,5.13082793493229));
#40635=CARTESIAN_POINT('Ctrl Pts',(-4.47097018224745,1.18514270861215,5.11510038944369));
#40636=CARTESIAN_POINT('Ctrl Pts',(-4.47647380461819,1.30000000000054,5.09522151936374));
#40637=CARTESIAN_POINT('Ctrl Pts',(-4.35196499893507,-1.30000000000136,
4.88399187949457));
#40638=CARTESIAN_POINT('Ctrl Pts',(-4.35056153135029,-1.18514270861271,
4.91699062520585));
#40639=CARTESIAN_POINT('Ctrl Pts',(-4.34188287937219,-1.0684760419456,4.94817247295909));
#40640=CARTESIAN_POINT('Ctrl Pts',(-4.3050263258002,-0.79477268400087,5.01601138142398));
#40641=CARTESIAN_POINT('Ctrl Pts',(-4.25072828537927,-0.636309800095212,
5.05472404794897));
#40642=CARTESIAN_POINT('Ctrl Pts',(-4.20167033752839,-0.319434907277167,
5.11145251868633));
#40643=CARTESIAN_POINT('Ctrl Pts',(-4.17027754713746,-0.158333333333336,
5.13542659898148));
#40644=CARTESIAN_POINT('Ctrl Pts',(-4.18369951910936,0.158333333333338,
5.16273757843257));
#40645=CARTESIAN_POINT('Ctrl Pts',(-4.22883734848563,0.319434907277175,
5.16678173691335));
#40646=CARTESIAN_POINT('Ctrl Pts',(-4.30457682258443,0.636309800095222,
5.16424312854174));
#40647=CARTESIAN_POINT('Ctrl Pts',(-4.37296413646412,0.794772684000861,
5.15522516137196));
#40648=CARTESIAN_POINT('Ctrl Pts',(-4.43103930909429,1.06847604194531,5.1282867857786));
#40649=CARTESIAN_POINT('Ctrl Pts',(-4.44820285993171,1.18514270861215,5.11269495333857));
#40650=CARTESIAN_POINT('Ctrl Pts',(-4.45739137127217,1.30000000000054,5.09317191308771));
#40651=CARTESIAN_POINT('Ctrl Pts',(-4.32737417007851,-1.30000000000136,
4.88468811680626));
#40652=CARTESIAN_POINT('Ctrl Pts',(-4.32124043958264,-1.18514270861271,
4.91789151964559));
#40653=CARTESIAN_POINT('Ctrl Pts',(-4.30911969341762,-1.0684760419456,4.94927348967718));
#40654=CARTESIAN_POINT('Ctrl Pts',(-4.26728714113541,-0.794772684000867,
5.01756424422933));
#40655=CARTESIAN_POINT('Ctrl Pts',(-4.2140559268287,-0.63630980009521,5.05677413527469));
#40656=CARTESIAN_POINT('Ctrl Pts',(-4.1648465877658,-0.319434907277165,
5.11348677088921));
#40657=CARTESIAN_POINT('Ctrl Pts',(-4.13494732008885,-0.158333333333336,
5.13724902899869));
#40658=CARTESIAN_POINT('Ctrl Pts',(-4.14806315658605,0.158333333333338,
5.16352102529718));
#40659=CARTESIAN_POINT('Ctrl Pts',(-4.19122796504154,0.319434907277177,
5.16619566615263));
#40660=CARTESIAN_POINT('Ctrl Pts',(-4.26684838183568,0.636309800095222,
5.16266130049346));
#40661=CARTESIAN_POINT('Ctrl Pts',(-4.33434492497626,0.794772684000858,
5.15357916495107));
#40662=CARTESIAN_POINT('Ctrl Pts',(-4.39758617759598,1.06847604194531,5.12669405868028));
#40663=CARTESIAN_POINT('Ctrl Pts',(-4.4183085151726,1.18514270861215,5.11124790801923));
#40664=CARTESIAN_POINT('Ctrl Pts',(-4.43237839538611,1.30000000000054,5.09199317301038));
#40665=CARTESIAN_POINT('Ctrl Pts',(-4.30272254767684,-1.30000000000136,
4.88526757993008));
#40666=CARTESIAN_POINT('Ctrl Pts',(-4.29183336543115,-1.18514270861271,
4.91860694219569));
#40667=CARTESIAN_POINT('Ctrl Pts',(-4.27623603569334,-1.06847604194559,
4.95009040893693));
#40668=CARTESIAN_POINT('Ctrl Pts',(-4.22932632119549,-0.794772684000859,
5.01853602542309));
#40669=CARTESIAN_POINT('Ctrl Pts',(-4.17698541530236,-0.636309800095208,
5.05771031248182));
#40670=CARTESIAN_POINT('Ctrl Pts',(-4.12765193878455,-0.319434907277166,
5.11448930759117));
#40671=CARTESIAN_POINT('Ctrl Pts',(-4.09939356743927,-0.158333333333336,
5.13843780656823));
#40672=CARTESIAN_POINT('Ctrl Pts',(-4.11244871156721,0.158333333333338,
5.16449616510372));
#40673=CARTESIAN_POINT('Ctrl Pts',(-4.15396287852574,0.319434907277175,
5.16698457503574));
#40674=CARTESIAN_POINT('Ctrl Pts',(-4.2294800310024,0.63630980009522,5.16251350014463));
#40675=CARTESIAN_POINT('Ctrl Pts',(-4.29575238020146,0.794772684000857,
5.1521719621219));
#40676=CARTESIAN_POINT('Ctrl Pts',(-4.36396151425919,1.06847604194531,5.12463779817001));
#40677=CARTESIAN_POINT('Ctrl Pts',(-4.38817637480601,1.18514270861215,5.10910488156731));
#40678=CARTESIAN_POINT('Ctrl Pts',(-4.40708088916356,1.30000000000054,5.08995756769537));
#40679=CARTESIAN_POINT('Ctrl Pts',(-4.27815205391509,-1.30000000000136,
4.88612008534165));
#40680=CARTESIAN_POINT('Ctrl Pts',(-4.26247420431945,-1.18514270861271,
4.91954146733436));
#40681=CARTESIAN_POINT('Ctrl Pts',(-4.24343209635956,-1.0684760419456,4.95125381830094));
#40682=CARTESIAN_POINT('Ctrl Pts',(-4.19166890777269,-0.794772684000865,
5.02056748950684));
#40683=CARTESIAN_POINT('Ctrl Pts',(-4.14075814958985,-0.636309800095208,
5.06129138348443));
#40684=CARTESIAN_POINT('Ctrl Pts',(-4.09139626798141,-0.319434907277164,
5.1184462415078));
#40685=CARTESIAN_POINT('Ctrl Pts',(-4.06445906870166,-0.158333333333335,
5.14166936941548));
#40686=CARTESIAN_POINT('Ctrl Pts',(-4.077222140461,0.158333333333337,5.16683024787989));
#40687=CARTESIAN_POINT('Ctrl Pts',(-4.11699151010801,0.319434907277173,
5.16882586619956));
#40688=CARTESIAN_POINT('Ctrl Pts',(-4.19221010102953,0.636309800095218,
5.16280403349833));
#40689=CARTESIAN_POINT('Ctrl Pts',(-4.25705109432503,0.794772684000854,
5.15054725916305));
#40690=CARTESIAN_POINT('Ctrl Pts',(-4.33027708204415,1.06847604194531,5.12250447261737));
#40691=CARTESIAN_POINT('Ctrl Pts',(-4.3580759818353,1.18514270861215,5.1071645586451));
#40692=CARTESIAN_POINT('Ctrl Pts',(-4.38197696462424,1.30000000000054,5.08862341390855));
#40693=CARTESIAN_POINT('Ctrl Pts',(-4.25367312510128,-1.30000000000136,
4.88733406444623));
#40694=CARTESIAN_POINT('Ctrl Pts',(-4.23349817359138,-1.1851427086127,4.92168444828486));
#40695=CARTESIAN_POINT('Ctrl Pts',(-4.21113464578801,-1.06847604194559,
4.95398061417029));
#40696=CARTESIAN_POINT('Ctrl Pts',(-4.15441437369286,-0.79477268400086,
5.02384556377463));
#40697=CARTESIAN_POINT('Ctrl Pts',(-4.10397583550923,-0.636309800095207,
5.06331287038023));
#40698=CARTESIAN_POINT('Ctrl Pts',(-4.05453479166089,-0.319434907277165,
5.12067245588504));
#40699=CARTESIAN_POINT('Ctrl Pts',(-4.02967050652154,-0.158333333333335,
5.14532610117804));
#40700=CARTESIAN_POINT('Ctrl Pts',(-4.04233335055355,0.158333333333337,
5.17017149405673));
#40701=CARTESIAN_POINT('Ctrl Pts',(-4.07995175634696,0.319434907277172,
5.17049886858399));
#40702=CARTESIAN_POINT('Ctrl Pts',(-4.15500017782648,0.636309800095217,
5.16347129713085));
#40703=CARTESIAN_POINT('Ctrl Pts',(-4.21902871529604,0.794772684000855,
5.1514565662729));
#40704=CARTESIAN_POINT('Ctrl Pts',(-4.29723796226783,1.0684760419453,5.12277114120179));
#40705=CARTESIAN_POINT('Ctrl Pts',(-4.32846609096306,1.18514270861214,5.10706392718239));
#40706=CARTESIAN_POINT('Ctrl Pts',(-4.35706846327762,1.30000000000053,5.08806635675711));
#40707=CARTESIAN_POINT('Ctrl Pts',(-4.22347137391488,-1.30000000000136,
4.88985984435287));
#40708=CARTESIAN_POINT('Ctrl Pts',(-4.19726403779595,-1.18514270861271,
4.92425217904836));
#40709=CARTESIAN_POINT('Ctrl Pts',(-4.17057834860845,-1.06847604194559,
4.95683493041622));
#40710=CARTESIAN_POINT('Ctrl Pts',(-4.10782397684903,-0.79477268400086,
5.02792710474016));
#40711=CARTESIAN_POINT('Ctrl Pts',(-4.05936422436221,-0.636309800095202,
5.06979779123566));
#40712=CARTESIAN_POINT('Ctrl Pts',(-4.00989238454398,-0.31943490727716,
5.12764546106457));
#40713=CARTESIAN_POINT('Ctrl Pts',(-3.98654644901798,-0.158333333333334,
5.15103547557789));
#40714=CARTESIAN_POINT('Ctrl Pts',(-3.99873859858878,0.158333333333336,
5.1745258202819));
#40715=CARTESIAN_POINT('Ctrl Pts',(-4.0341451811996,0.319434907277171,5.17421957459374));
#40716=CARTESIAN_POINT('Ctrl Pts',(-4.10871941292505,0.636309800095212,
5.16504821135669));
#40717=CARTESIAN_POINT('Ctrl Pts',(-4.17095302500774,0.794772684000845,
5.150729827345));
#40718=CARTESIAN_POINT('Ctrl Pts',(-4.25523270922204,1.06847604194529,5.12075283767295));
#40719=CARTESIAN_POINT('Ctrl Pts',(-4.29082094784555,1.18514270861214,5.10486131848044));
#40720=CARTESIAN_POINT('Ctrl Pts',(-4.32551587266625,1.30000000000053,5.08605420816752));
#40721=CARTESIAN_POINT('Ctrl Pts',(-4.19598697828295,-1.30000000000135,
4.89148680791286));
#40722=CARTESIAN_POINT('Ctrl Pts',(-4.1646778729705,-1.1851427086127,4.92683910406031));
#40723=CARTESIAN_POINT('Ctrl Pts',(-4.13427147073223,-1.06847604194559,
4.96014889185388));
#40724=CARTESIAN_POINT('Ctrl Pts',(-4.06611202346847,-0.794772684000858,
5.03238256235729));
#40725=CARTESIAN_POINT('Ctrl Pts',(-4.01854562515569,-0.636309800095203,
5.07387317587653));
#40726=CARTESIAN_POINT('Ctrl Pts',(-3.96924679223899,-0.319434907277162,
5.13265453529849));
#40727=CARTESIAN_POINT('Ctrl Pts',(-3.94828394958136,-0.158333333333334,
5.1576571823155));
#40728=CARTESIAN_POINT('Ctrl Pts',(-3.96041752040512,0.158333333333336,
5.18102679218327));
#40729=CARTESIAN_POINT('Ctrl Pts',(-3.99345908856316,0.31943490727717,5.17927584842867));
#40730=CARTESIAN_POINT('Ctrl Pts',(-4.06758484757638,0.636309800095213,
5.16833686890515));
#40731=CARTESIAN_POINT('Ctrl Pts',(-4.12834371072759,0.794772684000849,
5.15257450864102));
#40732=CARTESIAN_POINT('Ctrl Pts',(-4.2181230949946,1.0684760419453,5.12153335051156));
#40733=CARTESIAN_POINT('Ctrl Pts',(-4.25763397221813,1.18514270861214,5.1054019255452));
#40734=CARTESIAN_POINT('Ctrl Pts',(-4.29779355787003,1.30000000000053,5.08657564277847));
#40735=CARTESIAN_POINT('Ctrl Pts',(-4.17817781145185,-1.30000000000135,
4.89391064073081));
#40736=CARTESIAN_POINT('Ctrl Pts',(-4.14343156900407,-1.1851427086127,4.9298229981819));
#40737=CARTESIAN_POINT('Ctrl Pts',(-4.11053739623518,-1.06847604194558,
4.96361408938916));
#40738=CARTESIAN_POINT('Ctrl Pts',(-4.03882392814598,-0.794772684000855,
5.03677772058128));
#40739=CARTESIAN_POINT('Ctrl Pts',(-3.99217793424401,-0.636309800095202,
5.07891426934365));
#40740=CARTESIAN_POINT('Ctrl Pts',(-3.94275628542362,-0.319434907277162,
5.13770211516119));
#40741=CARTESIAN_POINT('Ctrl Pts',(-3.92269078973397,-0.158333333333334,
5.16192232746968));
#40742=CARTESIAN_POINT('Ctrl Pts',(-3.93459308666009,0.158333333333336,
5.18469929682841));
#40743=CARTESIAN_POINT('Ctrl Pts',(-3.9664220559315,0.319434907277171,5.18295439880769));
#40744=CARTESIAN_POINT('Ctrl Pts',(-4.04037059975343,0.636309800095213,
5.17117604923734));
#40745=CARTESIAN_POINT('Ctrl Pts',(-4.10022631076594,0.794772684000849,
5.15474803524041));
#40746=CARTESIAN_POINT('Ctrl Pts',(-4.19346831247043,1.0684760419453,5.12236157619796));
#40747=CARTESIAN_POINT('Ctrl Pts',(-4.23543357124736,1.18514270861213,5.10556374198919));
#40748=CARTESIAN_POINT('Ctrl Pts',(-4.27900308121998,1.30000000000052,5.08598697165455));
#40749=CARTESIAN_POINT('Ctrl Pts',(-4.16614832183943,-1.30000000000135,
4.89515416503372));
#40750=CARTESIAN_POINT('Ctrl Pts',(-4.12927305326624,-1.1851427086127,4.93187374670616));
#40751=CARTESIAN_POINT('Ctrl Pts',(-4.09481646701293,-1.06847604194558,
4.96624192261934));
#40752=CARTESIAN_POINT('Ctrl Pts',(-4.02080249976618,-0.794772684000856,
5.04020706660765));
#40753=CARTESIAN_POINT('Ctrl Pts',(-3.97448924330781,-0.636309800095203,
5.0820240583604));
#40754=CARTESIAN_POINT('Ctrl Pts',(-3.92502015216261,-0.319434907277163,
5.14089736102373));
#40755=CARTESIAN_POINT('Ctrl Pts',(-3.90579764168114,-0.158333333333334,
5.16522599392556));
#40756=CARTESIAN_POINT('Ctrl Pts',(-3.91763888697422,0.158333333333336,
5.18786464483484));
#40757=CARTESIAN_POINT('Ctrl Pts',(-3.94860628975023,0.31943490727717,5.18601843378387));
#40758=CARTESIAN_POINT('Ctrl Pts',(-4.02239140907987,0.636309800095213,
5.1735766603289));
#40759=CARTESIAN_POINT('Ctrl Pts',(-4.08155211767191,0.794772684000849,
5.15644136256273));
#40760=CARTESIAN_POINT('Ctrl Pts',(-4.1771132744239,1.0684760419453,5.1231992607686));
#40761=CARTESIAN_POINT('Ctrl Pts',(-4.220744319771,1.18514270861214,5.10604551223169));
#40762=CARTESIAN_POINT('Ctrl Pts',(-4.26664152659707,1.30000000000053,5.0861272892833));
#40763=CARTESIAN_POINT('Ctrl Pts',(-4.1508669168539,-1.30000000000135,4.89606494834189));
#40764=CARTESIAN_POINT('Ctrl Pts',(-4.11107919495639,-1.1851427086127,4.93312453755988));
#40765=CARTESIAN_POINT('Ctrl Pts',(-4.07455046284514,-1.06847604194559,
4.9678928592167));
#40766=CARTESIAN_POINT('Ctrl Pts',(-3.99769070248542,-0.794772684000857,
5.04292135118991));
#40767=CARTESIAN_POINT('Ctrl Pts',(-3.95237996500392,-0.636309800095203,
5.08586704224943));
#40768=CARTESIAN_POINT('Ctrl Pts',(-3.90310151350184,-0.319434907277162,
5.1455008236609));
#40769=CARTESIAN_POINT('Ctrl Pts',(-3.88492029224199,-0.158333333333334,
5.16994987776997));
#40770=CARTESIAN_POINT('Ctrl Pts',(-3.89655168321942,0.158333333333336,
5.19206004283178));
#40771=CARTESIAN_POINT('Ctrl Pts',(-3.9261827815684,0.319434907277171,5.1894116045783));
#40772=CARTESIAN_POINT('Ctrl Pts',(-3.99952326972462,0.636309800095214,
5.17544516685783));
#40773=CARTESIAN_POINT('Ctrl Pts',(-4.05759908040726,0.794772684000849,
5.15669555841508));
#40774=CARTESIAN_POINT('Ctrl Pts',(-4.15617967915481,1.0684760419453,5.12274651323053));
#40775=CARTESIAN_POINT('Ctrl Pts',(-4.20203738654327,1.18514270861213,5.10559522792422));
#40776=CARTESIAN_POINT('Ctrl Pts',(-4.25108091289353,1.30000000000052,5.08598794103589));
#40777=CARTESIAN_POINT('Ctrl Pts',(-4.13323139050191,-1.30000000000135,
4.89899172467419));
#40778=CARTESIAN_POINT('Ctrl Pts',(-4.09014474267955,-1.1851427086127,4.93699722021868));
#40779=CARTESIAN_POINT('Ctrl Pts',(-4.05121499879604,-1.06847604194558,
4.97248672392271));
#40780=CARTESIAN_POINT('Ctrl Pts',(-3.97088278224124,-0.794772684000856,
5.04866213265584));
#40781=CARTESIAN_POINT('Ctrl Pts',(-3.92632338133767,-0.636309800095201,
5.09175632655176));
#40782=CARTESIAN_POINT('Ctrl Pts',(-3.87691545645197,-0.319434907277162,
5.15138050949605));
#40783=CARTESIAN_POINT('Ctrl Pts',(-3.85972265622446,-0.158333333333333,
5.17531708798847));
#40784=CARTESIAN_POINT('Ctrl Pts',(-3.87114337975094,0.158333333333336,
5.19692904080684));
#40785=CARTESIAN_POINT('Ctrl Pts',(-3.89949164386545,0.31943490727717,5.19410951983121));
#40786=CARTESIAN_POINT('Ctrl Pts',(-3.97270307504151,0.636309800095212,
5.17951539476134));
#40787=CARTESIAN_POINT('Ctrl Pts',(-4.03003677717091,0.794772684000847,
5.16065805954507));
#40788=CARTESIAN_POINT('Ctrl Pts',(-4.13208575882067,1.06847604194529,5.12540031643046));
#40789=CARTESIAN_POINT('Ctrl Pts',(-4.18036558146868,1.18514270861213,5.1074772650306));
#40790=CARTESIAN_POINT('Ctrl Pts',(-4.23275200389592,1.30000000000052,5.08689293279707));
#40791=CARTESIAN_POINT('Ctrl Pts',(-4.10625889988844,-1.30000000000135,
4.90204030255314));
#40792=CARTESIAN_POINT('Ctrl Pts',(-4.05808112442856,-1.1851427086127,4.94104135877227));
#40793=CARTESIAN_POINT('Ctrl Pts',(-4.01551425518549,-1.06847604194559,
4.97747714274429));
#40794=CARTESIAN_POINT('Ctrl Pts',(-3.93013858757992,-0.794772684000858,
5.05572480060138));
#40795=CARTESIAN_POINT('Ctrl Pts',(-3.88710540052421,-0.636309800095203,
5.10008878779615));
#40796=CARTESIAN_POINT('Ctrl Pts',(-3.83817100406078,-0.319434907277162,
5.16133735665563));
#40797=CARTESIAN_POINT('Ctrl Pts',(-3.82328588369641,-0.158333333333334,
5.18648529424092));
#40798=CARTESIAN_POINT('Ctrl Pts',(-3.83439947201774,0.158333333333336,
5.20739268922943));
#40799=CARTESIAN_POINT('Ctrl Pts',(-3.86001471967997,0.31943490727717,5.20245646788849));
#40800=CARTESIAN_POINT('Ctrl Pts',(-3.93236777784375,0.636309800095212,
5.18521180474951));
#40801=CARTESIAN_POINT('Ctrl Pts',(-3.98813117380777,0.79477268400085,5.16473826409429));
#40802=CARTESIAN_POINT('Ctrl Pts',(-4.09528276000506,1.06847604194529,5.12731890285593));
#40803=CARTESIAN_POINT('Ctrl Pts',(-4.14728494579063,1.18514270861213,5.10855990412802));
#40804=CARTESIAN_POINT('Ctrl Pts',(-4.20490736605451,1.30000000000052,5.08723936162831));
#40805=CARTESIAN_POINT('Ctrl Pts',(-4.07668616191916,-1.30000000000134,
4.90655222882955));
#40806=CARTESIAN_POINT('Ctrl Pts',(-4.02302103967041,-1.18514270861269,
4.94721000383966));
#40807=CARTESIAN_POINT('Ctrl Pts',(-3.97655137533068,-1.06847604194558,
4.98511937718202));
#40808=CARTESIAN_POINT('Ctrl Pts',(-3.88582010169789,-0.794772684000854,
5.0663482556785));
#40809=CARTESIAN_POINT('Ctrl Pts',(-3.84484404947985,-0.636309800095198,
5.11281258867805));
#40810=CARTESIAN_POINT('Ctrl Pts',(-3.79596540058121,-0.319434907277159,
5.17472528225949));
#40811=CARTESIAN_POINT('Ctrl Pts',(-3.7823500380607,-0.158333333333333,
5.19817022424681));
#40812=CARTESIAN_POINT('Ctrl Pts',(-3.79296246664124,0.158333333333335,
5.21799372334928));
#40813=CARTESIAN_POINT('Ctrl Pts',(-3.81658630793045,0.319434907277169,
5.21329214661253));
#40814=CARTESIAN_POINT('Ctrl Pts',(-3.88831191200828,0.636309800095209,
5.19395864824761));
#40815=CARTESIAN_POINT('Ctrl Pts',(-3.94196785883248,0.794772684000841,
5.1708896797082));
#40816=CARTESIAN_POINT('Ctrl Pts',(-4.05479149099295,1.06847604194529,5.13099102890868));
#40817=CARTESIAN_POINT('Ctrl Pts',(-4.11096942696579,1.18514270861213,5.1113232273092));
#40818=CARTESIAN_POINT('Ctrl Pts',(-4.17448812907675,1.30000000000052,5.08925827165065));
#40819=CARTESIAN_POINT('Ctrl Pts',(-4.04716803737985,-1.30000000000135,
4.91112623751931));
#40820=CARTESIAN_POINT('Ctrl Pts',(-3.9881710480236,-1.1851427086127,4.95362920167102));
#40821=CARTESIAN_POINT('Ctrl Pts',(-3.93793472154304,-1.06847604194558,
4.99319008793396));
#40822=CARTESIAN_POINT('Ctrl Pts',(-3.84211764143791,-0.794772684000852,
5.07778686084563));
#40823=CARTESIAN_POINT('Ctrl Pts',(-3.80313764148869,-0.636309800095198,
5.12615186704337));
#40824=CARTESIAN_POINT('Ctrl Pts',(-3.75484016665707,-0.319434907277159,
5.18987579309421));
#40825=CARTESIAN_POINT('Ctrl Pts',(-3.74336735637233,-0.158333333333332,
5.21365277657516));
#40826=CARTESIAN_POINT('Ctrl Pts',(-3.75358889560144,0.158333333333335,
5.23271082624441));
#40827=CARTESIAN_POINT('Ctrl Pts',(-3.77449313381615,0.319434907277168,
5.22659823861587));
#40828=CARTESIAN_POINT('Ctrl Pts',(-3.84522054790868,0.636309800095208,
5.20453295999464));
#40829=CARTESIAN_POINT('Ctrl Pts',(-3.89696787912242,0.794772684000843,
5.17961206984491));
#40830=CARTESIAN_POINT('Ctrl Pts',(-4.01503333068514,1.06847604194529,5.13639017041117));
#40831=CARTESIAN_POINT('Ctrl Pts',(-4.07510406689772,1.18514270861212,5.11518154429486));
#40832=CARTESIAN_POINT('Ctrl Pts',(-4.14413938009749,1.30000000000051,5.0914734507979));
#40833=CARTESIAN_POINT('Ctrl Pts',(-4.02686024311897,-1.30000000000134,
4.91538283693451));
#40834=CARTESIAN_POINT('Ctrl Pts',(-3.96400923923139,-1.1851427086127,4.95925335681388));
#40835=CARTESIAN_POINT('Ctrl Pts',(-3.91108111387555,-1.06847604194558,
5.00009937316502));
#40836=CARTESIAN_POINT('Ctrl Pts',(-3.81173039054196,-0.794772684000857,
5.08747463395353));
#40837=CARTESIAN_POINT('Ctrl Pts',(-3.77482876016749,-0.636309800095199,
5.13859565593173));
#40838=CARTESIAN_POINT('Ctrl Pts',(-3.72633243605006,-0.319434907277159,
5.20226275136205));
#40839=CARTESIAN_POINT('Ctrl Pts',(-3.71468118444881,-0.158333333333333,
5.22245677431171));
#40840=CARTESIAN_POINT('Ctrl Pts',(-3.72435431344552,0.158333333333335,
5.2404040033757));
#40841=CARTESIAN_POINT('Ctrl Pts',(-3.74458434460951,0.319434907277169,
5.23620771392481));
#40842=CARTESIAN_POINT('Ctrl Pts',(-3.81501324700601,0.636309800095209,
5.21306881395242));
#40843=CARTESIAN_POINT('Ctrl Pts',(-3.86503295408965,0.794772684000844,
5.18590559368825));
#40844=CARTESIAN_POINT('Ctrl Pts',(-3.9868511233865,1.06847604194529,5.14013147276438));
#40845=CARTESIAN_POINT('Ctrl Pts',(-4.04973779600462,1.18514270861212,5.11779749257155));
#40846=CARTESIAN_POINT('Ctrl Pts',(-4.12278056956027,1.30000000000051,5.09294345303549));
#40847=CARTESIAN_POINT('Ctrl Pts',(-4.01232252275008,-1.30000000000134,
4.91808539201452));
#40848=CARTESIAN_POINT('Ctrl Pts',(-3.94726047781966,-1.18514270861269,
4.96365346105024));
#40849=CARTESIAN_POINT('Ctrl Pts',(-3.89264513091886,-1.06847604194558,
5.00556768762124));
#40850=CARTESIAN_POINT('Ctrl Pts',(-3.79060671611871,-0.794772684000853,
5.09395682887023));
#40851=CARTESIAN_POINT('Ctrl Pts',(-3.75355156744856,-0.636309800095198,
5.14338738082634));
#40852=CARTESIAN_POINT('Ctrl Pts',(-3.70466736151699,-0.319434907277159,
5.20626768635415));
#40853=CARTESIAN_POINT('Ctrl Pts',(-3.69371769727687,-0.158333333333333,
5.22571268347603));
#40854=CARTESIAN_POINT('Ctrl Pts',(-3.70361224364535,0.158333333333335,
5.2441977360215));
#40855=CARTESIAN_POINT('Ctrl Pts',(-3.72370836064582,0.319434907277169,
5.24208037810435));
#40856=CARTESIAN_POINT('Ctrl Pts',(-3.79427085791425,0.636309800095209,
5.21921036128222));
#40857=CARTESIAN_POINT('Ctrl Pts',(-3.8431400259095,0.794772684000843,5.19086038002993));
#40858=CARTESIAN_POINT('Ctrl Pts',(-3.96751938670524,1.06847604194529,5.14371082198786));
#40859=CARTESIAN_POINT('Ctrl Pts',(-4.03228901928671,1.18514270861212,5.12068238772968));
#40860=CARTESIAN_POINT('Ctrl Pts',(-4.10798906787067,1.30000000000051,5.09503481582645));
#40861=CARTESIAN_POINT('Ctrl Pts',(-3.99512086302667,-1.30000000000134,
4.92222147175269));
#40862=CARTESIAN_POINT('Ctrl Pts',(-3.92707232624567,-1.18514270861269,
4.96998997195516));
#40863=CARTESIAN_POINT('Ctrl Pts',(-3.87008579662005,-1.06847604194558,
5.01313728134372));
#40864=CARTESIAN_POINT('Ctrl Pts',(-3.76399096254472,-0.794772684000854,
5.10214032237463));
#40865=CARTESIAN_POINT('Ctrl Pts',(-3.72603399380682,-0.636309800095198,
5.14824835584075));
#40866=CARTESIAN_POINT('Ctrl Pts',(-3.67610766531818,-0.319434907277159,
5.20923720889898));
#40867=CARTESIAN_POINT('Ctrl Pts',(-3.6661554730306,-0.158333333333333,
5.22783807506664));
#40868=CARTESIAN_POINT('Ctrl Pts',(-3.67599170976141,0.158333333333335,
5.2462475697323));
#40869=CARTESIAN_POINT('Ctrl Pts',(-3.69515914265524,0.319434907277168,
5.24522806832112));
#40870=CARTESIAN_POINT('Ctrl Pts',(-3.76638610152451,0.636309800095208,
5.22342487136686));
#40871=CARTESIAN_POINT('Ctrl Pts',(-3.81538419450183,0.794772684000843,
5.19662287275888));
#40872=CARTESIAN_POINT('Ctrl Pts',(-3.94378191370543,1.06847604194529,5.14863512557791));
#40873=CARTESIAN_POINT('Ctrl Pts',(-4.01108528305494,1.18514270861213,5.12465321506705));
#40874=CARTESIAN_POINT('Ctrl Pts',(-4.09011340671507,1.30000000000051,5.09746151167872));
#40875=CARTESIAN_POINT('Ctrl Pts',(-3.983352778511,-1.30000000000134,4.92491429713353));
#40876=CARTESIAN_POINT('Ctrl Pts',(-3.91381537680073,-1.18514270861269,
4.97543838782684));
#40877=CARTESIAN_POINT('Ctrl Pts',(-3.8555022312982,-1.06847604194558,5.01986946156966));
#40878=CARTESIAN_POINT('Ctrl Pts',(-3.74671747692744,-0.794772684000851,
5.10843804226175));
#40879=CARTESIAN_POINT('Ctrl Pts',(-3.70705838932681,-0.636309800095196,
5.14816850605185));
#40880=CARTESIAN_POINT('Ctrl Pts',(-3.65612349313465,-0.319434907277159,
5.20582783218244));
#40881=CARTESIAN_POINT('Ctrl Pts',(-3.64724201481597,-0.158333333333332,
5.22424600109739));
#40882=CARTESIAN_POINT('Ctrl Pts',(-3.65704996975845,0.158333333333335,
5.24249822284547));
#40883=CARTESIAN_POINT('Ctrl Pts',(-3.67523755008907,0.319434907277167,
5.24161469395223));
#40884=CARTESIAN_POINT('Ctrl Pts',(-3.74717278258778,0.636309800095206,
5.22259549162792));
#40885=CARTESIAN_POINT('Ctrl Pts',(-3.79716553103066,0.79477268400084,5.20123433415373));
#40886=CARTESIAN_POINT('Ctrl Pts',(-3.92828386839274,1.06847604194529,5.15372462655724));
#40887=CARTESIAN_POINT('Ctrl Pts',(-3.99710096186636,1.18514270861212,5.12872323336551));
#40888=CARTESIAN_POINT('Ctrl Pts',(-4.07797887898274,1.30000000000051,5.09928563899242));
#40889=CARTESIAN_POINT('Ctrl Pts',(-3.97477914228554,-1.30000000000134,
4.92421546647393));
#40890=CARTESIAN_POINT('Ctrl Pts',(-3.90549290340884,-1.18514270861269,
4.9747309843426));
#40891=CARTESIAN_POINT('Ctrl Pts',(-3.84729017393187,-1.06847604194558,
5.01883535605274));
#40892=CARTESIAN_POINT('Ctrl Pts',(-3.73843534938597,-0.794772684000851,
5.10591424758072));
#40893=CARTESIAN_POINT('Ctrl Pts',(-3.69814954202848,-0.636309800095196,
5.14315668292551));
#40894=CARTESIAN_POINT('Ctrl Pts',(-3.64686579593571,-0.319434907277159,
5.19916589978869));
#40895=CARTESIAN_POINT('Ctrl Pts',(-3.6379450782909,-0.158333333333332,
5.21761871575033));
#40896=CARTESIAN_POINT('Ctrl Pts',(-3.64772547716596,0.158333333333335,
5.23563571893282));
#40897=CARTESIAN_POINT('Ctrl Pts',(-3.66586376136843,0.319434907277167,
5.23420897929763));
#40898=CARTESIAN_POINT('Ctrl Pts',(-3.73821592466294,0.636309800095206,
5.21691754730656));
#40899=CARTESIAN_POINT('Ctrl Pts',(-3.78913144751244,0.79477268400084,5.19908697787931));
#40900=CARTESIAN_POINT('Ctrl Pts',(-3.92026688586173,1.06847604194529,5.15292277487033));
#40901=CARTESIAN_POINT('Ctrl Pts',(-3.98887475074047,1.18514270861212,5.12794379392484));
#40902=CARTESIAN_POINT('Ctrl Pts',(-4.06932680828339,1.30000000000051,5.09796860496417));
#40903=CARTESIAN_POINT('Ctrl Pts',(-3.97477914228473,-1.3,4.92421546647452));
#40904=CARTESIAN_POINT('Ctrl Pts',(-3.90549290340839,-1.18514270861178,
4.97473098434294));
#40905=CARTESIAN_POINT('Ctrl Pts',(-3.84729017393168,-1.06847604194512,
5.01883535605289));
#40906=CARTESIAN_POINT('Ctrl Pts',(-3.73843534938597,-0.794772684000851,
5.10591424758072));
#40907=CARTESIAN_POINT('Ctrl Pts',(-3.69814954202848,-0.636309800095197,
5.14315668292551));
#40908=CARTESIAN_POINT('Ctrl Pts',(-3.64686579593571,-0.319434907277159,
5.19916589978868));
#40909=CARTESIAN_POINT('Ctrl Pts',(-3.6379450782909,-0.158333333333332,
5.21761871575033));
#40910=CARTESIAN_POINT('Ctrl Pts',(-3.64772547716596,0.158333333333334,
5.23563571893282));
#40911=CARTESIAN_POINT('Ctrl Pts',(-3.66586376136842,0.319434907277167,
5.23420897929763));
#40912=CARTESIAN_POINT('Ctrl Pts',(-3.73821592466293,0.636309800095206,
5.21691754730656));
#40913=CARTESIAN_POINT('Ctrl Pts',(-3.78913144751243,0.79477268400084,5.19908697787931));
#40914=CARTESIAN_POINT('Ctrl Pts',(-3.92026688586164,1.06847604194511,5.15292277487035));
#40915=CARTESIAN_POINT('Ctrl Pts',(-3.98887475074027,1.18514270861178,5.12794379392492));
#40916=CARTESIAN_POINT('Ctrl Pts',(-4.06932680828303,1.3,5.09796860496431));
#40917=CARTESIAN_POINT('',(-4.38974166843611,-1.2,4.91249741324829));
#40918=CARTESIAN_POINT('Ctrl Pts',(-4.38974166843611,-1.2,4.91249741324829));
#40919=CARTESIAN_POINT('Ctrl Pts',(-4.37461051593519,-1.211983516113,4.90939208523401));
#40920=CARTESIAN_POINT('Ctrl Pts',(-4.34731408198419,-1.23320834189274,
4.90307035926027));
#40921=CARTESIAN_POINT('Ctrl Pts',(-4.30332881373785,-1.26800264000266,
4.89446891161289));
#40922=CARTESIAN_POINT('Ctrl Pts',(-4.28396809346178,-1.28318693061577,
4.89052779190164));
#40923=CARTESIAN_POINT('Ctrl Pts',(-4.26288026198571,-1.29999999996411,
4.88691723617146));
#40924=CARTESIAN_POINT('',(-4.45989076532205,-0.653834841370044,5.05247250051788));
#40925=CARTESIAN_POINT('Ctrl Pts',(-4.45989076535295,-0.653834841368788,
5.0524725004975));
#40926=CARTESIAN_POINT('Ctrl Pts',(-4.45290452376729,-0.71730390830208,
5.03796378089337));
#40927=CARTESIAN_POINT('Ctrl Pts',(-4.44705077906394,-0.764712012454701,
5.0259462125413));
#40928=CARTESIAN_POINT('Ctrl Pts',(-4.42424443208212,-0.949624929693292,
4.97968576415318));
#40929=CARTESIAN_POINT('Ctrl Pts',(-4.41009602593574,-1.05881338582905,
4.95155764066304));
#40930=CARTESIAN_POINT('Ctrl Pts',(-4.38974166843611,-1.2,4.91249741324829));
#40931=CARTESIAN_POINT('',(-4.51863764645953,0.653834841531101,5.17900672440537));
#40932=CARTESIAN_POINT('Ctrl Pts',(-4.51863764645953,0.653834841531102,
5.17900672440538));
#40933=CARTESIAN_POINT('Ctrl Pts',(-4.47706146767404,0.575967435244021,
5.1784184981011));
#40934=CARTESIAN_POINT('Ctrl Pts',(-4.44192892421759,0.49363270220023,5.17716396632452));
#40935=CARTESIAN_POINT('Ctrl Pts',(-4.39149772313144,0.338127729760966,
5.17291995537731));
#40936=CARTESIAN_POINT('Ctrl Pts',(-4.37381871579893,0.265652356086789,
5.17019838028741));
#40937=CARTESIAN_POINT('Ctrl Pts',(-4.35075689041254,0.129712176552852,
5.16231216794911));
#40938=CARTESIAN_POINT('Ctrl Pts',(-4.34396311929369,0.0666225871102778,
5.1575862721065));
#40939=CARTESIAN_POINT('Ctrl Pts',(-4.3380158949138,-0.0595427376094998,
5.14565883562823));
#40940=CARTESIAN_POINT('Ctrl Pts',(-4.33880327069977,-0.122774428304041,
5.13837690399667));
#40941=CARTESIAN_POINT('Ctrl Pts',(-4.34923014512322,-0.260123906820502,
5.12045087664636));
#40942=CARTESIAN_POINT('Ctrl Pts',(-4.36045995272139,-0.333941086098924,
5.10943130653841));
#40943=CARTESIAN_POINT('Ctrl Pts',(-4.3972325539662,-0.491209295028013,
5.08375339409386));
#40944=CARTESIAN_POINT('Ctrl Pts',(-4.42491420924364,-0.574352714525261,
5.06856467535912));
#40945=CARTESIAN_POINT('Ctrl Pts',(-4.45989076527149,-0.65383484138658,
5.05247250048966));
#40946=CARTESIAN_POINT('',(-4.48863704729437,1.2,5.11322318930451));
#40947=CARTESIAN_POINT('Ctrl Pts',(-4.48863704729437,1.2,5.11322318930451));
#40948=CARTESIAN_POINT('Ctrl Pts',(-4.49416731133851,1.13013423818568,5.12511873459839));
#40949=CARTESIAN_POINT('Ctrl Pts',(-4.49993170183524,1.05323108968555,5.13758912248786));
#40950=CARTESIAN_POINT('Ctrl Pts',(-4.5137823832937,0.796443355018211,5.16814456459401));
#40951=CARTESIAN_POINT('Ctrl Pts',(-4.51601205652913,0.739828131497515,
5.17313629937876));
#40952=CARTESIAN_POINT('Ctrl Pts',(-4.51863764645953,0.653834841531102,
5.17900672440538));
#40953=CARTESIAN_POINT('Ctrl Pts',(-4.36610424565707,1.30000000000001,5.08821551382361));
#40954=CARTESIAN_POINT('Ctrl Pts',(-4.38654452017538,1.28314808556143,5.09177297168868));
#40955=CARTESIAN_POINT('Ctrl Pts',(-4.40703706424362,1.26652555865796,5.09607491528727));
#40956=CARTESIAN_POINT('Ctrl Pts',(-4.44785780404133,1.2330928376765,5.10412551204498));
#40957=CARTESIAN_POINT('Ctrl Pts',(-4.46873140079917,1.21600397350301,5.10836902693465));
#40958=CARTESIAN_POINT('Ctrl Pts',(-4.48863704729437,1.2,5.11322318930451));
#40959=CARTESIAN_POINT('Ctrl Pts',(-3.97477914228473,-1.3,4.92421546647452));
#40960=CARTESIAN_POINT('Ctrl Pts',(-3.90549290340839,-1.18514270861178,
4.97473098434294));
#40961=CARTESIAN_POINT('Ctrl Pts',(-3.84729017393168,-1.06847604194512,
5.01883535605288));
#40962=CARTESIAN_POINT('Ctrl Pts',(-3.73843534938597,-0.794772684000851,
5.10591424758072));
#40963=CARTESIAN_POINT('Ctrl Pts',(-3.69814954202848,-0.636309800095196,
5.1431566829255));
#40964=CARTESIAN_POINT('Ctrl Pts',(-3.64686579593571,-0.319434907277159,
5.19916589978868));
#40965=CARTESIAN_POINT('Ctrl Pts',(-3.63794507829089,-0.158333333333332,
5.21761871575032));
#40966=CARTESIAN_POINT('Ctrl Pts',(-3.64772547716596,0.158333333333334,
5.23563571893282));
#40967=CARTESIAN_POINT('Ctrl Pts',(-3.66586376136842,0.319434907277167,
5.23420897929763));
#40968=CARTESIAN_POINT('Ctrl Pts',(-3.73821592466293,0.636309800095206,
5.21691754730656));
#40969=CARTESIAN_POINT('Ctrl Pts',(-3.78913144751243,0.79477268400084,5.19908697787931));
#40970=CARTESIAN_POINT('Ctrl Pts',(-3.92026688586164,1.06847604194511,5.15292277487035));
#40971=CARTESIAN_POINT('Ctrl Pts',(-3.98887475074026,1.18514270861178,5.12794379392492));
#40972=CARTESIAN_POINT('Ctrl Pts',(-4.06932680828303,1.3,5.09796860496431));
#40973=CARTESIAN_POINT('Ctrl Pts',(-3.93487809212144,-1.3,4.85843541273091));
#40974=CARTESIAN_POINT('Ctrl Pts',(-3.86662549823904,-1.18514270861178,
4.91034106835601));
#40975=CARTESIAN_POINT('Ctrl Pts',(-3.809178223755,-1.06847604194512,4.9553862039665));
#40976=CARTESIAN_POINT('Ctrl Pts',(-3.70142597681593,-0.794772684000851,
5.04360030479917));
#40977=CARTESIAN_POINT('Ctrl Pts',(-3.6609356094067,-0.636309800095196,
5.08015487886936));
#40978=CARTESIAN_POINT('Ctrl Pts',(-3.60969614500507,-0.319434907277159,
5.13549872192357));
#40979=CARTESIAN_POINT('Ctrl Pts',(-3.60031408828523,-0.158333333333332,
5.1527988809256));
#40980=CARTESIAN_POINT('Ctrl Pts',(-3.61040534854147,0.158333333333334,
5.17063640820599));
#40981=CARTESIAN_POINT('Ctrl Pts',(-3.62931119341529,0.319434907277167,
5.17018552840934));
#40982=CARTESIAN_POINT('Ctrl Pts',(-3.70226172817696,0.636309800095206,
5.1531884342533));
#40983=CARTESIAN_POINT('Ctrl Pts',(-3.75367067633866,0.79477268400084,5.13587894966475));
#40984=CARTESIAN_POINT('Ctrl Pts',(-3.88437428339459,1.06847604194511,5.08819228178639));
#40985=CARTESIAN_POINT('Ctrl Pts',(-3.95254515033271,1.18514270861178,5.06208867567562));
#40986=CARTESIAN_POINT('Ctrl Pts',(-4.0323101357604,1.3,5.03052325501342));
#40987=CARTESIAN_POINT('Ctrl Pts',(-3.89497704195815,-1.3,4.7926553589873));
#40988=CARTESIAN_POINT('Ctrl Pts',(-3.8277580930697,-1.18514270861178,4.84595115236908));
#40989=CARTESIAN_POINT('Ctrl Pts',(-3.77106627357833,-1.06847604194512,
4.89193705188011));
#40990=CARTESIAN_POINT('Ctrl Pts',(-3.66441660424588,-0.794772684000851,
4.98128636201762));
#40991=CARTESIAN_POINT('Ctrl Pts',(-3.62372167678492,-0.636309800095196,
5.01715307481322));
#40992=CARTESIAN_POINT('Ctrl Pts',(-3.57252649407444,-0.319434907277159,
5.07183154405846));
#40993=CARTESIAN_POINT('Ctrl Pts',(-3.56268309827957,-0.158333333333332,
5.08797904610087));
#40994=CARTESIAN_POINT('Ctrl Pts',(-3.57308521991697,0.158333333333334,
5.10563709747917));
#40995=CARTESIAN_POINT('Ctrl Pts',(-3.59275862546217,0.319434907277167,
5.10616207752106));
#40996=CARTESIAN_POINT('Ctrl Pts',(-3.66630753169098,0.636309800095206,
5.08945932120005));
#40997=CARTESIAN_POINT('Ctrl Pts',(-3.71820990516489,0.79477268400084,5.07267092145019));
#40998=CARTESIAN_POINT('Ctrl Pts',(-3.84848168092753,1.06847604194511,5.02346178870243));
#40999=CARTESIAN_POINT('Ctrl Pts',(-3.91621554992515,1.18514270861178,4.99623355742632));
#41000=CARTESIAN_POINT('Ctrl Pts',(-3.99529346323778,1.3,4.96307790506253));
#41001=CARTESIAN_POINT('Ctrl Pts',(-3.85507599179486,-1.3,4.7268753052437));
#41002=CARTESIAN_POINT('Ctrl Pts',(-3.78889068790036,-1.18514270861178,
4.78156123638215));
#41003=CARTESIAN_POINT('Ctrl Pts',(-3.73295432340165,-1.06847604194512,
4.82848789979372));
#41004=CARTESIAN_POINT('Ctrl Pts',(-3.62740723167583,-0.794772684000851,
4.91897241923607));
#41005=CARTESIAN_POINT('Ctrl Pts',(-3.58650774416313,-0.636309800095196,
4.95415127075708));
#41006=CARTESIAN_POINT('Ctrl Pts',(-3.5353568431438,-0.319434907277159,
5.00816436619335));
#41007=CARTESIAN_POINT('Ctrl Pts',(-3.52505210827391,-0.158333333333332,
5.02315921127615));
#41008=CARTESIAN_POINT('Ctrl Pts',(-3.53576509129248,0.158333333333334,
5.04063778675235));
#41009=CARTESIAN_POINT('Ctrl Pts',(-3.55620605750904,0.319434907277167,
5.04213862663277));
#41010=CARTESIAN_POINT('Ctrl Pts',(-3.630353335205,0.636309800095206,5.02573020814679));
#41011=CARTESIAN_POINT('Ctrl Pts',(-3.68274913399112,0.79477268400084,5.00946289323563));
#41012=CARTESIAN_POINT('Ctrl Pts',(-3.81258907846048,1.06847604194511,4.95873129561847));
#41013=CARTESIAN_POINT('Ctrl Pts',(-3.8798859495176,1.18514270861178,4.93037843917702));
#41014=CARTESIAN_POINT('Ctrl Pts',(-3.95827679071515,1.3,4.89563255511164));
#41015=CARTESIAN_POINT('Ctrl Pts',(-3.85507599179486,-1.3,4.7268753052437));
#41016=CARTESIAN_POINT('Ctrl Pts',(-3.78889068790036,-1.18514270861178,
4.78156123638215));
#41017=CARTESIAN_POINT('Ctrl Pts',(-3.73295432340165,-1.06847604194512,
4.82848789979373));
#41018=CARTESIAN_POINT('Ctrl Pts',(-3.62740723167583,-0.794772684000851,
4.91897241923607));
#41019=CARTESIAN_POINT('Ctrl Pts',(-3.58650774416314,-0.636309800095197,
4.95415127075708));
#41020=CARTESIAN_POINT('Ctrl Pts',(-3.5353568431438,-0.319434907277159,
5.00816436619336));
#41021=CARTESIAN_POINT('Ctrl Pts',(-3.52505210827391,-0.158333333333332,
5.02315921127615));
#41022=CARTESIAN_POINT('Ctrl Pts',(-3.53576509129248,0.158333333333334,
5.04063778675235));
#41023=CARTESIAN_POINT('Ctrl Pts',(-3.55620605750904,0.319434907277167,
5.04213862663277));
#41024=CARTESIAN_POINT('Ctrl Pts',(-3.630353335205,0.636309800095206,5.0257302081468));
#41025=CARTESIAN_POINT('Ctrl Pts',(-3.68274913399112,0.79477268400084,5.00946289323563));
#41026=CARTESIAN_POINT('Ctrl Pts',(-3.81258907846048,1.06847604194511,4.95873129561847));
#41027=CARTESIAN_POINT('Ctrl Pts',(-3.87988594951759,1.18514270861178,4.93037843917702));
#41028=CARTESIAN_POINT('Ctrl Pts',(-3.95827679071515,1.3,4.89563255511164));
#41029=CARTESIAN_POINT('Ctrl Pts',(-3.85507599179492,-1.30000000000009,
4.72687530524365));
#41030=CARTESIAN_POINT('Ctrl Pts',(-3.78889068790039,-1.18514270861184,
4.78156123638212));
#41031=CARTESIAN_POINT('Ctrl Pts',(-3.73295432340166,-1.06847604194515,
4.82848789979372));
#41032=CARTESIAN_POINT('Ctrl Pts',(-3.62740723167584,-0.794772684000851,
4.91897241923607));
#41033=CARTESIAN_POINT('Ctrl Pts',(-3.58650774416314,-0.636309800095197,
4.95415127075708));
#41034=CARTESIAN_POINT('Ctrl Pts',(-3.53535684314381,-0.319434907277159,
5.00816436619336));
#41035=CARTESIAN_POINT('Ctrl Pts',(-3.52505210827391,-0.158333333333332,
5.02315921127615));
#41036=CARTESIAN_POINT('Ctrl Pts',(-3.53576509129248,0.158333333333334,
5.04063778675235));
#41037=CARTESIAN_POINT('Ctrl Pts',(-3.55620605750904,0.319434907277167,
5.04213862663278));
#41038=CARTESIAN_POINT('Ctrl Pts',(-3.630353335205,0.636309800095206,5.0257302081468));
#41039=CARTESIAN_POINT('Ctrl Pts',(-3.68274913399112,0.79477268400084,5.00946289323563));
#41040=CARTESIAN_POINT('Ctrl Pts',(-3.81258907846121,1.06847604194665,4.95873129561818));
#41041=CARTESIAN_POINT('Ctrl Pts',(-3.87988594951935,1.18514270861482,4.93037843917628));
#41042=CARTESIAN_POINT('Ctrl Pts',(-3.95827679071822,1.30000000000449,4.89563255511028));
#41043=CARTESIAN_POINT('Ctrl Pts',(-3.85719962537667,-1.30000000000009,
4.72144101857419));
#41044=CARTESIAN_POINT('Ctrl Pts',(-3.79118274867503,-1.18514270861184,
4.77655201804504));
#41045=CARTESIAN_POINT('Ctrl Pts',(-3.73516370159793,-1.06847604194515,
4.82359200889143));
#41046=CARTESIAN_POINT('Ctrl Pts',(-3.62884548276946,-0.794772684000851,
4.91361815354223));
#41047=CARTESIAN_POINT('Ctrl Pts',(-3.58621520077171,-0.636309800095197,
4.94708737832572));
#41048=CARTESIAN_POINT('Ctrl Pts',(-3.53420574800354,-0.319434907277159,
5.00028383521863));
#41049=CARTESIAN_POINT('Ctrl Pts',(-3.52419820392418,-0.158333333333332,
5.01548821170247));
#41050=CARTESIAN_POINT('Ctrl Pts',(-3.53503780509133,0.158333333333334,
5.03306110286902));
#41051=CARTESIAN_POINT('Ctrl Pts',(-3.55544568808847,0.319434907277167,
5.03457304854717));
#41052=CARTESIAN_POINT('Ctrl Pts',(-3.63042937353099,0.636309800095206,
5.01891607505766));
#41053=CARTESIAN_POINT('Ctrl Pts',(-3.68405272961868,0.79477268400084,5.00383993978519));
#41054=CARTESIAN_POINT('Ctrl Pts',(-3.81472938980192,1.06847604194665,4.95364536025774));
#41055=CARTESIAN_POINT('Ctrl Pts',(-3.88225168770668,1.18514270861482,4.92533765577221));
#41056=CARTESIAN_POINT('Ctrl Pts',(-3.96073119936994,1.30000000000449,4.89044962038628));
#41057=CARTESIAN_POINT('Ctrl Pts',(-3.86187573129453,-1.30000000000009,
4.71383403293714));
#41058=CARTESIAN_POINT('Ctrl Pts',(-3.79719254535568,-1.18514270861185,
4.76895782901383));
#41059=CARTESIAN_POINT('Ctrl Pts',(-3.74183062561163,-1.06847604194515,
4.8157035538932));
#41060=CARTESIAN_POINT('Ctrl Pts',(-3.63546750551163,-0.794772684000853,
4.90434050932157));
#41061=CARTESIAN_POINT('Ctrl Pts',(-3.5900034586632,-0.636309800095197,
4.93531705592154));
#41062=CARTESIAN_POINT('Ctrl Pts',(-3.53661622228163,-0.319434907277158,
4.9872084206034));
#41063=CARTESIAN_POINT('Ctrl Pts',(-3.526536583893,-0.158333333333332,5.00288186391973));
#41064=CARTESIAN_POINT('Ctrl Pts',(-3.5375239175476,0.158333333333335,5.0205842461583));
#41065=CARTESIAN_POINT('Ctrl Pts',(-3.55824068036155,0.319434907277168,
5.02179590511999));
#41066=CARTESIAN_POINT('Ctrl Pts',(-3.63472167526744,0.636309800095207,
5.00762775887785));
#41067=CARTESIAN_POINT('Ctrl Pts',(-3.69099520684581,0.79477268400084,4.99509019029861));
#41068=CARTESIAN_POINT('Ctrl Pts',(-3.82174855505815,1.06847604194665,4.94631026905389));
#41069=CARTESIAN_POINT('Ctrl Pts',(-3.88865832024127,1.18514270861482,4.91828639197139));
#41070=CARTESIAN_POINT('Ctrl Pts',(-3.96587957105504,1.30000000000449,4.88335365823918));
#41071=CARTESIAN_POINT('Ctrl Pts',(-3.86961810893474,-1.30000000000009,
4.70440940889747));
#41072=CARTESIAN_POINT('Ctrl Pts',(-3.80754393917446,-1.18514270861185,
4.75854778066665));
#41073=CARTESIAN_POINT('Ctrl Pts',(-3.75381010225335,-1.06847604194515,
4.80426737477683));
#41074=CARTESIAN_POINT('Ctrl Pts',(-3.6489420268847,-0.794772684000851,
4.89043972278178));
#41075=CARTESIAN_POINT('Ctrl Pts',(-3.60079303589911,-0.636309800095196,
4.91916901559123));
#41076=CARTESIAN_POINT('Ctrl Pts',(-3.5460877997684,-0.319434907277158,
4.96957153261453));
#41077=CARTESIAN_POINT('Ctrl Pts',(-3.53514448494892,-0.158333333333332,
4.98573028016685));
#41078=CARTESIAN_POINT('Ctrl Pts',(-3.54619199064349,0.158333333333334,
5.00349880643113));
#41079=CARTESIAN_POINT('Ctrl Pts',(-3.56772207273765,0.319434907277168,
5.00409256128365));
#41080=CARTESIAN_POINT('Ctrl Pts',(-3.64586877350843,0.636309800095207,
4.99195282032989));
#41081=CARTESIAN_POINT('Ctrl Pts',(-3.70552748394763,0.794772684000839,
4.98285922822908));
#41082=CARTESIAN_POINT('Ctrl Pts',(-3.83480395680561,1.06847604194665,4.93653280029006));
#41083=CARTESIAN_POINT('Ctrl Pts',(-3.89992716386784,1.18514270861482,4.909242080837));
#41084=CARTESIAN_POINT('Ctrl Pts',(-3.97421458305709,1.30000000000449,4.8747136360225));
#41085=CARTESIAN_POINT('Ctrl Pts',(-3.87691755596594,-1.30000000000009,
4.69490664118848));
#41086=CARTESIAN_POINT('Ctrl Pts',(-3.81674813898273,-1.18514270861185,
4.74765414340193));
#41087=CARTESIAN_POINT('Ctrl Pts',(-3.76434400552701,-1.06847604194515,
4.79224680303008));
#41088=CARTESIAN_POINT('Ctrl Pts',(-3.66121933222148,-0.794772684000854,
4.87642544975936));
#41089=CARTESIAN_POINT('Ctrl Pts',(-3.61227744010187,-0.636309800095198,
4.90461839926761));
#41090=CARTESIAN_POINT('Ctrl Pts',(-3.55719693985597,-0.31943490727716,
4.95430228759037));
#41091=CARTESIAN_POINT('Ctrl Pts',(-3.54533126716359,-0.158333333333332,
4.97059092996656));
#41092=CARTESIAN_POINT('Ctrl Pts',(-3.55641159744232,0.158333333333335,
4.98842836728334));
#41093=CARTESIAN_POINT('Ctrl Pts',(-3.57877257621962,0.319434907277167,
4.98880961480654));
#41094=CARTESIAN_POINT('Ctrl Pts',(-3.65761456359265,0.636309800095207,
4.9778375119829));
#41095=CARTESIAN_POINT('Ctrl Pts',(-3.71873653204119,0.794772684000842,
4.97018331391904));
#41096=CARTESIAN_POINT('Ctrl Pts',(-3.84636899840465,1.06847604194666,4.9259261637555));
#41097=CARTESIAN_POINT('Ctrl Pts',(-3.91006561500535,1.18514270861482,4.89959200043321));
#41098=CARTESIAN_POINT('Ctrl Pts',(-3.98221148276658,1.3000000000045,4.86608095420555));
#41099=CARTESIAN_POINT('Ctrl Pts',(-3.88601526735229,-1.3000000000001,4.68298671678652));
#41100=CARTESIAN_POINT('Ctrl Pts',(-3.82789893469574,-1.18514270861185,
4.73382883581962));
#41101=CARTESIAN_POINT('Ctrl Pts',(-3.77707208302522,-1.06847604194515,
4.77714616311773));
#41102=CARTESIAN_POINT('Ctrl Pts',(-3.67649204712285,-0.794772684000852,
4.85983408054075));
#41103=CARTESIAN_POINT('Ctrl Pts',(-3.62803813052283,-0.636309800095198,
4.88966447649553));
#41104=CARTESIAN_POINT('Ctrl Pts',(-3.57285551823652,-0.319434907277159,
4.93918402311753));
#41105=CARTESIAN_POINT('Ctrl Pts',(-3.55916791444883,-0.158333333333333,
4.9546365788754));
#41106=CARTESIAN_POINT('Ctrl Pts',(-3.56990613195591,0.158333333333335,
4.97203904858936));
#41107=CARTESIAN_POINT('Ctrl Pts',(-3.59322204533834,0.319434907277168,
4.97211877620001));
#41108=CARTESIAN_POINT('Ctrl Pts',(-3.67253843601065,0.636309800095208,
4.96185624229368));
#41109=CARTESIAN_POINT('Ctrl Pts',(-3.73506171307405,0.794772684000842,
4.955175041043));
#41110=CARTESIAN_POINT('Ctrl Pts',(-3.86047195508732,1.06847604194666,4.91278091488119));
#41111=CARTESIAN_POINT('Ctrl Pts',(-3.92239820161952,1.18514270861482,4.88740444501922));
#41112=CARTESIAN_POINT('Ctrl Pts',(-3.99196524782343,1.3000000000045,4.85500235165368));
#41113=CARTESIAN_POINT('Ctrl Pts',(-3.89491361629381,-1.3000000000001,4.67070753187993));
#41114=CARTESIAN_POINT('Ctrl Pts',(-3.83893894854118,-1.18514270861185,
4.71945502898068));
#41115=CARTESIAN_POINT('Ctrl Pts',(-3.78979225765621,-1.06847604194515,
4.76138456315725));
#41116=CARTESIAN_POINT('Ctrl Pts',(-3.69202756244646,-0.794772684000855,
4.84249931679602));
#41117=CARTESIAN_POINT('Ctrl Pts',(-3.64419754857245,-0.636309800095201,
4.87401768374301));
#41118=CARTESIAN_POINT('Ctrl Pts',(-3.58939362681402,-0.319434907277161,
4.92386667443013));
#41119=CARTESIAN_POINT('Ctrl Pts',(-3.57413548094992,-0.158333333333333,
4.93886520909327));
#41120=CARTESIAN_POINT('Ctrl Pts',(-3.58534511953175,0.158333333333335,
4.95696636476547));
#41121=CARTESIAN_POINT('Ctrl Pts',(-3.61097395478874,0.319434907277168,
4.95861683227717));
#41122=CARTESIAN_POINT('Ctrl Pts',(-3.69031998230916,0.636309800095209,
4.94859652448346));
#41123=CARTESIAN_POINT('Ctrl Pts',(-3.75189333622018,0.794772684000847,
4.93969710293881));
#41124=CARTESIAN_POINT('Ctrl Pts',(-3.87425501353822,1.06847604194666,4.89845975445627));
#41125=CARTESIAN_POINT('Ctrl Pts',(-3.93437172036864,1.18514270861483,4.87424558338349));
#41126=CARTESIAN_POINT('Ctrl Pts',(-4.00163929786509,1.3000000000045,4.84366736140181));
#41127=CARTESIAN_POINT('Ctrl Pts',(-3.90299367365699,-1.3000000000001,4.65757823073421));
#41128=CARTESIAN_POINT('Ctrl Pts',(-3.84907963830677,-1.18514270861185,
4.7043243450785));
#41129=CARTESIAN_POINT('Ctrl Pts',(-3.80159394234937,-1.06847604194515,
4.74498916226841));
#41130=CARTESIAN_POINT('Ctrl Pts',(-3.70674323518918,-0.794772684000856,
4.82488401195993));
#41131=CARTESIAN_POINT('Ctrl Pts',(-3.65963597807638,-0.636309800095201,
4.85818914450328));
#41132=CARTESIAN_POINT('Ctrl Pts',(-3.60586222489922,-0.319434907277161,
4.90926246644672));
#41133=CARTESIAN_POINT('Ctrl Pts',(-3.59017934567842,-0.158333333333333,
4.92529238592121));
#41134=CARTESIAN_POINT('Ctrl Pts',(-3.60179395376847,0.158333333333335,
4.94401705810809));
#41135=CARTESIAN_POINT('Ctrl Pts',(-3.62840541558098,0.319434907277168,
4.94554572747288));
#41136=CARTESIAN_POINT('Ctrl Pts',(-3.70723467370267,0.636309800095209,
4.93498844237129));
#41137=CARTESIAN_POINT('Ctrl Pts',(-3.76801153668662,0.794772684000845,
4.92403147914096));
#41138=CARTESIAN_POINT('Ctrl Pts',(-3.88764112416407,1.06847604194666,4.88409836430707));
#41139=CARTESIAN_POINT('Ctrl Pts',(-3.9461792048465,1.18514270861483,4.86118862156217));
#41140=CARTESIAN_POINT('Ctrl Pts',(-4.01147215050509,1.3000000000045,4.83265470181636));
#41141=CARTESIAN_POINT('Ctrl Pts',(-3.90989779693675,-1.30000000000011,
4.64755288062261));
#41142=CARTESIAN_POINT('Ctrl Pts',(-3.85774919301543,-1.18514270861186,
4.6927615254062));
#41143=CARTESIAN_POINT('Ctrl Pts',(-3.81163105041348,-1.06847604194516,
4.73240221316335));
#41144=CARTESIAN_POINT('Ctrl Pts',(-3.71902048713749,-0.794772684000856,
4.81111703737771));
#41145=CARTESIAN_POINT('Ctrl Pts',(-3.67209309642864,-0.636309800095202,
4.84536348279141));
#41146=CARTESIAN_POINT('Ctrl Pts',(-3.61893232916747,-0.319434907277161,
4.89715154894492));
#41147=CARTESIAN_POINT('Ctrl Pts',(-3.60306622995126,-0.158333333333333,
4.91427581209853));
#41148=CARTESIAN_POINT('Ctrl Pts',(-3.61471415449658,0.158333333333336,
4.93306287156498));
#41149=CARTESIAN_POINT('Ctrl Pts',(-3.64145681552091,0.319434907277169,
4.93345505829791));
#41150=CARTESIAN_POINT('Ctrl Pts',(-3.71991477675818,0.636309800095211,
4.9225230197917));
#41151=CARTESIAN_POINT('Ctrl Pts',(-3.78099635420355,0.794772684000847,
4.91129657713904));
#41152=CARTESIAN_POINT('Ctrl Pts',(-3.89845061218902,1.06847604194666,4.87256374236237));
#41153=CARTESIAN_POINT('Ctrl Pts',(-3.95554548416997,1.18514270861483,4.85052729323673));
#41154=CARTESIAN_POINT('Ctrl Pts',(-4.01889363195879,1.3000000000045,4.82322040396743));
#41155=CARTESIAN_POINT('Ctrl Pts',(-3.92221206525848,-1.30000000000011,
4.63033050218808));
#41156=CARTESIAN_POINT('Ctrl Pts',(-3.8726683820101,-1.18514270861186,4.67235347215618));
#41157=CARTESIAN_POINT('Ctrl Pts',(-3.82860854712782,-1.06847604194516,
4.70985685555733));
#41158=CARTESIAN_POINT('Ctrl Pts',(-3.73949030117575,-0.794772684000857,
4.7860560246303));
#41159=CARTESIAN_POINT('Ctrl Pts',(-3.69315893855885,-0.636309800095202,
4.82223357701685));
#41160=CARTESIAN_POINT('Ctrl Pts',(-3.64107903602519,-0.319434907277161,
4.87522861122178));
#41161=CARTESIAN_POINT('Ctrl Pts',(-3.62459994389214,-0.158333333333333,
4.89377442775102));
#41162=CARTESIAN_POINT('Ctrl Pts',(-3.63685055307432,0.158333333333336,
4.91343611787957));
#41163=CARTESIAN_POINT('Ctrl Pts',(-3.66520128415716,0.31943490727717,4.91387516116949));
#41164=CARTESIAN_POINT('Ctrl Pts',(-3.74300673059837,0.636309800095211,
4.90230822867458));
#41165=CARTESIAN_POINT('Ctrl Pts',(-3.80286755801116,0.794772684000846,
4.88815756908362));
#41166=CARTESIAN_POINT('Ctrl Pts',(-3.91646823347156,1.06847604194666,4.85134128532008));
#41167=CARTESIAN_POINT('Ctrl Pts',(-3.97134781558832,1.18514270861483,4.83118714834847));
#41168=CARTESIAN_POINT('Ctrl Pts',(-4.03193345673457,1.30000000000451,4.80681527946886));
#41169=CARTESIAN_POINT('Ctrl Pts',(-3.93623661697016,-1.30000000000012,
4.60609932986889));
#41170=CARTESIAN_POINT('Ctrl Pts',(-3.88988848758903,-1.18514270861187,
4.64384498320135));
#41171=CARTESIAN_POINT('Ctrl Pts',(-3.84848197627912,-1.06847604194517,
4.67860153774707));
#41172=CARTESIAN_POINT('Ctrl Pts',(-3.76424077812082,-0.794772684000869,
4.75199071560809));
#41173=CARTESIAN_POINT('Ctrl Pts',(-3.71958858051035,-0.636309800095212,
4.79165991930544));
#41174=CARTESIAN_POINT('Ctrl Pts',(-3.66959157094361,-0.319434907277166,
4.84701784672139));
#41175=CARTESIAN_POINT('Ctrl Pts',(-3.65291612803299,-0.158333333333335,
4.8682313224775));
#41176=CARTESIAN_POINT('Ctrl Pts',(-3.66532599911306,0.158333333333338,
4.88814222567686));
#41177=CARTESIAN_POINT('Ctrl Pts',(-3.69367882888989,0.319434907277172,
4.88577252352626));
#41178=CARTESIAN_POINT('Ctrl Pts',(-3.77044586990941,0.636309800095218,
4.87314533844164));
#41179=CARTESIAN_POINT('Ctrl Pts',(-3.83063440064933,0.794772684000859,
4.85792393697454));
#41180=CARTESIAN_POINT('Ctrl Pts',(-3.93970515880007,1.06847604194668,4.82420737950992));
#41181=CARTESIAN_POINT('Ctrl Pts',(-3.99166519338934,1.18514270861485,4.80639044485926));
#41182=CARTESIAN_POINT('Ctrl Pts',(-4.048372572834,1.30000000000452,4.78535122396292));
#41183=CARTESIAN_POINT('Ctrl Pts',(-3.95284745610305,-1.30000000000013,
4.58042969910378));
#41184=CARTESIAN_POINT('Ctrl Pts',(-3.91072378417741,-1.18514270861188,
4.61419652857939));
#41185=CARTESIAN_POINT('Ctrl Pts',(-3.87246653076059,-1.06847604194518,
4.64611776351736));
#41186=CARTESIAN_POINT('Ctrl Pts',(-3.79301682226017,-0.794772684000873,
4.71559850945336));
#41187=CARTESIAN_POINT('Ctrl Pts',(-3.74773301943357,-0.636309800095213,
4.75619944846116));
#41188=CARTESIAN_POINT('Ctrl Pts',(-3.6987758134057,-0.319434907277167,
4.81258658242706));
#41189=CARTESIAN_POINT('Ctrl Pts',(-3.68181816367919,-0.158333333333336,
4.83651187898168));
#41190=CARTESIAN_POINT('Ctrl Pts',(-3.69492372703802,0.158333333333338,
4.85735934309548));
#41191=CARTESIAN_POINT('Ctrl Pts',(-3.72467603759297,0.319434907277175,
4.85379520621468));
#41192=CARTESIAN_POINT('Ctrl Pts',(-3.80096161861959,0.636309800095222,
4.84086342271053));
#41193=CARTESIAN_POINT('Ctrl Pts',(-3.86090246302895,0.79477268400086,4.8235616603301));
#41194=CARTESIAN_POINT('Ctrl Pts',(-3.9653366829377,1.06847604194668,4.79377615092503));
#41195=CARTESIAN_POINT('Ctrl Pts',(-4.01436420907048,1.18514270861485,4.77896071898002));
#41196=CARTESIAN_POINT('Ctrl Pts',(-4.06721355720645,1.30000000000453,4.76222289844965));
#41197=CARTESIAN_POINT('Ctrl Pts',(-3.96535170192484,-1.30000000000013,
4.5590274851764));
#41198=CARTESIAN_POINT('Ctrl Pts',(-3.92546910793081,-1.18514270861188,
4.58834962547774));
#41199=CARTESIAN_POINT('Ctrl Pts',(-3.88907325183375,-1.06847604194518,
4.61727115350065));
#41200=CARTESIAN_POINT('Ctrl Pts',(-3.81304660534494,-0.794772684000875,
4.68316017446002));
#41201=CARTESIAN_POINT('Ctrl Pts',(-3.76891047771894,-0.636309800095216,
4.726329929948));
#41202=CARTESIAN_POINT('Ctrl Pts',(-3.72148492134035,-0.319434907277169,
4.78428593600164));
#41203=CARTESIAN_POINT('Ctrl Pts',(-3.70435257527215,-0.158333333333337,
4.81042011216846));
#41204=CARTESIAN_POINT('Ctrl Pts',(-3.71797010330905,0.158333333333339,
4.83191259389462));
#41205=CARTESIAN_POINT('Ctrl Pts',(-3.7484901200146,0.319434907277175,4.82693408344865));
#41206=CARTESIAN_POINT('Ctrl Pts',(-3.82412180348236,0.636309800095224,
4.81344278511243));
#41207=CARTESIAN_POINT('Ctrl Pts',(-3.88373399482127,0.794772684000864,
4.79439433692748));
#41208=CARTESIAN_POINT('Ctrl Pts',(-3.98441581257107,1.06847604194669,4.76771271056547));
#41209=CARTESIAN_POINT('Ctrl Pts',(-4.03112104102182,1.18514270861486,4.75531895237286));
#41210=CARTESIAN_POINT('Ctrl Pts',(-4.08095006964814,1.30000000000453,4.74208092338814));
#41211=CARTESIAN_POINT('Ctrl Pts',(-3.97449901676934,-1.30000000000014,
4.54274237531137));
#41212=CARTESIAN_POINT('Ctrl Pts',(-3.93709157683421,-1.18514270861188,
4.56961294297179));
#41213=CARTESIAN_POINT('Ctrl Pts',(-3.90259013536087,-1.06847604194518,
4.59683916670406));
#41214=CARTESIAN_POINT('Ctrl Pts',(-3.8295983413575,-0.794772684000875,
4.6605588267877));
#41215=CARTESIAN_POINT('Ctrl Pts',(-3.78563727997431,-0.636309800095219,
4.70491822702643));
#41216=CARTESIAN_POINT('Ctrl Pts',(-3.73875498329855,-0.319434907277172,
4.76335431154097));
#41217=CARTESIAN_POINT('Ctrl Pts',(-3.72082588163312,-0.158333333333338,
4.7903395778526));
#41218=CARTESIAN_POINT('Ctrl Pts',(-3.73460539730176,0.15833333333334,4.81205747381827));
#41219=CARTESIAN_POINT('Ctrl Pts',(-3.76596561796686,0.319434907277177,
4.80633812157363));
#41220=CARTESIAN_POINT('Ctrl Pts',(-3.84162545483092,0.636309800095228,
4.79306048198457));
#41221=CARTESIAN_POINT('Ctrl Pts',(-3.9017991424465,0.794772684000869,4.77368450597758));
#41222=CARTESIAN_POINT('Ctrl Pts',(-3.99984738133293,1.06847604194669,4.74955254208256));
#41223=CARTESIAN_POINT('Ctrl Pts',(-4.0447207637576,1.18514270861486,4.73886648778137));
#41224=CARTESIAN_POINT('Ctrl Pts',(-4.09202607903803,1.30000000000454,4.72794021217183));
#41225=CARTESIAN_POINT('Ctrl Pts',(-3.98365558285505,-1.30000000000014,
4.52648867384936));
#41226=CARTESIAN_POINT('Ctrl Pts',(-3.94802546111216,-1.18514270861189,
4.55015011718819));
#41227=CARTESIAN_POINT('Ctrl Pts',(-3.91493284176103,-1.06847604194519,
4.57514792636692));
#41228=CARTESIAN_POINT('Ctrl Pts',(-3.84434440905465,-0.79477268400088,
4.63598513879361));
#41229=CARTESIAN_POINT('Ctrl Pts',(-3.80070404932378,-0.636309800095222,
4.68163239936094));
#41230=CARTESIAN_POINT('Ctrl Pts',(-3.7548189954872,-0.319434907277172,
4.74103728856512));
#41231=CARTESIAN_POINT('Ctrl Pts',(-3.73701840812171,-0.158333333333338,
4.76994052592333));
#41232=CARTESIAN_POINT('Ctrl Pts',(-3.75125591399722,0.15833333333334,4.79220492185405));
#41233=CARTESIAN_POINT('Ctrl Pts',(-3.78319980310662,0.319434907277177,
4.78544165923762));
#41234=CARTESIAN_POINT('Ctrl Pts',(-3.85827751831032,0.636309800095229,
4.77164117845782));
#41235=CARTESIAN_POINT('Ctrl Pts',(-3.91787090844986,0.794772684000871,
4.75057341116541));
#41236=CARTESIAN_POINT('Ctrl Pts',(-4.01327299532946,1.0684760419467,4.72897368026303));
#41237=CARTESIAN_POINT('Ctrl Pts',(-4.0565883586806,1.18514270861487,4.72032166145382));
#41238=CARTESIAN_POINT('Ctrl Pts',(-4.10192305696814,1.30000000000455,4.71236734699421));
#41239=CARTESIAN_POINT('Ctrl Pts',(-3.99622589356072,-1.30000000000016,
4.50522626952481));
#41240=CARTESIAN_POINT('Ctrl Pts',(-3.96314346622973,-1.1851427086119,4.52480713643115));
#41241=CARTESIAN_POINT('Ctrl Pts',(-3.93206737704905,-1.0684760419452,4.54698942543475));
#41242=CARTESIAN_POINT('Ctrl Pts',(-3.86491043678513,-0.79477268400089,
4.6042447560422));
#41243=CARTESIAN_POINT('Ctrl Pts',(-3.82191124009897,-0.636309800095231,
4.65186512030542));
#41244=CARTESIAN_POINT('Ctrl Pts',(-3.77703914577215,-0.319434907277177,
4.71221083099536));
#41245=CARTESIAN_POINT('Ctrl Pts',(-3.75874478410963,-0.15833333333334,
4.74291980786877));
#41246=CARTESIAN_POINT('Ctrl Pts',(-3.77306480043963,0.158333333333343,
4.76531045862233));
#41247=CARTESIAN_POINT('Ctrl Pts',(-3.80530761257115,0.319434907277183,
4.75658141089551));
#41248=CARTESIAN_POINT('Ctrl Pts',(-3.88010540199207,0.636309800095239,
4.74268045395068));
#41249=CARTESIAN_POINT('Ctrl Pts',(-3.94055736214315,0.794772684000886,
4.72130122573096));
#41250=CARTESIAN_POINT('Ctrl Pts',(-4.0327770399233,1.06847604194671,4.70349046048285));
#41251=CARTESIAN_POINT('Ctrl Pts',(-4.07387487551302,1.18514270861488,4.6973834864128));
#41252=CARTESIAN_POINT('Ctrl Pts',(-4.11615206525699,1.30000000000456,4.69287915859477));
#41253=CARTESIAN_POINT('Ctrl Pts',(-4.01031583526455,-1.30000000000017,
4.47694433028216));
#41254=CARTESIAN_POINT('Ctrl Pts',(-3.98029476906993,-1.18514270861191,
4.49132307749177));
#41255=CARTESIAN_POINT('Ctrl Pts',(-3.95161936908155,-1.06847604194521,
4.50987032045911));
#41256=CARTESIAN_POINT('Ctrl Pts',(-3.88848221675032,-0.794772684000896,
4.56234822118198));
#41257=CARTESIAN_POINT('Ctrl Pts',(-3.84583979836555,-0.636309800095234,
4.61188462104922));
#41258=CARTESIAN_POINT('Ctrl Pts',(-3.80253997352847,-0.319434907277178,
4.67367470421467));
#41259=CARTESIAN_POINT('Ctrl Pts',(-3.78430984984646,-0.158333333333341,
4.70731587685121));
#41260=CARTESIAN_POINT('Ctrl Pts',(-3.79966229070426,0.158333333333344,
4.73088970509215));
#41261=CARTESIAN_POINT('Ctrl Pts',(-3.83342601590674,0.319434907277185,
4.72108767838593));
#41262=CARTESIAN_POINT('Ctrl Pts',(-3.90762864613288,0.636309800095243,
4.70677535294558));
#41263=CARTESIAN_POINT('Ctrl Pts',(-3.96698159486524,0.794772684000887,
4.68245666916534));
#41264=CARTESIAN_POINT('Ctrl Pts',(-4.05510064076927,1.06847604194672,4.66923727521721));
#41265=CARTESIAN_POINT('Ctrl Pts',(-4.09379252591144,1.18514270861489,4.66674044423394));
#41266=CARTESIAN_POINT('Ctrl Pts',(-4.13303282635611,1.30000000000457,4.66746896808078));
#41267=CARTESIAN_POINT('Ctrl Pts',(-4.02533150000358,-1.30000000000019,
4.44972631117233));
#41268=CARTESIAN_POINT('Ctrl Pts',(-3.99818829069229,-1.18514270861194,
4.45873161766262));
#41269=CARTESIAN_POINT('Ctrl Pts',(-3.97173680431925,-1.06847604194523,
4.47346910582672));
#41270=CARTESIAN_POINT('Ctrl Pts',(-3.91222659756186,-0.794772684000915,
4.52075813809573));
#41271=CARTESIAN_POINT('Ctrl Pts',(-3.86967653948471,-0.636309800095248,
4.57189844720796));
#41272=CARTESIAN_POINT('Ctrl Pts',(-3.82766115997983,-0.319434907277185,
4.63479501999804));
#41273=CARTESIAN_POINT('Ctrl Pts',(-3.80975372220844,-0.158333333333345,
4.67164424552778));
#41274=CARTESIAN_POINT('Ctrl Pts',(-3.82541765453887,0.158333333333347,
4.69556075515344));
#41275=CARTESIAN_POINT('Ctrl Pts',(-3.85900783513208,0.319434907277191,
4.68273321963391));
#41276=CARTESIAN_POINT('Ctrl Pts',(-3.93289120133694,0.636309800095256,
4.66833861003533));
#41277=CARTESIAN_POINT('Ctrl Pts',(-3.9936989809741,0.794772684000906,4.64407164915053));
#41278=CARTESIAN_POINT('Ctrl Pts',(-4.07811909590979,1.06847604194674,4.63587130536479));
#41279=CARTESIAN_POINT('Ctrl Pts',(-4.11414421160011,1.18514270861491,4.63665058559084));
#41280=CARTESIAN_POINT('Ctrl Pts',(-4.14965210329837,1.30000000000459,4.64175877101514));
#41281=CARTESIAN_POINT('Ctrl Pts',(-4.0360507106705,-1.30000000000021,4.42659910168526));
#41282=CARTESIAN_POINT('Ctrl Pts',(-4.01146896352685,-1.18514270861195,
4.43159793854085));
#41283=CARTESIAN_POINT('Ctrl Pts',(-3.98697845367857,-1.06847604194524,
4.4434927580042));
#41284=CARTESIAN_POINT('Ctrl Pts',(-3.93061125302358,-0.794772684000924,
4.48690326987556));
#41285=CARTESIAN_POINT('Ctrl Pts',(-3.88813086765443,-0.636309800095255,
4.53933364653334));
#41286=CARTESIAN_POINT('Ctrl Pts',(-3.84690700499389,-0.319434907277188,
4.60282749835033));
#41287=CARTESIAN_POINT('Ctrl Pts',(-3.82843070636847,-0.158333333333347,
4.64126716597781));
#41288=CARTESIAN_POINT('Ctrl Pts',(-3.84484044798012,0.158333333333349,
4.66599872978517));
#41289=CARTESIAN_POINT('Ctrl Pts',(-3.8802125113638,0.319434907277196,4.65293701987225));
#41290=CARTESIAN_POINT('Ctrl Pts',(-3.95387184199184,0.636309800095264,
4.63850292495207));
#41291=CARTESIAN_POINT('Ctrl Pts',(-4.01366771231441,0.794772684000916,
4.61179490949894));
#41292=CARTESIAN_POINT('Ctrl Pts',(-4.09496763252197,1.06847604194675,4.60742569516046));
#41293=CARTESIAN_POINT('Ctrl Pts',(-4.12917353775639,1.18514270861492,4.61118505258874));
#41294=CARTESIAN_POINT('Ctrl Pts',(-4.16239362522605,1.3000000000046,4.6205950384371));
#41295=CARTESIAN_POINT('Ctrl Pts',(-4.04477970179641,-1.30000000000023,
4.41003624342554));
#41296=CARTESIAN_POINT('Ctrl Pts',(-4.02136831371039,-1.18514270861197,
4.41125620031957));
#41297=CARTESIAN_POINT('Ctrl Pts',(-3.99789837729298,-1.06847604194526,
4.42055226385903));
#41298=CARTESIAN_POINT('Ctrl Pts',(-3.94354287066604,-0.794772684000933,
4.46068545227691));
#41299=CARTESIAN_POINT('Ctrl Pts',(-3.90219970141365,-0.636309800095262,
4.51518220755499));
#41300=CARTESIAN_POINT('Ctrl Pts',(-3.86170898623137,-0.319434907277191,
4.57925305208586));
#41301=CARTESIAN_POINT('Ctrl Pts',(-3.84262697093746,-0.158333333333348,
4.61872494239754));
#41302=CARTESIAN_POINT('Ctrl Pts',(-3.85883879658361,0.158333333333351,
4.64323152261604));
#41303=CARTESIAN_POINT('Ctrl Pts',(-3.89409505320355,0.319434907277199,
4.62836362481254));
#41304=CARTESIAN_POINT('Ctrl Pts',(-3.96768464649077,0.636309800095271,
4.6140124978342));
#41305=CARTESIAN_POINT('Ctrl Pts',(-4.02858131432634,0.794772684000922,
4.58756582937971));
#41306=CARTESIAN_POINT('Ctrl Pts',(-4.10809241924047,1.06847604194676,4.58667675920439));
#41307=CARTESIAN_POINT('Ctrl Pts',(-4.14092316209739,1.18514270861494,4.59265010414313));
#41308=CARTESIAN_POINT('Ctrl Pts',(-4.17216723667044,1.30000000000462,4.60498163955622));
#41309=CARTESIAN_POINT('Ctrl Pts',(-4.05315766169742,-1.30000000000024,
4.39308255428406));
#41310=CARTESIAN_POINT('Ctrl Pts',(-4.03176153817544,-1.18514270861198,
4.3914028397508));
#41311=CARTESIAN_POINT('Ctrl Pts',(-4.00973387879023,-1.06847604194527,
4.39854270840336));
#41312=CARTESIAN_POINT('Ctrl Pts',(-3.95738660480989,-0.794772684000944,
4.43541223482741));
#41313=CARTESIAN_POINT('Ctrl Pts',(-3.91512622505095,-0.636309800095271,
4.48986981328023));
#41314=CARTESIAN_POINT('Ctrl Pts',(-3.87511537833164,-0.319434907277196,
4.55426694040123));
#41315=CARTESIAN_POINT('Ctrl Pts',(-3.85635181656492,-0.158333333333351,
4.59570057419642));
#41316=CARTESIAN_POINT('Ctrl Pts',(-3.87336540944652,0.158333333333353,
4.62105810311818));
#41317=CARTESIAN_POINT('Ctrl Pts',(-3.90969641020897,0.319434907277205,
4.60572169867666));
#41318=CARTESIAN_POINT('Ctrl Pts',(-3.98323457595251,0.636309800095281,
4.59146931564705));
#41319=CARTESIAN_POINT('Ctrl Pts',(-4.04374029903339,0.794772684000934,
4.56362142462193));
#41320=CARTESIAN_POINT('Ctrl Pts',(-4.12095507618445,1.06847604194678,4.565645711017));
#41321=CARTESIAN_POINT('Ctrl Pts',(-4.15236704819326,1.18514270861496,4.57378414311225));
#41322=CARTESIAN_POINT('Ctrl Pts',(-4.18176757627142,1.30000000000464,4.58918476872954));
#41323=CARTESIAN_POINT('Ctrl Pts',(-4.05971024575106,-1.30000000000026,
4.37855021491459));
#41324=CARTESIAN_POINT('Ctrl Pts',(-4.03944010098985,-1.185142708612,4.37390448857528));
#41325=CARTESIAN_POINT('Ctrl Pts',(-4.01834201970723,-1.06847604194529,
4.37897822127184));
#41326=CARTESIAN_POINT('Ctrl Pts',(-3.96768853229509,-0.794772684000953,
4.41315345354163));
#41327=CARTESIAN_POINT('Ctrl Pts',(-3.92596056098777,-0.636309800095277,
4.46888157145737));
#41328=CARTESIAN_POINT('Ctrl Pts',(-3.88669101787428,-0.319434907277199,
4.53388301937142));
#41329=CARTESIAN_POINT('Ctrl Pts',(-3.86791555360218,-0.158333333333352,
4.5766746106872));
#41330=CARTESIAN_POINT('Ctrl Pts',(-3.88503542645838,0.158333333333355,
4.60212638313186));
#41331=CARTESIAN_POINT('Ctrl Pts',(-3.92138353528705,0.319434907277208,
4.58543081985728));
#41332=CARTESIAN_POINT('Ctrl Pts',(-3.99460276338386,0.636309800095287,
4.57096049756234));
#41333=CARTESIAN_POINT('Ctrl Pts',(-4.05521956108513,0.794772684000941,
4.54243681909545));
#41334=CARTESIAN_POINT('Ctrl Pts',(-4.13093904277844,1.06847604194679,4.54734319695209));
#41335=CARTESIAN_POINT('Ctrl Pts',(-4.16138437224898,1.18514270861497,4.55751673590934));
#41336=CARTESIAN_POINT('Ctrl Pts',(-4.18949887324812,1.30000000000466,4.57574002464891));
#41337=CARTESIAN_POINT('Ctrl Pts',(-4.06445732467908,-1.30000000000026,
4.36854383193775));
#41338=CARTESIAN_POINT('Ctrl Pts',(-4.04514166945636,-1.185142708612,4.3619891298598));
#41339=CARTESIAN_POINT('Ctrl Pts',(-4.02476778473141,-1.06847604194529,
4.36569082763837));
#41340=CARTESIAN_POINT('Ctrl Pts',(-3.97525531338687,-0.794772684000957,
4.3979368254833));
#41341=CARTESIAN_POINT('Ctrl Pts',(-3.93341152373033,-0.636309800095281,
4.45406514905449));
#41342=CARTESIAN_POINT('Ctrl Pts',(-3.89458212873724,-0.319434907277201,
4.51941368543153));
#41343=CARTESIAN_POINT('Ctrl Pts',(-3.8760499641768,-0.158333333333353,
4.56340730429001));
#41344=CARTESIAN_POINT('Ctrl Pts',(-3.89339287804238,0.158333333333355,
4.58908470969992));
#41345=CARTESIAN_POINT('Ctrl Pts',(-3.92985203416142,0.31943490727721,4.57155721434891));
#41346=CARTESIAN_POINT('Ctrl Pts',(-4.00281797176179,0.636309800095291,
4.55690514198218));
#41347=CARTESIAN_POINT('Ctrl Pts',(-4.06330625342903,0.794772684000946,
4.52768205603544));
#41348=CARTESIAN_POINT('Ctrl Pts',(-4.13790416980033,1.06847604194679,4.53452040294592));
#41349=CARTESIAN_POINT('Ctrl Pts',(-4.16766698018009,1.18514270861497,4.54610951803909));
#41350=CARTESIAN_POINT('Ctrl Pts',(-4.19490192706749,1.30000000000466,4.5663276812336));
#41351=CARTESIAN_POINT('Ctrl Pts',(-4.06705508691299,-1.30000000000026,
4.36271599905377));
#41352=CARTESIAN_POINT('Ctrl Pts',(-4.04819781681766,-1.185142708612,4.35498856748228));
#41353=CARTESIAN_POINT('Ctrl Pts',(-4.02819820124502,-1.06847604194529,
4.35786950352306));
#41354=CARTESIAN_POINT('Ctrl Pts',(-3.97935604178485,-0.794772684000958,
4.38903249348759));
#41355=CARTESIAN_POINT('Ctrl Pts',(-3.93770563105166,-0.636309800095281,
4.44564169612304));
#41356=CARTESIAN_POINT('Ctrl Pts',(-3.89913897665286,-0.319434907277201,
4.51119311873859));
#41357=CARTESIAN_POINT('Ctrl Pts',(-3.88051985306727,-0.158333333333353,
4.55564108778732));
#41358=CARTESIAN_POINT('Ctrl Pts',(-3.89798339080602,0.158333333333356,
4.58144045044047));
#41359=CARTESIAN_POINT('Ctrl Pts',(-3.93464408535983,0.31943490727721,4.56358073874647));
#41360=CARTESIAN_POINT('Ctrl Pts',(-4.00760529664738,0.636309800095291,
4.54897383853482));
#41361=CARTESIAN_POINT('Ctrl Pts',(-4.06817540954463,0.794772684000946,
4.51952082489925));
#41362=CARTESIAN_POINT('Ctrl Pts',(-4.14211531990086,1.06847604194679,4.52744400370944));
#41363=CARTESIAN_POINT('Ctrl Pts',(-4.17143295339994,1.18514270861497,4.53978182164816));
#41364=CARTESIAN_POINT('Ctrl Pts',(-4.19806237294838,1.30000000000466,4.56102780700135));
#41365=CARTESIAN_POINT('Ctrl Pts',(-4.06960995733231,-1.30000000000027,
4.35684872627253));
#41366=CARTESIAN_POINT('Ctrl Pts',(-4.05116147748774,-1.185142708612,4.34790089113822));
#41367=CARTESIAN_POINT('Ctrl Pts',(-4.03151088950341,-1.06847604194529,
4.34993686239268));
#41368=CARTESIAN_POINT('Ctrl Pts',(-3.98333698988926,-0.794772684000959,
4.38001515334615));
#41369=CARTESIAN_POINT('Ctrl Pts',(-3.9419995353561,-0.636309800095282,
4.43722225727209));
#41370=CARTESIAN_POINT('Ctrl Pts',(-3.90370251970226,-0.319434907277201,
4.50298036197511));
#41371=CARTESIAN_POINT('Ctrl Pts',(-3.88490128407447,-0.158333333333353,
4.54778387694354));
#41372=CARTESIAN_POINT('Ctrl Pts',(-3.90248210251331,0.158333333333356,
4.57370156077579));
#41373=CARTESIAN_POINT('Ctrl Pts',(-3.93940097966221,0.319434907277211,
4.55556904755597));
#41374=CARTESIAN_POINT('Ctrl Pts',(-4.01241538664902,0.636309800095292,
4.54106894432917));
#41375=CARTESIAN_POINT('Ctrl Pts',(-4.07312995568607,0.794772684000947,
4.51145405644919));
#41376=CARTESIAN_POINT('Ctrl Pts',(-4.14640902016603,1.0684760419468,4.52045822043791));
#41377=CARTESIAN_POINT('Ctrl Pts',(-4.17526173596065,1.18514270861498,4.53352292266838));
#41378=CARTESIAN_POINT('Ctrl Pts',(-4.20124737579323,1.30000000000467,4.55575475817572));
#41379=CARTESIAN_POINT('Ctrl Pts',(-4.07182740503528,-1.30000000000027,
4.35169963014855));
#41380=CARTESIAN_POINT('Ctrl Pts',(-4.05371561684914,-1.18514270861201,
4.34166407547363));
#41381=CARTESIAN_POINT('Ctrl Pts',(-4.03435707227047,-1.0684760419453,4.34294808869059));
#41382=CARTESIAN_POINT('Ctrl Pts',(-3.98675470495063,-0.794772684000962,
4.37206488238973));
#41383=CARTESIAN_POINT('Ctrl Pts',(-3.94571668949595,-0.636309800095284,
4.42982081128793));
#41384=CARTESIAN_POINT('Ctrl Pts',(-3.90765324417452,-0.319434907277203,
4.49575512646909));
#41385=CARTESIAN_POINT('Ctrl Pts',(-3.88867494866334,-0.158333333333354,
4.54084804338412));
#41386=CARTESIAN_POINT('Ctrl Pts',(-3.90635099096263,0.158333333333356,
4.56686010837275));
#41387=CARTESIAN_POINT('Ctrl Pts',(-3.94349412896054,0.319434907277212,
4.54848825366666));
#41388=CARTESIAN_POINT('Ctrl Pts',(-4.01656674894129,0.636309800095295,
4.53409446564822));
#41389=CARTESIAN_POINT('Ctrl Pts',(-4.07742558185216,0.79477268400095,4.504357605896));
#41390=CARTESIAN_POINT('Ctrl Pts',(-4.15014770605485,1.0684760419468,4.51432989344033));
#41391=CARTESIAN_POINT('Ctrl Pts',(-4.17860290790803,1.18514270861498,4.52804006765191));
#41392=CARTESIAN_POINT('Ctrl Pts',(-4.20403459866709,1.30000000000467,4.55114378230678));
#41393=CARTESIAN_POINT('Ctrl Pts',(-4.07378205567366,-1.30000000000027,
4.34733952649448));
#41394=CARTESIAN_POINT('Ctrl Pts',(-4.05601587975433,-1.18514270861201,
4.33642721040689));
#41395=CARTESIAN_POINT('Ctrl Pts',(-4.03693065025124,-1.0684760419453,4.33708909914715));
#41396=CARTESIAN_POINT('Ctrl Pts',(-3.98979267445783,-0.794772684000963,
4.36535692311163));
#41397=CARTESIAN_POINT('Ctrl Pts',(-3.94881824813616,-0.636309800095285,
4.4233944643206));
#41398=CARTESIAN_POINT('Ctrl Pts',(-3.91093324152037,-0.319434907277203,
4.48945994370647));
#41399=CARTESIAN_POINT('Ctrl Pts',(-3.89195250433436,-0.158333333333354,
4.5349504853283));
#41400=CARTESIAN_POINT('Ctrl Pts',(-3.90971358737913,0.158333333333357,
4.56104504815378));
#41401=CARTESIAN_POINT('Ctrl Pts',(-3.94695751173222,0.319434907277212,
4.54237412458506));
#41402=CARTESIAN_POINT('Ctrl Pts',(-4.01999781572536,0.636309800095296,
4.52798450551081));
#41403=CARTESIAN_POINT('Ctrl Pts',(-4.08088588357391,0.794772684000951,
4.49804108521699));
#41404=CARTESIAN_POINT('Ctrl Pts',(-4.15316659797322,1.0684760419468,4.50888162745255));
#41405=CARTESIAN_POINT('Ctrl Pts',(-4.1813310257165,1.18514270861498,4.52319857025606));
#41406=CARTESIAN_POINT('Ctrl Pts',(-4.2063722382038,1.30000000000467,4.54713998681093));
#41407=CARTESIAN_POINT('Ctrl Pts',(-4.07476796326869,-1.30000000000027,
4.34516801520838));
#41408=CARTESIAN_POINT('Ctrl Pts',(-4.0571842873435,-1.18514270861201,4.33382683689759));
#41409=CARTESIAN_POINT('Ctrl Pts',(-4.03823961387944,-1.0684760419453,4.33418150808252));
#41410=CARTESIAN_POINT('Ctrl Pts',(-3.99132945172717,-0.794772684000963,
4.36202062155324));
#41411=CARTESIAN_POINT('Ctrl Pts',(-3.95035421507057,-0.636309800095285,
4.42016702771697));
#41412=CARTESIAN_POINT('Ctrl Pts',(-3.91255408456978,-0.319434907277203,
4.48629402063484));
#41413=CARTESIAN_POINT('Ctrl Pts',(-3.89359611246056,-0.158333333333354,
4.53200735080797));
#41414=CARTESIAN_POINT('Ctrl Pts',(-3.91140026048978,0.158333333333357,
4.55814338650856));
#41415=CARTESIAN_POINT('Ctrl Pts',(-3.94868044270104,0.319434907277212,
4.53930842922341));
#41416=CARTESIAN_POINT('Ctrl Pts',(-4.02169108565547,0.636309800095296,
4.52490657176991));
#41417=CARTESIAN_POINT('Ctrl Pts',(-4.08257726430552,0.794772684000951,
4.49484203590736));
#41418=CARTESIAN_POINT('Ctrl Pts',(-4.15464328483979,1.0684760419468,4.50612305542115));
#41419=CARTESIAN_POINT('Ctrl Pts',(-4.18267079146387,1.18514270861498,4.5207524088254));
#41420=CARTESIAN_POINT('Ctrl Pts',(-4.20753109473177,1.30000000000467,4.54512798028933));
#41421=CARTESIAN_POINT('Ctrl Pts',(-4.0755963351847,-1.30000000000027,4.343365203512));
#41422=CARTESIAN_POINT('Ctrl Pts',(-4.05817216723079,-1.18514270861201,
4.33167394277198));
#41423=CARTESIAN_POINT('Ctrl Pts',(-4.03934756240527,-1.0684760419453,4.33177550395673));
#41424=CARTESIAN_POINT('Ctrl Pts',(-3.99262367007915,-0.794772684000964,
4.35925390840294));
#41425=CARTESIAN_POINT('Ctrl Pts',(-3.95162253941972,-0.636309800095286,
4.4174663035074));
#41426=CARTESIAN_POINT('Ctrl Pts',(-3.91388933069293,-0.319434907277203,
4.48364095991923));
#41427=CARTESIAN_POINT('Ctrl Pts',(-3.89496806491384,-0.158333333333354,
4.52955769033492));
#41428=CARTESIAN_POINT('Ctrl Pts',(-3.91280861896672,0.158333333333357,
4.55572856504316));
#41429=CARTESIAN_POINT('Ctrl Pts',(-3.95010917144022,0.319434907277213,
4.53674679937419));
#41430=CARTESIAN_POINT('Ctrl Pts',(-4.02308494460944,0.636309800095296,
4.52232393398548));
#41431=CARTESIAN_POINT('Ctrl Pts',(-4.08395642161417,0.794772684000952,
4.49214430080419));
#41432=CARTESIAN_POINT('Ctrl Pts',(-4.15584772598368,1.0684760419468,4.50379674968262));
#41433=CARTESIAN_POINT('Ctrl Pts',(-4.18376742435588,1.18514270861498,4.51869311565342));
#41434=CARTESIAN_POINT('Ctrl Pts',(-4.20848773927385,1.30000000000467,4.54344193424129));
#41435=CARTESIAN_POINT('Ctrl Pts',(-4.07617844698269,-1.30000000000027,
4.34210553749473));
#41436=CARTESIAN_POINT('Ctrl Pts',(-4.05886853271517,-1.18514270861201,
4.33017180869061));
#41437=CARTESIAN_POINT('Ctrl Pts',(-4.04012894708355,-1.0684760419453,4.33009717417551));
#41438=CARTESIAN_POINT('Ctrl Pts',(-3.99353392857743,-0.794772684000964,
4.35732163372633));
#41439=CARTESIAN_POINT('Ctrl Pts',(-3.95250552735942,-0.636309800095285,
4.41557122350499));
#41440=CARTESIAN_POINT('Ctrl Pts',(-3.91481729305289,-0.319434907277203,
4.48177742096665));
#41441=CARTESIAN_POINT('Ctrl Pts',(-3.89592732961037,-0.158333333333354,
4.52784211054421));
#41442=CARTESIAN_POINT('Ctrl Pts',(-3.91379354357892,0.158333333333357,
4.5540374451459));
#41443=CARTESIAN_POINT('Ctrl Pts',(-3.95110567192063,0.319434907277212,
4.53495015271741));
#41444=CARTESIAN_POINT('Ctrl Pts',(-4.02405366565505,0.636309800095296,
4.52050896061406));
#41445=CARTESIAN_POINT('Ctrl Pts',(-4.08490984854949,0.794772684000951,
4.49024337789042));
#41446=CARTESIAN_POINT('Ctrl Pts',(-4.15668026845033,1.0684760419468,4.50215724002482));
#41447=CARTESIAN_POINT('Ctrl Pts',(-4.18452673106562,1.18514270861498,4.51724284036248));
#41448=CARTESIAN_POINT('Ctrl Pts',(-4.20915290087706,1.30000000000467,4.54225697157188));
#41449=CARTESIAN_POINT('Ctrl Pts',(-4.07651119518558,-1.30000000000027,
4.34138587295175));
#41450=CARTESIAN_POINT('Ctrl Pts',(-4.05926672083395,-1.18514270861201,
4.32931375912153));
#41451=CARTESIAN_POINT('Ctrl Pts',(-4.04057572742151,-1.0684760419453,4.32913846182814));
#41452=CARTESIAN_POINT('Ctrl Pts',(-3.99405404511275,-0.794772684000964,
4.35621751616241));
#41453=CARTESIAN_POINT('Ctrl Pts',(-3.95300924305191,-0.636309800095286,
4.41448753386619));
#41454=CARTESIAN_POINT('Ctrl Pts',(-3.91534619356815,-0.319434907277203,
4.48071122904653));
#41455=CARTESIAN_POINT('Ctrl Pts',(-3.8964740374384,-0.158333333333354,
4.52686037862302));
#41456=CARTESIAN_POINT('Ctrl Pts',(-3.91435493136644,0.158333333333357,
4.55306968517405));
#41457=CARTESIAN_POINT('Ctrl Pts',(-3.95167403545791,0.319434907277213,
4.53392243415286));
#41458=CARTESIAN_POINT('Ctrl Pts',(-4.02460616709662,0.636309800095296,
4.51947075644012));
#41459=CARTESIAN_POINT('Ctrl Pts',(-4.08545325821297,0.794772684000952,
4.48915571499051));
#41460=CARTESIAN_POINT('Ctrl Pts',(-4.15715456522845,1.0684760419468,4.50121887134314));
#41461=CARTESIAN_POINT('Ctrl Pts',(-4.18495922253128,1.18514270861498,4.51641261846914));
#41462=CARTESIAN_POINT('Ctrl Pts',(-4.20953169812499,1.30000000000467,4.54157841932003));
#41463=CARTESIAN_POINT('Ctrl Pts',(-4.0806826240262,-1.30000000000026,4.33240215395594));
#41464=CARTESIAN_POINT('Ctrl Pts',(-4.0642693119333,-1.185142708612,4.31861318319468));
#41465=CARTESIAN_POINT('Ctrl Pts',(-4.04619118718315,-1.06847604194529,
4.31718503134182));
#41466=CARTESIAN_POINT('Ctrl Pts',(-4.00058105221098,-0.794772684000956,
4.34244167931267));
#41467=CARTESIAN_POINT('Ctrl Pts',(-3.95928783985939,-0.63630980009528,
4.40092469193015));
#41468=CARTESIAN_POINT('Ctrl Pts',(-3.9219354987454,-0.3194349072772,4.46736338887183));
#41469=CARTESIAN_POINT('Ctrl Pts',(-3.90332070102475,-0.158333333333353,
4.51460279714578));
#41470=CARTESIAN_POINT('Ctrl Pts',(-3.92138590261326,0.158333333333355,
4.54098727600189));
#41471=CARTESIAN_POINT('Ctrl Pts',(-3.95877154922175,0.319434907277209,
4.52106999256588));
#41472=CARTESIAN_POINT('Ctrl Pts',(-4.03148405249346,0.63630980009529,4.50646466195632));
#41473=CARTESIAN_POINT('Ctrl Pts',(-4.0921896614291,0.794772684000944,4.47550072168819));
#41474=CARTESIAN_POINT('Ctrl Pts',(-4.16303645037653,1.06847604194679,4.48944001093828));
#41475=CARTESIAN_POINT('Ctrl Pts',(-4.19033219163003,1.18514270861497,4.50600028157021));
#41476=CARTESIAN_POINT('Ctrl Pts',(-4.21425672433371,1.30000000000466,4.53308702101923));
#41477=CARTESIAN_POINT('Ctrl Pts',(-4.08578157732975,-1.30000000000017,
4.32042629907166));
#41478=CARTESIAN_POINT('Ctrl Pts',(-4.07007024809314,-1.18514270861192,
4.30404680569939));
#41479=CARTESIAN_POINT('Ctrl Pts',(-4.05259844372008,-1.06847604194522,
4.30081044198283));
#41480=CARTESIAN_POINT('Ctrl Pts',(-4.00816803064877,-0.794772684000903,
4.323697053144));
#41481=CARTESIAN_POINT('Ctrl Pts',(-3.96756936439682,-0.636309800095236,
4.38344510315474));
#41482=CARTESIAN_POINT('Ctrl Pts',(-3.93051351281629,-0.319434907277178,
4.45003209527494));
#41483=CARTESIAN_POINT('Ctrl Pts',(-3.91109268706373,-0.158333333333342,
4.49752712836088));
#41484=CARTESIAN_POINT('Ctrl Pts',(-3.92937723674118,0.158333333333344,
4.52411954299308));
#41485=CARTESIAN_POINT('Ctrl Pts',(-3.96770347442269,0.319434907277188,
4.50407794674818));
#41486=CARTESIAN_POINT('Ctrl Pts',(-4.04073898546218,0.636309800095246,
4.48990394827263));
#41487=CARTESIAN_POINT('Ctrl Pts',(-4.10178143156629,0.794772684000887,
4.45866869142062));
#41488=CARTESIAN_POINT('Ctrl Pts',(-4.17122427188609,1.06847604194672,4.47470220563348));
#41489=CARTESIAN_POINT('Ctrl Pts',(-4.19750573591507,1.18514270861489,4.49264029465091));
#41490=CARTESIAN_POINT('Ctrl Pts',(-4.22000943150921,1.30000000000458,4.52157615848325));
#41491=CARTESIAN_POINT('Ctrl Pts',(-4.09331244521649,-1.30000000000017,
4.30275010216493));
#41492=CARTESIAN_POINT('Ctrl Pts',(-4.07889947091004,-1.18514270861191,
4.28280901708745));
#41493=CARTESIAN_POINT('Ctrl Pts',(-4.0624485095636,-1.06847604194521,4.27703120279117));
#41494=CARTESIAN_POINT('Ctrl Pts',(-4.01973534008945,-0.794772684000897,
4.29640328477619));
#41495=CARTESIAN_POINT('Ctrl Pts',(-3.97918498540679,-0.636309800095234,
4.35705200337412));
#41496=CARTESIAN_POINT('Ctrl Pts',(-3.94305310777462,-0.319434907277177,
4.4243589211843));
#41497=CARTESIAN_POINT('Ctrl Pts',(-3.9242643166955,-0.158333333333341,
4.47407181160574));
#41498=CARTESIAN_POINT('Ctrl Pts',(-3.94294764768243,0.158333333333344,
4.50103789779718));
#41499=CARTESIAN_POINT('Ctrl Pts',(-3.98106324580862,0.319434907277186,
4.47918045867553));
#41500=CARTESIAN_POINT('Ctrl Pts',(-4.05394100901404,0.636309800095243,
4.46498994412542));
#41501=CARTESIAN_POINT('Ctrl Pts',(-4.11561930612219,0.794772684000886,
4.43346165272628));
#41502=CARTESIAN_POINT('Ctrl Pts',(-4.18338547543249,1.06847604194672,4.45303985345004));
#41503=CARTESIAN_POINT('Ctrl Pts',(-4.20846400323075,1.18514270861489,4.47335156716181));
#41504=CARTESIAN_POINT('Ctrl Pts',(-4.22928759511669,1.30000000000457,4.50550031693583));
#41505=CARTESIAN_POINT('Ctrl Pts',(-4.09981791650217,-1.30000000000014,
4.28826914137295));
#41506=CARTESIAN_POINT('Ctrl Pts',(-4.08628630099172,-1.18514270861189,
4.26516743964962));
#41507=CARTESIAN_POINT('Ctrl Pts',(-4.07057910070482,-1.06847604194519,
4.25716837306077));
#41508=CARTESIAN_POINT('Ctrl Pts',(-4.02926628976959,-0.794772684000882,
4.27357903746517));
#41509=CARTESIAN_POINT('Ctrl Pts',(-3.98935503195134,-0.636309800095219,
4.33555643280158));
#41510=CARTESIAN_POINT('Ctrl Pts',(-3.95369594844587,-0.319434907277169,
4.40315775455899));
#41511=CARTESIAN_POINT('Ctrl Pts',(-3.93440263235354,-0.158333333333338,
4.45368910120049));
#41512=CARTESIAN_POINT('Ctrl Pts',(-3.95325279450177,0.15833333333334,4.48080656867185));
#41513=CARTESIAN_POINT('Ctrl Pts',(-3.9920825684725,0.31943490727718,4.45834310390304));
#41514=CARTESIAN_POINT('Ctrl Pts',(-4.06474014002973,0.63630980009523,4.44404218515899));
#41515=CARTESIAN_POINT('Ctrl Pts',(-4.12579708803599,0.794772684000868,
4.41107252450283));
#41516=CARTESIAN_POINT('Ctrl Pts',(-4.19234153738619,1.06847604194669,4.43379393986699));
#41517=CARTESIAN_POINT('Ctrl Pts',(-4.21676455980824,1.18514270861486,4.45644933462131));
#41518=CARTESIAN_POINT('Ctrl Pts',(-4.23680597824331,1.30000000000454,4.49192486533015));
#41519=CARTESIAN_POINT('Ctrl Pts',(-4.10447237338379,-1.30000000000009,
4.27614207678306));
#41520=CARTESIAN_POINT('Ctrl Pts',(-4.09194245717073,-1.18514270861184,
4.2508161108859));
#41521=CARTESIAN_POINT('Ctrl Pts',(-4.07697631455589,-1.06847604194515,
4.24119459589098));
#41522=CARTESIAN_POINT('Ctrl Pts',(-4.03677336079552,-0.794772684000851,
4.25524739472406));
#41523=CARTESIAN_POINT('Ctrl Pts',(-3.99658000879901,-0.636309800095196,
4.31752624590585));
#41524=CARTESIAN_POINT('Ctrl Pts',(-3.96131125941241,-0.319434907277159,
4.38536988024674));
#41525=CARTESIAN_POINT('Ctrl Pts',(-3.94221421725175,-0.158333333333332,
4.43711332662375));
#41526=CARTESIAN_POINT('Ctrl Pts',(-3.96153146945923,0.158333333333334,
4.46466796059675));
#41527=CARTESIAN_POINT('Ctrl Pts',(-4.00084366734633,0.319434907277167,
4.44163678847937));
#41528=CARTESIAN_POINT('Ctrl Pts',(-4.07363130377439,0.636309800095206,
4.42756192963099));
#41529=CARTESIAN_POINT('Ctrl Pts',(-4.13491566051425,0.79477268400084,4.39420947636221));
#41530=CARTESIAN_POINT('Ctrl Pts',(-4.2001773567588,1.06847604194665,4.41909437826389));
#41531=CARTESIAN_POINT('Ctrl Pts',(-4.2237055778276,1.18514270861482,4.44321476474922));
#41532=CARTESIAN_POINT('Ctrl Pts',(-4.24251264984492,1.30000000000449,4.48068378576307));
#41533=CARTESIAN_POINT('Ctrl Pts',(-4.1068263035497,-1.30000000000009,4.27010956050353));
#41534=CARTESIAN_POINT('Ctrl Pts',(-4.09477284803651,-1.18514270861184,
4.24364885985208));
#41535=CARTESIAN_POINT('Ctrl Pts',(-4.08016499765827,-1.06847604194515,
4.23320479314715));
#41536=CARTESIAN_POINT('Ctrl Pts',(-4.04051677785084,-0.794772684000851,
4.24607853826344));
#41537=CARTESIAN_POINT('Ctrl Pts',(-4.00023280952129,-0.636309800095196,
4.30855406036573));
#41538=CARTESIAN_POINT('Ctrl Pts',(-3.96518266532825,-0.319434907277159,
4.37654239510443));
#41539=CARTESIAN_POINT('Ctrl Pts',(-3.94621238249089,-0.158333333333332,
4.42892451651668));
#41540=CARTESIAN_POINT('Ctrl Pts',(-3.96570274858202,0.158333333333334,
4.4566379756269));
#41541=CARTESIAN_POINT('Ctrl Pts',(-4.00511469268083,0.319434907277167,
4.43317916190864));
#41542=CARTESIAN_POINT('Ctrl Pts',(-4.07792758948219,0.636309800095206,
4.41917677348901));
#41543=CARTESIAN_POINT('Ctrl Pts',(-4.13939176391744,0.79477268400084,4.38569778430648));
#41544=CARTESIAN_POINT('Ctrl Pts',(-4.20407556081238,1.06847604194665,4.41173100097376));
#41545=CARTESIAN_POINT('Ctrl Pts',(-4.22718893277774,1.18514270861482,4.4366187769645));
#41546=CARTESIAN_POINT('Ctrl Pts',(-4.24541645780335,1.30000000000449,4.47512551407637));
#41547=CARTESIAN_POINT('',(-4.17593868493484,1.2,4.54217455432741));
#41548=CARTESIAN_POINT('Ctrl Pts',(-4.17593868493484,1.2,4.54217455432741));
#41549=CARTESIAN_POINT('Ctrl Pts',(-4.16901601660958,1.21680579524014,4.56259728301513));
#41550=CARTESIAN_POINT('Ctrl Pts',(-4.16300578492447,1.23314690844626,4.58370303854393));
#41551=CARTESIAN_POINT('Ctrl Pts',(-4.1545018888868,1.25329336998206,4.60811707509031));
#41552=CARTESIAN_POINT('Ctrl Pts',(-4.14807300204321,1.2694610942917,4.62828193480215));
#41553=CARTESIAN_POINT('Ctrl Pts',(-4.13466409677427,1.30000000000457,4.66483672975458));
#41554=CARTESIAN_POINT('',(-4.08975874196504,0.653834841344428,4.41138503336645));
#41555=CARTESIAN_POINT('Ctrl Pts',(-4.08975874202889,0.653834841330258,
4.41138503339054));
#41556=CARTESIAN_POINT('Ctrl Pts',(-4.09901811358657,0.718638123439281,
4.42496474813322));
#41557=CARTESIAN_POINT('Ctrl Pts',(-4.10674533909062,0.76741425862607,4.43641655083457));
#41558=CARTESIAN_POINT('Ctrl Pts',(-4.13510310832554,0.949812869163378,
4.47884925432005));
#41559=CARTESIAN_POINT('Ctrl Pts',(-4.15038021112835,1.04737206040077,4.50201743277146));
#41560=CARTESIAN_POINT('Ctrl Pts',(-4.17593868493484,1.2,4.54217455432741));
#41561=CARTESIAN_POINT('',(-4.00955034077163,-0.653834841531101,4.2972416454658));
#41562=CARTESIAN_POINT('Ctrl Pts',(-4.00955034077163,-0.653834841531101,
4.2972416454658));
#41563=CARTESIAN_POINT('Ctrl Pts',(-3.98922114642734,-0.575773430286786,
4.33363222664404));
#41564=CARTESIAN_POINT('Ctrl Pts',(-3.97295095567435,-0.493715214159444,
4.36480298849665));
#41565=CARTESIAN_POINT('Ctrl Pts',(-3.95138355862527,-0.337919910603026,
4.41065868247051));
#41566=CARTESIAN_POINT('Ctrl Pts',(-3.94493706115634,-0.265431772585284,
4.42737607545058));
#41567=CARTESIAN_POINT('Ctrl Pts',(-3.94024074313496,-0.129514456287131,
4.45124910131288));
#41568=CARTESIAN_POINT('Ctrl Pts',(-3.94090248953005,-0.0665357281317122,
4.45942280949019));
#41569=CARTESIAN_POINT('Ctrl Pts',(-3.94821669426181,0.059433837259308,
4.47048031964631));
#41570=CARTESIAN_POINT('Ctrl Pts',(-3.95489966438366,0.122552721787618,
4.47343903772257));
#41571=CARTESIAN_POINT('Ctrl Pts',(-3.97557216957931,0.259899473210395,
4.47332978277809));
#41572=CARTESIAN_POINT('Ctrl Pts',(-3.99068691758134,0.33378875434452,4.46904341456148));
#41573=CARTESIAN_POINT('Ctrl Pts',(-4.03133525559469,0.491508692492687,
4.44985940941304));
#41574=CARTESIAN_POINT('Ctrl Pts',(-4.05855333857085,0.57491234045661,4.43346975741753));
#41575=CARTESIAN_POINT('Ctrl Pts',(-4.08975874199201,0.653834841365264,
4.41138503347903));
#41576=CARTESIAN_POINT('',(-4.05151251933775,-1.2,4.35610367529872));
#41577=CARTESIAN_POINT('Ctrl Pts',(-4.05151251933775,-1.2,4.35610367529872));
#41578=CARTESIAN_POINT('Ctrl Pts',(-4.0362541407868,-1.0595561432162,4.33436606440657));
#41579=CARTESIAN_POINT('Ctrl Pts',(-4.03163913266016,-0.995649072863461,
4.32796968390379));
#41580=CARTESIAN_POINT('Ctrl Pts',(-4.01413485426632,-0.767227637119597,
4.30353523810531));
#41581=CARTESIAN_POINT('Ctrl Pts',(-4.0115930994257,-0.700415831212995,
4.30006328704156));
#41582=CARTESIAN_POINT('Ctrl Pts',(-4.00955034077163,-0.653834841531101,
4.2972416454658));
#41583=CARTESIAN_POINT('Ctrl Pts',(-4.01183482598955,-1.30000000000003,
4.47462271804853));
#41584=CARTESIAN_POINT('Ctrl Pts',(-4.01895306804897,-1.2829962502188,4.45484161273068));
#41585=CARTESIAN_POINT('Ctrl Pts',(-4.02279613541952,-1.27299706132954,
4.44272395376719));
#41586=CARTESIAN_POINT('Ctrl Pts',(-4.03630670458889,-1.23988587305819,
4.40402165458145));
#41587=CARTESIAN_POINT('Ctrl Pts',(-4.0448273625933,-1.21898355874907,4.37962197974009));
#41588=CARTESIAN_POINT('Ctrl Pts',(-4.05151251933775,-1.2,4.35610367529872));
#41589=CARTESIAN_POINT('Origin',(0.,1.25,7.2));
#41590=CARTESIAN_POINT('Origin',(0.,1.2,7.2));
#41591=CARTESIAN_POINT('Origin',(0.,0.92691742076555,7.2));
#41592=CARTESIAN_POINT('Origin',(0.,0.653834841531101,7.2));
#41593=CARTESIAN_POINT('Origin',(0.,0.,7.2));
#41594=CARTESIAN_POINT('Origin',(0.,-0.653834841531101,7.2));
#41595=CARTESIAN_POINT('Origin',(0.,-0.926917420765551,7.2));
#41596=CARTESIAN_POINT('Origin',(0.,-1.2,7.2));
#41597=CARTESIAN_POINT('Origin',(0.,-1.25,7.2));
#41598=CARTESIAN_POINT('Ctrl Pts',(-3.90341546958844,-1.30000000000013,
4.00440153710639));
#41599=CARTESIAN_POINT('Ctrl Pts',(-3.93440493784207,-1.18514270861187,
4.0336361797219));
#41600=CARTESIAN_POINT('Ctrl Pts',(-3.95093219463971,-1.06847604194516,
4.06330904847551));
#41601=CARTESIAN_POINT('Ctrl Pts',(-3.9557028624898,-0.794772684000851,
4.13287170137922));
#41602=CARTESIAN_POINT('Ctrl Pts',(-3.90486897722008,-0.636309800095197,
4.18098202838527));
#41603=CARTESIAN_POINT('Ctrl Pts',(-3.86905149194761,-0.319434907277159,
4.24590423237585));
#41604=CARTESIAN_POINT('Ctrl Pts',(-3.83456187378936,-0.158333333333332,
4.27613804652327));
#41605=CARTESIAN_POINT('Ctrl Pts',(-3.85489608531651,0.158333333333334,
4.30323841603711));
#41606=CARTESIAN_POINT('Ctrl Pts',(-3.9105765830082,0.319434907277167,4.30138357064611));
#41607=CARTESIAN_POINT('Ctrl Pts',(-3.986068422003,0.636309800095206,4.28905845346891));
#41608=CARTESIAN_POINT('Ctrl Pts',(-4.05793460521832,0.794772684000841,
4.27005212095193));
#41609=CARTESIAN_POINT('Ctrl Pts',(-4.08243023811812,1.06847604194587,4.23632262916638));
#41610=CARTESIAN_POINT('Ctrl Pts',(-4.07701141444102,1.18514270861327,4.21920234377186));
#41611=CARTESIAN_POINT('Ctrl Pts',(-4.05557051525711,1.30000000000221,4.199562020176));
#41612=CARTESIAN_POINT('Ctrl Pts',(-3.89104835659712,-1.30000000000013,
4.00648970721449));
#41613=CARTESIAN_POINT('Ctrl Pts',(-3.91970579181625,-1.18514270861187,
4.03618536988084));
#41614=CARTESIAN_POINT('Ctrl Pts',(-3.9345169961985,-1.06847604194516,4.06617305571521));
#41615=CARTESIAN_POINT('Ctrl Pts',(-3.93674627813055,-0.794772684000851,
4.13612524094578));
#41616=CARTESIAN_POINT('Ctrl Pts',(-3.8862642118845,-0.636309800095197,
4.18397173789519));
#41617=CARTESIAN_POINT('Ctrl Pts',(-3.8503244914224,-0.319434907277159,
4.24880110462245));
#41618=CARTESIAN_POINT('Ctrl Pts',(-3.81670994248296,-0.158333333333332,
4.27910948723805));
#41619=CARTESIAN_POINT('Ctrl Pts',(-3.83684904091065,0.158333333333334,
4.3057824152448));
#41620=CARTESIAN_POINT('Ctrl Pts',(-3.89139304806992,0.319434907277167,
4.30329173640962));
#41621=CARTESIAN_POINT('Ctrl Pts',(-3.96674475597724,0.636309800095206,
4.2904613776932));
#41622=CARTESIAN_POINT('Ctrl Pts',(-4.0381808448611,0.794772684000841,4.27150585840089));
#41623=CARTESIAN_POINT('Ctrl Pts',(-4.06526201563984,1.06847604194587,4.23744989520493));
#41624=CARTESIAN_POINT('Ctrl Pts',(-4.06162921507938,1.18514270861327,4.22015646238466));
#41625=CARTESIAN_POINT('Ctrl Pts',(-4.04264117858458,1.30000000000221,4.2003111613139));
#41626=CARTESIAN_POINT('Ctrl Pts',(-3.86661484837121,-1.30000000000009,
4.01111768457726));
#41627=CARTESIAN_POINT('Ctrl Pts',(-3.88996380996409,-1.18514270861183,
4.04060036765782));
#41628=CARTESIAN_POINT('Ctrl Pts',(-3.9009745686697,-1.06847604194513,4.0705809196837));
#41629=CARTESIAN_POINT('Ctrl Pts',(-3.89790790705575,-0.794772684000829,
4.1409921693144));
#41630=CARTESIAN_POINT('Ctrl Pts',(-3.84917492123562,-0.63630980009518,
4.19026026497731));
#41631=CARTESIAN_POINT('Ctrl Pts',(-3.81325488317549,-0.319434907277152,
4.2554023339609));
#41632=CARTESIAN_POINT('Ctrl Pts',(-3.78099858233076,-0.158333333333329,
4.28508308114211));
#41633=CARTESIAN_POINT('Ctrl Pts',(-3.80083048546607,0.158333333333331,
4.31108897200467));
#41634=CARTESIAN_POINT('Ctrl Pts',(-3.85350460551506,0.319434907277162,
4.3081787780579));
#41635=CARTESIAN_POINT('Ctrl Pts',(-3.92862733347231,0.636309800095193,
4.2944512740811));
#41636=CARTESIAN_POINT('Ctrl Pts',(-3.99882638092636,0.794772684000823,
4.27482471898379));
#41637=CARTESIAN_POINT('Ctrl Pts',(-4.03108771157174,1.06847604194584,4.24009901002036));
#41638=CARTESIAN_POINT('Ctrl Pts',(-4.03110099808034,1.18514270861324,4.22258713986118));
#41639=CARTESIAN_POINT('Ctrl Pts',(-4.01716283646121,1.30000000000217,4.2025948722388));
#41640=CARTESIAN_POINT('Ctrl Pts',(-3.84163939128475,-1.30000000000008,
4.01575214899236));
#41641=CARTESIAN_POINT('Ctrl Pts',(-3.86056353497618,-1.18514270861182,
4.04677393771985));
#41642=CARTESIAN_POINT('Ctrl Pts',(-3.86827184668624,-1.06847604194511,
4.07775329050274));
#41643=CARTESIAN_POINT('Ctrl Pts',(-3.8601687731825,-0.794772684000817,
4.14922375730824));
#41644=CARTESIAN_POINT('Ctrl Pts',(-3.81170264137483,-0.636309800095171,
4.19713572363613));
#41645=CARTESIAN_POINT('Ctrl Pts',(-3.77539078952671,-0.319434907277146,
4.26183594430695));
#41646=CARTESIAN_POINT('Ctrl Pts',(-3.74490615950961,-0.158333333333326,
4.2916228682938));
#41647=CARTESIAN_POINT('Ctrl Pts',(-3.76449993658487,0.158333333333328,
4.31711707741851));
#41648=CARTESIAN_POINT('Ctrl Pts',(-3.81530634625955,0.319434907277153,
4.31388176381152));
#41649=CARTESIAN_POINT('Ctrl Pts',(-3.89004642236894,0.63630980009518,4.29895756126248));
#41650=CARTESIAN_POINT('Ctrl Pts',(-3.95862216654278,0.79477268400081,4.27791873481429));
#41651=CARTESIAN_POINT('Ctrl Pts',(-3.99611319657198,1.06847604194582,4.24240864936715));
#41652=CARTESIAN_POINT('Ctrl Pts',(-3.99989511980788,1.18514270861322,4.224777018362));
#41653=CARTESIAN_POINT('Ctrl Pts',(-3.99123048855958,1.30000000000215,4.20488475656349));
#41654=CARTESIAN_POINT('Ctrl Pts',(-3.8286278109767,-1.30000000000007,4.01822206427942));
#41655=CARTESIAN_POINT('Ctrl Pts',(-3.84480093063131,-1.18514270861181,
4.04928111560884));
#41656=CARTESIAN_POINT('Ctrl Pts',(-3.85053359401985,-1.06847604194511,
4.08035218408484));
#41657=CARTESIAN_POINT('Ctrl Pts',(-3.83965765068204,-0.794772684000815,
4.15216033002293));
#41658=CARTESIAN_POINT('Ctrl Pts',(-3.79199422350366,-0.636309800095168,
4.20057565258571));
#41659=CARTESIAN_POINT('Ctrl Pts',(-3.7557711364051,-0.319434907277145,
4.26559035383413));
#41660=CARTESIAN_POINT('Ctrl Pts',(-3.72624824301149,-0.158333333333325,
4.29549393781957));
#41661=CARTESIAN_POINT('Ctrl Pts',(-3.74569302684835,0.158333333333327,
4.32067544009606));
#41662=CARTESIAN_POINT('Ctrl Pts',(-3.79525526709828,0.319434907277153,
4.31675986160739));
#41663=CARTESIAN_POINT('Ctrl Pts',(-3.86987489674091,0.636309800095178,
4.30139527837829));
#41664=CARTESIAN_POINT('Ctrl Pts',(-3.93806495582426,0.794772684000808,
4.28057716166906));
#41665=CARTESIAN_POINT('Ctrl Pts',(-3.97829562722386,1.06847604194582,4.24465368868101));
#41666=CARTESIAN_POINT('Ctrl Pts',(-3.98395365181045,1.18514270861321,4.22675274202847));
#41667=CARTESIAN_POINT('Ctrl Pts',(-3.97785533402799,1.30000000000214,4.20650078908409));
#41668=CARTESIAN_POINT('Ctrl Pts',(-3.82710684528072,-1.30000000000007,
4.01852991983173));
#41669=CARTESIAN_POINT('Ctrl Pts',(-3.84295899747086,-1.18514270861181,
4.04959891491916));
#41670=CARTESIAN_POINT('Ctrl Pts',(-3.84846039396343,-1.06847604194511,
4.08068334373606));
#41671=CARTESIAN_POINT('Ctrl Pts',(-3.83725740408892,-0.794772684000815,
4.15253024772438));
#41672=CARTESIAN_POINT('Ctrl Pts',(-3.78967982079165,-0.636309800095169,
4.20098843507329));
#41673=CARTESIAN_POINT('Ctrl Pts',(-3.75346683494883,-0.319434907277145,
4.26603985549636));
#41674=CARTESIAN_POINT('Ctrl Pts',(-3.72406481821863,-0.158333333333325,
4.29597213108033));
#41675=CARTESIAN_POINT('Ctrl Pts',(-3.74349214685304,0.158333333333327,
4.32111727724511));
#41676=CARTESIAN_POINT('Ctrl Pts',(-3.79290325446431,0.319434907277153,
4.31711286623261));
#41677=CARTESIAN_POINT('Ctrl Pts',(-3.86750330211314,0.636309800095178,
4.30168595699973));
#41678=CARTESIAN_POINT('Ctrl Pts',(-3.93564235693815,0.794772684000808,
4.28088239017744));
#41679=CARTESIAN_POINT('Ctrl Pts',(-3.97619443018704,1.06847604194582,4.24490823250405));
#41680=CARTESIAN_POINT('Ctrl Pts',(-3.98207420706277,1.18514270861321,4.22697751851431));
#41681=CARTESIAN_POINT('Ctrl Pts',(-3.97628027090713,1.30000000000214,4.20668797041776));
#41682=CARTESIAN_POINT('Ctrl Pts',(-3.82444661259715,-1.30000000000007,
4.01907178088306));
#41683=CARTESIAN_POINT('Ctrl Pts',(-3.83974163577605,-1.18514270861181,
4.05016618767936));
#41684=CARTESIAN_POINT('Ctrl Pts',(-3.84484114962181,-1.06847604194511,
4.08127899892876));
#41685=CARTESIAN_POINT('Ctrl Pts',(-3.83306838059555,-0.794772684000815,
4.15319833497988));
#41686=CARTESIAN_POINT('Ctrl Pts',(-3.78563780298979,-0.636309800095169,
4.20172638828723));
#41687=CARTESIAN_POINT('Ctrl Pts',(-3.74943701118573,-0.319434907277146,
4.26683200753139));
#41688=CARTESIAN_POINT('Ctrl Pts',(-3.72023757771806,-0.158333333333325,
4.29679732018735));
#41689=CARTESIAN_POINT('Ctrl Pts',(-3.73963440904793,0.158333333333328,
4.32187909990591));
#41690=CARTESIAN_POINT('Ctrl Pts',(-3.78879227213193,0.319434907277153,
4.31774099149246));
#41691=CARTESIAN_POINT('Ctrl Pts',(-3.86335907746366,0.636309800095178,
4.30220677550402));
#41692=CARTESIAN_POINT('Ctrl Pts',(-3.9313998840663,0.794772684000808,4.28141073634073));
#41693=CARTESIAN_POINT('Ctrl Pts',(-3.97251266409711,1.06847604194582,4.24534445646052));
#41694=CARTESIAN_POINT('Ctrl Pts',(-3.9787810112287,1.18514270861321,4.2273627215518));
#41695=CARTESIAN_POINT('Ctrl Pts',(-3.97352150639511,1.30000000000214,4.20701100790716));
#41696=CARTESIAN_POINT('Ctrl Pts',(-3.81915395213725,-1.30000000000007,
4.02020751913203));
#41697=CARTESIAN_POINT('Ctrl Pts',(-3.83336539572861,-1.18514270861181,
4.05140900057002));
#41698=CARTESIAN_POINT('Ctrl Pts',(-3.83767878966736,-1.06847604194511,
4.08261106947747));
#41699=CARTESIAN_POINT('Ctrl Pts',(-3.82477711776183,-0.794772684000815,
4.15469544777816));
#41700=CARTESIAN_POINT('Ctrl Pts',(-3.7775995078436,-0.636309800095168,
4.20328916354697));
#41701=CARTESIAN_POINT('Ctrl Pts',(-3.74139562495426,-0.319434907277145,
4.26845329303305));
#41702=CARTESIAN_POINT('Ctrl Pts',(-3.7125803976688,-0.158333333333325,
4.29844492512511));
#41703=CARTESIAN_POINT('Ctrl Pts',(-3.73191725698259,0.158333333333327,
4.32340352741718));
#41704=CARTESIAN_POINT('Ctrl Pts',(-3.78061130320096,0.319434907277153,
4.3190820784816));
#41705=CARTESIAN_POINT('Ctrl Pts',(-3.8550990434907,0.636309800095178,4.30330738580016));
#41706=CARTESIAN_POINT('Ctrl Pts',(-3.92287596258615,0.794772684000807,
4.28239104658693));
#41707=CARTESIAN_POINT('Ctrl Pts',(-3.96510110964664,1.06847604194582,4.24612188585345));
#41708=CARTESIAN_POINT('Ctrl Pts',(-3.97215501839537,1.18514270861321,4.22805477717417));
#41709=CARTESIAN_POINT('Ctrl Pts',(-3.96798513432618,1.30000000000214,4.20762013559235));
#41710=CARTESIAN_POINT('Ctrl Pts',(-3.81315583966002,-1.30000000000007,
4.0216054592221));
#41711=CARTESIAN_POINT('Ctrl Pts',(-3.8262311916753,-1.18514270861182,4.05311260169393));
#41712=CARTESIAN_POINT('Ctrl Pts',(-3.82970664459084,-1.06847604194511,
4.08452506541706));
#41713=CARTESIAN_POINT('Ctrl Pts',(-3.81555794871411,-0.794772684000816,
4.15687541380941));
#41714=CARTESIAN_POINT('Ctrl Pts',(-3.76855240047573,-0.63630980009517,
4.20533651202818));
#41715=CARTESIAN_POINT('Ctrl Pts',(-3.73224815440427,-0.319434907277146,
4.27039003013774));
#41716=CARTESIAN_POINT('Ctrl Pts',(-3.70377100950362,-0.158333333333325,
4.30021903851715));
#41717=CARTESIAN_POINT('Ctrl Pts',(-3.72304001329379,0.158333333333328,
4.32504230140401));
#41718=CARTESIAN_POINT('Ctrl Pts',(-3.77135999334345,0.319434907277154,
4.32081643901291));
#41719=CARTESIAN_POINT('Ctrl Pts',(-3.84574495956043,0.63630980009518,4.30473755434541));
#41720=CARTESIAN_POINT('Ctrl Pts',(-3.91304112819147,0.794772684000809,
4.28332116762538));
#41721=CARTESIAN_POINT('Ctrl Pts',(-3.956511644309,1.06847604194582,4.24676844297429));
#41722=CARTESIAN_POINT('Ctrl Pts',(-3.96448243439118,1.18514270861322,4.22864330258963));
#41723=CARTESIAN_POINT('Ctrl Pts',(-3.96160723886955,1.30000000000215,4.2082153419099));
#41724=CARTESIAN_POINT('Ctrl Pts',(-3.80715438504397,-1.30000000000007,
4.02300105414969));
#41725=CARTESIAN_POINT('Ctrl Pts',(-3.81909176514673,-1.18514270861182,
4.05481311590196));
#41726=CARTESIAN_POINT('Ctrl Pts',(-3.82173114234454,-1.06847604194511,
4.08644103377522));
#41727=CARTESIAN_POINT('Ctrl Pts',(-3.80634838490757,-0.794772684000818,
4.15908244200738));
#41728=CARTESIAN_POINT('Ctrl Pts',(-3.75954037010185,-0.636309800095171,
4.20745421948047));
#41729=CARTESIAN_POINT('Ctrl Pts',(-3.72315249890494,-0.319434907277147,
4.27242666413317));
#41730=CARTESIAN_POINT('Ctrl Pts',(-3.69501795631059,-0.158333333333326,
4.30210029916821));
#41731=CARTESIAN_POINT('Ctrl Pts',(-3.71421357862602,0.158333333333328,
4.32678066237708));
#41732=CARTESIAN_POINT('Ctrl Pts',(-3.76214214475683,0.319434907277154,
4.32262400819918));
#41733=CARTESIAN_POINT('Ctrl Pts',(-3.83641121627868,0.636309800095181,
4.30621955644676));
#41734=CARTESIAN_POINT('Ctrl Pts',(-3.90322589564299,0.79477268400081,4.28430194023565));
#41735=CARTESIAN_POINT('Ctrl Pts',(-3.94793323256432,1.06847604194582,4.24744674986031));
#41736=CARTESIAN_POINT('Ctrl Pts',(-3.95681676141385,1.18514270861322,4.22925357514636));
#41737=CARTESIAN_POINT('Ctrl Pts',(-3.9552316695297,1.30000000000215,4.2088204720126));
#41738=CARTESIAN_POINT('Ctrl Pts',(-3.80114234291894,-1.30000000000007,
4.0243783591317));
#41739=CARTESIAN_POINT('Ctrl Pts',(-3.81192416135968,-1.18514270861182,
4.05646416886568));
#41740=CARTESIAN_POINT('Ctrl Pts',(-3.81371945824022,-1.06847604194511,
4.08829360459836));
#41741=CARTESIAN_POINT('Ctrl Pts',(-3.79710629063061,-0.794772684000818,
4.16123369336721));
#41742=CARTESIAN_POINT('Ctrl Pts',(-3.75053327720066,-0.636309800095171,
4.20958397466905));
#41743=CARTESIAN_POINT('Ctrl Pts',(-3.71409328185195,-0.319434907277147,
4.27453344748291));
#41744=CARTESIAN_POINT('Ctrl Pts',(-3.68633034992726,-0.158333333333326,
4.30410581984449));
#41745=CARTESIAN_POINT('Ctrl Pts',(-3.70544254508084,0.158333333333328,
4.3286249931167));
#41746=CARTESIAN_POINT('Ctrl Pts',(-3.75290823669572,0.319434907277154,
4.32440253561861));
#41747=CARTESIAN_POINT('Ctrl Pts',(-3.82707546000951,0.63630980009518,4.30770469251513));
#41748=CARTESIAN_POINT('Ctrl Pts',(-3.89351928822256,0.794772684000811,
4.28550667350574));
#41749=CARTESIAN_POINT('Ctrl Pts',(-3.93946473095619,1.06847604194583,4.24835060648487));
#41750=CARTESIAN_POINT('Ctrl Pts',(-3.94923896567685,1.18514270861322,4.23004437469339));
#41751=CARTESIAN_POINT('Ctrl Pts',(-3.94889935540516,1.30000000000215,4.20951539575585));
#41752=CARTESIAN_POINT('Ctrl Pts',(-3.78440028110535,-1.30000000000008,
4.02778953669477));
#41753=CARTESIAN_POINT('Ctrl Pts',(-3.79171108268268,-1.18514270861182,
4.06011172210803));
#41754=CARTESIAN_POINT('Ctrl Pts',(-3.79101861768583,-1.06847604194512,
4.09220196366834));
#41755=CARTESIAN_POINT('Ctrl Pts',(-3.77092973818161,-0.794772684000821,
4.16580100460297));
#41756=CARTESIAN_POINT('Ctrl Pts',(-3.72537387638473,-0.636309800095172,
4.21473776392922));
#41757=CARTESIAN_POINT('Ctrl Pts',(-3.68913832694495,-0.319434907277146,
4.28025055716962));
#41758=CARTESIAN_POINT('Ctrl Pts',(-3.66274336562862,-0.158333333333326,
4.31018669309415));
#41759=CARTESIAN_POINT('Ctrl Pts',(-3.68168289994384,0.158333333333328,
4.33436533221495));
#41760=CARTESIAN_POINT('Ctrl Pts',(-3.72752328510863,0.319434907277155,
4.32930246592143));
#41761=CARTESIAN_POINT('Ctrl Pts',(-3.80130684170286,0.636309800095182,
4.311624907316));
#41762=CARTESIAN_POINT('Ctrl Pts',(-3.86685632366673,0.794772684000811,
4.2889357991253));
#41763=CARTESIAN_POINT('Ctrl Pts',(-3.9162208030225,1.06847604194583,4.25097921818241));
#41764=CARTESIAN_POINT('Ctrl Pts',(-3.92843965377663,1.18514270861322,4.23234236241147));
#41765=CARTESIAN_POINT('Ctrl Pts',(-3.93150930130592,1.30000000000215,4.21149864832987));
#41766=CARTESIAN_POINT('Ctrl Pts',(-3.75431580962117,-1.30000000000009,
4.03469504713538));
#41767=CARTESIAN_POINT('Ctrl Pts',(-3.75593416776671,-1.18514270861183,
4.06853321701457));
#41768=CARTESIAN_POINT('Ctrl Pts',(-3.75106608557199,-1.06847604194513,
4.10171222975162));
#41769=CARTESIAN_POINT('Ctrl Pts',(-3.72483486705178,-0.794772684000829,
4.17683960175068));
#41770=CARTESIAN_POINT('Ctrl Pts',(-3.68022258902514,-0.636309800095178,
4.22530365278323));
#41771=CARTESIAN_POINT('Ctrl Pts',(-3.64379213672342,-0.31943490727715,
4.29082854797332));
#41772=CARTESIAN_POINT('Ctrl Pts',(-3.61957756337174,-0.158333333333327,
4.32080382713417));
#41773=CARTESIAN_POINT('Ctrl Pts',(-3.63812902402165,0.15833333333333,4.34421786945562));
#41774=CARTESIAN_POINT('Ctrl Pts',(-3.68120840915105,0.319434907277156,
4.33799029755456));
#41775=CARTESIAN_POINT('Ctrl Pts',(-3.75478857736182,0.636309800095186,
4.31947846925158));
#41776=CARTESIAN_POINT('Ctrl Pts',(-3.81957493385749,0.794772684000819,
4.29756971904014));
#41777=CARTESIAN_POINT('Ctrl Pts',(-3.87514362963652,1.06847604194584,4.25811941793536));
#41778=CARTESIAN_POINT('Ctrl Pts',(-3.89158284045524,1.18514270861323,4.23843792787219));
#41779=CARTESIAN_POINT('Ctrl Pts',(-3.90040763271295,1.30000000000216,4.21615152131645));
#41780=CARTESIAN_POINT('Ctrl Pts',(-3.71845854499846,-1.30000000000011,
4.04341913141646));
#41781=CARTESIAN_POINT('Ctrl Pts',(-3.71281545479014,-1.18514270861185,
4.07842216145478));
#41782=CARTESIAN_POINT('Ctrl Pts',(-3.70278387581907,-1.06847604194514,
4.11269641728366));
#41783=CARTESIAN_POINT('Ctrl Pts',(-3.66947063462934,-0.794772684000839,
4.19019319057521));
#41784=CARTESIAN_POINT('Ctrl Pts',(-3.62762195270144,-0.636309800095187,
4.24076083845827));
#41785=CARTESIAN_POINT('Ctrl Pts',(-3.5912064928209,-0.319434907277154,
4.30672857459846));
#41786=CARTESIAN_POINT('Ctrl Pts',(-3.56856204276642,-0.15833333333333,
4.33500412610548));
#41787=CARTESIAN_POINT('Ctrl Pts',(-3.58636155667854,0.158333333333332,
4.35711349894132));
#41788=CARTESIAN_POINT('Ctrl Pts',(-3.62682870546288,0.319434907277161,
4.3508833371881));
#41789=CARTESIAN_POINT('Ctrl Pts',(-3.69945326777052,0.636309800095196,
4.33008113051802));
#41790=CARTESIAN_POINT('Ctrl Pts',(-3.76132565597827,0.79477268400083,4.30531932672598));
#41791=CARTESIAN_POINT('Ctrl Pts',(-3.82420327488111,1.06847604194585,4.2637660533126));
#41792=CARTESIAN_POINT('Ctrl Pts',(-3.84607635354761,1.18514270861325,4.24349148729524));
#41793=CARTESIAN_POINT('Ctrl Pts',(-3.86260511950287,1.30000000000218,4.2209292276207));
#41794=CARTESIAN_POINT('Ctrl Pts',(-3.68860773760897,-1.30000000000011,
4.05087423379425));
#41795=CARTESIAN_POINT('Ctrl Pts',(-3.67760555817564,-1.18514270861185,
4.08800447745914));
#41796=CARTESIAN_POINT('Ctrl Pts',(-3.66363318323603,-1.06847604194514,
4.12379980892036));
#41797=CARTESIAN_POINT('Ctrl Pts',(-3.62449245615642,-0.794772684000841,
4.20341027118856));
#41798=CARTESIAN_POINT('Ctrl Pts',(-3.58335565480229,-0.636309800095186,
4.25310147302822));
#41799=CARTESIAN_POINT('Ctrl Pts',(-3.54690519449343,-0.319434907277153,
4.31936861187515));
#41800=CARTESIAN_POINT('Ctrl Pts',(-3.52667420534236,-0.15833333333333,
4.34804547385783));
#41801=CARTESIAN_POINT('Ctrl Pts',(-3.54433517289505,0.158333333333332,
4.36990767094282));
#41802=CARTESIAN_POINT('Ctrl Pts',(-3.58234467633409,0.319434907277164,
4.36321247602415));
#41803=CARTESIAN_POINT('Ctrl Pts',(-3.65452982167986,0.636309800095198,
4.34123370676381));
#41804=CARTESIAN_POINT('Ctrl Pts',(-3.71489062245268,0.794772684000828,
4.3159194258204));
#41805=CARTESIAN_POINT('Ctrl Pts',(-3.78361743146054,1.06847604194585,4.27215390529769));
#41806=CARTESIAN_POINT('Ctrl Pts',(-3.80964766432572,1.18514270861325,4.25065806866689));
#41807=CARTESIAN_POINT('Ctrl Pts',(-3.83195884101573,1.30000000000218,4.22661086756729));
#41808=CARTESIAN_POINT('Ctrl Pts',(-3.6713578924185,-1.30000000000011,4.05637552490219));
#41809=CARTESIAN_POINT('Ctrl Pts',(-3.65681897753628,-1.18514270861185,
4.0942929127349));
#41810=CARTESIAN_POINT('Ctrl Pts',(-3.6403280952585,-1.06847604194515,4.13077476054769));
#41811=CARTESIAN_POINT('Ctrl Pts',(-3.59772142303366,-0.79477268400084,
4.21173874253912));
#41812=CARTESIAN_POINT('Ctrl Pts',(-3.55785138804934,-0.636309800095187,
4.26226292612346));
#41813=CARTESIAN_POINT('Ctrl Pts',(-3.52149059562518,-0.319434907277154,
4.32889163046889));
#41814=CARTESIAN_POINT('Ctrl Pts',(-3.50238889835621,-0.15833333333333,
4.35729267517949));
#41815=CARTESIAN_POINT('Ctrl Pts',(-3.51943719293129,0.158333333333332,
4.37812398711004));
#41816=CARTESIAN_POINT('Ctrl Pts',(-3.55538048430167,0.319434907277164,
4.37016213958272));
#41817=CARTESIAN_POINT('Ctrl Pts',(-3.62688845923927,0.636309800095198,
4.34676402724258));
#41818=CARTESIAN_POINT('Ctrl Pts',(-3.68630461596718,0.794772684000829,
4.32100136029989));
#41819=CARTESIAN_POINT('Ctrl Pts',(-3.75871889523108,1.06847604194585,4.27621495187951));
#41820=CARTESIAN_POINT('Ctrl Pts',(-3.78740784200528,1.18514270861325,4.25427972662216));
#41821=CARTESIAN_POINT('Ctrl Pts',(-3.81344027727371,1.30000000000218,4.22979565281272));
#41822=CARTESIAN_POINT('Ctrl Pts',(-3.65953806887845,-1.30000000000011,
4.05956467038674));
#41823=CARTESIAN_POINT('Ctrl Pts',(-3.64275164454373,-1.18514270861185,
4.09817936736322));
#41824=CARTESIAN_POINT('Ctrl Pts',(-3.62465461865293,-1.06847604194515,
4.13523172571671));
#41825=CARTESIAN_POINT('Ctrl Pts',(-3.57981911676806,-0.79477268400084,
4.21722077104828));
#41826=CARTESIAN_POINT('Ctrl Pts',(-3.54071399063127,-0.636309800095187,
4.26816764904755));
#41827=CARTESIAN_POINT('Ctrl Pts',(-3.50437272359351,-0.319434907277154,
4.33496727815371));
#41828=CARTESIAN_POINT('Ctrl Pts',(-3.48584156137425,-0.15833333333333,
4.36287047623089));
#41829=CARTESIAN_POINT('Ctrl Pts',(-3.50275255446116,0.158333333333332,
4.38348922139645));
#41830=CARTESIAN_POINT('Ctrl Pts',(-3.53796421858062,0.319434907277164,
4.37580411999686));
#41831=CARTESIAN_POINT('Ctrl Pts',(-3.60922145485592,0.636309800095198,
4.35181948231638));
#41832=CARTESIAN_POINT('Ctrl Pts',(-3.66769099794688,0.794772684000829,
4.32523451559654));
#41833=CARTESIAN_POINT('Ctrl Pts',(-3.74237473288132,1.06847604194585,4.2794300918488));
#41834=CARTESIAN_POINT('Ctrl Pts',(-3.77275449553502,1.18514270861325,4.25704763651013));
#41835=CARTESIAN_POINT('Ctrl Pts',(-3.80118619929431,1.30000000000218,4.23210976365206));
#41836=CARTESIAN_POINT('Ctrl Pts',(-3.64763149426099,-1.30000000000011,
4.06262355022668));
#41837=CARTESIAN_POINT('Ctrl Pts',(-3.62864155950371,-1.18514270861185,
4.10200475472687));
#41838=CARTESIAN_POINT('Ctrl Pts',(-3.60894451243852,-1.06847604194515,
4.13963634627431));
#41839=CARTESIAN_POINT('Ctrl Pts',(-3.56180682244858,-0.79477268400084,
4.22253089499322));
#41840=CARTESIAN_POINT('Ctrl Pts',(-3.52315869206691,-0.636309800095187,
4.2734045470392));
#41841=CARTESIAN_POINT('Ctrl Pts',(-3.4868951844582,-0.319434907277153,
4.34047108936095));
#41842=CARTESIAN_POINT('Ctrl Pts',(-3.46930116449699,-0.15833333333333,
4.36847389132249));
#41843=CARTESIAN_POINT('Ctrl Pts',(-3.48621641437049,0.158333333333332,
4.38910402940942));
#41844=CARTESIAN_POINT('Ctrl Pts',(-3.52056315194149,0.319434907277165,
4.38145890581359));
#41845=CARTESIAN_POINT('Ctrl Pts',(-3.59161287212262,0.636309800095199,
4.35696945019006));
#41846=CARTESIAN_POINT('Ctrl Pts',(-3.64938437719694,0.794772684000828,
4.33002585779554));
#41847=CARTESIAN_POINT('Ctrl Pts',(-3.72617585145565,1.06847604194585,4.28292121233611));
#41848=CARTESIAN_POINT('Ctrl Pts',(-3.75808826963396,1.18514270861325,4.25980910066091));
#41849=CARTESIAN_POINT('Ctrl Pts',(-3.78867292218844,1.30000000000218,4.23397473293081));
#41850=CARTESIAN_POINT('Ctrl Pts',(-3.63356070629899,-1.30000000000011,
4.06771912618167));
#41851=CARTESIAN_POINT('Ctrl Pts',(-3.61190523818026,-1.18514270861185,
4.10821439751999));
#41852=CARTESIAN_POINT('Ctrl Pts',(-3.59025924039026,-1.06847604194514,
4.14666172767279));
#41853=CARTESIAN_POINT('Ctrl Pts',(-3.54027453358219,-0.794772684000836,
4.23075159786));
#41854=CARTESIAN_POINT('Ctrl Pts',(-3.50209435486207,-0.636309800095187,
4.28136659178616));
#41855=CARTESIAN_POINT('Ctrl Pts',(-3.46581721460012,-0.319434907277155,
4.34858660764036));
#41856=CARTESIAN_POINT('Ctrl Pts',(-3.44938662503235,-0.15833333333333,
4.37668899529829));
#41857=CARTESIAN_POINT('Ctrl Pts',(-3.46605537953192,0.158333333333332,
4.39693214740327));
#41858=CARTESIAN_POINT('Ctrl Pts',(-3.49899661499291,0.319434907277164,
4.3888337043609));
#41859=CARTESIAN_POINT('Ctrl Pts',(-3.56954886382728,0.636309800095199,
4.36333478022166));
#41860=CARTESIAN_POINT('Ctrl Pts',(-3.62626490666719,0.79477268400083,4.33560657240965));
#41861=CARTESIAN_POINT('Ctrl Pts',(-3.70599662287337,1.06847604194585,4.28742033396522));
#41862=CARTESIAN_POINT('Ctrl Pts',(-3.74008348373225,1.18514270861325,4.26385395901444));
#41863=CARTESIAN_POINT('Ctrl Pts',(-3.77374429985551,1.30000000000219,4.23757924625945));
#41864=CARTESIAN_POINT('Ctrl Pts',(-3.61556442432805,-1.30000000000011,
4.07212390020608));
#41865=CARTESIAN_POINT('Ctrl Pts',(-3.59052030686365,-1.18514270861186,
4.11364527817067));
#41866=CARTESIAN_POINT('Ctrl Pts',(-3.56647933735157,-1.06847604194515,
4.15297548954064));
#41867=CARTESIAN_POINT('Ctrl Pts',(-3.51325736084816,-0.79477268400084,
4.23877411261215));
#41868=CARTESIAN_POINT('Ctrl Pts',(-3.47636400274692,-0.636309800095187,
4.29023140353388));
#41869=CARTESIAN_POINT('Ctrl Pts',(-3.44039829889856,-0.319434907277154,
4.3581552682494));
#41870=CARTESIAN_POINT('Ctrl Pts',(-3.42520449940565,-0.15833333333333,
4.38612618263592));
#41871=CARTESIAN_POINT('Ctrl Pts',(-3.44162252975853,0.158333333333333,
4.40597806540559));
#41872=CARTESIAN_POINT('Ctrl Pts',(-3.47291449043845,0.319434907277166,
4.39739377561058));
#41873=CARTESIAN_POINT('Ctrl Pts',(-3.54297409043778,0.636309800095201,
4.37085446412307));
#41874=CARTESIAN_POINT('Ctrl Pts',(-3.59866509550172,0.794772684000828,
4.34260442254614));
#41875=CARTESIAN_POINT('Ctrl Pts',(-3.68176721306064,1.06847604194585,4.29282591017169));
#41876=CARTESIAN_POINT('Ctrl Pts',(-3.71830307599038,1.18514270861325,4.26842376765041));
#41877=CARTESIAN_POINT('Ctrl Pts',(-3.75540297439542,1.30000000000219,4.24116675613916));
#41878=CARTESIAN_POINT('Ctrl Pts',(-3.58711823022728,-1.30000000000012,
4.08187617918603));
#41879=CARTESIAN_POINT('Ctrl Pts',(-3.55703818746489,-1.18514270861186,
4.12606687667337));
#41880=CARTESIAN_POINT('Ctrl Pts',(-3.52932505513652,-1.06847604194515,
4.16736681533446));
#41881=CARTESIAN_POINT('Ctrl Pts',(-3.4707702120663,-0.794772684000845,
4.25609970448304));
#41882=CARTESIAN_POINT('Ctrl Pts',(-3.43493185365833,-0.636309800095188,
4.3072299850739));
#41883=CARTESIAN_POINT('Ctrl Pts',(-3.39880756631888,-0.319434907277153,
4.37525690461322));
#41884=CARTESIAN_POINT('Ctrl Pts',(-3.38531233642891,-0.15833333333333,
4.40243413564541));
#41885=CARTESIAN_POINT('Ctrl Pts',(-3.4013848592705,0.158333333333332,4.42178376594812));
#41886=CARTESIAN_POINT('Ctrl Pts',(-3.43075527646008,0.319434907277165,
4.41374302140569));
#41887=CARTESIAN_POINT('Ctrl Pts',(-3.50002009385822,0.636309800095199,
4.38556406417354));
#41888=CARTESIAN_POINT('Ctrl Pts',(-3.55338726970055,0.794772684000829,
4.35551705671428));
#41889=CARTESIAN_POINT('Ctrl Pts',(-3.64165109224554,1.06847604194585,4.3023569314744));
#41890=CARTESIAN_POINT('Ctrl Pts',(-3.68208795061293,1.18514270861325,4.27625721711571));
#41891=CARTESIAN_POINT('Ctrl Pts',(-3.7247555290648,1.30000000000219,4.24706883683798));
#41892=CARTESIAN_POINT('Ctrl Pts',(-3.55260469525799,-1.30000000000013,
4.09307313514165));
#41893=CARTESIAN_POINT('Ctrl Pts',(-3.51599860018384,-1.18514270861187,
4.13977663726978));
#41894=CARTESIAN_POINT('Ctrl Pts',(-3.4836881878147,-1.06847604194516,4.18318196651927));
#41895=CARTESIAN_POINT('Ctrl Pts',(-3.41896855796307,-0.794772684000852,
4.27583752114506));
#41896=CARTESIAN_POINT('Ctrl Pts',(-3.38579619940448,-0.636309800095194,
4.32868261121145));
#41897=CARTESIAN_POINT('Ctrl Pts',(-3.35021088767458,-0.319434907277156,
4.39795974131661));
#41898=CARTESIAN_POINT('Ctrl Pts',(-3.33895965600612,-0.158333333333331,
4.42451926233091));
#41899=CARTESIAN_POINT('Ctrl Pts',(-3.35416769676493,0.158333333333334,
4.44259925854089));
#41900=CARTESIAN_POINT('Ctrl Pts',(-3.3798535907571,0.319434907277166,4.43309851697437));
#41901=CARTESIAN_POINT('Ctrl Pts',(-3.44799190268464,0.636309800095204,
4.40272918236057));
#41902=CARTESIAN_POINT('Ctrl Pts',(-3.49965209936142,0.794772684000837,
4.37224889095022));
#41903=CARTESIAN_POINT('Ctrl Pts',(-3.59461129635381,1.06847604194586,4.31581467525283));
#41904=CARTESIAN_POINT('Ctrl Pts',(-3.63986382502676,1.18514270861326,4.28787725427043));
#41905=CARTESIAN_POINT('Ctrl Pts',(-3.68926456457954,1.3000000000022,4.25643069318731));
#41906=CARTESIAN_POINT('Ctrl Pts',(-3.51930456141979,-1.30000000000012,
4.10610119875616));
#41907=CARTESIAN_POINT('Ctrl Pts',(-3.47679339664398,-1.18514270861187,
4.15620402739542));
#41908=CARTESIAN_POINT('Ctrl Pts',(-3.44027748426465,-1.06847604194516,
4.20225635359855));
#41909=CARTESIAN_POINT('Ctrl Pts',(-3.36976865406716,-0.794772684000851,
4.29928896893633));
#41910=CARTESIAN_POINT('Ctrl Pts',(-3.33846439006812,-0.636309800095195,
4.35256429357893));
#41911=CARTESIAN_POINT('Ctrl Pts',(-3.30350362107075,-0.319434907277157,
4.42313821531253));
#41912=CARTESIAN_POINT('Ctrl Pts',(-3.2950140387051,-0.158333333333331,
4.44979162859018));
#41913=CARTESIAN_POINT('Ctrl Pts',(-3.30974033139481,0.158333333333334,
4.46726854132644));
#41914=CARTESIAN_POINT('Ctrl Pts',(-3.33228828599363,0.319434907277166,
4.4573449276509));
#41915=CARTESIAN_POINT('Ctrl Pts',(-3.39860595874978,0.636309800095204,
4.42389203444187));
#41916=CARTESIAN_POINT('Ctrl Pts',(-3.44700228067872,0.794772684000838,
4.3906779224758));
#41917=CARTESIAN_POINT('Ctrl Pts',(-3.54746472936924,1.06847604194586,4.32916181010615));
#41918=CARTESIAN_POINT('Ctrl Pts',(-3.59712526653284,1.18514270861326,4.29874098381307));
#41919=CARTESIAN_POINT('Ctrl Pts',(-3.65295986932236,1.3000000000022,4.26452737687521));
#41920=CARTESIAN_POINT('Ctrl Pts',(-3.49661091395701,-1.30000000000013,
4.11413655268895));
#41921=CARTESIAN_POINT('Ctrl Pts',(-3.45011915750405,-1.18514270861187,
4.16652547909603));
#41922=CARTESIAN_POINT('Ctrl Pts',(-3.41086452260909,-1.06847604194516,
4.21449705032962));
#41923=CARTESIAN_POINT('Ctrl Pts',(-3.33689766171916,-0.794772684000854,
4.31511600241951));
#41924=CARTESIAN_POINT('Ctrl Pts',(-3.30782791401481,-0.636309800095197,
4.37008747128378));
#41925=CARTESIAN_POINT('Ctrl Pts',(-3.27333584165758,-0.319434907277158,
4.44160920954462));
#41926=CARTESIAN_POINT('Ctrl Pts',(-3.26576691168355,-0.158333333333332,
4.46697499616923));
#41927=CARTESIAN_POINT('Ctrl Pts',(-3.27995148589563,0.158333333333334,
4.48374512833731));
#41928=CARTESIAN_POINT('Ctrl Pts',(-3.30069357725885,0.319434907277166,
4.47396915205645));
#41929=CARTESIAN_POINT('Ctrl Pts',(-3.36613878105895,0.636309800095205,
4.43901119610255));
#41930=CARTESIAN_POINT('Ctrl Pts',(-3.41270262200034,0.794772684000842,
4.40457380667172));
#41931=CARTESIAN_POINT('Ctrl Pts',(-3.51714301368748,1.06847604194587,4.34010113139227));
#41932=CARTESIAN_POINT('Ctrl Pts',(-3.56984368213801,1.18514270861327,4.30813563801336));
#41933=CARTESIAN_POINT('Ctrl Pts',(-3.63003664337549,1.3000000000022,4.27211248343603));
#41934=CARTESIAN_POINT('Ctrl Pts',(-3.48026786811643,-1.30000000000013,
4.12106457332582));
#41935=CARTESIAN_POINT('Ctrl Pts',(-3.43093260187443,-1.18514270861187,
4.17522456495776));
#41936=CARTESIAN_POINT('Ctrl Pts',(-3.38969237482348,-1.06847604194516,
4.22461579029388));
#41937=CARTESIAN_POINT('Ctrl Pts',(-3.31312036019499,-0.794772684000855,
4.32770259736936));
#41938=CARTESIAN_POINT('Ctrl Pts',(-3.2852530347015,-0.636309800095197,
4.38320513518303));
#41939=CARTESIAN_POINT('Ctrl Pts',(-3.25127324659019,-0.319434907277158,
4.45562741250426));
#41940=CARTESIAN_POINT('Ctrl Pts',(-3.24509750630817,-0.158333333333332,
4.4811080411042));
#41941=CARTESIAN_POINT('Ctrl Pts',(-3.25898349185269,0.158333333333334,
4.49753113167441));
#41942=CARTESIAN_POINT('Ctrl Pts',(-3.27800174177641,0.319434907277166,
4.48731914643));
#41943=CARTESIAN_POINT('Ctrl Pts',(-3.34239176789908,0.636309800095205,
4.45070104795185));
#41944=CARTESIAN_POINT('Ctrl Pts',(-3.38742168602886,0.794772684000841,
4.41514966687841));
#41945=CARTESIAN_POINT('Ctrl Pts',(-3.49425950296388,1.06847604194587,4.34772615902328));
#41946=CARTESIAN_POINT('Ctrl Pts',(-3.54892812844116,1.18514270861327,4.31421384968507));
#41947=CARTESIAN_POINT('Ctrl Pts',(-3.61201924717566,1.30000000000221,4.27637436927206));
#41948=CARTESIAN_POINT('Ctrl Pts',(-3.46382778992357,-1.30000000000013,
4.12803241400119));
#41949=CARTESIAN_POINT('Ctrl Pts',(-3.41146750570951,-1.18514270861187,
4.18402399680214));
#41950=CARTESIAN_POINT('Ctrl Pts',(-3.3681873035808,-1.06847604194516,4.23499486878468));
#41951=CARTESIAN_POINT('Ctrl Pts',(-3.28917818457007,-0.794772684000853,
4.3411489333721));
#41952=CARTESIAN_POINT('Ctrl Pts',(-3.26373615514406,-0.636309800095198,
4.39887115096453));
#41953=CARTESIAN_POINT('Ctrl Pts',(-3.22952693615524,-0.319434907277159,
4.47121868105204));
#41954=CARTESIAN_POINT('Ctrl Pts',(-3.22229030655688,-0.158333333333332,
4.49332297409223));
#41955=CARTESIAN_POINT('Ctrl Pts',(-3.23547273092916,0.158333333333335,
4.50884588070143));
#41956=CARTESIAN_POINT('Ctrl Pts',(-3.25440588827726,0.319434907277168,
4.50056659336102));
#41957=CARTESIAN_POINT('Ctrl Pts',(-3.31849342097841,0.636309800095207,
4.46329660824968));
#41958=CARTESIAN_POINT('Ctrl Pts',(-3.36175685995594,0.794772684000843,
4.4262982431313));
#41959=CARTESIAN_POINT('Ctrl Pts',(-3.47143153257499,1.06847604194587,4.35623152583864));
#41960=CARTESIAN_POINT('Ctrl Pts',(-3.52832586892842,1.18514270861327,4.32133830834972));
#41961=CARTESIAN_POINT('Ctrl Pts',(-3.59464043970546,1.3000000000022,4.28188115906025));
#41962=CARTESIAN_POINT('Ctrl Pts',(-3.45023815468823,-1.30000000000013,
4.13378441999163));
#41963=CARTESIAN_POINT('Ctrl Pts',(-3.3960810685282,-1.18514270861187,4.19189169633376));
#41964=CARTESIAN_POINT('Ctrl Pts',(-3.35137666661798,-1.06847604194516,
4.24424595181811));
#41965=CARTESIAN_POINT('Ctrl Pts',(-3.26993814674045,-0.794772684000854,
4.35190412635052));
#41966=CARTESIAN_POINT('Ctrl Pts',(-3.24392557829603,-0.636309800095196,
4.40789981041734));
#41967=CARTESIAN_POINT('Ctrl Pts',(-3.20919341227392,-0.319434907277158,
4.47958200878044));
#41968=CARTESIAN_POINT('Ctrl Pts',(-3.20258671706639,-0.158333333333332,
4.50096078898671));
#41969=CARTESIAN_POINT('Ctrl Pts',(-3.21611606139103,0.158333333333334,
4.51699295065536));
#41970=CARTESIAN_POINT('Ctrl Pts',(-3.23530081306674,0.319434907277167,
4.51069926136688));
#41971=CARTESIAN_POINT('Ctrl Pts',(-3.29952898420167,0.636309800095206,
4.47360253689704));
#41972=CARTESIAN_POINT('Ctrl Pts',(-3.34140203455991,0.79477268400084,4.43565677950861));
#41973=CARTESIAN_POINT('Ctrl Pts',(-3.4532367242705,1.06847604194587,4.36364692568768));
#41974=CARTESIAN_POINT('Ctrl Pts',(-3.51179788486564,1.18514270861327,4.32765145244664));
#41975=CARTESIAN_POINT('Ctrl Pts',(-3.5805111127637,1.3000000000022,4.28683090345569));
#41976=CARTESIAN_POINT('Ctrl Pts',(-3.43424348033285,-1.30000000000013,
4.14136931464995));
#41977=CARTESIAN_POINT('Ctrl Pts',(-3.37761591825326,-1.18514270861187,
4.20224824815626));
#41978=CARTESIAN_POINT('Ctrl Pts',(-3.33084628881046,-1.06847604194516,
4.25630452445111));
#41979=CARTESIAN_POINT('Ctrl Pts',(-3.24557288502897,-0.794772684000852,
4.36542363358686));
#41980=CARTESIAN_POINT('Ctrl Pts',(-3.21802118521138,-0.636309800095197,
4.41840494779706));
#41981=CARTESIAN_POINT('Ctrl Pts',(-3.18186739102292,-0.319434907277158,
4.48844291347954));
#41982=CARTESIAN_POINT('Ctrl Pts',(-3.17601304436626,-0.158333333333332,
4.50871929661483));
#41983=CARTESIAN_POINT('Ctrl Pts',(-3.18946211499878,0.158333333333334,
4.5246793556689));
#41984=CARTESIAN_POINT('Ctrl Pts',(-3.20799122165873,0.319434907277167,
4.51968844978846));
#41985=CARTESIAN_POINT('Ctrl Pts',(-3.27311701935999,0.636309800095206,
4.48353404979024));
#41986=CARTESIAN_POINT('Ctrl Pts',(-3.31545583686005,0.794772684000839,
4.44710357338116));
#41987=CARTESIAN_POINT('Ctrl Pts',(-3.43107074058742,1.06847604194587,4.37346615706425));
#41988=CARTESIAN_POINT('Ctrl Pts',(-3.49192164587793,1.18514270861327,4.3360203117187));
#41989=CARTESIAN_POINT('Ctrl Pts',(-3.5635780485896,1.30000000000221,4.29300353001613));
#41990=CARTESIAN_POINT('Ctrl Pts',(-3.42329004793798,-1.30000000000013,
4.14644476697421));
#41991=CARTESIAN_POINT('Ctrl Pts',(-3.36577675441716,-1.18514270861187,
4.2103224238295));
#41992=CARTESIAN_POINT('Ctrl Pts',(-3.31797563071955,-1.06847604194516,
4.26590655668718));
#41993=CARTESIAN_POINT('Ctrl Pts',(-3.22998252760054,-0.794772684000851,
4.3751573236078));
#41994=CARTESIAN_POINT('Ctrl Pts',(-3.19945051412029,-0.636309800095197,
4.42226516939946));
#41995=CARTESIAN_POINT('Ctrl Pts',(-3.16161671560352,-0.319434907277159,
4.48925446130297));
#41996=CARTESIAN_POINT('Ctrl Pts',(-3.15675867153595,-0.158333333333332,
4.50911671221123));
#41997=CARTESIAN_POINT('Ctrl Pts',(-3.17014714941586,0.158333333333334,
4.52493089062661));
#41998=CARTESIAN_POINT('Ctrl Pts',(-3.18775359149336,0.319434907277167,
4.52028525838109));
#41999=CARTESIAN_POINT('Ctrl Pts',(-3.25416255205695,0.636309800095206,
4.48672549544153));
#42000=CARTESIAN_POINT('Ctrl Pts',(-3.29862160463215,0.794772684000841,
4.45543705365187));
#42001=CARTESIAN_POINT('Ctrl Pts',(-3.41699686809868,1.06847604194587,4.38170451193648));
#42002=CARTESIAN_POINT('Ctrl Pts',(-3.47911206103844,1.18514270861327,4.3429415809095));
#42003=CARTESIAN_POINT('Ctrl Pts',(-3.55210218159892,1.30000000000221,4.29733180410432));
#42004=CARTESIAN_POINT('Ctrl Pts',(-3.41475847117046,-1.30000000000013,
4.14754376664529));
#42005=CARTESIAN_POINT('Ctrl Pts',(-3.35748906958223,-1.18514270861187,
4.21136081832333));
#42006=CARTESIAN_POINT('Ctrl Pts',(-3.30972802388308,-1.06847604194516,
4.26660243158902));
#42007=CARTESIAN_POINT('Ctrl Pts',(-3.22135665799747,-0.794772684000851,
4.37441063103652));
#42008=CARTESIAN_POINT('Ctrl Pts',(-3.18969432988981,-0.636309800095197,
4.41921512013816));
#42009=CARTESIAN_POINT('Ctrl Pts',(-3.15117622767193,-0.319434907277159,
4.48466289159347));
#42010=CARTESIAN_POINT('Ctrl Pts',(-3.14628700527777,-0.158333333333332,
4.50456719074197));
#42011=CARTESIAN_POINT('Ctrl Pts',(-3.15959962456678,0.158333333333334,
4.52015701991036));
#42012=CARTESIAN_POINT('Ctrl Pts',(-3.17704490789093,0.319434907277167,
4.51499029662226));
#42013=CARTESIAN_POINT('Ctrl Pts',(-3.24422091196343,0.636309800095206,
4.48303386330206));
#42014=CARTESIAN_POINT('Ctrl Pts',(-3.29031662464092,0.794772684000841,
4.45500700215256));
#42015=CARTESIAN_POINT('Ctrl Pts',(-3.40898836153085,1.06847604194587,4.38258700702605));
#42016=CARTESIAN_POINT('Ctrl Pts',(-3.47090355779054,1.18514270861327,4.34388949955489));
#42017=CARTESIAN_POINT('Ctrl Pts',(-3.54336535263131,1.30000000000221,4.29784241707766));
#42018=CARTESIAN_POINT('Ctrl Pts',(-3.4147584711704,-1.3,4.14754376664537));
#42019=CARTESIAN_POINT('Ctrl Pts',(-3.35748906958219,-1.18514270861178,
4.21136081832337));
#42020=CARTESIAN_POINT('Ctrl Pts',(-3.30972802388306,-1.06847604194512,
4.26660243158903));
#42021=CARTESIAN_POINT('Ctrl Pts',(-3.22135665799746,-0.794772684000851,
4.37441063103652));
#42022=CARTESIAN_POINT('Ctrl Pts',(-3.18969432988981,-0.636309800095197,
4.41921512013816));
#42023=CARTESIAN_POINT('Ctrl Pts',(-3.15117622767193,-0.319434907277159,
4.48466289159347));
#42024=CARTESIAN_POINT('Ctrl Pts',(-3.14628700527777,-0.158333333333332,
4.50456719074197));
#42025=CARTESIAN_POINT('Ctrl Pts',(-3.15959962456677,0.158333333333334,
4.52015701991036));
#42026=CARTESIAN_POINT('Ctrl Pts',(-3.17704490789093,0.319434907277167,
4.51499029662225));
#42027=CARTESIAN_POINT('Ctrl Pts',(-3.24422091196343,0.636309800095206,
4.48303386330206));
#42028=CARTESIAN_POINT('Ctrl Pts',(-3.29031662464091,0.79477268400084,4.45500700215256));
#42029=CARTESIAN_POINT('Ctrl Pts',(-3.40898836153052,1.06847604194511,4.38258700702625));
#42030=CARTESIAN_POINT('Ctrl Pts',(-3.47090355778974,1.18514270861178,4.34388949955539));
#42031=CARTESIAN_POINT('Ctrl Pts',(-3.54336535262991,1.3,4.29784241707854));
#42032=CARTESIAN_POINT('',(-3.81821580258393,-1.2,4.04980507192042));
#42033=CARTESIAN_POINT('Ctrl Pts',(-3.81821580258393,-1.2,4.04980507192042));
#42034=CARTESIAN_POINT('Ctrl Pts',(-3.79663896512829,-1.21681884435473,
4.05008069226545));
#42035=CARTESIAN_POINT('Ctrl Pts',(-3.77476731607508,-1.23326256677479,
4.04950363407841));
#42036=CARTESIAN_POINT('Ctrl Pts',(-3.73353702923591,-1.26513182561291,
4.04995352778724));
#42037=CARTESIAN_POINT('Ctrl Pts',(-3.70428420443725,-1.28769911124913,
4.05034302515998));
#42038=CARTESIAN_POINT('Ctrl Pts',(-3.68874885778907,-1.30000000000011,
4.05109036900727));
#42039=CARTESIAN_POINT('',(-3.9159353778062,-0.653834841366393,4.17213769856117));
#42040=CARTESIAN_POINT('Ctrl Pts',(-3.91593537783278,-0.653834841365109,
4.17213769853421));
#42041=CARTESIAN_POINT('Ctrl Pts',(-3.90613053706298,-0.717011608251444,
4.1594570945233));
#42042=CARTESIAN_POINT('Ctrl Pts',(-3.89800867385936,-0.763800251277795,
4.14904820577532));
#42043=CARTESIAN_POINT('Ctrl Pts',(-3.86595009357095,-0.949632484189618,
4.10837225465677));
#42044=CARTESIAN_POINT('Ctrl Pts',(-3.84681431306324,-1.05559152095179,
4.08446809663331));
#42045=CARTESIAN_POINT('Ctrl Pts',(-3.81821580258393,-1.2,4.04980507192042));
#42046=CARTESIAN_POINT('',(-3.99970644340963,0.653834841531101,4.28369268310978));
#42047=CARTESIAN_POINT('Ctrl Pts',(-3.99970644340963,0.6538348415311,4.28369268310978));
#42048=CARTESIAN_POINT('Ctrl Pts',(-3.95893262294855,0.57599820463906,4.29175829619443));
#42049=CARTESIAN_POINT('Ctrl Pts',(-3.92430183446496,0.493642228123361,
4.29784729680954));
#42050=CARTESIAN_POINT('Ctrl Pts',(-3.87408300678057,0.338139647427855,
4.30417357553207));
#42051=CARTESIAN_POINT('Ctrl Pts',(-3.85621798073113,0.265662533938239,
4.30517989396827));
#42052=CARTESIAN_POINT('Ctrl Pts',(-3.83201526376916,0.129716559933793,
4.30225619578907));
#42053=CARTESIAN_POINT('Ctrl Pts',(-3.82438757785205,0.0666261450806326,
4.29904673876848));
#42054=CARTESIAN_POINT('Ctrl Pts',(-3.81608778926841,-0.0595425750673727,
4.28861323503182));
#42055=CARTESIAN_POINT('Ctrl Pts',(-3.8153399913931,-0.122776762279469,
4.28132116280713));
#42056=CARTESIAN_POINT('Ctrl Pts',(-3.82180214781733,-0.260118331359305,
4.26160750787843));
#42057=CARTESIAN_POINT('Ctrl Pts',(-3.83048941390645,-0.333929032933066,
4.24848954767565));
#42058=CARTESIAN_POINT('Ctrl Pts',(-3.86113063405387,-0.491198314909897,
4.21574382130922));
#42059=CARTESIAN_POINT('Ctrl Pts',(-3.88506981710094,-0.574355267118962,
4.19514942756914));
#42060=CARTESIAN_POINT('Ctrl Pts',(-3.91593537774962,-0.653834841383305,
4.17213769854369));
#42061=CARTESIAN_POINT('',(-3.95679688799543,1.2,4.22573397505373));
#42062=CARTESIAN_POINT('Ctrl Pts',(-3.95679688799543,1.2,4.22573397505373));
#42063=CARTESIAN_POINT('Ctrl Pts',(-3.96321789915741,1.1438091496454,4.23427612857006));
#42064=CARTESIAN_POINT('Ctrl Pts',(-3.97238904100963,1.06112401913765,4.24651281010962));
#42065=CARTESIAN_POINT('Ctrl Pts',(-3.99275128256726,0.796649264003109,
4.27414929727633));
#42066=CARTESIAN_POINT('Ctrl Pts',(-3.99594086764057,0.739302270217887,
4.27852820761727));
#42067=CARTESIAN_POINT('Ctrl Pts',(-3.99970644340963,0.653834841531101,
4.28369268310978));
#42068=CARTESIAN_POINT('Ctrl Pts',(-3.83164255233655,1.30000000000218,4.22661550567326));
#42069=CARTESIAN_POINT('Ctrl Pts',(-3.85239777077144,1.28312717632915,4.22583975108101));
#42070=CARTESIAN_POINT('Ctrl Pts',(-3.87333078582076,1.26644671368672,4.22568281356069));
#42071=CARTESIAN_POINT('Ctrl Pts',(-3.92060649073197,1.2288596279006,4.22565598187284));
#42072=CARTESIAN_POINT('Ctrl Pts',(-3.93585305697864,1.21625420944408,4.22492296870073));
#42073=CARTESIAN_POINT('Ctrl Pts',(-3.95679688799543,1.2,4.22573397505373));
#42074=CARTESIAN_POINT('Ctrl Pts',(-3.4147584711704,-1.3,4.14754376664537));
#42075=CARTESIAN_POINT('Ctrl Pts',(-3.35748906958219,-1.18514270861178,
4.21136081832337));
#42076=CARTESIAN_POINT('Ctrl Pts',(-3.30972802388306,-1.06847604194512,
4.26660243158904));
#42077=CARTESIAN_POINT('Ctrl Pts',(-3.22135665799747,-0.794772684000851,
4.37441063103652));
#42078=CARTESIAN_POINT('Ctrl Pts',(-3.18969432988981,-0.636309800095197,
4.41921512013816));
#42079=CARTESIAN_POINT('Ctrl Pts',(-3.15117622767193,-0.319434907277159,
4.48466289159347));
#42080=CARTESIAN_POINT('Ctrl Pts',(-3.14628700527777,-0.158333333333332,
4.50456719074198));
#42081=CARTESIAN_POINT('Ctrl Pts',(-3.15959962456678,0.158333333333334,
4.52015701991036));
#42082=CARTESIAN_POINT('Ctrl Pts',(-3.17704490789093,0.319434907277167,
4.51499029662225));
#42083=CARTESIAN_POINT('Ctrl Pts',(-3.24422091196343,0.636309800095206,
4.48303386330206));
#42084=CARTESIAN_POINT('Ctrl Pts',(-3.29031662464091,0.79477268400084,4.45500700215256));
#42085=CARTESIAN_POINT('Ctrl Pts',(-3.40898836153052,1.06847604194511,4.38258700702625));
#42086=CARTESIAN_POINT('Ctrl Pts',(-3.47090355778975,1.18514270861178,4.34388949955539));
#42087=CARTESIAN_POINT('Ctrl Pts',(-3.54336535262991,1.3,4.29784241707854));
#42088=CARTESIAN_POINT('Ctrl Pts',(-3.3620529124905,-1.3,4.09149705970477));
#42089=CARTESIAN_POINT('Ctrl Pts',(-3.30608359416459,-1.18514270861178,
4.15645896441576));
#42090=CARTESIAN_POINT('Ctrl Pts',(-3.25925709076723,-1.06847604194512,
4.21246371570874));
#42091=CARTESIAN_POINT('Ctrl Pts',(-3.17220023180818,-0.794772684000851,
4.32115307863962));
#42092=CARTESIAN_POINT('Ctrl Pts',(-3.14019479937607,-0.636309800095197,
4.36532726831211));
#42093=CARTESIAN_POINT('Ctrl Pts',(-3.10158167219449,-0.319434907277159,
4.43011499929132));
#42094=CARTESIAN_POINT('Ctrl Pts',(-3.09600154123356,-0.158333333333332,
4.44898774758743));
#42095=CARTESIAN_POINT('Ctrl Pts',(-3.10958091369845,0.158333333333334,
4.46433739111742));
#42096=CARTESIAN_POINT('Ctrl Pts',(-3.12797987732075,0.319434907277167,
4.45996561795205));
#42097=CARTESIAN_POINT('Ctrl Pts',(-3.19580237328514,0.636309800095206,
4.42817268205552));
#42098=CARTESIAN_POINT('Ctrl Pts',(-3.24248906837777,0.79477268400084,4.40055292989982));
#42099=CARTESIAN_POINT('Ctrl Pts',(-3.36042187227873,1.06847604194511,4.32673352218863));
#42100=CARTESIAN_POINT('Ctrl Pts',(-3.42167579733126,1.18514270861178,4.28702682229126));
#42101=CARTESIAN_POINT('Ctrl Pts',(-3.49313490646867,1.3,4.23956710881605));
#42102=CARTESIAN_POINT('Ctrl Pts',(-3.3093473538106,-1.3,4.03545035276417));
#42103=CARTESIAN_POINT('Ctrl Pts',(-3.25467811874699,-1.18514270861178,
4.10155711050815));
#42104=CARTESIAN_POINT('Ctrl Pts',(-3.20878615765139,-1.06847604194512,
4.15832499982844));
#42105=CARTESIAN_POINT('Ctrl Pts',(-3.12304380561889,-0.794772684000851,
4.26789552624273));
#42106=CARTESIAN_POINT('Ctrl Pts',(-3.09069526886232,-0.636309800095197,
4.31143941648607));
#42107=CARTESIAN_POINT('Ctrl Pts',(-3.05198711671704,-0.319434907277159,
4.37556710698916));
#42108=CARTESIAN_POINT('Ctrl Pts',(-3.04571607718935,-0.158333333333332,
4.39340830443289));
#42109=CARTESIAN_POINT('Ctrl Pts',(-3.05956220283012,0.158333333333334,
4.40851776232448));
#42110=CARTESIAN_POINT('Ctrl Pts',(-3.07891484675056,0.319434907277167,
4.40494093928184));
#42111=CARTESIAN_POINT('Ctrl Pts',(-3.14738383460685,0.636309800095206,
4.37331150080897));
#42112=CARTESIAN_POINT('Ctrl Pts',(-3.19466151211463,0.79477268400084,4.34609885764707));
#42113=CARTESIAN_POINT('Ctrl Pts',(-3.31185538302693,1.06847604194511,4.27088003735101));
#42114=CARTESIAN_POINT('Ctrl Pts',(-3.37244803687278,1.18514270861178,4.23016414502714));
#42115=CARTESIAN_POINT('Ctrl Pts',(-3.44290446030743,1.3,4.18129180055356));
#42116=CARTESIAN_POINT('Ctrl Pts',(-3.25664179513071,-1.3,3.97940364582358));
#42117=CARTESIAN_POINT('Ctrl Pts',(-3.20327264332939,-1.18514270861178,
4.04665525660054));
#42118=CARTESIAN_POINT('Ctrl Pts',(-3.15831522453555,-1.06847604194512,
4.10418628394814));
#42119=CARTESIAN_POINT('Ctrl Pts',(-3.0738873794296,-0.794772684000851,
4.21463797384583));
#42120=CARTESIAN_POINT('Ctrl Pts',(-3.04119573834857,-0.636309800095197,
4.25755156466003));
#42121=CARTESIAN_POINT('Ctrl Pts',(-3.0023925612396,-0.319434907277159,
4.321019214687));
#42122=CARTESIAN_POINT('Ctrl Pts',(-2.99543061314513,-0.158333333333332,
4.33782886127834));
#42123=CARTESIAN_POINT('Ctrl Pts',(-3.00954349196179,0.158333333333334,
4.35269813353154));
#42124=CARTESIAN_POINT('Ctrl Pts',(-3.02984981618038,0.319434907277167,
4.34991626061163));
#42125=CARTESIAN_POINT('Ctrl Pts',(-3.09896529592856,0.636309800095206,
4.31845031956243));
#42126=CARTESIAN_POINT('Ctrl Pts',(-3.14683395585149,0.79477268400084,4.29164478539433));
#42127=CARTESIAN_POINT('Ctrl Pts',(-3.26328889377514,1.06847604194511,4.21502655251339));
#42128=CARTESIAN_POINT('Ctrl Pts',(-3.32322027641429,1.18514270861178,4.17330146776301));
#42129=CARTESIAN_POINT('Ctrl Pts',(-3.39267401414619,1.3,4.12301649229107));
#42130=CARTESIAN_POINT('Ctrl Pts',(-3.2566417951307,-1.3,3.97940364582357));
#42131=CARTESIAN_POINT('Ctrl Pts',(-3.20327264332939,-1.18514270861178,
4.04665525660054));
#42132=CARTESIAN_POINT('Ctrl Pts',(-3.15831522453555,-1.06847604194512,
4.10418628394814));
#42133=CARTESIAN_POINT('Ctrl Pts',(-3.0738873794296,-0.794772684000851,
4.21463797384583));
#42134=CARTESIAN_POINT('Ctrl Pts',(-3.04119573834857,-0.636309800095197,
4.25755156466003));
#42135=CARTESIAN_POINT('Ctrl Pts',(-3.0023925612396,-0.319434907277159,
4.321019214687));
#42136=CARTESIAN_POINT('Ctrl Pts',(-2.99543061314513,-0.158333333333332,
4.33782886127834));
#42137=CARTESIAN_POINT('Ctrl Pts',(-3.00954349196179,0.158333333333334,
4.35269813353154));
#42138=CARTESIAN_POINT('Ctrl Pts',(-3.02984981618038,0.319434907277167,
4.34991626061163));
#42139=CARTESIAN_POINT('Ctrl Pts',(-3.09896529592856,0.636309800095206,
4.31845031956243));
#42140=CARTESIAN_POINT('Ctrl Pts',(-3.14683395585149,0.79477268400084,4.29164478539433));
#42141=CARTESIAN_POINT('Ctrl Pts',(-3.26328889377514,1.06847604194511,4.21502655251339));
#42142=CARTESIAN_POINT('Ctrl Pts',(-3.32322027641429,1.18514270861178,4.17330146776301));
#42143=CARTESIAN_POINT('Ctrl Pts',(-3.39267401414619,1.3,4.12301649229107));
#42144=CARTESIAN_POINT('Ctrl Pts',(-3.25664179513354,-1.30000000000611,
3.97940364582));
#42145=CARTESIAN_POINT('Ctrl Pts',(-3.20327264333099,-1.18514270861592,
4.0466552565985));
#42146=CARTESIAN_POINT('Ctrl Pts',(-3.15831522453619,-1.06847604194722,
4.10418628394729));
#42147=CARTESIAN_POINT('Ctrl Pts',(-3.0738873794296,-0.794772684000851,
4.21463797384583));
#42148=CARTESIAN_POINT('Ctrl Pts',(-3.04119573834857,-0.636309800095196,
4.25755156466002));
#42149=CARTESIAN_POINT('Ctrl Pts',(-3.0023925612396,-0.319434907277159,
4.321019214687));
#42150=CARTESIAN_POINT('Ctrl Pts',(-2.99543061314513,-0.158333333333332,
4.33782886127834));
#42151=CARTESIAN_POINT('Ctrl Pts',(-3.00954349196179,0.158333333333335,
4.35269813353154));
#42152=CARTESIAN_POINT('Ctrl Pts',(-3.02984981618038,0.319434907277167,
4.34991626061163));
#42153=CARTESIAN_POINT('Ctrl Pts',(-3.09896529592856,0.636309800095206,
4.31845031956243));
#42154=CARTESIAN_POINT('Ctrl Pts',(-3.1468339558515,0.79477268400084,4.29164478539433));
#42155=CARTESIAN_POINT('Ctrl Pts',(-3.26328889377516,1.06847604194515,4.21502655251339));
#42156=CARTESIAN_POINT('Ctrl Pts',(-3.32322027641433,1.18514270861185,4.17330146776299));
#42157=CARTESIAN_POINT('Ctrl Pts',(-3.39267401414626,1.30000000000011,4.12301649229103));
#42158=CARTESIAN_POINT('Ctrl Pts',(-3.25806285817801,-1.30000000000611,
3.97076805174582));
#42159=CARTESIAN_POINT('Ctrl Pts',(-3.205073391371,-1.18514270861592,4.03859080490488));
#42160=CARTESIAN_POINT('Ctrl Pts',(-3.1600300020756,-1.06847604194722,4.09631389470334));
#42161=CARTESIAN_POINT('Ctrl Pts',(-3.07432779056413,-0.794772684000851,
4.20633353680762));
#42162=CARTESIAN_POINT('Ctrl Pts',(-3.03856351369519,-0.636309800095196,
4.24727850529637));
#42163=CARTESIAN_POINT('Ctrl Pts',(-2.99824596803585,-0.319434907277159,
4.3098157201942));
#42164=CARTESIAN_POINT('Ctrl Pts',(-2.99178541067128,-0.158333333333332,
4.32684011158175));
#42165=CARTESIAN_POINT('Ctrl Pts',(-3.00611348034728,0.158333333333335,
4.34180827774425));
#42166=CARTESIAN_POINT('Ctrl Pts',(-3.02637472769607,0.319434907277167,
4.33905301707054));
#42167=CARTESIAN_POINT('Ctrl Pts',(-3.0969517540897,0.636309800095206,4.30842876377872));
#42168=CARTESIAN_POINT('Ctrl Pts',(-3.14699300261569,0.79477268400084,4.28298811859785));
#42169=CARTESIAN_POINT('Ctrl Pts',(-3.26484306624896,1.06847604194515,4.20689686568334));
#42170=CARTESIAN_POINT('Ctrl Pts',(-3.32511928141128,1.18514270861185,4.16516772553438));
#42171=CARTESIAN_POINT('Ctrl Pts',(-3.39465878596431,1.30000000000011,4.11464652916436));
#42172=CARTESIAN_POINT('Ctrl Pts',(-3.26355683794006,-1.30000000000611,
3.95979817224215));
#42173=CARTESIAN_POINT('Ctrl Pts',(-3.21328208042939,-1.18514270861592,
4.0265607791208));
#42174=CARTESIAN_POINT('Ctrl Pts',(-3.16968027363,-1.06847604194722,4.08316229727592));
#42175=CARTESIAN_POINT('Ctrl Pts',(-3.08436722847501,-0.794772684000851,
4.19044897963791));
#42176=CARTESIAN_POINT('Ctrl Pts',(-3.04372887954816,-0.636309800095196,
4.22876197668635));
#42177=CARTESIAN_POINT('Ctrl Pts',(-3.00097363294721,-0.319434907277158,
4.28975854866143));
#42178=CARTESIAN_POINT('Ctrl Pts',(-2.9940717486982,-0.158333333333332,
4.30766530460587));
#42179=CARTESIAN_POINT('Ctrl Pts',(-3.00853457043408,0.158333333333334,
4.32270439001546));
#42180=CARTESIAN_POINT('Ctrl Pts',(-3.02930099488942,0.319434907277168,
4.31898820290654));
#42181=CARTESIAN_POINT('Ctrl Pts',(-3.10273462440665,0.636309800095207,
4.29035353222686));
#42182=CARTESIAN_POINT('Ctrl Pts',(-3.15832171757233,0.794772684000839,
4.2685072783921));
#42183=CARTESIAN_POINT('Ctrl Pts',(-3.27575339640767,1.06847604194515,4.19510813771776));
#42184=CARTESIAN_POINT('Ctrl Pts',(-3.33439709308209,1.18514270861185,4.15424263112017));
#42185=CARTESIAN_POINT('Ctrl Pts',(-3.40085266393565,1.30000000000011,4.10428338621672));
#42186=CARTESIAN_POINT('Ctrl Pts',(-3.27139143945092,-1.30000000000611,
3.94354916079341));
#42187=CARTESIAN_POINT('Ctrl Pts',(-3.2236147785624,-1.18514270861592,4.00762409194011));
#42188=CARTESIAN_POINT('Ctrl Pts',(-3.1817037058285,-1.06847604194722,4.06211089398943));
#42189=CARTESIAN_POINT('Ctrl Pts',(-3.09843142557671,-0.794772684000852,
4.16583581045613));
#42190=CARTESIAN_POINT('Ctrl Pts',(-3.05636248871783,-0.636309800095195,
4.20354929061984));
#42191=CARTESIAN_POINT('Ctrl Pts',(-3.0127970512512,-0.319434907277157,
4.26358364111853));
#42192=CARTESIAN_POINT('Ctrl Pts',(-3.00456157037485,-0.158333333333332,
4.28203282078132));
#42193=CARTESIAN_POINT('Ctrl Pts',(-3.01907439990511,0.158333333333334,
4.29714778439741));
#42194=CARTESIAN_POINT('Ctrl Pts',(-3.04094799380849,0.319434907277168,
4.29274048634797));
#42195=CARTESIAN_POINT('Ctrl Pts',(-3.11585675460528,0.636309800095206,
4.2656800191969));
#42196=CARTESIAN_POINT('Ctrl Pts',(-3.17432845417982,0.794772684000837,
4.24572071661066));
#42197=CARTESIAN_POINT('Ctrl Pts',(-3.28992154460439,1.06847604194514,4.17598916099776));
#42198=CARTESIAN_POINT('Ctrl Pts',(-3.34665848187483,1.18514270861185,4.13699699483715));
#42199=CARTESIAN_POINT('Ctrl Pts',(-3.41009639071706,1.30000000000011,4.08919686913195));
#42200=CARTESIAN_POINT('Ctrl Pts',(-3.27795985063405,-1.30000000000611,
3.93013440105912));
#42201=CARTESIAN_POINT('Ctrl Pts',(-3.23176837726564,-1.18514270861592,
3.99193424901875));
#42202=CARTESIAN_POINT('Ctrl Pts',(-3.19110448689979,-1.06847604194722,
4.04484845525556));
#42203=CARTESIAN_POINT('Ctrl Pts',(-3.10993258789721,-0.79477268400085,
4.14656324716606));
#42204=CARTESIAN_POINT('Ctrl Pts',(-3.06862068700424,-0.636309800095195,
4.18572618426736));
#42205=CARTESIAN_POINT('Ctrl Pts',(-3.0248287334282,-0.319434907277157,
4.24554097765999));
#42206=CARTESIAN_POINT('Ctrl Pts',(-3.01456605891873,-0.158333333333332,
4.26346731127332));
#42207=CARTESIAN_POINT('Ctrl Pts',(-3.02863558681848,0.158333333333334,
4.27820542858103));
#42208=CARTESIAN_POINT('Ctrl Pts',(-3.05144876662552,0.319434907277168,
4.27337147994046));
#42209=CARTESIAN_POINT('Ctrl Pts',(-3.12699347516112,0.636309800095206,
4.24692940859356));
#42210=CARTESIAN_POINT('Ctrl Pts',(-3.18702881370645,0.794772684000838,
4.22764105496139));
#42211=CARTESIAN_POINT('Ctrl Pts',(-3.30082919306778,1.06847604194514,4.16015384976511));
#42212=CARTESIAN_POINT('Ctrl Pts',(-3.35602879228581,1.18514270861185,4.12243609134989));
#42213=CARTESIAN_POINT('Ctrl Pts',(-3.41716802321599,1.30000000000011,4.07621328500152));
#42214=CARTESIAN_POINT('Ctrl Pts',(-3.28595994929404,-1.30000000000611,
3.91027551687813));
#42215=CARTESIAN_POINT('Ctrl Pts',(-3.2420905880153,-1.18514270861592,3.968611702584));
#42216=CARTESIAN_POINT('Ctrl Pts',(-3.20336557148759,-1.06847604194722,
4.01919298846687));
#42217=CARTESIAN_POINT('Ctrl Pts',(-3.12578750189388,-0.794772684000852,
4.11813050765343));
#42218=CARTESIAN_POINT('Ctrl Pts',(-3.08610042440403,-0.636309800095197,
4.1596488236161));
#42219=CARTESIAN_POINT('Ctrl Pts',(-3.04324732235638,-0.319434907277159,
4.22008752447184));
#42220=CARTESIAN_POINT('Ctrl Pts',(-3.0309531963189,-0.158333333333332,
4.23806527243021));
#42221=CARTESIAN_POINT('Ctrl Pts',(-3.04589376909181,0.158333333333335,
4.25365591864516));
#42222=CARTESIAN_POINT('Ctrl Pts',(-3.07203097741551,0.319434907277168,
4.25007434060128));
#42223=CARTESIAN_POINT('Ctrl Pts',(-3.14755245954411,0.636309800095207,
4.22382572574053));
#42224=CARTESIAN_POINT('Ctrl Pts',(-3.20561951200525,0.794772684000841,
4.20171706188599));
#42225=CARTESIAN_POINT('Ctrl Pts',(-3.3156778941382,1.06847604194515,4.13672768270597));
#42226=CARTESIAN_POINT('Ctrl Pts',(-3.36881803271244,1.18514270861185,4.10116981737023));
#42227=CARTESIAN_POINT('Ctrl Pts',(-3.42745811430053,1.30000000000011,4.05818558085193));
#42228=CARTESIAN_POINT('Ctrl Pts',(-3.29748931314334,-1.30000000000611,
3.88213052763613));
#42229=CARTESIAN_POINT('Ctrl Pts',(-3.2569492466075,-1.18514270861592,3.93577431355857));
#42230=CARTESIAN_POINT('Ctrl Pts',(-3.22092245125702,-1.06847604194722,
3.98315214489975));
#42231=CARTESIAN_POINT('Ctrl Pts',(-3.14811990617741,-0.794772684000853,
4.07812880461706));
#42232=CARTESIAN_POINT('Ctrl Pts',(-3.10947546491154,-0.636309800095198,
4.12194180838791));
#42233=CARTESIAN_POINT('Ctrl Pts',(-3.06883066630633,-0.319434907277159,
4.18411013249147));
#42234=CARTESIAN_POINT('Ctrl Pts',(-3.05699213746686,-0.158333333333333,
4.20506573259321));
#42235=CARTESIAN_POINT('Ctrl Pts',(-3.07256295007946,0.158333333333335,
4.22128286789914));
#42236=CARTESIAN_POINT('Ctrl Pts',(-3.0991454499967,0.319434907277169,4.21564572797228));
#42237=CARTESIAN_POINT('Ctrl Pts',(-3.17319108942998,0.636309800095209,
4.18834107734958));
#42238=CARTESIAN_POINT('Ctrl Pts',(-3.23007521026095,0.794772684000841,
4.16375332661296));
#42239=CARTESIAN_POINT('Ctrl Pts',(-3.33538101452519,1.06847604194515,4.10257677300761));
#42240=CARTESIAN_POINT('Ctrl Pts',(-3.38579275753287,1.18514270861186,4.07009490138206));
#42241=CARTESIAN_POINT('Ctrl Pts',(-3.44103326284687,1.30000000000012,4.03161222137201));
#42242=CARTESIAN_POINT('Ctrl Pts',(-3.30875979617058,-1.30000000000611,
3.85378158568818));
#42243=CARTESIAN_POINT('Ctrl Pts',(-3.27064737527123,-1.18514270861592,
3.9019632576688));
#42244=CARTESIAN_POINT('Ctrl Pts',(-3.23673083703896,-1.06847604194722,
3.94561126100005));
#42245=CARTESIAN_POINT('Ctrl Pts',(-3.16807017708734,-0.794772684000851,
4.03597319891018));
#42246=CARTESIAN_POINT('Ctrl Pts',(-3.13150462642579,-0.636309800095197,
4.0827832669738));
#42247=CARTESIAN_POINT('Ctrl Pts',(-3.09279402632734,-0.319434907277159,
4.146306287326));
#42248=CARTESIAN_POINT('Ctrl Pts',(-3.08017399670196,-0.158333333333332,
4.16914997500591));
#42249=CARTESIAN_POINT('Ctrl Pts',(-3.09653279165281,0.158333333333335,
4.18611012399854));
#42250=CARTESIAN_POINT('Ctrl Pts',(-3.12489551101782,0.319434907277167,
4.17959188889426));
#42251=CARTESIAN_POINT('Ctrl Pts',(-3.19818276051303,0.636309800095207,
4.15190830177058));
#42252=CARTESIAN_POINT('Ctrl Pts',(-3.25373505452989,0.794772684000841,
4.12473716299461));
#42253=CARTESIAN_POINT('Ctrl Pts',(-3.35449395304018,1.06847604194515,4.06769620182046));
#42254=CARTESIAN_POINT('Ctrl Pts',(-3.40226962042289,1.18514270861185,4.03845444996479));
#42255=CARTESIAN_POINT('Ctrl Pts',(-3.45420616150834,1.30000000000011,4.00466186476983));
#42256=CARTESIAN_POINT('Ctrl Pts',(-3.32193490365172,-1.30000000000611,
3.81588673765455));
#42257=CARTESIAN_POINT('Ctrl Pts',(-3.2875391164165,-1.18514270861592,3.85747304046494));
#42258=CARTESIAN_POINT('Ctrl Pts',(-3.25661318991723,-1.06847604194721,
3.8965122795001));
#42259=CARTESIAN_POINT('Ctrl Pts',(-3.19318418543743,-0.794772684000845,
3.98081650458433));
#42260=CARTESIAN_POINT('Ctrl Pts',(-3.15739817658905,-0.636309800095194,
4.02997403698598));
#42261=CARTESIAN_POINT('Ctrl Pts',(-3.12146849871559,-0.319434907277158,
4.09548539166518));
#42262=CARTESIAN_POINT('Ctrl Pts',(-3.11025557411671,-0.158333333333332,
4.12276309903158));
#42263=CARTESIAN_POINT('Ctrl Pts',(-3.1275586928241,0.158333333333334,4.14054924283807));
#42264=CARTESIAN_POINT('Ctrl Pts',(-3.15583820679444,0.319434907277169,
4.13078769536379));
#42265=CARTESIAN_POINT('Ctrl Pts',(-3.2274948848356,0.636309800095207,4.10205537276763));
#42266=CARTESIAN_POINT('Ctrl Pts',(-3.28207121742321,0.794772684000837,
4.07229262101088));
#42267=CARTESIAN_POINT('Ctrl Pts',(-3.37785103265727,1.06847604194514,4.02135229624977));
#42268=CARTESIAN_POINT('Ctrl Pts',(-3.42272547575968,1.18514270861185,3.99670187214208));
#42269=CARTESIAN_POINT('Ctrl Pts',(-3.4710148289416,1.30000000000011,3.96945120299074));
#42270=CARTESIAN_POINT('Ctrl Pts',(-3.33101474967611,-1.30000000000612,
3.78965575124489));
#42271=CARTESIAN_POINT('Ctrl Pts',(-3.29858563030453,-1.18514270861593,
3.82621989841157));
#42272=CARTESIAN_POINT('Ctrl Pts',(-3.26933486265743,-1.06847604194723,
3.86176300858679));
#42273=CARTESIAN_POINT('Ctrl Pts',(-3.20910236610783,-0.794772684000861,
3.94151590375758));
#42274=CARTESIAN_POINT('Ctrl Pts',(-3.17470958618622,-0.636309800095198,
3.99291442590289));
#42275=CARTESIAN_POINT('Ctrl Pts',(-3.14021637230009,-0.319434907277157,
4.05932035846933));
#42276=CARTESIAN_POINT('Ctrl Pts',(-3.12848888765305,-0.158333333333333,
4.08838076058789));
#42277=CARTESIAN_POINT('Ctrl Pts',(-3.14639876148324,0.158333333333335,
4.10668526422045));
#42278=CARTESIAN_POINT('Ctrl Pts',(-3.17576205181717,0.31943490727717,4.0956754808042));
#42279=CARTESIAN_POINT('Ctrl Pts',(-3.24729464621603,0.63630980009521,4.06707164949187));
#42280=CARTESIAN_POINT('Ctrl Pts',(-3.30201291805993,0.79477268400084,4.03617403304907));
#42281=CARTESIAN_POINT('Ctrl Pts',(-3.39445885475758,1.06847604194515,3.98957972939292));
#42282=CARTESIAN_POINT('Ctrl Pts',(-3.4371405930767,1.18514270861185,3.96797542650248));
#42283=CARTESIAN_POINT('Ctrl Pts',(-3.48248764917809,1.30000000000012,3.94493576828523));
#42284=CARTESIAN_POINT('Ctrl Pts',(-3.3399062448374,-1.30000000000612,3.75968650438954));
#42285=CARTESIAN_POINT('Ctrl Pts',(-3.30990435433654,-1.18514270861593,
3.79086721926482));
#42286=CARTESIAN_POINT('Ctrl Pts',(-3.28263249593294,-1.06847604194722,
3.82262158044737));
#42287=CARTESIAN_POINT('Ctrl Pts',(-3.22593596759032,-0.794772684000856,
3.89730574494384));
#42288=CARTESIAN_POINT('Ctrl Pts',(-3.19242642144331,-0.6363098000952,3.95066436682348));
#42289=CARTESIAN_POINT('Ctrl Pts',(-3.15954151902818,-0.31943490727716,
4.01805835857427));
#42290=CARTESIAN_POINT('Ctrl Pts',(-3.14791830028498,-0.158333333333333,
4.04962461397864));
#42291=CARTESIAN_POINT('Ctrl Pts',(-3.16645071717067,0.158333333333336,
4.0684300663336));
#42292=CARTESIAN_POINT('Ctrl Pts',(-3.19653610248528,0.319434907277171,
4.05560767286993));
#42293=CARTESIAN_POINT('Ctrl Pts',(-3.26731329855029,0.636309800095212,
4.02664448876788));
#42294=CARTESIAN_POINT('Ctrl Pts',(-3.32125873700668,0.794772684000845,
3.99378941694402));
#42295=CARTESIAN_POINT('Ctrl Pts',(-3.41034596179839,1.06847604194515,3.95229414260646));
#42296=CARTESIAN_POINT('Ctrl Pts',(-3.45105881184621,1.18514270861186,3.93443571615802));
#42297=CARTESIAN_POINT('Ctrl Pts',(-3.49392195333653,1.30000000000012,3.91668062997042));
#42298=CARTESIAN_POINT('Ctrl Pts',(-3.34788849600256,-1.30000000000612,
3.73634894724596));
#42299=CARTESIAN_POINT('Ctrl Pts',(-3.31937411472217,-1.18514270861593,
3.76289356830514));
#42300=CARTESIAN_POINT('Ctrl Pts',(-3.29337082538162,-1.06847604194722,
3.79138747063358));
#42301=CARTESIAN_POINT('Ctrl Pts',(-3.23909914978854,-0.794772684000859,
3.86171731488158));
#42302=CARTESIAN_POINT('Ctrl Pts',(-3.2065171165066,-0.6363098000952,3.91679063131027));
#42303=CARTESIAN_POINT('Ctrl Pts',(-3.17499828999647,-0.319434907277159,
3.98503060092698));
#42304=CARTESIAN_POINT('Ctrl Pts',(-3.16371986733513,-0.158333333333333,
4.01880826653251));
#42305=CARTESIAN_POINT('Ctrl Pts',(-3.18254911001473,0.158333333333336,
4.03785829462972));
#42306=CARTESIAN_POINT('Ctrl Pts',(-3.21244993587892,0.319434907277171,
4.02299152238729));
#42307=CARTESIAN_POINT('Ctrl Pts',(-3.28274389109813,0.636309800095212,
3.99383849579238));
#42308=CARTESIAN_POINT('Ctrl Pts',(-3.33709854669969,0.794772684000844,
3.96021965052572));
#42309=CARTESIAN_POINT('Ctrl Pts',(-3.42376567995241,1.06847604194515,3.92302093447304));
#42310=CARTESIAN_POINT('Ctrl Pts',(-3.4628662367082,1.18514270861185,3.90813573323397));
#42311=CARTESIAN_POINT('Ctrl Pts',(-3.50355235956844,1.30000000000012,3.89446727658678));
#42312=CARTESIAN_POINT('Ctrl Pts',(-3.35676926861817,-1.30000000000612,
3.70282586044512));
#42313=CARTESIAN_POINT('Ctrl Pts',(-3.33044341345346,-1.18514270861593,
3.72314360027605));
#42314=CARTESIAN_POINT('Ctrl Pts',(-3.30627800160764,-1.06847604194723,
3.74724744299701));
#42315=CARTESIAN_POINT('Ctrl Pts',(-3.25544212223206,-0.79477268400086,
3.81167879672225));
#42316=CARTESIAN_POINT('Ctrl Pts',(-3.22403125657669,-0.636309800095206,
3.86898925355682));
#42317=CARTESIAN_POINT('Ctrl Pts',(-3.19432000284549,-0.319434907277165,
3.93827378933774));
#42318=CARTESIAN_POINT('Ctrl Pts',(-3.18317958250032,-0.158333333333334,
3.97475658534395));
#42319=CARTESIAN_POINT('Ctrl Pts',(-3.20290264786813,0.158333333333337,
3.99448700000565));
#42320=CARTESIAN_POINT('Ctrl Pts',(-3.23381791153657,0.319434907277169,
3.97783115213726));
#42321=CARTESIAN_POINT('Ctrl Pts',(-3.30359816134704,0.636309800095214,
3.94853941864496));
#42322=CARTESIAN_POINT('Ctrl Pts',(-3.3571095554096,0.794772684000856,3.91277821411019));
#42323=CARTESIAN_POINT('Ctrl Pts',(-3.44061455907929,1.06847604194516,3.88159668193594));
#42324=CARTESIAN_POINT('Ctrl Pts',(-3.4778644029592,1.18514270861186,3.87107111210848));
#42325=CARTESIAN_POINT('Ctrl Pts',(-3.51621786879574,1.30000000000012,3.86351730234215));
#42326=CARTESIAN_POINT('Ctrl Pts',(-3.36716075715539,-1.30000000000613,
3.66682073682202));
#42327=CARTESIAN_POINT('Ctrl Pts',(-3.34305466705167,-1.18514270861594,
3.68024022105575));
#42328=CARTESIAN_POINT('Ctrl Pts',(-3.3206574889083,-1.06847604194723,3.6993943697633));
#42329=CARTESIAN_POINT('Ctrl Pts',(-3.27286345535249,-0.794772684000868,
3.7568925072017));
#42330=CARTESIAN_POINT('Ctrl Pts',(-3.24167631719755,-0.636309800095208,
3.81587829399618));
#42331=CARTESIAN_POINT('Ctrl Pts',(-3.21373542909072,-0.319434907277165,
3.88613588118528));
#42332=CARTESIAN_POINT('Ctrl Pts',(-3.20374354149421,-0.158333333333335,
3.92626801976877));
#42333=CARTESIAN_POINT('Ctrl Pts',(-3.22437374685318,0.158333333333337,
3.94665109634336));
#42334=CARTESIAN_POINT('Ctrl Pts',(-3.25532686899206,0.319434907277173,
3.92722022169921));
#42335=CARTESIAN_POINT('Ctrl Pts',(-3.32461571737934,0.636309800095218,
3.89783336911054));
#42336=CARTESIAN_POINT('Ctrl Pts',(-3.37849095171978,0.794772684000857,
3.86076254193301));
#42337=CARTESIAN_POINT('Ctrl Pts',(-3.45862581829949,1.06847604194517,3.83618478432541));
#42338=CARTESIAN_POINT('Ctrl Pts',(-3.49365249706183,1.18514270861187,3.8302359484682));
#42339=CARTESIAN_POINT('Ctrl Pts',(-3.5290184401336,1.30000000000013,3.82897707732643));
#42340=CARTESIAN_POINT('Ctrl Pts',(-3.37613355071707,-1.30000000000613,
3.6299006776286));
#42341=CARTESIAN_POINT('Ctrl Pts',(-3.35360976259546,-1.18514270861594,
3.63602839514691));
#42342=CARTESIAN_POINT('Ctrl Pts',(-3.33267522134864,-1.06847604194723,
3.65004964033677));
#42343=CARTESIAN_POINT('Ctrl Pts',(-3.2879837213368,-0.794772684000865,
3.70067714968141));
#42344=CARTESIAN_POINT('Ctrl Pts',(-3.25891404695727,-0.636309800095211,
3.76260732504619));
#42345=CARTESIAN_POINT('Ctrl Pts',(-3.23251598801179,-0.319434907277168,
3.83361198066054));
#42346=CARTESIAN_POINT('Ctrl Pts',(-3.22162837572759,-0.158333333333335,
3.87588330921695));
#42347=CARTESIAN_POINT('Ctrl Pts',(-3.24278997166649,0.158333333333337,
3.89664102996846));
#42348=CARTESIAN_POINT('Ctrl Pts',(-3.27503321896417,0.31943490727717,3.87539089328648));
#42349=CARTESIAN_POINT('Ctrl Pts',(-3.34414068152806,0.636309800095217,
3.8461315485306));
#42350=CARTESIAN_POINT('Ctrl Pts',(-3.39755546629246,0.794772684000862,
3.80710534260456));
#42351=CARTESIAN_POINT('Ctrl Pts',(-3.47488930401332,1.06847604194517,3.78953560103793));
#42352=CARTESIAN_POINT('Ctrl Pts',(-3.5081939264536,1.18514270861187,3.78853090162309));
#42353=CARTESIAN_POINT('Ctrl Pts',(-3.54132821848589,1.30000000000013,3.79412679289453));
#42354=CARTESIAN_POINT('Ctrl Pts',(-3.38313772104073,-1.30000000000614,
3.60245047971202));
#42355=CARTESIAN_POINT('Ctrl Pts',(-3.3620903583262,-1.18514270861595,3.60332356220316));
#42356=CARTESIAN_POINT('Ctrl Pts',(-3.34227587486447,-1.06847604194724,
3.61352266758018));
#42357=CARTESIAN_POINT('Ctrl Pts',(-3.29934865190506,-0.79477268400087,
3.65862961985557));
#42358=CARTESIAN_POINT('Ctrl Pts',(-3.26989719363775,-0.636309800095214,
3.72141918826026));
#42359=CARTESIAN_POINT('Ctrl Pts',(-3.24457504885916,-0.319434907277169,
3.79292662824594));
#42360=CARTESIAN_POINT('Ctrl Pts',(-3.23475116607984,-0.158333333333336,
3.83798840641589));
#42361=CARTESIAN_POINT('Ctrl Pts',(-3.25678466785586,0.158333333333339,
3.85932996227175));
#42362=CARTESIAN_POINT('Ctrl Pts',(-3.28925648289735,0.319434907277174,
3.83617137686758));
#42363=CARTESIAN_POINT('Ctrl Pts',(-3.35820773366914,0.636309800095222,
3.80699113557097));
#42364=CARTESIAN_POINT('Ctrl Pts',(-3.41172663140231,0.794772684000866,
3.76685913072204));
#42365=CARTESIAN_POINT('Ctrl Pts',(-3.48704582484666,1.06847604194518,3.75459317631157));
#42366=CARTESIAN_POINT('Ctrl Pts',(-3.51902987619849,1.18514270861188,3.75725936825981));
#42367=CARTESIAN_POINT('Ctrl Pts',(-3.55039509091127,1.30000000000014,3.76790122932218));
#42368=CARTESIAN_POINT('Ctrl Pts',(-3.38728869726105,-1.30000000000614,
3.58381770307506));
#42369=CARTESIAN_POINT('Ctrl Pts',(-3.36704988134032,-1.18514270861595,
3.58108052935757));
#42370=CARTESIAN_POINT('Ctrl Pts',(-3.34791840522007,-1.06847604194724,
3.58869613419906));
#42371=CARTESIAN_POINT('Ctrl Pts',(-3.30627904460568,-0.794772684000871,
3.63020669441649));
#42372=CARTESIAN_POINT('Ctrl Pts',(-3.27715565086726,-0.636309800095213,
3.69395775582164));
#42373=CARTESIAN_POINT('Ctrl Pts',(-3.25278861508665,-0.319434907277168,
3.76595015077511));
#42374=CARTESIAN_POINT('Ctrl Pts',(-3.24365681828501,-0.158333333333336,
3.81284424669156));
#42375=CARTESIAN_POINT('Ctrl Pts',(-3.26602170365329,0.158333333333338,
3.83439736280539));
#42376=CARTESIAN_POINT('Ctrl Pts',(-3.29827221014194,0.319434907277173,
3.80972345816915));
#42377=CARTESIAN_POINT('Ctrl Pts',(-3.36665942123245,0.636309800095221,
3.78027442478073));
#42378=CARTESIAN_POINT('Ctrl Pts',(-3.41969919892025,0.794772684000864,
3.73900508051313));
#42379=CARTESIAN_POINT('Ctrl Pts',(-3.49390610955008,1.06847604194518,3.73043394287847));
#42380=CARTESIAN_POINT('Ctrl Pts',(-3.52531250203841,1.18514270861188,3.7357606961922));
#42381=CARTESIAN_POINT('Ctrl Pts',(-3.55600386504045,1.30000000000014,3.75012433070975));
#42382=CARTESIAN_POINT('Ctrl Pts',(-3.38926080300867,-1.30000000000614,
3.57444602733469));
#42383=CARTESIAN_POINT('Ctrl Pts',(-3.36929494337846,-1.18514270861595,
3.5698257263846));
#42384=CARTESIAN_POINT('Ctrl Pts',(-3.35043925926547,-1.06847604194724,
3.57611046617764));
#42385=CARTESIAN_POINT('Ctrl Pts',(-3.30944358443281,-0.794772684000869,
3.61582229801963));
#42386=CARTESIAN_POINT('Ctrl Pts',(-3.28084291417713,-0.636309800095212,
3.68027275809969));
#42387=CARTESIAN_POINT('Ctrl Pts',(-3.25691196489572,-0.319434907277168,
3.75247029427834));
#42388=CARTESIAN_POINT('Ctrl Pts',(-3.2476757322749,-0.158333333333336,
3.79997891584379));
#42389=CARTESIAN_POINT('Ctrl Pts',(-3.27028036494494,0.158333333333338,
3.8216909020588));
#42390=CARTESIAN_POINT('Ctrl Pts',(-3.30284156658081,0.319434907277174,
3.79654749839507));
#42391=CARTESIAN_POINT('Ctrl Pts',(-3.37134925175474,0.636309800095222,
3.76724512890989));
#42392=CARTESIAN_POINT('Ctrl Pts',(-3.42455080838407,0.794772684000863,
3.72569454678701));
#42393=CARTESIAN_POINT('Ctrl Pts',(-3.49809669875276,1.06847604194517,3.71889511869807));
#42394=CARTESIAN_POINT('Ctrl Pts',(-3.52902804544423,1.18514270861188,3.72541911643121));
#42395=CARTESIAN_POINT('Ctrl Pts',(-3.55905544803037,1.30000000000014,3.74141033237353));
#42396=CARTESIAN_POINT('Ctrl Pts',(-3.39080022004117,-1.30000000000614,
3.56657258907557));
#42397=CARTESIAN_POINT('Ctrl Pts',(-3.37096541358638,-1.18514270861595,
3.56032254232818));
#42398=CARTESIAN_POINT('Ctrl Pts',(-3.35228764005807,-1.06847604194724,
3.56546600434905));
#42399=CARTESIAN_POINT('Ctrl Pts',(-3.31181122425609,-0.794772684000869,
3.60366971508127));
#42400=CARTESIAN_POINT('Ctrl Pts',(-3.28384244468666,-0.636309800095213,
3.66883132141165));
#42401=CARTESIAN_POINT('Ctrl Pts',(-3.26030123191267,-0.319434907277168,
3.74121307600204));
#42402=CARTESIAN_POINT('Ctrl Pts',(-3.25088044244533,-0.158333333333336,
3.78916350670144));
#42403=CARTESIAN_POINT('Ctrl Pts',(-3.2736344675113,0.158333333333338,3.81097066546428));
#42404=CARTESIAN_POINT('Ctrl Pts',(-3.30643375805074,0.319434907277174,
3.78542225373319));
#42405=CARTESIAN_POINT('Ctrl Pts',(-3.3750512688792,0.636309800095221,3.756248423968));
#42406=CARTESIAN_POINT('Ctrl Pts',(-3.42842023428127,0.794772684000864,
3.71448645638646));
#42407=CARTESIAN_POINT('Ctrl Pts',(-3.50147954230933,1.06847604194518,3.70920741083224));
#42408=CARTESIAN_POINT('Ctrl Pts',(-3.53204973076412,1.18514270861188,3.71675273500996));
#42409=CARTESIAN_POINT('Ctrl Pts',(-3.56156544034252,1.30000000000014,3.73412848657792));
#42410=CARTESIAN_POINT('Ctrl Pts',(-3.39199100145532,-1.30000000000614,
3.56113432904435));
#42411=CARTESIAN_POINT('Ctrl Pts',(-3.37235755683788,-1.18514270861595,
3.55381257366595));
#42412=CARTESIAN_POINT('Ctrl Pts',(-3.35384901121602,-1.06847604194724,
3.55818516674942));
#42413=CARTESIAN_POINT('Ctrl Pts',(-3.31368930992307,-0.794772684000869,
3.59530301589943));
#42414=CARTESIAN_POINT('Ctrl Pts',(-3.28579838077169,-0.636309800095212,
3.66073041711429));
#42415=CARTESIAN_POINT('Ctrl Pts',(-3.26248485028938,-0.319434907277167,
3.73321397902517));
#42416=CARTESIAN_POINT('Ctrl Pts',(-3.25320340928079,-0.158333333333336,
3.78164852128053));
#42417=CARTESIAN_POINT('Ctrl Pts',(-3.27607811504414,0.158333333333338,
3.80353128302652));
#42418=CARTESIAN_POINT('Ctrl Pts',(-3.30889516405502,0.319434907277174,
3.77760062047387));
#42419=CARTESIAN_POINT('Ctrl Pts',(-3.37745661286962,0.636309800095221,
3.74842549607253));
#42420=CARTESIAN_POINT('Ctrl Pts',(-3.43078684621723,0.794772684000862,
3.70640534718603));
#42421=CARTESIAN_POINT('Ctrl Pts',(-3.50356138026373,1.06847604194517,3.70222983579113));
#42422=CARTESIAN_POINT('Ctrl Pts',(-3.53395864103283,1.18514270861188,3.71054615707037));
#42423=CARTESIAN_POINT('Ctrl Pts',(-3.56325176334453,1.30000000000014,3.72898622379376));
#42424=CARTESIAN_POINT('Ctrl Pts',(-3.3925988698541,-1.30000000000614,3.55842326075474));
#42425=CARTESIAN_POINT('Ctrl Pts',(-3.37308151150911,-1.18514270861595,
3.55057546246673));
#42426=CARTESIAN_POINT('Ctrl Pts',(-3.35466355614072,-1.06847604194724,
3.55456645795605));
#42427=CARTESIAN_POINT('Ctrl Pts',(-3.31465423555151,-0.79477268400087,
3.59113643790015));
#42428=CARTESIAN_POINT('Ctrl Pts',(-3.28674928219221,-0.636309800095213,
3.65666323743037));
#42429=CARTESIAN_POINT('Ctrl Pts',(-3.26354044548759,-0.319434907277168,
3.7291920642993));
#42430=CARTESIAN_POINT('Ctrl Pts',(-3.25436486975235,-0.158333333333336,
3.77789205702812));
#42431=CARTESIAN_POINT('Ctrl Pts',(-3.27729915242542,0.158333333333338,
3.79981160017967));
#42432=CARTESIAN_POINT('Ctrl Pts',(-3.31010431598875,0.319434907277174,
3.77367584924757));
#42433=CARTESIAN_POINT('Ctrl Pts',(-3.37861234863815,0.636309800095221,
3.74448234879849));
#42434=CARTESIAN_POINT('Ctrl Pts',(-3.43188705685757,0.794772684000863,
3.70230766822783));
#42435=CARTESIAN_POINT('Ctrl Pts',(-3.50453022588138,1.06847604194517,3.69869139277083));
#42436=CARTESIAN_POINT('Ctrl Pts',(-3.53485775210915,1.18514270861188,3.7074047832426));
#42437=CARTESIAN_POINT('Ctrl Pts',(-3.564068268389,1.30000000000014,3.72639691583526));
#42438=CARTESIAN_POINT('Ctrl Pts',(-3.39294995992423,-1.30000000000614,
3.5568765891777));
#42439=CARTESIAN_POINT('Ctrl Pts',(-3.37350207458928,-1.18514270861595,
3.54873017946487));
#42440=CARTESIAN_POINT('Ctrl Pts',(-3.35513703086187,-1.06847604194724,
3.55250383045926));
#42441=CARTESIAN_POINT('Ctrl Pts',(-3.31521168667268,-0.794772684000869,
3.58875944400585));
#42442=CARTESIAN_POINT('Ctrl Pts',(-3.28728630738722,-0.636309800095212,
3.6543350335598));
#42443=CARTESIAN_POINT('Ctrl Pts',(-3.26413716692034,-0.319434907277167,
3.72688968551762));
#42444=CARTESIAN_POINT('Ctrl Pts',(-3.25503424564992,-0.158333333333336,
3.77574933319419));
#42445=CARTESIAN_POINT('Ctrl Pts',(-3.27800290583528,0.158333333333338,
3.79769006677565));
#42446=CARTESIAN_POINT('Ctrl Pts',(-3.31079220769387,0.319434907277174,
3.77143113154901));
#42447=CARTESIAN_POINT('Ctrl Pts',(-3.37926491037695,0.636309800095221,
3.74222384467635));
#42448=CARTESIAN_POINT('Ctrl Pts',(-3.43250619377278,0.794772684000862,
3.69995947942588));
#42449=CARTESIAN_POINT('Ctrl Pts',(-3.50507659147902,1.06847604194517,3.69666438138917));
#42450=CARTESIAN_POINT('Ctrl Pts',(-3.53536657239264,1.18514270861188,3.70560631562752));
#42451=CARTESIAN_POINT('Ctrl Pts',(-3.56453349805111,1.30000000000014,3.7249165099489));
#42452=CARTESIAN_POINT('Ctrl Pts',(-3.39595090217982,-1.30000000000614,
3.54374063920193));
#42453=CARTESIAN_POINT('Ctrl Pts',(-3.37712431335929,-1.18514270861595,
3.53307659206714));
#42454=CARTESIAN_POINT('Ctrl Pts',(-3.35922077748584,-1.06847604194724,
3.53501108173953));
#42455=CARTESIAN_POINT('Ctrl Pts',(-3.3199924649923,-0.794772684000869,
3.56858528022899));
#42456=CARTESIAN_POINT('Ctrl Pts',(-3.29181540136125,-0.636309800095212,
3.63452697929673));
#42457=CARTESIAN_POINT('Ctrl Pts',(-3.26909728302276,-0.319434907277167,
3.70725154333468));
#42458=CARTESIAN_POINT('Ctrl Pts',(-3.26054283291219,-0.158333333333336,
3.75742121604236));
#42459=CARTESIAN_POINT('Ctrl Pts',(-3.28381007894358,0.158333333333338,
3.77954503560209));
#42460=CARTESIAN_POINT('Ctrl Pts',(-3.31658660801587,0.319434907277172,
3.75231918720872));
#42461=CARTESIAN_POINT('Ctrl Pts',(-3.3847535052942,0.636309800095219,3.72298896000326));
#42462=CARTESIAN_POINT('Ctrl Pts',(-3.43756942643472,0.794772684000863,
3.67986752481284));
#42463=CARTESIAN_POINT('Ctrl Pts',(-3.50951277420466,1.06847604194517,3.67929368192812));
#42464=CARTESIAN_POINT('Ctrl Pts',(-3.53950604440435,1.18514270861188,3.69019148901067));
#42465=CARTESIAN_POINT('Ctrl Pts',(-3.56835097531788,1.30000000000013,3.71223549849759));
#42466=CARTESIAN_POINT('Ctrl Pts',(-3.40091752166454,-1.30000000000612,
3.51817485258119));
#42467=CARTESIAN_POINT('Ctrl Pts',(-3.3825190627201,-1.18514270861593,3.50224067487218));
#42468=CARTESIAN_POINT('Ctrl Pts',(-3.36511610557604,-1.06847604194723,
3.50043212764256));
#42469=CARTESIAN_POINT('Ctrl Pts',(-3.32721160143233,-0.794772684000861,
3.52888705397335));
#42470=CARTESIAN_POINT('Ctrl Pts',(-3.30030872076733,-0.636309800095203,
3.59661809923234));
#42471=CARTESIAN_POINT('Ctrl Pts',(-3.27877017942277,-0.319434907277162,
3.66986977447395));
#42472=CARTESIAN_POINT('Ctrl Pts',(-3.2703562795432,-0.158333333333334,
3.72194050984075));
#42473=CARTESIAN_POINT('Ctrl Pts',(-3.29412609583291,0.158333333333336,
3.74436766369114));
#42474=CARTESIAN_POINT('Ctrl Pts',(-3.32699824865703,0.319434907277173,
3.71537912026337));
#42475=CARTESIAN_POINT('Ctrl Pts',(-3.39555189840338,0.636309800095215,
3.68647567718409));
#42476=CARTESIAN_POINT('Ctrl Pts',(-3.44969761789044,0.794772684000848,
3.64319747826915));
#42477=CARTESIAN_POINT('Ctrl Pts',(-3.52005275577435,1.06847604194516,3.6475149776169));
#42478=CARTESIAN_POINT('Ctrl Pts',(-3.54871229088136,1.18514270861187,3.66159565030966));
#42479=CARTESIAN_POINT('Ctrl Pts',(-3.57557722882024,1.30000000000013,3.68788811020667));
#42480=CARTESIAN_POINT('Ctrl Pts',(-3.405827299293,-1.30000000000611,3.49305769738095));
#42481=CARTESIAN_POINT('Ctrl Pts',(-3.38807550315117,-1.18514270861592,
3.47209928049423));
#42482=CARTESIAN_POINT('Ctrl Pts',(-3.37125653663434,-1.06847604194722,
3.46667872482858));
#42483=CARTESIAN_POINT('Ctrl Pts',(-3.33455638240376,-0.794772684000851,
3.49005172462144));
#42484=CARTESIAN_POINT('Ctrl Pts',(-3.30823759879945,-0.636309800095196,
3.55911508787058));
#42485=CARTESIAN_POINT('Ctrl Pts',(-3.28760112788313,-0.319434907277159,
3.63271287357265));
#42486=CARTESIAN_POINT('Ctrl Pts',(-3.27942269200311,-0.158333333333332,
3.68669773611711));
#42487=CARTESIAN_POINT('Ctrl Pts',(-3.30384439390905,0.158333333333334,
3.70951459063184));
#42488=CARTESIAN_POINT('Ctrl Pts',(-3.3375004211861,0.319434907277167,3.67925227436011));
#42489=CARTESIAN_POINT('Ctrl Pts',(-3.40573136959718,0.636309800095206,
3.65028594953744));
#42490=CARTESIAN_POINT('Ctrl Pts',(-3.4585925712012,0.794772684000842,3.60508175016501));
#42491=CARTESIAN_POINT('Ctrl Pts',(-3.52792852763024,1.06847604194515,3.61461081427897));
#42492=CARTESIAN_POINT('Ctrl Pts',(-3.55620374536085,1.18514270861185,3.63247544804156));
#42493=CARTESIAN_POINT('Ctrl Pts',(-3.58274121443434,1.30000000000011,3.66407993679843));
#42494=CARTESIAN_POINT('Ctrl Pts',(-3.40792382026203,-1.30000000000611,
3.48027749552897));
#42495=CARTESIAN_POINT('Ctrl Pts',(-3.39063227265826,-1.18514270861592,
3.45690107898799));
#42496=CARTESIAN_POINT('Ctrl Pts',(-3.37417219529096,-1.06847604194722,
3.4497223830696));
#42497=CARTESIAN_POINT('Ctrl Pts',(-3.33806698632697,-0.794772684000851,
3.4705581343858));
#42498=CARTESIAN_POINT('Ctrl Pts',(-3.31165271079239,-0.636309800095196,
3.54004392440299));
#42499=CARTESIAN_POINT('Ctrl Pts',(-3.29150406597601,-0.319434907277159,
3.61383388564811));
#42500=CARTESIAN_POINT('Ctrl Pts',(-3.28383918476484,-0.158333333333332,
3.66901547560886));
#42501=CARTESIAN_POINT('Ctrl Pts',(-3.30866559173632,0.158333333333334,
3.69207105417689));
#42502=CARTESIAN_POINT('Ctrl Pts',(-3.34233892867208,0.319434907277167,
3.66093066788631));
#42503=CARTESIAN_POINT('Ctrl Pts',(-3.410649428729,0.636309800095206,3.6320956127618));
#42504=CARTESIAN_POINT('Ctrl Pts',(-3.46380979023612,0.79477268400084,3.58656909938636));
#42505=CARTESIAN_POINT('Ctrl Pts',(-3.5324927010696,1.06847604194515,3.59858491022785));
#42506=CARTESIAN_POINT('Ctrl Pts',(-3.56027544998898,1.18514270861185,3.61812328835454));
#42507=CARTESIAN_POINT('Ctrl Pts',(-3.58611066068062,1.30000000000011,3.65199884532431));
#42508=CARTESIAN_POINT('',(-3.53205673212874,1.2,3.73199261231698));
#42509=CARTESIAN_POINT('Ctrl Pts',(-3.53205673212874,1.2,3.73199261231698));
#42510=CARTESIAN_POINT('Ctrl Pts',(-3.52948084971163,1.21683760541185,3.75340201998427));
#42511=CARTESIAN_POINT('Ctrl Pts',(-3.52780194167531,1.23326792451706,3.77522907381777));
#42512=CARTESIAN_POINT('Ctrl Pts',(-3.52211206890299,1.27112122678138,3.82383590222122));
#42513=CARTESIAN_POINT('Ctrl Pts',(-3.51997651543627,1.28438964967196,3.84082124280845));
#42514=CARTESIAN_POINT('Ctrl Pts',(-3.51715936788841,1.30000000000012,3.86052549330383));
#42515=CARTESIAN_POINT('',(-3.42060206188123,0.653834841369693,3.62201431893726));
#42516=CARTESIAN_POINT('Ctrl Pts',(-3.42060206191022,0.653834841368434,
3.62201431891412));
#42517=CARTESIAN_POINT('Ctrl Pts',(-3.43225912838132,0.717398299039534,
3.63315863003243));
#42518=CARTESIAN_POINT('Ctrl Pts',(-3.44169414240865,0.763866154347927,
3.6422587392106));
#42519=CARTESIAN_POINT('Ctrl Pts',(-3.47884866191347,0.949862607754481,
3.6784459127313));
#42520=CARTESIAN_POINT('Ctrl Pts',(-3.50142427864103,1.05920663100849,3.70079441938718));
#42521=CARTESIAN_POINT('Ctrl Pts',(-3.53205673212874,1.2,3.73199261231697));
#42522=CARTESIAN_POINT('',(-3.3184146483206,-0.653834841531101,3.52704148923361));
#42523=CARTESIAN_POINT('Ctrl Pts',(-3.3184146483206,-0.6538348415311,3.52704148923361));
#42524=CARTESIAN_POINT('Ctrl Pts',(-3.30612811194715,-0.575978670096729,
3.56675882559093));
#42525=CARTESIAN_POINT('Ctrl Pts',(-3.29645819180146,-0.493638820710554,
3.60055778198947));
#42526=CARTESIAN_POINT('Ctrl Pts',(-3.28491094893504,-0.33813590691445,
3.64983331844457));
#42527=CARTESIAN_POINT('Ctrl Pts',(-3.28203919381975,-0.265660385906066,
3.66749140295376));
#42528=CARTESIAN_POINT('Ctrl Pts',(-3.28241544521535,-0.129716867465535,
3.69186530924249));
#42529=CARTESIAN_POINT('Ctrl Pts',(-3.28481094186636,-0.0666253188345313,
3.69978762165696));
#42530=CARTESIAN_POINT('Ctrl Pts',(-3.29431793587721,0.0595444211916306,
3.70913066613523));
#42531=CARTESIAN_POINT('Ctrl Pts',(-3.30148802195868,0.122778732322982,
3.71063286763887));
#42532=CARTESIAN_POINT('Ctrl Pts',(-3.32176075453611,0.260129204703633,
3.706256674953));
#42533=CARTESIAN_POINT('Ctrl Pts',(-3.33571117140391,0.333944924094639,
3.69898184713565));
#42534=CARTESIAN_POINT('Ctrl Pts',(-3.37149269979535,0.491211330758176,
3.67194126002883));
#42535=CARTESIAN_POINT('Ctrl Pts',(-3.39448994830551,0.57435513917775,3.65030538941433));
#42536=CARTESIAN_POINT('Ctrl Pts',(-3.42060206189246,0.653834841386266,
3.6220143189942));
#42537=CARTESIAN_POINT('',(-3.37166915868338,-1.2,3.57586602284307));
#42538=CARTESIAN_POINT('Ctrl Pts',(-3.37166915868338,-1.2,3.57586602284307));
#42539=CARTESIAN_POINT('Ctrl Pts',(-3.36161693023492,-1.12735839874247,
3.56651405383493));
#42540=CARTESIAN_POINT('Ctrl Pts',(-3.3499116696866,-1.03209555687847,3.55570207735526));
#42541=CARTESIAN_POINT('Ctrl Pts',(-3.32722961700632,-0.796656601307582,
3.535001960447));
#42542=CARTESIAN_POINT('Ctrl Pts',(-3.32318655071222,-0.739830804734627,
3.53135276875128));
#42543=CARTESIAN_POINT('Ctrl Pts',(-3.3184146483206,-0.653834841531101,
3.52704148923361));
#42544=CARTESIAN_POINT('Ctrl Pts',(-3.35764585633179,-1.3,3.70018367575412));
#42545=CARTESIAN_POINT('Ctrl Pts',(-3.36040387352645,-1.28300448077975,
3.67927748627612));
#42546=CARTESIAN_POINT('Ctrl Pts',(-3.36304294190339,-1.2660224815296,3.65834194442482));
#42547=CARTESIAN_POINT('Ctrl Pts',(-3.36818942120242,-1.22837741622835,
3.61141873178763));
#42548=CARTESIAN_POINT('Ctrl Pts',(-3.37032016522922,-1.21502229683377,
3.59512911028479));
#42549=CARTESIAN_POINT('Ctrl Pts',(-3.37166915868338,-1.2,3.57586602284307));
#42550=CARTESIAN_POINT('Origin',(0.,1.25,7.2));
#42551=CARTESIAN_POINT('Origin',(0.,1.2,7.2));
#42552=CARTESIAN_POINT('Origin',(0.,0.92691742076555,7.2));
#42553=CARTESIAN_POINT('Origin',(0.,0.653834841531101,7.2));
#42554=CARTESIAN_POINT('Origin',(0.,0.,7.2));
#42555=CARTESIAN_POINT('Origin',(0.,-0.653834841531101,7.2));
#42556=CARTESIAN_POINT('Origin',(0.,-0.926917420765551,7.2));
#42557=CARTESIAN_POINT('Origin',(0.,-1.2,7.2));
#42558=CARTESIAN_POINT('Origin',(0.,-1.25,7.2));
#42559=CARTESIAN_POINT('Ctrl Pts',(-3.15371419665032,-1.30000000000011,
3.26266732036565));
#42560=CARTESIAN_POINT('Ctrl Pts',(-3.19010469464727,-1.18514270861185,
3.28482004315617));
#42561=CARTESIAN_POINT('Ctrl Pts',(-3.21244012754456,-1.06847604194515,
3.31040827862903));
#42562=CARTESIAN_POINT('Ctrl Pts',(-3.231569433639,-0.794772684000851,3.37745894304843));
#42563=CARTESIAN_POINT('Ctrl Pts',(-3.19184909016007,-0.636309800095197,
3.43508690301717));
#42564=CARTESIAN_POINT('Ctrl Pts',(-3.17031238807978,-0.319434907277159,
3.50603727500875));
#42565=CARTESIAN_POINT('Ctrl Pts',(-3.14286241424732,-0.158333333333332,
3.54278120260502));
#42566=CARTESIAN_POINT('Ctrl Pts',(-3.16838675811282,0.158333333333334,
3.56506164372392));
#42567=CARTESIAN_POINT('Ctrl Pts',(-3.22246485929617,0.319434907277167,
3.55167070473433));
#42568=CARTESIAN_POINT('Ctrl Pts',(-3.29374448453208,0.636309800095206,
3.52391928505034));
#42569=CARTESIAN_POINT('Ctrl Pts',(-3.36008858048819,0.79477268400084,3.49038646683519));
#42570=CARTESIAN_POINT('Ctrl Pts',(-3.37703616936998,1.0684760419452,3.45230111691743));
#42571=CARTESIAN_POINT('Ctrl Pts',(-3.36817625250791,1.18514270861195,3.43668158762793));
#42572=CARTESIAN_POINT('Ctrl Pts',(-3.3431204355269,1.30000000000025,3.42192826582706));
#42573=CARTESIAN_POINT('Ctrl Pts',(-3.14205148972774,-1.30000000000011,
3.26728112631937));
#42574=CARTESIAN_POINT('Ctrl Pts',(-3.17625676666542,-1.18514270861185,
3.29036965169776));
#42575=CARTESIAN_POINT('Ctrl Pts',(-3.19697910116141,-1.06847604194515,
3.31662261210206));
#42576=CARTESIAN_POINT('Ctrl Pts',(-3.2137035450423,-0.794772684000851,
3.38458268047563));
#42577=CARTESIAN_POINT('Ctrl Pts',(-3.17427247914414,-0.636309800095197,
3.44187942841939));
#42578=CARTESIAN_POINT('Ctrl Pts',(-3.152596911054,-0.319434907277159,3.51276440598953));
#42579=CARTESIAN_POINT('Ctrl Pts',(-3.12601838773468,-0.158333333333332,
3.54939933543317));
#42580=CARTESIAN_POINT('Ctrl Pts',(-3.1512630121036,0.158333333333334,3.57130224196186));
#42581=CARTESIAN_POINT('Ctrl Pts',(-3.20409726059295,0.319434907277167,
3.55752565368255));
#42582=CARTESIAN_POINT('Ctrl Pts',(-3.27513477131917,0.636309800095206,
3.52930916809052));
#42583=CARTESIAN_POINT('Ctrl Pts',(-3.34106873620035,0.794772684000841,
3.49591547434885));
#42584=CARTESIAN_POINT('Ctrl Pts',(-3.3604774855321,1.06847604194519,3.45697322365221));
#42585=CARTESIAN_POINT('Ctrl Pts',(-3.35332856352237,1.18514270861194,3.44081299553763));
#42586=CARTESIAN_POINT('Ctrl Pts',(-3.33062939108222,1.30000000000025,3.42534919668245));
#42587=CARTESIAN_POINT('Ctrl Pts',(-3.11914435783443,-1.3,3.27690233901048));
#42588=CARTESIAN_POINT('Ctrl Pts',(-3.14787640739775,-1.18514270861176,
3.30061684476125));
#42589=CARTESIAN_POINT('Ctrl Pts',(-3.16474054018966,-1.06847604194507,
3.32749513738329));
#42590=CARTESIAN_POINT('Ctrl Pts',(-3.17628279868663,-0.794772684000792,
3.39689835091026));
#42591=CARTESIAN_POINT('Ctrl Pts',(-3.13918954893612,-0.636309800095149,
3.4556066653861));
#42592=CARTESIAN_POINT('Ctrl Pts',(-3.11771305468591,-0.319434907277135,
3.52692777173361));
#42593=CARTESIAN_POINT('Ctrl Pts',(-3.09226790959551,-0.15833333333332,
3.56258567354113));
#42594=CARTESIAN_POINT('Ctrl Pts',(-3.11713198495812,0.158333333333322,
3.58397698227228));
#42595=CARTESIAN_POINT('Ctrl Pts',(-3.16816605272952,0.319434907277142,
3.57033367148446));
#42596=CARTESIAN_POINT('Ctrl Pts',(-3.23881241642369,0.636309800095157,
3.54131553965297));
#42597=CARTESIAN_POINT('Ctrl Pts',(-3.3032657471794,0.794772684000782,3.50735791283628));
#42598=CARTESIAN_POINT('Ctrl Pts',(-3.32762855144439,1.06847604194511,3.4667109095563));
#42599=CARTESIAN_POINT('Ctrl Pts',(-3.32404137473076,1.18514270861185,3.44962602756524));
#42600=CARTESIAN_POINT('Ctrl Pts',(-3.30632126606804,1.30000000000015,3.43305084518312));
#42601=CARTESIAN_POINT('Ctrl Pts',(-3.09566895515122,-1.29999999999991,
3.28663238688277));
#42602=CARTESIAN_POINT('Ctrl Pts',(-3.12059772278264,-1.18514270861168,
3.31300758471133));
#42603=CARTESIAN_POINT('Ctrl Pts',(-3.13456318990637,-1.06847604194499,
3.34169118337383));
#42604=CARTESIAN_POINT('Ctrl Pts',(-3.14149879537078,-0.794772684000733,
3.41328890213884));
#42605=CARTESIAN_POINT('Ctrl Pts',(-3.10412801503358,-0.6363098000951,3.47031589024842));
#42606=CARTESIAN_POINT('Ctrl Pts',(-3.0820837770709,-0.31943490727711,3.5411760881235));
#42607=CARTESIAN_POINT('Ctrl Pts',(-3.05843946489796,-0.158333333333308,
3.57662503034522));
#42608=CARTESIAN_POINT('Ctrl Pts',(-3.08288767088593,0.15833333333331,3.59746865711391));
#42609=CARTESIAN_POINT('Ctrl Pts',(-3.13190938357248,0.31943490727712,3.58374411199378));
#42610=CARTESIAN_POINT('Ctrl Pts',(-3.20186015445897,0.636309800095111,
3.55354681530502));
#42611=CARTESIAN_POINT('Ctrl Pts',(-3.26445103385548,0.79477268400072,3.51857734110229));
#42612=CARTESIAN_POINT('Ctrl Pts',(-3.29376359632755,1.06847604194503,3.47607578299549));
#42613=CARTESIAN_POINT('Ctrl Pts',(-3.29383959420351,1.18514270861177,3.45809270241767));
#42614=CARTESIAN_POINT('Ctrl Pts',(-3.28130326779873,1.30000000000005,3.44052389092852));
#42615=CARTESIAN_POINT('Ctrl Pts',(-3.08348406279076,-1.29999999999989,
3.29178592705251));
#42616=CARTESIAN_POINT('Ctrl Pts',(-3.10574135532356,-1.18514270861166,
3.31878401257237));
#42617=CARTESIAN_POINT('Ctrl Pts',(-3.1177990022455,-1.06847604194498,3.34797513593898));
#42618=CARTESIAN_POINT('Ctrl Pts',(-3.12209135696599,-0.794772684000721,
3.42047882672178));
#42619=CARTESIAN_POINT('Ctrl Pts',(-3.08557745324672,-0.636309800095091,
3.47779171195928));
#42620=CARTESIAN_POINT('Ctrl Pts',(-3.06368580467661,-0.319434907277105,
3.54894189029846));
#42621=CARTESIAN_POINT('Ctrl Pts',(-3.04103908370401,-0.158333333333306,
3.58434443660176));
#42622=CARTESIAN_POINT('Ctrl Pts',(-3.06527529127201,0.158333333333308,
3.60491194509535));
#42623=CARTESIAN_POINT('Ctrl Pts',(-3.1129143893084,0.319434907277115,3.59075180290206));
#42624=CARTESIAN_POINT('Ctrl Pts',(-3.18263318481277,0.636309800095101,
3.560121444678));
#42625=CARTESIAN_POINT('Ctrl Pts',(-3.24487283518939,0.794772684000708,
3.52542348705439));
#42626=CARTESIAN_POINT('Ctrl Pts',(-3.27677865511172,1.06847604194502,3.48194717796983));
#42627=CARTESIAN_POINT('Ctrl Pts',(-3.2786394826502,1.18514270861175,3.46331755726819));
#42628=CARTESIAN_POINT('Ctrl Pts',(-3.26855029050992,1.30000000000003,3.44487759911162));
#42629=CARTESIAN_POINT('Ctrl Pts',(-3.08205935007171,-1.29999999999989,
3.29240216820087));
#42630=CARTESIAN_POINT('Ctrl Pts',(-3.10400423132416,-1.18514270861166,
3.31947608592427));
#42631=CARTESIAN_POINT('Ctrl Pts',(-3.11583818999718,-1.06847604194498,
3.34872805720068));
#42632=CARTESIAN_POINT('Ctrl Pts',(-3.11981874806555,-0.794772684000722,
3.42133770211157));
#42633=CARTESIAN_POINT('Ctrl Pts',(-3.08339916127519,-0.636309800095091,
3.47867637348839));
#42634=CARTESIAN_POINT('Ctrl Pts',(-3.06152505959721,-0.319434907277105,
3.54986039366487));
#42635=CARTESIAN_POINT('Ctrl Pts',(-3.03900126112515,-0.158333333333306,
3.58526433599475));
#42636=CARTESIAN_POINT('Ctrl Pts',(-3.06321279567437,0.158333333333308,
3.60579986109024));
#42637=CARTESIAN_POINT('Ctrl Pts',(-3.11068637074057,0.319434907277115,
3.5915851808083));
#42638=CARTESIAN_POINT('Ctrl Pts',(-3.18037387911668,0.636309800095102,
3.56089893154296));
#42639=CARTESIAN_POINT('Ctrl Pts',(-3.24256754226884,0.794772684000709,
3.52622689366647));
#42640=CARTESIAN_POINT('Ctrl Pts',(-3.27477723977453,1.06847604194502,3.48263421993515));
#42641=CARTESIAN_POINT('Ctrl Pts',(-3.27684855707369,1.18514270861175,3.46392909138567));
#42642=CARTESIAN_POINT('Ctrl Pts',(-3.26704880710871,1.30000000000003,3.44538848747727));
#42643=CARTESIAN_POINT('Ctrl Pts',(-3.07957071202657,-1.29999999999989,
3.29348617113064));
#42644=CARTESIAN_POINT('Ctrl Pts',(-3.10097599588882,-1.18514270861166,
3.3207009380138));
#42645=CARTESIAN_POINT('Ctrl Pts',(-3.11242278613173,-1.06847604194498,
3.3500643110132));
#42646=CARTESIAN_POINT('Ctrl Pts',(-3.11586104906488,-0.794772684000723,
3.42286328672011));
#42647=CARTESIAN_POINT('Ctrl Pts',(-3.07959939578454,-0.636309800095091,
3.48023920795107));
#42648=CARTESIAN_POINT('Ctrl Pts',(-3.05774875845631,-0.319434907277105,
3.55147401268194));
#42649=CARTESIAN_POINT('Ctrl Pts',(-3.03543093345207,-0.158333333333306,
3.58686927769264));
#42650=CARTESIAN_POINT('Ctrl Pts',(-3.05959934586064,0.158333333333308,
3.60734904397365));
#42651=CARTESIAN_POINT('Ctrl Pts',(-3.10679673806732,0.319434907277115,
3.59305548667019));
#42652=CARTESIAN_POINT('Ctrl Pts',(-3.1764281201781,0.636309800095102,3.56226964135765));
#42653=CARTESIAN_POINT('Ctrl Pts',(-3.23852516459111,0.794772684000709,
3.52762287869824));
#42654=CARTESIAN_POINT('Ctrl Pts',(-3.27126447143197,1.06847604194502,3.48382384133118));
#42655=CARTESIAN_POINT('Ctrl Pts',(-3.27370599441798,1.18514270861175,3.46498887056446));
#42656=CARTESIAN_POINT('Ctrl Pts',(-3.26441740756945,1.30000000000003,3.44627790939293));
#42657=CARTESIAN_POINT('Ctrl Pts',(-3.07462972908329,-1.29999999999989,
3.29569736909264));
#42658=CARTESIAN_POINT('Ctrl Pts',(-3.0949973182512,-1.18514270861166,3.32324213265696));
#42659=CARTESIAN_POINT('Ctrl Pts',(-3.1056939176873,-1.06847604194498,3.35285651108147));
#42660=CARTESIAN_POINT('Ctrl Pts',(-3.1080632812767,-0.794772684000723,
3.42605287393027));
#42661=CARTESIAN_POINT('Ctrl Pts',(-3.07206550985617,-0.636309800095092,
3.48344369259152));
#42662=CARTESIAN_POINT('Ctrl Pts',(-3.05022332264847,-0.319434907277106,
3.55473556987429));
#42663=CARTESIAN_POINT('Ctrl Pts',(-3.02828321681205,-0.158333333333306,
3.59007251318586));
#42664=CARTESIAN_POINT('Ctrl Pts',(-3.05236555158785,0.158333333333308,
3.61044215962353));
#42665=CARTESIAN_POINT('Ctrl Pts',(-3.09907076018363,0.319434907277115,
3.59606523135911));
#42666=CARTESIAN_POINT('Ctrl Pts',(-3.1685761801224,0.636309800095102,3.56506231885714));
#42667=CARTESIAN_POINT('Ctrl Pts',(-3.23039443701896,0.79477268400071,3.53035810324074));
#42668=CARTESIAN_POINT('Ctrl Pts',(-3.26417942019128,1.06847604194502,3.48612906482662));
#42669=CARTESIAN_POINT('Ctrl Pts',(-3.26737047710198,1.18514270861175,3.46704586685332));
#42670=CARTESIAN_POINT('Ctrl Pts',(-3.25912832356508,1.30000000000004,3.44802458278879));
#42671=CARTESIAN_POINT('Ctrl Pts',(-3.0676595775245,-1.2999999999999,3.29896557246829));
#42672=CARTESIAN_POINT('Ctrl Pts',(-3.0867124448927,-1.18514270861167,3.32717423455316));
#42673=CARTESIAN_POINT('Ctrl Pts',(-3.09643635911263,-1.06847604194499,
3.35726087101869));
#42674=CARTESIAN_POINT('Ctrl Pts',(-3.09734879819989,-0.794772684000731,
3.43110551657187));
#42675=CARTESIAN_POINT('Ctrl Pts',(-3.06153419114781,-0.636309800095098,
3.48829716508222));
#42676=CARTESIAN_POINT('Ctrl Pts',(-3.03954610633718,-0.319434907277109,
3.5594860621202));
#42677=CARTESIAN_POINT('Ctrl Pts',(-3.01798147324096,-0.158333333333308,
3.59454111589124));
#42678=CARTESIAN_POINT('Ctrl Pts',(-3.04194629752898,0.15833333333331,3.6147638751156));
#42679=CARTESIAN_POINT('Ctrl Pts',(-3.08821940758376,0.319434907277118,
3.6006024733673));
#42680=CARTESIAN_POINT('Ctrl Pts',(-3.15750734699938,0.636309800095107,
3.56923932045797));
#42681=CARTESIAN_POINT('Ctrl Pts',(-3.2185773149754,0.794772684000717,3.53401193423179));
#42682=CARTESIAN_POINT('Ctrl Pts',(-3.25381704576848,1.06847604194503,3.48911870634936));
#42683=CARTESIAN_POINT('Ctrl Pts',(-3.25812502168796,1.18514270861176,3.46973891452785));
#42684=CARTESIAN_POINT('Ctrl Pts',(-3.25148699982729,1.30000000000005,3.45041194577712));
#42685=CARTESIAN_POINT('Ctrl Pts',(-3.05929002312837,-1.29999999999991,
3.30288696422167));
#42686=CARTESIAN_POINT('Ctrl Pts',(-3.07677393383664,-1.18514270861168,
3.33190463910303));
#42687=CARTESIAN_POINT('Ctrl Pts',(-3.08534480279262,-1.06847604194499,
3.3625757915735));
#42688=CARTESIAN_POINT('Ctrl Pts',(-3.08455431518175,-0.794772684000734,
3.43725215353119));
#42689=CARTESIAN_POINT('Ctrl Pts',(-3.04902433433522,-0.636309800095101,
3.49427720425505));
#42690=CARTESIAN_POINT('Ctrl Pts',(-3.02689025391295,-0.31943490727711,
3.56537546901684));
#42691=CARTESIAN_POINT('Ctrl Pts',(-3.00576181446938,-0.158333333333308,
3.60007454025842));
#42692=CARTESIAN_POINT('Ctrl Pts',(-3.02955809413638,0.15833333333331,3.62009213531368));
#42693=CARTESIAN_POINT('Ctrl Pts',(-3.0752577679684,0.319434907277119,3.6061306943942));
#42694=CARTESIAN_POINT('Ctrl Pts',(-3.14428462971439,0.63630980009511,3.57434016945101));
#42695=CARTESIAN_POINT('Ctrl Pts',(-3.20455259630907,0.794772684000721,
3.53860178011621));
#42696=CARTESIAN_POINT('Ctrl Pts',(-3.2414986960271,1.06847604194503,3.49286218100061));
#42697=CARTESIAN_POINT('Ctrl Pts',(-3.24710266824222,1.18514270861176,3.47307108281982));
#42698=CARTESIAN_POINT('Ctrl Pts',(-3.24231801509243,1.30000000000005,3.45328786409621));
#42699=CARTESIAN_POINT('Ctrl Pts',(-3.04795105160112,-1.29999999999992,
3.30790732462681));
#42700=CARTESIAN_POINT('Ctrl Pts',(-3.06306779676184,-1.18514270861169,
3.3376911266136));
#42701=CARTESIAN_POINT('Ctrl Pts',(-3.06994766037203,-1.068476041945,3.3689676250005));
#42702=CARTESIAN_POINT('Ctrl Pts',(-3.06681267745931,-0.794772684000742,
3.44467102041343));
#42703=CARTESIAN_POINT('Ctrl Pts',(-3.03201375931715,-0.636309800095107,
3.5018731381446));
#42704=CARTESIAN_POINT('Ctrl Pts',(-3.01005996212089,-0.319434907277114,
3.5732854451987));
#42705=CARTESIAN_POINT('Ctrl Pts',(-2.98993876061887,-0.15833333333331,
3.60801054982657));
#42706=CARTESIAN_POINT('Ctrl Pts',(-3.01352943923577,0.158333333333312,
3.62777471043105));
#42707=CARTESIAN_POINT('Ctrl Pts',(-3.05789486132607,0.319434907277123,
3.61339757444287));
#42708=CARTESIAN_POINT('Ctrl Pts',(-3.12656995434065,0.636309800095117,
3.58105426454118));
#42709=CARTESIAN_POINT('Ctrl Pts',(-3.18632522509441,0.79477268400073,3.54534842162168));
#42710=CARTESIAN_POINT('Ctrl Pts',(-3.22561348356767,1.06847604194504,3.4985584054285));
#42711=CARTESIAN_POINT('Ctrl Pts',(-3.23288148404397,1.18514270861178,3.4781295861752));
#42712=CARTESIAN_POINT('Ctrl Pts',(-3.23041105367694,1.30000000000006,3.45752561193765));
#42713=CARTESIAN_POINT('Ctrl Pts',(-3.03373374036243,-1.29999999999993,
3.31415100966446));
#42714=CARTESIAN_POINT('Ctrl Pts',(-3.04590402957723,-1.1851427086117,3.34491311200048));
#42715=CARTESIAN_POINT('Ctrl Pts',(-3.05066932831086,-1.06847604194501,
3.37694967666605));
#42716=CARTESIAN_POINT('Ctrl Pts',(-3.04457111230556,-0.79477268400075,
3.45390481287289));
#42717=CARTESIAN_POINT('Ctrl Pts',(-3.01060375645462,-0.636309800095113,
3.51123269374844));
#42718=CARTESIAN_POINT('Ctrl Pts',(-2.98882960655681,-0.319434907277116,
3.58297929310441));
#42719=CARTESIAN_POINT('Ctrl Pts',(-2.96993063132861,-0.158333333333311,
3.61768107744254));
#42720=CARTESIAN_POINT('Ctrl Pts',(-2.99334906214383,0.158333333333313,
3.63722700691804));
#42721=CARTESIAN_POINT('Ctrl Pts',(-3.03630252279416,0.319434907277125,
3.62264763423389));
#42722=CARTESIAN_POINT('Ctrl Pts',(-3.10448273264278,0.636309800095122,
3.58954043317641));
#42723=CARTESIAN_POINT('Ctrl Pts',(-3.16322206646095,0.794772684000737,
3.55340286023055));
#42724=CARTESIAN_POINT('Ctrl Pts',(-3.2053322025275,1.06847604194505,3.50517104413015));
#42725=CARTESIAN_POINT('Ctrl Pts',(-3.21468940920784,1.18514270861179,3.48395990632891));
#42726=CARTESIAN_POINT('Ctrl Pts',(-3.21517590499961,1.30000000000008,3.46241539675136));
#42727=CARTESIAN_POINT('Ctrl Pts',(-3.01156878373355,-1.29999999999995,
3.32480522646398));
#42728=CARTESIAN_POINT('Ctrl Pts',(-3.01948628977715,-1.18514270861172,
3.35766374866596));
#42729=CARTESIAN_POINT('Ctrl Pts',(-3.02118250681312,-1.06847604194503,
3.39127799568841));
#42730=CARTESIAN_POINT('Ctrl Pts',(-3.01072868532105,-0.79477268400076,
3.47067950633485));
#42731=CARTESIAN_POINT('Ctrl Pts',(-2.97799510066786,-0.636309800095124,
3.52809178122447));
#42732=CARTESIAN_POINT('Ctrl Pts',(-2.95606711952232,-0.319434907277123,
3.59987576902135));
#42733=CARTESIAN_POINT('Ctrl Pts',(-2.93838859947651,-0.158333333333314,
3.63371139851771));
#42734=CARTESIAN_POINT('Ctrl Pts',(-2.96107261811187,0.158333333333316,
3.65239614836563));
#42735=CARTESIAN_POINT('Ctrl Pts',(-3.00164930281178,0.319434907277132,
3.63734668426724));
#42736=CARTESIAN_POINT('Ctrl Pts',(-3.06934679659287,0.636309800095134,
3.6034156103906));
#42737=CARTESIAN_POINT('Ctrl Pts',(-3.12735313425804,0.794772684000753,
3.56771055434906));
#42738=CARTESIAN_POINT('Ctrl Pts',(-3.17419280791191,1.06847604194507,3.51741101880181));
#42739=CARTESIAN_POINT('Ctrl Pts',(-3.18682899964134,1.18514270861181,3.49484687460461));
#42740=CARTESIAN_POINT('Ctrl Pts',(-3.19182622395639,1.3000000000001,3.47149139136714));
#42741=CARTESIAN_POINT('Ctrl Pts',(-2.98920415737631,-1.29999999999999,
3.33528254069167));
#42742=CARTESIAN_POINT('Ctrl Pts',(-2.99287348828336,-1.18514270861175,
3.37024236873661));
#42743=CARTESIAN_POINT('Ctrl Pts',(-2.99145726917786,-1.06847604194506,
3.40538690733707));
#42744=CARTESIAN_POINT('Ctrl Pts',(-2.97643688184066,-0.794772684000781,
3.48700454047947));
#42745=CARTESIAN_POINT('Ctrl Pts',(-2.94442040650366,-0.636309800095141,
3.54393732114147));
#42746=CARTESIAN_POINT('Ctrl Pts',(-2.92239826111222,-0.319434907277131,
3.61582450591124));
#42747=CARTESIAN_POINT('Ctrl Pts',(-2.90632539982685,-0.158333333333318,
3.6491943202188));
#42748=CARTESIAN_POINT('Ctrl Pts',(-2.92891834946343,0.15833333333332,3.66776284890486));
#42749=CARTESIAN_POINT('Ctrl Pts',(-2.96796626022347,0.31943490727714,3.65327266521064));
#42750=CARTESIAN_POINT('Ctrl Pts',(-3.03523030742018,0.636309800095151,
3.61857454417012));
#42751=CARTESIAN_POINT('Ctrl Pts',(-3.09163350657476,0.794772684000771,
3.58225353266621));
#42752=CARTESIAN_POINT('Ctrl Pts',(-3.14269960151707,1.0684760419451,3.52928505221333));
#42753=CARTESIAN_POINT('Ctrl Pts',(-3.15845027867044,1.18514270861184,3.505173206469));
#42754=CARTESIAN_POINT('Ctrl Pts',(-3.16784701266196,1.30000000000014,3.47987760749274));
#42755=CARTESIAN_POINT('Ctrl Pts',(-2.96717582248572,-1.3,3.34612443025397));
#42756=CARTESIAN_POINT('Ctrl Pts',(-2.96644096907686,-1.18514270861176,
3.38304333254976));
#42757=CARTESIAN_POINT('Ctrl Pts',(-2.96194864866568,-1.06847604194507,
3.41977717338575));
#42758=CARTESIAN_POINT('Ctrl Pts',(-2.94288998937622,-0.79477268400079,
3.50421216530303));
#42759=CARTESIAN_POINT('Ctrl Pts',(-2.91305103557942,-0.636309800095149,
3.56223763206484));
#42760=CARTESIAN_POINT('Ctrl Pts',(-2.89118884891162,-0.319434907277136,
3.63451512537704));
#42761=CARTESIAN_POINT('Ctrl Pts',(-2.87592686550002,-0.15833333333332,
3.66657569218735));
#42762=CARTESIAN_POINT('Ctrl Pts',(-2.89772479923798,0.158333333333322,
3.68426376399353));
#42763=CARTESIAN_POINT('Ctrl Pts',(-2.93478382345054,0.319434907277142,
3.66981881317108));
#42764=CARTESIAN_POINT('Ctrl Pts',(-3.00104865048769,0.636309800095157,
3.6337182358295));
#42765=CARTESIAN_POINT('Ctrl Pts',(-3.05541968820448,0.794772684000783,
3.59628564676238));
#42766=CARTESIAN_POINT('Ctrl Pts',(-3.11093941743452,1.06847604194512,3.54089763150643));
#42767=CARTESIAN_POINT('Ctrl Pts',(-3.13009221058491,1.18514270861186,3.51556002773706));
#42768=CARTESIAN_POINT('Ctrl Pts',(-3.14436536331071,1.30000000000015,3.48886023967439));
#42769=CARTESIAN_POINT('Ctrl Pts',(-2.95059618965475,-1.30000000000001,
3.35424938277405));
#42770=CARTESIAN_POINT('Ctrl Pts',(-2.94719414326373,-1.18514270861177,
3.39331003261898));
#42771=CARTESIAN_POINT('Ctrl Pts',(-2.94065773409478,-1.06847604194508,
3.43150988911155));
#42772=CARTESIAN_POINT('Ctrl Pts',(-2.9183163162662,-0.794772684000798,
3.5177705946194));
#42773=CARTESIAN_POINT('Ctrl Pts',(-2.8879929083895,-0.636309800095153,
3.57433989673292));
#42774=CARTESIAN_POINT('Ctrl Pts',(-2.86607142352026,-0.319434907277137,
3.64670989540203));
#42775=CARTESIAN_POINT('Ctrl Pts',(-2.85281501287045,-0.158333333333321,
3.67927548148163));
#42776=CARTESIAN_POINT('Ctrl Pts',(-2.87473723910272,0.158333333333323,
3.69709296118341));
#42777=CARTESIAN_POINT('Ctrl Pts',(-2.91016801870854,0.319434907277144,
3.682547053866));
#42778=CARTESIAN_POINT('Ctrl Pts',(-2.97622990338684,0.636309800095162,
3.64605811352108));
#42779=CARTESIAN_POINT('Ctrl Pts',(-3.03014457191045,0.794772684000788,
3.60909008270178));
#42780=CARTESIAN_POINT('Ctrl Pts',(-3.08869601229283,1.06847604194512,3.55153153788718));
#42781=CARTESIAN_POINT('Ctrl Pts',(-3.10993754230562,1.18514270861186,3.5247245089168));
#42782=CARTESIAN_POINT('Ctrl Pts',(-3.12707585333436,1.30000000000016,3.496025412272));
#42783=CARTESIAN_POINT('Ctrl Pts',(-2.93496317665334,-1.30000000000002,
3.3633063159341));
#42784=CARTESIAN_POINT('Ctrl Pts',(-2.92816594708533,-1.18514270861178,
3.40376717196528));
#42785=CARTESIAN_POINT('Ctrl Pts',(-2.91928145969323,-1.06847604194509,
3.44313428112175));
#42786=CARTESIAN_POINT('Ctrl Pts',(-2.89393453335372,-0.794772684000804,
3.5315534045525));
#42787=CARTESIAN_POINT('Ctrl Pts',(-2.86549588577109,-0.636309800095158,
3.5891825598255));
#42788=CARTESIAN_POINT('Ctrl Pts',(-2.84376814101127,-0.31943490727714,
3.66192324514565));
#42789=CARTESIAN_POINT('Ctrl Pts',(-2.83123177913598,-0.158333333333322,
3.69363560007842));
#42790=CARTESIAN_POINT('Ctrl Pts',(-2.85212603576051,0.158333333333324,
3.7103411018121));
#42791=CARTESIAN_POINT('Ctrl Pts',(-2.88524411637506,0.319434907277146,
3.69495745864312));
#42792=CARTESIAN_POINT('Ctrl Pts',(-2.95016857461147,0.636309800095166,
3.65701217155733));
#42793=CARTESIAN_POINT('Ctrl Pts',(-3.00278299985719,0.794772684000794,
3.6194600238106));
#42794=CARTESIAN_POINT('Ctrl Pts',(-3.06482687763757,1.06847604194513,3.56024830517271));
#42795=CARTESIAN_POINT('Ctrl Pts',(-3.08871428890777,1.18514270861187,3.53261894563116));
#42796=CARTESIAN_POINT('Ctrl Pts',(-3.10963261570928,1.30000000000017,3.50299078553598));
#42797=CARTESIAN_POINT('Ctrl Pts',(-2.91812360584106,-1.30000000000003,
3.37118251970176));
#42798=CARTESIAN_POINT('Ctrl Pts',(-2.90835133164569,-1.18514270861179,
3.41346968432624));
#42799=CARTESIAN_POINT('Ctrl Pts',(-2.89732666173695,-1.06847604194509,
3.45420874668576));
#42800=CARTESIAN_POINT('Ctrl Pts',(-2.86896418413129,-0.79477268400081,
3.54474770462891));
#42801=CARTESIAN_POINT('Ctrl Pts',(-2.84132230949808,-0.636309800095161,
3.60227634535726));
#42802=CARTESIAN_POINT('Ctrl Pts',(-2.81975603492678,-0.31943490727714,
3.67534138165594));
#42803=CARTESIAN_POINT('Ctrl Pts',(-2.80832531294812,-0.158333333333323,
3.70658812804784));
#42804=CARTESIAN_POINT('Ctrl Pts',(-2.82933027822802,0.158333333333325,
3.72342674960999));
#42805=CARTESIAN_POINT('Ctrl Pts',(-2.86165499703511,0.31943490727715,3.70888506187108));
#42806=CARTESIAN_POINT('Ctrl Pts',(-2.92623290821954,0.636309800095171,
3.6703911433026));
#42807=CARTESIAN_POINT('Ctrl Pts',(-2.97738454099281,0.794772684000797,
3.63216348213907));
#42808=CARTESIAN_POINT('Ctrl Pts',(-3.04213962224978,1.06847604194513,3.57041424133755));
#42809=CARTESIAN_POINT('Ctrl Pts',(-3.06811606390625,1.18514270861188,3.5413129890768));
#42810=CARTESIAN_POINT('Ctrl Pts',(-3.09203887195526,1.30000000000018,3.50983944286344));
#42811=CARTESIAN_POINT('Ctrl Pts',(-2.90564932299591,-1.30000000000003,
3.37931771926188));
#42812=CARTESIAN_POINT('Ctrl Pts',(-2.89344317979173,-1.18514270861179,
3.42319211348459));
#42813=CARTESIAN_POINT('Ctrl Pts',(-2.88063148381286,-1.06847604194509,
3.46508542032316));
#42814=CARTESIAN_POINT('Ctrl Pts',(-2.84963495508069,-0.79477268400081,
3.55729063167506));
#42815=CARTESIAN_POINT('Ctrl Pts',(-2.82234920049889,-0.636309800095163,
3.61442241467706));
#42816=CARTESIAN_POINT('Ctrl Pts',(-2.80075798336809,-0.319434907277142,
3.68759947538144));
#42817=CARTESIAN_POINT('Ctrl Pts',(-2.79049462724478,-0.158333333333324,
3.71871421775334));
#42818=CARTESIAN_POINT('Ctrl Pts',(-2.81118495158267,0.158333333333326,
3.73522940676952));
#42819=CARTESIAN_POINT('Ctrl Pts',(-2.84203410447534,0.319434907277151,
3.72051732347584));
#42820=CARTESIAN_POINT('Ctrl Pts',(-2.90598293766052,0.636309800095173,
3.68120972904556));
#42821=CARTESIAN_POINT('Ctrl Pts',(-2.95615812849188,0.794772684000799,
3.64268392562299));
#42822=CARTESIAN_POINT('Ctrl Pts',(-3.02343030207539,1.06847604194514,3.57911464656462));
#42823=CARTESIAN_POINT('Ctrl Pts',(-3.05130248589471,1.18514270861188,3.5489630235154));
#42824=CARTESIAN_POINT('Ctrl Pts',(-3.07792722226875,1.30000000000018,3.51617656284739));
#42825=CARTESIAN_POINT('Ctrl Pts',(-2.89444547446341,-1.30000000000004,
3.38460967377958));
#42826=CARTESIAN_POINT('Ctrl Pts',(-2.88025475037004,-1.18514270861179,
3.42970791994923));
#42827=CARTESIAN_POINT('Ctrl Pts',(-2.86605623064443,-1.0684760419451,3.47256285200525));
#42828=CARTESIAN_POINT('Ctrl Pts',(-2.83323680020414,-0.794772684000812,
3.56638381377852));
#42829=CARTESIAN_POINT('Ctrl Pts',(-2.806797447228,-0.636309800095164,3.623775853036));
#42830=CARTESIAN_POINT('Ctrl Pts',(-2.785528981377,-0.319434907277142,3.69738903397588));
#42831=CARTESIAN_POINT('Ctrl Pts',(-2.77617802870274,-0.158333333333324,
3.72836872085716));
#42832=CARTESIAN_POINT('Ctrl Pts',(-2.79663721708606,0.158333333333326,
3.74464778453676));
#42833=CARTESIAN_POINT('Ctrl Pts',(-2.82624199019963,0.319434907277151,
3.72974883334975));
#42834=CARTESIAN_POINT('Ctrl Pts',(-2.88960266939197,0.636309800095174,
3.68969891281971));
#42835=CARTESIAN_POINT('Ctrl Pts',(-2.93881369270205,0.7947726840008,3.65072013162558));
#42836=CARTESIAN_POINT('Ctrl Pts',(-3.00821350617473,1.06847604194514,3.58581320002371));
#42837=CARTESIAN_POINT('Ctrl Pts',(-3.03772064583979,1.18514270861188,3.55494927288839));
#42838=CARTESIAN_POINT('Ctrl Pts',(-3.06669431743411,1.30000000000018,3.52131722426934));
#42839=CARTESIAN_POINT('Ctrl Pts',(-2.87330971922871,-1.30000000000004,
3.39645550931658));
#42840=CARTESIAN_POINT('Ctrl Pts',(-2.8551151553052,-1.1851427086118,3.44396806456762));
#42841=CARTESIAN_POINT('Ctrl Pts',(-2.83807033144944,-1.0684760419451,3.48867366979621));
#42842=CARTESIAN_POINT('Ctrl Pts',(-2.80134950809849,-0.794772684000815,
3.58546794511965));
#42843=CARTESIAN_POINT('Ctrl Pts',(-2.77633178278127,-0.636309800095167,
3.64310304084678));
#42844=CARTESIAN_POINT('Ctrl Pts',(-2.75528781624004,-0.319434907277144,
3.71716182931582));
#42845=CARTESIAN_POINT('Ctrl Pts',(-2.74728825573495,-0.158333333333325,
3.74738689262068));
#42846=CARTESIAN_POINT('Ctrl Pts',(-2.76738199808109,0.158333333333327,
3.76330543314258));
#42847=CARTESIAN_POINT('Ctrl Pts',(-2.79518745255115,0.319434907277151,
3.74874413442973));
#42848=CARTESIAN_POINT('Ctrl Pts',(-2.85774725188071,0.636309800095175,
3.70762922705557));
#42849=CARTESIAN_POINT('Ctrl Pts',(-2.90540089433975,0.794772684000803,
3.66821008494076));
#42850=CARTESIAN_POINT('Ctrl Pts',(-2.97837586044864,1.06847604194514,3.59988687467182));
#42851=CARTESIAN_POINT('Ctrl Pts',(-3.01059956725001,1.18514270861189,3.56698250495343));
#42852=CARTESIAN_POINT('Ctrl Pts',(-3.04345882201318,1.30000000000019,3.53074835161764));
#42853=CARTESIAN_POINT('Ctrl Pts',(-2.84986342692003,-1.30000000000005,
3.41016373782283));
#42854=CARTESIAN_POINT('Ctrl Pts',(-2.8278002227937,-1.18514270861181,3.46104959590005));
#42855=CARTESIAN_POINT('Ctrl Pts',(-2.80797992245507,-1.06847604194511,
3.50827599494446));
#42856=CARTESIAN_POINT('Ctrl Pts',(-2.76737262007632,-0.794772684000818,
3.60892434190774));
#42857=CARTESIAN_POINT('Ctrl Pts',(-2.74358827141872,-0.63630980009517,
3.66642463388269));
#42858=CARTESIAN_POINT('Ctrl Pts',(-2.7225206234019,-0.319434907277146,
3.74071141836457));
#42859=CARTESIAN_POINT('Ctrl Pts',(-2.71569615971129,-0.158333333333326,
3.76977449773877));
#42860=CARTESIAN_POINT('Ctrl Pts',(-2.73515410718614,0.158333333333328,
3.78508150889321));
#42861=CARTESIAN_POINT('Ctrl Pts',(-2.76108477126121,0.319434907277156,
3.77105713136288));
#42862=CARTESIAN_POINT('Ctrl Pts',(-2.82250334076209,0.636309800095182,
3.7284961532079));
#42863=CARTESIAN_POINT('Ctrl Pts',(-2.86770375781189,0.794772684000808,
3.68782644460456));
#42864=CARTESIAN_POINT('Ctrl Pts',(-2.9449882645546,1.06847604194515,3.61598218052369));
#42865=CARTESIAN_POINT('Ctrl Pts',(-2.98061577717813,1.1851427086119,3.58116393341142));
#42866=CARTESIAN_POINT('Ctrl Pts',(-3.01841720312947,1.3000000000002,3.54262615901515));
#42867=CARTESIAN_POINT('Ctrl Pts',(-2.81674957134945,-1.30000000000007,
3.43070471365389));
#42868=CARTESIAN_POINT('Ctrl Pts',(-2.78856312709208,-1.18514270861182,
3.48590126687021));
#42869=CARTESIAN_POINT('Ctrl Pts',(-2.76447074598642,-1.06847604194512,
3.5364820539981));
#42870=CARTESIAN_POINT('Ctrl Pts',(-2.71827063086294,-0.794772684000828,
3.64267044787023));
#42871=CARTESIAN_POINT('Ctrl Pts',(-2.69707890134858,-0.636309800095181,
3.7007813262518));
#42872=CARTESIAN_POINT('Ctrl Pts',(-2.67718366416938,-0.319434907277152,
3.77653842687141));
#42873=CARTESIAN_POINT('Ctrl Pts',(-2.67360251051884,-0.158333333333328,
3.80535560502423));
#42874=CARTESIAN_POINT('Ctrl Pts',(-2.69217396507023,0.15833333333333,3.81984616809613));
#42875=CARTESIAN_POINT('Ctrl Pts',(-2.71361121935058,0.319434907277159,
3.80495169052859));
#42876=CARTESIAN_POINT('Ctrl Pts',(-2.77279229669294,0.63630980009519,3.75986751852911));
#42877=CARTESIAN_POINT('Ctrl Pts',(-2.81558792137091,0.794772684000822,
3.71868470650039));
#42878=CARTESIAN_POINT('Ctrl Pts',(-2.89829007054551,1.06847604194517,3.64094211848186));
#42879=CARTESIAN_POINT('Ctrl Pts',(-2.93814406855001,1.18514270861192,3.60262063460224));
#42880=CARTESIAN_POINT('Ctrl Pts',(-2.98205336859798,1.30000000000022,3.55962955254944));
#42881=CARTESIAN_POINT('Ctrl Pts',(-2.79130385555554,-1.30000000000009,
3.44659963092747));
#42882=CARTESIAN_POINT('Ctrl Pts',(-2.75880839581699,-1.18514270861184,
3.50557743686655));
#42883=CARTESIAN_POINT('Ctrl Pts',(-2.73177596756767,-1.06847604194514,
3.55912180261392));
#42884=CARTESIAN_POINT('Ctrl Pts',(-2.68194634610882,-0.794772684000846,
3.6702676652052));
#42885=CARTESIAN_POINT('Ctrl Pts',(-2.66344640491833,-0.63630980009519,
3.72941821861195));
#42886=CARTESIAN_POINT('Ctrl Pts',(-2.64402530993783,-0.319434907277155,
3.80590712414196));
#42887=CARTESIAN_POINT('Ctrl Pts',(-2.6411804093813,-0.158333333333331,
3.83290762524055));
#42888=CARTESIAN_POINT('Ctrl Pts',(-2.65893027932983,0.158333333333333,
3.8466908829489));
#42889=CARTESIAN_POINT('Ctrl Pts',(-2.67853367145776,0.319434907277164,
3.83273256017458));
#42890=CARTESIAN_POINT('Ctrl Pts',(-2.73612933986299,0.6363098000952,3.78582868351487));
#42891=CARTESIAN_POINT('Ctrl Pts',(-2.77568686749433,0.794772684000833,
3.74284458125839));
#42892=CARTESIAN_POINT('Ctrl Pts',(-2.86255676382707,1.06847604194518,3.66051962129997));
#42893=CARTESIAN_POINT('Ctrl Pts',(-2.90591827320911,1.18514270861193,3.61973496937537));
#42894=CARTESIAN_POINT('Ctrl Pts',(-2.95503853269762,1.30000000000023,3.57380109025177));
#42895=CARTESIAN_POINT('Ctrl Pts',(-2.76631964265226,-1.3000000000001,3.46290077644001));
#42896=CARTESIAN_POINT('Ctrl Pts',(-2.72970063932157,-1.18514270861185,
3.52572570840152));
#42897=CARTESIAN_POINT('Ctrl Pts',(-2.6998918952725,-1.06847604194514,3.58230084560764));
#42898=CARTESIAN_POINT('Ctrl Pts',(-2.64676079462857,-0.794772684000846,
3.69856245421907));
#42899=CARTESIAN_POINT('Ctrl Pts',(-2.63084342365516,-0.636309800095192,
3.75862307933041));
#42900=CARTESIAN_POINT('Ctrl Pts',(-2.61262197752267,-0.319434907277157,
3.83646439589201));
#42901=CARTESIAN_POINT('Ctrl Pts',(-2.61177277019272,-0.158333333333331,
3.8628068404394));
#42902=CARTESIAN_POINT('Ctrl Pts',(-2.62883796386496,0.158333333333333,
3.87603367277299));
#42903=CARTESIAN_POINT('Ctrl Pts',(-2.64544299217718,0.319434907277164,
3.86194356483978));
#42904=CARTESIAN_POINT('Ctrl Pts',(-2.7010921069768,0.636309800095201,3.81302933099263));
#42905=CARTESIAN_POINT('Ctrl Pts',(-2.73826067334614,0.794772684000835,
3.76925102704878));
#42906=CARTESIAN_POINT('Ctrl Pts',(-2.82855844984348,1.06847604194519,3.68175244662319));
#42907=CARTESIAN_POINT('Ctrl Pts',(-2.87481506609588,1.18514270861194,3.63794176287807));
#42908=CARTESIAN_POINT('Ctrl Pts',(-2.92824173701734,1.30000000000024,3.58819528871212));
#42909=CARTESIAN_POINT('Ctrl Pts',(-2.74946991434193,-1.3000000000001,3.4750205202169));
#42910=CARTESIAN_POINT('Ctrl Pts',(-2.70989262720101,-1.18514270861185,
3.54066783837951));
#42911=CARTESIAN_POINT('Ctrl Pts',(-2.67815184852736,-1.06847604194515,
3.59951550166289));
#42912=CARTESIAN_POINT('Ctrl Pts',(-2.62292820231771,-0.79477268400085,
3.71975681324494));
#42913=CARTESIAN_POINT('Ctrl Pts',(-2.61001698334349,-0.636309800095195,
3.78147580120014));
#42914=CARTESIAN_POINT('Ctrl Pts',(-2.59160966732343,-0.319434907277159,
3.85936426630499));
#42915=CARTESIAN_POINT('Ctrl Pts',(-2.58917887281194,-0.158333333333332,
3.88254430379007));
#42916=CARTESIAN_POINT('Ctrl Pts',(-2.60530601519066,0.158333333333334,
3.89499485143002));
#42917=CARTESIAN_POINT('Ctrl Pts',(-2.62206510686829,0.319434907277166,
3.88292248440957));
#42918=CARTESIAN_POINT('Ctrl Pts',(-2.67698636889789,0.636309800095204,
3.83313023249387));
#42919=CARTESIAN_POINT('Ctrl Pts',(-2.7116317122864,0.79477268400084,3.78796944947533));
#42920=CARTESIAN_POINT('Ctrl Pts',(-2.80431412364808,1.06847604194519,3.69660834519858));
#42921=CARTESIAN_POINT('Ctrl Pts',(-2.85269008915142,1.18514270861194,3.65063022732966));
#42922=CARTESIAN_POINT('Ctrl Pts',(-2.9093232385014,1.30000000000025,3.59822082837069));
#42923=CARTESIAN_POINT('Ctrl Pts',(-2.73730164354872,-1.3000000000001,3.48341371040716));
#42924=CARTESIAN_POINT('Ctrl Pts',(-2.69639517330247,-1.18514270861185,
3.55150847404721));
#42925=CARTESIAN_POINT('Ctrl Pts',(-2.66354727608036,-1.06847604194515,
3.61201581798988));
#42926=CARTESIAN_POINT('Ctrl Pts',(-2.60627897809573,-0.794772684000851,
3.73427142959104));
#42927=CARTESIAN_POINT('Ctrl Pts',(-2.59253840770018,-0.636309800095194,
3.79450670463528));
#42928=CARTESIAN_POINT('Ctrl Pts',(-2.57345094230685,-0.319434907277157,
3.87182862652423));
#42929=CARTESIAN_POINT('Ctrl Pts',(-2.57134736188519,-0.158333333333332,
3.89403237082244));
#42930=CARTESIAN_POINT('Ctrl Pts',(-2.58789598152809,0.158333333333334,
3.90688493738757));
#42931=CARTESIAN_POINT('Ctrl Pts',(-2.60538706360735,0.319434907277166,
3.89677292530911));
#42932=CARTESIAN_POINT('Ctrl Pts',(-2.6605479894059,0.636309800095203,3.84718052087746));
#42933=CARTESIAN_POINT('Ctrl Pts',(-2.6936693350233,0.794772684000836,3.80141423297618));
#42934=CARTESIAN_POINT('Ctrl Pts',(-2.78812801035164,1.06847604194519,3.70775389303389));
#42935=CARTESIAN_POINT('Ctrl Pts',(-2.8379363203858,1.18514270861194,3.66037192978858));
#42936=CARTESIAN_POINT('Ctrl Pts',(-2.89666527994333,1.30000000000025,3.60615009400136));
#42937=CARTESIAN_POINT('Ctrl Pts',(-2.72326627312501,-1.3000000000001,3.49418507966825));
#42938=CARTESIAN_POINT('Ctrl Pts',(-2.68052794672654,-1.18514270861185,
3.56550529007524));
#42939=CARTESIAN_POINT('Ctrl Pts',(-2.64601630303685,-1.06847604194515,
3.62810375107432));
#42940=CARTESIAN_POINT('Ctrl Pts',(-2.58529278488251,-0.79477268400085,
3.75256973284915));
#42941=CARTESIAN_POINT('Ctrl Pts',(-2.56937357584712,-0.636309800095195,
3.81013291795898));
#42942=CARTESIAN_POINT('Ctrl Pts',(-2.5485676946795,-0.319434907277158,
3.88615363414296));
#42943=CARTESIAN_POINT('Ctrl Pts',(-2.54703863299078,-0.158333333333332,
3.9071876744658));
#42944=CARTESIAN_POINT('Ctrl Pts',(-2.56350678782447,0.158333333333334,
3.91999872873124));
#42945=CARTESIAN_POINT('Ctrl Pts',(-2.58059607962984,0.319434907277166,
3.91126747183114));
#42946=CARTESIAN_POINT('Ctrl Pts',(-2.63679578372307,0.636309800095204,
3.86237726186916));
#42947=CARTESIAN_POINT('Ctrl Pts',(-2.67065942773071,0.794772684000837,
3.81796691311235));
#42948=CARTESIAN_POINT('Ctrl Pts',(-2.76844578138871,1.06847604194519,3.72190506081139));
#42949=CARTESIAN_POINT('Ctrl Pts',(-2.82018062835327,1.18514270861195,3.67262192434545));
#42950=CARTESIAN_POINT('Ctrl Pts',(-2.88132223312535,1.30000000000025,3.61563726783222));
#42951=CARTESIAN_POINT('Ctrl Pts',(-2.71361311550265,-1.30000000000011,
3.50143025308128));
#42952=CARTESIAN_POINT('Ctrl Pts',(-2.67063753707723,-1.18514270861185,
3.57586971597518));
#42953=CARTESIAN_POINT('Ctrl Pts',(-2.63543757366511,-1.06847604194515,
3.64017761461974));
#42954=CARTESIAN_POINT('Ctrl Pts',(-2.57208184264171,-0.794772684000851,
3.76533578501125));
#42955=CARTESIAN_POINT('Ctrl Pts',(-2.55201129877974,-0.636309800095197,
3.81776217389487));
#42956=CARTESIAN_POINT('Ctrl Pts',(-2.52893211648025,-0.319434907277159,
3.89115367806483));
#42957=CARTESIAN_POINT('Ctrl Pts',(-2.52830982650113,-0.158333333333332,
3.91159193529207));
#42958=CARTESIAN_POINT('Ctrl Pts',(-2.54469368659007,0.158333333333334,
3.92427691489317));
#42959=CARTESIAN_POINT('Ctrl Pts',(-2.56094950441052,0.319434907277167,
3.9160722157167));
#42960=CARTESIAN_POINT('Ctrl Pts',(-2.61892980279681,0.636309800095206,
3.86943861483994));
#42961=CARTESIAN_POINT('Ctrl Pts',(-2.65591208556864,0.79477268400084,3.82959034377962));
#42962=CARTESIAN_POINT('Ctrl Pts',(-2.75637070809807,1.0684760419452,3.73285743382662));
#42963=CARTESIAN_POINT('Ctrl Pts',(-2.80906926850999,1.18514270861195,3.68202709105594));
#42964=CARTESIAN_POINT('Ctrl Pts',(-2.87098157399966,1.30000000000025,3.62223849792565));
#42965=CARTESIAN_POINT('Ctrl Pts',(-2.70549646903683,-1.30000000000011,
3.50427905152384));
#42966=CARTESIAN_POINT('Ctrl Pts',(-2.66274685239523,-1.18514270861185,
3.57860852562495));
#42967=CARTESIAN_POINT('Ctrl Pts',(-2.62751487735364,-1.06847604194515,
3.64257305686797));
#42968=CARTESIAN_POINT('Ctrl Pts',(-2.56348922287021,-0.794772684000851,
3.76639882859812));
#42969=CARTESIAN_POINT('Ctrl Pts',(-2.54183416968341,-0.636309800095197,
3.81680720028708));
#42970=CARTESIAN_POINT('Ctrl Pts',(-2.5177651372377,-0.319434907277159,
3.88883314466868));
#42971=CARTESIAN_POINT('Ctrl Pts',(-2.5171210925739,-0.158333333333332,
3.90931901361983));
#42972=CARTESIAN_POINT('Ctrl Pts',(-2.53338410693288,0.158333333333334,
3.92180031843115));
#42973=CARTESIAN_POINT('Ctrl Pts',(-2.54937394678571,0.319434907277167,
3.91311942209051));
#42974=CARTESIAN_POINT('Ctrl Pts',(-2.60843787791201,0.636309800095206,
3.86789463692126));
#42975=CARTESIAN_POINT('Ctrl Pts',(-2.64769917658169,0.79477268400084,3.83089639236956));
#42976=CARTESIAN_POINT('Ctrl Pts',(-2.74872068765948,1.0684760419452,3.73538570642258));
#42977=CARTESIAN_POINT('Ctrl Pts',(-2.80123722412075,1.18514270861195,3.68466093919396));
#42978=CARTESIAN_POINT('Ctrl Pts',(-2.8625418281136,1.30000000000025,3.62455444166347));
#42979=CARTESIAN_POINT('Ctrl Pts',(-2.70549646903679,-1.3,3.50427905152391));
#42980=CARTESIAN_POINT('Ctrl Pts',(-2.6627468523952,-1.18514270861178,3.57860852562499));
#42981=CARTESIAN_POINT('Ctrl Pts',(-2.62751487735363,-1.06847604194512,
3.64257305686799));
#42982=CARTESIAN_POINT('Ctrl Pts',(-2.56348922287021,-0.794772684000851,
3.76639882859813));
#42983=CARTESIAN_POINT('Ctrl Pts',(-2.54183416968341,-0.636309800095197,
3.81680720028709));
#42984=CARTESIAN_POINT('Ctrl Pts',(-2.5177651372377,-0.319434907277159,
3.88883314466869));
#42985=CARTESIAN_POINT('Ctrl Pts',(-2.5171210925739,-0.158333333333332,
3.90931901361984));
#42986=CARTESIAN_POINT('Ctrl Pts',(-2.53338410693288,0.158333333333334,
3.92180031843115));
#42987=CARTESIAN_POINT('Ctrl Pts',(-2.54937394678571,0.319434907277167,
3.91311942209052));
#42988=CARTESIAN_POINT('Ctrl Pts',(-2.60843787791201,0.636309800095206,
3.86789463692126));
#42989=CARTESIAN_POINT('Ctrl Pts',(-2.64769917658169,0.79477268400084,3.83089639236956));
#42990=CARTESIAN_POINT('Ctrl Pts',(-2.74872068765945,1.06847604194511,3.73538570642261));
#42991=CARTESIAN_POINT('Ctrl Pts',(-2.80123722412067,1.18514270861178,3.68466093919403));
#42992=CARTESIAN_POINT('Ctrl Pts',(-2.86254182811346,1.3,3.6245544416636));
#42993=CARTESIAN_POINT('',(-3.07985614647943,-1.2,3.32482437598077));
#42994=CARTESIAN_POINT('Ctrl Pts',(-3.07985614647943,-1.2,3.32482437598077));
#42995=CARTESIAN_POINT('Ctrl Pts',(-3.05880159510405,-1.21682960324337,
3.32958843015044));
#42996=CARTESIAN_POINT('Ctrl Pts',(-3.03724401462398,-1.23325611740907,
3.33351507474704));
#42997=CARTESIAN_POINT('Ctrl Pts',(-3.00530433450824,-1.258663098968,3.3408068297737));
#42998=CARTESIAN_POINT('Ctrl Pts',(-2.99504539268032,-1.26676816617002,
3.34309739992352));
#42999=CARTESIAN_POINT('Ctrl Pts',(-2.97658205919368,-1.28145232253012,
3.34737148534885));
#43000=CARTESIAN_POINT('Ctrl Pts',(-2.96351143750541,-1.29188182284861,
3.35046321236999));
#43001=CARTESIAN_POINT('Ctrl Pts',(-2.95536211928798,-1.29845781721288,
3.35249474764391));
#43002=CARTESIAN_POINT('Ctrl Pts',(-2.95440882469644,-1.29922951092393,
3.35273562153213));
#43003=CARTESIAN_POINT('Ctrl Pts',(-2.95346134579773,-1.30000000000001,
3.35297958429143));
#43004=CARTESIAN_POINT('',(-3.20083482100771,-0.653834841416722,3.42413500660232));
#43005=CARTESIAN_POINT('Ctrl Pts',(-3.20083482102253,-0.653834841416035,
3.42413500658066));
#43006=CARTESIAN_POINT('Ctrl Pts',(-3.18844346496178,-0.717856496133803,
3.41363074225233));
#43007=CARTESIAN_POINT('Ctrl Pts',(-3.17828009865403,-0.76380352052981,
3.40509366942734));
#43008=CARTESIAN_POINT('Ctrl Pts',(-3.13843063020648,-0.949540435597171,
3.37194717193105));
#43009=CARTESIAN_POINT('Ctrl Pts',(-3.11738257533065,-1.04584243573993,
3.35464908943026));
#43010=CARTESIAN_POINT('Ctrl Pts',(-3.07985614647943,-1.2,3.32482437598077));
#43011=CARTESIAN_POINT('',(-3.30596887606183,0.653834841531101,3.5158352655574));
#43012=CARTESIAN_POINT('Ctrl Pts',(-3.30596887606183,0.653834841531103,
3.5158352655574));
#43013=CARTESIAN_POINT('Ctrl Pts',(-3.26766136519301,0.57579115138873,3.53224551669641));
#43014=CARTESIAN_POINT('Ctrl Pts',(-3.23529265065951,0.493921174124157,
3.54536768290475));
#43015=CARTESIAN_POINT('Ctrl Pts',(-3.18741895852824,0.338203882217178,
3.56202990461054));
#43016=CARTESIAN_POINT('Ctrl Pts',(-3.17012611474238,0.26571581271928,3.566711121231));
#43017=CARTESIAN_POINT('Ctrl Pts',(-3.14580748980259,0.129742913188357,
3.56886089494024));
#43018=CARTESIAN_POINT('Ctrl Pts',(-3.13766993333606,0.0666421442921237,
3.56730149091443));
#43019=CARTESIAN_POINT('Ctrl Pts',(-3.12737311469443,-0.059551760498374,
3.55881396747486));
#43020=CARTESIAN_POINT('Ctrl Pts',(-3.12512389889361,-0.12280055430268,
3.55183348127266));
#43021=CARTESIAN_POINT('Ctrl Pts',(-3.12735116187767,-0.260149022110592,
3.531205618682));
#43022=CARTESIAN_POINT('Ctrl Pts',(-3.1331253832472,-0.333947687247939,
3.51657228235298));
#43023=CARTESIAN_POINT('Ctrl Pts',(-3.15628326243836,-0.491233450801308,
3.47816085215487));
#43024=CARTESIAN_POINT('Ctrl Pts',(-3.17536914576921,-0.57417245107474,
3.45312723759055));
#43025=CARTESIAN_POINT('Ctrl Pts',(-3.20083482096744,-0.653834841428439,
3.42413500659914));
#43026=CARTESIAN_POINT('',(-3.25186354350228,1.2,3.46799202915631));
#43027=CARTESIAN_POINT('Ctrl Pts',(-3.25186354350228,1.2,3.46799202915631));
#43028=CARTESIAN_POINT('Ctrl Pts',(-3.26156466363528,1.13197267961548,3.47644504403145));
#43029=CARTESIAN_POINT('Ctrl Pts',(-3.27383226153768,1.03501542741823,3.48720372632373));
#43030=CARTESIAN_POINT('Ctrl Pts',(-3.29731825275506,0.795382507989234,
3.50806756723355));
#43031=CARTESIAN_POINT('Ctrl Pts',(-3.30107256523771,0.741804412431255,
3.51144158276664));
#43032=CARTESIAN_POINT('Ctrl Pts',(-3.30596887606183,0.653834841531101,
3.5158352655574));
#43033=CARTESIAN_POINT('Ctrl Pts',(-3.12967817046589,1.29999999999997,3.4949204395439));
#43034=CARTESIAN_POINT('Ctrl Pts',(-3.14980150842174,1.28313646799302,3.48984401448758));
#43035=CARTESIAN_POINT('Ctrl Pts',(-3.1703340625042,1.26654363612861,3.48553070234103));
#43036=CARTESIAN_POINT('Ctrl Pts',(-3.20568221938911,1.23742285157402,3.47748741921129));
#43037=CARTESIAN_POINT('Ctrl Pts',(-3.22638995040895,1.22006242765915,3.47240583757775));
#43038=CARTESIAN_POINT('Ctrl Pts',(-3.25186354350228,1.2,3.46799202915631));
#43039=CARTESIAN_POINT('Ctrl Pts',(-2.70549646903679,-1.3,3.50427905152391));
#43040=CARTESIAN_POINT('Ctrl Pts',(-2.6627468523952,-1.18514270861178,3.57860852562499));
#43041=CARTESIAN_POINT('Ctrl Pts',(-2.62751487735363,-1.06847604194512,
3.64257305686799));
#43042=CARTESIAN_POINT('Ctrl Pts',(-2.56348922287021,-0.794772684000851,
3.76639882859812));
#43043=CARTESIAN_POINT('Ctrl Pts',(-2.54183416968341,-0.636309800095197,
3.81680720028708));
#43044=CARTESIAN_POINT('Ctrl Pts',(-2.5177651372377,-0.319434907277159,
3.88883314466869));
#43045=CARTESIAN_POINT('Ctrl Pts',(-2.5171210925739,-0.158333333333332,
3.90931901361984));
#43046=CARTESIAN_POINT('Ctrl Pts',(-2.53338410693288,0.158333333333335,
3.92180031843115));
#43047=CARTESIAN_POINT('Ctrl Pts',(-2.54937394678571,0.319434907277167,
3.91311942209052));
#43048=CARTESIAN_POINT('Ctrl Pts',(-2.60843787791201,0.636309800095206,
3.86789463692126));
#43049=CARTESIAN_POINT('Ctrl Pts',(-2.64769917658169,0.79477268400084,3.83089639236956));
#43050=CARTESIAN_POINT('Ctrl Pts',(-2.74872068765945,1.06847604194511,3.73538570642261));
#43051=CARTESIAN_POINT('Ctrl Pts',(-2.80123722412067,1.18514270861178,3.68466093919403));
#43052=CARTESIAN_POINT('Ctrl Pts',(-2.86254182811346,1.3,3.6245544416636));
#43053=CARTESIAN_POINT('Ctrl Pts',(-2.64228988766393,-1.3,3.46041520142157));
#43054=CARTESIAN_POINT('Ctrl Pts',(-2.60104997267594,-1.18514270861178,
3.53559420826078));
#43055=CARTESIAN_POINT('Ctrl Pts',(-2.5668907832622,-1.06847604194512,3.60011089886413));
#43056=CARTESIAN_POINT('Ctrl Pts',(-2.50433411476486,-0.794772684000851,
3.72452527718372));
#43057=CARTESIAN_POINT('Ctrl Pts',(-2.48221240828625,-0.636309800095197,
3.77438845839854));
#43058=CARTESIAN_POINT('Ctrl Pts',(-2.45791319726889,-0.319434907277159,
3.84578854257292));
#43059=CARTESIAN_POINT('Ctrl Pts',(-2.4563788705663,-0.158333333333332,
3.86540905050109));
#43060=CARTESIAN_POINT('Ctrl Pts',(-2.47285287150207,0.158333333333335,
3.87759995720264));
#43061=CARTESIAN_POINT('Ctrl Pts',(-2.48994083087453,0.319434907277167,
3.86949835813398));
#43062=CARTESIAN_POINT('Ctrl Pts',(-2.54967111951957,0.636309800095206,
3.82429908435506));
#43063=CARTESIAN_POINT('Ctrl Pts',(-2.58959512893996,0.79477268400084,3.7875761803357));
#43064=CARTESIAN_POINT('Ctrl Pts',(-2.68960290025109,1.06847604194511,3.69085029513349));
#43065=CARTESIAN_POINT('Ctrl Pts',(-2.7412627929643,1.18514270861178,3.63927587476892));
#43066=CARTESIAN_POINT('Ctrl Pts',(-2.80129291984328,1.3,3.57799608569654));
#43067=CARTESIAN_POINT('Ctrl Pts',(-2.57908330629107,-1.3,3.41655135131923));
#43068=CARTESIAN_POINT('Ctrl Pts',(-2.53935309295667,-1.18514270861178,
3.49257989089658));
#43069=CARTESIAN_POINT('Ctrl Pts',(-2.50626668917078,-1.06847604194512,
3.55764874086027));
#43070=CARTESIAN_POINT('Ctrl Pts',(-2.4451790066595,-0.794772684000851,
3.68265172576931));
#43071=CARTESIAN_POINT('Ctrl Pts',(-2.42259064688909,-0.636309800095197,
3.73196971650999));
#43072=CARTESIAN_POINT('Ctrl Pts',(-2.39806125730008,-0.319434907277159,
3.80274394047715));
#43073=CARTESIAN_POINT('Ctrl Pts',(-2.3956366485587,-0.158333333333332,
3.82149908738234));
#43074=CARTESIAN_POINT('Ctrl Pts',(-2.41232163607126,0.158333333333335,
3.83339959597414));
#43075=CARTESIAN_POINT('Ctrl Pts',(-2.43050771496334,0.319434907277167,
3.82587729417744));
#43076=CARTESIAN_POINT('Ctrl Pts',(-2.49090436112714,0.636309800095206,
3.78070353178886));
#43077=CARTESIAN_POINT('Ctrl Pts',(-2.53149108129823,0.79477268400084,3.74425596830185));
#43078=CARTESIAN_POINT('Ctrl Pts',(-2.63048511284273,1.06847604194511,3.64631488384437));
#43079=CARTESIAN_POINT('Ctrl Pts',(-2.68128836180793,1.18514270861178,3.59389081034381));
#43080=CARTESIAN_POINT('Ctrl Pts',(-2.74004401157309,1.3,3.53143772972948));
#43081=CARTESIAN_POINT('Ctrl Pts',(-2.5158767249182,-1.3,3.37268750121688));
#43082=CARTESIAN_POINT('Ctrl Pts',(-2.47765621323741,-1.18514270861178,
3.44956557353237));
#43083=CARTESIAN_POINT('Ctrl Pts',(-2.44564259507935,-1.06847604194512,
3.51518658285641));
#43084=CARTESIAN_POINT('Ctrl Pts',(-2.38602389855415,-0.794772684000851,
3.64077817435491));
#43085=CARTESIAN_POINT('Ctrl Pts',(-2.36296888549193,-0.636309800095197,
3.68955097462145));
#43086=CARTESIAN_POINT('Ctrl Pts',(-2.33820931733128,-0.319434907277159,
3.75969933838138));
#43087=CARTESIAN_POINT('Ctrl Pts',(-2.33489442655109,-0.158333333333332,
3.77758912426359));
#43088=CARTESIAN_POINT('Ctrl Pts',(-2.35179040064045,0.158333333333335,
3.78919923474563));
#43089=CARTESIAN_POINT('Ctrl Pts',(-2.37107459905216,0.319434907277167,
3.7822562302209));
#43090=CARTESIAN_POINT('Ctrl Pts',(-2.43213760273471,0.636309800095206,
3.73710797922266));
#43091=CARTESIAN_POINT('Ctrl Pts',(-2.4733870336565,0.79477268400084,3.70093575626799));
#43092=CARTESIAN_POINT('Ctrl Pts',(-2.57136732543437,1.06847604194511,3.60177947255526));
#43093=CARTESIAN_POINT('Ctrl Pts',(-2.62131393065155,1.18514270861178,3.54850574591871));
#43094=CARTESIAN_POINT('Ctrl Pts',(-2.67879510330291,1.3,3.48487937376242));
#43095=CARTESIAN_POINT('Ctrl Pts',(-2.5158767249182,-1.3,3.37268750121688));
#43096=CARTESIAN_POINT('Ctrl Pts',(-2.47765621323741,-1.18514270861178,
3.44956557353237));
#43097=CARTESIAN_POINT('Ctrl Pts',(-2.44564259507935,-1.06847604194512,
3.51518658285641));
#43098=CARTESIAN_POINT('Ctrl Pts',(-2.38602389855415,-0.794772684000851,
3.64077817435491));
#43099=CARTESIAN_POINT('Ctrl Pts',(-2.36296888549193,-0.636309800095197,
3.68955097462145));
#43100=CARTESIAN_POINT('Ctrl Pts',(-2.33820931733128,-0.319434907277159,
3.75969933838138));
#43101=CARTESIAN_POINT('Ctrl Pts',(-2.33489442655109,-0.158333333333332,
3.77758912426359));
#43102=CARTESIAN_POINT('Ctrl Pts',(-2.35179040064045,0.158333333333334,
3.78919923474563));
#43103=CARTESIAN_POINT('Ctrl Pts',(-2.37107459905216,0.319434907277167,
3.7822562302209));
#43104=CARTESIAN_POINT('Ctrl Pts',(-2.4321376027347,0.636309800095206,3.73710797922267));
#43105=CARTESIAN_POINT('Ctrl Pts',(-2.4733870336565,0.79477268400084,3.70093575626799));
#43106=CARTESIAN_POINT('Ctrl Pts',(-2.57136732543437,1.06847604194511,3.60177947255526));
#43107=CARTESIAN_POINT('Ctrl Pts',(-2.62131393065155,1.18514270861178,3.54850574591871));
#43108=CARTESIAN_POINT('Ctrl Pts',(-2.67879510330291,1.3,3.48487937376242));
#43109=CARTESIAN_POINT('Ctrl Pts',(-2.51587672491883,-1.30000000000188,
3.37268750121562));
#43110=CARTESIAN_POINT('Ctrl Pts',(-2.47765621323776,-1.18514270861306,
3.44956557353166));
#43111=CARTESIAN_POINT('Ctrl Pts',(-2.44564259507949,-1.06847604194576,
3.51518658285611));
#43112=CARTESIAN_POINT('Ctrl Pts',(-2.38602389855415,-0.794772684000851,
3.64077817435491));
#43113=CARTESIAN_POINT('Ctrl Pts',(-2.36296888549193,-0.636309800095197,
3.68955097462145));
#43114=CARTESIAN_POINT('Ctrl Pts',(-2.33820931733127,-0.319434907277159,
3.75969933838138));
#43115=CARTESIAN_POINT('Ctrl Pts',(-2.33489442655109,-0.158333333333332,
3.77758912426359));
#43116=CARTESIAN_POINT('Ctrl Pts',(-2.35179040064045,0.158333333333335,
3.78919923474563));
#43117=CARTESIAN_POINT('Ctrl Pts',(-2.37107459905216,0.319434907277167,
3.7822562302209));
#43118=CARTESIAN_POINT('Ctrl Pts',(-2.43213760273471,0.636309800095207,
3.73710797922267));
#43119=CARTESIAN_POINT('Ctrl Pts',(-2.4733870336565,0.79477268400084,3.70093575626799));
#43120=CARTESIAN_POINT('Ctrl Pts',(-2.57136732543453,1.06847604194556,3.6017794725551));
#43121=CARTESIAN_POINT('Ctrl Pts',(-2.62131393065193,1.18514270861267,3.5485057459183));
#43122=CARTESIAN_POINT('Ctrl Pts',(-2.67879510330356,1.30000000000132,3.48487937376169));
#43123=CARTESIAN_POINT('Ctrl Pts',(-2.51547129336111,-1.30000000000188,
3.36394515997075));
#43124=CARTESIAN_POINT('Ctrl Pts',(-2.47774091682546,-1.18514270861306,
3.44130295288659));
#43125=CARTESIAN_POINT('Ctrl Pts',(-2.44568313885693,-1.06847604194576,
3.50712970190754));
#43126=CARTESIAN_POINT('Ctrl Pts',(-2.38472809610279,-0.794772684000851,
3.63256364256694));
#43127=CARTESIAN_POINT('Ctrl Pts',(-2.35825829212047,-0.636309800095197,
3.68004967653104));
#43128=CARTESIAN_POINT('Ctrl Pts',(-2.33182399965475,-0.319434907277159,
3.74960279232756));
#43129=CARTESIAN_POINT('Ctrl Pts',(-2.32904419096771,-0.158333333333332,
3.76759838532249));
#43130=CARTESIAN_POINT('Ctrl Pts',(-2.34617121467972,0.158333333333335,
3.77926048794922));
#43131=CARTESIAN_POINT('Ctrl Pts',(-2.36541685425652,0.319434907277167,
3.77235288613749));
#43132=CARTESIAN_POINT('Ctrl Pts',(-2.42808446300845,0.636309800095207,
3.72772405736545));
#43133=CARTESIAN_POINT('Ctrl Pts',(-2.47174278263682,0.79477268400084,3.69243519072899));
#43134=CARTESIAN_POINT('Ctrl Pts',(-2.57119727857627,1.06847604194556,3.59350430826072));
#43135=CARTESIAN_POINT('Ctrl Pts',(-2.62148033773407,1.18514270861267,3.54015492013262));
#43136=CARTESIAN_POINT('Ctrl Pts',(-2.67899628990966,1.30000000000132,3.47627965714654));
#43137=CARTESIAN_POINT('Ctrl Pts',(-2.51853827080824,-1.30000000000189,
3.35206487685959));
#43138=CARTESIAN_POINT('Ctrl Pts',(-2.48323413486177,-1.18514270861306,
3.42782456306498));
#43139=CARTESIAN_POINT('Ctrl Pts',(-2.45234882369544,-1.06847604194577,
3.49225791361269));
#43140=CARTESIAN_POINT('Ctrl Pts',(-2.39120594554101,-0.794772684000855,
3.61494574203019));
#43141=CARTESIAN_POINT('Ctrl Pts',(-2.3594335950636,-0.6363098000952,3.66087544146455));
#43142=CARTESIAN_POINT('Ctrl Pts',(-2.33031342459444,-0.319434907277161,
3.72943794009915));
#43143=CARTESIAN_POINT('Ctrl Pts',(-2.32730904942448,-0.158333333333333,
3.74839715610966));
#43144=CARTESIAN_POINT('Ctrl Pts',(-2.34458564073266,0.158333333333335,
3.76010251086989));
#43145=CARTESIAN_POINT('Ctrl Pts',(-2.36410755575917,0.319434907277168,
3.75214497427109));
#43146=CARTESIAN_POINT('Ctrl Pts',(-2.42996503192065,0.636309800095209,
3.70885877648818));
#43147=CARTESIAN_POINT('Ctrl Pts',(-2.47977225887544,0.794772684000846,
3.67592019371372));
#43148=CARTESIAN_POINT('Ctrl Pts',(-2.57938359964614,1.06847604194557,3.57970434673727));
#43149=CARTESIAN_POINT('Ctrl Pts',(-2.62825978626735,1.18514270861267,3.52753909508197));
#43150=CARTESIAN_POINT('Ctrl Pts',(-2.68289410105402,1.30000000000132,3.46485686677906));
#43151=CARTESIAN_POINT('Ctrl Pts',(-2.52292752087448,-1.30000000000189,
3.33458767675074));
#43152=CARTESIAN_POINT('Ctrl Pts',(-2.48950805307769,-1.18514270861306,
3.40719198419399));
#43153=CARTESIAN_POINT('Ctrl Pts',(-2.45982937263478,-1.06847604194577,
3.46919618877897));
#43154=CARTESIAN_POINT('Ctrl Pts',(-2.39990765074157,-0.794772684000851,
3.58794994712263));
#43155=CARTESIAN_POINT('Ctrl Pts',(-2.36656127553431,-0.636309800095197,
3.63356590556153));
#43156=CARTESIAN_POINT('Ctrl Pts',(-2.33639476318404,-0.319434907277158,
3.70132582143229));
#43157=CARTESIAN_POINT('Ctrl Pts',(-2.3321583303109,-0.158333333333332,
3.72107192945569));
#43158=CARTESIAN_POINT('Ctrl Pts',(-2.34950231633539,0.158333333333335,
3.73284122474502));
#43159=CARTESIAN_POINT('Ctrl Pts',(-2.37002428895053,0.319434907277167,
3.72400619726931));
#43160=CARTESIAN_POINT('Ctrl Pts',(-2.43767523089105,0.636309800095207,
3.68196761012071));
#43161=CARTESIAN_POINT('Ctrl Pts',(-2.49068724875985,0.79477268400084,3.65027347088613));
#43162=CARTESIAN_POINT('Ctrl Pts',(-2.58924608413157,1.06847604194556,3.55802851883701));
#43163=CARTESIAN_POINT('Ctrl Pts',(-2.63663527394617,1.18514270861267,3.50809174964151));
#43164=CARTESIAN_POINT('Ctrl Pts',(-2.68875118570763,1.30000000000132,3.4481476329803));
#43165=CARTESIAN_POINT('Ctrl Pts',(-2.52626319062645,-1.30000000000189,
3.31997332758331));
#43166=CARTESIAN_POINT('Ctrl Pts',(-2.49390945973534,-1.18514270861307,
3.39004411305226));
#43167=CARTESIAN_POINT('Ctrl Pts',(-2.46513663227325,-1.06847604194577,
3.45027777812963));
#43168=CARTESIAN_POINT('Ctrl Pts',(-2.40693824812987,-0.794772684000855,
3.56670387814771));
#43169=CARTESIAN_POINT('Ctrl Pts',(-2.37477597879238,-0.6363098000952,3.61364878594488));
#43170=CARTESIAN_POINT('Ctrl Pts',(-2.34450584441073,-0.31943490727716,
3.68133034339864));
#43171=CARTESIAN_POINT('Ctrl Pts',(-2.3383164193559,-0.158333333333333,
3.70105402547771));
#43172=CARTESIAN_POINT('Ctrl Pts',(-2.35514613629035,0.158333333333335,
3.71254944309585));
#43173=CARTESIAN_POINT('Ctrl Pts',(-2.37631674908184,0.319434907277168,
3.70302032704325));
#43174=CARTESIAN_POINT('Ctrl Pts',(-2.44463312595647,0.636309800095209,
3.66140384860793));
#43175=CARTESIAN_POINT('Ctrl Pts',(-2.49930521873998,0.794772684000844,
3.63002735427069));
#43176=CARTESIAN_POINT('Ctrl Pts',(-2.59662799796044,1.06847604194557,3.54034136887886));
#43177=CARTESIAN_POINT('Ctrl Pts',(-2.64282176914256,1.18514270861267,3.49197249566252));
#43178=CARTESIAN_POINT('Ctrl Pts',(-2.69308188654657,1.30000000000132,3.43405648911277));
#43179=CARTESIAN_POINT('Ctrl Pts',(-2.52947109631203,-1.3000000000019,3.30515554054755));
#43180=CARTESIAN_POINT('Ctrl Pts',(-2.4982353574683,-1.18514270861307,3.37242269051184));
#43181=CARTESIAN_POINT('Ctrl Pts',(-2.47043731159163,-1.06847604194577,
3.43068854649148));
#43182=CARTESIAN_POINT('Ctrl Pts',(-2.4141600230987,-0.794772684000854,
3.54449954004145));
#43183=CARTESIAN_POINT('Ctrl Pts',(-2.38321138359984,-0.636309800095201,
3.59271601910825));
#43184=CARTESIAN_POINT('Ctrl Pts',(-2.35338894010272,-0.319434907277161,
3.66052836665431));
#43185=CARTESIAN_POINT('Ctrl Pts',(-2.3455486272765,-0.158333333333333,
3.6804690126673));
#43186=CARTESIAN_POINT('Ctrl Pts',(-2.36312304611341,0.158333333333335,
3.69242853718606));
#43187=CARTESIAN_POINT('Ctrl Pts',(-2.38713818590456,0.319434907277169,
3.68343593736614));
#43188=CARTESIAN_POINT('Ctrl Pts',(-2.45560932304154,0.63630980009521,3.642044588671));
#43189=CARTESIAN_POINT('Ctrl Pts',(-2.50846844727388,0.794772684000845,
3.60899746335514));
#43190=CARTESIAN_POINT('Ctrl Pts',(-2.60345505149333,1.06847604194557,3.52162332902105));
#43191=CARTESIAN_POINT('Ctrl Pts',(-2.6484597732741,1.18514270861268,3.47506651058648));
#43192=CARTESIAN_POINT('Ctrl Pts',(-2.69735303546953,1.30000000000133,3.41977389893987));
#43193=CARTESIAN_POINT('Ctrl Pts',(-2.53134877776986,-1.3000000000019,3.28980202776907));
#43194=CARTESIAN_POINT('Ctrl Pts',(-2.50121228756566,-1.18514270861307,
3.35442528940338));
#43195=CARTESIAN_POINT('Ctrl Pts',(-2.47444764782297,-1.06847604194577,
3.41088093356189));
#43196=CARTESIAN_POINT('Ctrl Pts',(-2.42040562487214,-0.794772684000858,
3.52243593518531));
#43197=CARTESIAN_POINT('Ctrl Pts',(-2.39088943992526,-0.636309800095202,
3.57201352308727));
#43198=CARTESIAN_POINT('Ctrl Pts',(-2.36256753038988,-0.31943490727716,
3.64055918748032));
#43199=CARTESIAN_POINT('Ctrl Pts',(-2.35485164728609,-0.158333333333334,
3.66166760646211));
#43200=CARTESIAN_POINT('Ctrl Pts',(-2.3729430685714,0.158333333333336,3.67396851024435));
#43201=CARTESIAN_POINT('Ctrl Pts',(-2.39748268499734,0.319434907277171,
3.66427636246471));
#43202=CARTESIAN_POINT('Ctrl Pts',(-2.46523770616973,0.636309800095212,
3.62258868625159));
#43203=CARTESIAN_POINT('Ctrl Pts',(-2.51686220295093,0.794772684000845,
3.58818042239233));
#43204=CARTESIAN_POINT('Ctrl Pts',(-2.60992269931834,1.06847604194557,3.50312536915743));
#43205=CARTESIAN_POINT('Ctrl Pts',(-2.65397997707813,1.18514270861268,3.45837677647556));
#43206=CARTESIAN_POINT('Ctrl Pts',(-2.70181209195141,1.30000000000133,3.40569677205695));
#43207=CARTESIAN_POINT('Ctrl Pts',(-2.53635588003711,-1.3000000000019,3.26613435433843));
#43208=CARTESIAN_POINT('Ctrl Pts',(-2.50805836951591,-1.18514270861307,
3.3264578589723));
#43209=CARTESIAN_POINT('Ctrl Pts',(-2.48283369508773,-1.06847604194577,
3.3798771798381));
#43210=CARTESIAN_POINT('Ctrl Pts',(-2.43165851707361,-0.794772684000857,
3.48733645185484));
#43211=CARTESIAN_POINT('Ctrl Pts',(-2.40309141806982,-0.6363098000952,3.53841937537954));
#43212=CARTESIAN_POINT('Ctrl Pts',(-2.37626797477541,-0.319434907277159,
3.60766339284895));
#43213=CARTESIAN_POINT('Ctrl Pts',(-2.36878433321108,-0.158333333333333,
3.63071322404922));
#43214=CARTESIAN_POINT('Ctrl Pts',(-2.38740199596886,0.158333333333336,
3.64334586191059));
#43215=CARTESIAN_POINT('Ctrl Pts',(-2.41247548198169,0.319434907277172,
3.63220119159509));
#43216=CARTESIAN_POINT('Ctrl Pts',(-2.4793153556881,0.636309800095213,3.59017076609043));
#43217=CARTESIAN_POINT('Ctrl Pts',(-2.52996061380194,0.794772684000844,
3.55424616566083));
#43218=CARTESIAN_POINT('Ctrl Pts',(-2.61989032360897,1.06847604194557,3.47305078123809));
#43219=CARTESIAN_POINT('Ctrl Pts',(-2.66218344562222,1.18514270861267,3.4311513215582));
#43220=CARTESIAN_POINT('Ctrl Pts',(-2.70784245049735,1.30000000000132,3.38249887552958));
#43221=CARTESIAN_POINT('Ctrl Pts',(-2.54098117524275,-1.30000000000194,
3.23262551129656));
#43222=CARTESIAN_POINT('Ctrl Pts',(-2.5137239795217,-1.18514270861311,3.2864637443441));
#43223=CARTESIAN_POINT('Ctrl Pts',(-2.48977880870604,-1.0684760419458,3.3353958627565));
#43224=CARTESIAN_POINT('Ctrl Pts',(-2.44211211400679,-0.79477268400088,
3.43710473885357));
#43225=CARTESIAN_POINT('Ctrl Pts',(-2.41706898213178,-0.636309800095219,
3.4911932805752));
#43226=CARTESIAN_POINT('Ctrl Pts',(-2.39356025850244,-0.319434907277169,
3.56193348901071));
#43227=CARTESIAN_POINT('Ctrl Pts',(-2.38679878295003,-0.158333333333338,
3.58777302468684));
#43228=CARTESIAN_POINT('Ctrl Pts',(-2.40650274675603,0.15833333333334,3.60107340307502));
#43229=CARTESIAN_POINT('Ctrl Pts',(-2.43222643859139,0.31943490727718,3.58806460049873));
#43230=CARTESIAN_POINT('Ctrl Pts',(-2.49738160405796,0.63630980009523,3.54537293881767));
#43231=CARTESIAN_POINT('Ctrl Pts',(-2.5454550115792,0.794772684000866,3.50665907806544));
#43232=CARTESIAN_POINT('Ctrl Pts',(-2.63149657495587,1.0684760419456,3.43086506796219));
#43233=CARTESIAN_POINT('Ctrl Pts',(-2.67191622125882,1.18514270861271,3.39310031169925));
#43234=CARTESIAN_POINT('Ctrl Pts',(-2.71551130923304,1.30000000000137,3.35037921770225));
#43235=CARTESIAN_POINT('Ctrl Pts',(-2.54607194775883,-1.30000000000194,
3.19608939128788));
#43236=CARTESIAN_POINT('Ctrl Pts',(-2.52146571190023,-1.18514270861311,
3.24347357409477));
#43237=CARTESIAN_POINT('Ctrl Pts',(-2.49960544585642,-1.06847604194581,
3.28775993886287));
#43238=CARTESIAN_POINT('Ctrl Pts',(-2.45544759776561,-0.794772684000886,
3.38291372154783));
#43239=CARTESIAN_POINT('Ctrl Pts',(-2.430480323573,-0.636309800095224,3.43848528660745));
#43240=CARTESIAN_POINT('Ctrl Pts',(-2.40891442716951,-0.319434907277172,
3.50999985813467));
#43241=CARTESIAN_POINT('Ctrl Pts',(-2.40350022809356,-0.158333333333339,
3.53915059384038));
#43242=CARTESIAN_POINT('Ctrl Pts',(-2.42416152391693,0.158333333333341,
3.55297228552503));
#43243=CARTESIAN_POINT('Ctrl Pts',(-2.44991916944357,0.319434907277179,
3.53741124744924));
#43244=CARTESIAN_POINT('Ctrl Pts',(-2.51421807406285,0.636309800095232,
3.49452302187417));
#43245=CARTESIAN_POINT('Ctrl Pts',(-2.56169302483603,0.794772684000873,
3.45408481116691));
#43246=CARTESIAN_POINT('Ctrl Pts',(-2.64468685271695,1.06847604194561,3.38495701231189));
#43247=CARTESIAN_POINT('Ctrl Pts',(-2.68331682422934,1.18514270861272,3.35190032778415));
#43248=CARTESIAN_POINT('Ctrl Pts',(-2.72465181438882,1.30000000000137,3.31570982141567));
#43249=CARTESIAN_POINT('Ctrl Pts',(-2.54893825527318,-1.30000000000195,
3.1715295558725));
#43250=CARTESIAN_POINT('Ctrl Pts',(-2.52456767240702,-1.18514270861312,
3.2139499308541));
#43251=CARTESIAN_POINT('Ctrl Pts',(-2.50318298479296,-1.06847604194582,
3.25474400510964));
#43252=CARTESIAN_POINT('Ctrl Pts',(-2.46067809377112,-0.794772684000895,
3.34522939744867));
#43253=CARTESIAN_POINT('Ctrl Pts',(-2.43785098142268,-0.636309800095231,
3.40270562498112));
#43254=CARTESIAN_POINT('Ctrl Pts',(-2.41819118871568,-0.319434907277175,
3.47496318623089));
#43255=CARTESIAN_POINT('Ctrl Pts',(-2.41324425637799,-0.158333333333341,
3.50605275406172));
#43256=CARTESIAN_POINT('Ctrl Pts',(-2.43459928047454,0.158333333333343,
3.52024485921037));
#43257=CARTESIAN_POINT('Ctrl Pts',(-2.46065104029608,0.319434907277184,
3.50319259994508));
#43258=CARTESIAN_POINT('Ctrl Pts',(-2.52431911196031,0.63630980009524,3.46015864451169));
#43259=CARTESIAN_POINT('Ctrl Pts',(-2.57105352724188,0.794772684000883,
3.41837301501752));
#43260=CARTESIAN_POINT('Ctrl Pts',(-2.65183111157973,1.06847604194562,3.35356418715493));
#43261=CARTESIAN_POINT('Ctrl Pts',(-2.68921977408514,1.18514270861273,3.32360433739698));
#43262=CARTESIAN_POINT('Ctrl Pts',(-2.72903147594052,1.30000000000138,3.29173797805909));
#43263=CARTESIAN_POINT('Ctrl Pts',(-2.55043866196968,-1.30000000000196,
3.15283126618602));
#43264=CARTESIAN_POINT('Ctrl Pts',(-2.52735906897743,-1.18514270861313,
3.19201784177817));
#43265=CARTESIAN_POINT('Ctrl Pts',(-2.50701882331754,-1.06847604194582,
3.23049388197808));
#43266=CARTESIAN_POINT('Ctrl Pts',(-2.46635722713344,-0.794772684000895,
3.31773975304688));
#43267=CARTESIAN_POINT('Ctrl Pts',(-2.44399336583575,-0.636309800095233,
3.37614613933208));
#43268=CARTESIAN_POINT('Ctrl Pts',(-2.42503654909892,-0.319434907277177,
3.44862255465249));
#43269=CARTESIAN_POINT('Ctrl Pts',(-2.41986793208942,-0.158333333333341,
3.48088506283785));
#43270=CARTESIAN_POINT('Ctrl Pts',(-2.44157186869421,0.158333333333343,
3.49526279903694));
#43271=CARTESIAN_POINT('Ctrl Pts',(-2.46817051309274,0.319434907277183,
3.47722483799343));
#43272=CARTESIAN_POINT('Ctrl Pts',(-2.53189461930863,0.636309800095241,
3.43434687115883));
#43273=CARTESIAN_POINT('Ctrl Pts',(-2.57870590041425,0.794772684000886,
3.39189384649464));
#43274=CARTESIAN_POINT('Ctrl Pts',(-2.65818528340837,1.06847604194562,3.33052500181169));
#43275=CARTESIAN_POINT('Ctrl Pts',(-2.69470560532199,1.18514270861274,3.30292603445292));
#43276=CARTESIAN_POINT('Ctrl Pts',(-2.73334256925239,1.30000000000139,3.27429239865887));
#43277=CARTESIAN_POINT('Ctrl Pts',(-2.55358415559061,-1.30000000000197,
3.12519350169584));
#43278=CARTESIAN_POINT('Ctrl Pts',(-2.53103602156771,-1.18514270861314,
3.15892145377589));
#43279=CARTESIAN_POINT('Ctrl Pts',(-2.51131793932318,-1.06847604194584,
3.19350862461068));
#43280=CARTESIAN_POINT('Ctrl Pts',(-2.4723032105075,-0.794772684000908,
3.27539687558823));
#43281=CARTESIAN_POINT('Ctrl Pts',(-2.45134421773899,-0.636309800095241,
3.33546738470793));
#43282=CARTESIAN_POINT('Ctrl Pts',(-2.43421476586456,-0.319434907277181,
3.40861739061838));
#43283=CARTESIAN_POINT('Ctrl Pts',(-2.43012713057062,-0.158333333333343,
3.44332102563396));
#43284=CARTESIAN_POINT('Ctrl Pts',(-2.45236775886849,0.158333333333345,
3.45797138395048));
#43285=CARTESIAN_POINT('Ctrl Pts',(-2.47853889838145,0.319434907277189,
3.43785084550915));
#43286=CARTESIAN_POINT('Ctrl Pts',(-2.54129095915557,0.63630980009525,3.39467957195464));
#43287=CARTESIAN_POINT('Ctrl Pts',(-2.58736634141913,0.794772684000896,
3.35079547747347));
#43288=CARTESIAN_POINT('Ctrl Pts',(-2.66489054887304,1.06847604194564,3.29456729103865));
#43289=CARTESIAN_POINT('Ctrl Pts',(-2.70037289791079,1.18514270861275,3.27063264666337));
#43290=CARTESIAN_POINT('Ctrl Pts',(-2.73778023913444,1.30000000000141,3.24710245636084));
#43291=CARTESIAN_POINT('Ctrl Pts',(-2.55593709808298,-1.30000000000202,
3.08759717673342));
#43292=CARTESIAN_POINT('Ctrl Pts',(-2.53449134505796,-1.18514270861318,
3.11424537955628));
#43293=CARTESIAN_POINT('Ctrl Pts',(-2.51587115807294,-1.06847604194588,
3.14377869822358));
#43294=CARTESIAN_POINT('Ctrl Pts',(-2.47938242398696,-0.794772684000935,
3.21867176723112));
#43295=CARTESIAN_POINT('Ctrl Pts',(-2.46021519347327,-0.636309800095264,
3.28089625856297));
#43296=CARTESIAN_POINT('Ctrl Pts',(-2.44514895149305,-0.319434907277192,
3.35472334103413));
#43297=CARTESIAN_POINT('Ctrl Pts',(-2.44164372936051,-0.158333333333349,
3.39222589801146));
#43298=CARTESIAN_POINT('Ctrl Pts',(-2.46468090308572,0.158333333333351,
3.40726305730602));
#43299=CARTESIAN_POINT('Ctrl Pts',(-2.49106278789201,0.319434907277199,
3.38476509205472));
#43300=CARTESIAN_POINT('Ctrl Pts',(-2.55338104347357,0.636309800095272,
3.34163395814732));
#43301=CARTESIAN_POINT('Ctrl Pts',(-2.59898610889037,0.794772684000924,
3.29609989894042));
#43302=CARTESIAN_POINT('Ctrl Pts',(-2.67459867825352,1.06847604194568,3.24706841498202));
#43303=CARTESIAN_POINT('Ctrl Pts',(-2.70896671379464,1.18514270861279,3.22815047231979));
#43304=CARTESIAN_POINT('Ctrl Pts',(-2.74497290532134,1.30000000000146,3.21153849960543));
#43305=CARTESIAN_POINT('Ctrl Pts',(-2.55909406402193,-1.30000000000205,
3.04400046157339));
#43306=CARTESIAN_POINT('Ctrl Pts',(-2.5382866672259,-1.18514270861321,3.06214142930381));
#43307=CARTESIAN_POINT('Ctrl Pts',(-2.52034870426,-1.0684760419459,3.08553727610246));
#43308=CARTESIAN_POINT('Ctrl Pts',(-2.48553738750759,-0.794772684000951,
3.15172618441284));
#43309=CARTESIAN_POINT('Ctrl Pts',(-2.46731670249777,-0.636309800095274,
3.2159249062016));
#43310=CARTESIAN_POINT('Ctrl Pts',(-2.45457240355061,-0.319434907277196,
3.29045296825996));
#43311=CARTESIAN_POINT('Ctrl Pts',(-2.45309797862502,-0.158333333333352,
3.33175999081764));
#43312=CARTESIAN_POINT('Ctrl Pts',(-2.4775003642474,0.158333333333354,3.34740226567864));
#43313=CARTESIAN_POINT('Ctrl Pts',(-2.50375051020395,0.319434907277208,
3.32197121857406));
#43314=CARTESIAN_POINT('Ctrl Pts',(-2.56544025428757,0.636309800095285,
3.27882931284725));
#43315=CARTESIAN_POINT('Ctrl Pts',(-2.61047096591202,0.794772684000935,
3.23138292291287));
#43316=CARTESIAN_POINT('Ctrl Pts',(-2.68375360165742,1.06847604194569,3.19067109065635));
#43317=CARTESIAN_POINT('Ctrl Pts',(-2.71677357684178,1.18514270861281,3.17755924429881));
#43318=CARTESIAN_POINT('Ctrl Pts',(-2.75109218958555,1.30000000000148,3.16895819524558));
#43319=CARTESIAN_POINT('Ctrl Pts',(-2.55969404135944,-1.30000000000211,
3.01222601946097));
#43320=CARTESIAN_POINT('Ctrl Pts',(-2.53876245937103,-1.18514270861326,
3.02409177121432));
#43321=CARTESIAN_POINT('Ctrl Pts',(-2.52106667650709,-1.06847604194595,
3.043027194833));
#43322=CARTESIAN_POINT('Ctrl Pts',(-2.48766122135914,-0.794772684000989,
3.10310416770247));
#43323=CARTESIAN_POINT('Ctrl Pts',(-2.47212874699672,-0.636309800095306,
3.16950845560562));
#43324=CARTESIAN_POINT('Ctrl Pts',(-2.46094251411636,-0.319434907277213,
3.24444466879074));
#43325=CARTESIAN_POINT('Ctrl Pts',(-2.4590317912922,-0.158333333333359,
3.28762636471884));
#43326=CARTESIAN_POINT('Ctrl Pts',(-2.48383371179482,0.158333333333362,
3.30343883720611));
#43327=CARTESIAN_POINT('Ctrl Pts',(-2.51066893582012,0.319434907277222,
3.27622966764146));
#43328=CARTESIAN_POINT('Ctrl Pts',(-2.57212520691001,0.636309800095316,
3.2331763041556));
#43329=CARTESIAN_POINT('Ctrl Pts',(-2.61640131477568,0.794772684000977,
3.18420338560199));
#43330=CARTESIAN_POINT('Ctrl Pts',(-2.68867278939858,1.06847604194574,3.14971672375969));
#43331=CARTESIAN_POINT('Ctrl Pts',(-2.72120196670161,1.18514270861287,3.14095830281351));
#43332=CARTESIAN_POINT('Ctrl Pts',(-2.75497667786541,1.30000000000154,3.13836945897594));
#43333=CARTESIAN_POINT('Ctrl Pts',(-2.56116907507594,-1.30000000000213,
2.98723486350912));
#43334=CARTESIAN_POINT('Ctrl Pts',(-2.54075722636678,-1.18514270861329,
2.99432776760199));
#43335=CARTESIAN_POINT('Ctrl Pts',(-2.52343611256515,-1.06847604194597,
3.00976701257515));
#43336=CARTESIAN_POINT('Ctrl Pts',(-2.49056109054234,-0.794772684001007,
3.06471647418665));
#43337=CARTESIAN_POINT('Ctrl Pts',(-2.47447675889149,-0.636309800095319,
3.13180258532495));
#43338=CARTESIAN_POINT('Ctrl Pts',(-2.46408895434673,-0.319434907277219,
3.20688977378303));
#43339=CARTESIAN_POINT('Ctrl Pts',(-2.46347706359624,-0.158333333333363,
3.25223928787584));
#43340=CARTESIAN_POINT('Ctrl Pts',(-2.48922823124499,0.158333333333365,
3.26843939953327));
#43341=CARTESIAN_POINT('Ctrl Pts',(-2.51624885866665,0.31943490727723,3.23967905792092));
#43342=CARTESIAN_POINT('Ctrl Pts',(-2.5777505168142,0.63630980009533,3.19679784157907));
#43343=CARTESIAN_POINT('Ctrl Pts',(-2.62193161309762,0.794772684000992,
3.14684768294999));
#43344=CARTESIAN_POINT('Ctrl Pts',(-2.6932852563524,1.06847604194577,3.11728699184811));
#43345=CARTESIAN_POINT('Ctrl Pts',(-2.72522894628803,1.1851427086129,3.11191854353062));
#43346=CARTESIAN_POINT('Ctrl Pts',(-2.7582299779073,1.30000000000157,3.11397737474212));
#43347=CARTESIAN_POINT('Ctrl Pts',(-2.56104903447691,-1.30000000000216,
2.97280661034047));
#43348=CARTESIAN_POINT('Ctrl Pts',(-2.54061337483588,-1.18514270861331,
2.97710536479362));
#43349=CARTESIAN_POINT('Ctrl Pts',(-2.52338049166604,-1.06847604194599,
2.99053937526616));
#43350=CARTESIAN_POINT('Ctrl Pts',(-2.49096813847904,-0.794772684001021,
3.04267889582866));
#43351=CARTESIAN_POINT('Ctrl Pts',(-2.47557323327233,-0.636309800095332,
3.11052944246156));
#43352=CARTESIAN_POINT('Ctrl Pts',(-2.46599547637307,-0.319434907277227,
3.18583494016677));
#43353=CARTESIAN_POINT('Ctrl Pts',(-2.4659166650027,-0.158333333333366,
3.23232159152127));
#43354=CARTESIAN_POINT('Ctrl Pts',(-2.49195600008211,0.158333333333368,
3.24863192396712));
#43355=CARTESIAN_POINT('Ctrl Pts',(-2.5187862531373,0.319434907277236,3.21887732256778));
#43356=CARTESIAN_POINT('Ctrl Pts',(-2.57995375081713,0.636309800095343,
3.1759357894701));
#43357=CARTESIAN_POINT('Ctrl Pts',(-2.62365207930783,0.79477268400101,3.12524345459197));
#43358=CARTESIAN_POINT('Ctrl Pts',(-2.69472279222533,1.06847604194579,3.09855134679839));
#43359=CARTESIAN_POINT('Ctrl Pts',(-2.72660847127242,1.18514270861292,3.09520649332736));
#43360=CARTESIAN_POINT('Ctrl Pts',(-2.759615951174,1.30000000000159,3.1000708108091));
#43361=CARTESIAN_POINT('Ctrl Pts',(-2.56127831437987,-1.30000000000217,
2.96331663785848));
#43362=CARTESIAN_POINT('Ctrl Pts',(-2.54088772104557,-1.18514270861332,
2.96577295199612));
#43363=CARTESIAN_POINT('Ctrl Pts',(-2.52372474541954,-1.06847604194599,
2.97787241373934));
#43364=CARTESIAN_POINT('Ctrl Pts',(-2.49153128087079,-0.794772684001023,
3.02810219092903));
#43365=CARTESIAN_POINT('Ctrl Pts',(-2.47626833169421,-0.636309800095335,
3.09633903590505));
#43366=CARTESIAN_POINT('Ctrl Pts',(-2.46717038202176,-0.319434907277228,
3.17176849844764));
#43367=CARTESIAN_POINT('Ctrl Pts',(-2.46767312849726,-0.158333333333367,
3.21910192517114));
#43368=CARTESIAN_POINT('Ctrl Pts',(-2.49392386739101,0.158333333333369,
3.23549299195286));
#43369=CARTESIAN_POINT('Ctrl Pts',(-2.52048923570689,0.319434907277237,
3.20501930950502));
#43370=CARTESIAN_POINT('Ctrl Pts',(-2.58139311453956,0.636309800095345,
3.1620226074916));
#43371=CARTESIAN_POINT('Ctrl Pts',(-2.62481842336647,0.794772684001014,
3.1108597619245));
#43372=CARTESIAN_POINT('Ctrl Pts',(-2.69570834867789,1.06847604194579,3.08608229682891));
#43373=CARTESIAN_POINT('Ctrl Pts',(-2.72755502603203,1.18514270861292,3.08408474375722));
#43374=CARTESIAN_POINT('Ctrl Pts',(-2.76056275880354,1.3000000000016,3.09081488415818));
#43375=CARTESIAN_POINT('Ctrl Pts',(-2.56135590679036,-1.30000000000217,
2.95696190589203));
#43376=CARTESIAN_POINT('Ctrl Pts',(-2.54098096164571,-1.18514270861332,
2.958186745425));
#43377=CARTESIAN_POINT('Ctrl Pts',(-2.5238612674274,-1.068476041946,2.96939659408028));
#43378=CARTESIAN_POINT('Ctrl Pts',(-2.4918316298507,-0.794772684001025,
3.01836095556312));
#43379=CARTESIAN_POINT('Ctrl Pts',(-2.47673724160775,-0.636309800095336,
3.08688334195185));
#43380=CARTESIAN_POINT('Ctrl Pts',(-2.46795275175855,-0.319434907277229,
3.16239073869001));
#43381=CARTESIAN_POINT('Ctrl Pts',(-2.46873478549739,-0.158333333333367,
3.21024437564977));
#43382=CARTESIAN_POINT('Ctrl Pts',(-2.49514977379312,0.158333333333369,
3.2266994418965));
#43383=CARTESIAN_POINT('Ctrl Pts',(-2.52165728592964,0.319434907277237,
3.19579667183401));
#43384=CARTESIAN_POINT('Ctrl Pts',(-2.58246579417548,0.636309800095345,
3.15279715001001));
#43385=CARTESIAN_POINT('Ctrl Pts',(-2.62574992097367,0.794772684001014,
3.10133790237474));
#43386=CARTESIAN_POINT('Ctrl Pts',(-2.69649403174895,1.0684760419458,3.07782558277605));
#43387=CARTESIAN_POINT('Ctrl Pts',(-2.72828231736828,1.18514270861293,3.07671215017822));
#43388=CARTESIAN_POINT('Ctrl Pts',(-2.76123638437994,1.3000000000016,3.08466289691952));
#43389=CARTESIAN_POINT('Ctrl Pts',(-2.56131487123015,-1.30000000000217,
2.94897114298167));
#43390=CARTESIAN_POINT('Ctrl Pts',(-2.54081396862634,-1.18514270861332,
2.94860460594914));
#43391=CARTESIAN_POINT('Ctrl Pts',(-2.52367827482182,-1.068476041946,2.95867756677743));
#43392=CARTESIAN_POINT('Ctrl Pts',(-2.49186569968375,-0.794772684001026,
3.00606544985243));
#43393=CARTESIAN_POINT('Ctrl Pts',(-2.47737488468038,-0.636309800095337,
3.07508978567909));
#43394=CARTESIAN_POINT('Ctrl Pts',(-2.46900076333603,-0.319434907277229,
3.15069628767783));
#43395=CARTESIAN_POINT('Ctrl Pts',(-2.4697992228176,-0.158333333333367,
3.19906700330485));
#43396=CARTESIAN_POINT('Ctrl Pts',(-2.49641269429515,0.15833333333337,3.21559961047872));
#43397=CARTESIAN_POINT('Ctrl Pts',(-2.52305451573685,0.319434907277238,
3.18424456747001));
#43398=CARTESIAN_POINT('Ctrl Pts',(-2.58395421093877,0.636309800095347,
3.14132982636881));
#43399=CARTESIAN_POINT('Ctrl Pts',(-2.62729716662013,0.794772684001016,
3.0896021960587));
#43400=CARTESIAN_POINT('Ctrl Pts',(-2.69782820934637,1.0684760419458,3.06765706675948));
#43401=CARTESIAN_POINT('Ctrl Pts',(-2.72945689966399,1.18514270861293,3.06761092476609));
#43402=CARTESIAN_POINT('Ctrl Pts',(-2.76218400533566,1.3000000000016,3.07701787410579));
#43403=CARTESIAN_POINT('Ctrl Pts',(-2.56121597939136,-1.30000000000218,
2.94175952744392));
#43404=CARTESIAN_POINT('Ctrl Pts',(-2.5405367478716,-1.18514270861333,2.93993767742452));
#43405=CARTESIAN_POINT('Ctrl Pts',(-2.52334870506496,-1.06847604194601,
2.94897403450116));
#43406=CARTESIAN_POINT('Ctrl Pts',(-2.49170623206277,-0.794772684001033,
2.9949344576338));
#43407=CARTESIAN_POINT('Ctrl Pts',(-2.4778709967323,-0.636309800095342,
3.06445299246228));
#43408=CARTESIAN_POINT('Ctrl Pts',(-2.46986253282946,-0.319434907277232,
3.14014390285027));
#43409=CARTESIAN_POINT('Ctrl Pts',(-2.47058571822193,-0.158333333333368,
3.18894004954346));
#43410=CARTESIAN_POINT('Ctrl Pts',(-2.49736140057388,0.158333333333371,
3.20553401239655));
#43411=CARTESIAN_POINT('Ctrl Pts',(-2.52415581516235,0.31943490727724,3.17378572875201));
#43412=CARTESIAN_POINT('Ctrl Pts',(-2.5851931833126,0.636309800095352,3.13097096387433));
#43413=CARTESIAN_POINT('Ctrl Pts',(-2.62865750910726,0.794772684001022,
3.07903191620791));
#43414=CARTESIAN_POINT('Ctrl Pts',(-2.69903491426331,1.06847604194581,3.05851252393744));
#43415=CARTESIAN_POINT('Ctrl Pts',(-2.73052608489709,1.18514270861294,3.05942872360747));
#43416=CARTESIAN_POINT('Ctrl Pts',(-2.76304465521239,1.30000000000161,3.07014320754303));
#43417=CARTESIAN_POINT('Ctrl Pts',(-2.56122885626145,-1.30000000000218,
2.93698156749451));
#43418=CARTESIAN_POINT('Ctrl Pts',(-2.54051001622556,-1.18514270861333,
2.93421867273334));
#43419=CARTESIAN_POINT('Ctrl Pts',(-2.52331921064371,-1.06847604194601,
2.94257575738084));
#43420=CARTESIAN_POINT('Ctrl Pts',(-2.49175547611056,-0.794772684001034,
2.9875716717238));
#43421=CARTESIAN_POINT('Ctrl Pts',(-2.47808947499982,-0.636309800095343,
3.057320333101));
#43422=CARTESIAN_POINT('Ctrl Pts',(-2.47029675512753,-0.319434907277232,
3.13305829083749));
#43423=CARTESIAN_POINT('Ctrl Pts',(-2.47118148600144,-0.158333333333369,
3.18221951764537));
#43424=CARTESIAN_POINT('Ctrl Pts',(-2.49806846737449,0.158333333333371,
3.19885423538708));
#43425=CARTESIAN_POINT('Ctrl Pts',(-2.52483193154344,0.319434907277241,
3.16679107533292));
#43426=CARTESIAN_POINT('Ctrl Pts',(-2.58584095910954,0.636309800095353,
3.12399303132165));
#43427=CARTESIAN_POINT('Ctrl Pts',(-2.62924834691998,0.794772684001023,
3.07185364297797));
#43428=CARTESIAN_POINT('Ctrl Pts',(-2.69957568789046,1.06847604194581,3.05230697577233));
#43429=CARTESIAN_POINT('Ctrl Pts',(-2.73104801847194,1.18514270861294,3.05389572675833));
#43430=CARTESIAN_POINT('Ctrl Pts',(-2.76355057961355,1.30000000000162,3.06553425668826));
#43431=CARTESIAN_POINT('Ctrl Pts',(-2.56124558852298,-1.30000000000218,
2.93459651930118));
#43432=CARTESIAN_POINT('Ctrl Pts',(-2.54051875074545,-1.18514270861333,
2.93136751692711));
#43433=CARTESIAN_POINT('Ctrl Pts',(-2.52333126833281,-1.06847604194601,
2.93938673770933));
#43434=CARTESIAN_POINT('Ctrl Pts',(-2.49180136455417,-0.794772684001035,
2.98389838764611));
#43435=CARTESIAN_POINT('Ctrl Pts',(-2.4781799529861,-0.636309800095344,
3.05374721821014));
#43436=CARTESIAN_POINT('Ctrl Pts',(-2.47048954832231,-0.319434907277232,
3.12950674724737));
#43437=CARTESIAN_POINT('Ctrl Pts',(-2.47148414771184,-0.158333333333369,
3.17886164663329));
#43438=CARTESIAN_POINT('Ctrl Pts',(-2.49842744874293,0.158333333333371,
3.19551677007893));
#43439=CARTESIAN_POINT('Ctrl Pts',(-2.52515869307151,0.319434907277241,
3.16328952071116));
#43440=CARTESIAN_POINT('Ctrl Pts',(-2.58613667884508,0.636309800095353,
3.12049277631889));
#43441=CARTESIAN_POINT('Ctrl Pts',(-2.62949397568524,0.794772684001024,
3.06824394144028));
#43442=CARTESIAN_POINT('Ctrl Pts',(-2.69980382558699,1.06847604194581,3.04918675646232));
#43443=CARTESIAN_POINT('Ctrl Pts',(-2.73127752759753,1.18514270861294,3.05111631983744));
#43444=CARTESIAN_POINT('Ctrl Pts',(-2.76379040283277,1.30000000000162,3.06322459582634));
#43445=CARTESIAN_POINT('Ctrl Pts',(-2.56126911392072,-1.30000000000218,
2.93261264944325));
#43446=CARTESIAN_POINT('Ctrl Pts',(-2.5405458456593,-1.18514270861333,2.92899904773324));
#43447=CARTESIAN_POINT('Ctrl Pts',(-2.52336522141286,-1.06847604194601,
2.93673825224489));
#43448=CARTESIAN_POINT('Ctrl Pts',(-2.49185875880972,-0.794772684001035,
2.98084461638238));
#43449=CARTESIAN_POINT('Ctrl Pts',(-2.47823984512274,-0.636309800095344,
3.050764003082));
#43450=CARTESIAN_POINT('Ctrl Pts',(-2.47063003330241,-0.319434907277232,
3.12653989178922));
#43451=CARTESIAN_POINT('Ctrl Pts',(-2.47174166797301,-0.158333333333369,
3.17606598907416));
#43452=CARTESIAN_POINT('Ctrl Pts',(-2.49873241433156,0.158333333333371,
3.19273812989693));
#43453=CARTESIAN_POINT('Ctrl Pts',(-2.52542186010774,0.319434907277241,
3.1603681777678));
#43454=CARTESIAN_POINT('Ctrl Pts',(-2.5863592866705,0.636309800095354,3.11756635750561));
#43455=CARTESIAN_POINT('Ctrl Pts',(-2.62965670193438,0.794772684001024,
3.06521852198832));
#43456=CARTESIAN_POINT('Ctrl Pts',(-2.69995809385392,1.06847604194581,3.04657175301279));
#43457=CARTESIAN_POINT('Ctrl Pts',(-2.73144190887693,1.18514270861294,3.04878909121335));
#43458=CARTESIAN_POINT('Ctrl Pts',(-2.76397867128422,1.30000000000162,3.06129526297312));
#43459=CARTESIAN_POINT('Ctrl Pts',(-2.5612881662613,-1.30000000000218,2.93122497760151));
#43460=CARTESIAN_POINT('Ctrl Pts',(-2.54057050258479,-1.18514270861333,
2.92734335101429));
#43461=CARTESIAN_POINT('Ctrl Pts',(-2.52339581008036,-1.06847604194601,
2.93488699092271));
#43462=CARTESIAN_POINT('Ctrl Pts',(-2.49190380678617,-0.794772684001035,
2.97870895943272));
#43463=CARTESIAN_POINT('Ctrl Pts',(-2.47827575857435,-0.636309800095344,
3.04867365985667));
#43464=CARTESIAN_POINT('Ctrl Pts',(-2.47071941768915,-0.319434907277232,
3.12445989077146));
#43465=CARTESIAN_POINT('Ctrl Pts',(-2.47191831288654,-0.158333333333369,
3.17410783091974));
#43466=CARTESIAN_POINT('Ctrl Pts',(-2.49894254244825,0.158333333333371,
3.19079190973));
#43467=CARTESIAN_POINT('Ctrl Pts',(-2.52560116743548,0.319434907277241,
3.15832142852038));
#43468=CARTESIAN_POINT('Ctrl Pts',(-2.58650656512886,0.636309800095354,
3.11551448505154));
#43469=CARTESIAN_POINT('Ctrl Pts',(-2.62975530020764,0.794772684001024,
3.06309450093283));
#43470=CARTESIAN_POINT('Ctrl Pts',(-2.70005209913077,1.06847604194581,3.04473548722388));
#43471=CARTESIAN_POINT('Ctrl Pts',(-2.73154553314448,1.18514270861294,3.04715527914781));
#43472=CARTESIAN_POINT('Ctrl Pts',(-2.76410352167112,1.30000000000162,3.05994179976178));
#43473=CARTESIAN_POINT('Ctrl Pts',(-2.56129985436376,-1.30000000000218,
2.93043234734907));
#43474=CARTESIAN_POINT('Ctrl Pts',(-2.54058590945191,-1.18514270861333,
2.92639775725202));
#43475=CARTESIAN_POINT('Ctrl Pts',(-2.52341477430191,-1.06847604194601,
2.93382970795896));
#43476=CARTESIAN_POINT('Ctrl Pts',(-2.49193061631822,-0.794772684001036,
2.97748900397935));
#43477=CARTESIAN_POINT('Ctrl Pts',(-2.47829498062337,-0.636309800095344,
3.04747869460039));
#43478=CARTESIAN_POINT('Ctrl Pts',(-2.47076939216646,-0.319434907277233,
3.12327092089488));
#43479=CARTESIAN_POINT('Ctrl Pts',(-2.47202102417737,-0.158333333333369,
3.17298960622546));
#43480=CARTESIAN_POINT('Ctrl Pts',(-2.49906424625836,0.158333333333371,
3.18968044522044));
#43481=CARTESIAN_POINT('Ctrl Pts',(-2.52570272600367,0.319434907277241,
3.1571515288977));
#43482=CARTESIAN_POINT('Ctrl Pts',(-2.58658835737259,0.636309800095354,
3.11434105534365));
#43483=CARTESIAN_POINT('Ctrl Pts',(-2.62980856665228,0.794772684001024,
3.06187948966555));
#43484=CARTESIAN_POINT('Ctrl Pts',(-2.70010357285852,1.06847604194581,3.04368526313072));
#43485=CARTESIAN_POINT('Ctrl Pts',(-2.73160332904789,1.18514270861294,3.04622110339926));
#43486=CARTESIAN_POINT('Ctrl Pts',(-2.76417473792659,1.30000000000162,3.05916839044075));
#43487=CARTESIAN_POINT('Ctrl Pts',(-2.56149026715371,-1.30000000000216,
2.91735327145688));
#43488=CARTESIAN_POINT('Ctrl Pts',(-2.54084897406474,-1.18514270861331,
2.91079953441578));
#43489=CARTESIAN_POINT('Ctrl Pts',(-2.52374038681034,-1.06847604194599,
2.91639044658124));
#43490=CARTESIAN_POINT('Ctrl Pts',(-2.49237738488491,-0.794772684001022,
2.95736314133742));
#43491=CARTESIAN_POINT('Ctrl Pts',(-2.47858976511407,-0.636309800095333,
3.0277554918797));
#43492=CARTESIAN_POINT('Ctrl Pts',(-2.47153047171005,-0.319434907277227,
3.10363055568692));
#43493=CARTESIAN_POINT('Ctrl Pts',(-2.47359874066084,-0.158333333333366,
3.15449480879278));
#43494=CARTESIAN_POINT('Ctrl Pts',(-2.50096233759851,0.158333333333368,
3.17129923809903));
#43495=CARTESIAN_POINT('Ctrl Pts',(-2.52734748101025,0.319434907277235,
3.13783675396691));
#43496=CARTESIAN_POINT('Ctrl Pts',(-2.5879245755808,0.636309800095342,3.09497436480464));
#43497=CARTESIAN_POINT('Ctrl Pts',(-2.63063176748115,0.794772684001011,
3.04181088542121));
#43498=CARTESIAN_POINT('Ctrl Pts',(-2.70087971632417,1.06847604194579,3.02632671178359));
#43499=CARTESIAN_POINT('Ctrl Pts',(-2.73247885494392,1.18514270861292,3.03077395956638));
#43500=CARTESIAN_POINT('Ctrl Pts',(-2.76526939807227,1.30000000000159,3.04637098015453));
#43501=CARTESIAN_POINT('Ctrl Pts',(-2.56087008524915,-1.30000000000202,
2.89145016916653));
#43502=CARTESIAN_POINT('Ctrl Pts',(-2.53960255952203,-1.18514270861318,
2.87970907731183));
#43503=CARTESIAN_POINT('Ctrl Pts',(-2.52223142494676,-1.06847604194587,
2.88157206655941));
#43504=CARTESIAN_POINT('Ctrl Pts',(-2.49110207202559,-0.794772684000928,
2.91730409324431));
#43505=CARTESIAN_POINT('Ctrl Pts',(-2.4787850160475,-0.636309800095263,
2.9891211391137));
#43506=CARTESIAN_POINT('Ctrl Pts',(-2.47303673739557,-0.319434907277193,
3.06528465111095));
#43507=CARTESIAN_POINT('Ctrl Pts',(-2.4758155227965,-0.158333333333348,
3.11803020288129));
#43508=CARTESIAN_POINT('Ctrl Pts',(-2.50383353435718,0.158333333333351,
3.13506318529158));
#43509=CARTESIAN_POINT('Ctrl Pts',(-2.52987163915752,0.319434907277197,
3.09984011298672));
#43510=CARTESIAN_POINT('Ctrl Pts',(-2.59106333172505,0.63630980009527,3.05737448948734));
#43511=CARTESIAN_POINT('Ctrl Pts',(-2.63544492476371,0.794772684000922,
3.00395850467053));
#43512=CARTESIAN_POINT('Ctrl Pts',(-2.70502550336271,1.06847604194568,2.99349161372486));
#43513=CARTESIAN_POINT('Ctrl Pts',(-2.73580288446904,1.18514270861279,3.00122553922847));
#43514=CARTESIAN_POINT('Ctrl Pts',(-2.76723879242068,1.30000000000146,3.02122411948956));
#43515=CARTESIAN_POINT('Ctrl Pts',(-2.56068515941495,-1.30000000000188,
2.86595196820463));
#43516=CARTESIAN_POINT('Ctrl Pts',(-2.53896378271869,-1.18514270861306,
2.84914234896317));
#43517=CARTESIAN_POINT('Ctrl Pts',(-2.52138535408007,-1.06847604194576,
2.8473371052107));
#43518=CARTESIAN_POINT('Ctrl Pts',(-2.49034670617944,-0.794772684000851,
2.87782973999923));
#43519=CARTESIAN_POINT('Ctrl Pts',(-2.47896213176933,-0.636309800095197,
2.95085588585943));
#43520=CARTESIAN_POINT('Ctrl Pts',(-2.47407845732068,-0.319434907277159,
3.02713594692395));
#43521=CARTESIAN_POINT('Ctrl Pts',(-2.47730282393709,-0.158333333333332,
3.08164150312981));
#43522=CARTESIAN_POINT('Ctrl Pts',(-2.50593474386354,0.158333333333335,
3.09888219729377));
#43523=CARTESIAN_POINT('Ctrl Pts',(-2.5325634168507,0.319434907277167,3.06228370370256));
#43524=CARTESIAN_POINT('Ctrl Pts',(-2.59328091776413,0.636309800095207,
3.01976435072494));
#43525=CARTESIAN_POINT('Ctrl Pts',(-2.63558849376141,0.79477268400084,2.96455750976156));
#43526=CARTESIAN_POINT('Ctrl Pts',(-2.70539049701901,1.06847604194556,2.95946258502623));
#43527=CARTESIAN_POINT('Ctrl Pts',(-2.73676209961397,1.18514270861267,2.97105808535257));
#43528=CARTESIAN_POINT('Ctrl Pts',(-2.76929060401276,1.30000000000132,2.99645449013761));
#43529=CARTESIAN_POINT('Ctrl Pts',(-2.56007871299464,-1.30000000000188,
2.85301515320661));
#43530=CARTESIAN_POINT('Ctrl Pts',(-2.53830479690512,-1.18514270861306,
2.83374468235308));
#43531=CARTESIAN_POINT('Ctrl Pts',(-2.52071187691441,-1.06847604194576,
2.83014510068077));
#43532=CARTESIAN_POINT('Ctrl Pts',(-2.48972764967806,-0.794772684000851,
2.85803223588308));
#43533=CARTESIAN_POINT('Ctrl Pts',(-2.47833749752908,-0.636309800095197,
2.93149143136161));
#43534=CARTESIAN_POINT('Ctrl Pts',(-2.47397094455174,-0.319434907277159,
3.00785804372322));
#43535=CARTESIAN_POINT('Ctrl Pts',(-2.47794645705588,-0.158333333333332,
3.06342740196054));
#43536=CARTESIAN_POINT('Ctrl Pts',(-2.50702387179274,0.158333333333335,
3.08081746057002));
#43537=CARTESIAN_POINT('Ctrl Pts',(-2.53348691515876,0.319434907277167,
3.04335648601618));
#43538=CARTESIAN_POINT('Ctrl Pts',(-2.5943095218286,0.636309800095207,3.00094899446167));
#43539=CARTESIAN_POINT('Ctrl Pts',(-2.63684270751801,0.79477268400084,2.94536468398828));
#43540=CARTESIAN_POINT('Ctrl Pts',(-2.70652295950989,1.06847604194556,2.94283794041207));
#43541=CARTESIAN_POINT('Ctrl Pts',(-2.73776084593945,1.18514270861267,2.95617299979562));
#43542=CARTESIAN_POINT('Ctrl Pts',(-2.77007461961902,1.30000000000132,2.98393685223179));
#43543=CARTESIAN_POINT('',(-2.73381727423405,1.2,3.07341023227417));
#43544=CARTESIAN_POINT('Ctrl Pts',(-2.73381727423405,1.2,3.07341023227417));
#43545=CARTESIAN_POINT('Ctrl Pts',(-2.73580502907171,1.21681156976446,3.09489320825098));
#43546=CARTESIAN_POINT('Ctrl Pts',(-2.73871695256444,1.23323051929576,3.11658988393981));
#43547=CARTESIAN_POINT('Ctrl Pts',(-2.74231883146871,1.26415219681706,3.15632227320206));
#43548=CARTESIAN_POINT('Ctrl Pts',(-2.74473649442256,1.28359571150105,3.18148300895735));
#43549=CARTESIAN_POINT('Ctrl Pts',(-2.74608525934289,1.30000000000146,3.2023111991545));
#43550=CARTESIAN_POINT('',(-2.60194865074143,0.653834841416716,2.98901873446979));
#43551=CARTESIAN_POINT('Ctrl Pts',(-2.60194865075745,0.65383484141603,2.989018734449));
#43552=CARTESIAN_POINT('Ctrl Pts',(-2.61579853831374,0.71799825259359,2.99757652513191));
#43553=CARTESIAN_POINT('Ctrl Pts',(-2.62696193981467,0.76351236162102,3.00454348125093));
#43554=CARTESIAN_POINT('Ctrl Pts',(-2.67092267687889,0.949774304316204,
3.03227820052749));
#43555=CARTESIAN_POINT('Ctrl Pts',(-2.69392872614227,1.04621155459823,3.04698453746189));
#43556=CARTESIAN_POINT('Ctrl Pts',(-2.73381727423405,1.2,3.07341023227417));
#43557=CARTESIAN_POINT('',(-2.48224831221779,-0.653834841531101,2.91736724473229));
#43558=CARTESIAN_POINT('Ctrl Pts',(-2.48224831221779,-0.653834841531099,
2.91736724473229));
#43559=CARTESIAN_POINT('Ctrl Pts',(-2.4784792853279,-0.575798967915911,
2.958866742215));
#43560=CARTESIAN_POINT('Ctrl Pts',(-2.47600965983172,-0.493921361947821,
2.99371556393921));
#43561=CARTESIAN_POINT('Ctrl Pts',(-2.47496436360723,-0.338198104431773,
3.04440076767245));
#43562=CARTESIAN_POINT('Ctrl Pts',(-2.47585304481096,-0.265712087248226,
3.06229123000691));
#43563=CARTESIAN_POINT('Ctrl Pts',(-2.48131735719936,-0.129742360743047,
3.08607972132565));
#43564=CARTESIAN_POINT('Ctrl Pts',(-2.48531283701423,-0.0666417585396564,
3.09333573958426));
#43565=CARTESIAN_POINT('Ctrl Pts',(-2.49656567467154,0.0595518523103038,
3.10050515929398));
#43566=CARTESIAN_POINT('Ctrl Pts',(-2.5038994701171,0.122798807524931,3.10048726948258));
#43567=CARTESIAN_POINT('Ctrl Pts',(-2.52282835424652,0.260150875487055,
3.09199370964883));
#43568=CARTESIAN_POINT('Ctrl Pts',(-2.53495970880385,0.333952437389984,
3.08197833173551));
#43569=CARTESIAN_POINT('Ctrl Pts',(-2.56433395610792,0.49123816976692,3.04808238203451));
#43570=CARTESIAN_POINT('Ctrl Pts',(-2.58224470446943,0.574172359428836,
3.02219716120638));
#43571=CARTESIAN_POINT('Ctrl Pts',(-2.6019486507569,0.653834841428434,2.98901873450711));
#43572=CARTESIAN_POINT('',(-2.54441412395572,-1.2,2.9540069752984));
#43573=CARTESIAN_POINT('Ctrl Pts',(-2.54441412395572,-1.2,2.9540069752984));
#43574=CARTESIAN_POINT('Ctrl Pts',(-2.53391960792159,-1.13536848923257,
2.94771812963474));
#43575=CARTESIAN_POINT('Ctrl Pts',(-2.51976513845017,-1.03917846089085,
2.93929182203061));
#43576=CARTESIAN_POINT('Ctrl Pts',(-2.49231083191816,-0.795650855253786,
2.92319530513295));
#43577=CARTESIAN_POINT('Ctrl Pts',(-2.4879173222092,-0.741453969039744,
2.92065304841597));
#43578=CARTESIAN_POINT('Ctrl Pts',(-2.48224831221779,-0.653834841531101,
2.91736724473229));
#43579=CARTESIAN_POINT('Ctrl Pts',(-2.5566292407628,-1.30000000000004,3.07857464882885));
#43580=CARTESIAN_POINT('Ctrl Pts',(-2.55515567833128,-1.2829468561125,3.05759280558607));
#43581=CARTESIAN_POINT('Ctrl Pts',(-2.55296732838268,-1.26611601653633,
3.03648706140119));
#43582=CARTESIAN_POINT('Ctrl Pts',(-2.54981115104406,-1.23888922084291,
3.00267573436432));
#43583=CARTESIAN_POINT('Ctrl Pts',(-2.54792518421048,-1.21938151191995,
2.97870604444334));
#43584=CARTESIAN_POINT('Ctrl Pts',(-2.54441412395572,-1.2,2.9540069752984));
#43585=CARTESIAN_POINT('Origin',(0.,1.25,7.2));
#43586=CARTESIAN_POINT('Origin',(0.,1.2,7.2));
#43587=CARTESIAN_POINT('Origin',(0.,0.92691742076555,7.2));
#43588=CARTESIAN_POINT('Origin',(0.,0.653834841531101,7.2));
#43589=CARTESIAN_POINT('Origin',(0.,0.,7.2));
#43590=CARTESIAN_POINT('Origin',(0.,-0.653834841531101,7.2));
#43591=CARTESIAN_POINT('Origin',(0.,-0.926917420765551,7.2));
#43592=CARTESIAN_POINT('Origin',(0.,-1.2,7.2));
#43593=CARTESIAN_POINT('Origin',(0.,-1.25,7.2));
#43594=CARTESIAN_POINT('Ctrl Pts',(-2.26618048011826,-1.30000000000181,
2.69301343514311));
#43595=CARTESIAN_POINT('Ctrl Pts',(-2.3063815684754,-1.18514270861301,2.70711605782214));
#43596=CARTESIAN_POINT('Ctrl Pts',(-2.33354901187764,-1.06847604194574,
2.72750133133817));
#43597=CARTESIAN_POINT('Ctrl Pts',(-2.36620091374758,-0.794772684000851,
2.78910957149348));
#43598=CARTESIAN_POINT('Ctrl Pts',(-2.33933008166882,-0.636309800095197,
2.85373654604466));
#43599=CARTESIAN_POINT('Ctrl Pts',(-2.33301542000619,-0.319434907277159,
2.92761421432354));
#43600=CARTESIAN_POINT('Ctrl Pts',(-2.31380478607559,-0.158333333333332,
2.96926236941578));
#43601=CARTESIAN_POINT('Ctrl Pts',(-2.34340372597314,0.158333333333334,
2.98574911994944));
#43602=CARTESIAN_POINT('Ctrl Pts',(-2.3935159581309,0.319434907277167,2.96140733565195));
#43603=CARTESIAN_POINT('Ctrl Pts',(-2.45746810794752,0.636309800095206,
2.91944248366745));
#43604=CARTESIAN_POINT('Ctrl Pts',(-2.51539056129684,0.79477268400084,2.87284872481844));
#43605=CARTESIAN_POINT('Ctrl Pts',(-2.52404941520302,1.06847604194579,2.83207202931349));
#43606=CARTESIAN_POINT('Ctrl Pts',(-2.51213562603719,1.18514270861311,2.81863590450963));
#43607=CARTESIAN_POINT('Ctrl Pts',(-2.4845599506917,1.30000000000198,2.80941437546059));
#43608=CARTESIAN_POINT('Ctrl Pts',(-2.25573189552084,-1.30000000000181,
2.69995123148277));
#43609=CARTESIAN_POINT('Ctrl Pts',(-2.2939900794401,-1.185142708613,2.71542354022312));
#43610=CARTESIAN_POINT('Ctrl Pts',(-2.31971787859578,-1.06847604194573,
2.73679439485206));
#43611=CARTESIAN_POINT('Ctrl Pts',(-2.35020654597518,-0.794772684000847,
2.79979216527225));
#43612=CARTESIAN_POINT('Ctrl Pts',(-2.32354980721586,-0.636309800095194,
2.86403502138493));
#43613=CARTESIAN_POINT('Ctrl Pts',(-2.31708571783413,-0.319434907277157,
2.93787759613429));
#43614=CARTESIAN_POINT('Ctrl Pts',(-2.2987048291419,-0.158333333333332,
2.9792379501954));
#43615=CARTESIAN_POINT('Ctrl Pts',(-2.32795166822999,0.158333333333334,
2.99541357312894));
#43616=CARTESIAN_POINT('Ctrl Pts',(-2.37676704786357,0.319434907277166,
2.97095317842074));
#43617=CARTESIAN_POINT('Ctrl Pts',(-2.44038568131416,0.636309800095204,
2.92858376177118));
#43618=CARTESIAN_POINT('Ctrl Pts',(-2.49793589154108,0.794772684000836,
2.88221135823736));
#43619=CARTESIAN_POINT('Ctrl Pts',(-2.50882396394661,1.06847604194578,2.84008478326095));
#43620=CARTESIAN_POINT('Ctrl Pts',(-2.49847136268352,1.18514270861311,2.82576403936588));
#43621=CARTESIAN_POINT('Ctrl Pts',(-2.47305311705583,1.30000000000198,2.81535758493964));
#43622=CARTESIAN_POINT('Ctrl Pts',(-2.24023758932582,-1.30000000000177,
2.71044742385437));
#43623=CARTESIAN_POINT('Ctrl Pts',(-2.27464917943828,-1.18514270861297,
2.72728042721628));
#43624=CARTESIAN_POINT('Ctrl Pts',(-2.29769987754193,-1.06847604194571,
2.74975004762311));
#43625=CARTESIAN_POINT('Ctrl Pts',(-2.32470566815866,-0.794772684000827,
2.81468107877005));
#43626=CARTESIAN_POINT('Ctrl Pts',(-2.30007955902539,-0.636309800095177,
2.87967363864554));
#43627=CARTESIAN_POINT('Ctrl Pts',(-2.29369713320137,-0.319434907277148,
2.95370134444852));
#43628=CARTESIAN_POINT('Ctrl Pts',(-2.27561853252957,-0.158333333333327,
2.99387261037791));
#43629=CARTESIAN_POINT('Ctrl Pts',(-2.30447284024276,0.158333333333329,
3.00970660738443));
#43630=CARTESIAN_POINT('Ctrl Pts',(-2.35230439668206,0.319434907277157,
2.98587434975564));
#43631=CARTESIAN_POINT('Ctrl Pts',(-2.41563048835693,0.636309800095186,
2.94307068412525));
#43632=CARTESIAN_POINT('Ctrl Pts',(-2.47192554671346,0.794772684000815,
2.89644828076972));
#43633=CARTESIAN_POINT('Ctrl Pts',(-2.48619431364992,1.06847604194576,2.85230756492692));
#43634=CARTESIAN_POINT('Ctrl Pts',(-2.47832233997716,1.18514270861308,2.83676282415757));
#43635=CARTESIAN_POINT('Ctrl Pts',(-2.45640197213473,1.30000000000194,2.82478022293255));
#43636=CARTESIAN_POINT('Ctrl Pts',(-2.22015396647836,-1.30000000000176,
2.72496915303494));
#43637=CARTESIAN_POINT('Ctrl Pts',(-2.25087006485636,-1.18514270861296,
2.74472365449367));
#43638=CARTESIAN_POINT('Ctrl Pts',(-2.27113584128439,-1.06847604194569,
2.76926324165332));
#43639=CARTESIAN_POINT('Ctrl Pts',(-2.29381150470358,-0.794772684000816,
2.83700910234178));
#43640=CARTESIAN_POINT('Ctrl Pts',(-2.26906479704234,-0.636309800095173,
2.90079934686356));
#43641=CARTESIAN_POINT('Ctrl Pts',(-2.26248272481726,-0.319434907277148,
2.97484635426529));
#43642=CARTESIAN_POINT('Ctrl Pts',(-2.24666840933008,-0.158333333333326,
3.01490679633203));
#43643=CARTESIAN_POINT('Ctrl Pts',(-2.27501627587942,0.158333333333328,
3.03030387788487));
#43644=CARTESIAN_POINT('Ctrl Pts',(-2.32020441102578,0.319434907277153,
3.00625628639059));
#43645=CARTESIAN_POINT('Ctrl Pts',(-2.38243925368409,0.63630980009518,2.96231774832919));
#43646=CARTESIAN_POINT('Ctrl Pts',(-2.43709121076443,0.794772684000812,
2.91538998751791));
#43647=CARTESIAN_POINT('Ctrl Pts',(-2.45575844588796,1.06847604194575,2.86846020459651));
#43648=CARTESIAN_POINT('Ctrl Pts',(-2.4511861078754,1.18514270861307,2.85126535631407));
#43649=CARTESIAN_POINT('Ctrl Pts',(-2.43396107745452,1.30000000000192,2.83718982385607));
#43650=CARTESIAN_POINT('Ctrl Pts',(-2.20918327510351,-1.30000000000174,
2.73201602488139));
#43651=CARTESIAN_POINT('Ctrl Pts',(-2.23786695827226,-1.18514270861294,
2.75316866377135));
#43652=CARTESIAN_POINT('Ctrl Pts',(-2.25666445064859,-1.06847604194567,
2.77874389990702));
#43653=CARTESIAN_POINT('Ctrl Pts',(-2.27725134000709,-0.794772684000803,
2.84804489606377));
#43654=CARTESIAN_POINT('Ctrl Pts',(-2.25314430197671,-0.63630980009516,
2.91177053549845));
#43655=CARTESIAN_POINT('Ctrl Pts',(-2.24635850625787,-0.319434907277141,
2.98574247512785));
#43656=CARTESIAN_POINT('Ctrl Pts',(-2.23079433029514,-0.158333333333323,
3.02501430692331));
#43657=CARTESIAN_POINT('Ctrl Pts',(-2.25886970073135,0.158333333333325,
3.04017865402025));
#43658=CARTESIAN_POINT('Ctrl Pts',(-2.30343128907705,0.319434907277148,
3.01660940791817));
#43659=CARTESIAN_POINT('Ctrl Pts',(-2.36552645982439,0.636309800095169,
2.97242979818955));
#43660=CARTESIAN_POINT('Ctrl Pts',(-2.4194102278767,0.794772684000795,2.92542134923293));
#43661=CARTESIAN_POINT('Ctrl Pts',(-2.44036738855896,1.06847604194573,2.8770660452405));
#43662=CARTESIAN_POINT('Ctrl Pts',(-2.43745361027784,1.18514270861305,2.85897966453637));
#43663=CARTESIAN_POINT('Ctrl Pts',(-2.42255447539554,1.3000000000019,2.8437381224859));
#43664=CARTESIAN_POINT('Ctrl Pts',(-2.20346973531821,-1.30000000000173,
2.73604655795091));
#43665=CARTESIAN_POINT('Ctrl Pts',(-2.23082832504476,-1.18514270861294,
2.7578092215297));
#43666=CARTESIAN_POINT('Ctrl Pts',(-2.24868608239779,-1.06847604194567,
2.78385225923261));
#43667=CARTESIAN_POINT('Ctrl Pts',(-2.26799225089751,-0.794772684000801,
2.85390540673059));
#43668=CARTESIAN_POINT('Ctrl Pts',(-2.24435183302002,-0.636309800095158,
2.91767688584819));
#43669=CARTESIAN_POINT('Ctrl Pts',(-2.2376941901163,-0.31943490727714,2.99179590928583));
#43670=CARTESIAN_POINT('Ctrl Pts',(-2.22268877944014,-0.158333333333323,
3.0309717544654));
#43671=CARTESIAN_POINT('Ctrl Pts',(-2.25062408390699,0.158333333333325,
3.046016730154));
#43672=CARTESIAN_POINT('Ctrl Pts',(-2.29437339664253,0.319434907277148,
3.02233571445109));
#43673=CARTESIAN_POINT('Ctrl Pts',(-2.35628618826155,0.636309800095168,
2.97794590344119));
#43674=CARTESIAN_POINT('Ctrl Pts',(-2.41003977131771,0.794772684000792,
2.9311343199028));
#43675=CARTESIAN_POINT('Ctrl Pts',(-2.43223231681768,1.06847604194572,2.88198830670547));
#43676=CARTESIAN_POINT('Ctrl Pts',(-2.43016869531126,1.18514270861304,2.8633680524723));
#43677=CARTESIAN_POINT('Ctrl Pts',(-2.41643512166632,1.3000000000019,2.84740103207989));
#43678=CARTESIAN_POINT('Ctrl Pts',(-2.20220161285603,-1.30000000000173,
2.736943664336));
#43679=CARTESIAN_POINT('Ctrl Pts',(-2.22927156689297,-1.18514270861294,
2.75884624111174));
#43680=CARTESIAN_POINT('Ctrl Pts',(-2.24692402372033,-1.06847604194567,
2.78499587321189));
#43681=CARTESIAN_POINT('Ctrl Pts',(-2.26594842783543,-0.794772684000802,
2.85521830199896));
#43682=CARTESIAN_POINT('Ctrl Pts',(-2.2424061778417,-0.636309800095159,
2.91899593966009));
#43683=CARTESIAN_POINT('Ctrl Pts',(-2.23577092804783,-0.31943490727714,
2.99314298560829));
#43684=CARTESIAN_POINT('Ctrl Pts',(-2.22088144654913,-0.158333333333323,
3.03229096841701));
#43685=CARTESIAN_POINT('Ctrl Pts',(-2.24878591432589,0.158333333333325,
3.04730973287704));
#43686=CARTESIAN_POINT('Ctrl Pts',(-2.29236670423403,0.319434907277148,
3.02361353216002));
#43687=CARTESIAN_POINT('Ctrl Pts',(-2.35423860798645,0.636309800095168,
2.97917660229254));
#43688=CARTESIAN_POINT('Ctrl Pts',(-2.40795028438503,0.794772684000792,
2.93239806134971));
#43689=CARTESIAN_POINT('Ctrl Pts',(-2.43041593543582,1.06847604194572,2.88307512146419));
#43690=CARTESIAN_POINT('Ctrl Pts',(-2.42854286265926,1.18514270861304,2.86433755511563));
#43691=CARTESIAN_POINT('Ctrl Pts',(-2.41507216920065,1.3000000000019,2.84821249549997));
#43692=CARTESIAN_POINT('Ctrl Pts',(-2.19999465780069,-1.30000000000173,
2.73852275171296));
#43693=CARTESIAN_POINT('Ctrl Pts',(-2.2265649885852,-1.18514270861294,2.76067455593726));
#43694=CARTESIAN_POINT('Ctrl Pts',(-2.24386117344665,-1.06847604194567,
2.78701316951011));
#43695=CARTESIAN_POINT('Ctrl Pts',(-2.2623936881977,-0.794772684000802,
2.85753300304829));
#43696=CARTESIAN_POINT('Ctrl Pts',(-2.2390139300092,-0.636309800095159,
2.92131431647447));
#43697=CARTESIAN_POINT('Ctrl Pts',(-2.23241366923983,-0.31943490727714,
2.99550733624859));
#43698=CARTESIAN_POINT('Ctrl Pts',(-2.21772704650828,-0.158333333333323,
3.03460660392587));
#43699=CARTESIAN_POINT('Ctrl Pts',(-2.24557742550624,0.158333333333325,
3.04957956852225));
#43700=CARTESIAN_POINT('Ctrl Pts',(-2.28886747707637,0.319434907277148,
3.02586029132576));
#43701=CARTESIAN_POINT('Ctrl Pts',(-2.35066304626681,0.636309800095168,
2.98133703992553));
#43702=CARTESIAN_POINT('Ctrl Pts',(-2.40428872280094,0.794772684000793,
2.93460592573491));
#43703=CARTESIAN_POINT('Ctrl Pts',(-2.42722935465882,1.06847604194573,2.88497087357005));
#43704=CARTESIAN_POINT('Ctrl Pts',(-2.425690744435,1.18514270861304,2.86602878533394));
#43705=CARTESIAN_POINT('Ctrl Pts',(-2.41268337449024,1.3000000000019,2.84962978378401));
#43706=CARTESIAN_POINT('Ctrl Pts',(-2.19687172842388,-1.30000000000173,
2.74080211112429));
#43707=CARTESIAN_POINT('Ctrl Pts',(-2.22276863898883,-1.18514270861294,
2.76334050676099));
#43708=CARTESIAN_POINT('Ctrl Pts',(-2.23957943286202,-1.06847604194567,
2.78996699298122));
#43709=CARTESIAN_POINT('Ctrl Pts',(-2.25742498246745,-0.794772684000802,
2.86092380982778));
#43710=CARTESIAN_POINT('Ctrl Pts',(-2.23422822527225,-0.636309800095159,
2.92467365053622));
#43711=CARTESIAN_POINT('Ctrl Pts',(-2.22763998419137,-0.31943490727714,
2.99890348786697));
#43712=CARTESIAN_POINT('Ctrl Pts',(-2.21320683729874,-0.158333333333323,
3.03790452917699));
#43713=CARTESIAN_POINT('Ctrl Pts',(-2.24098092916929,0.158333333333325,
3.05281353014586));
#43714=CARTESIAN_POINT('Ctrl Pts',(-2.28391842045281,0.319434907277148,
3.02911205885407));
#43715=CARTESIAN_POINT('Ctrl Pts',(-2.34559301506903,0.636309800095169,
2.98445522198158));
#43716=CARTESIAN_POINT('Ctrl Pts',(-2.39900929438297,0.794772684000794,
2.93772042282925));
#43717=CARTESIAN_POINT('Ctrl Pts',(-2.42261750004445,1.06847604194573,2.88763026047032));
#43718=CARTESIAN_POINT('Ctrl Pts',(-2.4215675118097,1.18514270861305,2.86840485303774));
#43719=CARTESIAN_POINT('Ctrl Pts',(-2.40924841787956,1.3000000000019,2.85163621343437));
#43720=CARTESIAN_POINT('Ctrl Pts',(-2.19316744487638,-1.30000000000174,
2.74357227885489));
#43721=CARTESIAN_POINT('Ctrl Pts',(-2.21833012274304,-1.18514270861294,
2.7666303563685));
#43722=CARTESIAN_POINT('Ctrl Pts',(-2.23460232797405,-1.06847604194567,
2.79363545208276));
#43723=CARTESIAN_POINT('Ctrl Pts',(-2.25165560697981,-0.794772684000803,
2.86514102717516));
#43724=CARTESIAN_POINT('Ctrl Pts',(-2.22859618268033,-0.63630980009516,
2.92879166006676));
#43725=CARTESIAN_POINT('Ctrl Pts',(-2.22195206858178,-0.31943490727714,
3.00301196088743));
#43726=CARTESIAN_POINT('Ctrl Pts',(-2.2077469105008,-0.158333333333323,
3.04183500405772));
#43727=CARTESIAN_POINT('Ctrl Pts',(-2.23542982559815,0.158333333333325,
3.05666885096073));
#43728=CARTESIAN_POINT('Ctrl Pts',(-2.2780636700841,0.319434907277148,3.03308550913707));
#43729=CARTESIAN_POINT('Ctrl Pts',(-2.33957680654361,0.636309800095169,
2.98825399010626));
#43730=CARTESIAN_POINT('Ctrl Pts',(-2.39259171033951,0.794772684000794,
2.94139027310225));
#43731=CARTESIAN_POINT('Ctrl Pts',(-2.4169793379928,1.06847604194573,2.89073594490276));
#43732=CARTESIAN_POINT('Ctrl Pts',(-2.41653230162815,1.18514270861305,2.87118437238136));
#43733=CARTESIAN_POINT('Ctrl Pts',(-2.40508172853836,1.3000000000019,2.85400760908834));
#43734=CARTESIAN_POINT('Ctrl Pts',(-2.1882615792186,-1.30000000000174,2.74729347372498));
#43735=CARTESIAN_POINT('Ctrl Pts',(-2.21251194251739,-1.18514270861294,
2.77109483631768));
#43736=CARTESIAN_POINT('Ctrl Pts',(-2.22810677709066,-1.06847604194568,
2.79863555033522));
#43737=CARTESIAN_POINT('Ctrl Pts',(-2.24413796180227,-0.794772684000805,
2.87089875906258));
#43738=CARTESIAN_POINT('Ctrl Pts',(-2.22119516131167,-0.636309800095161,
2.93436736296658));
#43739=CARTESIAN_POINT('Ctrl Pts',(-2.21442134321395,-0.319434907277141,
3.00853253480121));
#43740=CARTESIAN_POINT('Ctrl Pts',(-2.20045776457667,-0.158333333333323,
3.04706852295238));
#43741=CARTESIAN_POINT('Ctrl Pts',(-2.22801848204205,0.158333333333325,
3.06180316130134));
#43742=CARTESIAN_POINT('Ctrl Pts',(-2.2703440691031,0.319434907277149,3.038456775792));
#43743=CARTESIAN_POINT('Ctrl Pts',(-2.33162491225292,0.63630980009517,2.99337827183899));
#43744=CARTESIAN_POINT('Ctrl Pts',(-2.38397630173446,0.794772684000795,
2.94623641534027));
#43745=CARTESIAN_POINT('Ctrl Pts',(-2.40938468889191,1.06847604194573,2.8948141664764));
#43746=CARTESIAN_POINT('Ctrl Pts',(-2.40975612978786,1.18514270861305,2.87483947628986));
#43747=CARTESIAN_POINT('Ctrl Pts',(-2.3995006622528,1.3000000000019,2.85714888206791));
#43748=CARTESIAN_POINT('Ctrl Pts',(-2.18212017945675,-1.30000000000174,
2.75194076206201));
#43749=CARTESIAN_POINT('Ctrl Pts',(-2.20522580669821,-1.18514270861294,
2.77666914190148));
#43750=CARTESIAN_POINT('Ctrl Pts',(-2.21997833269593,-1.06847604194568,
2.80488347370449));
#43751=CARTESIAN_POINT('Ctrl Pts',(-2.23476228407815,-0.794772684000806,
2.87811747082507));
#43752=CARTESIAN_POINT('Ctrl Pts',(-2.2120269831232,-0.636309800095161,
2.94140396771728));
#43753=CARTESIAN_POINT('Ctrl Pts',(-2.20512598857467,-0.319434907277141,
3.01552645780187));
#43754=CARTESIAN_POINT('Ctrl Pts',(-2.19146800850019,-0.158333333333323,
3.0537060746734));
#43755=CARTESIAN_POINT('Ctrl Pts',(-2.21885670803492,0.158333333333325,
3.06830343605117));
#43756=CARTESIAN_POINT('Ctrl Pts',(-2.26073620860078,0.319434907277149,
3.0452087803244));
#43757=CARTESIAN_POINT('Ctrl Pts',(-2.32172961572616,0.63630980009517,2.99982685870441));
#43758=CARTESIAN_POINT('Ctrl Pts',(-2.37334890728109,0.794772684000796,
2.95241607700585));
#43759=CARTESIAN_POINT('Ctrl Pts',(-2.40000587537004,1.06847604194573,2.90001138005715));
#43760=CARTESIAN_POINT('Ctrl Pts',(-2.40136335569043,1.18514270861305,2.87947725010413));
#43761=CARTESIAN_POINT('Ctrl Pts',(-2.3925395025835,1.30000000000191,2.86109304172183));
#43762=CARTESIAN_POINT('Ctrl Pts',(-2.17208212925898,-1.30000000000174,
2.75921618055832));
#43763=CARTESIAN_POINT('Ctrl Pts',(-2.19303494876364,-1.18514270861295,
2.78518939374164));
#43764=CARTESIAN_POINT('Ctrl Pts',(-2.20626192734724,-1.06847604194568,
2.8143499086739));
#43765=CARTESIAN_POINT('Ctrl Pts',(-2.21897065584651,-0.794772684000809,
2.88907983636582));
#43766=CARTESIAN_POINT('Ctrl Pts',(-2.19699313048707,-0.636309800095163,
2.95239100512114));
#43767=CARTESIAN_POINT('Ctrl Pts',(-2.1903252370132,-0.319434907277142,
3.02677694489908));
#43768=CARTESIAN_POINT('Ctrl Pts',(-2.17763876613698,-0.158333333333324,
3.06475897608085));
#43769=CARTESIAN_POINT('Ctrl Pts',(-2.2047633195661,0.158333333333326,3.0791437952662));
#43770=CARTESIAN_POINT('Ctrl Pts',(-2.24525338460493,0.319434907277149,
3.05592173076589));
#43771=CARTESIAN_POINT('Ctrl Pts',(-2.30578888329971,0.636309800095172,
3.01007248348909));
#43772=CARTESIAN_POINT('Ctrl Pts',(-2.35692263128715,0.794772684000799,
2.96280581578494));
#43773=CARTESIAN_POINT('Ctrl Pts',(-2.3856458783688,1.06847604194573,2.90888116363136));
#43774=CARTESIAN_POINT('Ctrl Pts',(-2.38849242500615,1.18514270861305,2.88737253804549));
#43775=CARTESIAN_POINT('Ctrl Pts',(-2.38175228892037,1.30000000000191,2.86769727068581));
#43776=CARTESIAN_POINT('Ctrl Pts',(-2.15949961246368,-1.30000000000175,
2.76829662997937));
#43777=CARTESIAN_POINT('Ctrl Pts',(-2.17777936667385,-1.18514270861295,
2.79584352702837));
#43778=CARTESIAN_POINT('Ctrl Pts',(-2.18909913156332,-1.06847604194569,
2.82618941541642));
#43779=CARTESIAN_POINT('Ctrl Pts',(-2.19917108529723,-0.794772684000813,
2.90276071819625));
#43780=CARTESIAN_POINT('Ctrl Pts',(-2.1780294378193,-0.636309800095167,
2.96601852987045));
#43781=CARTESIAN_POINT('Ctrl Pts',(-2.17159203546571,-0.319434907277144,
3.04068386847602));
#43782=CARTESIAN_POINT('Ctrl Pts',(-2.16007347128678,-0.158333333333325,
3.07837413098288));
#43783=CARTESIAN_POINT('Ctrl Pts',(-2.18697813276709,0.158333333333327,
3.09257702156199));
#43784=CARTESIAN_POINT('Ctrl Pts',(-2.22605377032027,0.319434907277152,
3.06945503396162));
#43785=CARTESIAN_POINT('Ctrl Pts',(-2.28596511485657,0.636309800095176,
3.02297569925729));
#43786=CARTESIAN_POINT('Ctrl Pts',(-2.33604912362317,0.794772684000802,
2.97552561301708));
#43787=CARTESIAN_POINT('Ctrl Pts',(-2.36723098225282,1.06847604194574,2.91960304856153));
#43788=CARTESIAN_POINT('Ctrl Pts',(-2.37194882244496,1.18514270861306,2.89688745512843));
#43789=CARTESIAN_POINT('Ctrl Pts',(-2.36788703163017,1.30000000000192,2.87566307427989));
#43790=CARTESIAN_POINT('Ctrl Pts',(-2.1400296612085,-1.30000000000177,2.78332408910354));
#43791=CARTESIAN_POINT('Ctrl Pts',(-2.15457256128359,-1.18514270861297,
2.81379802010596));
#43792=CARTESIAN_POINT('Ctrl Pts',(-2.16321725789178,-1.0684760419457,2.84632547071609));
#43793=CARTESIAN_POINT('Ctrl Pts',(-2.16956220648216,-0.794772684000821,
2.92621442981849));
#43794=CARTESIAN_POINT('Ctrl Pts',(-2.14972875993447,-0.636309800095173,
2.98935755509729));
#43795=CARTESIAN_POINT('Ctrl Pts',(-2.14315859529316,-0.319434907277147,
3.06409898165379));
#43796=CARTESIAN_POINT('Ctrl Pts',(-2.13261471316304,-0.158333333333326,
3.10066177827065));
#43797=CARTESIAN_POINT('Ctrl Pts',(-2.15855621259014,0.158333333333328,
3.11412656762498));
#43798=CARTESIAN_POINT('Ctrl Pts',(-2.19511681652783,0.319434907277155,
3.09096870395781));
#43799=CARTESIAN_POINT('Ctrl Pts',(-2.25437472507939,0.636309800095182,
3.04377600700554));
#43800=CARTESIAN_POINT('Ctrl Pts',(-2.3039528815301,0.79477268400081,2.99699282002359));
#43801=CARTESIAN_POINT('Ctrl Pts',(-2.33931845409527,1.06847604194575,2.9380534808914));
#43802=CARTESIAN_POINT('Ctrl Pts',(-2.34693156225004,1.18514270861307,2.91330860187064));
#43803=CARTESIAN_POINT('Ctrl Pts',(-2.34684933261967,1.30000000000193,2.88933149982177));
#43804=CARTESIAN_POINT('Ctrl Pts',(-2.12052229387443,-1.30000000000177,
2.79835037140423));
#43805=CARTESIAN_POINT('Ctrl Pts',(-2.13136849242446,-1.18514270861297,
2.83178169880633));
#43806=CARTESIAN_POINT('Ctrl Pts',(-2.13727436244986,-1.06847604194571,
2.86644568934175));
#43807=CARTESIAN_POINT('Ctrl Pts',(-2.13950495647254,-0.794772684000832,
2.94937414041727));
#43808=CARTESIAN_POINT('Ctrl Pts',(-2.12000342318202,-0.636309800095182,
3.01169593614363));
#43809=CARTESIAN_POINT('Ctrl Pts',(-2.11330403078325,-0.319434907277152,
3.08651916057855));
#43810=CARTESIAN_POINT('Ctrl Pts',(-2.10434476941678,-0.158333333333328,
3.12238322192707));
#43811=CARTESIAN_POINT('Ctrl Pts',(-2.13034146592244,0.158333333333331,
3.13588233349007));
#43812=CARTESIAN_POINT('Ctrl Pts',(-2.16577982275893,0.319434907277158,
3.11378008751628));
#43813=CARTESIAN_POINT('Ctrl Pts',(-2.22445000215898,0.63630980009519,3.0659184726177));
#43814=CARTESIAN_POINT('Ctrl Pts',(-2.27190223565677,0.794772684000822,
3.01853364691345));
#43815=CARTESIAN_POINT('Ctrl Pts',(-2.31094248435717,1.06847604194576,2.9561752512662));
#43816=CARTESIAN_POINT('Ctrl Pts',(-2.32142648933868,1.18514270861309,2.92938028086924));
#43817=CARTESIAN_POINT('Ctrl Pts',(-2.32549542222303,1.30000000000195,2.9027829789448));
#43818=CARTESIAN_POINT('Ctrl Pts',(-2.10347617539217,-1.30000000000177,
2.81152704880114));
#43819=CARTESIAN_POINT('Ctrl Pts',(-2.11086560738165,-1.18514270861298,
2.8474047904178));
#43820=CARTESIAN_POINT('Ctrl Pts',(-2.1144218880465,-1.06847604194571,2.88398421097988));
#43821=CARTESIAN_POINT('Ctrl Pts',(-2.1137822614346,-0.794772684000831,
2.97011100890035));
#43822=CARTESIAN_POINT('Ctrl Pts',(-2.0965574929,-0.636309800095182,3.03312580480178));
#43823=CARTESIAN_POINT('Ctrl Pts',(-2.09019094570269,-0.319434907277152,
3.10834249787361));
#43824=CARTESIAN_POINT('Ctrl Pts',(-2.08177200594073,-0.158333333333328,
3.14299917059874));
#43825=CARTESIAN_POINT('Ctrl Pts',(-2.10676491187636,0.158333333333331,
3.15576783442169));
#43826=CARTESIAN_POINT('Ctrl Pts',(-2.14013723911703,0.319434907277159,
3.13379548380685));
#43827=CARTESIAN_POINT('Ctrl Pts',(-2.19749303240763,0.636309800095191,
3.08475943756395));
#43828=CARTESIAN_POINT('Ctrl Pts',(-2.24307107389101,0.794772684000823,
3.03682872907093));
#43829=CARTESIAN_POINT('Ctrl Pts',(-2.28547810640088,1.06847604194576,2.97158445453326));
#43830=CARTESIAN_POINT('Ctrl Pts',(-2.29865486786559,1.18514270861309,2.94312676280035));
#43831=CARTESIAN_POINT('Ctrl Pts',(-2.30665195775685,1.30000000000195,2.91445320824332));
#43832=CARTESIAN_POINT('Ctrl Pts',(-2.09398294748795,-1.30000000000178,
2.8192464505879));
#43833=CARTESIAN_POINT('Ctrl Pts',(-2.09985007592462,-1.18514270861298,
2.85683927055206));
#43834=CARTESIAN_POINT('Ctrl Pts',(-2.10222809132688,-1.06847604194571,
2.89462699936486));
#43835=CARTESIAN_POINT('Ctrl Pts',(-2.09966123352232,-0.794772684000831,
2.98237449076318));
#43836=CARTESIAN_POINT('Ctrl Pts',(-2.08208718234733,-0.636309800095182,
3.04461861941498));
#43837=CARTESIAN_POINT('Ctrl Pts',(-2.07559300407143,-0.319434907277152,
3.11983369483043));
#43838=CARTESIAN_POINT('Ctrl Pts',(-2.06819301628649,-0.158333333333329,
3.15429316403017));
#43839=CARTESIAN_POINT('Ctrl Pts',(-2.09333845137421,0.158333333333331,
3.16717379427419));
#43840=CARTESIAN_POINT('Ctrl Pts',(-2.12609654828513,0.319434907277159,
3.14569509865548));
#43841=CARTESIAN_POINT('Ctrl Pts',(-2.18337696560044,0.636309800095192,
3.09651295484401));
#43842=CARTESIAN_POINT('Ctrl Pts',(-2.22838428511871,0.794772684000823,
3.04869857741907));
#43843=CARTESIAN_POINT('Ctrl Pts',(-2.27254192517896,1.06847604194577,2.9816729024378));
#43844=CARTESIAN_POINT('Ctrl Pts',(-2.28698030954534,1.18514270861309,2.95204360255291));
#43845=CARTESIAN_POINT('Ctrl Pts',(-2.2967428720978,1.30000000000195,2.92179793393659));
#43846=CARTESIAN_POINT('Ctrl Pts',(-2.07970877079305,-1.30000000000178,
2.8307951811348));
#43847=CARTESIAN_POINT('Ctrl Pts',(-2.08302898344803,-1.18514270861298,
2.87077956661394));
#43848=CARTESIAN_POINT('Ctrl Pts',(-2.0835761767988,-1.06847604194571,2.91033894438351));
#43849=CARTESIAN_POINT('Ctrl Pts',(-2.07843407357136,-0.794772684000834,
3.00074716802572));
#43850=CARTESIAN_POINT('Ctrl Pts',(-2.06151116195105,-0.636309800095184,
3.06266775736981));
#43851=CARTESIAN_POINT('Ctrl Pts',(-2.05524410150916,-0.319434907277153,
3.13817562028094));
#43852=CARTESIAN_POINT('Ctrl Pts',(-2.04939411901467,-0.158333333333329,
3.17235824501512));
#43853=CARTESIAN_POINT('Ctrl Pts',(-2.07382117261851,0.158333333333331,
3.18471694876148));
#43854=CARTESIAN_POINT('Ctrl Pts',(-2.10395999875305,0.31943490727716,3.1627504266277));
#43855=CARTESIAN_POINT('Ctrl Pts',(-2.16026473232455,0.636309800095193,
3.11270682165839));
#43856=CARTESIAN_POINT('Ctrl Pts',(-2.20487943480485,0.794772684000825,
3.06536588123936));
#43857=CARTESIAN_POINT('Ctrl Pts',(-2.25180834481438,1.06847604194577,2.99577491820494));
#43858=CARTESIAN_POINT('Ctrl Pts',(-2.268229373859,1.18514270861309,2.96446341176438));
#43859=CARTESIAN_POINT('Ctrl Pts',(-2.28075764569255,1.30000000000195,2.93196374818161));
#43860=CARTESIAN_POINT('Ctrl Pts',(-2.05852013350791,-1.30000000000178,
2.84828080309916));
#43861=CARTESIAN_POINT('Ctrl Pts',(-2.05770642325508,-1.18514270861298,
2.89165118560606));
#43862=CARTESIAN_POINT('Ctrl Pts',(-2.05536294566111,-1.06847604194572,
2.93377693261711));
#43863=CARTESIAN_POINT('Ctrl Pts',(-2.04641497502104,-0.794772684000837,
3.02822047845532));
#43864=CARTESIAN_POINT('Ctrl Pts',(-2.03146347072319,-0.636309800095184,
3.09031719439697));
#43865=CARTESIAN_POINT('Ctrl Pts',(-2.02542091010615,-0.319434907277152,
3.16617875754651));
#43866=CARTESIAN_POINT('Ctrl Pts',(-2.02041466212552,-0.158333333333329,
3.19890879492926));
#43867=CARTESIAN_POINT('Ctrl Pts',(-2.04436817801832,0.158333333333332,
3.21095252400229));
#43868=CARTESIAN_POINT('Ctrl Pts',(-2.07318118945325,0.319434907277163,
3.1901606890519));
#43869=CARTESIAN_POINT('Ctrl Pts',(-2.12831426138427,0.636309800095196,
3.13904628501572));
#43870=CARTESIAN_POINT('Ctrl Pts',(-2.17009567002426,0.794772684000824,
3.09077697976127));
#43871=CARTESIAN_POINT('Ctrl Pts',(-2.22069839553814,1.06847604194577,3.01697886521116));
#43872=CARTESIAN_POINT('Ctrl Pts',(-2.24018483798486,1.18514270861309,2.98320571956108));
#43873=CARTESIAN_POINT('Ctrl Pts',(-2.25725367801904,1.30000000000195,2.94760389756012));
#43874=CARTESIAN_POINT('Ctrl Pts',(-2.03123509006447,-1.30000000000179,
2.87227242206237));
#43875=CARTESIAN_POINT('Ctrl Pts',(-2.02551307888917,-1.18514270861299,
2.92058116074944));
#43876=CARTESIAN_POINT('Ctrl Pts',(-2.01962846565359,-1.06847604194572,
2.96635206631251));
#43877=CARTESIAN_POINT('Ctrl Pts',(-2.00565818857887,-0.79477268400084,
3.06622911239301));
#43878=CARTESIAN_POINT('Ctrl Pts',(-1.99181080380806,-0.636309800095189,
3.12752722261015));
#43879=CARTESIAN_POINT('Ctrl Pts',(-1.98623956884247,-0.319434907277156,
3.20398179778877));
#43880=CARTESIAN_POINT('Ctrl Pts',(-1.9840531135405,-0.15833333333333,3.23592205753177));
#43881=CARTESIAN_POINT('Ctrl Pts',(-2.00742959667819,0.158333333333333,
3.24758646395566));
#43882=CARTESIAN_POINT('Ctrl Pts',(-2.03277848779165,0.319434907277164,
3.22718563067376));
#43883=CARTESIAN_POINT('Ctrl Pts',(-2.08640193473761,0.6363098000952,3.17474518670082));
#43884=CARTESIAN_POINT('Ctrl Pts',(-2.12635002237642,0.794772684000832,
3.12672289098513));
#43885=CARTESIAN_POINT('Ctrl Pts',(-2.18177959699018,1.06847604194578,3.04725857901514));
#43886=CARTESIAN_POINT('Ctrl Pts',(-2.20492375066508,1.1851427086131,3.00986786508781));
#43887=CARTESIAN_POINT('Ctrl Pts',(-2.22721864903267,1.30000000000196,2.96948359344209));
#43888=CARTESIAN_POINT('Ctrl Pts',(-2.00791251142467,-1.3000000000018,2.8919145647167));
#43889=CARTESIAN_POINT('Ctrl Pts',(-1.9982083112576,-1.185142708613,2.94439906337569));
#43890=CARTESIAN_POINT('Ctrl Pts',(-1.98961105134247,-1.06847604194573,
2.99335513283515));
#43891=CARTESIAN_POINT('Ctrl Pts',(-1.97230691448723,-0.794772684000846,
3.09830206960359));
#43892=CARTESIAN_POINT('Ctrl Pts',(-1.96086800613691,-0.636309800095193,
3.15990898663756));
#43893=CARTESIAN_POINT('Ctrl Pts',(-1.95598036571629,-0.319434907277157,
3.23703223019669));
#43894=CARTESIAN_POINT('Ctrl Pts',(-1.9550549983292,-0.158333333333331,
3.26756876591028));
#43895=CARTESIAN_POINT('Ctrl Pts',(-1.97758329963365,0.158333333333334,
3.27869728916384));
#43896=CARTESIAN_POINT('Ctrl Pts',(-2.00066280746554,0.319434907277165,
3.25911472318076));
#43897=CARTESIAN_POINT('Ctrl Pts',(-2.05220111428241,0.636309800095203,
3.20501503316702));
#43898=CARTESIAN_POINT('Ctrl Pts',(-2.08860480006725,0.794772684000836,
3.15574523365688));
#43899=CARTESIAN_POINT('Ctrl Pts',(-2.14776574424549,1.06847604194578,3.07136984319128));
#43900=CARTESIAN_POINT('Ctrl Pts',(-2.17424128073391,1.18514270861311,3.0311778824398));
#43901=CARTESIAN_POINT('Ctrl Pts',(-2.20158377310493,1.30000000000197,2.98731694105318));
#43902=CARTESIAN_POINT('Ctrl Pts',(-1.99091305460786,-1.3000000000018,2.90872364328237));
#43903=CARTESIAN_POINT('Ctrl Pts',(-1.97826555025034,-1.185142708613,2.96473708658292));
#43904=CARTESIAN_POINT('Ctrl Pts',(-1.96758712102958,-1.06847604194573,
3.01631961176005));
#43905=CARTESIAN_POINT('Ctrl Pts',(-1.94746677079526,-0.794772684000843,
3.12524925670047));
#43906=CARTESIAN_POINT('Ctrl Pts',(-1.93723551063555,-0.636309800095191,
3.18660767585824));
#43907=CARTESIAN_POINT('Ctrl Pts',(-1.93242227851553,-0.319434907277156,
3.26396326267609));
#43908=CARTESIAN_POINT('Ctrl Pts',(-1.93235644974084,-0.158333333333331,
3.29329477084362));
#43909=CARTESIAN_POINT('Ctrl Pts',(-1.95417726778959,0.158333333333333,
3.30399040075478));
#43910=CARTESIAN_POINT('Ctrl Pts',(-1.97540017859542,0.319434907277166,
3.28501519179955));
#43911=CARTESIAN_POINT('Ctrl Pts',(-2.02601282840697,0.636309800095202,
3.23013702520077));
#43912=CARTESIAN_POINT('Ctrl Pts',(-2.06124729895273,0.794772684000832,
3.18111749727711));
#43913=CARTESIAN_POINT('Ctrl Pts',(-2.1232755139284,1.06847604194578,3.09271303762915));
#43914=CARTESIAN_POINT('Ctrl Pts',(-2.15194224912549,1.18514270861311,3.04991798288438));
#43915=CARTESIAN_POINT('Ctrl Pts',(-2.18242600362851,1.30000000000197,3.00259488826848));
#43916=CARTESIAN_POINT('Ctrl Pts',(-1.96891126495522,-1.30000000000181,
2.92924299368055));
#43917=CARTESIAN_POINT('Ctrl Pts',(-1.95238134199195,-1.18514270861301,
2.98950952795956));
#43918=CARTESIAN_POINT('Ctrl Pts',(-1.93907081124648,-1.06847604194574,
3.04433306419302));
#43919=CARTESIAN_POINT('Ctrl Pts',(-1.91575826252225,-0.794772684000849,
3.15841198594957));
#43920=CARTESIAN_POINT('Ctrl Pts',(-1.90770834455703,-0.636309800095193,
3.21988669858922));
#43921=CARTESIAN_POINT('Ctrl Pts',(-1.90414604058418,-0.319434907277156,
3.29824867101159));
#43922=CARTESIAN_POINT('Ctrl Pts',(-1.90653906674807,-0.158333333333331,
3.32692479228438));
#43923=CARTESIAN_POINT('Ctrl Pts',(-1.92757773297685,0.158333333333334,
3.33716497021942));
#43924=CARTESIAN_POINT('Ctrl Pts',(-1.94526711991391,0.319434907277167,
3.31825387261697));
#43925=CARTESIAN_POINT('Ctrl Pts',(-1.9936314909294,0.636309800095204,3.26171826035597));
#43926=CARTESIAN_POINT('Ctrl Pts',(-2.02662383139231,0.794772684000835,
3.21243371031589));
#43927=CARTESIAN_POINT('Ctrl Pts',(-2.0918247018996,1.06847604194578,3.11874594249202));
#43928=CARTESIAN_POINT('Ctrl Pts',(-2.12322116663215,1.18514270861311,3.07271557600675));
#43929=CARTESIAN_POINT('Ctrl Pts',(-2.15779105518492,1.30000000000197,3.02120880625334));
#43930=CARTESIAN_POINT('Ctrl Pts',(-1.94765865101397,-1.30000000000181,
2.95030374733435));
#43931=CARTESIAN_POINT('Ctrl Pts',(-1.92790508340059,-1.18514270861301,
3.01529722891932));
#43932=CARTESIAN_POINT('Ctrl Pts',(-1.91241996451229,-1.06847604194574,
3.07368996789426));
#43933=CARTESIAN_POINT('Ctrl Pts',(-1.8865072125481,-0.79477268400085,3.19333984045024));
#43934=CARTESIAN_POINT('Ctrl Pts',(-1.88064166515752,-0.636309800095194,
3.25489131573297));
#43935=CARTESIAN_POINT('Ctrl Pts',(-1.87760737563781,-0.319434907277157,
3.33380328845345));
#43936=CARTESIAN_POINT('Ctrl Pts',(-1.88074975802209,-0.158333333333332,
3.36074548314115));
#43937=CARTESIAN_POINT('Ctrl Pts',(-1.90100645273083,0.158333333333334,
3.37055545712555));
#43938=CARTESIAN_POINT('Ctrl Pts',(-1.91703990929339,0.319434907277168,
3.35292765819496));
#43939=CARTESIAN_POINT('Ctrl Pts',(-1.96353725276719,0.636309800095206,
3.29500735330529));
#43940=CARTESIAN_POINT('Ctrl Pts',(-1.99317440489421,0.794772684000836,
3.24479804609362));
#43941=CARTESIAN_POINT('Ctrl Pts',(-2.06134479848186,1.06847604194578,3.14565226416201));
#43942=CARTESIAN_POINT('Ctrl Pts',(-2.09551677023677,1.18514270861311,3.09637362817448));
#43943=CARTESIAN_POINT('Ctrl Pts',(-2.13435227632445,1.30000000000197,3.04073289148445));
#43944=CARTESIAN_POINT('Ctrl Pts',(-1.92692142534705,-1.30000000000181,
2.97161824960565));
#43945=CARTESIAN_POINT('Ctrl Pts',(-1.90386729002269,-1.18514270861301,
3.04116990549215));
#43946=CARTESIAN_POINT('Ctrl Pts',(-1.88627914618779,-1.06847604194574,
3.1030746797732));
#43947=CARTESIAN_POINT('Ctrl Pts',(-1.85827454924163,-0.794772684000848,
3.22842126610778));
#43948=CARTESIAN_POINT('Ctrl Pts',(-1.85546010955687,-0.636309800095197,
3.29049806719072));
#43949=CARTESIAN_POINT('Ctrl Pts',(-1.85388606537692,-0.31943490727716,
3.37048814797755));
#43950=CARTESIAN_POINT('Ctrl Pts',(-1.85855087100812,-0.158333333333332,
3.39623907172838));
#43951=CARTESIAN_POINT('Ctrl Pts',(-1.87792710232795,0.158333333333335,
3.40560369589062));
#43952=CARTESIAN_POINT('Ctrl Pts',(-1.89118745073622,0.319434907277167,
3.38857027282163));
#43953=CARTESIAN_POINT('Ctrl Pts',(-1.93518522291873,0.636309800095207,
3.32897340111308));
#43954=CARTESIAN_POINT('Ctrl Pts',(-1.96192720746975,0.794772684000843,
3.27822717572058));
#43955=CARTESIAN_POINT('Ctrl Pts',(-2.03215435767296,1.06847604194579,3.17319269348169));
#43956=CARTESIAN_POINT('Ctrl Pts',(-2.06847889453793,1.18514270861311,3.12033804137314));
#43957=CARTESIAN_POINT('Ctrl Pts',(-2.11072923711717,1.30000000000197,3.06009427260624));
#43958=CARTESIAN_POINT('Ctrl Pts',(-1.9148887376745,-1.30000000000181,2.98475844866592));
#43959=CARTESIAN_POINT('Ctrl Pts',(-1.88985290696311,-1.18514270861301,
3.05722651271223));
#43960=CARTESIAN_POINT('Ctrl Pts',(-1.87105265739054,-1.06847604194574,
3.12140222165167));
#43961=CARTESIAN_POINT('Ctrl Pts',(-1.84202575975531,-0.79477268400085,
3.25050394843119));
#43962=CARTESIAN_POINT('Ctrl Pts',(-1.84214725933546,-0.636309800095196,
3.31351072436173));
#43963=CARTESIAN_POINT('Ctrl Pts',(-1.84031348410914,-0.319434907277158,
3.39351117217984));
#43964=CARTESIAN_POINT('Ctrl Pts',(-1.84277573687377,-0.158333333333332,
3.41669588220879));
#43965=CARTESIAN_POINT('Ctrl Pts',(-1.8611725008453,0.158333333333335,3.42554170833206));
#43966=CARTESIAN_POINT('Ctrl Pts',(-1.87510093760627,0.319434907277169,
3.41028277821626));
#43967=CARTESIAN_POINT('Ctrl Pts',(-1.91849382563582,0.636309800095207,
3.35017470917515));
#43968=CARTESIAN_POINT('Ctrl Pts',(-1.94297883551598,0.794772684000839,
3.29878979088092));
#43969=CARTESIAN_POINT('Ctrl Pts',(-2.01463555477941,1.06847604194579,3.19013975303558));
#43970=CARTESIAN_POINT('Ctrl Pts',(-2.05239181690791,1.18514270861311,3.13509827737979));
#43971=CARTESIAN_POINT('Ctrl Pts',(-2.09688680253882,1.30000000000198,3.07204590157093));
#43972=CARTESIAN_POINT('Ctrl Pts',(-1.90476633611223,-1.30000000000181,
2.9955128759078));
#43973=CARTESIAN_POINT('Ctrl Pts',(-1.87892882368393,-1.18514270861301,
3.07063333458284));
#43974=CARTESIAN_POINT('Ctrl Pts',(-1.85938481786887,-1.06847604194574,
3.13665012918577));
#43975=CARTESIAN_POINT('Ctrl Pts',(-1.82877351395948,-0.794772684000852,
3.26813084614438));
#43976=CARTESIAN_POINT('Ctrl Pts',(-1.82777277121735,-0.636309800095196,
3.32985571507095));
#43977=CARTESIAN_POINT('Ctrl Pts',(-1.82519920803595,-0.319434907277158,
3.40946759971276));
#43978=CARTESIAN_POINT('Ctrl Pts',(-1.82786500157534,-0.158333333333332,
3.43168651366379));
#43979=CARTESIAN_POINT('Ctrl Pts',(-1.84675980907114,0.158333333333334,
3.44083983489165));
#43980=CARTESIAN_POINT('Ctrl Pts',(-1.8617377834321,0.319434907277168,3.42729831431622));
#43981=CARTESIAN_POINT('Ctrl Pts',(-1.90534698658927,0.636309800095207,
3.36730051672168));
#43982=CARTESIAN_POINT('Ctrl Pts',(-1.92818929679077,0.79477268400084,3.31562202142933));
#43983=CARTESIAN_POINT('Ctrl Pts',(-2.00107159200056,1.06847604194579,3.20434538599608));
#43984=CARTESIAN_POINT('Ctrl Pts',(-2.03992589311055,1.18514270861311,3.14763454428652));
#43985=CARTESIAN_POINT('Ctrl Pts',(-2.08608645028931,1.30000000000198,3.08238039314089));
#43986=CARTESIAN_POINT('Ctrl Pts',(-1.89326780681869,-1.30000000000181,
3.00896395652527));
#43987=CARTESIAN_POINT('Ctrl Pts',(-1.86630488495873,-1.18514270861301,
3.0876216818592));
#43988=CARTESIAN_POINT('Ctrl Pts',(-1.84556737380607,-1.06847604194574,
3.15603233359385));
#43989=CARTESIAN_POINT('Ctrl Pts',(-1.81204151864165,-0.794772684000851,
3.29040183467012));
#43990=CARTESIAN_POINT('Ctrl Pts',(-1.80838728385254,-0.636309800095196,
3.34998635143928));
#43991=CARTESIAN_POINT('Ctrl Pts',(-1.80384325729454,-0.319434907277158,
3.42867224736089));
#43992=CARTESIAN_POINT('Ctrl Pts',(-1.80676462972489,-0.158333333333332,
3.44958860602811));
#43993=CARTESIAN_POINT('Ctrl Pts',(-1.82555746981584,0.158333333333334,
3.45870878323941));
#43994=CARTESIAN_POINT('Ctrl Pts',(-1.84045866753833,0.319434907277167,
3.44661867877365));
#43995=CARTESIAN_POINT('Ctrl Pts',(-1.8852587262344,0.636309800095206,3.3871086271648));
#43996=CARTESIAN_POINT('Ctrl Pts',(-1.90913160377284,0.79477268400084,3.33661715000765));
#43997=CARTESIAN_POINT('Ctrl Pts',(-1.98479359038803,1.06847604194579,3.22231077812534));
#43998=CARTESIAN_POINT('Ctrl Pts',(-2.02514552074472,1.18514270861311,3.1633424593463));
#43999=CARTESIAN_POINT('Ctrl Pts',(-2.07309811100521,1.30000000000198,3.0948848147077));
#44000=CARTESIAN_POINT('Ctrl Pts',(-1.88533826855982,-1.30000000000181,
3.01806098483422));
#44001=CARTESIAN_POINT('Ctrl Pts',(-1.8587786442265,-1.18514270861301,3.09980889203863));
#44002=CARTESIAN_POINT('Ctrl Pts',(-1.83771824840901,-1.06847604194574,
3.17002999271618));
#44003=CARTESIAN_POINT('Ctrl Pts',(-1.80176883894142,-0.794772684000851,
3.30562555395723));
#44004=CARTESIAN_POINT('Ctrl Pts',(-1.79303694377367,-0.636309800095197,
3.36107920116882));
#44005=CARTESIAN_POINT('Ctrl Pts',(-1.78572104870416,-0.319434907277159,
3.43766535670148));
#44006=CARTESIAN_POINT('Ctrl Pts',(-1.78936170987159,-0.158333333333332,
3.45778637033323));
#44007=CARTESIAN_POINT('Ctrl Pts',(-1.8080248988652,0.158333333333334,3.4667877566422));
#44008=CARTESIAN_POINT('Ctrl Pts',(-1.82221963518582,0.319434907277167,
3.45538257525931));
#44009=CARTESIAN_POINT('Ctrl Pts',(-1.869237254135,0.636309800095206,3.39771324857652));
#44010=CARTESIAN_POINT('Ctrl Pts',(-1.89712646388558,0.79477268400084,3.35104670890408));
#44011=CARTESIAN_POINT('Ctrl Pts',(-1.97527792161989,1.06847604194579,3.23554112305398));
#44012=CARTESIAN_POINT('Ctrl Pts',(-2.01625666953888,1.18514270861311,3.1748648984291));
#44013=CARTESIAN_POINT('Ctrl Pts',(-2.06438529512048,1.30000000000198,3.10351053739022));
#44014=CARTESIAN_POINT('Ctrl Pts',(-1.87799128879426,-1.30000000000181,
3.02253507588625));
#44015=CARTESIAN_POINT('Ctrl Pts',(-1.85162982048175,-1.18514270861301,
3.10412841772033));
#44016=CARTESIAN_POINT('Ctrl Pts',(-1.83046672246869,-1.06847604194574,
3.17402030998991));
#44017=CARTESIAN_POINT('Ctrl Pts',(-1.79358500771746,-0.794772684000851,
3.30845187359642));
#44018=CARTESIAN_POINT('Ctrl Pts',(-1.78288365918825,-0.636309800095197,
3.36226104014369));
#44019=CARTESIAN_POINT('Ctrl Pts',(-1.77431562872861,-0.319434907277159,
3.43771727806328));
#44020=CARTESIAN_POINT('Ctrl Pts',(-1.77794490963746,-0.158333333333332,
3.4578893860418));
#44021=CARTESIAN_POINT('Ctrl Pts',(-1.79644754730033,0.158333333333334,
3.46671667358385));
#44022=CARTESIAN_POINT('Ctrl Pts',(-1.8102831109525,0.319434907277167,3.45490100101633));
#44023=CARTESIAN_POINT('Ctrl Pts',(-1.85865359192218,0.636309800095206,
3.39838440412251));
#44024=CARTESIAN_POINT('Ctrl Pts',(-1.8893645694356,0.79477268400084,3.35403177699279));
#44025=CARTESIAN_POINT('Ctrl Pts',(-1.96832072991261,1.06847604194579,3.23960467551191));
#44026=CARTESIAN_POINT('Ctrl Pts',(-2.00914338193045,1.18514270861311,3.17906956425754));
#44027=CARTESIAN_POINT('Ctrl Pts',(-2.05661148970959,1.30000000000198,3.10753059403805));
#44028=CARTESIAN_POINT('Ctrl Pts',(-1.87799128879384,-1.3,3.02253507588753));
#44029=CARTESIAN_POINT('Ctrl Pts',(-1.85162982048153,-1.18514270861178,
3.10412841772107));
#44030=CARTESIAN_POINT('Ctrl Pts',(-1.8304667224686,-1.06847604194512,3.17402030999021));
#44031=CARTESIAN_POINT('Ctrl Pts',(-1.79358500771746,-0.794772684000851,
3.30845187359642));
#44032=CARTESIAN_POINT('Ctrl Pts',(-1.78288365918825,-0.636309800095197,
3.36226104014369));
#44033=CARTESIAN_POINT('Ctrl Pts',(-1.77431562872862,-0.319434907277159,
3.43771727806328));
#44034=CARTESIAN_POINT('Ctrl Pts',(-1.77794490963746,-0.158333333333332,
3.45788938604181));
#44035=CARTESIAN_POINT('Ctrl Pts',(-1.79644754730033,0.158333333333334,
3.46671667358385));
#44036=CARTESIAN_POINT('Ctrl Pts',(-1.8102831109525,0.319434907277167,3.45490100101633));
#44037=CARTESIAN_POINT('Ctrl Pts',(-1.85865359192218,0.636309800095206,
3.39838440412251));
#44038=CARTESIAN_POINT('Ctrl Pts',(-1.8893645694356,0.79477268400084,3.35403177699279));
#44039=CARTESIAN_POINT('Ctrl Pts',(-1.96832072991242,1.06847604194511,3.23960467551219));
#44040=CARTESIAN_POINT('Ctrl Pts',(-2.00914338192998,1.18514270861178,3.17906956425824));
#44041=CARTESIAN_POINT('Ctrl Pts',(-2.05661148970878,1.3,3.10753059403928));
#44042=CARTESIAN_POINT('',(-2.20676493717361,-1.2,2.76912102263432));
#44043=CARTESIAN_POINT('Ctrl Pts',(-2.20676493717361,-1.2,2.76912102263432));
#44044=CARTESIAN_POINT('Ctrl Pts',(-2.18959342499164,-1.21474920900201,
2.77704610786863));
#44045=CARTESIAN_POINT('Ctrl Pts',(-2.18825900990267,-1.21544842993642,
2.77717319380777));
#44046=CARTESIAN_POINT('Ctrl Pts',(-2.16536120078355,-1.23449324006335,
2.78712413918319));
#44047=CARTESIAN_POINT('Ctrl Pts',(-2.16384270892882,-1.23586773324202,
2.78790177160257));
#44048=CARTESIAN_POINT('Ctrl Pts',(-2.12798513336799,-1.26665429549693,
2.80466996299418));
#44049=CARTESIAN_POINT('Ctrl Pts',(-2.11236536519738,-1.2798581653664,2.81178284923323));
#44050=CARTESIAN_POINT('Ctrl Pts',(-2.08925763079311,-1.30000000000178,
2.82307156191063));
#44051=CARTESIAN_POINT('',(-2.3458424267643,-0.653834841421144,2.84115573706238));
#44052=CARTESIAN_POINT('Ctrl Pts',(-2.34584242677385,-0.653834841420469,
2.84115573703903));
#44053=CARTESIAN_POINT('Ctrl Pts',(-2.33125630278765,-0.719118562165429,
2.83330577809928));
#44054=CARTESIAN_POINT('Ctrl Pts',(-2.31992974450258,-0.763459406308881,
2.82727725267908));
#44055=CARTESIAN_POINT('Ctrl Pts',(-2.27425749731053,-0.94963865469992,
2.80324291065325));
#44056=CARTESIAN_POINT('Ctrl Pts',(-2.24776174106812,-1.05261022998892,
2.78953916310548));
#44057=CARTESIAN_POINT('Ctrl Pts',(-2.20676493717361,-1.2,2.76912102263432));
#44058=CARTESIAN_POINT('',(-2.46774460503139,0.653834841531101,2.90899352548397));
#44059=CARTESIAN_POINT('Ctrl Pts',(-2.46774460503139,0.6538348415311,2.90899352548397));
#44060=CARTESIAN_POINT('Ctrl Pts',(-2.43367455207709,0.575764716732145,
2.93301788730227));
#44061=CARTESIAN_POINT('Ctrl Pts',(-2.40473079536294,0.49386600743549,2.95258260670437));
#44062=CARTESIAN_POINT('Ctrl Pts',(-2.3613241452078,0.338182309445636,2.97879498027382));
#44063=CARTESIAN_POINT('Ctrl Pts',(-2.34534839465029,0.26570061668282,2.98694809138619));
#44064=CARTESIAN_POINT('Ctrl Pts',(-2.32198141046681,0.129734501997336,
2.99409093181665));
#44065=CARTESIAN_POINT('Ctrl Pts',(-2.3137066916505,0.0666508202182009,
2.99426128761355));
#44066=CARTESIAN_POINT('Ctrl Pts',(-2.30187610082096,-0.0595255417580441,
2.98810497259799));
#44067=CARTESIAN_POINT('Ctrl Pts',(-2.29822356580874,-0.122765063402191,
2.98174712248733));
#44068=CARTESIAN_POINT('Ctrl Pts',(-2.29616337797591,-0.260131979528658,
2.96113524134179));
#44069=CARTESIAN_POINT('Ctrl Pts',(-2.29882503835795,-0.333936745811711,
2.94565054396205));
#44070=CARTESIAN_POINT('Ctrl Pts',(-2.31352704947006,-0.49110863627357,
2.90332005827053));
#44071=CARTESIAN_POINT('Ctrl Pts',(-2.32698048328179,-0.574253237247853,
2.87477504935862));
#44072=CARTESIAN_POINT('Ctrl Pts',(-2.34584242672574,-0.65383484143241,
2.84115573706742));
#44073=CARTESIAN_POINT('',(-2.40496089006672,1.2,2.8734929657691));
#44074=CARTESIAN_POINT('Ctrl Pts',(-2.40496089006672,1.2,2.8734929657691));
#44075=CARTESIAN_POINT('Ctrl Pts',(-2.41287040100767,1.15218563167953,2.87788959897044));
#44076=CARTESIAN_POINT('Ctrl Pts',(-2.42731667097231,1.06332654423114,2.88594041030948));
#44077=CARTESIAN_POINT('Ctrl Pts',(-2.45656691359185,0.804836252522856,
2.90256835751397));
#44078=CARTESIAN_POINT('Ctrl Pts',(-2.46205856622822,0.741545664188083,
2.90572350208414));
#44079=CARTESIAN_POINT('Ctrl Pts',(-2.46774460503139,0.653834841531101,
2.90899352548397));
#44080=CARTESIAN_POINT('Ctrl Pts',(-2.29120499224679,1.30000000000195,2.92532110171016));
#44081=CARTESIAN_POINT('Ctrl Pts',(-2.29212457406799,1.29919343636464,2.92489887509983));
#44082=CARTESIAN_POINT('Ctrl Pts',(-2.29304015951971,1.29838659872316,2.92447432719573));
#44083=CARTESIAN_POINT('Ctrl Pts',(-2.31180419504521,1.28165454130476,2.91555298390577));
#44084=CARTESIAN_POINT('Ctrl Pts',(-2.3297873229645,1.26578478037346,2.90724018576387));
#44085=CARTESIAN_POINT('Ctrl Pts',(-2.35953440176376,1.23935794201536,2.89336991066159));
#44086=CARTESIAN_POINT('Ctrl Pts',(-2.38221727164868,1.21902715818375,2.88261970932993));
#44087=CARTESIAN_POINT('Ctrl Pts',(-2.40496089006672,1.2,2.8734929657691));
#44088=CARTESIAN_POINT('Ctrl Pts',(-1.87799128879384,-1.3,3.02253507588753));
#44089=CARTESIAN_POINT('Ctrl Pts',(-1.85162982048153,-1.18514270861178,
3.10412841772107));
#44090=CARTESIAN_POINT('Ctrl Pts',(-1.8304667224686,-1.06847604194512,3.17402030999022));
#44091=CARTESIAN_POINT('Ctrl Pts',(-1.79358500771746,-0.794772684000851,
3.30845187359642));
#44092=CARTESIAN_POINT('Ctrl Pts',(-1.78288365918825,-0.636309800095196,
3.36226104014369));
#44093=CARTESIAN_POINT('Ctrl Pts',(-1.77431562872861,-0.319434907277159,
3.43771727806328));
#44094=CARTESIAN_POINT('Ctrl Pts',(-1.77794490963746,-0.158333333333332,
3.4578893860418));
#44095=CARTESIAN_POINT('Ctrl Pts',(-1.79644754730033,0.158333333333335,
3.46671667358385));
#44096=CARTESIAN_POINT('Ctrl Pts',(-1.8102831109525,0.319434907277167,3.45490100101633));
#44097=CARTESIAN_POINT('Ctrl Pts',(-1.85865359192218,0.636309800095206,
3.39838440412251));
#44098=CARTESIAN_POINT('Ctrl Pts',(-1.8893645694356,0.79477268400084,3.35403177699279));
#44099=CARTESIAN_POINT('Ctrl Pts',(-1.96832072991242,1.06847604194511,3.23960467551219));
#44100=CARTESIAN_POINT('Ctrl Pts',(-2.00914338192998,1.18514270861178,3.17906956425824));
#44101=CARTESIAN_POINT('Ctrl Pts',(-2.05661148970878,1.3,3.10753059403928));
#44102=CARTESIAN_POINT('Ctrl Pts',(-1.80704611563284,-1.3,2.99277114335502));
#44103=CARTESIAN_POINT('Ctrl Pts',(-1.78233798615881,-1.18514270861178,
3.07488156897468));
#44104=CARTESIAN_POINT('Ctrl Pts',(-1.76233903122006,-1.06847604194512,
3.14509050992361));
#44105=CARTESIAN_POINT('Ctrl Pts',(-1.72701657977794,-0.794772684000851,
3.27979239829291));
#44106=CARTESIAN_POINT('Ctrl Pts',(-1.71574542397768,-0.636309800095196,
3.33316531076088));
#44107=CARTESIAN_POINT('Ctrl Pts',(-1.70682212124655,-0.319434907277159,
3.4080572218364));
#44108=CARTESIAN_POINT('Ctrl Pts',(-1.70940065624172,-0.158333333333332,
3.42756797905052));
#44109=CARTESIAN_POINT('Ctrl Pts',(-1.72804929275646,0.158333333333335,
3.43606734780233));
#44110=CARTESIAN_POINT('Ctrl Pts',(-1.74307942205737,0.319434907277167,
3.42459000158545));
#44111=CARTESIAN_POINT('Ctrl Pts',(-1.79210700315155,0.636309800095206,
3.36795981507847));
#44112=CARTESIAN_POINT('Ctrl Pts',(-1.82352345611137,0.79477268400084,3.32373872631714));
#44113=CARTESIAN_POINT('Ctrl Pts',(-1.90123537533585,1.06847604194511,3.20833374894953));
#44114=CARTESIAN_POINT('Ctrl Pts',(-1.9410434505065,1.18514270861178,3.14714565776922));
#44115=CARTESIAN_POINT('Ctrl Pts',(-1.98702099052592,1.3,3.07472401393519));
#44116=CARTESIAN_POINT('Ctrl Pts',(-1.73610094247183,-1.3,2.96300721082251));
#44117=CARTESIAN_POINT('Ctrl Pts',(-1.71304615183608,-1.18514270861178,
3.0456347202283));
#44118=CARTESIAN_POINT('Ctrl Pts',(-1.69421133997151,-1.06847604194512,
3.11616070985699));
#44119=CARTESIAN_POINT('Ctrl Pts',(-1.66044815183843,-0.794772684000851,
3.2511329229894));
#44120=CARTESIAN_POINT('Ctrl Pts',(-1.64860718876712,-0.636309800095196,
3.30406958137807));
#44121=CARTESIAN_POINT('Ctrl Pts',(-1.63932861376449,-0.319434907277159,
3.37839716560952));
#44122=CARTESIAN_POINT('Ctrl Pts',(-1.64085640284598,-0.158333333333332,
3.39724657205923));
#44123=CARTESIAN_POINT('Ctrl Pts',(-1.65965103821258,0.158333333333335,
3.4054180220208));
#44124=CARTESIAN_POINT('Ctrl Pts',(-1.67587573316224,0.319434907277167,
3.39427900215456));
#44125=CARTESIAN_POINT('Ctrl Pts',(-1.72556041438091,0.636309800095206,
3.33753522603443));
#44126=CARTESIAN_POINT('Ctrl Pts',(-1.75768234278715,0.79477268400084,3.29344567564149));
#44127=CARTESIAN_POINT('Ctrl Pts',(-1.83415002075929,1.06847604194511,3.17706282238686));
#44128=CARTESIAN_POINT('Ctrl Pts',(-1.87294351908302,1.18514270861178,3.11522175128021));
#44129=CARTESIAN_POINT('Ctrl Pts',(-1.91743049134307,1.3,3.04191743383109));
#44130=CARTESIAN_POINT('Ctrl Pts',(-1.66515576931082,-1.3,2.93324327829));
#44131=CARTESIAN_POINT('Ctrl Pts',(-1.64375431751336,-1.18514270861178,
3.01638787148191));
#44132=CARTESIAN_POINT('Ctrl Pts',(-1.62608364872297,-1.06847604194512,
3.08723090979038));
#44133=CARTESIAN_POINT('Ctrl Pts',(-1.59387972389892,-0.794772684000851,
3.22247344768588));
#44134=CARTESIAN_POINT('Ctrl Pts',(-1.58146895355655,-0.636309800095196,
3.27497385199526));
#44135=CARTESIAN_POINT('Ctrl Pts',(-1.57183510628243,-0.319434907277159,
3.34873710938264));
#44136=CARTESIAN_POINT('Ctrl Pts',(-1.57231214945024,-0.158333333333332,
3.36692516506794));
#44137=CARTESIAN_POINT('Ctrl Pts',(-1.5912527836687,0.158333333333335,3.37476869623928));
#44138=CARTESIAN_POINT('Ctrl Pts',(-1.6086720442671,0.319434907277167,3.36396800272368));
#44139=CARTESIAN_POINT('Ctrl Pts',(-1.65901382561028,0.636309800095206,
3.30711063699039));
#44140=CARTESIAN_POINT('Ctrl Pts',(-1.69184122946292,0.79477268400084,3.26315262496584));
#44141=CARTESIAN_POINT('Ctrl Pts',(-1.76706466618272,1.06847604194511,3.1457918958242));
#44142=CARTESIAN_POINT('Ctrl Pts',(-1.80484358765954,1.18514270861178,3.08329784479119));
#44143=CARTESIAN_POINT('Ctrl Pts',(-1.84783999216022,1.3,3.00911085372699));
#44144=CARTESIAN_POINT('Ctrl Pts',(-1.66515576931082,-1.3,2.93324327829));
#44145=CARTESIAN_POINT('Ctrl Pts',(-1.64375431751336,-1.18514270861178,
3.01638787148191));
#44146=CARTESIAN_POINT('Ctrl Pts',(-1.62608364872297,-1.06847604194512,
3.08723090979038));
#44147=CARTESIAN_POINT('Ctrl Pts',(-1.59387972389891,-0.794772684000851,
3.22247344768589));
#44148=CARTESIAN_POINT('Ctrl Pts',(-1.58146895355655,-0.636309800095197,
3.27497385199526));
#44149=CARTESIAN_POINT('Ctrl Pts',(-1.57183510628243,-0.319434907277159,
3.34873710938264));
#44150=CARTESIAN_POINT('Ctrl Pts',(-1.57231214945024,-0.158333333333332,
3.36692516506795));
#44151=CARTESIAN_POINT('Ctrl Pts',(-1.5912527836687,0.158333333333334,3.37476869623928));
#44152=CARTESIAN_POINT('Ctrl Pts',(-1.6086720442671,0.319434907277167,3.36396800272368));
#44153=CARTESIAN_POINT('Ctrl Pts',(-1.65901382561028,0.636309800095206,
3.30711063699039));
#44154=CARTESIAN_POINT('Ctrl Pts',(-1.69184122946292,0.79477268400084,3.26315262496584));
#44155=CARTESIAN_POINT('Ctrl Pts',(-1.76706466618272,1.06847604194511,3.1457918958242));
#44156=CARTESIAN_POINT('Ctrl Pts',(-1.80484358765954,1.18514270861178,3.08329784479119));
#44157=CARTESIAN_POINT('Ctrl Pts',(-1.84783999216021,1.3,3.00911085372699));
#44158=CARTESIAN_POINT('Ctrl Pts',(-1.6651557693112,-1.30000000000205,2.93324327828851));
#44159=CARTESIAN_POINT('Ctrl Pts',(-1.64375431751357,-1.18514270861317,
3.01638787148107));
#44160=CARTESIAN_POINT('Ctrl Pts',(-1.62608364872305,-1.06847604194582,
3.08723090979004));
#44161=CARTESIAN_POINT('Ctrl Pts',(-1.59387972389891,-0.794772684000851,
3.22247344768589));
#44162=CARTESIAN_POINT('Ctrl Pts',(-1.58146895355655,-0.636309800095197,
3.27497385199526));
#44163=CARTESIAN_POINT('Ctrl Pts',(-1.57183510628243,-0.319434907277159,
3.34873710938264));
#44164=CARTESIAN_POINT('Ctrl Pts',(-1.57231214945024,-0.158333333333332,
3.36692516506795));
#44165=CARTESIAN_POINT('Ctrl Pts',(-1.5912527836687,0.158333333333334,3.37476869623928));
#44166=CARTESIAN_POINT('Ctrl Pts',(-1.6086720442671,0.319434907277167,3.36396800272368));
#44167=CARTESIAN_POINT('Ctrl Pts',(-1.65901382561028,0.636309800095206,
3.30711063699039));
#44168=CARTESIAN_POINT('Ctrl Pts',(-1.69184122946292,0.79477268400084,3.26315262496584));
#44169=CARTESIAN_POINT('Ctrl Pts',(-1.76706466618285,1.06847604194558,3.145791895824));
#44170=CARTESIAN_POINT('Ctrl Pts',(-1.80484358765984,1.1851427086127,3.0832978447907));
#44171=CARTESIAN_POINT('Ctrl Pts',(-1.84783999216072,1.30000000000136,3.00911085372612));
#44172=CARTESIAN_POINT('Ctrl Pts',(-1.66294156245583,-1.30000000000205,
2.92477627213571));
#44173=CARTESIAN_POINT('Ctrl Pts',(-1.64211927469575,-1.18514270861317,
3.00828819805516));
#44174=CARTESIAN_POINT('Ctrl Pts',(-1.62444818678095,-1.06847604194582,
3.07934166149543));
#44175=CARTESIAN_POINT('Ctrl Pts',(-1.59090434064678,-0.794772684000851,
3.21470783560491));
#44176=CARTESIAN_POINT('Ctrl Pts',(-1.57488586700129,-0.636309800095197,
3.26665956749681));
#44177=CARTESIAN_POINT('Ctrl Pts',(-1.56349013315575,-0.319434907277159,
3.34018877927888));
#44178=CARTESIAN_POINT('Ctrl Pts',(-1.56451256412486,-0.158333333333332,
3.35836908011497));
#44179=CARTESIAN_POINT('Ctrl Pts',(-1.5836900087521,0.158333333333334,3.3662154293602));
#44180=CARTESIAN_POINT('Ctrl Pts',(-1.60107891375656,0.319434907277167,
3.35545738175593));
#44181=CARTESIAN_POINT('Ctrl Pts',(-1.65309822965177,0.636309800095206,
3.29877447147387));
#44182=CARTESIAN_POINT('Ctrl Pts',(-1.6884655423189,0.79477268400084,3.25517967618859));
#44183=CARTESIAN_POINT('Ctrl Pts',(-1.7651778318562,1.06847604194558,3.13773291845356));
#44184=CARTESIAN_POINT('Ctrl Pts',(-1.80327012403915,1.1851427086127,3.07509490660645));
#44185=CARTESIAN_POINT('Ctrl Pts',(-1.84624880073476,1.30000000000136,3.00065723250455));
#44186=CARTESIAN_POINT('Ctrl Pts',(-1.6634305875893,-1.30000000000205,2.91253818382459));
#44187=CARTESIAN_POINT('Ctrl Pts',(-1.64459250993632,-1.18514270861317,
2.99401342938536));
#44188=CARTESIAN_POINT('Ctrl Pts',(-1.62774351228504,-1.06847604194582,
3.06348347679413));
#44189=CARTESIAN_POINT('Ctrl Pts',(-1.59341412979825,-0.794772684000852,
3.19623877438057));
#44190=CARTESIAN_POINT('Ctrl Pts',(-1.57193522590822,-0.636309800095198,
3.24776859715612));
#44191=CARTESIAN_POINT('Ctrl Pts',(-1.5577591921755,-0.31943490727716,3.32089454575369));
#44192=CARTESIAN_POINT('Ctrl Pts',(-1.55879969010269,-0.158333333333332,
3.34004933420448));
#44193=CARTESIAN_POINT('Ctrl Pts',(-1.5782014042107,0.158333333333335,3.34793016181554));
#44194=CARTESIAN_POINT('Ctrl Pts',(-1.59575204221966,0.319434907277167,
3.33615308111097));
#44195=CARTESIAN_POINT('Ctrl Pts',(-1.65109905999309,0.636309800095207,
3.28010462985753));
#44196=CARTESIAN_POINT('Ctrl Pts',(-1.69266556144995,0.794772684000843,
3.23744188421739));
#44197=CARTESIAN_POINT('Ctrl Pts',(-1.77009640342744,1.06847604194558,3.12257100392356));
#44198=CARTESIAN_POINT('Ctrl Pts',(-1.80712529462456,1.1851427086127,3.06137163709183));
#44199=CARTESIAN_POINT('Ctrl Pts',(-1.84766613462215,1.30000000000136,2.98869625112208));
#44200=CARTESIAN_POINT('Ctrl Pts',(-1.66409924349422,-1.30000000000205,
2.89751233934654));
#44201=CARTESIAN_POINT('Ctrl Pts',(-1.64632958993895,-1.18514270861317,
2.97603885688088));
#44202=CARTESIAN_POINT('Ctrl Pts',(-1.63008699942642,-1.06847604194582,
3.0432812599093));
#44203=CARTESIAN_POINT('Ctrl Pts',(-1.59609118714013,-0.794772684000853,
3.17255610081311));
#44204=CARTESIAN_POINT('Ctrl Pts',(-1.57317224543321,-0.636309800095198,
3.22410152369958));
#44205=CARTESIAN_POINT('Ctrl Pts',(-1.55789432690329,-0.31943490727716,
3.2967365657438));
#44206=CARTESIAN_POINT('Ctrl Pts',(-1.55797756487196,-0.158333333333332,
3.31675875423184));
#44207=CARTESIAN_POINT('Ctrl Pts',(-1.57736992673725,0.158333333333335,
3.32465368269152));
#44208=CARTESIAN_POINT('Ctrl Pts',(-1.59551109084602,0.319434907277167,
3.31191728904508));
#44209=CARTESIAN_POINT('Ctrl Pts',(-1.65266890419111,0.636309800095207,
3.25660440914048));
#44210=CARTESIAN_POINT('Ctrl Pts',(-1.69746082551081,0.794772684000843,
3.2145123098584));
#44211=CARTESIAN_POINT('Ctrl Pts',(-1.77471532910312,1.06847604194558,3.10313038179039));
#44212=CARTESIAN_POINT('Ctrl Pts',(-1.81082374324295,1.1851427086127,3.04402618572621));
#44213=CARTESIAN_POINT('Ctrl Pts',(-1.84959995947889,1.30000000000136,2.97403090315142));
#44214=CARTESIAN_POINT('Ctrl Pts',(-1.66413304228575,-1.30000000000205,
2.88855088157018));
#44215=CARTESIAN_POINT('Ctrl Pts',(-1.64663626767473,-1.18514270861317,
2.96549279537844));
#44216=CARTESIAN_POINT('Ctrl Pts',(-1.63063860211263,-1.06847604194582,
3.03158626229152));
#44217=CARTESIAN_POINT('Ctrl Pts',(-1.59714403614094,-0.794772684000851,
3.15921331026086));
#44218=CARTESIAN_POINT('Ctrl Pts',(-1.57468838437964,-0.636309800095196,
3.21118033024189));
#44219=CARTESIAN_POINT('Ctrl Pts',(-1.55933444655545,-0.319434907277159,
3.2837230199588));
#44220=CARTESIAN_POINT('Ctrl Pts',(-1.55861332258574,-0.158333333333332,
3.3040487115858));
#44221=CARTESIAN_POINT('Ctrl Pts',(-1.57793062519727,0.158333333333334,
3.31193446863975));
#44222=CARTESIAN_POINT('Ctrl Pts',(-1.59655517071776,0.319434907277167,
3.29881934722603));
#44223=CARTESIAN_POINT('Ctrl Pts',(-1.6541370369876,0.636309800095206,3.24371468381404));
#44224=CARTESIAN_POINT('Ctrl Pts',(-1.69949833972927,0.79477268400084,3.20151300621913));
#44225=CARTESIAN_POINT('Ctrl Pts',(-1.77645424648232,1.06847604194558,3.09181239223893));
#44226=CARTESIAN_POINT('Ctrl Pts',(-1.81221516246302,1.1851427086127,3.03380698464707));
#44227=CARTESIAN_POINT('Ctrl Pts',(-1.85042563388831,1.30000000000136,2.96528150044712));
#44228=CARTESIAN_POINT('Ctrl Pts',(-1.66445586874822,-1.30000000000205,
2.87650429183539));
#44229=CARTESIAN_POINT('Ctrl Pts',(-1.64746654614293,-1.18514270861317,
2.9511617041883));
#44230=CARTESIAN_POINT('Ctrl Pts',(-1.63193905490586,-1.06847604194582,
3.01562362169735));
#44231=CARTESIAN_POINT('Ctrl Pts',(-1.59944456678331,-0.79477268400085,
3.14098991401421));
#44232=CARTESIAN_POINT('Ctrl Pts',(-1.57799348539188,-0.636309800095196,
3.19378108820808));
#44233=CARTESIAN_POINT('Ctrl Pts',(-1.56251739556673,-0.319434907277159,
3.26627299656452));
#44234=CARTESIAN_POINT('Ctrl Pts',(-1.56021766016936,-0.158333333333332,
3.2869567263082));
#44235=CARTESIAN_POINT('Ctrl Pts',(-1.579297386822,0.158333333333334,3.29478244210874));
#44236=CARTESIAN_POINT('Ctrl Pts',(-1.59876559119614,0.319434907277167,
3.28109624173003));
#44237=CARTESIAN_POINT('Ctrl Pts',(-1.65699880469742,0.636309800095206,
3.22623170912691));
#44238=CARTESIAN_POINT('Ctrl Pts',(-1.70337675684885,0.794772684000841,
3.18387226395826));
#44239=CARTESIAN_POINT('Ctrl Pts',(-1.77954758974758,1.06847604194558,3.07646752958768));
#44240=CARTESIAN_POINT('Ctrl Pts',(-1.81453396341162,1.1851427086127,3.01996849556075));
#44241=CARTESIAN_POINT('Ctrl Pts',(-1.8515351795853,1.30000000000136,2.95346195727836));
#44242=CARTESIAN_POINT('Ctrl Pts',(-1.6643498478883,-1.30000000000205,2.86438665854125));
#44243=CARTESIAN_POINT('Ctrl Pts',(-1.64770189067232,-1.18514270861317,
2.93671789636582));
#44244=CARTESIAN_POINT('Ctrl Pts',(-1.63257569066065,-1.06847604194582,
2.99951947166058));
#44245=CARTESIAN_POINT('Ctrl Pts',(-1.60114670621631,-0.794772684000852,
3.12258824715685));
#44246=CARTESIAN_POINT('Ctrl Pts',(-1.58096527207976,-0.636309800095197,
3.17617757885722));
#44247=CARTESIAN_POINT('Ctrl Pts',(-1.56597543955806,-0.319434907277159,
3.24871816508311));
#44248=CARTESIAN_POINT('Ctrl Pts',(-1.5625222458354,-0.158333333333332,
3.26983928041926));
#44249=CARTESIAN_POINT('Ctrl Pts',(-1.58229897393715,0.158333333333335,
3.27791706510464));
#44250=CARTESIAN_POINT('Ctrl Pts',(-1.60405941583045,0.319434907277167,
3.26421397218699));
#44251=CARTESIAN_POINT('Ctrl Pts',(-1.66232624433739,0.636309800095206,
3.2094711399786));
#44252=CARTESIAN_POINT('Ctrl Pts',(-1.70674106971239,0.794772684000841,
3.16603757837));
#44253=CARTESIAN_POINT('Ctrl Pts',(-1.7814897873636,1.06847604194558,3.06076487540826));
#44254=CARTESIAN_POINT('Ctrl Pts',(-1.81592523135305,1.1851427086127,3.00585484616171));
#44255=CARTESIAN_POINT('Ctrl Pts',(-1.85244016917363,1.30000000000136,2.94160344004275));
#44256=CARTESIAN_POINT('Ctrl Pts',(-1.6631939573514,-1.30000000000205,2.84901103609872));
#44257=CARTESIAN_POINT('Ctrl Pts',(-1.64705706006683,-1.18514270861317,
2.9185030775211));
#44258=CARTESIAN_POINT('Ctrl Pts',(-1.63254236060157,-1.06847604194582,
2.97929848142592));
#44259=CARTESIAN_POINT('Ctrl Pts',(-1.60275810266336,-0.794772684000852,
3.09965705410264));
#44260=CARTESIAN_POINT('Ctrl Pts',(-1.58418289260517,-0.636309800095198,
3.15426789047404));
#44261=CARTESIAN_POINT('Ctrl Pts',(-1.57071860895688,-0.31943490727716,
3.22719026526377));
#44262=CARTESIAN_POINT('Ctrl Pts',(-1.56750832525203,-0.158333333333333,
3.24939746337031));
#44263=CARTESIAN_POINT('Ctrl Pts',(-1.58796133864451,0.158333333333335,
3.25773482052459));
#44264=CARTESIAN_POINT('Ctrl Pts',(-1.61042546287198,0.319434907277168,
3.24333833946108));
#44265=CARTESIAN_POINT('Ctrl Pts',(-1.66799369092752,0.636309800095208,
3.18847128887226));
#44266=CARTESIAN_POINT('Ctrl Pts',(-1.71065823061011,0.794772684000842,
3.14386957635525));
#44267=CARTESIAN_POINT('Ctrl Pts',(-1.78396337875779,1.06847604194558,3.04127089324132));
#44268=CARTESIAN_POINT('Ctrl Pts',(-1.81786493103005,1.1851427086127,2.98834641861744));
#44269=CARTESIAN_POINT('Ctrl Pts',(-1.85393695316482,1.30000000000136,2.92690863763393));
#44270=CARTESIAN_POINT('Ctrl Pts',(-1.66287285385524,-1.30000000000205,
2.83684381205742));
#44271=CARTESIAN_POINT('Ctrl Pts',(-1.64725497954519,-1.18514270861317,
2.90406038665813));
#44272=CARTESIAN_POINT('Ctrl Pts',(-1.63324137758571,-1.06847604194582,
2.96322801795107));
#44273=CARTESIAN_POINT('Ctrl Pts',(-1.60457334371134,-0.794772684000851,
3.08132241345498));
#44274=CARTESIAN_POINT('Ctrl Pts',(-1.58670059956992,-0.636309800095199,
3.13658864538851));
#44275=CARTESIAN_POINT('Ctrl Pts',(-1.57416217922139,-0.319434907277161,
3.20973093233505));
#44276=CARTESIAN_POINT('Ctrl Pts',(-1.57145871032908,-0.158333333333333,
3.23293006393472));
#44277=CARTESIAN_POINT('Ctrl Pts',(-1.59198547972842,0.158333333333335,
3.24130131732167));
#44278=CARTESIAN_POINT('Ctrl Pts',(-1.61389591587228,0.319434907277167,
3.2259155780679));
#44279=CARTESIAN_POINT('Ctrl Pts',(-1.67093422945697,0.636309800095208,
3.17096125429362));
#44280=CARTESIAN_POINT('Ctrl Pts',(-1.71365199342114,0.794772684000845,
3.12595232475909));
#44281=CARTESIAN_POINT('Ctrl Pts',(-1.78590535661653,1.06847604194558,3.02559590726589));
#44282=CARTESIAN_POINT('Ctrl Pts',(-1.81916201847011,1.1851427086127,2.97422359191595));
#44283=CARTESIAN_POINT('Ctrl Pts',(-1.85439953850088,1.30000000000137,2.91491953577721));
#44284=CARTESIAN_POINT('Ctrl Pts',(-1.66271526553442,-1.30000000000205,
2.81567174026498));
#44285=CARTESIAN_POINT('Ctrl Pts',(-1.64733326715726,-1.18514270861317,
2.87877836473091));
#44286=CARTESIAN_POINT('Ctrl Pts',(-1.63372876473195,-1.06847604194582,
2.93500590630431));
#44287=CARTESIAN_POINT('Ctrl Pts',(-1.60640601379383,-0.794772684000853,
3.04901071798214));
#44288=CARTESIAN_POINT('Ctrl Pts',(-1.59014548366958,-0.636309800095198,
3.10548900822069));
#44289=CARTESIAN_POINT('Ctrl Pts',(-1.57918993708349,-0.31943490727716,
3.17897283262899));
#44290=CARTESIAN_POINT('Ctrl Pts',(-1.57682954384601,-0.158333333333333,
3.20368408591858));
#44291=CARTESIAN_POINT('Ctrl Pts',(-1.59835814895341,0.158333333333335,
3.21240825833507));
#44292=CARTESIAN_POINT('Ctrl Pts',(-1.62159262469254,0.319434907277169,
3.19611224149114));
#44293=CARTESIAN_POINT('Ctrl Pts',(-1.67773360519212,0.636309800095209,
3.14102820846237));
#44294=CARTESIAN_POINT('Ctrl Pts',(-1.71775765489709,0.794772684000843,
3.09437447173804));
#44295=CARTESIAN_POINT('Ctrl Pts',(-1.78801951448282,1.06847604194558,2.99783516422076));
#44296=CARTESIAN_POINT('Ctrl Pts',(-1.82058725945667,1.1851427086127,2.94928807339681));
#44297=CARTESIAN_POINT('Ctrl Pts',(-1.85530899384812,1.30000000000136,2.89398218083932));
#44298=CARTESIAN_POINT('Ctrl Pts',(-1.65979832631176,-1.30000000000206,
2.78782357681252));
#44299=CARTESIAN_POINT('Ctrl Pts',(-1.64451139891587,-1.18514270861318,
2.84560432644518));
#44300=CARTESIAN_POINT('Ctrl Pts',(-1.63145107469241,-1.06847604194583,
2.89805914319504));
#44301=CARTESIAN_POINT('Ctrl Pts',(-1.60642301178616,-0.794772684000855,
3.00693629302853));
#44302=CARTESIAN_POINT('Ctrl Pts',(-1.59352139913235,-0.6363098000952,3.06524726776171));
#44303=CARTESIAN_POINT('Ctrl Pts',(-1.5856238781577,-0.319434907277161,
3.13941797151494));
#44304=CARTESIAN_POINT('Ctrl Pts',(-1.58468073357809,-0.158333333333333,
3.16639877628142));
#44305=CARTESIAN_POINT('Ctrl Pts',(-1.60650273181183,0.158333333333336,
3.1752338562451));
#44306=CARTESIAN_POINT('Ctrl Pts',(-1.62810716868432,0.319434907277171,
3.15667163125066));
#44307=CARTESIAN_POINT('Ctrl Pts',(-1.68281880325298,0.636309800095212,
3.10134573013792));
#44308=CARTESIAN_POINT('Ctrl Pts',(-1.72250898922017,0.794772684000845,
3.05363894723006));
#44309=CARTESIAN_POINT('Ctrl Pts',(-1.79094505544908,1.06847604194558,2.96226328258396));
#44310=CARTESIAN_POINT('Ctrl Pts',(-1.82252646622328,1.18514270861271,2.91731703719297));
#44311=CARTESIAN_POINT('Ctrl Pts',(-1.85606585050729,1.30000000000137,2.86697768583429));
#44312=CARTESIAN_POINT('Ctrl Pts',(-1.65813795427186,-1.30000000000206,
2.75729053581678));
#44313=CARTESIAN_POINT('Ctrl Pts',(-1.64390914515786,-1.18514270861318,
2.8093649400208));
#44314=CARTESIAN_POINT('Ctrl Pts',(-1.63171417909869,-1.06847604194583,
2.85767162458352));
#44315=CARTESIAN_POINT('Ctrl Pts',(-1.60823995223305,-0.794772684000857,
2.96056554354104));
#44316=CARTESIAN_POINT('Ctrl Pts',(-1.59535384607131,-0.636309800095199,
3.01999716620689));
#44317=CARTESIAN_POINT('Ctrl Pts',(-1.58893802195987,-0.319434907277159,
3.0943983470608));
#44318=CARTESIAN_POINT('Ctrl Pts',(-1.58943971299835,-0.158333333333333,
3.12375775987157));
#44319=CARTESIAN_POINT('Ctrl Pts',(-1.61241973646776,0.158333333333335,
3.13295204857722));
#44320=CARTESIAN_POINT('Ctrl Pts',(-1.63445324641201,0.319434907277171,
3.11260068244772));
#44321=CARTESIAN_POINT('Ctrl Pts',(-1.68858379509115,0.636309800095212,
3.05730696727029));
#44322=CARTESIAN_POINT('Ctrl Pts',(-1.72680330457903,0.794772684000844,
3.00804889397381));
#44323=CARTESIAN_POINT('Ctrl Pts',(-1.79379646466053,1.06847604194558,2.92257770154279));
#44324=CARTESIAN_POINT('Ctrl Pts',(-1.82477850626238,1.1851427086127,2.88178580755026));
#44325=CARTESIAN_POINT('Ctrl Pts',(-1.85774373280798,1.30000000000137,2.83719933174886));
#44326=CARTESIAN_POINT('Ctrl Pts',(-1.65570779467915,-1.30000000000206,
2.73263328270126));
#44327=CARTESIAN_POINT('Ctrl Pts',(-1.6407096481972,-1.18514270861318,2.77980265176276));
#44328=CARTESIAN_POINT('Ctrl Pts',(-1.62827778845606,-1.06847604194583,
2.82459427115372));
#44329=CARTESIAN_POINT('Ctrl Pts',(-1.60548634122433,-0.794772684000854,
2.92257879507314));
#44330=CARTESIAN_POINT('Ctrl Pts',(-1.59504082893022,-0.636309800095202,
2.98341758453039));
#44331=CARTESIAN_POINT('Ctrl Pts',(-1.59073845452414,-0.319434907277163,
3.058177072881));
#44332=CARTESIAN_POINT('Ctrl Pts',(-1.59232101440582,-0.158333333333334,
3.08940613991731));
#44333=CARTESIAN_POINT('Ctrl Pts',(-1.616032042732,0.158333333333336,3.09880489324563));
#44334=CARTESIAN_POINT('Ctrl Pts',(-1.63781874036801,0.319434907277172,
3.07684736794034));
#44335=CARTESIAN_POINT('Ctrl Pts',(-1.69111493475241,0.636309800095214,
3.02149158425097));
#44336=CARTESIAN_POINT('Ctrl Pts',(-1.72816231837234,0.794772684000848,
2.97104767819662));
#44337=CARTESIAN_POINT('Ctrl Pts',(-1.79394620683948,1.06847604194559,2.89029168350367));
#44338=CARTESIAN_POINT('Ctrl Pts',(-1.82444853281462,1.18514270861271,2.85281575960377));
#44339=CARTESIAN_POINT('Ctrl Pts',(-1.85697777698072,1.30000000000138,2.8128201896021));
#44340=CARTESIAN_POINT('Ctrl Pts',(-1.6535760658804,-1.30000000000206,2.71409163860464));
#44341=CARTESIAN_POINT('Ctrl Pts',(-1.63905181668487,-1.18514270861318,
2.75780601699314));
#44342=CARTESIAN_POINT('Ctrl Pts',(-1.62709515198573,-1.06847604194583,
2.80010088337208));
#44343=CARTESIAN_POINT('Ctrl Pts',(-1.60540449843839,-0.794772684000856,
2.8945311290517));
#44344=CARTESIAN_POINT('Ctrl Pts',(-1.59579211137064,-0.636309800095201,
2.95622529437884));
#44345=CARTESIAN_POINT('Ctrl Pts',(-1.59231902228133,-0.319434907277162,
3.03107887714456));
#44346=CARTESIAN_POINT('Ctrl Pts',(-1.59397995331801,-0.158333333333334,
3.06351789461748));
#44347=CARTESIAN_POINT('Ctrl Pts',(-1.61802231115706,0.158333333333336,
3.07301813934396));
#44348=CARTESIAN_POINT('Ctrl Pts',(-1.63995039656627,0.319434907277172,
3.04994084003861));
#44349=CARTESIAN_POINT('Ctrl Pts',(-1.69331946124273,0.636309800095213,
2.99472074036669));
#44350=CARTESIAN_POINT('Ctrl Pts',(-1.73056578233587,0.794772684000846,
2.94366555047251));
#44351=CARTESIAN_POINT('Ctrl Pts',(-1.79568322889274,1.06847604194558,2.86651029602232));
#44352=CARTESIAN_POINT('Ctrl Pts',(-1.82570445831112,1.18514270861271,2.83149135893238));
#44353=CARTESIAN_POINT('Ctrl Pts',(-1.85755998737255,1.30000000000137,2.79485113552013));
#44354=CARTESIAN_POINT('Ctrl Pts',(-1.65142819925317,-1.30000000000207,
2.69555803570173));
#44355=CARTESIAN_POINT('Ctrl Pts',(-1.63652140704014,-1.18514270861319,
2.73564493465463));
#44356=CARTESIAN_POINT('Ctrl Pts',(-1.62445167600304,-1.06847604194583,
2.77532087071986));
#44357=CARTESIAN_POINT('Ctrl Pts',(-1.60312236163452,-0.794772684000861,
2.86603081369074));
#44358=CARTESIAN_POINT('Ctrl Pts',(-1.59467568431381,-0.636309800095204,
2.9286131284341));
#44359=CARTESIAN_POINT('Ctrl Pts',(-1.59244392772632,-0.319434907277163,
3.00363546569633));
#44360=CARTESIAN_POINT('Ctrl Pts',(-1.59497869398103,-0.158333333333334,
3.0374717690488));
#44361=CARTESIAN_POINT('Ctrl Pts',(-1.61951237737304,0.158333333333337,
3.04710102064039));
#44362=CARTESIAN_POINT('Ctrl Pts',(-1.64131649243037,0.319434907277172,
3.02284038948529));
#44363=CARTESIAN_POINT('Ctrl Pts',(-1.69391839341423,0.636309800095215,
2.9675412817542));
#44364=CARTESIAN_POINT('Ctrl Pts',(-1.72981398463404,0.79477268400085,2.91548409447979));
#44365=CARTESIAN_POINT('Ctrl Pts',(-1.79427708629069,1.06847604194559,2.84192785080469));
#44366=CARTESIAN_POINT('Ctrl Pts',(-1.82420907094672,1.18514270861271,2.80946186186775));
#44367=CARTESIAN_POINT('Ctrl Pts',(-1.85616935214488,1.30000000000138,2.77636965635346));
#44368=CARTESIAN_POINT('Ctrl Pts',(-1.64970395610035,-1.30000000000206,
2.67712374665188));
#44369=CARTESIAN_POINT('Ctrl Pts',(-1.63440903515699,-1.18514270861318,
2.71358619627383));
#44370=CARTESIAN_POINT('Ctrl Pts',(-1.62220300990044,-1.06847604194583,
2.75064175423077));
#44371=CARTESIAN_POINT('Ctrl Pts',(-1.60114061671888,-0.79477268400086,
2.83761770495476));
#44372=CARTESIAN_POINT('Ctrl Pts',(-1.59362974755288,-0.636309800095204,
2.90104169110795));
#44373=CARTESIAN_POINT('Ctrl Pts',(-1.59270208718653,-0.319434907277163,
2.97624828130659));
#44374=CARTESIAN_POINT('Ctrl Pts',(-1.59648220610092,-0.158333333333334,
3.01156179865048));
#44375=CARTESIAN_POINT('Ctrl Pts',(-1.62153353448204,0.158333333333336,
3.02132088132003));
#44376=CARTESIAN_POINT('Ctrl Pts',(-1.6425998838543,0.319434907277172,2.99572297667271));
#44377=CARTESIAN_POINT('Ctrl Pts',(-1.69497258163952,0.636309800095215,
2.9404834803997));
#44378=CARTESIAN_POINT('Ctrl Pts',(-1.73105396418615,0.79477268400085,2.88781469783114));
#44379=CARTESIAN_POINT('Ctrl Pts',(-1.79525935632945,1.06847604194559,2.81796705538706));
#44380=CARTESIAN_POINT('Ctrl Pts',(-1.8250096066763,1.18514270861271,2.78803607922216));
#44381=CARTESIAN_POINT('Ctrl Pts',(-1.85671797215536,1.30000000000137,2.75840858319625));
#44382=CARTESIAN_POINT('Ctrl Pts',(-1.64667893682967,-1.30000000000207,
2.65843106406495));
#44383=CARTESIAN_POINT('Ctrl Pts',(-1.63153020095824,-1.18514270861319,
2.69137902331279));
#44384=CARTESIAN_POINT('Ctrl Pts',(-1.61958797589396,-1.06847604194584,
2.72589590660544));
#44385=CARTESIAN_POINT('Ctrl Pts',(-1.59940672838645,-0.794772684000862,
2.80926134049572));
#44386=CARTESIAN_POINT('Ctrl Pts',(-1.59315953932626,-0.636309800095206,
2.87360157089387));
#44387=CARTESIAN_POINT('Ctrl Pts',(-1.5929026847311,-0.319434907277164,
2.94883520381411));
#44388=CARTESIAN_POINT('Ctrl Pts',(-1.59639986569456,-0.158333333333335,
2.98526311606199));
#44389=CARTESIAN_POINT('Ctrl Pts',(-1.62132464236181,0.158333333333337,
2.99500225307932));
#44390=CARTESIAN_POINT('Ctrl Pts',(-1.64226956594183,0.319434907277172,
2.96822463560951));
#44391=CARTESIAN_POINT('Ctrl Pts',(-1.69427956432727,0.636309800095216,
2.91300988879695));
#44392=CARTESIAN_POINT('Ctrl Pts',(-1.72997844828931,0.794772684000853,
2.85958385827857));
#44393=CARTESIAN_POINT('Ctrl Pts',(-1.79388216221858,1.06847604194559,2.79341742157915));
#44394=CARTESIAN_POINT('Ctrl Pts',(-1.8235455079832,1.18514270861271,2.76603529463722));
#44395=CARTESIAN_POINT('Ctrl Pts',(-1.85521064961836,1.30000000000138,2.73991203949251));
#44396=CARTESIAN_POINT('Ctrl Pts',(-1.64412111466084,-1.30000000000207,
2.6398651645125));
#44397=CARTESIAN_POINT('Ctrl Pts',(-1.62798260075153,-1.18514270861319,
2.66908877628028));
#44398=CARTESIAN_POINT('Ctrl Pts',(-1.6154792907022,-1.06847604194584,2.70090983214457));
#44399=CARTESIAN_POINT('Ctrl Pts',(-1.59499219134632,-0.794772684000864,
2.78042345245108));
#44400=CARTESIAN_POINT('Ctrl Pts',(-1.58973719006436,-0.636309800095206,
2.84557205418552));
#44401=CARTESIAN_POINT('Ctrl Pts',(-1.59118661578248,-0.319434907277163,
2.9210401630057));
#44402=CARTESIAN_POINT('Ctrl Pts',(-1.59649715240767,-0.158333333333335,
2.95903747823188));
#44403=CARTESIAN_POINT('Ctrl Pts',(-1.62285437331818,0.158333333333337,
2.96910203929093));
#44404=CARTESIAN_POINT('Ctrl Pts',(-1.64419807136409,0.319434907277175,
2.94127779762337));
#44405=CARTESIAN_POINT('Ctrl Pts',(-1.69583141121319,0.636309800095219,
2.88608944285955));
#44406=CARTESIAN_POINT('Ctrl Pts',(-1.72975502771052,0.794772684000852,
2.83157946580677));
#44407=CARTESIAN_POINT('Ctrl Pts',(-1.79329774536375,1.06847604194559,2.76909658247525));
#44408=CARTESIAN_POINT('Ctrl Pts',(-1.823107272097,1.18514270861271,2.7443281138452));
#44409=CARTESIAN_POINT('Ctrl Pts',(-1.85522103758111,1.30000000000138,2.72183770156036));
#44410=CARTESIAN_POINT('Ctrl Pts',(-1.64094945361943,-1.30000000000208,
2.61515000440255));
#44411=CARTESIAN_POINT('Ctrl Pts',(-1.62468107455144,-1.1851427086132,2.63963826366359));
#44412=CARTESIAN_POINT('Ctrl Pts',(-1.61217517672228,-1.06847604194585,
2.66801224695561));
#44413=CARTESIAN_POINT('Ctrl Pts',(-1.59197613528423,-0.79477268400087,
2.74253862440383));
#44414=CARTESIAN_POINT('Ctrl Pts',(-1.58721925808487,-0.636309800095212,
2.80864512682796));
#44415=CARTESIAN_POINT('Ctrl Pts',(-1.58961959416009,-0.319434907277167,
2.88415188749081));
#44416=CARTESIAN_POINT('Ctrl Pts',(-1.5962106690206,-0.158333333333336,
2.92397834243149));
#44417=CARTESIAN_POINT('Ctrl Pts',(-1.6224445641406,0.158333333333338,2.93401310656952));
#44418=CARTESIAN_POINT('Ctrl Pts',(-1.64189888908404,0.319434907277176,
2.90423138779478));
#44419=CARTESIAN_POINT('Ctrl Pts',(-1.69331905985183,0.636309800095222,
2.84914440685121));
#44420=CARTESIAN_POINT('Ctrl Pts',(-1.72885664617953,0.79477268400086,2.79412538512413));
#44421=CARTESIAN_POINT('Ctrl Pts',(-1.79247296240661,1.0684760419456,2.73665013861037));
#44422=CARTESIAN_POINT('Ctrl Pts',(-1.82203822932527,1.18514270861273,2.71524106197467));
#44423=CARTESIAN_POINT('Ctrl Pts',(-1.85363161708467,1.30000000000139,2.69730181325134));
#44424=CARTESIAN_POINT('Ctrl Pts',(-1.6362445112492,-1.30000000000209,2.59017900567184));
#44425=CARTESIAN_POINT('Ctrl Pts',(-1.61935634141682,-1.18514270861321,
2.60985405552272));
#44426=CARTESIAN_POINT('Ctrl Pts',(-1.60655803475591,-1.06847604194585,
2.63473402983644));
#44427=CARTESIAN_POINT('Ctrl Pts',(-1.58643978817718,-0.794772684000877,
2.70423616447344));
#44428=CARTESIAN_POINT('Ctrl Pts',(-1.58274842400019,-0.636309800095214,
2.77138539803646));
#44429=CARTESIAN_POINT('Ctrl Pts',(-1.58654761135435,-0.319434907277167,
2.84699453149146));
#44430=CARTESIAN_POINT('Ctrl Pts',(-1.59403516911422,-0.158333333333337,
2.88853699146736));
#44431=CARTESIAN_POINT('Ctrl Pts',(-1.62180505785957,0.158333333333339,
2.89889527495238));
#44432=CARTESIAN_POINT('Ctrl Pts',(-1.64291504432118,0.319434907277178,
2.86795875947623));
#44433=CARTESIAN_POINT('Ctrl Pts',(-1.69399524623128,0.636309800095225,
2.81294423600424));
#44434=CARTESIAN_POINT('Ctrl Pts',(-1.72652996574593,0.794772684000862,
2.75637597115294));
#44435=CARTESIAN_POINT('Ctrl Pts',(-1.78960294812671,1.0684760419456,2.70378004334336));
#44436=CARTESIAN_POINT('Ctrl Pts',(-1.81943005640006,1.18514270861273,2.68585139577623));
#44437=CARTESIAN_POINT('Ctrl Pts',(-1.85178231595841,1.30000000000139,2.67276092891958));
#44438=CARTESIAN_POINT('Ctrl Pts',(-1.63234955645659,-1.3000000000021,2.56539932197508));
#44439=CARTESIAN_POINT('Ctrl Pts',(-1.61422340273142,-1.18514270861321,
2.58016419306643));
#44440=CARTESIAN_POINT('Ctrl Pts',(-1.60076142905862,-1.06847604194586,
2.60149109593607));
#44441=CARTESIAN_POINT('Ctrl Pts',(-1.58043676580292,-0.794772684000878,
2.66592011413487));
#44442=CARTESIAN_POINT('Ctrl Pts',(-1.57894742814013,-0.636309800095219,
2.7342993560036));
#44443=CARTESIAN_POINT('Ctrl Pts',(-1.58377104162534,-0.31943490727717,
2.80991755850134));
#44444=CARTESIAN_POINT('Ctrl Pts',(-1.5914330166678,-0.158333333333338,
2.85304301060135));
#44445=CARTESIAN_POINT('Ctrl Pts',(-1.61892764149841,0.15833333333334,2.86333412198892));
#44446=CARTESIAN_POINT('Ctrl Pts',(-1.63880461079261,0.319434907277178,
2.83060339342189));
#44447=CARTESIAN_POINT('Ctrl Pts',(-1.68989529276597,0.636309800095229,
2.77573639335614));
#44448=CARTESIAN_POINT('Ctrl Pts',(-1.72352228384938,0.794772684000869,
2.71852594707303));
#44449=CARTESIAN_POINT('Ctrl Pts',(-1.78730622572994,1.06847604194561,2.67106706560053));
#44450=CARTESIAN_POINT('Ctrl Pts',(-1.81738454011351,1.18514270861274,2.65660361998266));
#44451=CARTESIAN_POINT('Ctrl Pts',(-1.84993146386848,1.3000000000014,2.64821992001154));
#44452=CARTESIAN_POINT('Ctrl Pts',(-1.62923415387097,-1.3000000000021,2.54677610074369));
#44453=CARTESIAN_POINT('Ctrl Pts',(-1.6108894203325,-1.18514270861322,2.55798510922409));
#44454=CARTESIAN_POINT('Ctrl Pts',(-1.59724221540616,-1.06847604194586,
2.57670468010306));
#44455=CARTESIAN_POINT('Ctrl Pts',(-1.57656667274378,-0.794772684000883,
2.63730153529417));
#44456=CARTESIAN_POINT('Ctrl Pts',(-1.57451719774664,-0.636309800095222,
2.70622110562794));
#44457=CARTESIAN_POINT('Ctrl Pts',(-1.57999669011221,-0.319434907277172,
2.7818349079464));
#44458=CARTESIAN_POINT('Ctrl Pts',(-1.58906586793436,-0.158333333333339,
2.82636372819642));
#44459=CARTESIAN_POINT('Ctrl Pts',(-1.61768822563586,0.158333333333341,
2.83686870991166));
#44460=CARTESIAN_POINT('Ctrl Pts',(-1.63807626269469,0.31943490727718,2.80310903570228));
#44461=CARTESIAN_POINT('Ctrl Pts',(-1.68919790812606,0.636309800095232,
2.74835504104364));
#44462=CARTESIAN_POINT('Ctrl Pts',(-1.72180197162245,0.794772684000873,
2.69026507416506));
#44463=CARTESIAN_POINT('Ctrl Pts',(-1.78546486858486,1.06847604194562,2.64651824311741));
#44464=CARTESIAN_POINT('Ctrl Pts',(-1.81565969751708,1.18514270861275,2.63463881062376));
#44465=CARTESIAN_POINT('Ctrl Pts',(-1.84849204622925,1.30000000000141,2.62981632781718));
#44466=CARTESIAN_POINT('Ctrl Pts',(-1.62566884587422,-1.30000000000211,
2.52960364403045));
#44467=CARTESIAN_POINT('Ctrl Pts',(-1.60649968537675,-1.18514270861322,
2.53746013654931));
#44468=CARTESIAN_POINT('Ctrl Pts',(-1.59239171942472,-1.06847604194587,
2.55374804287688));
#44469=CARTESIAN_POINT('Ctrl Pts',(-1.57149186767519,-0.794772684000888,
2.61085461747457));
#44470=CARTESIAN_POINT('Ctrl Pts',(-1.57054210463338,-0.636309800095227,
2.68052984997528));
#44471=CARTESIAN_POINT('Ctrl Pts',(-1.57704051133011,-0.319434907277174,
2.75619800745381));
#44472=CARTESIAN_POINT('Ctrl Pts',(-1.58707769310611,-0.15833333333334,
2.80195951806694));
#44473=CARTESIAN_POINT('Ctrl Pts',(-1.61588562542525,0.158333333333342,
2.81248517859209));
#44474=CARTESIAN_POINT('Ctrl Pts',(-1.63540582925339,0.319434907277182,
2.77750541926282));
#44475=CARTESIAN_POINT('Ctrl Pts',(-1.68606052407164,0.636309800095236,
2.72275563596497));
#44476=CARTESIAN_POINT('Ctrl Pts',(-1.71823122031223,0.794772684000878,
2.66397315520516));
#44477=CARTESIAN_POINT('Ctrl Pts',(-1.78242013395345,1.06847604194563,2.62375631750794));
#44478=CARTESIAN_POINT('Ctrl Pts',(-1.8130888217976,1.18514270861275,2.61431643519053));
#44479=CARTESIAN_POINT('Ctrl Pts',(-1.84664119520423,1.30000000000142,2.61284504941418));
#44480=CARTESIAN_POINT('Ctrl Pts',(-1.62331482812817,-1.30000000000211,
2.51716170796398));
#44481=CARTESIAN_POINT('Ctrl Pts',(-1.60372347681876,-1.18514270861323,
2.52260971504939));
#44482=CARTESIAN_POINT('Ctrl Pts',(-1.58935222110575,-1.06847604194587,
2.53714147663927));
#44483=CARTESIAN_POINT('Ctrl Pts',(-1.56821121055313,-0.794772684000889,
2.59169804308482));
#44484=CARTESIAN_POINT('Ctrl Pts',(-1.56747946744677,-0.636309800095227,
2.66182785185384));
#44485=CARTESIAN_POINT('Ctrl Pts',(-1.57461975734037,-0.319434907277174,
2.73752053848879));
#44486=CARTESIAN_POINT('Ctrl Pts',(-1.58562722961563,-0.15833333333334,
2.78421941340941));
#44487=CARTESIAN_POINT('Ctrl Pts',(-1.6148195448593,0.158333333333342,2.79480947981818));
#44488=CARTESIAN_POINT('Ctrl Pts',(-1.63396495408773,0.319434907277182,
2.75900164171681));
#44489=CARTESIAN_POINT('Ctrl Pts',(-1.68433070412041,0.636309800095237,
2.70426710279089));
#44490=CARTESIAN_POINT('Ctrl Pts',(-1.71596433378824,0.794772684000879,
2.64493461636281));
#44491=CARTESIAN_POINT('Ctrl Pts',(-1.78038983077672,1.06847604194563,2.60725219541814));
#44492=CARTESIAN_POINT('Ctrl Pts',(-1.81134588447279,1.18514270861276,2.59957287367714));
#44493=CARTESIAN_POINT('Ctrl Pts',(-1.84537058141848,1.30000000000142,2.6005255539508));
#44494=CARTESIAN_POINT('Ctrl Pts',(-1.62120595304708,-1.30000000000211,
2.50778328167275));
#44495=CARTESIAN_POINT('Ctrl Pts',(-1.6010197698275,-1.18514270861323,2.51138821153288));
#44496=CARTESIAN_POINT('Ctrl Pts',(-1.58632213734058,-1.06847604194587,
2.52458646089038));
#44497=CARTESIAN_POINT('Ctrl Pts',(-1.56504731621779,-0.794772684000891,
2.5772395443827));
#44498=CARTESIAN_POINT('Ctrl Pts',(-1.56528632124749,-0.636309800095228,
2.64782812100501));
#44499=CARTESIAN_POINT('Ctrl Pts',(-1.57293731981988,-0.319434907277175,
2.72353329223748));
#44500=CARTESIAN_POINT('Ctrl Pts',(-1.58397757912001,-0.15833333333334,
2.7708141309076));
#44501=CARTESIAN_POINT('Ctrl Pts',(-1.61340988959623,0.158333333333342,
2.78144311075226));
#44502=CARTESIAN_POINT('Ctrl Pts',(-1.63265735838685,0.319434907277183,
2.74508128852036));
#44503=CARTESIAN_POINT('Ctrl Pts',(-1.68321543296914,0.636309800095237,
2.69043580026173));
#44504=CARTESIAN_POINT('Ctrl Pts',(-1.71492527071949,0.79477268400088,2.63078860133227));
#44505=CARTESIAN_POINT('Ctrl Pts',(-1.77949867744253,1.06847604194563,2.59500012320804));
#44506=CARTESIAN_POINT('Ctrl Pts',(-1.81051752399895,1.18514270861276,2.58861007352683));
#44507=CARTESIAN_POINT('Ctrl Pts',(-1.84460378202186,1.30000000000142,2.59132148025061));
#44508=CARTESIAN_POINT('Ctrl Pts',(-1.61998967096031,-1.30000000000212,
2.50231677111702));
#44509=CARTESIAN_POINT('Ctrl Pts',(-1.59944335020525,-1.18514270861323,
2.50484457426506));
#44510=CARTESIAN_POINT('Ctrl Pts',(-1.58454208979709,-1.06847604194588,
2.51726296944205));
#44511=CARTESIAN_POINT('Ctrl Pts',(-1.56315841595922,-0.794772684000892,
2.56880119278524));
#44512=CARTESIAN_POINT('Ctrl Pts',(-1.56393073117033,-0.63630980009523,
2.63965316376642));
#44513=CARTESIAN_POINT('Ctrl Pts',(-1.57187486651392,-0.319434907277175,
2.71536415798917));
#44514=CARTESIAN_POINT('Ctrl Pts',(-1.5829735170385,-0.15833333333334,2.7629886917636));
#44515=CARTESIAN_POINT('Ctrl Pts',(-1.61254266333681,0.158333333333343,
2.77363889973037));
#44516=CARTESIAN_POINT('Ctrl Pts',(-1.63181530847559,0.319434907277183,
2.73694898722863));
#44517=CARTESIAN_POINT('Ctrl Pts',(-1.68246747459253,0.636309800095239,
2.68235237036807));
#44518=CARTESIAN_POINT('Ctrl Pts',(-1.71420345164054,0.794772684000881,
2.62251781380482));
#44519=CARTESIAN_POINT('Ctrl Pts',(-1.77889739114558,1.06847604194563,2.58784029560954));
#44520=CARTESIAN_POINT('Ctrl Pts',(-1.8099805829054,1.18514270861276,2.58220738149782));
#44521=CARTESIAN_POINT('Ctrl Pts',(-1.84414335715996,1.30000000000143,2.58595216597246));
#44522=CARTESIAN_POINT('Ctrl Pts',(-1.61900425859119,-1.30000000000212,
2.49763984030326));
#44523=CARTESIAN_POINT('Ctrl Pts',(-1.59822013030825,-1.18514270861323,
2.49925493119758));
#44524=CARTESIAN_POINT('Ctrl Pts',(-1.58317352130879,-1.06847604194588,
2.51100928224148));
#44525=CARTESIAN_POINT('Ctrl Pts',(-1.56166766178791,-0.794772684000893,
2.56158790390019));
#44526=CARTESIAN_POINT('Ctrl Pts',(-1.56266468437642,-0.63630980009523,
2.63263142885374));
#44527=CARTESIAN_POINT('Ctrl Pts',(-1.57083050532711,-0.319434907277176,
2.7083436091765));
#44528=CARTESIAN_POINT('Ctrl Pts',(-1.58215381353722,-0.15833333333334,
2.75629009811465));
#44529=CARTESIAN_POINT('Ctrl Pts',(-1.61183972911496,0.158333333333343,
2.76695697053588));
#44530=CARTESIAN_POINT('Ctrl Pts',(-1.63102197382705,0.319434907277183,
2.72996647897455));
#44531=CARTESIAN_POINT('Ctrl Pts',(-1.68165468319656,0.636309800095239,
2.67539302301664));
#44532=CARTESIAN_POINT('Ctrl Pts',(-1.71329828605972,0.794772684000882,
2.61537529648118));
#44533=CARTESIAN_POINT('Ctrl Pts',(-1.7781446537935,1.06847604194563,2.58165950682896));
#44534=CARTESIAN_POINT('Ctrl Pts',(-1.80934725931507,1.18514270861276,2.57668799123382));
#44535=CARTESIAN_POINT('Ctrl Pts',(-1.84368288056094,1.30000000000143,2.5813392760909));
#44536=CARTESIAN_POINT('Ctrl Pts',(-1.61852730161631,-1.30000000000212,
2.49530381627404));
#44537=CARTESIAN_POINT('Ctrl Pts',(-1.59764011390879,-1.18514270861323,
2.4964648606895));
#44538=CARTESIAN_POINT('Ctrl Pts',(-1.58252720222537,-1.06847604194588,
2.50788812094456));
#44539=CARTESIAN_POINT('Ctrl Pts',(-1.56095308566473,-0.794772684000893,
2.55798590888769));
#44540=CARTESIAN_POINT('Ctrl Pts',(-1.56200858938868,-0.63630980009523,
2.62911727391898));
#44541=CARTESIAN_POINT('Ctrl Pts',(-1.57027928739533,-0.319434907277176,
2.70482939298503));
#44542=CARTESIAN_POINT('Ctrl Pts',(-1.58175670986222,-0.158333333333341,
2.75294354038181));
#44543=CARTESIAN_POINT('Ctrl Pts',(-1.61150219129874,0.158333333333343,
2.76361871218339));
#44544=CARTESIAN_POINT('Ctrl Pts',(-1.63061450625396,0.319434907277183,
2.72647371958498));
#44545=CARTESIAN_POINT('Ctrl Pts',(-1.68121352353356,0.636309800095239,
2.67190733464389));
#44546=CARTESIAN_POINT('Ctrl Pts',(-1.71278158764814,0.794772684000882,
2.6117921551272));
#44547=CARTESIAN_POINT('Ctrl Pts',(-1.77771405955071,1.06847604194563,2.5785591023655));
#44548=CARTESIAN_POINT('Ctrl Pts',(-1.80899089960785,1.18514270861276,2.5739210942678));
#44549=CARTESIAN_POINT('Ctrl Pts',(-1.84343771862066,1.30000000000143,2.57903043520702));
#44550=CARTESIAN_POINT('Ctrl Pts',(-1.61805756187616,-1.30000000000212,
2.49296899520644));
#44551=CARTESIAN_POINT('Ctrl Pts',(-1.59707587812017,-1.18514270861323,
2.49367732789126));
#44552=CARTESIAN_POINT('Ctrl Pts',(-1.58189991142332,-1.06847604194588,
2.50477002389613));
#44553=CARTESIAN_POINT('Ctrl Pts',(-1.56025276024826,-0.794772684000893,
2.55438632740748));
#44554=CARTESIAN_POINT('Ctrl Pts',(-1.56133713044918,-0.63630980009523,
2.62560110280928));
#44555=CARTESIAN_POINT('Ctrl Pts',(-1.56970645949404,-0.319434907277176,
2.70131223625752));
#44556=CARTESIAN_POINT('Ctrl Pts',(-1.58135592754541,-0.158333333333341,
2.74959680823923));
#44557=CARTESIAN_POINT('Ctrl Pts',(-1.61116114362569,0.158333333333343,
2.76028010748835));
#44558=CARTESIAN_POINT('Ctrl Pts',(-1.63019435625302,0.319434907277183,
2.72297900142918));
#44559=CARTESIAN_POINT('Ctrl Pts',(-1.68074877410949,0.636309800095239,
2.66841756142733));
#44560=CARTESIAN_POINT('Ctrl Pts',(-1.71222593475649,0.794772684000882,
2.60820195246472));
#44561=CARTESIAN_POINT('Ctrl Pts',(-1.77724894761959,1.06847604194563,2.57545233030315));
#44562=CARTESIAN_POINT('Ctrl Pts',(-1.80860698165484,1.18514270861276,2.57114907090689));
#44563=CARTESIAN_POINT('Ctrl Pts',(-1.84317699679694,1.30000000000143,2.57671865005504));
#44564=CARTESIAN_POINT('Ctrl Pts',(-1.61593270096015,-1.30000000000211,
2.48208353539143));
#44565=CARTESIAN_POINT('Ctrl Pts',(-1.59458499586163,-1.18514270861323,
2.48069034169533));
#44566=CARTESIAN_POINT('Ctrl Pts',(-1.57914568209439,-1.06847604194587,
2.49024505217354));
#44567=CARTESIAN_POINT('Ctrl Pts',(-1.55712734461286,-0.794772684000891,
2.53761019355471));
#44568=CARTESIAN_POINT('Ctrl Pts',(-1.55809913997242,-0.636309800095228,
2.60917757859137));
#44569=CARTESIAN_POINT('Ctrl Pts',(-1.56690123771344,-0.319434907277175,
2.68488108825686));
#44570=CARTESIAN_POINT('Ctrl Pts',(-1.57954395119173,-0.15833333333334,
2.73399152492558));
#44571=CARTESIAN_POINT('Ctrl Pts',(-1.6096330744329,0.158333333333342,2.74471260480286));
#44572=CARTESIAN_POINT('Ctrl Pts',(-1.62818552780862,0.319434907277182,
2.70666397085689));
#44573=CARTESIAN_POINT('Ctrl Pts',(-1.67841987641955,0.636309800095237,
2.65210450105468));
#44574=CARTESIAN_POINT('Ctrl Pts',(-1.70933004796508,0.794772684000879,
2.59139161815161));
#44575=CARTESIAN_POINT('Ctrl Pts',(-1.77482473182672,1.06847604194563,2.56090741895018));
#44576=CARTESIAN_POINT('Ctrl Pts',(-1.80663255816778,1.18514270861276,2.55818010876215));
#44577=CARTESIAN_POINT('Ctrl Pts',(-1.84189798902335,1.30000000000143,2.5659209686695));
#44578=CARTESIAN_POINT('Ctrl Pts',(-1.61289545439995,-1.30000000000208,
2.46881380796962));
#44579=CARTESIAN_POINT('Ctrl Pts',(-1.59055835390608,-1.1851427086132,2.46479767353596));
#44580=CARTESIAN_POINT('Ctrl Pts',(-1.57452299098335,-1.06847604194584,
2.47244942941252));
#44581=CARTESIAN_POINT('Ctrl Pts',(-1.5520363692162,-0.79477268400087,2.51708167698579));
#44582=CARTESIAN_POINT('Ctrl Pts',(-1.5543243501601,-0.636309800095212,
2.58928478249518));
#44583=CARTESIAN_POINT('Ctrl Pts',(-1.56347676621394,-0.319434907277167,
2.66493381116114));
#44584=CARTESIAN_POINT('Ctrl Pts',(-1.57565570893638,-0.158333333333336,
2.71476774826991));
#44585=CARTESIAN_POINT('Ctrl Pts',(-1.60606953040166,0.158333333333338,
2.7255321629494));
#44586=CARTESIAN_POINT('Ctrl Pts',(-1.62530771097436,0.319434907277174,
2.68679337701408));
#44587=CARTESIAN_POINT('Ctrl Pts',(-1.67606240579018,0.636309800095221,
2.63239699956226));
#44588=CARTESIAN_POINT('Ctrl Pts',(-1.70707773163962,0.79477268400086,2.57124503444124));
#44589=CARTESIAN_POINT('Ctrl Pts',(-1.77268191365742,1.0684760419456,2.54339878674876));
#44590=CARTESIAN_POINT('Ctrl Pts',(-1.80448939996189,1.18514270861273,2.54246350348996));
#44591=CARTESIAN_POINT('Ctrl Pts',(-1.83970675304978,1.30000000000139,2.55264654579327));
#44592=CARTESIAN_POINT('Ctrl Pts',(-1.6085954580606,-1.30000000000208,2.45008653506969));
#44593=CARTESIAN_POINT('Ctrl Pts',(-1.58521230478708,-1.18514270861319,
2.44242543180878));
#44594=CARTESIAN_POINT('Ctrl Pts',(-1.56850756594605,-1.06847604194584,
2.44742086826609));
#44595=CARTESIAN_POINT('Ctrl Pts',(-1.54534475080307,-0.794772684000867,
2.48820046449719));
#44596=CARTESIAN_POINT('Ctrl Pts',(-1.54820936146995,-0.636309800095211,
2.56110497709644));
#44597=CARTESIAN_POINT('Ctrl Pts',(-1.55853298333244,-0.319434907277166,
2.63679338908053));
#44598=CARTESIAN_POINT('Ctrl Pts',(-1.5725199715987,-0.158333333333336,
2.68804907051085));
#44599=CARTESIAN_POINT('Ctrl Pts',(-1.60347643686853,0.158333333333338,
2.69888149381968));
#44600=CARTESIAN_POINT('Ctrl Pts',(-1.62148176391517,0.319434907277173,
2.65879822403054));
#44601=CARTESIAN_POINT('Ctrl Pts',(-1.6721042809138,0.636309800095219,2.60448214661314));
#44602=CARTESIAN_POINT('Ctrl Pts',(-1.70346837844412,0.794772684000858,
2.54272074724158));
#44603=CARTESIAN_POINT('Ctrl Pts',(-1.76979719708233,1.0684760419456,2.51872721614525));
#44604=CARTESIAN_POINT('Ctrl Pts',(-1.80202329644897,1.18514270861272,2.52041860498502));
#44605=CARTESIAN_POINT('Ctrl Pts',(-1.83776420731868,1.30000000000139,2.53418729322825));
#44606=CARTESIAN_POINT('Ctrl Pts',(-1.60534913147455,-1.30000000000206,
2.43454767824767));
#44607=CARTESIAN_POINT('Ctrl Pts',(-1.58082296890353,-1.18514270861318,
2.42381174236594));
#44608=CARTESIAN_POINT('Ctrl Pts',(-1.5634146055833,-1.06847604194583,2.42657298233486));
#44609=CARTESIAN_POINT('Ctrl Pts',(-1.53964134396266,-0.794772684000859,
2.46413317536291));
#44610=CARTESIAN_POINT('Ctrl Pts',(-1.54379214603354,-0.636309800095206,
2.53773502783626));
#44611=CARTESIAN_POINT('Ctrl Pts',(-1.55467398927249,-0.319434907277165,
2.61338443365141));
#44612=CARTESIAN_POINT('Ctrl Pts',(-1.56874971205332,-0.158333333333334,
2.66560188014383));
#44613=CARTESIAN_POINT('Ctrl Pts',(-1.59993362305996,0.158333333333337,
2.67645941661085));
#44614=CARTESIAN_POINT('Ctrl Pts',(-1.61815211777964,0.31943490727717,2.63546438865947));
#44615=CARTESIAN_POINT('Ctrl Pts',(-1.66852804156187,0.636309800095214,
2.5811877643467));
#44616=CARTESIAN_POINT('Ctrl Pts',(-1.69854082941393,0.794772684000854,
2.51862531634145));
#44617=CARTESIAN_POINT('Ctrl Pts',(-1.76573087147969,1.06847604194559,2.49789326835724));
#44618=CARTESIAN_POINT('Ctrl Pts',(-1.79880622192406,1.18514270861272,2.501866430681));
#44619=CARTESIAN_POINT('Ctrl Pts',(-1.83587284323888,1.30000000000138,2.51878689070282));
#44620=CARTESIAN_POINT('Ctrl Pts',(-1.60198733594496,-1.30000000000205,
2.42200092146299));
#44621=CARTESIAN_POINT('Ctrl Pts',(-1.57696419153587,-1.18514270861317,
2.40887668461549));
#44622=CARTESIAN_POINT('Ctrl Pts',(-1.55920094320137,-1.06847604194582,
2.4098895933856));
#44623=CARTESIAN_POINT('Ctrl Pts',(-1.53493609829261,-0.794772684000851,
2.44488924977912));
#44624=CARTESIAN_POINT('Ctrl Pts',(-1.53902558372091,-0.636309800095197,
2.51889895831909));
#44625=CARTESIAN_POINT('Ctrl Pts',(-1.55037005382429,-0.319434907277159,
2.59451606221727));
#44626=CARTESIAN_POINT('Ctrl Pts',(-1.56533425685721,-0.158333333333332,
2.64760234942825));
#44627=CARTESIAN_POINT('Ctrl Pts',(-1.59715844965934,0.158333333333334,
2.65854012062382));
#44628=CARTESIAN_POINT('Ctrl Pts',(-1.61542530252264,0.319434907277167,
2.61680038082727));
#44629=CARTESIAN_POINT('Ctrl Pts',(-1.66603874291415,0.636309800095206,
2.56263008158386));
#44630=CARTESIAN_POINT('Ctrl Pts',(-1.69601474884685,0.79477268400084,2.49962533899737));
#44631=CARTESIAN_POINT('Ctrl Pts',(-1.76343954853272,1.06847604194558,2.48139778494711));
#44632=CARTESIAN_POINT('Ctrl Pts',(-1.79665188668013,1.1851427086127,2.48708204616755));
#44633=CARTESIAN_POINT('Ctrl Pts',(-1.83389086552595,1.30000000000136,2.50634060135935));
#44634=CARTESIAN_POINT('Ctrl Pts',(-1.60034588134944,-1.30000000000205,
2.41573690783759));
#44635=CARTESIAN_POINT('Ctrl Pts',(-1.57504122138986,-1.18514270861317,
2.40141459471707));
#44636=CARTESIAN_POINT('Ctrl Pts',(-1.55708435379931,-1.06847604194582,
2.40155144628234));
#44637=CARTESIAN_POINT('Ctrl Pts',(-1.53257526769946,-0.794772684000851,
2.43527116374521));
#44638=CARTESIAN_POINT('Ctrl Pts',(-1.53670704324099,-0.636309800095197,
2.50949324534634));
#44639=CARTESIAN_POINT('Ctrl Pts',(-1.54831342142086,-0.319434907277159,
2.58509892141659));
#44640=CARTESIAN_POINT('Ctrl Pts',(-1.56375557866725,-0.158333333333332,
2.63862740032413));
#44641=CARTESIAN_POINT('Ctrl Pts',(-1.59581317861656,0.158333333333334,
2.64959190996706));
#44642=CARTESIAN_POINT('Ctrl Pts',(-1.61390936643398,0.319434907277167,
2.60744757149566));
#44643=CARTESIAN_POINT('Ctrl Pts',(-1.66458583994602,0.636309800095206,
2.55332105438581));
#44644=CARTESIAN_POINT('Ctrl Pts',(-1.69463294550622,0.79477268400084,2.49010824790527));
#44645=CARTESIAN_POINT('Ctrl Pts',(-1.76226517728142,1.06847604194558,2.47314938073029));
#44646=CARTESIAN_POINT('Ctrl Pts',(-1.79559295568808,1.1851427086127,2.47969831528682));
#44647=CARTESIAN_POINT('Ctrl Pts',(-1.83297302538704,1.30000000000136,2.50013704961196));
#44648=CARTESIAN_POINT('',(-1.81613517243772,1.2,2.59520325796734));
#44649=CARTESIAN_POINT('Ctrl Pts',(-1.81613517243772,1.2,2.59520325796734));
#44650=CARTESIAN_POINT('Ctrl Pts',(-1.82250678261496,1.21684007853956,2.61581873774569));
#44651=CARTESIAN_POINT('Ctrl Pts',(-1.83001234347906,1.23321800531665,2.63645045406549));
#44652=CARTESIAN_POINT('Ctrl Pts',(-1.84225408385894,1.26589996427597,2.67664972145215));
#44653=CARTESIAN_POINT('Ctrl Pts',(-1.8510324951693,1.28855401991379,2.70473410601027));
#44654=CARTESIAN_POINT('Ctrl Pts',(-1.85490568620932,1.30000000000138,2.71872508149132));
#44655=CARTESIAN_POINT('',(-1.66957757316342,0.653834841343326,2.54006322716652));
#44656=CARTESIAN_POINT('Ctrl Pts',(-1.66957757323826,0.653834841326689,
2.54006322715213));
#44657=CARTESIAN_POINT('Ctrl Pts',(-1.68487397676607,0.717899058900883,
2.54554367324531));
#44658=CARTESIAN_POINT('Ctrl Pts',(-1.69802885347761,0.767415508768553,
2.55032811960476));
#44659=CARTESIAN_POINT('Ctrl Pts',(-1.74589484775824,0.949818223351814,
2.56798214841286));
#44660=CARTESIAN_POINT('Ctrl Pts',(-1.77255449741379,1.04964523963697,2.5780150081523));
#44661=CARTESIAN_POINT('Ctrl Pts',(-1.81613517243772,1.2,2.59520325796734));
#44662=CARTESIAN_POINT('',(-1.53759581372214,-0.653834841531101,2.49486460198815));
#44663=CARTESIAN_POINT('Ctrl Pts',(-1.53759581372214,-0.6538348415311,2.49486460198815));
#44664=CARTESIAN_POINT('Ctrl Pts',(-1.54253896106846,-0.575773996990663,
2.5362541007448));
#44665=CARTESIAN_POINT('Ctrl Pts',(-1.54771098720326,-0.493714162387373,
2.57104087379186));
#44666=CARTESIAN_POINT('Ctrl Pts',(-1.55721339216251,-0.337911306543783,
2.62081608951078));
#44667=CARTESIAN_POINT('Ctrl Pts',(-1.56181618753724,-0.265423834229001,
2.63812662410482));
#44668=CARTESIAN_POINT('Ctrl Pts',(-1.57204015447595,-0.129509891678934,
2.66019653582912));
#44669=CARTESIAN_POINT('Ctrl Pts',(-1.57737847383145,-0.0665328266301909,
2.66641946766735));
#44670=CARTESIAN_POINT('Ctrl Pts',(-1.58979323208528,0.0594341807793119,
2.67106517994948));
#44671=CARTESIAN_POINT('Ctrl Pts',(-1.59693716234678,0.122550355968248,
2.66953017416603));
#44672=CARTESIAN_POINT('Ctrl Pts',(-1.61359765438044,0.259896461491062,
2.65729142037106));
#44673=CARTESIAN_POINT('Ctrl Pts',(-1.62330966879801,0.333789134744896,
2.64494004755738));
#44674=CARTESIAN_POINT('Ctrl Pts',(-1.64492474574799,0.491517033436927,
2.60552673792889));
#44675=CARTESIAN_POINT('Ctrl Pts',(-1.65731436333269,0.574921799602958,
2.57626786129867));
#44676=CARTESIAN_POINT('Ctrl Pts',(-1.66957757326119,0.6538348413646,2.540063227246));
#44677=CARTESIAN_POINT('',(-1.6061456467244,-1.2,2.51782142998494));
#44678=CARTESIAN_POINT('Ctrl Pts',(-1.6061456467244,-1.2,2.51782142998494));
#44679=CARTESIAN_POINT('Ctrl Pts',(-1.59629030340056,-1.14500162986664,
2.51444071382048));
#44680=CARTESIAN_POINT('Ctrl Pts',(-1.58195573524929,-1.06328611335836,
2.50954158073653));
#44681=CARTESIAN_POINT('Ctrl Pts',(-1.54495003427023,-0.766654883195457,
2.49724355903312));
#44682=CARTESIAN_POINT('Ctrl Pts',(-1.54083638237218,-0.699422956716546,
2.49592359059717));
#44683=CARTESIAN_POINT('Ctrl Pts',(-1.53759581372214,-0.653834841531101,
2.49486460198815));
#44684=CARTESIAN_POINT('Ctrl Pts',(-1.64377746965492,-1.30000000000001,
2.63705187074685));
#44685=CARTESIAN_POINT('Ctrl Pts',(-1.63611465680649,-1.27671330627714,
2.60953974040605));
#44686=CARTESIAN_POINT('Ctrl Pts',(-1.63296016223809,-1.27025479401098,
2.60156608361734));
#44687=CARTESIAN_POINT('Ctrl Pts',(-1.6216712464152,-1.2389971406116,2.5644647456061));
#44688=CARTESIAN_POINT('Ctrl Pts',(-1.6142786492348,-1.21821497175287,2.53986819629468));
#44689=CARTESIAN_POINT('Ctrl Pts',(-1.6061456467244,-1.2,2.51782142998494));
#44690=CARTESIAN_POINT('Origin',(0.,1.25,7.2));
#44691=CARTESIAN_POINT('Origin',(0.,1.2,7.2));
#44692=CARTESIAN_POINT('Origin',(0.,0.92691742076555,7.2));
#44693=CARTESIAN_POINT('Origin',(0.,0.653834841531101,7.2));
#44694=CARTESIAN_POINT('Origin',(0.,0.,7.2));
#44695=CARTESIAN_POINT('Origin',(0.,-0.653834841531101,7.2));
#44696=CARTESIAN_POINT('Origin',(0.,-0.926917420765551,7.2));
#44697=CARTESIAN_POINT('Origin',(0.,-1.2,7.2));
#44698=CARTESIAN_POINT('Origin',(0.,-1.25,7.2));
#44699=CARTESIAN_POINT('Ctrl Pts',(-1.27960380226531,-1.30000000000134,
2.32033648972617));
#44700=CARTESIAN_POINT('Ctrl Pts',(-1.32185850051481,-1.18514270861269,
2.32577266001068));
#44701=CARTESIAN_POINT('Ctrl Pts',(-1.35267060678123,-1.06847604194558,
2.34006403729773));
#44702=CARTESIAN_POINT('Ctrl Pts',(-1.39741805963368,-0.794772684000851,
2.39353727746485));
#44703=CARTESIAN_POINT('Ctrl Pts',(-1.38457112325749,-0.636309800095196,
2.46233875769595));
#44704=CARTESIAN_POINT('Ctrl Pts',(-1.39375448302828,-0.319434907277159,
2.53591491365396));
#44705=CARTESIAN_POINT('Ctrl Pts',(-1.38362278588515,-0.158333333333332,
2.58064707201462));
#44706=CARTESIAN_POINT('Ctrl Pts',(-1.41600270610974,0.158333333333334,
2.5906195818525));
#44707=CARTESIAN_POINT('Ctrl Pts',(-1.45995892423147,0.319434907277167,
2.55639080502576));
#44708=CARTESIAN_POINT('Ctrl Pts',(-1.51378858280534,0.636309800095206,
2.50204658614216));
#44709=CARTESIAN_POINT('Ctrl Pts',(-1.56075790439375,0.79477268400084,2.44442825750267));
#44710=CARTESIAN_POINT('Ctrl Pts',(-1.56074958985878,1.06847604194605,2.40274235367243));
#44711=CARTESIAN_POINT('Ctrl Pts',(-1.54630261814451,1.18514270861363,2.39207685648188));
#44712=CARTESIAN_POINT('Ctrl Pts',(-1.51741227377006,1.30000000000274,2.38879014525401));
#44713=CARTESIAN_POINT('Ctrl Pts',(-1.27082599327781,-1.30000000000134,
2.32929506146048));
#44714=CARTESIAN_POINT('Ctrl Pts',(-1.31146501795783,-1.18514270861269,
2.33647493942641));
#44715=CARTESIAN_POINT('Ctrl Pts',(-1.34107385349419,-1.06847604194558,
2.35202967938385));
#44716=CARTESIAN_POINT('Ctrl Pts',(-1.3839942433067,-0.794772684000851,
2.40731184698627));
#44717=CARTESIAN_POINT('Ctrl Pts',(-1.37127685908323,-0.636309800095196,
2.47569309018433));
#44718=CARTESIAN_POINT('Ctrl Pts',(-1.38030676013404,-0.319434907277159,
2.54926598726038));
#44719=CARTESIAN_POINT('Ctrl Pts',(-1.37092683910606,-0.158333333333332,
2.59354411999748));
#44720=CARTESIAN_POINT('Ctrl Pts',(-1.40289766570327,0.158333333333334,
2.60328550699441));
#44721=CARTESIAN_POINT('Ctrl Pts',(-1.44556071014892,0.319434907277167,
2.56921034248006));
#44722=CARTESIAN_POINT('Ctrl Pts',(-1.49898002676599,0.636309800095206,
2.51453974159158));
#44723=CARTESIAN_POINT('Ctrl Pts',(-1.54563126199517,0.79477268400084,2.45721532481951));
#44724=CARTESIAN_POINT('Ctrl Pts',(-1.54752279646356,1.06847604194605,2.41374555903559));
#44725=CARTESIAN_POINT('Ctrl Pts',(-1.53441897429966,1.18514270861363,2.40189018458686));
#44726=CARTESIAN_POINT('Ctrl Pts',(-1.50739255478877,1.30000000000274,2.39699588658379));
#44727=CARTESIAN_POINT('Ctrl Pts',(-1.25382084875496,-1.30000000000134,
2.34740604253439));
#44728=CARTESIAN_POINT('Ctrl Pts',(-1.28972468822729,-1.18514270861269,
2.35739030091737));
#44729=CARTESIAN_POINT('Ctrl Pts',(-1.31607146455883,-1.06847604194558,
2.3750904551144));
#44730=CARTESIAN_POINT('Ctrl Pts',(-1.35485906080004,-0.794772684000855,
2.43380661510325));
#44731=CARTESIAN_POINT('Ctrl Pts',(-1.34486661414017,-0.6363098000952,2.50253171557404));
#44732=CARTESIAN_POINT('Ctrl Pts',(-1.35423783295285,-0.319434907277161,
2.57641427780022));
#44733=CARTESIAN_POINT('Ctrl Pts',(-1.34545299100441,-0.158333333333334,
2.61932084915137));
#44734=CARTESIAN_POINT('Ctrl Pts',(-1.37684147327064,0.158333333333336,
2.62873770546943));
#44735=CARTESIAN_POINT('Ctrl Pts',(-1.41790578277615,0.319434907277172,
2.59551147340387));
#44736=CARTESIAN_POINT('Ctrl Pts',(-1.47065576940973,0.636309800095213,
2.54027367362798));
#44737=CARTESIAN_POINT('Ctrl Pts',(-1.51577444849718,0.794772684000848,
2.48306023107429));
#44738=CARTESIAN_POINT('Ctrl Pts',(-1.52150372805259,1.06847604194606,2.43601887531454));
#44739=CARTESIAN_POINT('Ctrl Pts',(-1.5112701521532,1.18514270861364,2.42186535768253));
#44740=CARTESIAN_POINT('Ctrl Pts',(-1.48832300752561,1.30000000000274,2.41392078227297));
#44741=CARTESIAN_POINT('Ctrl Pts',(-1.23606661107331,-1.30000000000135,
2.36612763766972));
#44742=CARTESIAN_POINT('Ctrl Pts',(-1.26952116487824,-1.1851427086127,2.38014288421496));
#44743=CARTESIAN_POINT('Ctrl Pts',(-1.29391544109559,-1.06847604194558,
2.40071154454898));
#44744=CARTESIAN_POINT('Ctrl Pts',(-1.32934004548617,-0.794772684000857,
2.46336896152491));
#44745=CARTESIAN_POINT('Ctrl Pts',(-1.31845784775975,-0.636309800095201,
2.53067644404618));
#44746=CARTESIAN_POINT('Ctrl Pts',(-1.32710927339012,-0.319434907277161,
2.60436541489617));
#44747=CARTESIAN_POINT('Ctrl Pts',(-1.31985493597403,-0.158333333333333,
2.64631125420172));
#44748=CARTESIAN_POINT('Ctrl Pts',(-1.35060848262527,0.158333333333336,
2.65538195322451));
#44749=CARTESIAN_POINT('Ctrl Pts',(-1.38976931133031,0.319434907277169,
2.62290932667077));
#44750=CARTESIAN_POINT('Ctrl Pts',(-1.44141218068745,0.63630980009521,2.56687682513414));
#44751=CARTESIAN_POINT('Ctrl Pts',(-1.48444786746984,0.794772684000846,
2.5095245660064));
#44752=CARTESIAN_POINT('Ctrl Pts',(-1.49401219558044,1.06847604194606,2.45872137820305));
#44753=CARTESIAN_POINT('Ctrl Pts',(-1.48679726350359,1.18514270861364,2.44221646020226));
#44754=CARTESIAN_POINT('Ctrl Pts',(-1.46822735610409,1.30000000000275,2.4311974417572));
#44755=CARTESIAN_POINT('Ctrl Pts',(-1.22651188656258,-1.30000000000135,
2.37636511902976));
#44756=CARTESIAN_POINT('Ctrl Pts',(-1.25763623352574,-1.1851427086127,2.39212732521069));
#44757=CARTESIAN_POINT('Ctrl Pts',(-1.28039582820086,-1.06847604194559,
2.41400536023505));
#44758=CARTESIAN_POINT('Ctrl Pts',(-1.31365079379327,-0.794772684000859,
2.47867678592274));
#44759=CARTESIAN_POINT('Ctrl Pts',(-1.30374727333792,-0.636309800095202,
2.54590402804441));
#44760=CARTESIAN_POINT('Ctrl Pts',(-1.31267808242576,-0.319434907277161,
2.61981138305767));
#44761=CARTESIAN_POINT('Ctrl Pts',(-1.30636129182997,-0.158333333333333,
2.66127968119591));
#44762=CARTESIAN_POINT('Ctrl Pts',(-1.33678585930284,0.158333333333336,
2.67017251962692));
#44763=CARTESIAN_POINT('Ctrl Pts',(-1.37441375777697,0.31943490727717,2.6378700495204));
#44764=CARTESIAN_POINT('Ctrl Pts',(-1.42564978301686,0.636309800095211,
2.58152070592476));
#44765=CARTESIAN_POINT('Ctrl Pts',(-1.46848285180204,0.794772684000847,
2.52459274777525));
#44766=CARTESIAN_POINT('Ctrl Pts',(-1.48013482532484,1.06847604194606,2.47172882045556));
#44767=CARTESIAN_POINT('Ctrl Pts',(-1.47436292824239,1.18514270861364,2.45382693016231));
#44768=CARTESIAN_POINT('Ctrl Pts',(-1.45777542648761,1.30000000000275,2.44090598491105));
#44769=CARTESIAN_POINT('Ctrl Pts',(-1.22442444283596,-1.30000000000135,
2.37865686158716));
#44770=CARTESIAN_POINT('Ctrl Pts',(-1.25505289579091,-1.1851427086127,2.39481804511272));
#44771=CARTESIAN_POINT('Ctrl Pts',(-1.27746084760478,-1.06847604194559,
2.41699283710455));
#44772=CARTESIAN_POINT('Ctrl Pts',(-1.31023669684865,-0.794772684000858,
2.48211368123284));
#44773=CARTESIAN_POINT('Ctrl Pts',(-1.30050800650126,-0.636309800095202,
2.54930273424566));
#44774=CARTESIAN_POINT('Ctrl Pts',(-1.30948713094632,-0.319434907277161,
2.62325238428033));
#44775=CARTESIAN_POINT('Ctrl Pts',(-1.3033888994581,-0.158333333333333,
2.66461967637659));
#44776=CARTESIAN_POINT('Ctrl Pts',(-1.33374295960405,0.158333333333336,
2.6734746150652));
#44777=CARTESIAN_POINT('Ctrl Pts',(-1.37104104789581,0.31943490727717,2.64121584584354));
#44778=CARTESIAN_POINT('Ctrl Pts',(-1.42216813151107,0.636309800095211,
2.58478653561258));
#44779=CARTESIAN_POINT('Ctrl Pts',(-1.46490901723515,0.794772684000847,
2.52792818187656));
#44780=CARTESIAN_POINT('Ctrl Pts',(-1.47701727843428,1.06847604194606,2.47460218551256));
#44781=CARTESIAN_POINT('Ctrl Pts',(-1.47157205898242,1.18514270861364,2.45639289956961));
#44782=CARTESIAN_POINT('Ctrl Pts',(-1.45544040246087,1.30000000000275,2.44305717558686));
#44783=CARTESIAN_POINT('Ctrl Pts',(-1.22080579827408,-1.30000000000135,
2.38268464037354));
#44784=CARTESIAN_POINT('Ctrl Pts',(-1.25061899143135,-1.1851427086127,2.39956860112986));
#44785=CARTESIAN_POINT('Ctrl Pts',(-1.27244311645034,-1.06847604194558,
2.42227751873145));
#44786=CARTESIAN_POINT('Ctrl Pts',(-1.30440486553836,-0.794772684000858,
2.48819647688559));
#44787=CARTESIAN_POINT('Ctrl Pts',(-1.29492903164232,-0.636309800095202,
2.55529457763855));
#44788=CARTESIAN_POINT('Ctrl Pts',(-1.3039387637522,-0.319434907277161,
2.62929274909087));
#44789=CARTESIAN_POINT('Ctrl Pts',(-1.29815594019608,-0.158333333333334,
2.67045024651218));
#44790=CARTESIAN_POINT('Ctrl Pts',(-1.32838573362059,0.158333333333336,
2.67923917825606));
#44791=CARTESIAN_POINT('Ctrl Pts',(-1.36520310306176,0.31943490727717,2.64710577115188));
#44792=CARTESIAN_POINT('Ctrl Pts',(-1.41613006072221,0.636309800095211,
2.59053101975602));
#44793=CARTESIAN_POINT('Ctrl Pts',(-1.45859660002129,0.794772684000847,
2.53373553247143));
#44794=CARTESIAN_POINT('Ctrl Pts',(-1.4714859764512,1.06847604194606,2.47959175086073));
#44795=CARTESIAN_POINT('Ctrl Pts',(-1.46662397060643,1.18514270861364,2.46085052592493));
#44796=CARTESIAN_POINT('Ctrl Pts',(-1.45132062545884,1.30000000000275,2.44680491288787));
#44797=CARTESIAN_POINT('Ctrl Pts',(-1.21577198318697,-1.30000000000135,
2.38850735409311));
#44798=CARTESIAN_POINT('Ctrl Pts',(-1.24465532214333,-1.1851427086127,2.40653337468798));
#44799=CARTESIAN_POINT('Ctrl Pts',(-1.26578380340772,-1.06847604194558,
2.43006992306755));
#44800=CARTESIAN_POINT('Ctrl Pts',(-1.29667954924419,-0.794772684000858,
2.49717447985452));
#44801=CARTESIAN_POINT('Ctrl Pts',(-1.28729106307725,-0.636309800095202,
2.56401627618933));
#44802=CARTESIAN_POINT('Ctrl Pts',(-1.29612334487574,-0.319434907277161,
2.63797875212365));
#44803=CARTESIAN_POINT('Ctrl Pts',(-1.29056461674117,-0.158333333333333,
2.67872437044246));
#44804=CARTESIAN_POINT('Ctrl Pts',(-1.32062377343709,0.158333333333336,
2.6874253957819));
#44805=CARTESIAN_POINT('Ctrl Pts',(-1.35713237397202,0.319434907277169,
2.65566379602382));
#44806=CARTESIAN_POINT('Ctrl Pts',(-1.4077141062757,0.636309800095211,2.59884824539572));
#44807=CARTESIAN_POINT('Ctrl Pts',(-1.44928781318403,0.794772684000847,
2.54188064926633));
#44808=CARTESIAN_POINT('Ctrl Pts',(-1.46323621952018,1.06847604194606,2.48653823443745));
#44809=CARTESIAN_POINT('Ctrl Pts',(-1.4592733781514,1.18514270861364,2.46707138622253));
#44810=CARTESIAN_POINT('Ctrl Pts',(-1.44530994715028,1.30000000000275,2.45209337053365));
#44811=CARTESIAN_POINT('Ctrl Pts',(-1.20972245596778,-1.30000000000135,
2.39549447794725));
#44812=CARTESIAN_POINT('Ctrl Pts',(-1.237498558214,-1.1851427086127,2.4148965304242));
#44813=CARTESIAN_POINT('Ctrl Pts',(-1.25780946550937,-1.06847604194558,
2.43943527698712));
#44814=CARTESIAN_POINT('Ctrl Pts',(-1.28748563080113,-0.794772684000858,
2.50799148143747));
#44815=CARTESIAN_POINT('Ctrl Pts',(-1.27829104603458,-0.636309800095201,
2.57456596436313));
#44816=CARTESIAN_POINT('Ctrl Pts',(-1.28695534553385,-0.319434907277161,
2.64850621105546));
#44817=CARTESIAN_POINT('Ctrl Pts',(-1.2816533068698,-0.158333333333333,
2.68875081698848));
#44818=CARTESIAN_POINT('Ctrl Pts',(-1.31147697540735,0.158333333333336,
2.69733396568411));
#44819=CARTESIAN_POINT('Ctrl Pts',(-1.34754226237417,0.31943490727717,2.66598781839734));
#44820=CARTESIAN_POINT('Ctrl Pts',(-1.39771277198078,0.636309800095211,
2.60888856392443));
#44821=CARTESIAN_POINT('Ctrl Pts',(-1.43834600690956,0.794772684000846,
2.55178056358252));
#44822=CARTESIAN_POINT('Ctrl Pts',(-1.45351266470549,1.06847604194606,2.49497238712087));
#44823=CARTESIAN_POINT('Ctrl Pts',(-1.450568752393,1.18514270861364,2.47460353456611));
#44824=CARTESIAN_POINT('Ctrl Pts',(-1.43811584358821,1.30000000000275,2.45845598409654));
#44825=CARTESIAN_POINT('Ctrl Pts',(-1.20140969808998,-1.30000000000135,
2.40469480865862));
#44826=CARTESIAN_POINT('Ctrl Pts',(-1.2273339447754,-1.1851427086127,2.42575973931006));
#44827=CARTESIAN_POINT('Ctrl Pts',(-1.24634695325279,-1.06847604194558,
2.45154000943944));
#44828=CARTESIAN_POINT('Ctrl Pts',(-1.27430446352586,-0.794772684000857,
2.52199096825796));
#44829=CARTESIAN_POINT('Ctrl Pts',(-1.2658664144435,-0.636309800095202,
2.58843684601312));
#44830=CARTESIAN_POINT('Ctrl Pts',(-1.27481917442567,-0.319434907277161,
2.66258895868815));
#44831=CARTESIAN_POINT('Ctrl Pts',(-1.2704285554692,-0.158333333333333,
2.70243931345991));
#44832=CARTESIAN_POINT('Ctrl Pts',(-1.29994796313376,0.158333333333336,
2.71086864410593));
#44833=CARTESIAN_POINT('Ctrl Pts',(-1.33461834788419,0.319434907277169,
2.67968218340169));
#44834=CARTESIAN_POINT('Ctrl Pts',(-1.38424570108484,0.636309800095211,
2.62222222152023));
#44835=CARTESIAN_POINT('Ctrl Pts',(-1.42444637983391,0.794772684000847,
2.56536279772913));
#44836=CARTESIAN_POINT('Ctrl Pts',(-1.44132255025392,1.06847604194606,2.50664038232994));
#44837=CARTESIAN_POINT('Ctrl Pts',(-1.4396328321968,1.18514270861364,2.4850086975055));
#44838=CARTESIAN_POINT('Ctrl Pts',(-1.42894832723144,1.30000000000275,2.4671640856031));
#44839=CARTESIAN_POINT('Ctrl Pts',(-1.19097545539289,-1.30000000000135,
2.41618611254718));
#44840=CARTESIAN_POINT('Ctrl Pts',(-1.21459984897074,-1.1851427086127,2.43934036867706));
#44841=CARTESIAN_POINT('Ctrl Pts',(-1.23198527911806,-1.06847604194558,
2.46667277011588));
#44842=CARTESIAN_POINT('Ctrl Pts',(-1.25773584707679,-0.794772684000856,
2.53946843676631));
#44843=CARTESIAN_POINT('Ctrl Pts',(-1.25010458507922,-0.636309800095201,
2.605689091021));
#44844=CARTESIAN_POINT('Ctrl Pts',(-1.25935605916739,-0.319434907277161,
2.68007355808535));
#44845=CARTESIAN_POINT('Ctrl Pts',(-1.25607343829891,-0.158333333333333,
2.71940706193143));
#44846=CARTESIAN_POINT('Ctrl Pts',(-1.28535661586508,0.158333333333336,
2.72771186106723));
#44847=CARTESIAN_POINT('Ctrl Pts',(-1.3186670069989,0.31943490727717,2.69691930460369));
#44848=CARTESIAN_POINT('Ctrl Pts',(-1.36754657543854,0.636309800095211,
2.63897009843824));
#44849=CARTESIAN_POINT('Ctrl Pts',(-1.40664865630924,0.794772684000846,
2.5821337587119));
#44850=CARTESIAN_POINT('Ctrl Pts',(-1.42552979444646,1.06847604194606,2.52095287146528));
#44851=CARTESIAN_POINT('Ctrl Pts',(-1.42543679622289,1.18514270861364,2.49775939915589));
#44852=CARTESIAN_POINT('Ctrl Pts',(-1.41707785469123,1.30000000000275,2.477855393651));
#44853=CARTESIAN_POINT('Ctrl Pts',(-1.17502706764918,-1.30000000000135,
2.43492203179261));
#44854=CARTESIAN_POINT('Ctrl Pts',(-1.19560300398521,-1.1851427086127,2.4617154878452));
#44855=CARTESIAN_POINT('Ctrl Pts',(-1.21082849739992,-1.06847604194558,
2.49173942274355));
#44856=CARTESIAN_POINT('Ctrl Pts',(-1.23364183953669,-0.794772684000853,
2.56856377101498));
#44857=CARTESIAN_POINT('Ctrl Pts',(-1.22731190864551,-0.636309800095201,
2.63442149983078));
#44858=CARTESIAN_POINT('Ctrl Pts',(-1.23645105326258,-0.319434907277162,
2.70890849458993));
#44859=CARTESIAN_POINT('Ctrl Pts',(-1.23384956357613,-0.158333333333333,
2.74691835519408));
#44860=CARTESIAN_POINT('Ctrl Pts',(-1.26201512338157,0.158333333333336,
2.75469106909033));
#44861=CARTESIAN_POINT('Ctrl Pts',(-1.29284074214967,0.319434907277169,
2.72437826502062));
#44862=CARTESIAN_POINT('Ctrl Pts',(-1.34095351347016,0.636309800095211,
2.66587783741269));
#44863=CARTESIAN_POINT('Ctrl Pts',(-1.37977554459473,0.794772684000847,
2.60983700343105));
#44864=CARTESIAN_POINT('Ctrl Pts',(-1.40211676589996,1.06847604194606,2.54483262312023));
#44865=CARTESIAN_POINT('Ctrl Pts',(-1.40441378045019,1.18514270861364,2.51904198433771));
#44866=CARTESIAN_POINT('Ctrl Pts',(-1.39933712267143,1.30000000000275,2.49559869435967));
#44867=CARTESIAN_POINT('Ctrl Pts',(-1.15904906517621,-1.30000000000135,
2.4536662687705));
#44868=CARTESIAN_POINT('Ctrl Pts',(-1.17661739972832,-1.1851427086127,2.48411798698703));
#44869=CARTESIAN_POINT('Ctrl Pts',(-1.18960431632116,-1.06847604194559,
2.51679950600914));
#44870=CARTESIAN_POINT('Ctrl Pts',(-1.20902269967893,-0.794772684000857,
2.59745163879659));
#44871=CARTESIAN_POINT('Ctrl Pts',(-1.20286196424972,-0.6363098000952,2.66244534596457));
#44872=CARTESIAN_POINT('Ctrl Pts',(-1.21188397483891,-0.31943490727716,
2.73703530247258));
#44873=CARTESIAN_POINT('Ctrl Pts',(-1.21065438480207,-0.158333333333333,
2.77401500061943));
#44874=CARTESIAN_POINT('Ctrl Pts',(-1.23889099773402,0.158333333333335,
2.78181435464434));
#44875=CARTESIAN_POINT('Ctrl Pts',(-1.26888848540362,0.319434907277168,
2.75279259424705));
#44876=CARTESIAN_POINT('Ctrl Pts',(-1.31630023357142,0.636309800095209,
2.69376633668697));
#44877=CARTESIAN_POINT('Ctrl Pts',(-1.352883146608,0.794772684000843,2.6375618120723));
#44878=CARTESIAN_POINT('Ctrl Pts',(-1.37811171409883,1.06847604194606,2.56845034247818));
#44879=CARTESIAN_POINT('Ctrl Pts',(-1.38279858713534,1.18514270861364,2.54006106243875));
#44880=CARTESIAN_POINT('Ctrl Pts',(-1.38125182115209,1.30000000000275,2.51319829671497));
#44881=CARTESIAN_POINT('Ctrl Pts',(-1.14511474947587,-1.30000000000135,
2.47009903743856));
#44882=CARTESIAN_POINT('Ctrl Pts',(-1.15981125650959,-1.1851427086127,2.50366280614491));
#44883=CARTESIAN_POINT('Ctrl Pts',(-1.17089890385113,-1.06847604194558,
2.53870677723349));
#44884=CARTESIAN_POINT('Ctrl Pts',(-1.1881763994475,-0.794772684000857,
2.62308492458678));
#44885=CARTESIAN_POINT('Ctrl Pts',(-1.18438946463272,-0.636309800095201,
2.68828438577407));
#44886=CARTESIAN_POINT('Ctrl Pts',(-1.19381691865822,-0.31943490727716,
2.76318909900355));
#44887=CARTESIAN_POINT('Ctrl Pts',(-1.19285882411596,-0.158333333333333,
2.79887261784234));
#44888=CARTESIAN_POINT('Ctrl Pts',(-1.21995946483943,0.158333333333335,
2.80616514085504));
#44889=CARTESIAN_POINT('Ctrl Pts',(-1.24796444411868,0.319434907277168,
2.77770066340956));
#44890=CARTESIAN_POINT('Ctrl Pts',(-1.29384854100992,0.636309800095209,
2.71779997124574));
#44891=CARTESIAN_POINT('Ctrl Pts',(-1.32848976308691,0.794772684000844,
2.66145357782913));
#44892=CARTESIAN_POINT('Ctrl Pts',(-1.35641019534391,1.06847604194606,2.58881860913373));
#44893=CARTESIAN_POINT('Ctrl Pts',(-1.36338321274031,1.18514270861364,2.55824206200308));
#44894=CARTESIAN_POINT('Ctrl Pts',(-1.36524352696298,1.30000000000275,2.52852995429933));
#44895=CARTESIAN_POINT('Ctrl Pts',(-1.13743240009045,-1.30000000000135,
2.47962282172612));
#44896=CARTESIAN_POINT('Ctrl Pts',(-1.1509959570983,-1.1851427086127,2.5151804811712));
#44897=CARTESIAN_POINT('Ctrl Pts',(-1.16118204640611,-1.06847604194558,
2.55165123117717));
#44898=CARTESIAN_POINT('Ctrl Pts',(-1.17691132438011,-0.794772684000856,
2.63801538149813));
#44899=CARTESIAN_POINT('Ctrl Pts',(-1.1726240599699,-0.6363098000952,2.70253446010115));
#44900=CARTESIAN_POINT('Ctrl Pts',(-1.18192552938848,-0.31943490727716,
2.77746372964283));
#44901=CARTESIAN_POINT('Ctrl Pts',(-1.18191990276965,-0.158333333333333,
2.81274083764786));
#44902=CARTESIAN_POINT('Ctrl Pts',(-1.20919352209051,0.158333333333335,
2.82011139846522));
#44903=CARTESIAN_POINT('Ctrl Pts',(-1.23670432785443,0.319434907277169,
2.79225951297756));
#44904=CARTESIAN_POINT('Ctrl Pts',(-1.28248558653756,0.636309800095209,
2.73223220317571));
#44905=CARTESIAN_POINT('Ctrl Pts',(-1.3165906333875,0.794772684000844,2.67611720090248));
#44906=CARTESIAN_POINT('Ctrl Pts',(-1.34585334028077,1.06847604194606,2.60137585827352));
#44907=CARTESIAN_POINT('Ctrl Pts',(-1.35381729827139,1.18514270861364,2.56939118976514));
#44908=CARTESIAN_POINT('Ctrl Pts',(-1.35707847272864,1.30000000000275,2.5377746105329));
#44909=CARTESIAN_POINT('Ctrl Pts',(-1.12587093071343,-1.30000000000135,
2.49388678129842));
#44910=CARTESIAN_POINT('Ctrl Pts',(-1.13743996805866,-1.1851427086127,2.5323131421853));
#44911=CARTESIAN_POINT('Ctrl Pts',(-1.14620340056342,-1.06847604194558,
2.57089746517517));
#44912=CARTESIAN_POINT('Ctrl Pts',(-1.15996717432731,-0.794772684000856,
2.66039989410707));
#44913=CARTESIAN_POINT('Ctrl Pts',(-1.15625211606956,-0.6363098000952,2.7244683950529));
#44914=CARTESIAN_POINT('Ctrl Pts',(-1.16583526707528,-0.31943490727716,
2.79963620118662));
#44915=CARTESIAN_POINT('Ctrl Pts',(-1.16728340571542,-0.158333333333333,
2.83431784556207));
#44916=CARTESIAN_POINT('Ctrl Pts',(-1.19374519866423,0.158333333333335,
2.84132697013958));
#44917=CARTESIAN_POINT('Ctrl Pts',(-1.2185960758806,0.319434907277168,2.81354432854277));
#44918=CARTESIAN_POINT('Ctrl Pts',(-1.26324525701596,0.636309800095209,
2.75287791467498));
#44919=CARTESIAN_POINT('Ctrl Pts',(-1.29706389338153,0.794772684000844,
2.69730718173339));
#44920=CARTESIAN_POINT('Ctrl Pts',(-1.3285043772527,1.06847604194606,2.61948048286637));
#44921=CARTESIAN_POINT('Ctrl Pts',(-1.33805819666283,1.18514270861364,2.58543820887738));
#44922=CARTESIAN_POINT('Ctrl Pts',(-1.34355641499993,1.30000000000275,2.55104195507566));
#44923=CARTESIAN_POINT('Ctrl Pts',(-1.10877976373815,-1.30000000000134,
2.51539512337627));
#44924=CARTESIAN_POINT('Ctrl Pts',(-1.11700749000313,-1.18514270861269,
2.55799245825637));
#44925=CARTESIAN_POINT('Ctrl Pts',(-1.12347620234645,-1.06847604194558,
2.59968793273419));
#44926=CARTESIAN_POINT('Ctrl Pts',(-1.13435654787238,-0.794772684000852,
2.69392934198306));
#44927=CARTESIAN_POINT('Ctrl Pts',(-1.13261330572799,-0.636309800095198,
2.75776369374303));
#44928=CARTESIAN_POINT('Ctrl Pts',(-1.14248599893863,-0.31943490727716,
2.83322910662972));
#44929=CARTESIAN_POINT('Ctrl Pts',(-1.14444452168738,-0.158333333333333,
2.86630795981827));
#44930=CARTESIAN_POINT('Ctrl Pts',(-1.17037651905704,0.158333333333335,
2.87310697666088));
#44931=CARTESIAN_POINT('Ctrl Pts',(-1.19418540652733,0.319434907277169,
2.84675453602205));
#44932=CARTESIAN_POINT('Ctrl Pts',(-1.23746957696803,0.636309800095209,
2.78528612061526));
#44933=CARTESIAN_POINT('Ctrl Pts',(-1.26831972181169,0.794772684000843,
2.72939423054381));
#44934=CARTESIAN_POINT('Ctrl Pts',(-1.30248061882999,1.06847604194605,2.64668881184621));
#44935=CARTESIAN_POINT('Ctrl Pts',(-1.31452253467142,1.18514270861363,2.60960180882215));
#44936=CARTESIAN_POINT('Ctrl Pts',(-1.32381937982096,1.30000000000274,2.57122791399057));
#44937=CARTESIAN_POINT('Ctrl Pts',(-1.08708000619844,-1.30000000000135,
2.5445357914544));
#44938=CARTESIAN_POINT('Ctrl Pts',(-1.09153397709107,-1.1851427086127,2.59298467877558));
#44939=CARTESIAN_POINT('Ctrl Pts',(-1.09529707688984,-1.06847604194558,
2.63898235718083));
#44940=CARTESIAN_POINT('Ctrl Pts',(-1.10239453979543,-0.794772684000857,
2.73958341314233));
#44941=CARTESIAN_POINT('Ctrl Pts',(-1.10156616025283,-0.636309800095197,
2.80240803093196));
#44942=CARTESIAN_POINT('Ctrl Pts',(-1.11201856565858,-0.319434907277157,
2.87835347963024));
#44943=CARTESIAN_POINT('Ctrl Pts',(-1.11656121087504,-0.158333333333332,
2.91006832634054));
#44944=CARTESIAN_POINT('Ctrl Pts',(-1.14185015937106,0.158333333333334,
2.91661637012575));
#44945=CARTESIAN_POINT('Ctrl Pts',(-1.16236219873307,0.319434907277167,
2.89137191942179));
#44946=CARTESIAN_POINT('Ctrl Pts',(-1.20389873928152,0.636309800095206,
2.82892252737393));
#44947=CARTESIAN_POINT('Ctrl Pts',(-1.23300565158259,0.794772684000839,
2.77365267741555));
#44948=CARTESIAN_POINT('Ctrl Pts',(-1.27070968714585,1.06847604194605,2.68440060237138));
#44949=CARTESIAN_POINT('Ctrl Pts',(-1.28557693600659,1.18514270861364,2.6430140566728));
#44950=CARTESIAN_POINT('Ctrl Pts',(-1.29899075380489,1.30000000000275,2.59887488144712));
#44951=CARTESIAN_POINT('Ctrl Pts',(-1.06835320849412,-1.30000000000135,
2.56859872678655));
#44952=CARTESIAN_POINT('Ctrl Pts',(-1.0697813225491,-1.18514270861269,2.62196120870789));
#44953=CARTESIAN_POINT('Ctrl Pts',(-1.07155378605604,-1.06847604194558,
2.67163925621292));
#44954=CARTESIAN_POINT('Ctrl Pts',(-1.07644404745808,-0.79477268400085,
2.77789370343844));
#44955=CARTESIAN_POINT('Ctrl Pts',(-1.07803733404953,-0.636309800095198,
2.84052147891033));
#44956=CARTESIAN_POINT('Ctrl Pts',(-1.08928731240602,-0.31943490727716,
2.91697449291878));
#44957=CARTESIAN_POINT('Ctrl Pts',(-1.09475033976786,-0.158333333333333,
2.9470431617148));
#44958=CARTESIAN_POINT('Ctrl Pts',(-1.11909912332319,0.158333333333335,
2.95324376931968));
#44959=CARTESIAN_POINT('Ctrl Pts',(-1.13758418362336,0.319434907277168,
2.92928290322638));
#44960=CARTESIAN_POINT('Ctrl Pts',(-1.17674711288214,0.636309800095208,
2.86564911735402));
#44961=CARTESIAN_POINT('Ctrl Pts',(-1.20212657848975,0.794772684000843,
2.80989517576845));
#44962=CARTESIAN_POINT('Ctrl Pts',(-1.24245750708116,1.06847604194606,2.71506152057097));
#44963=CARTESIAN_POINT('Ctrl Pts',(-1.25999884660707,1.18514270861364,2.67024063466379));
#44964=CARTESIAN_POINT('Ctrl Pts',(-1.27762376107978,1.30000000000274,2.62164883825135));
#44965=CARTESIAN_POINT('Ctrl Pts',(-1.05521937382473,-1.30000000000134,
2.58857464166986));
#44966=CARTESIAN_POINT('Ctrl Pts',(-1.05450214504509,-1.18514270861269,
2.64600090835846));
#44967=CARTESIAN_POINT('Ctrl Pts',(-1.0547849652932,-1.06847604194558,2.69868073338192));
#44968=CARTESIAN_POINT('Ctrl Pts',(-1.05774864995755,-0.79477268400085,
2.80941643797989));
#44969=CARTESIAN_POINT('Ctrl Pts',(-1.06047170225705,-0.636309800095197,
2.87155013435134));
#44970=CARTESIAN_POINT('Ctrl Pts',(-1.07184295676916,-0.319434907277159,
2.94821501020616));
#44971=CARTESIAN_POINT('Ctrl Pts',(-1.07789632591925,-0.158333333333333,
2.97692628369926));
#44972=CARTESIAN_POINT('Ctrl Pts',(-1.10146318465323,0.158333333333335,
2.9828505963045));
#44973=CARTESIAN_POINT('Ctrl Pts',(-1.11825852721492,0.319434907277168,
2.95986988768039));
#44974=CARTESIAN_POINT('Ctrl Pts',(-1.15635408084972,0.636309800095208,
2.89566706022621));
#44975=CARTESIAN_POINT('Ctrl Pts',(-1.1806416071217,0.79477268400084,2.84040087167772));
#44976=CARTESIAN_POINT('Ctrl Pts',(-1.22293951039675,1.06847604194605,2.74103002569047));
#44977=CARTESIAN_POINT('Ctrl Pts',(-1.24208305449305,1.18514270861364,2.69320736685689));
#44978=CARTESIAN_POINT('Ctrl Pts',(-1.26206094764959,1.30000000000275,2.64057600636506));
#44979=CARTESIAN_POINT('Ctrl Pts',(-1.03796310307453,-1.30000000000135,
2.61321937129804));
#44980=CARTESIAN_POINT('Ctrl Pts',(-1.03433234523134,-1.18514270861269,
2.67561294783302));
#44981=CARTESIAN_POINT('Ctrl Pts',(-1.03271434407037,-1.06847604194558,
2.73201023194115));
#44982=CARTESIAN_POINT('Ctrl Pts',(-1.033626308295,-0.794772684000851,2.84844660540857));
#44983=CARTESIAN_POINT('Ctrl Pts',(-1.03850907849285,-0.6363098000952,2.91024159152785));
#44984=CARTESIAN_POINT('Ctrl Pts',(-1.05131116122678,-0.319434907277162,
2.98762987114524));
#44985=CARTESIAN_POINT('Ctrl Pts',(-1.05962760847544,-0.158333333333333,
3.01518593090444));
#44986=CARTESIAN_POINT('Ctrl Pts',(-1.08233494867452,0.158333333333335,
3.02082749843731));
#44987=CARTESIAN_POINT('Ctrl Pts',(-1.09569345115491,0.319434907277167,
2.99864727175407));
#44988=CARTESIAN_POINT('Ctrl Pts',(-1.13124749047663,0.636309800095208,
2.93329174095001));
#44989=CARTESIAN_POINT('Ctrl Pts',(-1.15328508084511,0.794772684000849,
2.8782315917722));
#44990=CARTESIAN_POINT('Ctrl Pts',(-1.19758716438919,1.06847604194606,2.77303275852799));
#44991=CARTESIAN_POINT('Ctrl Pts',(-1.21872779041347,1.18514270861363,2.7214776851753));
#44992=CARTESIAN_POINT('Ctrl Pts',(-1.24183231204969,1.30000000000274,2.66390421538058));
#44993=CARTESIAN_POINT('Ctrl Pts',(-1.02154978498825,-1.30000000000134,
2.63823699667444));
#44994=CARTESIAN_POINT('Ctrl Pts',(-1.01574801095058,-1.18514270861269,
2.70592424384903));
#44995=CARTESIAN_POINT('Ctrl Pts',(-1.01274478987735,-1.06847604194558,
2.76626480042087));
#44996=CARTESIAN_POINT('Ctrl Pts',(-1.01227196560235,-0.794772684000852,
2.88869123219581));
#44997=CARTESIAN_POINT('Ctrl Pts',(-1.01930980404299,-0.636309800095198,
2.95010834994269));
#44998=CARTESIAN_POINT('Ctrl Pts',(-1.03274236210258,-0.319434907277159,
3.02792458695197));
#44999=CARTESIAN_POINT('Ctrl Pts',(-1.04142778207386,-0.158333333333333,
3.05362693099543));
#45000=CARTESIAN_POINT('Ctrl Pts',(-1.06328150122981,0.158333333333335,
3.05901061254694));
#45001=CARTESIAN_POINT('Ctrl Pts',(-1.07529158151554,0.319434907277169,
3.03843229550797));
#45002=CARTESIAN_POINT('Ctrl Pts',(-1.10873268435927,0.636309800095208,
2.97211112779765));
#45003=CARTESIAN_POINT('Ctrl Pts',(-1.12729379095584,0.794772684000842,
2.91684284841793));
#45004=CARTESIAN_POINT('Ctrl Pts',(-1.17336497585264,1.06847604194605,2.80568738725448));
#45005=CARTESIAN_POINT('Ctrl Pts',(-1.19654495568478,1.18514270861363,2.75037781389277));
#45006=CARTESIAN_POINT('Ctrl Pts',(-1.22296240651279,1.30000000000274,2.68787374759144));
#45007=CARTESIAN_POINT('Ctrl Pts',(-1.00569178470089,-1.30000000000134,
2.66339442293999));
#45008=CARTESIAN_POINT('Ctrl Pts',(-0.997606978305174,-1.18514270861269,
2.73622462125294));
#45009=CARTESIAN_POINT('Ctrl Pts',(-0.993275950842555,-1.06847604194558,
2.8004366432757));
#45010=CARTESIAN_POINT('Ctrl Pts',(-0.991942391261186,-0.794772684000851,
2.92886954842842));
#45011=CARTESIAN_POINT('Ctrl Pts',(-1.00208124996111,-0.6363098000952,2.99016914190514));
#45012=CARTESIAN_POINT('Ctrl Pts',(-1.01716774717545,-0.319434907277161,
3.06873680081757));
#45013=CARTESIAN_POINT('Ctrl Pts',(-1.02709000963087,-0.158333333333333,
3.09295577357895));
#45014=CARTESIAN_POINT('Ctrl Pts',(-1.04799004253004,0.158333333333335,
3.0980870815083));
#45015=CARTESIAN_POINT('Ctrl Pts',(-1.05741527487675,0.319434907277167,
3.07866838013204));
#45016=CARTESIAN_POINT('Ctrl Pts',(-1.0880630481429,0.636309800095208,3.01122712361042));
#45017=CARTESIAN_POINT('Ctrl Pts',(-1.10367721439058,0.794772684000846,
2.95603375362214));
#45018=CARTESIAN_POINT('Ctrl Pts',(-1.15053474805594,1.06847604194606,2.83869111901186));
#45019=CARTESIAN_POINT('Ctrl Pts',(-1.17507666076872,1.18514270861364,2.77943677977267));
#45020=CARTESIAN_POINT('Ctrl Pts',(-1.20387759611321,1.30000000000274,2.71172137984417));
#45021=CARTESIAN_POINT('Ctrl Pts',(-0.996652854808941,-1.30000000000134,
2.67874859209622));
#45022=CARTESIAN_POINT('Ctrl Pts',(-0.987235389768998,-1.18514270861269,
2.75484304608189));
#45023=CARTESIAN_POINT('Ctrl Pts',(-0.982190625604162,-1.06847604194558,
2.821528134996));
#45024=CARTESIAN_POINT('Ctrl Pts',(-0.980638024959095,-0.794772684000851,
2.95384651504136));
#45025=CARTESIAN_POINT('Ctrl Pts',(-0.993843850297619,-0.636309800095197,
3.01544607135719));
#45026=CARTESIAN_POINT('Ctrl Pts',(-1.00867880744322,-0.319434907277159,
3.09407798413982));
#45027=CARTESIAN_POINT('Ctrl Pts',(-1.01591199130173,-0.158333333333333,
3.11624435624655));
#45028=CARTESIAN_POINT('Ctrl Pts',(-1.03574610618998,0.158333333333335,
3.12107189416699));
#45029=CARTESIAN_POINT('Ctrl Pts',(-1.04619476393307,0.319434907277169,
3.10325045211595));
#45030=CARTESIAN_POINT('Ctrl Pts',(-1.07614449642726,0.636309800095208,
3.0354349239545));
#45031=CARTESIAN_POINT('Ctrl Pts',(-1.08941717942122,0.794772684000842,
2.98008553500352));
#45032=CARTESIAN_POINT('Ctrl Pts',(-1.13692092038242,1.06847604194605,2.85890915084214));
#45033=CARTESIAN_POINT('Ctrl Pts',(-1.16240855078136,1.18514270861363,2.79721822163055));
#45034=CARTESIAN_POINT('Ctrl Pts',(-1.19282120230414,1.30000000000274,2.7262891298835));
#45035=CARTESIAN_POINT('Ctrl Pts',(-0.988985336877648,-1.30000000000134,
2.69137107011124));
#45036=CARTESIAN_POINT('Ctrl Pts',(-0.979333756628179,-1.18514270861269,
2.77022516793836));
#45037=CARTESIAN_POINT('Ctrl Pts',(-0.973943685309453,-1.06847604194558,
2.83886483367411));
#45038=CARTESIAN_POINT('Ctrl Pts',(-0.971336480425084,-0.794772684000853,
2.97383881132026));
#45039=CARTESIAN_POINT('Ctrl Pts',(-0.983182267165968,-0.636309800095197,
3.03441947199261));
#45040=CARTESIAN_POINT('Ctrl Pts',(-0.997214190673696,-0.319434907277159,
3.11282563491179));
#45041=CARTESIAN_POINT('Ctrl Pts',(-1.00444416170132,-0.158333333333332,
3.13400485249189));
#45042=CARTESIAN_POINT('Ctrl Pts',(-1.02482927490377,0.158333333333335,
3.13902963959976));
#45043=CARTESIAN_POINT('Ctrl Pts',(-1.03666257867743,0.319434907277168,
3.12266994496896));
#45044=CARTESIAN_POINT('Ctrl Pts',(-1.0668461526339,0.636309800095207,3.0549170199033));
#45045=CARTESIAN_POINT('Ctrl Pts',(-1.07844903019705,0.794772684000841,
2.99962093111457));
#45046=CARTESIAN_POINT('Ctrl Pts',(-1.12660470913759,1.06847604194605,2.87562122050712));
#45047=CARTESIAN_POINT('Ctrl Pts',(-1.15281925740509,1.18514270861363,2.8120697940746));
#45048=CARTESIAN_POINT('Ctrl Pts',(-1.18440354487041,1.30000000000274,2.73864182128965));
#45049=CARTESIAN_POINT('Ctrl Pts',(-0.98053380401763,-1.30000000000134,
2.70691834098162));
#45050=CARTESIAN_POINT('Ctrl Pts',(-0.970516247771153,-1.18514270861269,
2.78946589370654));
#45051=CARTESIAN_POINT('Ctrl Pts',(-0.964456204955913,-1.06847604194558,
2.86069494939743));
#45052=CARTESIAN_POINT('Ctrl Pts',(-0.959598941469317,-0.794772684000851,
2.99910032496074));
#45053=CARTESIAN_POINT('Ctrl Pts',(-0.968405938412429,-0.636309800095197,
3.05813977615298));
#45054=CARTESIAN_POINT('Ctrl Pts',(-0.980318422822977,-0.319434907277159,
3.13605005232135));
#45055=CARTESIAN_POINT('Ctrl Pts',(-0.987526841201364,-0.158333333333332,
3.15590188031775));
#45056=CARTESIAN_POINT('Ctrl Pts',(-1.00780526691801,0.158333333333334,
3.16091545903217));
#45057=CARTESIAN_POINT('Ctrl Pts',(-1.01986572741626,0.319434907277167,
3.14599156573793));
#45058=CARTESIAN_POINT('Ctrl Pts',(-1.05131531031871,0.636309800095207,
3.07846803910757));
#45059=CARTESIAN_POINT('Ctrl Pts',(-1.06417222310146,0.794772684000841,
3.02411831903424));
#45060=CARTESIAN_POINT('Ctrl Pts',(-1.11441663505319,1.06847604194605,2.89657730305442));
#45061=CARTESIAN_POINT('Ctrl Pts',(-1.14162671491763,1.18514270861363,2.83050655264808));
#45062=CARTESIAN_POINT('Ctrl Pts',(-1.17429793045148,1.30000000000274,2.75357283179291));
#45063=CARTESIAN_POINT('Ctrl Pts',(-0.974665092423499,-1.30000000000134,
2.71746251872114));
#45064=CARTESIAN_POINT('Ctrl Pts',(-0.965682205213172,-1.18514270861269,
2.80294609442062));
#45065=CARTESIAN_POINT('Ctrl Pts',(-0.959681817346756,-1.06847604194558,
2.87601139807284));
#45066=CARTESIAN_POINT('Ctrl Pts',(-0.952709891133253,-0.794772684000851,
3.01611817347715));
#45067=CARTESIAN_POINT('Ctrl Pts',(-0.955698270378832,-0.636309800095196,
3.07217548853748));
#45068=CARTESIAN_POINT('Ctrl Pts',(-0.964465402259397,-0.319434907277159,
3.14860911293493));
#45069=CARTESIAN_POINT('Ctrl Pts',(-0.972209900210543,-0.158333333333332,
3.16753349812413));
#45070=CARTESIAN_POINT('Ctrl Pts',(-0.992336747193892,0.158333333333334,
3.17245788736581));
#45071=CARTESIAN_POINT('Ctrl Pts',(-1.00385002392357,0.319434907277167,
3.15835068493109));
#45072=CARTESIAN_POINT('Ctrl Pts',(-1.03785006787198,0.636309800095206,
3.09216605874643));
#45073=CARTESIAN_POINT('Ctrl Pts',(-1.05542731230797,0.79477268400084,3.04072080217647));
#45074=CARTESIAN_POINT('Ctrl Pts',(-1.10785601153169,1.06847604194605,2.9114906887883));
#45075=CARTESIAN_POINT('Ctrl Pts',(-1.1353239790356,1.18514270861363,2.84362042448228));
#45076=CARTESIAN_POINT('Ctrl Pts',(-1.16756547282413,1.30000000000274,2.76381882350857));
#45077=CARTESIAN_POINT('Ctrl Pts',(-0.968408877628683,-1.30000000000134,
2.72336636313462));
#45078=CARTESIAN_POINT('Ctrl Pts',(-0.959587680307202,-1.18514270861269,
2.80865755213462));
#45079=CARTESIAN_POINT('Ctrl Pts',(-0.953418388257857,-1.06847604194558,
2.88142219435957));
#45080=CARTESIAN_POINT('Ctrl Pts',(-0.945292521151705,-0.794772684000851,
3.02058424543828));
#45081=CARTESIAN_POINT('Ctrl Pts',(-0.94601257756158,-0.636309800095196,
3.07544248806072));
#45082=CARTESIAN_POINT('Ctrl Pts',(-0.953320013133083,-0.319434907277159,
3.151031219842));
#45083=CARTESIAN_POINT('Ctrl Pts',(-0.961064002623635,-0.158333333333332,
3.17000794893273));
#45084=CARTESIAN_POINT('Ctrl Pts',(-0.98099760953902,0.158333333333334,
3.17479542438189));
#45085=CARTESIAN_POINT('Ctrl Pts',(-0.992074216468526,0.319434907277167,
3.16036137717658));
#45086=CARTESIAN_POINT('Ctrl Pts',(-1.0276372251559,0.636309800095206,3.09502301503918));
#45087=CARTESIAN_POINT('Ctrl Pts',(-1.04845566442809,0.79477268400084,3.04525442796451));
#45088=CARTESIAN_POINT('Ctrl Pts',(-1.10189571121762,1.06847604194605,2.91691192436669));
#45089=CARTESIAN_POINT('Ctrl Pts',(-1.12924033300979,1.18514270861363,2.84921214392821));
#45090=CARTESIAN_POINT('Ctrl Pts',(-1.16079736048773,1.30000000000274,2.76936729730053));
#45091=CARTESIAN_POINT('Ctrl Pts',(-0.96840887762858,-1.3,2.72336636313561));
#45092=CARTESIAN_POINT('Ctrl Pts',(-0.959587680307154,-1.18514270861178,
2.80865755213519));
#45093=CARTESIAN_POINT('Ctrl Pts',(-0.953418388257844,-1.06847604194512,
2.88142219435981));
#45094=CARTESIAN_POINT('Ctrl Pts',(-0.945292521151705,-0.794772684000851,
3.02058424543828));
#45095=CARTESIAN_POINT('Ctrl Pts',(-0.94601257756158,-0.636309800095197,
3.07544248806072));
#45096=CARTESIAN_POINT('Ctrl Pts',(-0.953320013133083,-0.319434907277159,
3.151031219842));
#45097=CARTESIAN_POINT('Ctrl Pts',(-0.961064002623635,-0.158333333333332,
3.17000794893273));
#45098=CARTESIAN_POINT('Ctrl Pts',(-0.98099760953902,0.158333333333334,
3.17479542438189));
#45099=CARTESIAN_POINT('Ctrl Pts',(-0.992074216468526,0.319434907277167,
3.16036137717658));
#45100=CARTESIAN_POINT('Ctrl Pts',(-1.0276372251559,0.636309800095206,3.09502301503918));
#45101=CARTESIAN_POINT('Ctrl Pts',(-1.04845566442809,0.79477268400084,3.04525442796451));
#45102=CARTESIAN_POINT('Ctrl Pts',(-1.10189571121744,1.06847604194511,2.91691192436713));
#45103=CARTESIAN_POINT('Ctrl Pts',(-1.12924033300935,1.18514270861178,2.84921214392929));
#45104=CARTESIAN_POINT('Ctrl Pts',(-1.16079736048697,1.3,2.76936729730244));
#45105=CARTESIAN_POINT('',(-1.23744115436766,-1.2,2.40716791557672));
#45106=CARTESIAN_POINT('Ctrl Pts',(-1.23744115436766,-1.2,2.40716791557672));
#45107=CARTESIAN_POINT('Ctrl Pts',(-1.21281665208152,-1.22396325414416,
2.42555928291992));
#45108=CARTESIAN_POINT('Ctrl Pts',(-1.18823777366837,-1.2466437811891,2.44279487554561));
#45109=CARTESIAN_POINT('Ctrl Pts',(-1.16766532598256,-1.26666346483997,
2.45830035953809));
#45110=CARTESIAN_POINT('Ctrl Pts',(-1.15334387624282,-1.28037911840962,
2.46890623939148));
#45111=CARTESIAN_POINT('Ctrl Pts',(-1.13360931448736,-1.30000000000135,
2.48434204780559));
#45112=CARTESIAN_POINT('',(-1.38832545990542,-0.653834841419392,2.44867887665694));
#45113=CARTESIAN_POINT('Ctrl Pts',(-1.38832545991004,-0.653834841418722,
2.44867887663172));
#45114=CARTESIAN_POINT('Ctrl Pts',(-1.37270162777471,-0.717985758094171,
2.44411362764694));
#45115=CARTESIAN_POINT('Ctrl Pts',(-1.35994621619342,-0.764036487774388,
2.44044932934856));
#45116=CARTESIAN_POINT('Ctrl Pts',(-1.31012606770028,-0.949550441354697,
2.42639500235851));
#45117=CARTESIAN_POINT('Ctrl Pts',(-1.28369169731409,-1.04640534543883,
2.41910914870269));
#45118=CARTESIAN_POINT('Ctrl Pts',(-1.23744115436766,-1.2,2.40716791557672));
#45119=CARTESIAN_POINT('',(-1.52166805320867,0.653834841531101,2.48968935888044));
#45120=CARTESIAN_POINT('Ctrl Pts',(-1.52166805320867,0.653834841531103,
2.48968935888044));
#45121=CARTESIAN_POINT('Ctrl Pts',(-1.49343059891966,0.57602138259582,2.52017174762599));
#45122=CARTESIAN_POINT('Ctrl Pts',(-1.4690466730557,0.493680047789112,2.54546585877262));
#45123=CARTESIAN_POINT('Ctrl Pts',(-1.43213691154417,0.338203658968698,
2.58010273751869));
#45124=CARTESIAN_POINT('Ctrl Pts',(-1.41824662923231,0.265719696696191,
2.59141317455489));
#45125=CARTESIAN_POINT('Ctrl Pts',(-1.39691207797798,0.129748505774919,
2.60327111496509));
#45126=CARTESIAN_POINT('Ctrl Pts',(-1.38884650422918,0.0666446497396744,
2.60515759811574));
#45127=CARTESIAN_POINT('Ctrl Pts',(-1.37599030069352,-0.0595546290449114,
2.6015928052966));
#45128=CARTESIAN_POINT('Ctrl Pts',(-1.37109828489627,-0.122804233593781,
2.59613105082614));
#45129=CARTESIAN_POINT('Ctrl Pts',(-1.36475418668873,-0.260164762898064,
2.57638174285244));
#45130=CARTESIAN_POINT('Ctrl Pts',(-1.3640889993582,-0.333966755798492,
2.56066651484078));
#45131=CARTESIAN_POINT('Ctrl Pts',(-1.36961752260919,-0.491159093464661,
2.51618010434666));
#45132=CARTESIAN_POINT('Ctrl Pts',(-1.37686721292842,-0.574266001747902,
2.48547919212961));
#45133=CARTESIAN_POINT('Ctrl Pts',(-1.38832545986823,-0.653834841430835,
2.4486788766701));
#45134=CARTESIAN_POINT('',(-1.45284569372596,1.2,2.46800894017942));
#45135=CARTESIAN_POINT('Ctrl Pts',(-1.45284569372596,1.2,2.46800894017942));
#45136=CARTESIAN_POINT('Ctrl Pts',(-1.46404686295214,1.1381078493845,2.47144799369182));
#45137=CARTESIAN_POINT('Ctrl Pts',(-1.48005000616772,1.04094628811002,2.47640896356757));
#45138=CARTESIAN_POINT('Ctrl Pts',(-1.510530945921,0.796143969855592,2.48608811667857));
#45139=CARTESIAN_POINT('Ctrl Pts',(-1.51543685031566,0.741398697530247,
2.48767636587472));
#45140=CARTESIAN_POINT('Ctrl Pts',(-1.52166805320867,0.653834841531101,
2.48968935888044));
#45141=CARTESIAN_POINT('Ctrl Pts',(-1.35239702227521,1.30000000000275,2.54236945495733));
#45142=CARTESIAN_POINT('Ctrl Pts',(-1.35320800708816,1.29919411843786,2.54176576771413));
#45143=CARTESIAN_POINT('Ctrl Pts',(-1.35401460134667,1.29838796377945,2.54116064183015));
#45144=CARTESIAN_POINT('Ctrl Pts',(-1.37051248407318,1.28165666458978,2.52853345157028));
#45145=CARTESIAN_POINT('Ctrl Pts',(-1.38637763270161,1.26578864929006,2.51666625640002));
#45146=CARTESIAN_POINT('Ctrl Pts',(-1.41410479224254,1.23782621524452,2.49576387472157));
#45147=CARTESIAN_POINT('Ctrl Pts',(-1.43176600496645,1.21970424320237,2.48214896452996));
#45148=CARTESIAN_POINT('Ctrl Pts',(-1.45284569372596,1.2,2.46800894017942));
#45149=CARTESIAN_POINT('Ctrl Pts',(-0.96840887762858,-1.3,2.72336636313561));
#45150=CARTESIAN_POINT('Ctrl Pts',(-0.959587680307154,-1.18514270861178,
2.80865755213519));
#45151=CARTESIAN_POINT('Ctrl Pts',(-0.953418388257843,-1.06847604194512,
2.88142219435981));
#45152=CARTESIAN_POINT('Ctrl Pts',(-0.945292521151706,-0.794772684000851,
3.02058424543828));
#45153=CARTESIAN_POINT('Ctrl Pts',(-0.946012577561581,-0.636309800095197,
3.07544248806072));
#45154=CARTESIAN_POINT('Ctrl Pts',(-0.953320013133084,-0.319434907277159,
3.151031219842));
#45155=CARTESIAN_POINT('Ctrl Pts',(-0.961064002623636,-0.158333333333332,
3.17000794893273));
#45156=CARTESIAN_POINT('Ctrl Pts',(-0.98099760953902,0.158333333333334,
3.17479542438189));
#45157=CARTESIAN_POINT('Ctrl Pts',(-0.992074216468526,0.319434907277167,
3.16036137717658));
#45158=CARTESIAN_POINT('Ctrl Pts',(-1.0276372251559,0.636309800095206,3.09502301503918));
#45159=CARTESIAN_POINT('Ctrl Pts',(-1.04845566442809,0.79477268400084,3.04525442796451));
#45160=CARTESIAN_POINT('Ctrl Pts',(-1.10189571121744,1.06847604194511,2.91691192436713));
#45161=CARTESIAN_POINT('Ctrl Pts',(-1.12924033300935,1.18514270861178,2.84921214392929));
#45162=CARTESIAN_POINT('Ctrl Pts',(-1.16079736048698,1.3,2.76936729730244));
#45163=CARTESIAN_POINT('Ctrl Pts',(-0.892825757179276,-1.3,2.70900317484779));
#45164=CARTESIAN_POINT('Ctrl Pts',(-0.885729277039984,-1.18514270861178,
2.79445639963879));
#45165=CARTESIAN_POINT('Ctrl Pts',(-0.880764606872678,-1.06847604194512,
2.86728912331394));
#45166=CARTESIAN_POINT('Ctrl Pts',(-0.874220133109745,-0.794772684000851,
3.00639140283985));
#45167=CARTESIAN_POINT('Ctrl Pts',(-0.874292131581308,-0.636309800095197,
3.06094139417448));
#45168=CARTESIAN_POINT('Ctrl Pts',(-0.881134728284516,-0.319434907277159,
3.13605199626587));
#45169=CARTESIAN_POINT('Ctrl Pts',(-0.88771343062497,-0.158333333333332,
3.15460028905268));
#45170=CARTESIAN_POINT('Ctrl Pts',(-0.907721667816887,0.158333333333334,
3.15903665665579));
#45171=CARTESIAN_POINT('Ctrl Pts',(-0.92003707827324,0.319434907277167,
3.1446851783948));
#45172=CARTESIAN_POINT('Ctrl Pts',(-0.956219211262303,0.636309800095206,
3.07909909005189));
#45173=CARTESIAN_POINT('Ctrl Pts',(-0.97775505801435,0.79477268400084,3.02931249032378));
#45174=CARTESIAN_POINT('Ctrl Pts',(-1.02977474137891,1.06847604194511,2.90027217207626));
#45175=CARTESIAN_POINT('Ctrl Pts',(-1.0559911951017,1.18514270861178,2.83214462327784));
#45176=CARTESIAN_POINT('Ctrl Pts',(-1.08590670913801,1.3,2.75174629803529));
#45177=CARTESIAN_POINT('Ctrl Pts',(-0.817242636729971,-1.3,2.69463998655998));
#45178=CARTESIAN_POINT('Ctrl Pts',(-0.811870873772814,-1.18514270861178,
2.78025524714239));
#45179=CARTESIAN_POINT('Ctrl Pts',(-0.808110825487513,-1.06847604194512,
2.85315605226807));
#45180=CARTESIAN_POINT('Ctrl Pts',(-0.803147745067785,-0.794772684000851,
2.99219856024141));
#45181=CARTESIAN_POINT('Ctrl Pts',(-0.802571685601036,-0.636309800095197,
3.04644030028823));
#45182=CARTESIAN_POINT('Ctrl Pts',(-0.808949443435948,-0.319434907277159,
3.12107277268973));
#45183=CARTESIAN_POINT('Ctrl Pts',(-0.814362858626304,-0.158333333333332,
3.13919262917263));
#45184=CARTESIAN_POINT('Ctrl Pts',(-0.834445726094753,0.158333333333334,
3.14327788892968));
#45185=CARTESIAN_POINT('Ctrl Pts',(-0.847999940077955,0.319434907277167,
3.12900897961301));
#45186=CARTESIAN_POINT('Ctrl Pts',(-0.884801197368704,0.636309800095206,
3.06317516506461));
#45187=CARTESIAN_POINT('Ctrl Pts',(-0.907054451600613,0.79477268400084,
3.01337055268305));
#45188=CARTESIAN_POINT('Ctrl Pts',(-0.957653771540386,1.06847604194511,
2.88363241978539));
#45189=CARTESIAN_POINT('Ctrl Pts',(-0.98274205719405,1.18514270861178,2.81507710262639));
#45190=CARTESIAN_POINT('Ctrl Pts',(-1.01101605778904,1.3,2.73412529876815));
#45191=CARTESIAN_POINT('Ctrl Pts',(-0.741659516280667,-1.3,2.68027679827216));
#45192=CARTESIAN_POINT('Ctrl Pts',(-0.738012470505644,-1.18514270861178,
2.76605409464598));
#45193=CARTESIAN_POINT('Ctrl Pts',(-0.735457044102347,-1.06847604194512,
2.8390229812222));
#45194=CARTESIAN_POINT('Ctrl Pts',(-0.732075357025824,-0.794772684000851,
2.97800571764298));
#45195=CARTESIAN_POINT('Ctrl Pts',(-0.730851239620764,-0.636309800095197,
3.03193920640198));
#45196=CARTESIAN_POINT('Ctrl Pts',(-0.73676415858738,-0.319434907277159,
3.1060935491136));
#45197=CARTESIAN_POINT('Ctrl Pts',(-0.741012286627638,-0.158333333333332,
3.12378496929258));
#45198=CARTESIAN_POINT('Ctrl Pts',(-0.761169784372619,0.158333333333334,
3.12751912120358));
#45199=CARTESIAN_POINT('Ctrl Pts',(-0.775962801882669,0.319434907277167,
3.11333278083123));
#45200=CARTESIAN_POINT('Ctrl Pts',(-0.813383183475105,0.636309800095206,
3.04725124007732));
#45201=CARTESIAN_POINT('Ctrl Pts',(-0.836353845186877,0.79477268400084,
2.99742861504232));
#45202=CARTESIAN_POINT('Ctrl Pts',(-0.885532801701862,1.06847604194511,
2.86699266749452));
#45203=CARTESIAN_POINT('Ctrl Pts',(-0.909492919286398,1.18514270861178,
2.79800958197493));
#45204=CARTESIAN_POINT('Ctrl Pts',(-0.936125406440072,1.3,2.71650429950101));
#45205=CARTESIAN_POINT('Ctrl Pts',(-0.741659516280667,-1.3,2.68027679827216));
#45206=CARTESIAN_POINT('Ctrl Pts',(-0.738012470505644,-1.18514270861178,
2.76605409464599));
#45207=CARTESIAN_POINT('Ctrl Pts',(-0.735457044102347,-1.06847604194512,
2.8390229812222));
#45208=CARTESIAN_POINT('Ctrl Pts',(-0.732075357025824,-0.794772684000851,
2.97800571764298));
#45209=CARTESIAN_POINT('Ctrl Pts',(-0.730851239620763,-0.636309800095197,
3.03193920640198));
#45210=CARTESIAN_POINT('Ctrl Pts',(-0.736764158587379,-0.319434907277159,
3.1060935491136));
#45211=CARTESIAN_POINT('Ctrl Pts',(-0.741012286627637,-0.158333333333332,
3.12378496929258));
#45212=CARTESIAN_POINT('Ctrl Pts',(-0.761169784372619,0.158333333333334,
3.12751912120358));
#45213=CARTESIAN_POINT('Ctrl Pts',(-0.775962801882668,0.319434907277167,
3.11333278083123));
#45214=CARTESIAN_POINT('Ctrl Pts',(-0.813383183475106,0.636309800095206,
3.04725124007732));
#45215=CARTESIAN_POINT('Ctrl Pts',(-0.836353845186877,0.79477268400084,
2.99742861504232));
#45216=CARTESIAN_POINT('Ctrl Pts',(-0.885532801701861,1.06847604194511,
2.86699266749452));
#45217=CARTESIAN_POINT('Ctrl Pts',(-0.909492919286397,1.18514270861178,
2.79800958197494));
#45218=CARTESIAN_POINT('Ctrl Pts',(-0.936125406440072,1.3,2.71650429950101));
#45219=CARTESIAN_POINT('Ctrl Pts',(-0.74165951628067,-1.3000000000001,2.68027679827209));
#45220=CARTESIAN_POINT('Ctrl Pts',(-0.738012470505646,-1.18514270861185,
2.76605409464595));
#45221=CARTESIAN_POINT('Ctrl Pts',(-0.735457044102347,-1.06847604194515,
2.83902298122219));
#45222=CARTESIAN_POINT('Ctrl Pts',(-0.732075357025824,-0.794772684000851,
2.97800571764297));
#45223=CARTESIAN_POINT('Ctrl Pts',(-0.730851239620763,-0.636309800095196,
3.03193920640198));
#45224=CARTESIAN_POINT('Ctrl Pts',(-0.73676415858738,-0.319434907277159,
3.1060935491136));
#45225=CARTESIAN_POINT('Ctrl Pts',(-0.741012286627637,-0.158333333333332,
3.12378496929258));
#45226=CARTESIAN_POINT('Ctrl Pts',(-0.761169784372619,0.158333333333334,
3.12751912120358));
#45227=CARTESIAN_POINT('Ctrl Pts',(-0.775962801882669,0.319434907277167,
3.11333278083123));
#45228=CARTESIAN_POINT('Ctrl Pts',(-0.813383183475106,0.636309800095206,
3.04725124007732));
#45229=CARTESIAN_POINT('Ctrl Pts',(-0.836353845186877,0.79477268400084,
2.99742861504232));
#45230=CARTESIAN_POINT('Ctrl Pts',(-0.885532801702163,1.06847604194679,
2.86699266749372));
#45231=CARTESIAN_POINT('Ctrl Pts',(-0.909492919287077,1.18514270861508,
2.79800958197298));
#45232=CARTESIAN_POINT('Ctrl Pts',(-0.936125406441205,1.30000000000488,
2.71650429949754));
#45233=CARTESIAN_POINT('Ctrl Pts',(-0.73773330559217,-1.3000000000001,2.67245517600946));
#45234=CARTESIAN_POINT('Ctrl Pts',(-0.734729140499245,-1.18514270861185,
2.75847136303451));
#45235=CARTESIAN_POINT('Ctrl Pts',(-0.732217053975366,-1.06847604194515,
2.83164616358891));
#45236=CARTESIAN_POINT('Ctrl Pts',(-0.727550431498492,-0.794772684000851,
2.97102841978056));
#45237=CARTESIAN_POINT('Ctrl Pts',(-0.7226833723533,-0.636309800095196,
3.02517530962454));
#45238=CARTESIAN_POINT('Ctrl Pts',(-0.726824245379794,-0.319434907277159,
3.09946703800493));
#45239=CARTESIAN_POINT('Ctrl Pts',(-0.731604230865546,-0.158333333333332,
3.11703748029681));
#45240=CARTESIAN_POINT('Ctrl Pts',(-0.751993950054195,0.158333333333334,
3.12072515304754));
#45241=CARTESIAN_POINT('Ctrl Pts',(-0.766766141896399,0.319434907277167,
3.10658683795392));
#45242=CARTESIAN_POINT('Ctrl Pts',(-0.805863671213904,0.636309800095206,
3.04032716133598));
#45243=CARTESIAN_POINT('Ctrl Pts',(-0.831394255645057,0.79477268400084,
2.99033173914693));
#45244=CARTESIAN_POINT('Ctrl Pts',(-0.882011643621234,1.06847604194679,
2.85950209302966));
#45245=CARTESIAN_POINT('Ctrl Pts',(-0.906248352874114,1.18514270861508,
2.79031303915094));
#45246=CARTESIAN_POINT('Ctrl Pts',(-0.932811379683886,1.30000000000488,
2.70856623748196));
#45247=CARTESIAN_POINT('Ctrl Pts',(-0.735709753270855,-1.3000000000001,
2.66035632699752));
#45248=CARTESIAN_POINT('Ctrl Pts',(-0.734276224702703,-1.18514270861185,
2.7439279293322));
#45249=CARTESIAN_POINT('Ctrl Pts',(-0.732270057354958,-1.06847604194515,
2.81535450686582));
#45250=CARTESIAN_POINT('Ctrl Pts',(-0.726312499312411,-0.794772684000851,
2.95230675291205));
#45251=CARTESIAN_POINT('Ctrl Pts',(-0.715957485685984,-0.636309800095198,
3.0071883638833));
#45252=CARTESIAN_POINT('Ctrl Pts',(-0.717231377152474,-0.31943490727716,
3.08166701371969));
#45253=CARTESIAN_POINT('Ctrl Pts',(-0.722183463147362,-0.158333333333333,
3.10020625520556));
#45254=CARTESIAN_POINT('Ctrl Pts',(-0.742739360703625,0.158333333333335,
3.10387421830447));
#45255=CARTESIAN_POINT('Ctrl Pts',(-0.757379057429574,0.319434907277169,
3.08867052408036));
#45256=CARTESIAN_POINT('Ctrl Pts',(-0.799939881712645,0.636309800095209,
3.0223403580999));
#45257=CARTESIAN_POINT('Ctrl Pts',(-0.83200195614442,0.794772684000844,
2.97198639479701));
#45258=CARTESIAN_POINT('Ctrl Pts',(-0.883860679443162,1.06847604194679,
2.84356969105433));
#45259=CARTESIAN_POINT('Ctrl Pts',(-0.907297495995768,1.18514270861508,
2.77603315718813));
#45260=CARTESIAN_POINT('Ctrl Pts',(-0.931723409339857,1.30000000000488,
2.69654692219852));
#45261=CARTESIAN_POINT('Ctrl Pts',(-0.732581199673119,-1.3000000000001,
2.64260536769187));
#45262=CARTESIAN_POINT('Ctrl Pts',(-0.731581621758525,-1.18514270861185,
2.72252964260173));
#45263=CARTESIAN_POINT('Ctrl Pts',(-0.729689019270264,-1.06847604194515,
2.79124774140366));
#45264=CARTESIAN_POINT('Ctrl Pts',(-0.723253663494429,-0.794772684000852,
2.92411178804753));
#45265=CARTESIAN_POINT('Ctrl Pts',(-0.711354667280304,-0.636309800095197,
2.9793476780709));
#45266=CARTESIAN_POINT('Ctrl Pts',(-0.711355798935644,-0.319434907277159,
3.05351896672594));
#45267=CARTESIAN_POINT('Ctrl Pts',(-0.715491493976768,-0.158333333333332,
3.07327585441042));
#45268=CARTESIAN_POINT('Ctrl Pts',(-0.736146419548719,0.158333333333335,
3.07697661143391));
#45269=CARTESIAN_POINT('Ctrl Pts',(-0.7513715082161,0.319434907277168,3.06057021824835));
#45270=CARTESIAN_POINT('Ctrl Pts',(-0.79607904654136,0.636309800095207,
2.99465056472962));
#45271=CARTESIAN_POINT('Ctrl Pts',(-0.83154007459095,0.794772684000841,
2.94412507676054));
#45272=CARTESIAN_POINT('Ctrl Pts',(-0.884051830167423,1.06847604194679,
2.81976101536945));
#45273=CARTESIAN_POINT('Ctrl Pts',(-0.907042942513032,1.18514270861508,
2.75486405369761));
#45274=CARTESIAN_POINT('Ctrl Pts',(-0.930294773967327,1.30000000000488,
2.67890272438792));
#45275=CARTESIAN_POINT('Ctrl Pts',(-0.729771743392393,-1.30000000000009,
2.62789816097744));
#45276=CARTESIAN_POINT('Ctrl Pts',(-0.728734320005336,-1.18514270861185,
2.70507151758026));
#45277=CARTESIAN_POINT('Ctrl Pts',(-0.726954114717163,-1.06847604194515,
2.77180122606182));
#45278=CARTESIAN_POINT('Ctrl Pts',(-0.721125509588046,-0.794772684000851,
2.90183328548194));
#45279=CARTESIAN_POINT('Ctrl Pts',(-0.710774425642683,-0.636309800095197,
2.95779964073951));
#45280=CARTESIAN_POINT('Ctrl Pts',(-0.710606698362087,-0.319434907277159,
3.03193990563363));
#45281=CARTESIAN_POINT('Ctrl Pts',(-0.712952299894917,-0.158333333333332,
3.0524727895937));
#45282=CARTESIAN_POINT('Ctrl Pts',(-0.733016707245456,0.158333333333335,
3.05613067980892));
#45283=CARTESIAN_POINT('Ctrl Pts',(-0.748548602363565,0.319434907277168,
3.03882122131528));
#45284=CARTESIAN_POINT('Ctrl Pts',(-0.794040662364233,0.636309800095207,
2.9730167888235));
#45285=CARTESIAN_POINT('Ctrl Pts',(-0.831171375868185,0.794772684000842,
2.92211107346514));
#45286=CARTESIAN_POINT('Ctrl Pts',(-0.88358594787812,1.06847604194679,2.80059150689011));
#45287=CARTESIAN_POINT('Ctrl Pts',(-0.906111819380047,1.18514270861508,
2.73761477251729));
#45288=CARTESIAN_POINT('Ctrl Pts',(-0.928475236311926,1.30000000000488,
2.66426262139868));
#45289=CARTESIAN_POINT('Ctrl Pts',(-0.726505469227192,-1.3000000000001,
2.61305804659452));
#45290=CARTESIAN_POINT('Ctrl Pts',(-0.725318776084473,-1.18514270861185,
2.68722387894012));
#45291=CARTESIAN_POINT('Ctrl Pts',(-0.723622119673275,-1.06847604194515,
2.75176622967882));
#45292=CARTESIAN_POINT('Ctrl Pts',(-0.718524386780468,-0.794772684000852,
2.87863980385541));
#45293=CARTESIAN_POINT('Ctrl Pts',(-0.709931954095278,-0.636309800095197,
2.93527807660178));
#45294=CARTESIAN_POINT('Ctrl Pts',(-0.710293323618512,-0.319434907277159,
3.00935793161261));
#45295=CARTESIAN_POINT('Ctrl Pts',(-0.711181795360178,-0.158333333333332,
3.03075121606602));
#45296=CARTESIAN_POINT('Ctrl Pts',(-0.732159223967551,0.158333333333334,
3.03453740674467));
#45297=CARTESIAN_POINT('Ctrl Pts',(-0.750600978758044,0.319434907277167,
3.01658351261059));
#45298=CARTESIAN_POINT('Ctrl Pts',(-0.796324352907775,0.636309800095206,
2.95092226275884));
#45299=CARTESIAN_POINT('Ctrl Pts',(-0.830988928451572,0.794772684000842,
2.89920826232716));
#45300=CARTESIAN_POINT('Ctrl Pts',(-0.882215538271197,1.06847604194679,
2.78073762285996));
#45301=CARTESIAN_POINT('Ctrl Pts',(-0.904421541101885,1.18514270861508,
2.7198949897962));
#45302=CARTESIAN_POINT('Ctrl Pts',(-0.926659445505138,1.30000000000488,
2.64949127372461));
#45303=CARTESIAN_POINT('Ctrl Pts',(-0.718203659447294,-1.3000000000001,
2.58347432518368));
#45304=CARTESIAN_POINT('Ctrl Pts',(-0.71702626283155,-1.18514270861185,
2.65187970978938));
#45305=CARTESIAN_POINT('Ctrl Pts',(-0.715782659739986,-1.06847604194515,
2.71224520391757));
#45306=CARTESIAN_POINT('Ctrl Pts',(-0.712756737612827,-0.794772684000853,
2.83312781605184));
#45307=CARTESIAN_POINT('Ctrl Pts',(-0.707269685879409,-0.636309800095198,
2.89107118306634));
#45308=CARTESIAN_POINT('Ctrl Pts',(-0.710636393371801,-0.319434907277159,
2.96525869637214));
#45309=CARTESIAN_POINT('Ctrl Pts',(-0.712800720158232,-0.158333333333333,
2.98871655055816));
#45310=CARTESIAN_POINT('Ctrl Pts',(-0.73485780184828,0.158333333333335,
2.992681317029));
#45311=CARTESIAN_POINT('Ctrl Pts',(-0.753453663406939,0.319434907277168,
2.97294683811374));
#45312=CARTESIAN_POINT('Ctrl Pts',(-0.797657321518849,0.636309800095208,
2.90732696513016));
#45313=CARTESIAN_POINT('Ctrl Pts',(-0.829377614451152,0.794772684000843,
2.85419637011498));
#45314=CARTESIAN_POINT('Ctrl Pts',(-0.878922936927556,1.06847604194679,
2.74158131689578));
#45315=CARTESIAN_POINT('Ctrl Pts',(-0.900752807799096,1.18514270861508,
2.6848340433371));
#45316=CARTESIAN_POINT('Ctrl Pts',(-0.922966215277102,1.30000000000488,
2.62008637995976));
#45317=CARTESIAN_POINT('Ctrl Pts',(-0.711759248151161,-1.3000000000001,
2.55392799989938));
#45318=CARTESIAN_POINT('Ctrl Pts',(-0.709659453060768,-1.18514270861185,
2.61648977582277));
#45319=CARTESIAN_POINT('Ctrl Pts',(-0.708079464161582,-1.06847604194515,
2.67259991171752));
#45320=CARTESIAN_POINT('Ctrl Pts',(-0.705630230017321,-0.794772684000854,
2.78732097131632));
#45321=CARTESIAN_POINT('Ctrl Pts',(-0.702745937711363,-0.636309800095198,
2.84646488276085));
#45322=CARTESIAN_POINT('Ctrl Pts',(-0.708213072692534,-0.319434907277159,
2.92063246419698));
#45323=CARTESIAN_POINT('Ctrl Pts',(-0.711339447678475,-0.158333333333332,
2.94613913648399));
#45324=CARTESIAN_POINT('Ctrl Pts',(-0.734125218490468,0.158333333333334,
2.95019622821214));
#45325=CARTESIAN_POINT('Ctrl Pts',(-0.752687649534627,0.319434907277165,
2.92855294595052));
#45326=CARTESIAN_POINT('Ctrl Pts',(-0.795867927344174,0.636309800095205,
2.86304392466589));
#45327=CARTESIAN_POINT('Ctrl Pts',(-0.825869341580405,0.794772684000843,
2.80872865049762));
#45328=CARTESIAN_POINT('Ctrl Pts',(-0.874075887182553,1.06847604194679,
2.70213915588633));
#45329=CARTESIAN_POINT('Ctrl Pts',(-0.895466313933186,1.18514270861508,
2.64954635264564));
#45330=CARTESIAN_POINT('Ctrl Pts',(-0.917380340071678,1.30000000000488,
2.5904993888518));
#45331=CARTESIAN_POINT('Ctrl Pts',(-0.701409308678934,-1.3000000000001,
2.52143083639184));
#45332=CARTESIAN_POINT('Ctrl Pts',(-0.698426146535951,-1.18514270861184,
2.5776296854358));
#45333=CARTESIAN_POINT('Ctrl Pts',(-0.696567911764466,-1.06847604194514,
2.62909904971683));
#45334=CARTESIAN_POINT('Ctrl Pts',(-0.694873824972859,-0.794772684000843,
2.73707752168452));
#45335=CARTESIAN_POINT('Ctrl Pts',(-0.694381863306111,-0.636309800095195,
2.7974518787628));
#45336=CARTESIAN_POINT('Ctrl Pts',(-0.702953732513364,-0.319434907277159,
2.87160078252508));
#45337=CARTESIAN_POINT('Ctrl Pts',(-0.708896545536722,-0.158333333333332,
2.89942566072425));
#45338=CARTESIAN_POINT('Ctrl Pts',(-0.732779542220326,0.158333333333334,
2.90359846879207));
#45339=CARTESIAN_POINT('Ctrl Pts',(-0.749996430543724,0.319434907277167,
2.87983083089195));
#45340=CARTESIAN_POINT('Ctrl Pts',(-0.791545806470309,0.636309800095206,
2.81441703993551));
#45341=CARTESIAN_POINT('Ctrl Pts',(-0.819313612205697,0.794772684000841,
2.75876072363453));
#45342=CARTESIAN_POINT('Ctrl Pts',(-0.867005692102054,1.06847604194679,
2.65880185706368));
#45343=CARTESIAN_POINT('Ctrl Pts',(-0.888655048864636,1.18514270861508,
2.6107906112134));
#45344=CARTESIAN_POINT('Ctrl Pts',(-0.911309628168231,1.30000000000488,
2.55803660901066));
#45345=CARTESIAN_POINT('Ctrl Pts',(-0.695015042608171,-1.3000000000001,
2.49781259678561));
#45346=CARTESIAN_POINT('Ctrl Pts',(-0.691330264994516,-1.18514270861185,
2.54936798035452));
#45347=CARTESIAN_POINT('Ctrl Pts',(-0.689101790206814,-1.06847604194514,
2.59744566475941));
#45348=CARTESIAN_POINT('Ctrl Pts',(-0.687317918502706,-0.794772684000844,
2.7004805528623));
#45349=CARTESIAN_POINT('Ctrl Pts',(-0.687738816379448,-0.636309800095195,
2.76173681889702));
#45350=CARTESIAN_POINT('Ctrl Pts',(-0.697669729324493,-0.319434907277159,
2.83580174139693));
#45351=CARTESIAN_POINT('Ctrl Pts',(-0.705033470020429,-0.158333333333332,
2.86522201718424));
#45352=CARTESIAN_POINT('Ctrl Pts',(-0.729713908260099,0.158333333333334,
2.86945474364033));
#45353=CARTESIAN_POINT('Ctrl Pts',(-0.746638691550855,0.319434907277167,
2.84418733046913));
#45354=CARTESIAN_POINT('Ctrl Pts',(-0.787778355364049,0.636309800095205,
2.77890684388552));
#45355=CARTESIAN_POINT('Ctrl Pts',(-0.814620216025745,0.794772684000838,
2.72234169851759));
#45356=CARTESIAN_POINT('Ctrl Pts',(-0.862244632919749,1.06847604194679,
2.62725935743987));
#45357=CARTESIAN_POINT('Ctrl Pts',(-0.884070097538701,1.18514270861508,
2.58259634633224));
#45358=CARTESIAN_POINT('Ctrl Pts',(-0.907106181361594,1.30000000000488,
2.53442794642189));
#45359=CARTESIAN_POINT('Ctrl Pts',(-0.684471546903474,-1.3000000000001,
2.46831190594925));
#45360=CARTESIAN_POINT('Ctrl Pts',(-0.679292846719528,-1.18514270861185,
2.51407523067114));
#45361=CARTESIAN_POINT('Ctrl Pts',(-0.67636879885502,-1.06847604194515,
2.55792096534174));
#45362=CARTESIAN_POINT('Ctrl Pts',(-0.674822361233792,-0.794772684000854,
2.65478336710894));
#45363=CARTESIAN_POINT('Ctrl Pts',(-0.678478767580897,-0.636309800095198,
2.71713334559981));
#45364=CARTESIAN_POINT('Ctrl Pts',(-0.690659306413056,-0.319434907277159,
2.79107914598393));
#45365=CARTESIAN_POINT('Ctrl Pts',(-0.698803958562443,-0.158333333333332,
2.82247483191899));
#45366=CARTESIAN_POINT('Ctrl Pts',(-0.724331819242718,0.158333333333335,
2.82677431923026));
#45367=CARTESIAN_POINT('Ctrl Pts',(-0.741369687464005,0.319434907277167,
2.79964707518251));
#45368=CARTESIAN_POINT('Ctrl Pts',(-0.781890996115929,0.636309800095207,
2.73452225817136));
#45369=CARTESIAN_POINT('Ctrl Pts',(-0.807011700062937,0.794772684000841,
2.67680326982785));
#45370=CARTESIAN_POINT('Ctrl Pts',(-0.85439209018396,1.06847604194679,2.58778738955115));
#45371=CARTESIAN_POINT('Ctrl Pts',(-0.876453514898898,1.18514270861508,
2.54729514463003));
#45372=CARTESIAN_POINT('Ctrl Pts',(-0.900067149061703,1.30000000000489,
2.50484233099641));
#45373=CARTESIAN_POINT('Ctrl Pts',(-0.674261209315636,-1.3000000000001,
2.43590191982576));
#45374=CARTESIAN_POINT('Ctrl Pts',(-0.667529038149191,-1.18514270861185,
2.47530503846599));
#45375=CARTESIAN_POINT('Ctrl Pts',(-0.663661339171831,-1.06847604194515,
2.51449844127821));
#45376=CARTESIAN_POINT('Ctrl Pts',(-0.661343684596083,-0.794772684000854,
2.60455855687163));
#45377=CARTESIAN_POINT('Ctrl Pts',(-0.666221899005568,-0.636309800095196,
2.66807322957033));
#45378=CARTESIAN_POINT('Ctrl Pts',(-0.680453091202015,-0.319434907277157,
2.74185202409489));
#45379=CARTESIAN_POINT('Ctrl Pts',(-0.691402120595438,-0.158333333333332,
2.77541503050119));
#45380=CARTESIAN_POINT('Ctrl Pts',(-0.717772629253875,0.158333333333334,
2.77974510248551));
#45381=CARTESIAN_POINT('Ctrl Pts',(-0.733025999216182,0.319434907277166,
2.75050343715987));
#45382=CARTESIAN_POINT('Ctrl Pts',(-0.772852060962675,0.636309800095205,
2.68556247171395));
#45383=CARTESIAN_POINT('Ctrl Pts',(-0.797551059226474,0.794772684000838,
2.62665941880218));
#45384=CARTESIAN_POINT('Ctrl Pts',(-0.845717106904218,1.06847604194679,
2.54438330441938));
#45385=CARTESIAN_POINT('Ctrl Pts',(-0.868442268727925,1.18514270861508,
2.50850465450521));
#45386=CARTESIAN_POINT('Ctrl Pts',(-0.893043295063443,1.30000000000488,
2.47236163596295));
#45387=CARTESIAN_POINT('Ctrl Pts',(-0.665650684226199,-1.3000000000001,
2.41236448965116));
#45388=CARTESIAN_POINT('Ctrl Pts',(-0.657463728678987,-1.18514270861185,
2.4471572740478));
#45389=CARTESIAN_POINT('Ctrl Pts',(-0.652811062767846,-1.06847604194515,
2.48297516049676));
#45390=CARTESIAN_POINT('Ctrl Pts',(-0.65022738984203,-0.794772684000853,
2.56808983434933));
#45391=CARTESIAN_POINT('Ctrl Pts',(-0.657616410684264,-0.636309800095197,
2.63243055732278));
#45392=CARTESIAN_POINT('Ctrl Pts',(-0.673098780547473,-0.319434907277159,
2.70605930776217));
#45393=CARTESIAN_POINT('Ctrl Pts',(-0.684135212950933,-0.158333333333332,
2.74116263102348));
#45394=CARTESIAN_POINT('Ctrl Pts',(-0.710767709561529,0.158333333333335,
2.7455138041351));
#45395=CARTESIAN_POINT('Ctrl Pts',(-0.725987843158548,0.319434907277167,
2.71477983403209));
#45396=CARTESIAN_POINT('Ctrl Pts',(-0.765519694872641,0.636309800095206,
2.64997707848015));
#45397=CARTESIAN_POINT('Ctrl Pts',(-0.789120836171394,0.794772684000841,
2.59018019489115));
#45398=CARTESIAN_POINT('Ctrl Pts',(-0.837961494715776,1.06847604194679,
2.51279473146583));
#45399=CARTESIAN_POINT('Ctrl Pts',(-0.861369519587865,1.18514270861508,
2.48027014456695));
#45400=CARTESIAN_POINT('Ctrl Pts',(-0.887044257972772,1.30000000000488,
2.44871827047225));
#45401=CARTESIAN_POINT('Ctrl Pts',(-0.656870619801096,-1.3000000000001,
2.38886109932766));
#45402=CARTESIAN_POINT('Ctrl Pts',(-0.646955507175138,-1.18514270861185,
2.41906094384512));
#45403=CARTESIAN_POINT('Ctrl Pts',(-0.641172110179515,-1.06847604194515,
2.4515133873216));
#45404=CARTESIAN_POINT('Ctrl Pts',(-0.637356395807979,-0.794772684000853,
2.53168897806758));
#45405=CARTESIAN_POINT('Ctrl Pts',(-0.645440186674182,-0.636309800095197,
2.59683243151389));
#45406=CARTESIAN_POINT('Ctrl Pts',(-0.662856348260645,-0.319434907277158,
2.67029705351756));
#45407=CARTESIAN_POINT('Ctrl Pts',(-0.676859985583006,-0.158333333333332,
2.70693559241231));
#45408=CARTESIAN_POINT('Ctrl Pts',(-0.705025145353065,0.158333333333334,
2.71130040697335));
#45409=CARTESIAN_POINT('Ctrl Pts',(-0.719631034374305,0.319434907277168,
2.67907185952832));
#45410=CARTESIAN_POINT('Ctrl Pts',(-0.758680132565803,0.636309800095207,
2.614406028439));
#45411=CARTESIAN_POINT('Ctrl Pts',(-0.78073808948678,0.79477268400084,2.55371501141879));
#45412=CARTESIAN_POINT('Ctrl Pts',(-0.830246128428462,1.06847604194679,
2.48122741212257));
#45413=CARTESIAN_POINT('Ctrl Pts',(-0.854437405012396,1.18514270861508,
2.45206178512877));
#45414=CARTESIAN_POINT('Ctrl Pts',(-0.881389762575884,1.30000000000488,
2.42510772694649));
#45415=CARTESIAN_POINT('Ctrl Pts',(-0.649882878774368,-1.3000000000001,
2.36830415817458));
#45416=CARTESIAN_POINT('Ctrl Pts',(-0.638160393524729,-1.18514270861185,
2.39450573828197));
#45417=CARTESIAN_POINT('Ctrl Pts',(-0.631282124890061,-1.06847604194515,
2.42402609610759));
#45418=CARTESIAN_POINT('Ctrl Pts',(-0.626583057813851,-0.794772684000853,
2.49989106866049));
#45419=CARTESIAN_POINT('Ctrl Pts',(-0.636782937033632,-0.636309800095198,
2.56571734829579));
#45420=CARTESIAN_POINT('Ctrl Pts',(-0.655281941044772,-0.31943490727716,
2.63902174680975));
#45421=CARTESIAN_POINT('Ctrl Pts',(-0.669906857441273,-0.158333333333332,
2.67698930985721));
#45422=CARTESIAN_POINT('Ctrl Pts',(-0.698002341158252,0.158333333333335,
2.68135526233245));
#45423=CARTESIAN_POINT('Ctrl Pts',(-0.711418408796788,0.319434907277166,
2.64781596256982));
#45424=CARTESIAN_POINT('Ctrl Pts',(-0.750258894103182,0.636309800095206,
2.58327777225634));
#45425=CARTESIAN_POINT('Ctrl Pts',(-0.772698526102032,0.794772684000843,
2.52184053753016));
#45426=CARTESIAN_POINT('Ctrl Pts',(-0.823092540885076,1.06847604194679,
2.4536193870615));
#45427=CARTESIAN_POINT('Ctrl Pts',(-0.847808970160495,1.18514270861508,
2.4273725281449));
#45428=CARTESIAN_POINT('Ctrl Pts',(-0.875428126993862,1.30000000000488,
2.40440921850705));
#45429=CARTESIAN_POINT('Ctrl Pts',(-0.639601120729089,-1.3000000000001,
2.34486673133637));
#45430=CARTESIAN_POINT('Ctrl Pts',(-0.626738549432459,-1.18514270861185,
2.36648103949476));
#45431=CARTESIAN_POINT('Ctrl Pts',(-0.61911233014439,-1.06847604194515,
2.39264026996296));
#45432=CARTESIAN_POINT('Ctrl Pts',(-0.613591258637418,-0.794772684000853,
2.46357300522486));
#45433=CARTESIAN_POINT('Ctrl Pts',(-0.624299890124151,-0.636309800095198,
2.53021390656471));
#45434=CARTESIAN_POINT('Ctrl Pts',(-0.643934931957813,-0.319434907277159,
2.60333239070418));
#45435=CARTESIAN_POINT('Ctrl Pts',(-0.660036159520178,-0.158333333333332,
2.6427910421422));
#45436=CARTESIAN_POINT('Ctrl Pts',(-0.6894821708808,0.158333333333334,2.64714550972695));
#45437=CARTESIAN_POINT('Ctrl Pts',(-0.703672527292407,0.319434907277166,
2.61211559607771));
#45438=CARTESIAN_POINT('Ctrl Pts',(-0.742294519887011,0.636309800095206,
2.54771556581829));
#45439=CARTESIAN_POINT('Ctrl Pts',(-0.762328448713979,0.794772684000843,
2.48540404651612));
#45440=CARTESIAN_POINT('Ctrl Pts',(-0.813417169094425,1.06847604194679,
2.42206658400128));
#45441=CARTESIAN_POINT('Ctrl Pts',(-0.839076057957825,1.18514270861508,
2.39916544992552));
#45442=CARTESIAN_POINT('Ctrl Pts',(-0.868279421655417,1.30000000000488,
2.38077962241262));
#45443=CARTESIAN_POINT('Ctrl Pts',(-0.633197595098763,-1.3000000000001,
2.32729565509898));
#45444=CARTESIAN_POINT('Ctrl Pts',(-0.618269500330944,-1.18514270861185,
2.34551265657001));
#45445=CARTESIAN_POINT('Ctrl Pts',(-0.609375408590763,-1.06847604194515,
2.36917541648807));
#45446=CARTESIAN_POINT('Ctrl Pts',(-0.602768031506001,-0.794772684000852,
2.43642191705059));
#45447=CARTESIAN_POINT('Ctrl Pts',(-0.615898378255201,-0.636309800095197,
2.5036017450308));
#45448=CARTESIAN_POINT('Ctrl Pts',(-0.636425089780797,-0.319434907277159,
2.57656123962056));
#45449=CARTESIAN_POINT('Ctrl Pts',(-0.652741211014589,-0.158333333333332,
2.61715813013545));
#45450=CARTESIAN_POINT('Ctrl Pts',(-0.681838466694604,0.158333333333334,
2.62150905457092));
#45451=CARTESIAN_POINT('Ctrl Pts',(-0.694678941004356,0.319434907277166,
2.58535909389188));
#45452=CARTESIAN_POINT('Ctrl Pts',(-0.733300373197626,0.636309800095205,
2.52106656301223));
#45453=CARTESIAN_POINT('Ctrl Pts',(-0.754186571802129,0.794772684000841,
2.45811045351102));
#45454=CARTESIAN_POINT('Ctrl Pts',(-0.806660287751361,1.06847604194679,
2.39842947905507));
#45455=CARTESIAN_POINT('Ctrl Pts',(-0.833058301122932,1.18514270861508,
2.37803099503305));
#45456=CARTESIAN_POINT('Ctrl Pts',(-0.863140400574275,1.30000000000488,
2.36306770943312));
#45457=CARTESIAN_POINT('Ctrl Pts',(-0.626079773935383,-1.3000000000001,
2.30973009617971));
#45458=CARTESIAN_POINT('Ctrl Pts',(-0.610331537002746,-1.18514270861185,
2.32451224692394));
#45459=CARTESIAN_POINT('Ctrl Pts',(-0.600796482538009,-1.06847604194515,
2.34566182435764));
#45460=CARTESIAN_POINT('Ctrl Pts',(-0.593122293687099,-0.794772684000854,
2.40923160863995));
#45461=CARTESIAN_POINT('Ctrl Pts',(-0.605662884950393,-0.636309800095198,
2.47705840291504));
#45462=CARTESIAN_POINT('Ctrl Pts',(-0.626783724957263,-0.31943490727716,
2.54987862947416));
#45463=CARTESIAN_POINT('Ctrl Pts',(-0.64475703726334,-0.158333333333332,
2.5915580150273));
#45464=CARTESIAN_POINT('Ctrl Pts',(-0.675054189961014,0.158333333333335,
2.59588195696333));
#45465=CARTESIAN_POINT('Ctrl Pts',(-0.68829025443637,0.319434907277166,
2.55861394244903));
#45466=CARTESIAN_POINT('Ctrl Pts',(-0.727024398230972,0.636309800095206,
2.49442318749211));
#45467=CARTESIAN_POINT('Ctrl Pts',(-0.746734440543491,0.794772684000843,
2.43082141158967));
#45468=CARTESIAN_POINT('Ctrl Pts',(-0.799806743999464,1.06847604194679,
2.37479633394177));
#45469=CARTESIAN_POINT('Ctrl Pts',(-0.826812948308842,1.18514270861509,
2.3569008885581));
#45470=CARTESIAN_POINT('Ctrl Pts',(-0.857852323283982,1.30000000000489,
2.34536117797102));
#45471=CARTESIAN_POINT('Ctrl Pts',(-0.618516064350732,-1.3000000000001,
2.29220914266115));
#45472=CARTESIAN_POINT('Ctrl Pts',(-0.601165595952986,-1.18514270861185,
2.30359702422762));
#45473=CARTESIAN_POINT('Ctrl Pts',(-0.590600175185821,-1.06847604194515,
2.32225479356599));
#45474=CARTESIAN_POINT('Ctrl Pts',(-0.581866756979261,-0.794772684000851,
2.38215286830075));
#45475=CARTESIAN_POINT('Ctrl Pts',(-0.595610486910496,-0.636309800095198,
2.45054905609851));
#45476=CARTESIAN_POINT('Ctrl Pts',(-0.617792955535238,-0.31943490727716,
2.52319924712737));
#45477=CARTESIAN_POINT('Ctrl Pts',(-0.637167225744727,-0.158333333333332,
2.56596826351255));
#45478=CARTESIAN_POINT('Ctrl Pts',(-0.667637211820594,0.158333333333335,
2.57027127447384));
#45479=CARTESIAN_POINT('Ctrl Pts',(-0.679575339066228,0.319434907277167,
2.53190020337716));
#45480=CARTESIAN_POINT('Ctrl Pts',(-0.717742106842312,0.636309800095206,
2.46782156146033));
#45481=CARTESIAN_POINT('Ctrl Pts',(-0.736793863492731,0.794772684000843,
2.40358152724018));
#45482=CARTESIAN_POINT('Ctrl Pts',(-0.791249042953884,1.06847604194679,
2.35120291465679));
#45483=CARTESIAN_POINT('Ctrl Pts',(-0.819342336142497,1.18514270861508,
2.33580188756883));
#45484=CARTESIAN_POINT('Ctrl Pts',(-0.851957293094066,1.30000000000488,
2.32767259396157));
#45485=CARTESIAN_POINT('Ctrl Pts',(-0.612246541381865,-1.3000000000001,
2.27761837040574));
#45486=CARTESIAN_POINT('Ctrl Pts',(-0.593692384082968,-1.18514270861185,
2.28617858275121));
#45487=CARTESIAN_POINT('Ctrl Pts',(-0.582327596914736,-1.06847604194515,
2.30276101850632));
#45488=CARTESIAN_POINT('Ctrl Pts',(-0.572681548268638,-0.794772684000852,
2.3596027033221));
#45489=CARTESIAN_POINT('Ctrl Pts',(-0.587073082306584,-0.636309800095197,
2.42847805994353));
#45490=CARTESIAN_POINT('Ctrl Pts',(-0.610039797410067,-0.319434907277159,
2.50098775770488));
#45491=CARTESIAN_POINT('Ctrl Pts',(-0.630550292877451,-0.158333333333332,
2.54466283821605));
#45492=CARTESIAN_POINT('Ctrl Pts',(-0.661530881486414,0.158333333333334,
2.54894472302388));
#45493=CARTESIAN_POINT('Ctrl Pts',(-0.673037100073311,0.319434907277167,
2.50965063494088));
#45494=CARTESIAN_POINT('Ctrl Pts',(-0.711065100361274,0.636309800095206,
2.44566095314052));
#45495=CARTESIAN_POINT('Ctrl Pts',(-0.729521903519784,0.794772684000841,
2.38088662487286));
#45496=CARTESIAN_POINT('Ctrl Pts',(-0.78485352271252,1.06847604194679,2.33154535248203));
#45497=CARTESIAN_POINT('Ctrl Pts',(-0.813648477505016,1.18514270861508,
2.31822301554134));
#45498=CARTESIAN_POINT('Ctrl Pts',(-0.847287379379839,1.30000000000488,
2.31293635020378));
#45499=CARTESIAN_POINT('Ctrl Pts',(-0.607479816432377,-1.3000000000001,
2.26743691577883));
#45500=CARTESIAN_POINT('Ctrl Pts',(-0.587695759547648,-1.18514270861185,
2.27404585769401));
#45501=CARTESIAN_POINT('Ctrl Pts',(-0.575576671451465,-1.06847604194515,
2.28919013743464));
#45502=CARTESIAN_POINT('Ctrl Pts',(-0.565286764807315,-0.794772684000852,
2.34389479110354));
#45503=CARTESIAN_POINT('Ctrl Pts',(-0.581103229889194,-0.636309800095198,
2.41304642683953));
#45504=CARTESIAN_POINT('Ctrl Pts',(-0.604647533643777,-0.31943490727716,
2.48544261369419));
#45505=CARTESIAN_POINT('Ctrl Pts',(-0.625160380145147,-0.158333333333333,
2.52977641297451));
#45506=CARTESIAN_POINT('Ctrl Pts',(-0.656393070713214,0.158333333333335,
2.53404348737667));
#45507=CARTESIAN_POINT('Ctrl Pts',(-0.667950777501656,0.319434907277167,
2.49409069825917));
#45508=CARTESIAN_POINT('Ctrl Pts',(-0.706318549569805,0.636309800095207,
2.43015415578138));
#45509=CARTESIAN_POINT('Ctrl Pts',(-0.724906926658951,0.794772684000843,
2.36500191170995));
#45510=CARTESIAN_POINT('Ctrl Pts',(-0.780912404472189,1.06847604194679,
2.3177841641865));
#45511=CARTESIAN_POINT('Ctrl Pts',(-0.810088331584231,1.18514270861508,
2.30591686559178));
#45512=CARTESIAN_POINT('Ctrl Pts',(-0.844197489670253,1.30000000000488,
2.30262108171541));
#45513=CARTESIAN_POINT('Ctrl Pts',(-0.604931245382851,-1.3000000000001,
2.26160847477855));
#45514=CARTESIAN_POINT('Ctrl Pts',(-0.584616688670195,-1.18514270861185,
2.26709078669192));
#45515=CARTESIAN_POINT('Ctrl Pts',(-0.572137619939733,-1.06847604194515,
2.28140838306454));
#45516=CARTESIAN_POINT('Ctrl Pts',(-0.561410019466087,-0.794772684000852,
2.33489616950412));
#45517=CARTESIAN_POINT('Ctrl Pts',(-0.577462100406279,-0.636309800095198,
2.40424226993325));
#45518=CARTESIAN_POINT('Ctrl Pts',(-0.601293345077049,-0.31943490727716,
2.47657944903449));
#45519=CARTESIAN_POINT('Ctrl Pts',(-0.622290560639905,-0.158333333333332,
2.52126599426556));
#45520=CARTESIAN_POINT('Ctrl Pts',(-0.653684869393672,0.158333333333335,
2.52552193202855));
#45521=CARTESIAN_POINT('Ctrl Pts',(-0.664974269052977,0.319434907277167,
2.48520499120061));
#45522=CARTESIAN_POINT('Ctrl Pts',(-0.703273406820467,0.636309800095207,
2.42130532012318));
#45523=CARTESIAN_POINT('Ctrl Pts',(-0.721648145326729,0.794772684000843,
2.35593985539621));
#45524=CARTESIAN_POINT('Ctrl Pts',(-0.778134816358336,1.06847604194679,
2.30993383769245));
#45525=CARTESIAN_POINT('Ctrl Pts',(-0.807673287107374,1.18514270861508,
2.29889569734431));
#45526=CARTESIAN_POINT('Ctrl Pts',(-0.84229924175312,1.30000000000488,2.29673371702119));
#45527=CARTESIAN_POINT('Ctrl Pts',(-0.598705350401753,-1.3000000000001,
2.24702934100177));
#45528=CARTESIAN_POINT('Ctrl Pts',(-0.577243519645577,-1.18514270861185,
2.24968477596089));
#45529=CARTESIAN_POINT('Ctrl Pts',(-0.563936836727194,-1.06847604194515,
2.26193184984053));
#45530=CARTESIAN_POINT('Ctrl Pts',(-0.552035760129972,-0.794772684000849,
2.31238364522845));
#45531=CARTESIAN_POINT('Ctrl Pts',(-0.568119224396592,-0.636309800095196,
2.38225132653745));
#45532=CARTESIAN_POINT('Ctrl Pts',(-0.592507924008144,-0.319434907277159,
2.45445080627896));
#45533=CARTESIAN_POINT('Ctrl Pts',(-0.61496683549521,-0.158333333333332,
2.50000379678372));
#45534=CARTESIAN_POINT('Ctrl Pts',(-0.646767713304497,0.158333333333334,
2.50422821446524));
#45535=CARTESIAN_POINT('Ctrl Pts',(-0.657324107698235,0.319434907277167,
2.46300235975121));
#45536=CARTESIAN_POINT('Ctrl Pts',(-0.69523780390506,0.636309800095206,
2.3991984852663));
#45537=CARTESIAN_POINT('Ctrl Pts',(-0.712645846447726,0.794772684000841,
2.33331004648075));
#45538=CARTESIAN_POINT('Ctrl Pts',(-0.770431871534126,1.06847604194679,
2.29032952319989));
#45539=CARTESIAN_POINT('Ctrl Pts',(-0.801044784423362,1.18514270861508,
2.28135946244387));
#45540=CARTESIAN_POINT('Ctrl Pts',(-0.837257181124994,1.30000000000488,
2.28202401687493));
#45541=CARTESIAN_POINT('Ctrl Pts',(-0.587042649530746,-1.30000000000009,
2.22234384363184));
#45542=CARTESIAN_POINT('Ctrl Pts',(-0.562820500195641,-1.18514270861185,
2.22026829704167));
#45543=CARTESIAN_POINT('Ctrl Pts',(-0.547696655758405,-1.06847604194515,
2.2290358717163));
#45544=CARTESIAN_POINT('Ctrl Pts',(-0.533776454017415,-0.794772684000855,
2.27434050244266));
#45545=CARTESIAN_POINT('Ctrl Pts',(-0.551744662673875,-0.636309800095196,
2.34495835777017));
#45546=CARTESIAN_POINT('Ctrl Pts',(-0.57747337456279,-0.319434907277158,
2.41687595758322));
#45547=CARTESIAN_POINT('Ctrl Pts',(-0.601466469856508,-0.158333333333333,
2.46393265375855));
#45548=CARTESIAN_POINT('Ctrl Pts',(-0.633992379378982,0.158333333333335,
2.46809677024522));
#45549=CARTESIAN_POINT('Ctrl Pts',(-0.643460099385473,0.31943490727717,
2.42532591810735));
#45550=CARTESIAN_POINT('Ctrl Pts',(-0.682079987496844,0.636309800095208,
2.36164237349499));
#45551=CARTESIAN_POINT('Ctrl Pts',(-0.700867297629238,0.79477268400084,
2.29479462409256));
#45552=CARTESIAN_POINT('Ctrl Pts',(-0.760180383338873,1.06847604194679,
2.25693188947481));
#45553=CARTESIAN_POINT('Ctrl Pts',(-0.791453011033393,1.18514270861508,
2.25147872126339));
#45554=CARTESIAN_POINT('Ctrl Pts',(-0.828323829384959,1.30000000000488,
2.25696175970412));
#45555=CARTESIAN_POINT('Ctrl Pts',(-0.576486148454196,-1.3000000000001,
2.19912562163394));
#45556=CARTESIAN_POINT('Ctrl Pts',(-0.549805595338174,-1.18514270861185,
2.19260415017178));
#45557=CARTESIAN_POINT('Ctrl Pts',(-0.5330126429192,-1.06847604194515,2.19810476899683));
#45558=CARTESIAN_POINT('Ctrl Pts',(-0.517059899030671,-0.794772684000851,
2.23858573245206));
#45559=CARTESIAN_POINT('Ctrl Pts',(-0.536361982215063,-0.636309800095196,
2.30992895987017));
#45560=CARTESIAN_POINT('Ctrl Pts',(-0.562926419576893,-0.319434907277159,
2.38160063251548));
#45561=CARTESIAN_POINT('Ctrl Pts',(-0.588041432013228,-0.158333333333332,
2.43008246775003));
#45562=CARTESIAN_POINT('Ctrl Pts',(-0.621210414474164,0.158333333333334,
2.43418697459444));
#45563=CARTESIAN_POINT('Ctrl Pts',(-0.630650969299707,0.319434907277167,
2.38992172995728));
#45564=CARTESIAN_POINT('Ctrl Pts',(-0.668824987562712,0.636309800095206,
2.32638233568519));
#45565=CARTESIAN_POINT('Ctrl Pts',(-0.685020236270646,0.79477268400084,
2.25874033545448));
#45566=CARTESIAN_POINT('Ctrl Pts',(-0.746715246697685,1.06847604194679,
2.22569485762038));
#45567=CARTESIAN_POINT('Ctrl Pts',(-0.780090946625215,1.18514270861508,
2.22352789394532));
#45568=CARTESIAN_POINT('Ctrl Pts',(-0.820136862491639,1.30000000000488,
2.23349812949406));
#45569=CARTESIAN_POINT('Ctrl Pts',(-0.570670255377225,-1.3000000000001,
2.18755391703729));
#45570=CARTESIAN_POINT('Ctrl Pts',(-0.542940786613338,-1.18514270861185,
2.17880571545946));
#45571=CARTESIAN_POINT('Ctrl Pts',(-0.52540477270343,-1.06847604194515,
2.18267301919227));
#45572=CARTESIAN_POINT('Ctrl Pts',(-0.508441992410327,-0.794772684000851,
2.22075160545733));
#45573=CARTESIAN_POINT('Ctrl Pts',(-0.527915117224749,-0.636309800095196,
2.29249271205802));
#45574=CARTESIAN_POINT('Ctrl Pts',(-0.554987172141783,-0.319434907277159,
2.36403312099634));
#45575=CARTESIAN_POINT('Ctrl Pts',(-0.581221077759064,-0.158333333333332,
2.41318126918772));
#45576=CARTESIAN_POINT('Ctrl Pts',(-0.614857791973616,0.158333333333334,
2.41724102817915));
#45577=CARTESIAN_POINT('Ctrl Pts',(-0.623796233999666,0.319434907277167,
2.37225523561236));
#45578=CARTESIAN_POINT('Ctrl Pts',(-0.662111769288737,0.636309800095206,
2.30877528147271));
#45579=CARTESIAN_POINT('Ctrl Pts',(-0.678359592024735,0.79477268400084,
2.24069668195692));
#45580=CARTESIAN_POINT('Ctrl Pts',(-0.740987950519493,1.06847604194679,
2.21004687505626));
#45581=CARTESIAN_POINT('Ctrl Pts',(-0.774949037062878,1.18514270861508,
2.20952346492048));
#45582=CARTESIAN_POINT('Ctrl Pts',(-0.815761714366448,1.30000000000488,
2.22174381036905));
#45583=CARTESIAN_POINT('',(-0.819024792214424,1.2,2.31822794574162));
#45584=CARTESIAN_POINT('Ctrl Pts',(-0.819024792214424,1.2,2.31822794574162));
#45585=CARTESIAN_POINT('Ctrl Pts',(-0.82521597710165,1.20975290671087,2.32915586731225));
#45586=CARTESIAN_POINT('Ctrl Pts',(-0.831493530093656,1.21883993984152,
2.3394451037281));
#45587=CARTESIAN_POINT('Ctrl Pts',(-0.842725049707713,1.23553583411338,
2.35832248138883));
#45588=CARTESIAN_POINT('Ctrl Pts',(-0.843308014052171,1.23658026496901,
2.35947858996007));
#45589=CARTESIAN_POINT('Ctrl Pts',(-0.875337102299465,1.28817247228299,
2.41752300234903));
#45590=CARTESIAN_POINT('Ctrl Pts',(-0.877248816045502,1.29056256453409,
2.4203953723537));
#45591=CARTESIAN_POINT('Ctrl Pts',(-0.882736269392908,1.3,2.43100884057243));
#45592=CARTESIAN_POINT('',(-0.66423798661977,0.653834841417894,2.2947693329594));
#45593=CARTESIAN_POINT('Ctrl Pts',(-0.664237986625888,0.653834841417215,
2.29476933293416));
#45594=CARTESIAN_POINT('Ctrl Pts',(-0.680345878045539,0.717897660535232,
2.29695057049292));
#45595=CARTESIAN_POINT('Ctrl Pts',(-0.693505101313191,0.763966491903729,
2.29879280474844));
#45596=CARTESIAN_POINT('Ctrl Pts',(-0.727140785785948,0.885509443554027,
2.30366845023472));
#45597=CARTESIAN_POINT('Ctrl Pts',(-0.742080840142877,0.941055977840171,
2.30590657583669));
#45598=CARTESIAN_POINT('Ctrl Pts',(-0.770642745110105,1.03925891219064,
2.31034536042647));
#45599=CARTESIAN_POINT('Ctrl Pts',(-0.774973594025891,1.05301679619701,
2.31101997894399));
#45600=CARTESIAN_POINT('Ctrl Pts',(-0.799728192199698,1.13603289794848,
2.31501821430012));
#45601=CARTESIAN_POINT('Ctrl Pts',(-0.80800938904033,1.16420864772285,2.31637986922441));
#45602=CARTESIAN_POINT('Ctrl Pts',(-0.819024792214424,1.2,2.31822794574162));
#45603=CARTESIAN_POINT('',(-0.525742999963516,-0.653834841531101,2.27799895388173));
#45604=CARTESIAN_POINT('Ctrl Pts',(-0.525742999963516,-0.6538348415311,
2.27799895388173));
#45605=CARTESIAN_POINT('Ctrl Pts',(-0.539178158222297,-0.575804953766913,
2.31744060698703));
#45606=CARTESIAN_POINT('Ctrl Pts',(-0.5510914907315,-0.493927017715952,
2.35028134650557));
#45607=CARTESIAN_POINT('Ctrl Pts',(-0.570750430336647,-0.338205126032318,
2.39701000106415));
#45608=CARTESIAN_POINT('Ctrl Pts',(-0.578839025687772,-0.265719484524536,
2.41299248805411));
#45609=CARTESIAN_POINT('Ctrl Pts',(-0.593508015655536,-0.129748059605274,
2.43250299417119));
#45610=CARTESIAN_POINT('Ctrl Pts',(-0.60011071216539,-0.0666443969732617,
2.437507137828));
#45611=CARTESIAN_POINT('Ctrl Pts',(-0.613307700163344,0.0595551213823079,
2.43947987121095));
#45612=CARTESIAN_POINT('Ctrl Pts',(-0.619999920040576,0.122805235566241,
2.43648017139236));
#45613=CARTESIAN_POINT('Ctrl Pts',(-0.633837592454916,0.260158152186141,
2.42102084156086));
#45614=CARTESIAN_POINT('Ctrl Pts',(-0.640847266187103,0.333958596470524,
2.40693706705951));
#45615=CARTESIAN_POINT('Ctrl Pts',(-0.653889343793582,0.491154615715495,
2.36404811576026));
#45616=CARTESIAN_POINT('Ctrl Pts',(-0.659737685747932,0.574266546697417,
2.33304833098193));
#45617=CARTESIAN_POINT('Ctrl Pts',(-0.664237986648776,0.653834841429492,
2.29476933298692));
#45618=CARTESIAN_POINT('',(-0.597420188040714,-1.2,2.28618385377298));
#45619=CARTESIAN_POINT('Ctrl Pts',(-0.597420188040713,-1.2,2.28618385377298));
#45620=CARTESIAN_POINT('Ctrl Pts',(-0.58621931009426,-1.14022516977112,
2.28482205463156));
#45621=CARTESIAN_POINT('Ctrl Pts',(-0.570806616189584,-1.05518532565983,
2.28297763515456));
#45622=CARTESIAN_POINT('Ctrl Pts',(-0.538203119733082,-0.802969263789967,
2.27933097932797));
#45623=CARTESIAN_POINT('Ctrl Pts',(-0.531961053416311,-0.737455827809028,
2.27866313457685));
#45624=CARTESIAN_POINT('Ctrl Pts',(-0.525742999963516,-0.653834841531101,
2.27799895388173));
#45625=CARTESIAN_POINT('Ctrl Pts',(-0.65920976572758,-1.3,2.39500858640003));
#45626=CARTESIAN_POINT('Ctrl Pts',(-0.654919428780615,-1.29256895464929,
2.38691933116128));
#45627=CARTESIAN_POINT('Ctrl Pts',(-0.65006515276088,-1.28383644853562,
2.37744823415876));
#45628=CARTESIAN_POINT('Ctrl Pts',(-0.63921127668408,-1.26647251687147,
2.35848214642921));
#45629=CARTESIAN_POINT('Ctrl Pts',(-0.633575792945078,-1.25767778206492,
2.34887219755028));
#45630=CARTESIAN_POINT('Ctrl Pts',(-0.619746849269057,-1.23454545991039,
2.3237601019017));
#45631=CARTESIAN_POINT('Ctrl Pts',(-0.611419467297158,-1.22071295756083,
2.30875136315305));
#45632=CARTESIAN_POINT('Ctrl Pts',(-0.597420188040713,-1.2,2.28618385377298));
#45633=CARTESIAN_POINT('Origin',(0.,1.25,7.2));
#45634=CARTESIAN_POINT('Origin',(0.,1.2,7.2));
#45635=CARTESIAN_POINT('Origin',(0.,0.92691742076555,7.2));
#45636=CARTESIAN_POINT('Origin',(0.,0.653834841531101,7.2));
#45637=CARTESIAN_POINT('Origin',(0.,0.,7.2));
#45638=CARTESIAN_POINT('Origin',(0.,-0.653834841531101,7.2));
#45639=CARTESIAN_POINT('Origin',(0.,-0.926917420765551,7.2));
#45640=CARTESIAN_POINT('Origin',(0.,-1.2,7.2));
#45641=CARTESIAN_POINT('Origin',(0.,-1.25,7.2));
#45642=CARTESIAN_POINT('Ctrl Pts',(-0.23710229803321,-1.30000000000054,
2.16092425493151));
#45643=CARTESIAN_POINT('Ctrl Pts',(-0.279563873100975,-1.18514270861215,
2.1574563860945));
#45644=CARTESIAN_POINT('Ctrl Pts',(-0.312674005334788,-1.0684760419453,
2.16502926538751));
#45645=CARTESIAN_POINT('Ctrl Pts',(-0.367561330757957,-0.794772684000851,
2.20803046837806));
#45646=CARTESIAN_POINT('Ctrl Pts',(-0.36929976285042,-0.636309800095197,
2.27799949945684));
#45647=CARTESIAN_POINT('Ctrl Pts',(-0.393579787165995,-0.319434907277159,
2.34805851202106));
#45648=CARTESIAN_POINT('Ctrl Pts',(-0.392969830592777,-0.158333333333332,
2.39391966368106));
#45649=CARTESIAN_POINT('Ctrl Pts',(-0.426715573254503,0.158333333333334,
2.39694208628984));
#45650=CARTESIAN_POINT('Ctrl Pts',(-0.462594679682927,0.319434907277167,
2.35432227872907));
#45651=CARTESIAN_POINT('Ctrl Pts',(-0.503949232631023,0.636309800095206,
2.28997379608409));
#45652=CARTESIAN_POINT('Ctrl Pts',(-0.53791263772129,0.79477268400084,2.22384909509907));
#45653=CARTESIAN_POINT('Ctrl Pts',(-0.529237518130278,1.0684760419452,2.18307585697225));
#45654=CARTESIAN_POINT('Ctrl Pts',(-0.512888765856002,1.18514270861195,
2.17564712080097));
#45655=CARTESIAN_POINT('Ctrl Pts',(-0.483946399133539,1.30000000000025,
2.17843887244616));
#45656=CARTESIAN_POINT('Ctrl Pts',(-0.23037889702897,-1.30000000000054,
2.17151206948771));
#45657=CARTESIAN_POINT('Ctrl Pts',(-0.271622642083524,-1.18514270861215,
2.1700857215593));
#45658=CARTESIAN_POINT('Ctrl Pts',(-0.303818465808622,-1.0684760419453,
2.17914453006921));
#45659=CARTESIAN_POINT('Ctrl Pts',(-0.35729475106453,-0.794772684000851,
2.22429499885636));
#45660=CARTESIAN_POINT('Ctrl Pts',(-0.359072532092263,-0.636309800095197,
2.2938260406824));
#45661=CARTESIAN_POINT('Ctrl Pts',(-0.38320177356942,-0.319434907277159,
2.36391377144098));
#45662=CARTESIAN_POINT('Ctrl Pts',(-0.383232767764446,-0.158333333333332,
2.40917451598342));
#45663=CARTESIAN_POINT('Ctrl Pts',(-0.416530303335427,0.158333333333334,
2.41205592168762));
#45664=CARTESIAN_POINT('Ctrl Pts',(-0.451176432830852,0.319434907277167,
2.36985523556718));
#45665=CARTESIAN_POINT('Ctrl Pts',(-0.492061752143939,0.636309800095206,
2.30527281803725));
#45666=CARTESIAN_POINT('Ctrl Pts',(-0.525775129538417,0.79477268400084,
2.23950174011295));
#45667=CARTESIAN_POINT('Ctrl Pts',(-0.518587456936803,1.0684760419452,2.19658862087751));
#45668=CARTESIAN_POINT('Ctrl Pts',(-0.503305113780034,1.18514270861195,
2.18771675262694));
#45669=CARTESIAN_POINT('Ctrl Pts',(-0.475851704606216,1.30000000000025,
2.18854851535506));
#45670=CARTESIAN_POINT('Ctrl Pts',(-0.217486849125369,-1.30000000000053,
2.19275902390419));
#45671=CARTESIAN_POINT('Ctrl Pts',(-0.254683144397209,-1.18514270861214,
2.19506054551115));
#45672=CARTESIAN_POINT('Ctrl Pts',(-0.284135067288816,-1.06847604194529,
2.20689629477346));
#45673=CARTESIAN_POINT('Ctrl Pts',(-0.334283851550653,-0.794772684000841,
2.25626521650244));
#45674=CARTESIAN_POINT('Ctrl Pts',(-0.338793322038421,-0.636309800095192,
2.32556525340573));
#45675=CARTESIAN_POINT('Ctrl Pts',(-0.363329433692974,-0.319434907277158,
2.39588620577184));
#45676=CARTESIAN_POINT('Ctrl Pts',(-0.363675064915224,-0.158333333333331,
2.43968426685622));
#45677=CARTESIAN_POINT('Ctrl Pts',(-0.396341931007945,0.158333333333333,
2.44237024832289));
#45678=CARTESIAN_POINT('Ctrl Pts',(-0.429593854357203,0.319434907277163,
2.40133130890081));
#45679=CARTESIAN_POINT('Ctrl Pts',(-0.469702051421616,0.6363098000952,2.33633252607298));
#45680=CARTESIAN_POINT('Ctrl Pts',(-0.501938131550647,0.794772684000836,
2.2709886809046));
#45681=CARTESIAN_POINT('Ctrl Pts',(-0.497754652750861,1.06847604194519,
2.22378244535553));
#45682=CARTESIAN_POINT('Ctrl Pts',(-0.484798075460762,1.18514270861194,
2.21206487283401));
#45683=CARTESIAN_POINT('Ctrl Pts',(-0.460695793839825,1.30000000000024,
2.20906355799674));
#45684=CARTESIAN_POINT('Ctrl Pts',(-0.203987185474402,-1.30000000000052,
2.214758458624));
#45685=CARTESIAN_POINT('Ctrl Pts',(-0.23961805702658,-1.18514270861213,
2.22151036131582));
#45686=CARTESIAN_POINT('Ctrl Pts',(-0.267751852323117,-1.06847604194529,
2.23655683376414));
#45687=CARTESIAN_POINT('Ctrl Pts',(-0.315426801669056,-0.794772684000844,
2.29047931061677));
#45688=CARTESIAN_POINT('Ctrl Pts',(-0.318775093621048,-0.636309800095191,
2.35857908568481));
#45689=CARTESIAN_POINT('Ctrl Pts',(-0.342581858116448,-0.319434907277156,
2.42886303170086));
#45690=CARTESIAN_POINT('Ctrl Pts',(-0.344246402265609,-0.158333333333331,
2.47140640159224));
#45691=CARTESIAN_POINT('Ctrl Pts',(-0.37623154697275,0.158333333333332,
2.47388795006401));
#45692=CARTESIAN_POINT('Ctrl Pts',(-0.407774234211117,0.319434907277162,
2.43398194626325));
#45693=CARTESIAN_POINT('Ctrl Pts',(-0.446629603902531,0.636309800095197,
2.36843534653642));
#45694=CARTESIAN_POINT('Ctrl Pts',(-0.476792671236336,0.794772684000832,
2.30338734799053));
#45695=CARTESIAN_POINT('Ctrl Pts',(-0.475569911788654,1.06847604194519,
2.25170214312543));
#45696=CARTESIAN_POINT('Ctrl Pts',(-0.465073405724185,1.18514270861194,
2.23705598928701));
#45697=CARTESIAN_POINT('Ctrl Pts',(-0.444609680852444,1.30000000000024,
2.23013629167068));
#45698=CARTESIAN_POINT('Ctrl Pts',(-0.196765310466802,-1.30000000000052,
2.22675804947393));
#45699=CARTESIAN_POINT('Ctrl Pts',(-0.230479558059957,-1.18514270861213,
2.23570308762627));
#45700=CARTESIAN_POINT('Ctrl Pts',(-0.257286379630178,-1.06847604194529,
2.25237013581518));
#45701=CARTESIAN_POINT('Ctrl Pts',(-0.303257964204822,-0.794772684000841,
2.30871373933043));
#45702=CARTESIAN_POINT('Ctrl Pts',(-0.307547430038605,-0.636309800095188,
2.37653176265635));
#45703=CARTESIAN_POINT('Ctrl Pts',(-0.331675110731546,-0.319434907277154,
2.44697160924118));
#45704=CARTESIAN_POINT('Ctrl Pts',(-0.334160629348225,-0.15833333333333,
2.48885337959328));
#45705=CARTESIAN_POINT('Ctrl Pts',(-0.365788030374307,0.158333333333332,
2.49122950080718));
#45706=CARTESIAN_POINT('Ctrl Pts',(-0.395864725591021,0.319434907277162,
2.4518083484711));
#45707=CARTESIAN_POINT('Ctrl Pts',(-0.434255637160026,0.636309800095196,
2.38603637581062));
#45708=CARTESIAN_POINT('Ctrl Pts',(-0.464309478206796,0.794772684000828,
2.32144581257927));
#45709=CARTESIAN_POINT('Ctrl Pts',(-0.464699374822084,1.06847604194518,
2.26731063655238));
#45710=CARTESIAN_POINT('Ctrl Pts',(-0.455323241083783,1.18514270861193,
2.25099782135537));
#45711=CARTESIAN_POINT('Ctrl Pts',(-0.436402201809517,1.30000000000024,
2.24180530275743));
#45712=CARTESIAN_POINT('Ctrl Pts',(-0.195199715251824,-1.30000000000052,
2.22943365900812));
#45713=CARTESIAN_POINT('Ctrl Pts',(-0.228511605709378,-1.18514270861213,
2.23887200063285));
#45714=CARTESIAN_POINT('Ctrl Pts',(-0.255035966884731,-1.06847604194529,
2.25590238609696));
#45715=CARTESIAN_POINT('Ctrl Pts',(-0.300631996897572,-0.794772684000841,
2.31278512348812));
#45716=CARTESIAN_POINT('Ctrl Pts',(-0.3050843378607,-0.636309800095188,
2.38052940242937));
#45717=CARTESIAN_POINT('Ctrl Pts',(-0.329268192136499,-0.319434907277154,
2.45100060187918));
#45718=CARTESIAN_POINT('Ctrl Pts',(-0.331946826089393,-0.15833333333333,
2.49273820395524));
#45719=CARTESIAN_POINT('Ctrl Pts',(-0.363497908369338,0.158333333333332,
2.49509203294361));
#45720=CARTESIAN_POINT('Ctrl Pts',(-0.393261813609874,0.319434907277162,
2.4557823768547));
#45721=CARTESIAN_POINT('Ctrl Pts',(-0.431529408639268,0.636309800095196,
2.38995478658298));
#45722=CARTESIAN_POINT('Ctrl Pts',(-0.461506431291599,0.794772684000829,
2.32545116428567));
#45723=CARTESIAN_POINT('Ctrl Pts',(-0.462246199763164,1.06847604194518,
2.27076906174921));
#45724=CARTESIAN_POINT('Ctrl Pts',(-0.453125679257506,1.18514270861193,
2.25408765585355));
#45725=CARTESIAN_POINT('Ctrl Pts',(-0.434564419885971,1.30000000000024,
2.24439470007868));
#45726=CARTESIAN_POINT('Ctrl Pts',(-0.192498978829482,-1.30000000000052,
2.23412609993294));
#45727=CARTESIAN_POINT('Ctrl Pts',(-0.225164896758017,-1.18514270861213,
2.24444120170032));
#45728=CARTESIAN_POINT('Ctrl Pts',(-0.251230206622433,-1.06847604194529,
2.26211564508765));
#45729=CARTESIAN_POINT('Ctrl Pts',(-0.296197561681345,-0.794772684000842,
2.31994869644595));
#45730=CARTESIAN_POINT('Ctrl Pts',(-0.300879303052548,-0.636309800095188,
2.38755164020039));
#45731=CARTESIAN_POINT('Ctrl Pts',(-0.325102701053619,-0.319434907277154,
2.45806382649142));
#45732=CARTESIAN_POINT('Ctrl Pts',(-0.328044816463848,-0.15833333333333,
2.49953034053383));
#45733=CARTESIAN_POINT('Ctrl Pts',(-0.35945797715739,0.158333333333332,
2.50184484158941));
#45734=CARTESIAN_POINT('Ctrl Pts',(-0.388773823191552,0.319434907277163,
2.46275680073802));
#45735=CARTESIAN_POINT('Ctrl Pts',(-0.426815973398791,0.636309800095197,
2.39682877981381));
#45736=CARTESIAN_POINT('Ctrl Pts',(-0.456543389710484,0.794772684000829,
2.33244524985028));
#45737=CARTESIAN_POINT('Ctrl Pts',(-0.457879092298719,1.06847604194518,
2.27680127571584));
#45738=CARTESIAN_POINT('Ctrl Pts',(-0.449218539438891,1.18514270861193,
2.25947826437128));
#45739=CARTESIAN_POINT('Ctrl Pts',(-0.431319257561445,1.30000000000024,
2.24891845627251));
#45740=CARTESIAN_POINT('Ctrl Pts',(-0.188774259644139,-1.30000000000052,
2.24086591573252));
#45741=CARTESIAN_POINT('Ctrl Pts',(-0.220761800809493,-1.18514270861213,
2.25249001056503));
#45742=CARTESIAN_POINT('Ctrl Pts',(-0.246313953205146,-1.06847604194529,
2.27111754735347));
#45743=CARTESIAN_POINT('Ctrl Pts',(-0.290477501476522,-0.794772684000842,
2.3303302357127));
#45744=CARTESIAN_POINT('Ctrl Pts',(-0.295187700097743,-0.636309800095188,
2.39766367135058));
#45745=CARTESIAN_POINT('Ctrl Pts',(-0.319235607269039,-0.319434907277154,
2.46817891569942));
#45746=CARTESIAN_POINT('Ctrl Pts',(-0.322322740325068,-0.15833333333333,
2.5091980855775));
#45747=CARTESIAN_POINT('Ctrl Pts',(-0.353563922818734,0.158333333333332,
2.51146496858702));
#45748=CARTESIAN_POINT('Ctrl Pts',(-0.382669103484203,0.319434907277162,
2.47280848790605));
#45749=CARTESIAN_POINT('Ctrl Pts',(-0.420319849785342,0.636309800095197,
2.40671557072077));
#45750=CARTESIAN_POINT('Ctrl Pts',(-0.449113853348591,0.794772684000829,
2.34234273613684));
#45751=CARTESIAN_POINT('Ctrl Pts',(-0.451226557067176,1.06847604194518,
2.28530388129556));
#45752=CARTESIAN_POINT('Ctrl Pts',(-0.443293415857577,1.18514270861193,
2.26708407448722));
#45753=CARTESIAN_POINT('Ctrl Pts',(-0.42651262228199,1.30000000000024,2.25533446763348));
#45754=CARTESIAN_POINT('Ctrl Pts',(-0.184328545390968,-1.30000000000052,
2.24896206272598));
#45755=CARTESIAN_POINT('Ctrl Pts',(-0.215531490467412,-1.18514270861213,
2.26216516228258));
#45756=CARTESIAN_POINT('Ctrl Pts',(-0.24050201101214,-1.06847604194529,
2.28194518505679));
#45757=CARTESIAN_POINT('Ctrl Pts',(-0.283790761345431,-0.794772684000842,
2.34283500298682));
#45758=CARTESIAN_POINT('Ctrl Pts',(-0.288643793743644,-0.636309800095188,
2.40986833321706));
#45759=CARTESIAN_POINT('Ctrl Pts',(-0.312515191936046,-0.319434907277154,
2.48039519284905));
#45760=CARTESIAN_POINT('Ctrl Pts',(-0.315731313772672,-0.15833333333333,
2.52086741844874));
#45761=CARTESIAN_POINT('Ctrl Pts',(-0.34669078838051,0.158333333333332,
2.52306197531978));
#45762=CARTESIAN_POINT('Ctrl Pts',(-0.375413617338691,0.319434907277163,
2.48489524842215));
#45763=CARTESIAN_POINT('Ctrl Pts',(-0.41260931729808,0.636309800095197,
2.41861256260139));
#45764=CARTESIAN_POINT('Ctrl Pts',(-0.44050809088814,0.794772684000828,
2.35431264723303));
#45765=CARTESIAN_POINT('Ctrl Pts',(-0.443527260501794,1.06847604194518,
2.29559133893406));
#45766=CARTESIAN_POINT('Ctrl Pts',(-0.436404963162388,1.18514270861193,
2.27627729439076));
#45767=CARTESIAN_POINT('Ctrl Pts',(-0.420853481829084,1.30000000000024,
2.26306748382789));
#45768=CARTESIAN_POINT('Ctrl Pts',(-0.174910013499284,-1.30000000000052,
2.26503509219293));
#45769=CARTESIAN_POINT('Ctrl Pts',(-0.203859450038737,-1.18514270861213,
2.28124294331675));
#45770=CARTESIAN_POINT('Ctrl Pts',(-0.22727026814655,-1.06847604194529,
2.303239677686));
#45771=CARTESIAN_POINT('Ctrl Pts',(-0.268558624719782,-0.794772684000844,
2.36743001286962));
#45772=CARTESIAN_POINT('Ctrl Pts',(-0.274445600499521,-0.63630980009519,
2.43403204898114));
#45773=CARTESIAN_POINT('Ctrl Pts',(-0.298847530016446,-0.319434907277155,
2.50478811328702));
#45774=CARTESIAN_POINT('Ctrl Pts',(-0.303369005641152,-0.158333333333331,
2.54441508328069));
#45775=CARTESIAN_POINT('Ctrl Pts',(-0.33395136203271,0.158333333333332,
2.54650477121987));
#45776=CARTESIAN_POINT('Ctrl Pts',(-0.360815451669037,0.319434907277163,
2.50904263688917));
#45777=CARTESIAN_POINT('Ctrl Pts',(-0.397071501484818,0.636309800095199,
2.44239004595036));
#45778=CARTESIAN_POINT('Ctrl Pts',(-0.42418690064276,0.794772684000832,
2.37852820842571));
#45779=CARTESIAN_POINT('Ctrl Pts',(-0.429032737882111,1.06847604194518,
2.31644541810441));
#45780=CARTESIAN_POINT('Ctrl Pts',(-0.423348465701274,1.18514270861193,
2.29488743588331));
#45781=CARTESIAN_POINT('Ctrl Pts',(-0.409882337954649,1.30000000000024,
2.2786448109771));
#45782=CARTESIAN_POINT('Ctrl Pts',(-0.161385254501694,-1.30000000000053,
2.2892981725789));
#45783=CARTESIAN_POINT('Ctrl Pts',(-0.187539772745063,-1.18514270861214,
2.31015635569105));
#45784=CARTESIAN_POINT('Ctrl Pts',(-0.209011612456179,-1.06847604194529,
2.33557535851787));
#45785=CARTESIAN_POINT('Ctrl Pts',(-0.247797933439514,-0.794772684000842,
2.40483474603162));
#45786=CARTESIAN_POINT('Ctrl Pts',(-0.255171667431664,-0.636309800095193,
2.47076334358962));
#45787=CARTESIAN_POINT('Ctrl Pts',(-0.279737090842208,-0.319434907277158,
2.54171341616012));
#45788=CARTESIAN_POINT('Ctrl Pts',(-0.285111694857768,-0.158333333333332,
2.5798145786153));
#45789=CARTESIAN_POINT('Ctrl Pts',(-0.314492438641538,0.158333333333333,
2.58160947030076));
#45790=CARTESIAN_POINT('Ctrl Pts',(-0.338654340348441,0.319434907277165,
2.54524103218855));
#45791=CARTESIAN_POINT('Ctrl Pts',(-0.373618100687796,0.636309800095203,
2.47807365514528));
#45792=CARTESIAN_POINT('Ctrl Pts',(-0.399938319148561,0.794772684000837,
2.4149649714314));
#45793=CARTESIAN_POINT('Ctrl Pts',(-0.407722780808801,1.06847604194519,
2.3478777040346));
#45794=CARTESIAN_POINT('Ctrl Pts',(-0.404239921251716,1.18514270861194,
2.32295585827381));
#45795=CARTESIAN_POINT('Ctrl Pts',(-0.393904597127559,1.30000000000024,
2.30215175898006));
#45796=CARTESIAN_POINT('Ctrl Pts',(-0.146809047088256,-1.30000000000053,
2.31639257663108));
#45797=CARTESIAN_POINT('Ctrl Pts',(-0.17035904517932,-1.18514270861214,
2.34253335301815));
#45798=CARTESIAN_POINT('Ctrl Pts',(-0.189882529958076,-1.0684760419453,
2.37180591564467));
#45799=CARTESIAN_POINT('Ctrl Pts',(-0.225683634204065,-0.79477268400085,
2.44666644399284));
#45800=CARTESIAN_POINT('Ctrl Pts',(-0.233149339068538,-0.636309800095195,
2.51151894746034));
#45801=CARTESIAN_POINT('Ctrl Pts',(-0.257520567695809,-0.319434907277158,
2.58260649354533));
#45802=CARTESIAN_POINT('Ctrl Pts',(-0.264089158815809,-0.158333333333332,
2.61904131619651));
#45803=CARTESIAN_POINT('Ctrl Pts',(-0.293310913161025,0.158333333333334,
2.62079205167843));
#45804=CARTESIAN_POINT('Ctrl Pts',(-0.316494245938754,0.319434907277166,
2.58614460955811));
#45805=CARTESIAN_POINT('Ctrl Pts',(-0.350565709671562,0.636309800095204,
2.51854854226647));
#45806=CARTESIAN_POINT('Ctrl Pts',(-0.374729044259226,0.794772684000838,
2.45598692227775));
#45807=CARTESIAN_POINT('Ctrl Pts',(-0.385059698318788,1.06847604194519,
2.38314652081434));
#45808=CARTESIAN_POINT('Ctrl Pts',(-0.383746823487437,1.18514270861194,
2.35440335971755));
#45809=CARTESIAN_POINT('Ctrl Pts',(-0.376649316470808,1.30000000000025,
2.32844694831461));
#45810=CARTESIAN_POINT('Ctrl Pts',(-0.13654826093367,-1.30000000000053,
2.33535361499277));
#45811=CARTESIAN_POINT('Ctrl Pts',(-0.15790384335973,-1.18514270861214,
2.36512816857481));
#45812=CARTESIAN_POINT('Ctrl Pts',(-0.176036468676417,-1.0684760419453,
2.3971009256881));
#45813=CARTESIAN_POINT('Ctrl Pts',(-0.210480784904201,-0.794772684000849,
2.47604268065416));
#45814=CARTESIAN_POINT('Ctrl Pts',(-0.220295824447027,-0.636309800095195,
2.54059970789379));
#45815=CARTESIAN_POINT('Ctrl Pts',(-0.245157968739213,-0.319434907277158,
2.61191683972681));
#45816=CARTESIAN_POINT('Ctrl Pts',(-0.251778225887239,-0.158333333333332,
2.64703880121469));
#45817=CARTESIAN_POINT('Ctrl Pts',(-0.279851723982855,0.158333333333334,
2.64854512769776));
#45818=CARTESIAN_POINT('Ctrl Pts',(-0.30128193470898,0.319434907277167,
2.61487674221445));
#45819=CARTESIAN_POINT('Ctrl Pts',(-0.333650395581517,0.636309800095205,
2.54673533789483));
#45820=CARTESIAN_POINT('Ctrl Pts',(-0.355724212092589,0.794772684000839,
2.48439750673184));
#45821=CARTESIAN_POINT('Ctrl Pts',(-0.367923974421454,1.06847604194519,
2.40754388914988));
#45822=CARTESIAN_POINT('Ctrl Pts',(-0.368405927183787,1.18514270861194,
2.37619008452405));
#45823=CARTESIAN_POINT('Ctrl Pts',(-0.364089007642033,1.30000000000025,
2.34674955861646));
#45824=CARTESIAN_POINT('Ctrl Pts',(-0.131007506657736,-1.30000000000053,
2.34626587470766));
#45825=CARTESIAN_POINT('Ctrl Pts',(-0.151677974919239,-1.18514270861214,
2.37822797434374));
#45826=CARTESIAN_POINT('Ctrl Pts',(-0.169230547683712,-1.0684760419453,
2.41178482509803));
#45827=CARTESIAN_POINT('Ctrl Pts',(-0.202577539818775,-0.794772684000848,
2.49299205747734));
#45828=CARTESIAN_POINT('Ctrl Pts',(-0.211744813925583,-0.636309800095194,
2.55698483279202));
#45829=CARTESIAN_POINT('Ctrl Pts',(-0.236497253167826,-0.319434907277158,
2.62835347341668));
#45830=CARTESIAN_POINT('Ctrl Pts',(-0.244001971332526,-0.158333333333332,
2.66288630110204));
#45831=CARTESIAN_POINT('Ctrl Pts',(-0.27224584620091,0.158333333333334,
2.66442924486541));
#45832=CARTESIAN_POINT('Ctrl Pts',(-0.293250336416526,0.319434907277167,
2.6314482563698));
#45833=CARTESIAN_POINT('Ctrl Pts',(-0.325488171395546,0.636309800095204,
2.56320436175243));
#45834=CARTESIAN_POINT('Ctrl Pts',(-0.347152213240066,0.794772684000837,
2.50122002778829));
#45835=CARTESIAN_POINT('Ctrl Pts',(-0.360242452059197,1.06847604194519,
2.42203040362271));
#45836=CARTESIAN_POINT('Ctrl Pts',(-0.361398471314416,1.18514270861194,
2.38909240542061));
#45837=CARTESIAN_POINT('Ctrl Pts',(-0.358044230481204,1.30000000000025,
2.35749466305292));
#45838=CARTESIAN_POINT('Ctrl Pts',(-0.117086432067252,-1.30000000000053,
2.37352320141344));
#45839=CARTESIAN_POINT('Ctrl Pts',(-0.135464168151512,-1.18514270861214,
2.41084675042037));
#45840=CARTESIAN_POINT('Ctrl Pts',(-0.151415182366122,-1.0684760419453,
2.44833956525444));
#45841=CARTESIAN_POINT('Ctrl Pts',(-0.182659003208377,-0.794772684000852,
2.53534650585518));
#45842=CARTESIAN_POINT('Ctrl Pts',(-0.192742903268561,-0.636309800095196,
2.59843213671961));
#45843=CARTESIAN_POINT('Ctrl Pts',(-0.218000695569017,-0.319434907277158,
2.67008470161751));
#45844=CARTESIAN_POINT('Ctrl Pts',(-0.227426550264204,-0.158333333333332,
2.70309560096028));
#45845=CARTESIAN_POINT('Ctrl Pts',(-0.254291257836203,0.158333333333334,
2.7043467724717));
#45846=CARTESIAN_POINT('Ctrl Pts',(-0.271370755899094,0.319434907277166,
2.67248169616074));
#45847=CARTESIAN_POINT('Ctrl Pts',(-0.301566418481218,0.636309800095204,
2.60359226481184));
#45848=CARTESIAN_POINT('Ctrl Pts',(-0.322608338668808,0.794772684000839,
2.54251943597892));
#45849=CARTESIAN_POINT('Ctrl Pts',(-0.338076543906821,1.06847604194519,
2.45752302061236));
#45850=CARTESIAN_POINT('Ctrl Pts',(-0.341108322545931,1.18514270861194,
2.42067933094224));
#45851=CARTESIAN_POINT('Ctrl Pts',(-0.340476266930105,1.30000000000025,
2.38378375038661));
#45852=CARTESIAN_POINT('Ctrl Pts',(-0.102459815942602,-1.30000000000054,
2.40364627470184));
#45853=CARTESIAN_POINT('Ctrl Pts',(-0.117674774015024,-1.18514270861215,
2.44677221732563));
#45854=CARTESIAN_POINT('Ctrl Pts',(-0.131530737499575,-1.0684760419453,
2.4885471284722));
#45855=CARTESIAN_POINT('Ctrl Pts',(-0.16040123566095,-0.794772684000851,
2.58193437727779));
#45856=CARTESIAN_POINT('Ctrl Pts',(-0.172912540708817,-0.6363098000952,
2.64425616831593));
#45857=CARTESIAN_POINT('Ctrl Pts',(-0.1989153384542,-0.319434907277161,
2.71624566671582));
#45858=CARTESIAN_POINT('Ctrl Pts',(-0.208972852561719,-0.158333333333333,
2.74727571056124));
#45859=CARTESIAN_POINT('Ctrl Pts',(-0.235436629275575,0.158333333333335,
2.74847840266072));
#45860=CARTESIAN_POINT('Ctrl Pts',(-0.251633688396625,0.319434907277168,
2.71862485889545));
#45861=CARTESIAN_POINT('Ctrl Pts',(-0.27996183079859,0.636309800095209,
2.64913850896298));
#45862=CARTESIAN_POINT('Ctrl Pts',(-0.297052837237228,0.794772684000849,
2.58836982198733));
#45863=CARTESIAN_POINT('Ctrl Pts',(-0.314711528711115,1.0684760419452,2.49688671813418));
#45864=CARTESIAN_POINT('Ctrl Pts',(-0.320125739500395,1.18514270861194,
2.4558064169721));
#45865=CARTESIAN_POINT('Ctrl Pts',(-0.323310367858915,1.30000000000024,
2.41324546052289));
#45866=CARTESIAN_POINT('Ctrl Pts',(-0.0865550189114888,-1.30000000000053,
2.43952180316623));
#45867=CARTESIAN_POINT('Ctrl Pts',(-0.0998021354031824,-1.18514270861214,
2.48981119458842));
#45868=CARTESIAN_POINT('Ctrl Pts',(-0.112284312155286,-1.0684760419453,
2.53683713334547));
#45869=CARTESIAN_POINT('Ctrl Pts',(-0.139353473679405,-0.794772684000851,
2.63793723087301));
#45870=CARTESIAN_POINT('Ctrl Pts',(-0.152637834139488,-0.636309800095197,
2.69899428288379));
#45871=CARTESIAN_POINT('Ctrl Pts',(-0.179118060090335,-0.319434907277159,
2.77130691967836));
#45872=CARTESIAN_POINT('Ctrl Pts',(-0.190776149896774,-0.158333333333333,
2.80013566926875));
#45873=CARTESIAN_POINT('Ctrl Pts',(-0.216342800555802,0.158333333333334,
2.80120353145493));
#45874=CARTESIAN_POINT('Ctrl Pts',(-0.230069884093391,0.319434907277167,
2.7734491731441));
#45875=CARTESIAN_POINT('Ctrl Pts',(-0.256036740898905,0.636309800095206,
2.70329839544103));
#45876=CARTESIAN_POINT('Ctrl Pts',(-0.270614438129939,0.794772684000843,
2.64345562366289));
#45877=CARTESIAN_POINT('Ctrl Pts',(-0.289603342540349,1.0684760419452,2.54405830878662));
#45878=CARTESIAN_POINT('Ctrl Pts',(-0.296607782659313,1.18514270861194,
2.49769499621475));
#45879=CARTESIAN_POINT('Ctrl Pts',(-0.302397069786226,1.30000000000025,
2.44799378564747));
#45880=CARTESIAN_POINT('Ctrl Pts',(-0.0768451818344205,-1.30000000000054,
2.46162868799514));
#45881=CARTESIAN_POINT('Ctrl Pts',(-0.0886298667164653,-1.18514270861215,
2.51630195144563));
#45882=CARTESIAN_POINT('Ctrl Pts',(-0.100195850955182,-1.0684760419453,
2.56655815518386));
#45883=CARTESIAN_POINT('Ctrl Pts',(-0.12641034607682,-0.794772684000849,
2.67245574797313));
#45884=CARTESIAN_POINT('Ctrl Pts',(-0.141376457236268,-0.636309800095196,
2.73290525740483));
#45885=CARTESIAN_POINT('Ctrl Pts',(-0.168174688062727,-0.319434907277159,
2.80543061378637));
#45886=CARTESIAN_POINT('Ctrl Pts',(-0.179809506090771,-0.158333333333332,
2.83277077134714));
#45887=CARTESIAN_POINT('Ctrl Pts',(-0.204422827610632,0.158333333333334,
2.83370548581378));
#45888=CARTESIAN_POINT('Ctrl Pts',(-0.216900306221677,0.319434907277168,
2.80728899553676));
#45889=CARTESIAN_POINT('Ctrl Pts',(-0.241258190720355,0.636309800095206,
2.7366900875382));
#45890=CARTESIAN_POINT('Ctrl Pts',(-0.253585277081685,0.79477268400084,
2.67725991227328));
#45891=CARTESIAN_POINT('Ctrl Pts',(-0.273931795003457,1.06847604194519,
2.57308619511324));
#45892=CARTESIAN_POINT('Ctrl Pts',(-0.282418983421977,1.18514270861194,
2.52356751859579));
#45893=CARTESIAN_POINT('Ctrl Pts',(-0.29058610656347,1.30000000000025,2.46962310770284));
#45894=CARTESIAN_POINT('Ctrl Pts',(-0.0646419694895159,-1.30000000000053,
2.49219986215409));
#45895=CARTESIAN_POINT('Ctrl Pts',(-0.0746299031266144,-1.18514270861214,
2.55291253567633));
#45896=CARTESIAN_POINT('Ctrl Pts',(-0.085042776570219,-1.0684760419453,
2.60760959069788));
#45897=CARTESIAN_POINT('Ctrl Pts',(-0.11008029327507,-0.794772684000852,
2.72007344774905));
#45898=CARTESIAN_POINT('Ctrl Pts',(-0.12639262512847,-0.636309800095197,
2.77954489993001));
#45899=CARTESIAN_POINT('Ctrl Pts',(-0.154435156546678,-0.319434907277159,
2.8524506143583));
#45900=CARTESIAN_POINT('Ctrl Pts',(-0.168270150482634,-0.158333333333332,
2.8780204502782));
#45901=CARTESIAN_POINT('Ctrl Pts',(-0.192020606839366,0.158333333333334,
2.87885542318024));
#45902=CARTESIAN_POINT('Ctrl Pts',(-0.201146304914863,0.319434907277166,
2.85409248168455));
#45903=CARTESIAN_POINT('Ctrl Pts',(-0.223090436112119,0.636309800095205,
2.78294474077531));
#45904=CARTESIAN_POINT('Ctrl Pts',(-0.234079952238902,0.794772684000841,
2.72448047421197));
#45905=CARTESIAN_POINT('Ctrl Pts',(-0.255131024103306,1.06847604194519,
2.61355633361972));
#45906=CARTESIAN_POINT('Ctrl Pts',(-0.264576696026548,1.18514270861194,
2.55949554128694));
#45907=CARTESIAN_POINT('Ctrl Pts',(-0.274355810882019,1.30000000000025,
2.4993889069393));
#45908=CARTESIAN_POINT('Ctrl Pts',(-0.0519913323925298,-1.30000000000053,
2.52275042090885));
#45909=CARTESIAN_POINT('Ctrl Pts',(-0.0603550360115123,-1.18514270861215,
2.58957328418298));
#45910=CARTESIAN_POINT('Ctrl Pts',(-0.0699500144714583,-1.0684760419453,
2.64878750700434));
#45911=CARTESIAN_POINT('Ctrl Pts',(-0.0949608253810958,-0.794772684000853,
2.76800672593707));
#45912=CARTESIAN_POINT('Ctrl Pts',(-0.114769504529623,-0.636309800095196,
2.82673663023976));
#45913=CARTESIAN_POINT('Ctrl Pts',(-0.144041513703257,-0.319434907277158,
2.90003545779939));
#45914=CARTESIAN_POINT('Ctrl Pts',(-0.157655646790745,-0.158333333333332,
2.92354881563667));
#45915=CARTESIAN_POINT('Ctrl Pts',(-0.180115264216867,0.158333333333334,
2.92426615222108));
#45916=CARTESIAN_POINT('Ctrl Pts',(-0.187731724656436,0.319434907277168,
2.90145517946238));
#45917=CARTESIAN_POINT('Ctrl Pts',(-0.20671177222343,0.636309800095206,
2.82964797001604));
#45918=CARTESIAN_POINT('Ctrl Pts',(-0.213393728431101,0.79477268400084,
2.77160923968283));
#45919=CARTESIAN_POINT('Ctrl Pts',(-0.235286231852892,1.06847604194519,
2.65393411759689));
#45920=CARTESIAN_POINT('Ctrl Pts',(-0.246410895641012,1.18514270861195,
2.59544671058704));
#45921=CARTESIAN_POINT('Ctrl Pts',(-0.259183769683156,1.30000000000025,
2.52940909662534));
#45922=CARTESIAN_POINT('Ctrl Pts',(-0.0414484880036898,-1.30000000000054,
2.55063756703304));
#45923=CARTESIAN_POINT('Ctrl Pts',(-0.0488098275549564,-1.18514270861215,
2.62300797498182));
#45924=CARTESIAN_POINT('Ctrl Pts',(-0.0579766463248268,-1.0684760419453,
2.68631168921085));
#45925=CARTESIAN_POINT('Ctrl Pts',(-0.0833248496788771,-0.794772684000855,
2.81161005666598));
#45926=CARTESIAN_POINT('Ctrl Pts',(-0.105626363343272,-0.636309800095197,
2.86953587407838));
#45927=CARTESIAN_POINT('Ctrl Pts',(-0.136562091200086,-0.319434907277158,
2.94320934801511));
#45928=CARTESIAN_POINT('Ctrl Pts',(-0.151314127698468,-0.158333333333332,
2.9650077768798));
#45929=CARTESIAN_POINT('Ctrl Pts',(-0.172923006523827,0.158333333333334,
2.96568282352302));
#45930=CARTESIAN_POINT('Ctrl Pts',(-0.178177065531442,0.319434907277166,
2.94454480196698));
#45931=CARTESIAN_POINT('Ctrl Pts',(-0.194521822168287,0.636309800095205,
2.87227616870795));
#45932=CARTESIAN_POINT('Ctrl Pts',(-0.198901964219526,0.794772684000839,
2.81502334955911));
#45933=CARTESIAN_POINT('Ctrl Pts',(-0.220501886149653,1.06847604194519,
2.69114356802193));
#45934=CARTESIAN_POINT('Ctrl Pts',(-0.232142923985034,1.18514270861195,
2.62849680372957));
#45935=CARTESIAN_POINT('Ctrl Pts',(-0.246075193808231,1.30000000000025,
2.55682624237401));
#45936=CARTESIAN_POINT('Ctrl Pts',(-0.0349002835201406,-1.30000000000054,
2.57033915626948));
#45937=CARTESIAN_POINT('Ctrl Pts',(-0.0414916171038198,-1.18514270861215,
2.64672432756028));
#45938=CARTESIAN_POINT('Ctrl Pts',(-0.0504134225591142,-1.06847604194531,
2.71299807230647));
#45939=CARTESIAN_POINT('Ctrl Pts',(-0.0764084341946251,-0.794772684000856,
2.84274426258533));
#45940=CARTESIAN_POINT('Ctrl Pts',(-0.102183974764143,-0.636309800095198,
2.90025606522728));
#45941=CARTESIAN_POINT('Ctrl Pts',(-0.133047562883809,-0.319434907277158,
2.974084380369));
#45942=CARTESIAN_POINT('Ctrl Pts',(-0.144704112048905,-0.158333333333333,
2.99426031153481));
#45943=CARTESIAN_POINT('Ctrl Pts',(-0.165081364601521,0.158333333333334,
2.99485565250151));
#45944=CARTESIAN_POINT('Ctrl Pts',(-0.171572628444762,0.319434907277168,
2.97524810931612));
#45945=CARTESIAN_POINT('Ctrl Pts',(-0.186757244390619,0.636309800095207,
2.90268736214996));
#45946=CARTESIAN_POINT('Ctrl Pts',(-0.188248554710682,0.79477268400084,
2.84579042814529));
#45947=CARTESIAN_POINT('Ctrl Pts',(-0.209521808555664,1.0684760419452,2.71738892262339));
#45948=CARTESIAN_POINT('Ctrl Pts',(-0.221625126237946,1.18514270861195,
2.65174871878311));
#45949=CARTESIAN_POINT('Ctrl Pts',(-0.23662335826476,1.30000000000025,2.57604856509829));
#45950=CARTESIAN_POINT('Ctrl Pts',(-0.029992213072004,-1.30000000000054,
2.58428069475767));
#45951=CARTESIAN_POINT('Ctrl Pts',(-0.0369470821443265,-1.18514270861215,
2.66342490778013));
#45952=CARTESIAN_POINT('Ctrl Pts',(-0.0459491733771234,-1.0684760419453,
2.73169045003337));
#45953=CARTESIAN_POINT('Ctrl Pts',(-0.0714752977231339,-0.794772684000853,
2.86426560336564));
#45954=CARTESIAN_POINT('Ctrl Pts',(-0.0957112928916897,-0.636309800095197,
2.92106492372564));
#45955=CARTESIAN_POINT('Ctrl Pts',(-0.125688940043713,-0.319434907277158,
2.99483448775138));
#45956=CARTESIAN_POINT('Ctrl Pts',(-0.137027468646895,-0.158333333333333,
3.01402881780954));
#45957=CARTESIAN_POINT('Ctrl Pts',(-0.157981527487602,0.158333333333334,
3.01470166475779));
#45958=CARTESIAN_POINT('Ctrl Pts',(-0.166223436350055,0.319434907277168,
2.99624892902451));
#45959=CARTESIAN_POINT('Ctrl Pts',(-0.181725666151248,0.636309800095206,
2.92370987232953));
#45960=CARTESIAN_POINT('Ctrl Pts',(-0.18163490289444,0.79477268400084,2.86722018173556));
#45961=CARTESIAN_POINT('Ctrl Pts',(-0.202993381777807,1.0684760419452,2.73591708451799));
#45962=CARTESIAN_POINT('Ctrl Pts',(-0.215428171523888,1.18514270861195,
2.66830058285085));
#45963=CARTESIAN_POINT('Ctrl Pts',(-0.231052456917079,1.30000000000025,
2.58990382504281));
#45964=CARTESIAN_POINT('Ctrl Pts',(-0.0249600309789205,-1.30000000000054,
2.60124271611029));
#45965=CARTESIAN_POINT('Ctrl Pts',(-0.0323202509065839,-1.18514270861215,
2.68407081700083));
#45966=CARTESIAN_POINT('Ctrl Pts',(-0.0412013170981547,-1.0684760419453,
2.7550046780852));
#45967=CARTESIAN_POINT('Ctrl Pts',(-0.065231815765751,-0.794772684000853,
2.89139801407353));
#45968=CARTESIAN_POINT('Ctrl Pts',(-0.0861519254167174,-0.636309800095197,
2.94731896886899));
#45969=CARTESIAN_POINT('Ctrl Pts',(-0.113985772631395,-0.319434907277158,
3.02104763479761));
#45970=CARTESIAN_POINT('Ctrl Pts',(-0.125109046164334,-0.158333333333332,
3.03895956505397));
#45971=CARTESIAN_POINT('Ctrl Pts',(-0.145969402090865,0.158333333333334,
3.0396453906214));
#45972=CARTESIAN_POINT('Ctrl Pts',(-0.154682023316671,0.319434907277167,
3.02254296395726));
#45973=CARTESIAN_POINT('Ctrl Pts',(-0.171425972763991,0.636309800095205,
2.94995935209706));
#45974=CARTESIAN_POINT('Ctrl Pts',(-0.172726418166373,0.794772684000839,
2.8941285969512));
#45975=CARTESIAN_POINT('Ctrl Pts',(-0.195368882082855,1.0684760419452,2.75892839454814));
#45976=CARTESIAN_POINT('Ctrl Pts',(-0.208249374524988,1.18514270861195,
2.68864308439401));
#45977=CARTESIAN_POINT('Ctrl Pts',(-0.224209275765781,1.30000000000026,
2.60659562204482));
#45978=CARTESIAN_POINT('Ctrl Pts',(-0.0213943747864332,-1.30000000000054,
2.6127724501415));
#45979=CARTESIAN_POINT('Ctrl Pts',(-0.0303808199747979,-1.18514270861215,
2.69825565188215));
#45980=CARTESIAN_POINT('Ctrl Pts',(-0.0397026858022174,-1.0684760419453,
2.77097185413313));
#45981=CARTESIAN_POINT('Ctrl Pts',(-0.0620129494732966,-0.794772684000851,
2.90946650530856));
#45982=CARTESIAN_POINT('Ctrl Pts',(-0.076590996619337,-0.636309800095197,
2.96367751455667));
#45983=CARTESIAN_POINT('Ctrl Pts',(-0.101057989717431,-0.319434907277159,
3.03661809166351));
#45984=CARTESIAN_POINT('Ctrl Pts',(-0.112567852729613,-0.158333333333332,
3.05351876196813));
#45985=CARTESIAN_POINT('Ctrl Pts',(-0.133278717910193,0.158333333333334,
3.05415093470282));
#45986=CARTESIAN_POINT('Ctrl Pts',(-0.141607349608986,0.319434907277167,
3.0379582636565));
#45987=CARTESIAN_POINT('Ctrl Pts',(-0.161103853485778,0.636309800095206,
2.96615092372332));
#45988=CARTESIAN_POINT('Ctrl Pts',(-0.167600922680341,0.79477268400084,
2.91217535482969));
#45989=CARTESIAN_POINT('Ctrl Pts',(-0.192015477656447,1.0684760419452,2.77486868997395));
#45990=CARTESIAN_POINT('Ctrl Pts',(-0.204772182759206,1.18514270861195,
2.70277064221539));
#45991=CARTESIAN_POINT('Ctrl Pts',(-0.219717436763986,1.30000000000025,
2.61800951420097));
#45992=CARTESIAN_POINT('Ctrl Pts',(-0.0165023515695407,-1.30000000000054,
2.61984802158576));
#45993=CARTESIAN_POINT('Ctrl Pts',(-0.0256069538907616,-1.18514270861215,
2.70510942351974));
#45994=CARTESIAN_POINT('Ctrl Pts',(-0.0347010954711869,-1.0684760419453,
2.77756665167126));
#45995=CARTESIAN_POINT('Ctrl Pts',(-0.0556862153948436,-0.794772684000851,
2.91537714081635));
#45996=CARTESIAN_POINT('Ctrl Pts',(-0.0677962068234773,-0.636309800095197,
2.9688868910723));
#45997=CARTESIAN_POINT('Ctrl Pts',(-0.090659738426676,-0.319434907277159,
3.04130452642146));
#45998=CARTESIAN_POINT('Ctrl Pts',(-0.102179986998412,-0.158333333333332,
3.05825650250268));
#45999=CARTESIAN_POINT('Ctrl Pts',(-0.122673368892049,0.158333333333334,
3.05879493020897));
#46000=CARTESIAN_POINT('Ctrl Pts',(-0.130506918224617,0.319434907277167,
3.04237334549098));
#46001=CARTESIAN_POINT('Ctrl Pts',(-0.151708180499798,0.636309800095206,
2.97106881806364));
#46002=CARTESIAN_POINT('Ctrl Pts',(-0.161724215836604,0.79477268400084,
2.91805939711538));
#46003=CARTESIAN_POINT('Ctrl Pts',(-0.187312562460002,1.0684760419452,2.78141067466404));
#46004=CARTESIAN_POINT('Ctrl Pts',(-0.199984062839926,1.18514270861195,
2.70950503030696));
#46005=CARTESIAN_POINT('Ctrl Pts',(-0.214250816488192,1.30000000000025,
2.62484391020782));
#46006=CARTESIAN_POINT('Ctrl Pts',(-0.0165023515695832,-1.3,2.61984802158616));
#46007=CARTESIAN_POINT('Ctrl Pts',(-0.0256069538907899,-1.18514270861178,
2.70510942351996));
#46008=CARTESIAN_POINT('Ctrl Pts',(-0.0347010954712011,-1.06847604194512,
2.77756665167135));
#46009=CARTESIAN_POINT('Ctrl Pts',(-0.0556862153948436,-0.794772684000851,
2.91537714081636));
#46010=CARTESIAN_POINT('Ctrl Pts',(-0.0677962068234773,-0.636309800095197,
2.9688868910723));
#46011=CARTESIAN_POINT('Ctrl Pts',(-0.0906597384266761,-0.319434907277159,
3.04130452642146));
#46012=CARTESIAN_POINT('Ctrl Pts',(-0.102179986998412,-0.158333333333332,
3.05825650250268));
#46013=CARTESIAN_POINT('Ctrl Pts',(-0.122673368892049,0.158333333333334,
3.05879493020897));
#46014=CARTESIAN_POINT('Ctrl Pts',(-0.130506918224617,0.319434907277167,
3.04237334549098));
#46015=CARTESIAN_POINT('Ctrl Pts',(-0.151708180499798,0.636309800095206,
2.97106881806364));
#46016=CARTESIAN_POINT('Ctrl Pts',(-0.161724215836604,0.79477268400084,
2.91805939711539));
#46017=CARTESIAN_POINT('Ctrl Pts',(-0.187312562459994,1.06847604194511,
2.78141067466408));
#46018=CARTESIAN_POINT('Ctrl Pts',(-0.199984062839908,1.18514270861178,
2.70950503030707));
#46019=CARTESIAN_POINT('Ctrl Pts',(-0.214250816488161,1.3,2.624843910208));
#46020=CARTESIAN_POINT('',(-0.213845469209945,-1.2,2.25462133752143));
#46021=CARTESIAN_POINT('Ctrl Pts',(-0.213845469209944,-1.2,2.25462133752143));
#46022=CARTESIAN_POINT('Ctrl Pts',(-0.204548853415621,-1.21101439883804,
2.2652440296684));
#46023=CARTESIAN_POINT('Ctrl Pts',(-0.194573317233004,-1.22173223319652,
2.27556637829925));
#46024=CARTESIAN_POINT('Ctrl Pts',(-0.176328391038453,-1.24278214089401,
2.29594391828212));
#46025=CARTESIAN_POINT('Ctrl Pts',(-0.167981216328268,-1.25266380271579,
2.30553832043326));
#46026=CARTESIAN_POINT('Ctrl Pts',(-0.146537790562717,-1.27799030514101,
2.33017925706331));
#46027=CARTESIAN_POINT('Ctrl Pts',(-0.143784999781138,-1.28105852037737,
2.33315876593495));
#46028=CARTESIAN_POINT('Ctrl Pts',(-0.128236474659343,-1.30000000000053,
2.35169561531438));
#46029=CARTESIAN_POINT('',(-0.370132009002969,-0.653834841418298,2.26385754909195));
#46030=CARTESIAN_POINT('Ctrl Pts',(-0.370132009002236,-0.653834841417621,
2.26385754906608));
#46031=CARTESIAN_POINT('Ctrl Pts',(-0.353920813038246,-0.717904873026858,
2.26264196775129));
#46032=CARTESIAN_POINT('Ctrl Pts',(-0.340646889995177,-0.76404242422158,
2.26170713554667));
#46033=CARTESIAN_POINT('Ctrl Pts',(-0.288948198313244,-0.949534604808305,
2.2583154474792));
#46034=CARTESIAN_POINT('Ctrl Pts',(-0.26137863609437,-1.04690484158362,
2.25667674178249));
#46035=CARTESIAN_POINT('Ctrl Pts',(-0.213845469209944,-1.2,2.25462133752143));
#46036=CARTESIAN_POINT('',(-0.509087305687289,0.653834841531101,2.27624836987201));
#46037=CARTESIAN_POINT('Ctrl Pts',(-0.509087305687289,0.6538348415311,2.27624836987201));
#46038=CARTESIAN_POINT('Ctrl Pts',(-0.487804298623256,0.576020454349171,
2.31193596787054));
#46039=CARTESIAN_POINT('Ctrl Pts',(-0.469211503005726,0.493680567759374,
2.34174637720171));
#46040=CARTESIAN_POINT('Ctrl Pts',(-0.440310963817089,0.338203591218837,
2.38330062796864));
#46041=CARTESIAN_POINT('Ctrl Pts',(-0.429076774576499,0.265718926343639,
2.39725207328199));
#46042=CARTESIAN_POINT('Ctrl Pts',(-0.410674103030229,0.129747729877892,
2.41328650637845));
#46043=CARTESIAN_POINT('Ctrl Pts',(-0.403176730549767,0.0666442716359389,
2.41680861876812));
#46044=CARTESIAN_POINT('Ctrl Pts',(-0.389859613444735,-0.0595545240722367,
2.41599461060225));
#46045=CARTESIAN_POINT('Ctrl Pts',(-0.383938144316827,-0.122803979681452,
2.41166924346832));
#46046=CARTESIAN_POINT('Ctrl Pts',(-0.373622084086818,-0.260161739957788,
2.39367060768024));
#46047=CARTESIAN_POINT('Ctrl Pts',(-0.369699318789559,-0.333963904502371,
2.37843693440692));
#46048=CARTESIAN_POINT('Ctrl Pts',(-0.365858759811961,-0.491156549484106,
2.33377361115453));
#46049=CARTESIAN_POINT('Ctrl Pts',(-0.366575240625937,-0.574264393662825,
2.30223676434492));
#46050=CARTESIAN_POINT('Ctrl Pts',(-0.370132008968997,-0.653834841429853,
2.26385754911276));
#46051=CARTESIAN_POINT('',(-0.437217345759296,1.2,2.26934679859076));
#46052=CARTESIAN_POINT('Ctrl Pts',(-0.437217345759296,1.2,2.26934679859076));
#46053=CARTESIAN_POINT('Ctrl Pts',(-0.451341357509953,1.12497957419401,
2.27059922148015));
#46054=CARTESIAN_POINT('Ctrl Pts',(-0.467276251271234,1.02797670902483,
2.27207424792545));
#46055=CARTESIAN_POINT('Ctrl Pts',(-0.497443621872752,0.796118559781083,
2.27504120190078));
#46056=CARTESIAN_POINT('Ctrl Pts',(-0.50257497511006,0.741382157389922,
2.27557503273473));
#46057=CARTESIAN_POINT('Ctrl Pts',(-0.50908730568729,0.653834841531101,
2.27624836987201));
#46058=CARTESIAN_POINT('Ctrl Pts',(-0.354392897366409,1.3,2.36296519815122));
#46059=CARTESIAN_POINT('Ctrl Pts',(-0.362135051021157,1.29069343462501,
2.35420092839924));
#46060=CARTESIAN_POINT('Ctrl Pts',(-0.367601211902519,1.28348293012651,
2.34732209545957));
#46061=CARTESIAN_POINT('Ctrl Pts',(-0.414027929604089,1.22697811672721,
2.29438949053698));
#46062=CARTESIAN_POINT('Ctrl Pts',(-0.426468674120977,1.21202615146349,
2.28046701772206));
#46063=CARTESIAN_POINT('Ctrl Pts',(-0.437217345759296,1.2,2.26934679859076));
#46064=CARTESIAN_POINT('Ctrl Pts',(-0.0165023515695832,-1.3,2.61984802158616));
#46065=CARTESIAN_POINT('Ctrl Pts',(-0.0256069538907899,-1.18514270861178,
2.70510942351996));
#46066=CARTESIAN_POINT('Ctrl Pts',(-0.0347010954712011,-1.06847604194512,
2.77756665167135));
#46067=CARTESIAN_POINT('Ctrl Pts',(-0.0556862153948436,-0.794772684000851,
2.91537714081635));
#46068=CARTESIAN_POINT('Ctrl Pts',(-0.0677962068234773,-0.636309800095196,
2.9688868910723));
#46069=CARTESIAN_POINT('Ctrl Pts',(-0.090659738426676,-0.319434907277159,
3.04130452642146));
#46070=CARTESIAN_POINT('Ctrl Pts',(-0.102179986998412,-0.158333333333332,
3.05825650250268));
#46071=CARTESIAN_POINT('Ctrl Pts',(-0.122673368892049,0.158333333333334,
3.05879493020897));
#46072=CARTESIAN_POINT('Ctrl Pts',(-0.130506918224617,0.319434907277167,
3.04237334549098));
#46073=CARTESIAN_POINT('Ctrl Pts',(-0.151708180499798,0.636309800095206,
2.97106881806364));
#46074=CARTESIAN_POINT('Ctrl Pts',(-0.161724215836604,0.79477268400084,
2.91805939711539));
#46075=CARTESIAN_POINT('Ctrl Pts',(-0.187312562459994,1.06847604194511,
2.78141067466408));
#46076=CARTESIAN_POINT('Ctrl Pts',(-0.199984062839908,1.18514270861178,
2.70950503030707));
#46077=CARTESIAN_POINT('Ctrl Pts',(-0.214250816488161,1.3,2.624843910208));
#46078=CARTESIAN_POINT('Ctrl Pts',(0.0604153711163316,-1.3,2.62151331779344));
#46079=CARTESIAN_POINT('Ctrl Pts',(0.0495900516861096,-1.18514270861178,
2.70657462578233));
#46080=CARTESIAN_POINT('Ctrl Pts',(0.039303457172531,-1.06847604194512,
2.77884799266893));
#46081=CARTESIAN_POINT('Ctrl Pts',(0.0167839283489731,-0.794772684000851,
2.91627122624936));
#46082=CARTESIAN_POINT('Ctrl Pts',(0.00537192228428135,-0.636309800095196,
2.96961420006941));
#46083=CARTESIAN_POINT('Ctrl Pts',(-0.0169375195429115,-0.319434907277159,
3.04166079944464));
#46084=CARTESIAN_POINT('Ctrl Pts',(-0.0272288683682577,-0.158333333333332,
3.05843597840478));
#46085=CARTESIAN_POINT('Ctrl Pts',(-0.0477222502618953,0.158333333333334,
3.05861545430687));
#46086=CARTESIAN_POINT('Ctrl Pts',(-0.0567846993408529,0.319434907277167,
3.04201707246781));
#46087=CARTESIAN_POINT('Ctrl Pts',(-0.0785400513920393,0.636309800095206,
2.97034150906653));
#46088=CARTESIAN_POINT('Ctrl Pts',(-0.0892540720927878,0.79477268400084,
2.91716531168238));
#46089=CARTESIAN_POINT('Ctrl Pts',(-0.113308009816262,1.06847604194511,
2.78012933366651));
#46090=CARTESIAN_POINT('Ctrl Pts',(-0.124787057263008,1.18514270861178,
2.7080398280447));
#46091=CARTESIAN_POINT('Ctrl Pts',(-0.137333093802246,1.3,2.62317861400072));
#46092=CARTESIAN_POINT('Ctrl Pts',(0.137333093802246,-1.3,2.62317861400072));
#46093=CARTESIAN_POINT('Ctrl Pts',(0.124787057263009,-1.18514270861178,
2.7080398280447));
#46094=CARTESIAN_POINT('Ctrl Pts',(0.113308009816263,-1.06847604194512,
2.7801293336665));
#46095=CARTESIAN_POINT('Ctrl Pts',(0.0892540720927901,-0.794772684000851,
2.91716531168237));
#46096=CARTESIAN_POINT('Ctrl Pts',(0.0785400513920396,-0.636309800095196,
2.97034150906653));
#46097=CARTESIAN_POINT('Ctrl Pts',(0.0567846993408532,-0.319434907277159,
3.04201707246781));
#46098=CARTESIAN_POINT('Ctrl Pts',(0.0477222502618961,-0.158333333333332,
3.05861545430687));
#46099=CARTESIAN_POINT('Ctrl Pts',(0.0272288683682586,0.158333333333334,
3.05843597840478));
#46100=CARTESIAN_POINT('Ctrl Pts',(0.0169375195429118,0.319434907277167,
3.04166079944463));
#46101=CARTESIAN_POINT('Ctrl Pts',(-0.00537192228428079,0.636309800095206,
2.96961420006942));
#46102=CARTESIAN_POINT('Ctrl Pts',(-0.016783928348971,0.79477268400084,
2.91627122624937));
#46103=CARTESIAN_POINT('Ctrl Pts',(-0.0393034571725295,1.06847604194511,
2.77884799266893));
#46104=CARTESIAN_POINT('Ctrl Pts',(-0.0495900516861082,1.18514270861178,
2.70657462578233));
#46105=CARTESIAN_POINT('Ctrl Pts',(-0.0604153711163307,1.3,2.62151331779344));
#46106=CARTESIAN_POINT('Ctrl Pts',(0.214250816488161,-1.3,2.62484391020801));
#46107=CARTESIAN_POINT('Ctrl Pts',(0.199984062839909,-1.18514270861178,
2.70950503030707));
#46108=CARTESIAN_POINT('Ctrl Pts',(0.187312562459995,-1.06847604194512,
2.78141067466408));
#46109=CARTESIAN_POINT('Ctrl Pts',(0.161724215836607,-0.794772684000851,
2.91805939711538));
#46110=CARTESIAN_POINT('Ctrl Pts',(0.151708180499798,-0.636309800095196,
2.97106881806364));
#46111=CARTESIAN_POINT('Ctrl Pts',(0.130506918224618,-0.319434907277159,
3.04237334549099));
#46112=CARTESIAN_POINT('Ctrl Pts',(0.12267336889205,-0.158333333333332,
3.05879493020897));
#46113=CARTESIAN_POINT('Ctrl Pts',(0.102179986998412,0.158333333333334,
3.05825650250268));
#46114=CARTESIAN_POINT('Ctrl Pts',(0.0906597384266764,0.319434907277167,
3.04130452642146));
#46115=CARTESIAN_POINT('Ctrl Pts',(0.0677962068234778,0.636309800095206,
2.9688868910723));
#46116=CARTESIAN_POINT('Ctrl Pts',(0.0556862153948456,0.79477268400084,
2.91537714081636));
#46117=CARTESIAN_POINT('Ctrl Pts',(0.0347010954712027,1.06847604194511,
2.77756665167135));
#46118=CARTESIAN_POINT('Ctrl Pts',(0.0256069538907915,1.18514270861178,
2.70510942351996));
#46119=CARTESIAN_POINT('Ctrl Pts',(0.0165023515695843,1.3,2.61984802158616));
#46120=CARTESIAN_POINT('Ctrl Pts',(0.214250816488161,-1.3,2.62484391020801));
#46121=CARTESIAN_POINT('Ctrl Pts',(0.199984062839909,-1.18514270861178,
2.70950503030707));
#46122=CARTESIAN_POINT('Ctrl Pts',(0.187312562459995,-1.06847604194512,
2.78141067466408));
#46123=CARTESIAN_POINT('Ctrl Pts',(0.161724215836607,-0.794772684000851,
2.91805939711538));
#46124=CARTESIAN_POINT('Ctrl Pts',(0.151708180499798,-0.636309800095197,
2.97106881806364));
#46125=CARTESIAN_POINT('Ctrl Pts',(0.130506918224618,-0.319434907277159,
3.04237334549099));
#46126=CARTESIAN_POINT('Ctrl Pts',(0.12267336889205,-0.158333333333332,
3.05879493020897));
#46127=CARTESIAN_POINT('Ctrl Pts',(0.102179986998412,0.158333333333334,
3.05825650250268));
#46128=CARTESIAN_POINT('Ctrl Pts',(0.0906597384266764,0.319434907277167,
3.04130452642146));
#46129=CARTESIAN_POINT('Ctrl Pts',(0.0677962068234777,0.636309800095206,
2.9688868910723));
#46130=CARTESIAN_POINT('Ctrl Pts',(0.0556862153948455,0.79477268400084,
2.91537714081636));
#46131=CARTESIAN_POINT('Ctrl Pts',(0.0347010954712026,1.06847604194511,
2.77756665167135));
#46132=CARTESIAN_POINT('Ctrl Pts',(0.0256069538907915,1.18514270861178,
2.70510942351996));
#46133=CARTESIAN_POINT('Ctrl Pts',(0.0165023515695843,1.3,2.61984802158616));
#46134=CARTESIAN_POINT('Ctrl Pts',(0.214250816488492,-1.30000000000266,
2.62484391020604));
#46135=CARTESIAN_POINT('Ctrl Pts',(0.199984062840105,-1.18514270861359,
2.70950503030596));
#46136=CARTESIAN_POINT('Ctrl Pts',(0.18731256246008,-1.06847604194603,2.78141067466363));
#46137=CARTESIAN_POINT('Ctrl Pts',(0.161724215836607,-0.794772684000851,
2.91805939711538));
#46138=CARTESIAN_POINT('Ctrl Pts',(0.151708180499798,-0.636309800095197,
2.97106881806364));
#46139=CARTESIAN_POINT('Ctrl Pts',(0.130506918224618,-0.319434907277159,
3.04237334549099));
#46140=CARTESIAN_POINT('Ctrl Pts',(0.12267336889205,-0.158333333333332,
3.05879493020897));
#46141=CARTESIAN_POINT('Ctrl Pts',(0.102179986998412,0.158333333333334,
3.05825650250268));
#46142=CARTESIAN_POINT('Ctrl Pts',(0.0906597384266765,0.319434907277167,
3.04130452642146));
#46143=CARTESIAN_POINT('Ctrl Pts',(0.0677962068234777,0.636309800095206,
2.9688868910723));
#46144=CARTESIAN_POINT('Ctrl Pts',(0.0556862153948455,0.79477268400084,
2.91537714081636));
#46145=CARTESIAN_POINT('Ctrl Pts',(0.0347010954711178,1.06847604194622,
2.7775666516708));
#46146=CARTESIAN_POINT('Ctrl Pts',(0.0256069538906217,1.18514270861395,
2.70510942351861));
#46147=CARTESIAN_POINT('Ctrl Pts',(0.0165023515693293,1.30000000000322,
2.61984802158377));
#46148=CARTESIAN_POINT('Ctrl Pts',(0.219717436762999,-1.30000000000266,
2.61800951425875));
#46149=CARTESIAN_POINT('Ctrl Pts',(0.204772182758639,-1.18514270861359,
2.70277064226634));
#46150=CARTESIAN_POINT('Ctrl Pts',(0.19201547765618,-1.06847604194603,2.7748686900201));
#46151=CARTESIAN_POINT('Ctrl Pts',(0.167600922680589,-0.794772684000851,
2.91217535486884));
#46152=CARTESIAN_POINT('Ctrl Pts',(0.1611038534861,-0.636309800095197,2.96615092375314));
#46153=CARTESIAN_POINT('Ctrl Pts',(0.141607349608946,-0.319434907277159,
3.0379582637104));
#46154=CARTESIAN_POINT('Ctrl Pts',(0.133278717909188,-0.158333333333332,
3.05415093481762));
#46155=CARTESIAN_POINT('Ctrl Pts',(0.112567852728384,0.158333333333334,
3.05351876207922));
#46156=CARTESIAN_POINT('Ctrl Pts',(0.10105798971678,0.319434907277167,3.03661809170896));
#46157=CARTESIAN_POINT('Ctrl Pts',(0.0765909966189229,0.636309800095206,
2.96367751457251));
#46158=CARTESIAN_POINT('Ctrl Pts',(0.0620129494727478,0.79477268400084,
2.90946650533395));
#46159=CARTESIAN_POINT('Ctrl Pts',(0.0397026858018158,1.06847604194622,
2.77097185416088));
#46160=CARTESIAN_POINT('Ctrl Pts',(0.0303808199744749,1.18514270861395,
2.69825565191217));
#46161=CARTESIAN_POINT('Ctrl Pts',(0.0213943747862455,1.30000000000322,
2.61277245017529));
#46162=CARTESIAN_POINT('Ctrl Pts',(0.224226242429926,-1.30000000000266,
2.60660085909856));
#46163=CARTESIAN_POINT('Ctrl Pts',(0.208257853828071,-1.18514270861359,
2.68864946051841));
#46164=CARTESIAN_POINT('Ctrl Pts',(0.195371213482085,-1.06847604194603,
2.7589356667499));
#46165=CARTESIAN_POINT('Ctrl Pts',(0.172719951292067,-0.794772684000849,
2.89413737790722));
#46166=CARTESIAN_POINT('Ctrl Pts',(0.171421999099358,-0.636309800095195,
2.94996853204855));
#46167=CARTESIAN_POINT('Ctrl Pts',(0.154677214871352,-0.319434907277157,
3.0225522636603));
#46168=CARTESIAN_POINT('Ctrl Pts',(0.145966428273531,-0.158333333333332,
3.03965369608755));
#46169=CARTESIAN_POINT('Ctrl Pts',(0.125103826804356,0.158333333333334,
3.03896798715647));
#46170=CARTESIAN_POINT('Ctrl Pts',(0.113974062136087,0.319434907277168,
3.02105717623826));
#46171=CARTESIAN_POINT('Ctrl Pts',(0.0861413866549122,0.636309800095206,
2.94732861089557));
#46172=CARTESIAN_POINT('Ctrl Pts',(0.0652329202269298,0.794772684000838,
2.89140877704261));
#46173=CARTESIAN_POINT('Ctrl Pts',(0.0412006114249792,1.06847604194621,
2.75501159968778));
#46174=CARTESIAN_POINT('Ctrl Pts',(0.0323159863042974,1.18514270861395,
2.68407500213889));
#46175=CARTESIAN_POINT('Ctrl Pts',(0.0249494320585472,1.30000000000321,
2.60124309110478));
#46176=CARTESIAN_POINT('Ctrl Pts',(0.230949458773703,-1.30000000000266,
2.58988253450759));
#46177=CARTESIAN_POINT('Ctrl Pts',(0.215310207632889,-1.18514270861359,
2.6682714894817));
#46178=CARTESIAN_POINT('Ctrl Pts',(0.202874571394742,-1.06847604194603,
2.73588386953428));
#46179=CARTESIAN_POINT('Ctrl Pts',(0.181546755250328,-0.79477268400085,
2.86718594935033));
#46180=CARTESIAN_POINT('Ctrl Pts',(0.181706589644006,-0.636309800095197,
2.92368822085034));
#46181=CARTESIAN_POINT('Ctrl Pts',(0.166279833913429,-0.319434907277159,
2.99623753732807));
#46182=CARTESIAN_POINT('Ctrl Pts',(0.158104188468809,-0.158333333333332,
3.01469934874809));
#46183=CARTESIAN_POINT('Ctrl Pts',(0.137147922657862,0.158333333333334,
3.0140255997615));
#46184=CARTESIAN_POINT('Ctrl Pts',(0.12572094355746,0.319434907277166,2.99481719140083));
#46185=CARTESIAN_POINT('Ctrl Pts',(0.0957040249390647,0.636309800095205,
2.92104388278613));
#46186=CARTESIAN_POINT('Ctrl Pts',(0.0714764819578855,0.79477268400084,
2.86424787169668));
#46187=CARTESIAN_POINT('Ctrl Pts',(0.0459616329290023,1.06847604194622,
2.73168073618549));
#46188=CARTESIAN_POINT('Ctrl Pts',(0.036969146524305,1.18514270861395,2.66342015805726));
#46189=CARTESIAN_POINT('Ctrl Pts',(0.0300286064412367,1.30000000000322,
2.5842824026674));
#46190=CARTESIAN_POINT('Ctrl Pts',(0.236845399224923,-1.30000000000266,
2.57610161912796));
#46191=CARTESIAN_POINT('Ctrl Pts',(0.221834012227604,-1.18514270861359,
2.65181796325388));
#46192=CARTESIAN_POINT('Ctrl Pts',(0.20970644697097,-1.06847604194603,2.71746793573469));
#46193=CARTESIAN_POINT('Ctrl Pts',(0.188351550244662,-0.794772684000849,
2.84587717312589));
#46194=CARTESIAN_POINT('Ctrl Pts',(0.186768855990391,-0.636309800095196,
2.90275724229796));
#46195=CARTESIAN_POINT('Ctrl Pts',(0.171469624012701,-0.319434907277159,
2.97530338117715));
#46196=CARTESIAN_POINT('Ctrl Pts',(0.164888391661675,-0.158333333333332,
2.99489344943572));
#46197=CARTESIAN_POINT('Ctrl Pts',(0.144505048078426,0.158333333333334,
2.99429991964275));
#46198=CARTESIAN_POINT('Ctrl Pts',(0.132951781539408,0.319434907277167,
2.97414934804337));
#46199=CARTESIAN_POINT('Ctrl Pts',(0.102150875569596,0.636309800095206,
2.90032695920638));
#46200=CARTESIAN_POINT('Ctrl Pts',(0.0764112209685388,0.79477268400084,
2.84281492452855));
#46201=CARTESIAN_POINT('Ctrl Pts',(0.0503921073465047,1.06847604194621,
2.71304101877748));
#46202=CARTESIAN_POINT('Ctrl Pts',(0.0414413960540642,1.18514270861395,
2.64674863185993));
#46203=CARTESIAN_POINT('Ctrl Pts',(0.0348026836530411,1.30000000000322,
2.57033817322763));
#46204=CARTESIAN_POINT('Ctrl Pts',(0.242960861231862,-1.30000000000267,
2.56222898063554));
#46205=CARTESIAN_POINT('Ctrl Pts',(0.2286894017545,-1.18514270861359,2.63502014154845));
#46206=CARTESIAN_POINT('Ctrl Pts',(0.216927525128715,-1.06847604194603,
2.6985053181899));
#46207=CARTESIAN_POINT('Ctrl Pts',(0.195552875595353,-0.79477268400085,
2.82367009107433));
#46208=CARTESIAN_POINT('Ctrl Pts',(0.192243349954664,-0.636309800095197,
2.88086591715262));
#46209=CARTESIAN_POINT('Ctrl Pts',(0.17650634197705,-0.31943490727716,2.95325496211296));
#46210=CARTESIAN_POINT('Ctrl Pts',(0.17113522051647,-0.158333333333332,
2.9739908358149));
#46211=CARTESIAN_POINT('Ctrl Pts',(0.149875803896344,0.158333333333334,
2.97333502370939));
#46212=CARTESIAN_POINT('Ctrl Pts',(0.135702605371645,0.319434907277167,
2.95194658007296));
#46213=CARTESIAN_POINT('Ctrl Pts',(0.104642184068728,0.636309800095206,
2.87821508900477));
#46214=CARTESIAN_POINT('Ctrl Pts',(0.0813510654142378,0.794772684000842,
2.82041706127865));
#46215=CARTESIAN_POINT('Ctrl Pts',(0.0558631364763465,1.06847604194622,
2.69388570487083));
#46216=CARTESIAN_POINT('Ctrl Pts',(0.0468095477267672,1.18514270861395,
2.62975762692213));
#46217=CARTESIAN_POINT('Ctrl Pts',(0.0397351502440323,1.30000000000322,
2.55627220676513));
#46218=CARTESIAN_POINT('Ctrl Pts',(0.250471543072162,-1.30000000000267,
2.54870591804654));
#46219=CARTESIAN_POINT('Ctrl Pts',(0.236868078466005,-1.18514270861359,
2.61871399047799));
#46220=CARTESIAN_POINT('Ctrl Pts',(0.225336052648485,-1.06847604194603,
2.68012857764004));
#46221=CARTESIAN_POINT('Ctrl Pts',(0.203480204027908,-0.79477268400085,
2.80215588983677));
#46222=CARTESIAN_POINT('Ctrl Pts',(0.1982073532554,-0.636309800095196,2.85960963436872));
#46223=CARTESIAN_POINT('Ctrl Pts',(0.180822474756462,-0.319434907277159,
2.93170916824689));
#46224=CARTESIAN_POINT('Ctrl Pts',(0.174664464262972,-0.158333333333332,
2.95331583529123));
#46225=CARTESIAN_POINT('Ctrl Pts',(0.152781665023936,0.158333333333334,
2.95263166308528));
#46226=CARTESIAN_POINT('Ctrl Pts',(0.138586582843348,0.319434907277166,
2.93036861580522));
#46227=CARTESIAN_POINT('Ctrl Pts',(0.108281872775913,0.636309800095205,
2.85681886216328));
#46228=CARTESIAN_POINT('Ctrl Pts',(0.0868071607438343,0.79477268400084,
2.79864821362611));
#46229=CARTESIAN_POINT('Ctrl Pts',(0.0615122998097732,1.06847604194621,
2.67512345987812));
#46230=CARTESIAN_POINT('Ctrl Pts',(0.0521573957606204,1.18514270861395,
2.61301343223756));
#46231=CARTESIAN_POINT('Ctrl Pts',(0.0443967956937546,1.30000000000321,
2.542262665811));
#46232=CARTESIAN_POINT('Ctrl Pts',(0.260324786692414,-1.30000000000267,
2.52661415542551));
#46233=CARTESIAN_POINT('Ctrl Pts',(0.247738100352481,-1.18514270861359,
2.59205864113441));
#46234=CARTESIAN_POINT('Ctrl Pts',(0.236730363824326,-1.06847604194603,
2.65010915080776));
#46235=CARTESIAN_POINT('Ctrl Pts',(0.214947980287267,-0.794772684000848,
2.76713587731543));
#46236=CARTESIAN_POINT('Ctrl Pts',(0.208042015085297,-0.636309800095196,
2.82525416350595));
#46237=CARTESIAN_POINT('Ctrl Pts',(0.189046709496585,-0.319434907277159,
2.89704085517984));
#46238=CARTESIAN_POINT('Ctrl Pts',(0.181568024952914,-0.158333333333332,
2.9200833086852));
#46239=CARTESIAN_POINT('Ctrl Pts',(0.159074504936224,0.158333333333334,
2.91935988914436));
#46240=CARTESIAN_POINT('Ctrl Pts',(0.145313591975273,0.319434907277168,
2.89560943657395));
#46241=CARTESIAN_POINT('Ctrl Pts',(0.115937067005509,0.636309800095207,
2.82231778098446));
#46242=CARTESIAN_POINT('Ctrl Pts',(0.0960962109841885,0.79477268400084,
2.76348818055815));
#46243=CARTESIAN_POINT('Ctrl Pts',(0.0710703651477984,1.06847604194621,
2.6449262435517));
#46244=CARTESIAN_POINT('Ctrl Pts',(0.0614821466118171,1.18514270861395,
2.5861599519411));
#46245=CARTESIAN_POINT('Ctrl Pts',(0.0531384709035037,1.30000000000322,
2.51994843809752));
#46246=CARTESIAN_POINT('Ctrl Pts',(0.276326377533243,-1.30000000000266,
2.49679480815817));
#46247=CARTESIAN_POINT('Ctrl Pts',(0.266773624550892,-1.18514270861358,
2.55639301755284));
#46248=CARTESIAN_POINT('Ctrl Pts',(0.257408085958808,-1.06847604194603,
2.61006830635916));
#46249=CARTESIAN_POINT('Ctrl Pts',(0.236204320935233,-0.79477268400085,
2.72038582977072));
#46250=CARTESIAN_POINT('Ctrl Pts',(0.224618722165695,-0.636309800095196,
2.77885015273103));
#46251=CARTESIAN_POINT('Ctrl Pts',(0.202026006127601,-0.319434907277159,
2.84988966203324));
#46252=CARTESIAN_POINT('Ctrl Pts',(0.192312128337127,-0.158333333333332,
2.87476074147654));
#46253=CARTESIAN_POINT('Ctrl Pts',(0.168505927894078,0.158333333333334,
2.87393181360536));
#46254=CARTESIAN_POINT('Ctrl Pts',(0.155246296971355,0.319434907277164,
2.84828171591575));
#46255=CARTESIAN_POINT('Ctrl Pts',(0.12765136371236,0.636309800095203,2.77545207791248));
#46256=CARTESIAN_POINT('Ctrl Pts',(0.111705856094525,0.79477268400084,2.715907240678));
#46257=CARTESIAN_POINT('Ctrl Pts',(0.0866203030801193,1.06847604194621,
2.60399740450606));
#46258=CARTESIAN_POINT('Ctrl Pts',(0.0760605815387644,1.18514270861395,
2.54966891900018));
#46259=CARTESIAN_POINT('Ctrl Pts',(0.0657997448446978,1.30000000000321,
2.48945356939939));
#46260=CARTESIAN_POINT('Ctrl Pts',(0.292202396494802,-1.30000000000266,
2.46694851625233));
#46261=CARTESIAN_POINT('Ctrl Pts',(0.283999061631066,-1.18514270861358,
2.52029688424042));
#46262=CARTESIAN_POINT('Ctrl Pts',(0.275487483908816,-1.06847604194603,
2.56938158427808));
#46263=CARTESIAN_POINT('Ctrl Pts',(0.255111933968273,-0.79477268400085,
2.6729271348159));
#46264=CARTESIAN_POINT('Ctrl Pts',(0.242813019657568,-0.636309800095196,
2.73248470123121));
#46265=CARTESIAN_POINT('Ctrl Pts',(0.218454706196389,-0.319434907277158,
2.8030732316513));
#46266=CARTESIAN_POINT('Ctrl Pts',(0.206026250815626,-0.158333333333332,
2.82968936167192));
#46267=CARTESIAN_POINT('Ctrl Pts',(0.181291452230541,0.158333333333334,
2.82874104483902));
#46268=CARTESIAN_POINT('Ctrl Pts',(0.169446802573742,0.319434907277166,
2.80118316000646));
#46269=CARTESIAN_POINT('Ctrl Pts',(0.142481675768436,0.636309800095204,
2.72864961011461));
#46270=CARTESIAN_POINT('Ctrl Pts',(0.127566010709557,0.794772684000839,
2.66809682197219));
#46271=CARTESIAN_POINT('Ctrl Pts',(0.101165243211556,1.06847604194621,2.56277705064535));
#46272=CARTESIAN_POINT('Ctrl Pts',(0.0894843035980192,1.18514270861395,
2.5129190957758));
#46273=CARTESIAN_POINT('Ctrl Pts',(0.07755033837604,1.30000000000322,2.45879221256219));
#46274=CARTESIAN_POINT('Ctrl Pts',(0.304272576971275,-1.30000000000266,
2.44537989334799));
#46275=CARTESIAN_POINT('Ctrl Pts',(0.298784633296944,-1.18514270861358,
2.49456792282061));
#46276=CARTESIAN_POINT('Ctrl Pts',(0.291942104826949,-1.06847604194603,
2.54054519967646));
#46277=CARTESIAN_POINT('Ctrl Pts',(0.273005133356464,-0.794772684000849,
2.63934442608221));
#46278=CARTESIAN_POINT('Ctrl Pts',(0.257978411602134,-0.636309800095195,
2.69920763652856));
#46279=CARTESIAN_POINT('Ctrl Pts',(0.231598787365596,-0.319434907277158,
2.76927187817773));
#46280=CARTESIAN_POINT('Ctrl Pts',(0.217472370399731,-0.158333333333332,
2.79715497595911));
#46281=CARTESIAN_POINT('Ctrl Pts',(0.191892554756733,0.158333333333334,
2.79608873751453));
#46282=CARTESIAN_POINT('Ctrl Pts',(0.180681897540819,0.319434907277165,
2.76714927918927));
#46283=CARTESIAN_POINT('Ctrl Pts',(0.154462832241876,0.636309800095203,
2.69489306602771));
#46284=CARTESIAN_POINT('Ctrl Pts',(0.141318825871087,0.794772684000838,
2.63374630787981));
#46285=CARTESIAN_POINT('Ctrl Pts',(0.114121379298996,1.06847604194621,2.53321905935691));
#46286=CARTESIAN_POINT('Ctrl Pts',(0.101502347942526,1.18514270861395,2.48657909896014));
#46287=CARTESIAN_POINT('Ctrl Pts',(0.0880370520859876,1.30000000000321,
2.43681369915072));
#46288=CARTESIAN_POINT('Ctrl Pts',(0.31391933706681,-1.30000000000266,2.4293389678366));
#46289=CARTESIAN_POINT('Ctrl Pts',(0.309400934569747,-1.18514270861358,
2.4751753199178));
#46290=CARTESIAN_POINT('Ctrl Pts',(0.303131998752341,-1.06847604194602,
2.5186753955374));
#46291=CARTESIAN_POINT('Ctrl Pts',(0.28460542075491,-0.794772684000844,
2.61377200638179));
#46292=CARTESIAN_POINT('Ctrl Pts',(0.268426823455187,-0.636309800095196,
2.67406955453933));
#46293=CARTESIAN_POINT('Ctrl Pts',(0.241218797163057,-0.31943490727716,
2.74387709408424));
#46294=CARTESIAN_POINT('Ctrl Pts',(0.226503729694203,-0.158333333333332,
2.77283473837323));
#46295=CARTESIAN_POINT('Ctrl Pts',(0.200615266855469,0.158333333333334,
2.77172723585368));
#46296=CARTESIAN_POINT('Ctrl Pts',(0.189810095540242,0.319434907277164,
2.74170569891167));
#46297=CARTESIAN_POINT('Ctrl Pts',(0.163535141174737,0.636309800095204,
2.66955342631916));
#46298=CARTESIAN_POINT('Ctrl Pts',(0.15047246735778,0.79477268400084,2.60778317810354));
#46299=CARTESIAN_POINT('Ctrl Pts',(0.122451069898524,1.06847604194622,2.51082597321505));
#46300=CARTESIAN_POINT('Ctrl Pts',(0.109283634712029,1.18514270861396,2.46662845922663));
#46301=CARTESIAN_POINT('Ctrl Pts',(0.0950781890041065,1.30000000000322,
2.42020261262772));
#46302=CARTESIAN_POINT('Ctrl Pts',(0.329357357760276,-1.30000000000267,
2.40248830162943));
#46303=CARTESIAN_POINT('Ctrl Pts',(0.327729674566757,-1.18514270861359,
2.4430275075526));
#46304=CARTESIAN_POINT('Ctrl Pts',(0.323315370461579,-1.06847604194603,
2.48259745426958));
#46305=CARTESIAN_POINT('Ctrl Pts',(0.306679793132641,-0.794772684000852,
2.57177276446023));
#46306=CARTESIAN_POINT('Ctrl Pts',(0.28829840342903,-0.636309800095199,
2.63268060877138));
#46307=CARTESIAN_POINT('Ctrl Pts',(0.259149536142379,-0.319434907277161,
2.70192493970066));
#46308=CARTESIAN_POINT('Ctrl Pts',(0.242095782310558,-0.158333333333333,
2.7324073631622));
#46309=CARTESIAN_POINT('Ctrl Pts',(0.215500324796916,0.158333333333335,
2.73118901208806));
#46310=CARTESIAN_POINT('Ctrl Pts',(0.206124614958519,0.319434907277165,
2.69952637433431));
#46311=CARTESIAN_POINT('Ctrl Pts',(0.180762332719264,0.636309800095206,
2.62772266811228));
#46312=CARTESIAN_POINT('Ctrl Pts',(0.169392553392926,0.794772684000845,
2.56516167402763));
#46313=CARTESIAN_POINT('Ctrl Pts',(0.139683659528629,1.06847604194622,2.47408974758264));
#46314=CARTESIAN_POINT('Ctrl Pts',(0.124995150673325,1.18514270861396,2.43385509284417));
#46315=CARTESIAN_POINT('Ctrl Pts',(0.108478012293625,1.30000000000322,2.39280744577801));
#46316=CARTESIAN_POINT('Ctrl Pts',(0.349313927641765,-1.30000000000266,
2.37063062041402));
#46317=CARTESIAN_POINT('Ctrl Pts',(0.350990972581243,-1.18514270861358,
2.40479535651899));
#46318=CARTESIAN_POINT('Ctrl Pts',(0.348696152747529,-1.06847604194603,
2.43963560104537));
#46319=CARTESIAN_POINT('Ctrl Pts',(0.334218857659674,-0.794772684000849,
2.52168409525648));
#46320=CARTESIAN_POINT('Ctrl Pts',(0.313241814432491,-0.636309800095198,
2.58331600960798));
#46321=CARTESIAN_POINT('Ctrl Pts',(0.28201046580892,-0.319434907277161,
2.65189738093111));
#46322=CARTESIAN_POINT('Ctrl Pts',(0.26266427967697,-0.158333333333332,
2.68426798688803));
#46323=CARTESIAN_POINT('Ctrl Pts',(0.235171728445277,0.158333333333334,
2.68288728323856));
#46324=CARTESIAN_POINT('Ctrl Pts',(0.227136327014149,0.319434907277165,
2.64919350404502));
#46325=CARTESIAN_POINT('Ctrl Pts',(0.20214130330482,0.636309800095205,2.57768255349322));
#46326=CARTESIAN_POINT('Ctrl Pts',(0.192061826528855,0.794772684000843,
2.5140529536976));
#46327=CARTESIAN_POINT('Ctrl Pts',(0.159730108434817,1.06847604194622,2.42994044625363));
#46328=CARTESIAN_POINT('Ctrl Pts',(0.143041737765,1.18514270861396,2.39442966052077));
#46329=CARTESIAN_POINT('Ctrl Pts',(0.123660199180121,1.30000000000322,2.35981727685218));
#46330=CARTESIAN_POINT('Ctrl Pts',(0.372656470855065,-1.30000000000266,
2.33357102415659));
#46331=CARTESIAN_POINT('Ctrl Pts',(0.378860083512457,-1.18514270861359,
2.36049270100928));
#46332=CARTESIAN_POINT('Ctrl Pts',(0.379623704547688,-1.06847604194603,
2.38996946461138));
#46333=CARTESIAN_POINT('Ctrl Pts',(0.368820352987192,-0.794772684000852,
2.46396944687276));
#46334=CARTESIAN_POINT('Ctrl Pts',(0.345641686475895,-0.636309800095197,
2.52656684485733));
#46335=CARTESIAN_POINT('Ctrl Pts',(0.312069213115202,-0.319434907277159,
2.59433277240725));
#46336=CARTESIAN_POINT('Ctrl Pts',(0.289014967455505,-0.158333333333332,
2.62862603375246));
#46337=CARTESIAN_POINT('Ctrl Pts',(0.260127011611611,0.158333333333334,
2.6269490852742));
#46338=CARTESIAN_POINT('Ctrl Pts',(0.25389123708121,0.319434907277168,2.59095897495413));
#46339=CARTESIAN_POINT('Ctrl Pts',(0.229440000513363,0.636309800095207,
2.51981775997691));
#46340=CARTESIAN_POINT('Ctrl Pts',(0.221050650127639,0.794772684000841,
2.45499750537546));
#46341=CARTESIAN_POINT('Ctrl Pts',(0.185638193159351,1.06847604194621,2.37897079950157));
#46342=CARTESIAN_POINT('Ctrl Pts',(0.166555801923257,1.18514270861395,2.3489356310057));
#46343=CARTESIAN_POINT('Ctrl Pts',(0.143719759911867,1.30000000000321,2.32177443791985));
#46344=CARTESIAN_POINT('Ctrl Pts',(0.39394052481098,-1.30000000000266,2.30216095517147));
#46345=CARTESIAN_POINT('Ctrl Pts',(0.404452058674696,-1.18514270861358,
2.3230082546088));
#46346=CARTESIAN_POINT('Ctrl Pts',(0.408035072497374,-1.06847604194603,
2.3479548710559));
#46347=CARTESIAN_POINT('Ctrl Pts',(0.400306283866768,-0.79477268400085,
2.41505678796012));
#46348=CARTESIAN_POINT('Ctrl Pts',(0.373759972065985,-0.636309800095195,
2.47811072112627));
#46349=CARTESIAN_POINT('Ctrl Pts',(0.338594991347445,-0.319434907277158,
2.54523185207478));
#46350=CARTESIAN_POINT('Ctrl Pts',(0.314328019102381,-0.158333333333332,
2.58157499811901));
#46351=CARTESIAN_POINT('Ctrl Pts',(0.284743021097901,0.158333333333334,
2.57973868058722));
#46352=CARTESIAN_POINT('Ctrl Pts',(0.279090057296803,0.319434907277166,
2.54158652617387));
#46353=CARTESIAN_POINT('Ctrl Pts',(0.254674771945333,0.636309800095204,
2.47066932183429));
#46354=CARTESIAN_POINT('Ctrl Pts',(0.247976474935861,0.794772684000839,
2.4048763179591));
#46355=CARTESIAN_POINT('Ctrl Pts',(0.209269561084131,1.06847604194621,2.33563397887084));
#46356=CARTESIAN_POINT('Ctrl Pts',(0.187703586226661,1.18514270861395,2.31019653209487));
#46357=CARTESIAN_POINT('Ctrl Pts',(0.161326425285709,1.30000000000321,2.28929408145285));
#46358=CARTESIAN_POINT('Ctrl Pts',(0.40889487947129,-1.30000000000266,2.27992493321004));
#46359=CARTESIAN_POINT('Ctrl Pts',(0.422184967800618,-1.18514270861358,
2.29642013808564));
#46360=CARTESIAN_POINT('Ctrl Pts',(0.427747944200723,-1.06847604194603,
2.31816505247727));
#46361=CARTESIAN_POINT('Ctrl Pts',(0.422748358194651,-0.79477268400085,
2.38052803395972));
#46362=CARTESIAN_POINT('Ctrl Pts',(0.395708521594285,-0.636309800095194,
2.44435535746079));
#46363=CARTESIAN_POINT('Ctrl Pts',(0.359515267236892,-0.319434907277157,
2.5110359405381));
#46364=CARTESIAN_POINT('Ctrl Pts',(0.332737872407183,-0.158333333333332,
2.54842435869403));
#46365=CARTESIAN_POINT('Ctrl Pts',(0.302246003276087,0.158333333333334,
2.54635870301532));
#46366=CARTESIAN_POINT('Ctrl Pts',(0.297763549222328,0.319434907277168,
2.50683793103993));
#46367=CARTESIAN_POINT('Ctrl Pts',(0.273411381106316,0.636309800095205,
2.43608561538753));
#46368=CARTESIAN_POINT('Ctrl Pts',(0.267494466492831,0.794772684000836,
2.36953155090904));
#46369=CARTESIAN_POINT('Ctrl Pts',(0.226281106273681,1.06847604194621,2.30504621887655));
#46370=CARTESIAN_POINT('Ctrl Pts',(0.202920164067203,1.18514270861395,2.28284713173985));
#46371=CARTESIAN_POINT('Ctrl Pts',(0.174038016187705,1.30000000000321,2.2663622682864));
#46372=CARTESIAN_POINT('Ctrl Pts',(0.418074677884182,-1.30000000000266,
2.26695241764461));
#46373=CARTESIAN_POINT('Ctrl Pts',(0.433173626250395,-1.18514270861358,
2.28093773627827));
#46374=CARTESIAN_POINT('Ctrl Pts',(0.439971210966554,-1.06847604194603,
2.30082141255031));
#46375=CARTESIAN_POINT('Ctrl Pts',(0.436497180799323,-0.79477268400085,
2.36038306856137));
#46376=CARTESIAN_POINT('Ctrl Pts',(0.40865778436878,-0.636309800095193,
2.42453753966287));
#46377=CARTESIAN_POINT('Ctrl Pts',(0.371625020041766,-0.319434907277156,
2.49089564224033));
#46378=CARTESIAN_POINT('Ctrl Pts',(0.343321720849447,-0.158333333333332,
2.52887802547803));
#46379=CARTESIAN_POINT('Ctrl Pts',(0.312521115164033,0.158333333333334,
2.52672711617914));
#46380=CARTESIAN_POINT('Ctrl Pts',(0.30912604342682,0.319434907277167,2.48650290222469));
#46381=CARTESIAN_POINT('Ctrl Pts',(0.285248874850876,0.636309800095204,
2.41594875265761));
#46382=CARTESIAN_POINT('Ctrl Pts',(0.280261066055348,0.794772684000835,
2.3490480138972));
#46383=CARTESIAN_POINT('Ctrl Pts',(0.23737752714204,1.06847604194621,2.28731304006279));
#46384=CARTESIAN_POINT('Ctrl Pts',(0.212698397801464,1.18514270861395,2.26695798367019));
#46385=CARTESIAN_POINT('Ctrl Pts',(0.181902834124258,1.30000000000321,2.25297065355183));
#46386=CARTESIAN_POINT('Ctrl Pts',(0.421712459977973,-1.30000000000266,
2.26175696623065));
#46387=CARTESIAN_POINT('Ctrl Pts',(0.43750869095182,-1.18514270861358,2.27473287610592));
#46388=CARTESIAN_POINT('Ctrl Pts',(0.444789040576102,-1.06847604194603,
2.29386986012942));
#46389=CARTESIAN_POINT('Ctrl Pts',(0.441934715123433,-0.79477268400085,
2.35231343536506));
#46390=CARTESIAN_POINT('Ctrl Pts',(0.413838630891733,-0.636309800095194,
2.41661236431494));
#46391=CARTESIAN_POINT('Ctrl Pts',(0.376520763295964,-0.319434907277157,
2.4828531706063));
#46392=CARTESIAN_POINT('Ctrl Pts',(0.347670115184739,-0.158333333333332,
2.52108833834578));
#46393=CARTESIAN_POINT('Ctrl Pts',(0.31668812795415,0.158333333333334,2.51889016933317));
#46394=CARTESIAN_POINT('Ctrl Pts',(0.313584493009362,0.319434907277167,
2.47835102502749));
#46395=CARTESIAN_POINT('Ctrl Pts',(0.289774779982301,0.636309800095205,
2.4078482290991));
#46396=CARTESIAN_POINT('Ctrl Pts',(0.285062270626377,0.794772684000836,
2.34078811305393));
#46397=CARTESIAN_POINT('Ctrl Pts',(0.241559388623895,1.06847604194621,2.2801638124301));
#46398=CARTESIAN_POINT('Ctrl Pts',(0.216415631024418,1.18514270861395,2.26056002576535));
#46399=CARTESIAN_POINT('Ctrl Pts',(0.184958901503789,1.30000000000321,2.24759446582433));
#46400=CARTESIAN_POINT('Ctrl Pts',(0.426467295636889,-1.30000000000266,
2.25532274225131));
#46401=CARTESIAN_POINT('Ctrl Pts',(0.443311053594282,-1.18514270861358,
2.26708819267389));
#46402=CARTESIAN_POINT('Ctrl Pts',(0.451276277723858,-1.06847604194603,
2.2853159470878));
#46403=CARTESIAN_POINT('Ctrl Pts',(0.449166349613946,-0.794772684000851,
2.3423549212329));
#46404=CARTESIAN_POINT('Ctrl Pts',(0.420250688541158,-0.636309800095194,
2.40669534522819));
#46405=CARTESIAN_POINT('Ctrl Pts',(0.38253270170118,-0.319434907277156,
2.47277231690775));
#46406=CARTESIAN_POINT('Ctrl Pts',(0.353379877388863,-0.158333333333332,
2.51141997753213));
#46407=CARTESIAN_POINT('Ctrl Pts',(0.322197963808489,0.158333333333334,
2.5091693846688));
#46408=CARTESIAN_POINT('Ctrl Pts',(0.31925281525967,0.319434907277167,2.46818579243708));
#46409=CARTESIAN_POINT('Ctrl Pts',(0.295321436105165,0.636309800095204,
2.39769835401992));
#46410=CARTESIAN_POINT('Ctrl Pts',(0.290720125827061,0.794772684000836,
2.33038642787854));
#46411=CARTESIAN_POINT('Ctrl Pts',(0.246465322535933,1.06847604194621,2.27115459859657));
#46412=CARTESIAN_POINT('Ctrl Pts',(0.22082090736561,1.18514270861395,2.25250763524956));
#46413=CARTESIAN_POINT('Ctrl Pts',(0.188688341567717,1.30000000000321,2.24085297269625));
#46414=CARTESIAN_POINT('Ctrl Pts',(0.431244061790658,-1.30000000000266,
2.24889883901266));
#46415=CARTESIAN_POINT('Ctrl Pts',(0.44918891043392,-1.18514270861358,2.25946966602348));
#46416=CARTESIAN_POINT('Ctrl Pts',(0.457874292427998,-1.06847604194603,
2.27679853992569));
#46417=CARTESIAN_POINT('Ctrl Pts',(0.456548042029465,-0.79477268400085,
2.33244414553066));
#46418=CARTESIAN_POINT('Ctrl Pts',(0.42675065332855,-0.636309800095194,
2.39680886442213));
#46419=CARTESIAN_POINT('Ctrl Pts',(0.388657227913405,-0.319434907277157,
2.46272530928844));
#46420=CARTESIAN_POINT('Ctrl Pts',(0.359280563081143,-0.158333333333332,
2.5018011697518));
#46421=CARTESIAN_POINT('Ctrl Pts',(0.327911426643574,0.158333333333334,
2.49949964338542));
#46422=CARTESIAN_POINT('Ctrl Pts',(0.325087837645621,0.319434907277167,
2.45806354810334));
#46423=CARTESIAN_POINT('Ctrl Pts',(0.300977517076595,0.636309800095205,
2.38757864463434));
#46424=CARTESIAN_POINT('Ctrl Pts',(0.29642792391652,0.794772684000837,2.32000272570592));
#46425=CARTESIAN_POINT('Ctrl Pts',(0.251374607794543,1.06847604194621,2.2621518191359));
#46426=CARTESIAN_POINT('Ctrl Pts',(0.225216317221286,1.18514270861395,2.24445776965328));
#46427=CARTESIAN_POINT('Ctrl Pts',(0.192401647234186,1.30000000000321,2.23411118455496));
#46428=CARTESIAN_POINT('Ctrl Pts',(0.434968111342912,-1.30000000000266,
2.24373301200879));
#46429=CARTESIAN_POINT('Ctrl Pts',(0.45367912391193,-1.18514270861358,2.25331589338534));
#46430=CARTESIAN_POINT('Ctrl Pts',(0.462894100371637,-1.06847604194603,
2.26991264920826));
#46431=CARTESIAN_POINT('Ctrl Pts',(0.462244796355266,-0.79477268400085,
2.3244579284205));
#46432=CARTESIAN_POINT('Ctrl Pts',(0.432134940692004,-0.636309800095194,
2.3889523875418));
#46433=CARTESIAN_POINT('Ctrl Pts',(0.393770443913773,-0.319434907277157,
2.45475031567949));
#46434=CARTESIAN_POINT('Ctrl Pts',(0.363881237815788,-0.158333333333332,
2.49407930368688));
#46435=CARTESIAN_POINT('Ctrl Pts',(0.332358601705216,0.158333333333334,
2.4917337701187));
#46436=CARTESIAN_POINT('Ctrl Pts',(0.32985431461743,0.319434907277167,2.44999237980584));
#46437=CARTESIAN_POINT('Ctrl Pts',(0.305783344501939,0.636309800095205,
2.37955297547693));
#46438=CARTESIAN_POINT('Ctrl Pts',(0.301461610194176,0.794772684000836,
2.31180726361137));
#46439=CARTESIAN_POINT('Ctrl Pts',(0.255690569076344,1.06847604194621,2.25504263684815));
#46440=CARTESIAN_POINT('Ctrl Pts',(0.229015385646448,1.18514270861395,2.23808652659971));
#46441=CARTESIAN_POINT('Ctrl Pts',(0.195477606502444,1.30000000000321,2.22874560969204));
#46442=CARTESIAN_POINT('Ctrl Pts',(0.444046225881081,-1.30000000000266,
2.23075538235043));
#46443=CARTESIAN_POINT('Ctrl Pts',(0.464468729347459,-1.18514270861358,
2.23781146152863));
#46444=CARTESIAN_POINT('Ctrl Pts',(0.474925864707435,-1.06847604194603,
2.25255510224292));
#46445=CARTESIAN_POINT('Ctrl Pts',(0.476061945440884,-0.79477268400085,
2.30437566678773));
#46446=CARTESIAN_POINT('Ctrl Pts',(0.4458294729986,-0.636309800095193,2.36937781124614));
#46447=CARTESIAN_POINT('Ctrl Pts',(0.40693603065916,-0.319434907277156,
2.43492261629408));
#46448=CARTESIAN_POINT('Ctrl Pts',(0.375388524791862,-0.158333333333332,
2.47478419915548));
#46449=CARTESIAN_POINT('Ctrl Pts',(0.343486689041014,0.158333333333334,
2.47232706794512));
#46450=CARTESIAN_POINT('Ctrl Pts',(0.34194369713619,0.319434907277167,2.42986309442985));
#46451=CARTESIAN_POINT('Ctrl Pts',(0.318276616010384,0.636309800095204,
2.35960917305316));
#46452=CARTESIAN_POINT('Ctrl Pts',(0.315058623268968,0.794772684000835,
2.29156351277918));
#46453=CARTESIAN_POINT('Ctrl Pts',(0.267355287317446,1.06847604194621,2.23748173841521));
#46454=CARTESIAN_POINT('Ctrl Pts',(0.23916384314239,1.18514270861395,2.22231775032448));
#46455=CARTESIAN_POINT('Ctrl Pts',(0.203429961342996,1.30000000000321,2.21539977033806));
#46456=CARTESIAN_POINT('Ctrl Pts',(0.456822167741165,-1.30000000000266,
2.21417858708722));
#46457=CARTESIAN_POINT('Ctrl Pts',(0.48001599689858,-1.18514270861358,2.21812257914067));
#46458=CARTESIAN_POINT('Ctrl Pts',(0.492364054998585,-1.06847604194603,
2.23054701527269));
#46459=CARTESIAN_POINT('Ctrl Pts',(0.495834638598456,-0.794772684000848,
2.2788414705659));
#46460=CARTESIAN_POINT('Ctrl Pts',(0.464178241790207,-0.636309800095195,
2.3441367559944));
#46461=CARTESIAN_POINT('Ctrl Pts',(0.424377110318727,-0.319434907277159,
2.40927007814988));
#46462=CARTESIAN_POINT('Ctrl Pts',(0.391483932513137,-0.158333333333332,
2.45001856419996));
#46463=CARTESIAN_POINT('Ctrl Pts',(0.358957885118911,0.158333333333334,
2.44737481851414));
#46464=CARTESIAN_POINT('Ctrl Pts',(0.358295891275019,0.319434907277166,
2.40388130228096));
#46465=CARTESIAN_POINT('Ctrl Pts',(0.333940058166144,0.636309800095204,
2.3335691697477));
#46466=CARTESIAN_POINT('Ctrl Pts',(0.329719331263256,0.794772684000838,
2.26456161591243));
#46467=CARTESIAN_POINT('Ctrl Pts',(0.280186944664852,1.06847604194621,2.21409181215293));
#46468=CARTESIAN_POINT('Ctrl Pts',(0.251063712196728,1.18514270861395,2.2014793933697));
#46469=CARTESIAN_POINT('Ctrl Pts',(0.214257982063227,1.30000000000322,2.19810106376029));
#46470=CARTESIAN_POINT('Ctrl Pts',(0.471738537321603,-1.30000000000266,
2.19359139467269));
#46471=CARTESIAN_POINT('Ctrl Pts',(0.498459191387175,-1.18514270861358,
2.1937443110641));
#46472=CARTESIAN_POINT('Ctrl Pts',(0.513214193008901,-1.06847604194603,
2.20334023080082));
#46473=CARTESIAN_POINT('Ctrl Pts',(0.519658147617168,-0.794772684000851,
2.24732395184364));
#46474=CARTESIAN_POINT('Ctrl Pts',(0.486124807402051,-0.636309800095196,
2.31292961454153));
#46475=CARTESIAN_POINT('Ctrl Pts',(0.445306741773112,-0.319434907277158,
2.3775858381244));
#46476=CARTESIAN_POINT('Ctrl Pts',(0.410835379031462,-0.158333333333332,
2.41946437558252));
#46477=CARTESIAN_POINT('Ctrl Pts',(0.377897425156198,0.158333333333334,
2.41669026139795));
#46478=CARTESIAN_POINT('Ctrl Pts',(0.378244631154653,0.319434907277167,
2.3719123868402));
#46479=CARTESIAN_POINT('Ctrl Pts',(0.354386666183597,0.636309800095206,
2.30186056246783));
#46480=CARTESIAN_POINT('Ctrl Pts',(0.352291225354584,0.794772684000839,
2.23246446357083));
#46481=CARTESIAN_POINT('Ctrl Pts',(0.29930915091305,1.06847604194621,2.18619019140374));
#46482=CARTESIAN_POINT('Ctrl Pts',(0.26747097145162,1.18514270861395,2.17636765664866));
#46483=CARTESIAN_POINT('Ctrl Pts',(0.226728589375274,1.30000000000321,2.17675300492898));
#46484=CARTESIAN_POINT('Ctrl Pts',(0.479899051869771,-1.30000000000266,
2.18349369390981));
#46485=CARTESIAN_POINT('Ctrl Pts',(0.508096939819008,-1.18514270861359,
2.18168193670886));
#46486=CARTESIAN_POINT('Ctrl Pts',(0.523912487535125,-1.06847604194603,
2.18983223891249));
#46487=CARTESIAN_POINT('Ctrl Pts',(0.531843883631617,-0.794772684000851,
2.23167541759282));
#46488=CARTESIAN_POINT('Ctrl Pts',(0.498005492387928,-0.636309800095197,
2.29762330707595));
#46489=CARTESIAN_POINT('Ctrl Pts',(0.456885556256962,-0.319434907277159,
2.3620887571749));
#46490=CARTESIAN_POINT('Ctrl Pts',(0.421622938295452,-0.158333333333332,
2.40449900401168));
#46491=CARTESIAN_POINT('Ctrl Pts',(0.388101299179105,0.158333333333334,
2.40154708985519));
#46492=CARTESIAN_POINT('Ctrl Pts',(0.388390780368124,0.319434907277167,
2.35598614174768));
#46493=CARTESIAN_POINT('Ctrl Pts',(0.364186147471471,0.636309800095206,
2.28591277009536));
#46494=CARTESIAN_POINT('Ctrl Pts',(0.362428040910858,0.79477268400084,2.21616273366966));
#46495=CARTESIAN_POINT('Ctrl Pts',(0.308246235571133,1.06847604194622,2.17208689777873));
#46496=CARTESIAN_POINT('Ctrl Pts',(0.275593257591481,1.18514270861395,2.16377105386994));
#46497=CARTESIAN_POINT('Ctrl Pts',(0.233740597530111,1.30000000000322,2.16621816223897));
#46498=CARTESIAN_POINT('Ctrl Pts',(0.483946399133603,-1.30000000000266,
2.17843887244765));
#46499=CARTESIAN_POINT('Ctrl Pts',(0.512888765856687,-1.18514270861359,
2.17564712079955));
#46500=CARTESIAN_POINT('Ctrl Pts',(0.529237518131318,-1.06847604194603,
2.18307585696931));
#46501=CARTESIAN_POINT('Ctrl Pts',(0.537912637722501,-0.794772684000851,
2.22384909509565));
#46502=CARTESIAN_POINT('Ctrl Pts',(0.503949232631998,-0.636309800095197,
2.28997379608543));
#46503=CARTESIAN_POINT('Ctrl Pts',(0.462594679683807,-0.319434907277159,
2.35432227873226));
#46504=CARTESIAN_POINT('Ctrl Pts',(0.426715573255356,-0.158333333333332,
2.39694208629252));
#46505=CARTESIAN_POINT('Ctrl Pts',(0.392969830593601,0.158333333333334,
2.39391966368364));
#46506=CARTESIAN_POINT('Ctrl Pts',(0.393579787166861,0.319434907277167,
2.34805851202242));
#46507=CARTESIAN_POINT('Ctrl Pts',(0.369299762851234,0.636309800095206,
2.27799949945949));
#46508=CARTESIAN_POINT('Ctrl Pts',(0.367561330758701,0.79477268400084,2.20803046838465));
#46509=CARTESIAN_POINT('Ctrl Pts',(0.312674005335227,1.06847604194622,2.16502926539412));
#46510=CARTESIAN_POINT('Ctrl Pts',(0.279563873101028,1.18514270861395,2.15745638610035));
#46511=CARTESIAN_POINT('Ctrl Pts',(0.237102298032725,1.30000000000322,2.1609242549359));
#46512=CARTESIAN_POINT('',(0.213860511246102,1.2,2.25462198798418));
#46513=CARTESIAN_POINT('Ctrl Pts',(0.213860511246104,1.2,2.25462198798418));
#46514=CARTESIAN_POINT('Ctrl Pts',(0.195886995792624,1.22118111428885,2.27504564220851));
#46515=CARTESIAN_POINT('Ctrl Pts',(0.176998222640389,1.24193578764922,2.29509804001042));
#46516=CARTESIAN_POINT('Ctrl Pts',(0.151092207988087,1.27245710963303,2.32479181701016));
#46517=CARTESIAN_POINT('Ctrl Pts',(0.137742735792041,1.2882450460087,2.34018786318843));
#46518=CARTESIAN_POINT('Ctrl Pts',(0.128170675826792,1.30000000000322,2.35169387540072));
#46519=CARTESIAN_POINT('',(0.370132030376144,0.653834841391769,2.26385755069956));
#46520=CARTESIAN_POINT('Ctrl Pts',(0.370132030358563,0.653834841386714,
2.26385755066746));
#46521=CARTESIAN_POINT('Ctrl Pts',(0.355372633079986,0.712189636236907,
2.26275083105034));
#46522=CARTESIAN_POINT('Ctrl Pts',(0.340070501696384,0.767445165592266,
2.26166968552551));
#46523=CARTESIAN_POINT('Ctrl Pts',(0.30758726046148,0.882924976234983,2.25953788508247));
#46524=CARTESIAN_POINT('Ctrl Pts',(0.292298074915713,0.939652190622242,
2.25860205979761));
#46525=CARTESIAN_POINT('Ctrl Pts',(0.263959382956805,1.03591237463789,2.25703347013213));
#46526=CARTESIAN_POINT('Ctrl Pts',(0.253916623229151,1.0684334822601,2.25650694870429));
#46527=CARTESIAN_POINT('Ctrl Pts',(0.235165173386919,1.13047486660148,2.25558124511564));
#46528=CARTESIAN_POINT('Ctrl Pts',(0.224576556021974,1.16564206843845,2.25508539822476));
#46529=CARTESIAN_POINT('Ctrl Pts',(0.213860511246104,1.2,2.25462198798418));
#46530=CARTESIAN_POINT('',(0.509087305688322,-0.653834841531101,2.27624836987211));
#46531=CARTESIAN_POINT('Ctrl Pts',(0.509087305688321,-0.653834841531104,
2.27624836987211));
#46532=CARTESIAN_POINT('Ctrl Pts',(0.487739282837231,-0.575782745252652,
2.31204498712868));
#46533=CARTESIAN_POINT('Ctrl Pts',(0.468923233250106,-0.493709515665895,
2.34172379348987));
#46534=CARTESIAN_POINT('Ctrl Pts',(0.439956689959719,-0.338081440925158,
2.38329158654632));
#46535=CARTESIAN_POINT('Ctrl Pts',(0.428678359570631,-0.265625141639599,
2.39723212646428));
#46536=CARTESIAN_POINT('Ctrl Pts',(0.410247542056258,-0.12969433266082,
2.4132538570188));
#46537=CARTESIAN_POINT('Ctrl Pts',(0.402792651297061,-0.0666403947625616,
2.41677473360006));
#46538=CARTESIAN_POINT('Ctrl Pts',(0.389535713993002,0.059482301318641,
2.41596967380273));
#46539=CARTESIAN_POINT('Ctrl Pts',(0.383648853857911,0.122682321790056,
2.41165594399881));
#46540=CARTESIAN_POINT('Ctrl Pts',(0.373499427988676,0.26006074221674,2.39368024622825));
#46541=CARTESIAN_POINT('Ctrl Pts',(0.369686868827108,0.333931391400696,
2.37844650643877));
#46542=CARTESIAN_POINT('Ctrl Pts',(0.366022638034873,0.491495423102932,
2.3336888357912));
#46543=CARTESIAN_POINT('Ctrl Pts',(0.366607600922235,0.574890353678907,
2.3019351734762));
#46544=CARTESIAN_POINT('Ctrl Pts',(0.370132030316485,0.653834841406594,
2.26385755072478));
#46545=CARTESIAN_POINT('',(0.437191572703802,-1.2,2.26934451327648));
#46546=CARTESIAN_POINT('Ctrl Pts',(0.437191572703802,-1.2,2.26934451327648));
#46547=CARTESIAN_POINT('Ctrl Pts',(0.450657019484388,-1.12876701747688,
2.2705384680906));
#46548=CARTESIAN_POINT('Ctrl Pts',(0.467003073169165,-1.03051724707754,
2.27204751542371));
#46549=CARTESIAN_POINT('Ctrl Pts',(0.49993829496903,-0.776505233457344,
2.27528643342527));
#46550=CARTESIAN_POINT('Ctrl Pts',(0.504034558319737,-0.721760519705801,
2.27572594515669));
#46551=CARTESIAN_POINT('Ctrl Pts',(0.509087305688321,-0.653834841531101,
2.27624836987212));
#46552=CARTESIAN_POINT('Ctrl Pts',(0.35416429646195,-1.3,2.36294845478037));
#46553=CARTESIAN_POINT('Ctrl Pts',(0.368383275106154,-1.28213859625167,
2.34608033732313));
#46554=CARTESIAN_POINT('Ctrl Pts',(0.383008753255496,-1.26440354740105,
2.32942146191478));
#46555=CARTESIAN_POINT('Ctrl Pts',(0.416069593475857,-1.22469302390907,
2.29227038705738));
#46556=CARTESIAN_POINT('Ctrl Pts',(0.423498885283735,-1.21525386319095,
2.28344411837659));
#46557=CARTESIAN_POINT('Ctrl Pts',(0.437191572703802,-1.2,2.26934451327648));
#46558=CARTESIAN_POINT('Origin',(0.,1.25,7.2));
#46559=CARTESIAN_POINT('Origin',(0.,1.2,7.2));
#46560=CARTESIAN_POINT('Origin',(0.,0.92691742076555,7.2));
#46561=CARTESIAN_POINT('Origin',(0.,0.653834841531101,7.2));
#46562=CARTESIAN_POINT('Origin',(0.,0.,7.2));
#46563=CARTESIAN_POINT('Origin',(0.,-0.653834841531101,7.2));
#46564=CARTESIAN_POINT('Origin',(0.,-0.926917420765551,7.2));
#46565=CARTESIAN_POINT('Origin',(0.,-1.2,7.2));
#46566=CARTESIAN_POINT('Origin',(0.,-1.25,7.2));
#46567=CARTESIAN_POINT('Ctrl Pts',(0.815761714367341,-1.30000000000348,
2.2217438103648));
#46568=CARTESIAN_POINT('Ctrl Pts',(0.774949037064399,-1.18514270861414,
2.20952346491477));
#46569=CARTESIAN_POINT('Ctrl Pts',(0.7409879505214,-1.06847604194631,2.21004687504984));
#46570=CARTESIAN_POINT('Ctrl Pts',(0.678359592026837,-0.794772684000851,
2.24069668195063));
#46571=CARTESIAN_POINT('Ctrl Pts',(0.662111769290086,-0.636309800095197,
2.30877528147029));
#46572=CARTESIAN_POINT('Ctrl Pts',(0.623796234000798,-0.319434907277159,
2.37225523561121));
#46573=CARTESIAN_POINT('Ctrl Pts',(0.614857791974963,-0.158333333333332,
2.4172410281768));
#46574=CARTESIAN_POINT('Ctrl Pts',(0.581221077760459,0.158333333333334,
2.41318126918527));
#46575=CARTESIAN_POINT('Ctrl Pts',(0.554987172143311,0.319434907277167,
2.36403312099341));
#46576=CARTESIAN_POINT('Ctrl Pts',(0.527915117225985,0.636309800095206,
2.29249271205691));
#46577=CARTESIAN_POINT('Ctrl Pts',(0.508441992410805,0.79477268400084,2.22075160546092));
#46578=CARTESIAN_POINT('Ctrl Pts',(0.525404772703901,1.06847604194528,2.18267301919523));
#46579=CARTESIAN_POINT('Ctrl Pts',(0.542940786614004,1.18514270861212,2.17880571546092));
#46580=CARTESIAN_POINT('Ctrl Pts',(0.570670255378281,1.30000000000051,2.18755391703607));
#46581=CARTESIAN_POINT('Ctrl Pts',(0.817949288434644,-1.30000000000348,
2.22762096990277));
#46582=CARTESIAN_POINT('Ctrl Pts',(0.777519991852497,-1.18514270861414,
2.21652567939064));
#46583=CARTESIAN_POINT('Ctrl Pts',(0.743851598618606,-1.06847604194631,
2.21787086628889));
#46584=CARTESIAN_POINT('Ctrl Pts',(0.681689914158223,-0.794772684000851,
2.24971850865432));
#46585=CARTESIAN_POINT('Ctrl Pts',(0.665468378431205,-0.636309800095197,
2.3175788085538));
#46586=CARTESIAN_POINT('Ctrl Pts',(0.627223601653558,-0.319434907277159,
2.38108848276862));
#46587=CARTESIAN_POINT('Ctrl Pts',(0.618034103229147,-0.158333333333332,
2.42571400136448));
#46588=CARTESIAN_POINT('Ctrl Pts',(0.584631254891397,0.158333333333334,
2.42163186844655));
#46589=CARTESIAN_POINT('Ctrl Pts',(0.558956795864976,0.319434907277167,
2.37281687672975));
#46590=CARTESIAN_POINT('Ctrl Pts',(0.532138549723521,0.636309800095206,
2.30121083594925));
#46591=CARTESIAN_POINT('Ctrl Pts',(0.512750945719485,0.79477268400084,2.22966866896796));
#46592=CARTESIAN_POINT('Ctrl Pts',(0.529208707810351,1.06847604194528,2.19038889410686));
#46593=CARTESIAN_POINT('Ctrl Pts',(0.546373190975948,1.18514270861212,2.18570493282075));
#46594=CARTESIAN_POINT('Ctrl Pts',(0.573578201918189,1.30000000000051,2.1933397693268));
#46595=CARTESIAN_POINT('Ctrl Pts',(0.822480438837854,-1.30000000000349,
2.23938366296825));
#46596=CARTESIAN_POINT('Ctrl Pts',(0.782697976355179,-1.18514270861414,
2.23053940047333));
#46597=CARTESIAN_POINT('Ctrl Pts',(0.749515793345079,-1.06847604194632,
2.23352974476871));
#46598=CARTESIAN_POINT('Ctrl Pts',(0.688106278482148,-0.794772684000857,
2.26777834749776));
#46599=CARTESIAN_POINT('Ctrl Pts',(0.67177948580503,-0.636309800095199,
2.33521414055764));
#46600=CARTESIAN_POINT('Ctrl Pts',(0.633792497448733,-0.319434907277159,
2.39877822350881));
#46601=CARTESIAN_POINT('Ctrl Pts',(0.624484670435901,-0.158333333333333,
2.44266448378591));
#46602=CARTESIAN_POINT('Ctrl Pts',(0.591715216368591,0.158333333333335,
2.43852754202018));
#46603=CARTESIAN_POINT('Ctrl Pts',(0.567079234854538,0.319434907277167,
2.39037832109855));
#46604=CARTESIAN_POINT('Ctrl Pts',(0.540709280232551,0.636309800095207,
2.3186442770227));
#46605=CARTESIAN_POINT('Ctrl Pts',(0.521366831150013,0.794772684000843,
2.24751275404973));
#46606=CARTESIAN_POINT('Ctrl Pts',(0.536815007810077,1.06847604194529,2.20583058195238));
#46607=CARTESIAN_POINT('Ctrl Pts',(0.553267033024608,1.18514270861212,2.19951049152181));
#46608=CARTESIAN_POINT('Ctrl Pts',(0.579484140188884,1.30000000000051,2.20491297848492));
#46609=CARTESIAN_POINT('Ctrl Pts',(0.827534611873413,-1.30000000000348,
2.25405439187517));
#46610=CARTESIAN_POINT('Ctrl Pts',(0.789705377274445,-1.18514270861414,
2.24801726208739));
#46611=CARTESIAN_POINT('Ctrl Pts',(0.757829796105519,-1.06847604194632,
2.25306288479746));
#46612=CARTESIAN_POINT('Ctrl Pts',(0.697944957365153,-0.794772684000858,
2.29032265799794));
#46613=CARTESIAN_POINT('Ctrl Pts',(0.680137957616897,-0.636309800095199,
2.35725623009178));
#46614=CARTESIAN_POINT('Ctrl Pts',(0.641914390341109,-0.319434907277159,
2.42091020322842));
#46615=CARTESIAN_POINT('Ctrl Pts',(0.632611912435405,-0.158333333333333,
2.46386008262676));
#46616=CARTESIAN_POINT('Ctrl Pts',(0.600064040384407,0.158333333333335,
2.45970027866479));
#46617=CARTESIAN_POINT('Ctrl Pts',(0.575717151510573,0.31943490727717,2.41247332235234));
#46618=CARTESIAN_POINT('Ctrl Pts',(0.549886712394817,0.636309800095209,
2.34058500462056));
#46619=CARTESIAN_POINT('Ctrl Pts',(0.53195046354595,0.794772684000843,2.26986813875903));
#46620=CARTESIAN_POINT('Ctrl Pts',(0.546133892069255,1.06847604194529,2.22516386723107));
#46621=CARTESIAN_POINT('Ctrl Pts',(0.561433503866172,1.18514270861212,2.21680472792377));
#46622=CARTESIAN_POINT('Ctrl Pts',(0.585893246800085,1.30000000000051,2.21943727199712));
#46623=CARTESIAN_POINT('Ctrl Pts',(0.833274616578554,-1.30000000000348,
2.27170676121989));
#46624=CARTESIAN_POINT('Ctrl Pts',(0.796691660229516,-1.18514270861414,
2.26906812379398));
#46625=CARTESIAN_POINT('Ctrl Pts',(0.765764921284813,-1.06847604194632,
2.27659600561126));
#46626=CARTESIAN_POINT('Ctrl Pts',(0.707384961176366,-0.794772684000854,
2.31747361181352));
#46627=CARTESIAN_POINT('Ctrl Pts',(0.689805300234883,-0.636309800095199,
2.38373849431988));
#46628=CARTESIAN_POINT('Ctrl Pts',(0.651479287123272,-0.31943490727716,
2.44749818966568));
#46629=CARTESIAN_POINT('Ctrl Pts',(0.640702068838736,-0.158333333333333,
2.48938875417485));
#46630=CARTESIAN_POINT('Ctrl Pts',(0.608698086977467,0.158333333333335,
2.48518269228587));
#46631=CARTESIAN_POINT('Ctrl Pts',(0.586397462498248,0.319434907277168,
2.43897134670432));
#46632=CARTESIAN_POINT('Ctrl Pts',(0.561721046259436,0.636309800095208,
2.36687788085369));
#46633=CARTESIAN_POINT('Ctrl Pts',(0.544514136142152,0.794772684000843,
2.29672597466129));
#46634=CARTESIAN_POINT('Ctrl Pts',(0.557236461195469,1.06847604194529,2.24839375600363));
#46635=CARTESIAN_POINT('Ctrl Pts',(0.571326105454448,1.18514270861212,2.23757572236879));
#46636=CARTESIAN_POINT('Ctrl Pts',(0.593998370865426,1.30000000000051,2.23686088167082));
#46637=CARTESIAN_POINT('Ctrl Pts',(0.838472051594579,-1.30000000000349,
2.28497244552649));
#46638=CARTESIAN_POINT('Ctrl Pts',(0.802393619181787,-1.18514270861415,
2.28487318828213));
#46639=CARTESIAN_POINT('Ctrl Pts',(0.771873709768992,-1.06847604194632,
2.29425687379296));
#46640=CARTESIAN_POINT('Ctrl Pts',(0.714207913647501,-0.794772684000862,
2.33784255934328));
#46641=CARTESIAN_POINT('Ctrl Pts',(0.696654586576742,-0.636309800095204,
2.40363091935228));
#46642=CARTESIAN_POINT('Ctrl Pts',(0.658879800371154,-0.319434907277162,
2.46744541131595));
#46643=CARTESIAN_POINT('Ctrl Pts',(0.64860187246558,-0.158333333333334,
2.50847000637261));
#46644=CARTESIAN_POINT('Ctrl Pts',(0.616923322998412,0.158333333333336,
2.50423682079874));
#46645=CARTESIAN_POINT('Ctrl Pts',(0.594328865496985,0.31943490727717,2.45887586832793));
#46646=CARTESIAN_POINT('Ctrl Pts',(0.570008485219607,0.636309800095213,
2.38664883575975));
#46647=CARTESIAN_POINT('Ctrl Pts',(0.554294603428068,0.794772684000849,
2.3168668138778));
#46648=CARTESIAN_POINT('Ctrl Pts',(0.565934859131679,1.06847604194529,2.26580745919462));
#46649=CARTESIAN_POINT('Ctrl Pts',(0.578992677077282,1.18514270861213,2.25314966902608));
#46650=CARTESIAN_POINT('Ctrl Pts',(0.600069677588373,1.30000000000052,2.2499357913958));
#46651=CARTESIAN_POINT('Ctrl Pts',(0.842426321676452,-1.30000000000349,
2.29673831794152));
#46652=CARTESIAN_POINT('Ctrl Pts',(0.807669532123175,-1.18514270861415,
2.29890154496789));
#46653=CARTESIAN_POINT('Ctrl Pts',(0.778044811919046,-1.06847604194632,
2.3099405040634));
#46654=CARTESIAN_POINT('Ctrl Pts',(0.721461888706337,-0.794772684000861,
2.35594742457385));
#46655=CARTESIAN_POINT('Ctrl Pts',(0.703138929641752,-0.636309800095203,
2.42131458953646));
#46656=CARTESIAN_POINT('Ctrl Pts',(0.664974654116365,-0.319434907277162,
2.48520860293727));
#46657=CARTESIAN_POINT('Ctrl Pts',(0.653927425302214,-0.158333333333334,
2.5255137757051));
#46658=CARTESIAN_POINT('Ctrl Pts',(0.62257423698162,0.158333333333336,2.52125543432605));
#46659=CARTESIAN_POINT('Ctrl Pts',(0.601347319644754,0.319434907277171,
2.47657922652961));
#46660=CARTESIAN_POINT('Ctrl Pts',(0.577523332854969,0.636309800095213,
2.40424082720034));
#46661=CARTESIAN_POINT('Ctrl Pts',(0.561729528529115,0.794772684000849,
2.33488259506381));
#46662=CARTESIAN_POINT('Ctrl Pts',(0.572424770514813,1.06847604194529,2.28139441775701));
#46663=CARTESIAN_POINT('Ctrl Pts',(0.584831835923992,1.18514270861213,2.26707904245198));
#46664=CARTESIAN_POINT('Ctrl Pts',(0.60501639278451,1.30000000000052,2.26160134186575));
#46665=CARTESIAN_POINT('Ctrl Pts',(0.8438497664825,-1.30000000000349,2.30115438810863));
#46666=CARTESIAN_POINT('Ctrl Pts',(0.809459220322253,-1.18514270861415,
2.30416804614865));
#46667=CARTESIAN_POINT('Ctrl Pts',(0.780093900817013,-1.06847604194632,
2.31582890677064));
#46668=CARTESIAN_POINT('Ctrl Pts',(0.723863417114391,-0.794772684000862,
2.36274459538565));
#46669=CARTESIAN_POINT('Ctrl Pts',(0.705401126882505,-0.636309800095203,
2.42795199955603));
#46670=CARTESIAN_POINT('Ctrl Pts',(0.667214983652006,-0.319434907277162,
2.49187283705493));
#46671=CARTESIAN_POINT('Ctrl Pts',(0.656010235704721,-0.158333333333334,
2.53190307843187));
#46672=CARTESIAN_POINT('Ctrl Pts',(0.624775101141794,0.158333333333336,
2.52763656325065));
#46673=CARTESIAN_POINT('Ctrl Pts',(0.603848368774456,0.319434907277171,
2.48322770226953));
#46674=CARTESIAN_POINT('Ctrl Pts',(0.580236583661767,0.636309800095213,
2.41084462918358));
#46675=CARTESIAN_POINT('Ctrl Pts',(0.564680105060892,0.794772684000849,
2.34162841200642));
#46676=CARTESIAN_POINT('Ctrl Pts',(0.57505182445287,1.06847604194529,2.28722736164216));
#46677=CARTESIAN_POINT('Ctrl Pts',(0.587180532214312,1.18514270861213,2.27229261411699));
#46678=CARTESIAN_POINT('Ctrl Pts',(0.606948414722484,1.30000000000052,2.26597131801177));
#46679=CARTESIAN_POINT('Ctrl Pts',(0.845225075246657,-1.30000000000349,
2.30557234964075));
#46680=CARTESIAN_POINT('Ctrl Pts',(0.81114213914197,-1.18514270861415,2.3094377763209));
#46681=CARTESIAN_POINT('Ctrl Pts',(0.782001214760848,-1.06847604194632,
2.32172138880894));
#46682=CARTESIAN_POINT('Ctrl Pts',(0.726096885546306,-0.794772684000862,
2.36954668425287));
#46683=CARTESIAN_POINT('Ctrl Pts',(0.707561471282311,-0.636309800095204,
2.43459335551303));
#46684=CARTESIAN_POINT('Ctrl Pts',(0.66940386339763,-0.319434907277162,
2.49853986597122));
#46685=CARTESIAN_POINT('Ctrl Pts',(0.658091989424287,-0.158333333333334,
2.53829296608385));
#46686=CARTESIAN_POINT('Ctrl Pts',(0.626973132394117,0.158333333333336,
2.53401917970609));
#46687=CARTESIAN_POINT('Ctrl Pts',(0.606257617298661,0.319434907277171,
2.48988288844787));
#46688=CARTESIAN_POINT('Ctrl Pts',(0.582878968391157,0.636309800095214,
2.41745383249566));
#46689=CARTESIAN_POINT('Ctrl Pts',(0.567689353837315,0.794772684000849,
2.34837164734979));
#46690=CARTESIAN_POINT('Ctrl Pts',(0.577756049883937,1.06847604194529,2.29305625514846));
#46691=CARTESIAN_POINT('Ctrl Pts',(0.589591259077048,1.18514270861213,2.2775028556469));
#46692=CARTESIAN_POINT('Ctrl Pts',(0.608904177752535,1.30000000000052,2.27034004029047));
#46693=CARTESIAN_POINT('Ctrl Pts',(0.84787373850355,-1.30000000000349,2.31441471133581));
#46694=CARTESIAN_POINT('Ctrl Pts',(0.814200412838562,-1.18514270861415,
2.319987142917));
#46695=CARTESIAN_POINT('Ctrl Pts',(0.7853851804585,-1.06847604194632,2.33351833085404));
#46696=CARTESIAN_POINT('Ctrl Pts',(0.730039396539782,-0.794772684000861,
2.38316440121895));
#46697=CARTESIAN_POINT('Ctrl Pts',(0.711571769008138,-0.636309800095203,
2.44788687284398));
#46698=CARTESIAN_POINT('Ctrl Pts',(0.673676578636946,-0.319434907277162,
2.51187945678191));
#46699=CARTESIAN_POINT('Ctrl Pts',(0.662395363999465,-0.158333333333334,
2.55106875502679));
#46700=CARTESIAN_POINT('Ctrl Pts',(0.631512165133043,0.158333333333336,
2.54678256436095));
#46701=CARTESIAN_POINT('Ctrl Pts',(0.610861968467718,0.31943490727717,2.50320992785811));
#46702=CARTESIAN_POINT('Ctrl Pts',(0.587985439671236,0.636309800095212,
2.43068456480014));
#46703=CARTESIAN_POINT('Ctrl Pts',(0.573946563231074,0.794772684000848,
2.3618426182233));
#46704=CARTESIAN_POINT('Ctrl Pts',(0.583473112734683,1.06847604194529,2.30469460083018));
#46705=CARTESIAN_POINT('Ctrl Pts',(0.594682459314614,1.18514270861213,2.28790715539512));
#46706=CARTESIAN_POINT('Ctrl Pts',(0.612977462187809,1.30000000000052,2.27906952371177));
#46707=CARTESIAN_POINT('Ctrl Pts',(0.852103938572023,-1.30000000000349,
2.32767411969882));
#46708=CARTESIAN_POINT('Ctrl Pts',(0.8194522968669,-1.18514270861415,2.33580350301075));
#46709=CARTESIAN_POINT('Ctrl Pts',(0.791333461953259,-1.06847604194632,
2.35120472677436));
#46710=CARTESIAN_POINT('Ctrl Pts',(0.736845018622613,-0.794772684000859,
2.40358404084236));
#46711=CARTESIAN_POINT('Ctrl Pts',(0.717802411277297,-0.636309800095203,
2.46782682103428));
#46712=CARTESIAN_POINT('Ctrl Pts',(0.679656280419845,-0.319434907277162,
2.53190271397085));
#46713=CARTESIAN_POINT('Ctrl Pts',(0.667771211845641,-0.158333333333334,
2.57026656208597));
#46714=CARTESIAN_POINT('Ctrl Pts',(0.637292788680856,0.158333333333336,
2.56596154500988));
#46715=CARTESIAN_POINT('Ctrl Pts',(0.617824840813535,0.31943490727717,2.52319718370858));
#46716=CARTESIAN_POINT('Ctrl Pts',(0.595670101735524,0.636309800095212,
2.45054679965987));
#46717=CARTESIAN_POINT('Ctrl Pts',(0.582135679870625,0.794772684000848,
2.38214575462174));
#46718=CARTESIAN_POINT('Ctrl Pts',(0.590787034920216,1.06847604194529,2.32224861478318));
#46719=CARTESIAN_POINT('Ctrl Pts',(0.601255474529726,1.18514270861213,2.30359241829711));
#46720=CARTESIAN_POINT('Ctrl Pts',(0.618447502712073,1.30000000000052,2.29220727775335));
#46721=CARTESIAN_POINT('Ctrl Pts',(0.857969453717047,-1.30000000000349,
2.34536437000766));
#46722=CARTESIAN_POINT('Ctrl Pts',(0.826874392876982,-1.18514270861415,
2.35690645245089));
#46723=CARTESIAN_POINT('Ctrl Pts',(0.799812377387329,-1.06847604194632,
2.37480354034066));
#46724=CARTESIAN_POINT('Ctrl Pts',(0.746610849436285,-0.794772684000859,
2.43083072756189));
#46725=CARTESIAN_POINT('Ctrl Pts',(0.726719229771669,-0.636309800095202,
2.49443343321409));
#46726=CARTESIAN_POINT('Ctrl Pts',(0.688052574451537,-0.319434907277161,
2.55861968388106));
#46727=CARTESIAN_POINT('Ctrl Pts',(0.675108317438119,-0.158333333333334,
2.59587838761032));
#46728=CARTESIAN_POINT('Ctrl Pts',(0.644961961098522,0.158333333333336,
2.59155173687621));
#46729=CARTESIAN_POINT('Ctrl Pts',(0.626942933423789,0.31943490727717,2.54987878732425));
#46730=CARTESIAN_POINT('Ctrl Pts',(0.605867655715064,0.636309800095211,
2.47705788552953));
#46731=CARTESIAN_POINT('Ctrl Pts',(0.593407148634716,0.794772684000847,
2.40922488538287));
#46732=CARTESIAN_POINT('Ctrl Pts',(0.601050462974228,1.06847604194529,2.34565394034333));
#46733=CARTESIAN_POINT('Ctrl Pts',(0.610545298265256,1.18514270861213,2.3245048766012));
#46734=CARTESIAN_POINT('Ctrl Pts',(0.626226461282443,1.30000000000052,2.3097242556889));
#46735=CARTESIAN_POINT('Ctrl Pts',(0.864892167006608,-1.30000000000349,
2.36896827823977));
#46736=CARTESIAN_POINT('Ctrl Pts',(0.835076211528464,-1.18514270861415,
2.38507496762836));
#46737=CARTESIAN_POINT('Ctrl Pts',(0.808890045383593,-1.06847604194632,
2.40630938309406));
#46738=CARTESIAN_POINT('Ctrl Pts',(0.756780302561369,-0.794772684000858,
2.46721120378601));
#46739=CARTESIAN_POINT('Ctrl Pts',(0.736004391759345,-0.636309800095201,
2.52995196405356));
#46740=CARTESIAN_POINT('Ctrl Pts',(0.697428015081395,-0.31943490727716,
2.59427726117001));
#46741=CARTESIAN_POINT('Ctrl Pts',(0.68434036320485,-0.158333333333333,
2.63004974172785));
#46742=CARTESIAN_POINT('Ctrl Pts',(0.655322158131372,0.158333333333335,
2.62569284382494));
#46743=CARTESIAN_POINT('Ctrl Pts',(0.639198686598927,0.319434907277169,
2.58547284172007));
#46744=CARTESIAN_POINT('Ctrl Pts',(0.619060029681164,0.63630980009521,2.5124574511204));
#46745=CARTESIAN_POINT('Ctrl Pts',(0.606808450459504,0.794772684000846,
2.44545422774618));
#46746=CARTESIAN_POINT('Ctrl Pts',(0.612845176618029,1.06847604194529,2.3769830649708));
#46747=CARTESIAN_POINT('Ctrl Pts',(0.621157569349446,1.18514270861213,2.35249169112608));
#46748=CARTESIAN_POINT('Ctrl Pts',(0.635169279741,1.30000000000051,2.33314757269551));
#46749=CARTESIAN_POINT('Ctrl Pts',(0.871983856110559,-1.30000000000349,
2.39259530305307));
#46750=CARTESIAN_POINT('Ctrl Pts',(0.843492504925306,-1.18514270861415,
2.41326700102741));
#46751=CARTESIAN_POINT('Ctrl Pts',(0.818280869489698,-1.06847604194632,
2.43783986036201));
#46752=CARTESIAN_POINT('Ctrl Pts',(0.767613747549898,-0.794772684000856,
2.50362054437507));
#46753=CARTESIAN_POINT('Ctrl Pts',(0.746699420507565,-0.636309800095201,
2.56550661167277));
#46754=CARTESIAN_POINT('Ctrl Pts',(0.708067863075721,-0.319434907277161,
2.62997336311469));
#46755=CARTESIAN_POINT('Ctrl Pts',(0.694162607171851,-0.158333333333333,
2.6642445087104));
#46756=CARTESIAN_POINT('Ctrl Pts',(0.665302359551536,0.158333333333335,
2.65987892344331));
#46757=CARTESIAN_POINT('Ctrl Pts',(0.6498918287039,0.319434907277168,2.62116799218465));
#46758=CARTESIAN_POINT('Ctrl Pts',(0.630665040150285,0.636309800095209,
2.54795999874999));
#46759=CARTESIAN_POINT('Ctrl Pts',(0.619960840132648,0.794772684000845,
2.48173444454022));
#46760=CARTESIAN_POINT('Ctrl Pts',(0.625102222111385,1.06847604194529,2.40833499866515));
#46761=CARTESIAN_POINT('Ctrl Pts',(0.632439243853823,1.18514270861213,2.38049291658993));
#46762=CARTESIAN_POINT('Ctrl Pts',(0.644887773587081,1.30000000000052,2.3565806528413));
#46763=CARTESIAN_POINT('Ctrl Pts',(0.8788002795845,-1.30000000000349,2.41622813084116));
#46764=CARTESIAN_POINT('Ctrl Pts',(0.851801484847447,-1.18514270861415,
2.44148383612387));
#46765=CARTESIAN_POINT('Ctrl Pts',(0.827464580237682,-1.06847604194632,
2.46940614964295));
#46766=CARTESIAN_POINT('Ctrl Pts',(0.77739096071164,-0.794772684000858,
2.54007267819047));
#46767=CARTESIAN_POINT('Ctrl Pts',(0.754165665727303,-0.636309800095201,
2.60107065326827));
#46768=CARTESIAN_POINT('Ctrl Pts',(0.715146022357394,-0.31943490727716,
2.66567920983969));
#46769=CARTESIAN_POINT('Ctrl Pts',(0.701755319112731,-0.158333333333333,
2.69847254135808));
#46770=CARTESIAN_POINT('Ctrl Pts',(0.674041403273267,0.158333333333335,
2.69410734100179));
#46771=CARTESIAN_POINT('Ctrl Pts',(0.659818978446064,0.319434907277168,
2.65690091063574));
#46772=CARTESIAN_POINT('Ctrl Pts',(0.642182073293505,0.636309800095209,
2.58349832102157));
#46773=CARTESIAN_POINT('Ctrl Pts',(0.633514118471711,0.794772684000844,
2.51804753122718));
#46774=CARTESIAN_POINT('Ctrl Pts',(0.637539702821843,1.06847604194529,2.43971769905602));
#46775=CARTESIAN_POINT('Ctrl Pts',(0.643595422408555,1.18514270861213,2.40852429620439));
#46776=CARTESIAN_POINT('Ctrl Pts',(0.653964335279407,1.30000000000051,2.38004357244173));
#46777=CARTESIAN_POINT('Ctrl Pts',(0.883492139156687,-1.30000000000349,
2.43396916719493));
#46778=CARTESIAN_POINT('Ctrl Pts',(0.856681013500535,-1.18514270861415,
2.46264282535752));
#46779=CARTESIAN_POINT('Ctrl Pts',(0.832636437723441,-1.06847604194632,
2.49306744915883));
#46780=CARTESIAN_POINT('Ctrl Pts',(0.783479941244749,-0.794772684000857,
2.56739949746954));
#46781=CARTESIAN_POINT('Ctrl Pts',(0.761811990638407,-0.636309800095201,
2.62778407484409));
#46782=CARTESIAN_POINT('Ctrl Pts',(0.722835384880657,-0.319434907277161,
2.69250196767029));
#46783=CARTESIAN_POINT('Ctrl Pts',(0.707689306788051,-0.158333333333333,
2.72414441130098));
#46784=CARTESIAN_POINT('Ctrl Pts',(0.679787873058307,0.158333333333335,
2.71977688689778));
#46785=CARTESIAN_POINT('Ctrl Pts',(0.666709735021752,0.319434907277167,
2.68371615702853));
#46786=CARTESIAN_POINT('Ctrl Pts',(0.649510613748425,0.636309800095208,
2.61020532966889));
#46787=CARTESIAN_POINT('Ctrl Pts',(0.640923069406501,0.794772684000846,
2.54540094788882));
#46788=CARTESIAN_POINT('Ctrl Pts',(0.644416052402014,1.06847604194529,2.46336564844072));
#46789=CARTESIAN_POINT('Ctrl Pts',(0.650065032644106,1.18514270861213,2.42963732643914));
#46790=CARTESIAN_POINT('Ctrl Pts',(0.659851010217308,1.30000000000052,2.39769072385965));
#46791=CARTESIAN_POINT('Ctrl Pts',(0.889558734078806,-1.30000000000349,
2.45759430808821));
#46792=CARTESIAN_POINT('Ctrl Pts',(0.864447810104551,-1.18514270861414,
2.49087694996875));
#46793=CARTESIAN_POINT('Ctrl Pts',(0.841353620899978,-1.06847604194632,
2.52466490734447));
#46794=CARTESIAN_POINT('Ctrl Pts',(0.79266048462534,-0.794772684000856,
2.60388922802155));
#46795=CARTESIAN_POINT('Ctrl Pts',(0.768013225048203,-0.636309800095199,
2.66334041368903));
#46796=CARTESIAN_POINT('Ctrl Pts',(0.728336186096216,-0.319434907277159,
2.72819115831008));
#46797=CARTESIAN_POINT('Ctrl Pts',(0.713521471386971,-0.158333333333333,
2.75836682748481));
#46798=CARTESIAN_POINT('Ctrl Pts',(0.687308314473149,0.158333333333335,
2.75402055085611));
#46799=CARTESIAN_POINT('Ctrl Pts',(0.676549378221223,0.319434907277169,
2.71949091277189));
#46800=CARTESIAN_POINT('Ctrl Pts',(0.661529476370098,0.636309800095208,
2.64580278422258));
#46801=CARTESIAN_POINT('Ctrl Pts',(0.654713806832131,0.794772684000841,
2.58177408144104));
#46802=CARTESIAN_POINT('Ctrl Pts',(0.657054029412615,1.06847604194529,2.49479983622051));
#46803=CARTESIAN_POINT('Ctrl Pts',(0.661390646011638,1.18514270861212,2.4577127159111));
#46804=CARTESIAN_POINT('Ctrl Pts',(0.669050883568385,1.30000000000051,2.42118640333487));
#46805=CARTESIAN_POINT('Ctrl Pts',(0.894786825006837,-1.30000000000348,
2.48121808219932));
#46806=CARTESIAN_POINT('Ctrl Pts',(0.870089124157715,-1.18514270861414,
2.51907311933544));
#46807=CARTESIAN_POINT('Ctrl Pts',(0.847384183496986,-1.06847604194632,
2.55620783446828));
#46808=CARTESIAN_POINT('Ctrl Pts',(0.799534903148645,-0.794772684000854,
2.64033236727146));
#46809=CARTESIAN_POINT('Ctrl Pts',(0.775766393023481,-0.636309800095198,
2.69895575203986));
#46810=CARTESIAN_POINT('Ctrl Pts',(0.736000855364474,-0.319434907277159,
2.76395207302188));
#46811=CARTESIAN_POINT('Ctrl Pts',(0.719880786059042,-0.158333333333333,
2.79258698076943));
#46812=CARTESIAN_POINT('Ctrl Pts',(0.693412198460061,0.158333333333335,
2.78825422777218));
#46813=CARTESIAN_POINT('Ctrl Pts',(0.68301387996786,0.319434907277168,2.75528325192732));
#46814=CARTESIAN_POINT('Ctrl Pts',(0.668966249908217,0.636309800095208,
2.68146817767856));
#46815=CARTESIAN_POINT('Ctrl Pts',(0.663916868088444,0.794772684000843,
2.61829877751067));
#46816=CARTESIAN_POINT('Ctrl Pts',(0.666256460671176,1.06847604194529,2.52637732519999));
#46817=CARTESIAN_POINT('Ctrl Pts',(0.670153579812955,1.18514270861212,2.48590479535088));
#46818=CARTESIAN_POINT('Ctrl Pts',(0.676935095157896,1.30000000000051,2.4447491263325));
#46819=CARTESIAN_POINT('Ctrl Pts',(0.900920744455079,-1.30000000000348,
2.50489467825102));
#46820=CARTESIAN_POINT('Ctrl Pts',(0.877338716593721,-1.18514270861414,
2.54735202983343));
#46821=CARTESIAN_POINT('Ctrl Pts',(0.855233562772959,-1.06847604194632,
2.58784497109303));
#46822=CARTESIAN_POINT('Ctrl Pts',(0.807578109807804,-0.794772684000853,
2.67685358516273));
#46823=CARTESIAN_POINT('Ctrl Pts',(0.781865791711984,-0.636309800095199,
2.73455216483046));
#46824=CARTESIAN_POINT('Ctrl Pts',(0.741131641213366,-0.31943490727716,
2.79966201910889));
#46825=CARTESIAN_POINT('Ctrl Pts',(0.724343372132867,-0.158333333333333,
2.82678245074128));
#46826=CARTESIAN_POINT('Ctrl Pts',(0.698885888203835,0.158333333333335,
2.8224844959558));
#46827=CARTESIAN_POINT('Ctrl Pts',(0.690689565611929,0.319434907277167,
2.79110176251162));
#46828=CARTESIAN_POINT('Ctrl Pts',(0.678605406869406,0.636309800095207,
2.7171646612579));
#46829=CARTESIAN_POINT('Ctrl Pts',(0.675175735315677,0.794772684000843,
2.65482275704941));
#46830=CARTESIAN_POINT('Ctrl Pts',(0.676706066558325,1.06847604194529,2.5579519195565));
#46831=CARTESIAN_POINT('Ctrl Pts',(0.679566040662273,1.18514270861212,2.51409824761092));
#46832=CARTESIAN_POINT('Ctrl Pts',(0.684623565179587,1.30000000000051,2.46832269985219));
#46833=CARTESIAN_POINT('Ctrl Pts',(0.90391928274594,-1.30000000000348,2.52258106592965));
#46834=CARTESIAN_POINT('Ctrl Pts',(0.880390345489287,-1.18514270861414,
2.5684617029937));
#46835=CARTESIAN_POINT('Ctrl Pts',(0.858348979019847,-1.06847604194631,
2.61145976839938));
#46836=CARTESIAN_POINT('Ctrl Pts',(0.81086559922143,-0.79477268400085,2.70413458403223));
#46837=CARTESIAN_POINT('Ctrl Pts',(0.78527553329063,-0.636309800095198,
2.76119931039013));
#46838=CARTESIAN_POINT('Ctrl Pts',(0.744792849592769,-0.31943490727716,
2.82643472239117));
#46839=CARTESIAN_POINT('Ctrl Pts',(0.728145602864073,-0.158333333333333,
2.85243807310469));
#46840=CARTESIAN_POINT('Ctrl Pts',(0.702967196216689,0.158333333333335,
2.84817008535361));
#46841=CARTESIAN_POINT('Ctrl Pts',(0.694751325057873,0.319434907277168,
2.81794370669857));
#46842=CARTESIAN_POINT('Ctrl Pts',(0.68330518681814,0.636309800095207,2.74392313105902));
#46843=CARTESIAN_POINT('Ctrl Pts',(0.680785537148619,0.794772684000843,
2.68225136282805));
#46844=CARTESIAN_POINT('Ctrl Pts',(0.682816849716337,1.06847604194529,2.58167296327534));
#46845=CARTESIAN_POINT('Ctrl Pts',(0.685764246691761,1.18514270861212,2.53527594870165));
#46846=CARTESIAN_POINT('Ctrl Pts',(0.690779760699591,1.30000000000051,2.48601858192366));
#46847=CARTESIAN_POINT('Ctrl Pts',(0.909809170319496,-1.30000000000348,
2.5462724368549));
#46848=CARTESIAN_POINT('Ctrl Pts',(0.88687330007218,-1.18514270861414,2.59673806151338));
#46849=CARTESIAN_POINT('Ctrl Pts',(0.86507605625583,-1.06847604194631,2.64307989218552));
#46850=CARTESIAN_POINT('Ctrl Pts',(0.817350517353609,-0.794772684000854,
2.74061200261849));
#46851=CARTESIAN_POINT('Ctrl Pts',(0.790156358795621,-0.636309800095199,
2.79673897566274));
#46852=CARTESIAN_POINT('Ctrl Pts',(0.748755125480717,-0.31943490727716,
2.86208266525968));
#46853=CARTESIAN_POINT('Ctrl Pts',(0.731538667378039,-0.158333333333333,
2.8865780598512));
#46854=CARTESIAN_POINT('Ctrl Pts',(0.707194541717449,0.158333333333335,
2.8823638986463));
#46855=CARTESIAN_POINT('Ctrl Pts',(0.700573425945651,0.319434907277167,
2.8537436091181));
#46856=CARTESIAN_POINT('Ctrl Pts',(0.691355618609777,0.636309800095207,
2.77963414761548));
#46857=CARTESIAN_POINT('Ctrl Pts',(0.691549177966722,0.794772684000843,
2.71882567537351));
#46858=CARTESIAN_POINT('Ctrl Pts',(0.693130508207208,1.06847604194529,2.61330408130346));
#46859=CARTESIAN_POINT('Ctrl Pts',(0.695036894474795,1.18514270861212,2.56351974022004));
#46860=CARTESIAN_POINT('Ctrl Pts',(0.698165167742923,1.30000000000051,2.50962744616575));
#46861=CARTESIAN_POINT('Ctrl Pts',(0.915082652483778,-1.30000000000348,
2.57870764115414));
#46862=CARTESIAN_POINT('Ctrl Pts',(0.892766917159951,-1.18514270861414,
2.63548079278448));
#46863=CARTESIAN_POINT('Ctrl Pts',(0.871247728879639,-1.06847604194631,
2.68642481038588));
#46864=CARTESIAN_POINT('Ctrl Pts',(0.823374282072721,-0.794772684000852,
2.79064921663921));
#46865=CARTESIAN_POINT('Ctrl Pts',(0.794677218926977,-0.636309800095197,
2.84550780327277));
#46866=CARTESIAN_POINT('Ctrl Pts',(0.752438118028174,-0.319434907277159,
2.9110027516138));
#46867=CARTESIAN_POINT('Ctrl Pts',(0.734524839113296,-0.158333333333332,
2.93339028932226));
#46868=CARTESIAN_POINT('Ctrl Pts',(0.711293802042359,0.158333333333334,
2.92927477868809));
#46869=CARTESIAN_POINT('Ctrl Pts',(0.70705880736915,0.319434907277168,2.90292244672223));
#46870=CARTESIAN_POINT('Ctrl Pts',(0.69977244719163,0.636309800095207,2.82873750113844));
#46871=CARTESIAN_POINT('Ctrl Pts',(0.700527288995702,0.794772684000841,
2.76912992220276));
#46872=CARTESIAN_POINT('Ctrl Pts',(0.702602766285981,1.06847604194528,2.65682156556838));
#46873=CARTESIAN_POINT('Ctrl Pts',(0.704531974766086,1.18514270861212,2.60237895529294));
#46874=CARTESIAN_POINT('Ctrl Pts',(0.707491994511347,1.30000000000051,2.54210786089436));
#46875=CARTESIAN_POINT('Ctrl Pts',(0.920469044817724,-1.30000000000348,
2.60822457195483));
#46876=CARTESIAN_POINT('Ctrl Pts',(0.898301433057237,-1.18514270861414,
2.6706818179568));
#46877=CARTESIAN_POINT('Ctrl Pts',(0.876625832255922,-1.06847604194631,
2.72576141099587));
#46878=CARTESIAN_POINT('Ctrl Pts',(0.827687501958213,-0.79477268400085,
2.83596243531162));
#46879=CARTESIAN_POINT('Ctrl Pts',(0.796999851289934,-0.636309800095195,
2.88958634448643));
#46880=CARTESIAN_POINT('Ctrl Pts',(0.753217519511882,-0.319434907277158,
2.95515815043732));
#46881=CARTESIAN_POINT('Ctrl Pts',(0.734354418192122,-0.158333333333332,
2.97563582202854));
#46882=CARTESIAN_POINT('Ctrl Pts',(0.711895970281559,0.158333333333334,
2.9716282579602));
#46883=CARTESIAN_POINT('Ctrl Pts',(0.709267921403271,0.319434907277166,
2.94735133204311));
#46884=CARTESIAN_POINT('Ctrl Pts',(0.705333696056776,0.636309800095204,
2.87319209469255));
#46885=CARTESIAN_POINT('Ctrl Pts',(0.710332355477971,0.794772684000837,
2.81480235774102));
#46886=CARTESIAN_POINT('Ctrl Pts',(0.71340381078195,1.06847604194528,2.69640362606351));
#46887=CARTESIAN_POINT('Ctrl Pts',(0.714828087227485,1.18514270861212,2.63774427434602));
#46888=CARTESIAN_POINT('Ctrl Pts',(0.716347120926098,1.30000000000051,2.57167599474888));
#46889=CARTESIAN_POINT('Ctrl Pts',(0.923992559503498,-1.30000000000348,
2.62890061695326));
#46890=CARTESIAN_POINT('Ctrl Pts',(0.901881354947266,-1.18514270861414,
2.69535387068794));
#46891=CARTESIAN_POINT('Ctrl Pts',(0.879974827805498,-1.06847604194631,
2.75333043280351));
#46892=CARTESIAN_POINT('Ctrl Pts',(0.829839213495544,-0.794772684000849,
2.86768503606482));
#46893=CARTESIAN_POINT('Ctrl Pts',(0.796781640694724,-0.636309800095195,
2.92033187439359));
#46894=CARTESIAN_POINT('Ctrl Pts',(0.752080256174901,-0.319434907277158,
2.98595958471202));
#46895=CARTESIAN_POINT('Ctrl Pts',(0.733844807360486,-0.158333333333332,
3.0052046640331));
#46896=CARTESIAN_POINT('Ctrl Pts',(0.712257063199493,0.158333333333334,
3.00131366662896));
#46897=CARTESIAN_POINT('Ctrl Pts',(0.710466878898138,0.319434907277167,
2.97846998365214));
#46898=CARTESIAN_POINT('Ctrl Pts',(0.708013675207788,0.636309800095205,
2.90432100677015));
#46899=CARTESIAN_POINT('Ctrl Pts',(0.714365401162632,0.794772684000839,
2.84677382123667));
#46900=CARTESIAN_POINT('Ctrl Pts',(0.718052883454901,1.06847604194528,2.7240992429047));
#46901=CARTESIAN_POINT('Ctrl Pts',(0.719470360074824,1.18514270861212,2.66248264767173));
#46902=CARTESIAN_POINT('Ctrl Pts',(0.72070913886503,1.3000000000005,2.59235073662463));
#46903=CARTESIAN_POINT('Ctrl Pts',(0.92529189916072,-1.30000000000348,2.63775451220662));
#46904=CARTESIAN_POINT('Ctrl Pts',(0.90286710161616,-1.18514270861414,2.70590656695599));
#46905=CARTESIAN_POINT('Ctrl Pts',(0.880718520683462,-1.06847604194631,
2.76512493099013));
#46906=CARTESIAN_POINT('Ctrl Pts',(0.830188983551121,-0.794772684000851,
2.88129258577059));
#46907=CARTESIAN_POINT('Ctrl Pts',(0.797251592334188,-0.636309800095197,
2.93363499971855));
#46908=CARTESIAN_POINT('Ctrl Pts',(0.752160119240198,-0.319434907277159,
2.99927731465237));
#46909=CARTESIAN_POINT('Ctrl Pts',(0.733263218353926,-0.158333333333332,
3.01787138809224));
#46910=CARTESIAN_POINT('Ctrl Pts',(0.711685603093662,0.158333333333334,
3.01399236569876));
#46911=CARTESIAN_POINT('Ctrl Pts',(0.710356982649902,0.319434907277167,
2.99180138145779));
#46912=CARTESIAN_POINT('Ctrl Pts',(0.708742289116701,0.636309800095206,
2.91768313620638));
#46913=CARTESIAN_POINT('Ctrl Pts',(0.71597300740823,0.794772684000841,2.86052978046723));
#46914=CARTESIAN_POINT('Ctrl Pts',(0.720292134275874,1.06847604194528,2.73602437620757));
#46915=CARTESIAN_POINT('Ctrl Pts',(0.721868578912404,1.18514270861212,2.6731325281192));
#46916=CARTESIAN_POINT('Ctrl Pts',(0.723151878203884,1.30000000000051,2.60124260806661));
#46917=CARTESIAN_POINT('Ctrl Pts',(0.926611318159751,-1.30000000000348,
2.64948665818269));
#46918=CARTESIAN_POINT('Ctrl Pts',(0.90445282821427,-1.18514270861414,2.71989773316588));
#46919=CARTESIAN_POINT('Ctrl Pts',(0.882280853198343,-1.06847604194631,
2.78074250462087));
#46920=CARTESIAN_POINT('Ctrl Pts',(0.831028002213023,-0.794772684000853,
2.89920602375347));
#46921=CARTESIAN_POINT('Ctrl Pts',(0.796094523755093,-0.636309800095197,
2.95088445224024));
#46922=CARTESIAN_POINT('Ctrl Pts',(0.750381762823946,-0.319434907277159,
3.01654690138816));
#46923=CARTESIAN_POINT('Ctrl Pts',(0.732176691888254,-0.158333333333332,
3.0345337535851));
#46924=CARTESIAN_POINT('Ctrl Pts',(0.711294701270189,0.158333333333334,
3.03075995137096));
#46925=CARTESIAN_POINT('Ctrl Pts',(0.710351572107801,0.319434907277166,
3.00935787644432));
#46926=CARTESIAN_POINT('Ctrl Pts',(0.709997615251027,0.636309800095205,
2.93527806331773));
#46927=CARTESIAN_POINT('Ctrl Pts',(0.718617994233884,0.794772684000841,
2.87864263863507));
#46928=CARTESIAN_POINT('Ctrl Pts',(0.723706711382351,1.06847604194528,2.75176911793317));
#46929=CARTESIAN_POINT('Ctrl Pts',(0.725391320126886,1.18514270861212,2.68722624494357));
#46930=CARTESIAN_POINT('Ctrl Pts',(0.726557820517936,1.3000000000005,2.61305934494899));
#46931=CARTESIAN_POINT('Ctrl Pts',(0.928513761894011,-1.30000000000348,
2.66427335298741));
#46932=CARTESIAN_POINT('Ctrl Pts',(0.90608019642325,-1.18514270861414,2.73763274798547));
#46933=CARTESIAN_POINT('Ctrl Pts',(0.883520193103324,-1.06847604194631,
2.80061671768325));
#46934=CARTESIAN_POINT('Ctrl Pts',(0.831109975596004,-0.794772684000851,
2.92215297954406));
#46935=CARTESIAN_POINT('Ctrl Pts',(0.794162608436584,-0.636309800095197,
2.9730779634235));
#46936=CARTESIAN_POINT('Ctrl Pts',(0.748684445248217,-0.31943490727716,
3.03888165819878));
#46937=CARTESIAN_POINT('Ctrl Pts',(0.733032893716133,-0.158333333333333,
3.05616629395804));
#46938=CARTESIAN_POINT('Ctrl Pts',(0.712915773366991,0.158333333333335,
3.05250175010369));
#46939=CARTESIAN_POINT('Ctrl Pts',(0.710588786918305,0.319434907277168,
3.03197974048681));
#46940=CARTESIAN_POINT('Ctrl Pts',(0.710733686134875,0.636309800095207,
2.95784151921007));
#46941=CARTESIAN_POINT('Ctrl Pts',(0.721034800362429,0.794772684000843,
2.90187893722154));
#46942=CARTESIAN_POINT('Ctrl Pts',(0.726882715325336,1.06847604194528,2.77183338838692));
#46943=CARTESIAN_POINT('Ctrl Pts',(0.728687491821999,1.18514270861212,2.70509393505239));
#46944=CARTESIAN_POINT('Ctrl Pts',(0.729765699114486,1.30000000000051,2.62790692781138));
#46945=CARTESIAN_POINT('Ctrl Pts',(0.930286002589785,-1.30000000000348,
2.67890363858943));
#46946=CARTESIAN_POINT('Ctrl Pts',(0.907045931711774,-1.18514270861414,
2.75486940600399));
#46947=CARTESIAN_POINT('Ctrl Pts',(0.884058946872757,-1.06847604194631,
2.8197689238864));
#46948=CARTESIAN_POINT('Ctrl Pts',(0.831539092744121,-0.794772684000853,
2.94413454308327));
#46949=CARTESIAN_POINT('Ctrl Pts',(0.796025953341132,-0.636309800095196,
2.99465196005428));
#46950=CARTESIAN_POINT('Ctrl Pts',(0.751325518317324,-0.319434907277158,
3.0605719012789));
#46951=CARTESIAN_POINT('Ctrl Pts',(0.736156135148362,-0.158333333333332,
3.07698411601015));
#46952=CARTESIAN_POINT('Ctrl Pts',(0.715522674806847,0.158333333333334,
3.07328619511169));
#46953=CARTESIAN_POINT('Ctrl Pts',(0.711372020014341,0.319434907277167,
3.05352879382717));
#46954=CARTESIAN_POINT('Ctrl Pts',(0.711368235162324,0.636309800095206,
2.9793579595281));
#46955=CARTESIAN_POINT('Ctrl Pts',(0.723265628623222,0.794772684000839,
2.92412391234324));
#46956=CARTESIAN_POINT('Ctrl Pts',(0.729702122581364,1.06847604194528,2.79125656303106));
#46957=CARTESIAN_POINT('Ctrl Pts',(0.731596041924747,1.18514270861212,2.72253590444958));
#46958=CARTESIAN_POINT('Ctrl Pts',(0.732597760872638,1.30000000000051,2.64260793958341));
#46959=CARTESIAN_POINT('Ctrl Pts',(0.9317290646797,-1.30000000000348,2.69655002042453));
#46960=CARTESIAN_POINT('Ctrl Pts',(0.907290115516676,-1.18514270861414,
2.77603993473538));
#46961=CARTESIAN_POINT('Ctrl Pts',(0.883846376138303,-1.06847604194631,
2.84357938770473));
#46962=CARTESIAN_POINT('Ctrl Pts',(0.831985781964135,-0.794772684000852,
2.97200107890404));
#46963=CARTESIAN_POINT('Ctrl Pts',(0.799949875653835,-0.636309800095197,
3.022356802163));
#46964=CARTESIAN_POINT('Ctrl Pts',(0.757395319589324,-0.319434907277159,
3.08868693309944));
#46965=CARTESIAN_POINT('Ctrl Pts',(0.742746847031083,-0.158333333333332,
3.10388657941746));
#46966=CARTESIAN_POINT('Ctrl Pts',(0.722185979795504,0.158333333333334,
3.10021804189515));
#46967=CARTESIAN_POINT('Ctrl Pts',(0.717232947701702,0.319434907277167,
3.08168140192397));
#46968=CARTESIAN_POINT('Ctrl Pts',(0.715952345132643,0.636309800095206,
3.00720339320853));
#46969=CARTESIAN_POINT('Ctrl Pts',(0.726294270879949,0.794772684000839,
2.95232337348871));
#46970=CARTESIAN_POINT('Ctrl Pts',(0.732256870087518,1.06847604194528,2.81536627845052));
#46971=CARTESIAN_POINT('Ctrl Pts',(0.734269534690587,1.18514270861212,2.74393616160032));
#46972=CARTESIAN_POINT('Ctrl Pts',(0.735713875635842,1.30000000000051,2.66035957958145));
#46973=CARTESIAN_POINT('Ctrl Pts',(0.932811379691018,-1.30000000000348,
2.70856623744797));
#46974=CARTESIAN_POINT('Ctrl Pts',(0.906248352880216,-1.18514270861414,
2.79031303912099));
#46975=CARTESIAN_POINT('Ctrl Pts',(0.882011643626692,-1.06847604194631,
2.85950209300221));
#46976=CARTESIAN_POINT('Ctrl Pts',(0.8313942556498,-0.794772684000851,2.99033173912196));
#46977=CARTESIAN_POINT('Ctrl Pts',(0.805863671216798,-0.636309800095197,
3.04032716132039));
#46978=CARTESIAN_POINT('Ctrl Pts',(0.76676614190522,-0.319434907277159,
3.10658683790933));
#46979=CARTESIAN_POINT('Ctrl Pts',(0.751993950076098,-0.158333333333332,
3.12072515293865));
#46980=CARTESIAN_POINT('Ctrl Pts',(0.731604230888438,0.158333333333334,
3.11703748018433));
#46981=CARTESIAN_POINT('Ctrl Pts',(0.72682424539096,0.319434907277167,3.0994670379522));
#46982=CARTESIAN_POINT('Ctrl Pts',(0.722683372359811,0.636309800095206,
3.02517530959544));
#46983=CARTESIAN_POINT('Ctrl Pts',(0.727550431506878,0.79477268400084,2.9710284197423));
#46984=CARTESIAN_POINT('Ctrl Pts',(0.732217053984722,1.06847604194528,2.83164616354321));
#46985=CARTESIAN_POINT('Ctrl Pts',(0.734729140509333,1.18514270861212,2.75847136298333));
#46986=CARTESIAN_POINT('Ctrl Pts',(0.7377333056033,1.30000000000051,2.67245517595061));
#46987=CARTESIAN_POINT('Ctrl Pts',(0.936125406440882,-1.30000000000348,
2.71650429949854));
#46988=CARTESIAN_POINT('Ctrl Pts',(0.909492919286885,-1.18514270861414,
2.79800958197354));
#46989=CARTESIAN_POINT('Ctrl Pts',(0.88553280170208,-1.06847604194631,2.86699266749395));
#46990=CARTESIAN_POINT('Ctrl Pts',(0.836353845186883,-0.794772684000851,
2.99742861504232));
#46991=CARTESIAN_POINT('Ctrl Pts',(0.813383183475108,-0.636309800095197,
3.04725124007732));
#46992=CARTESIAN_POINT('Ctrl Pts',(0.77596280188267,-0.319434907277159,
3.11333278083123));
#46993=CARTESIAN_POINT('Ctrl Pts',(0.761169784372622,-0.158333333333332,
3.12751912120358));
#46994=CARTESIAN_POINT('Ctrl Pts',(0.74101228662764,0.158333333333334,3.12378496929258));
#46995=CARTESIAN_POINT('Ctrl Pts',(0.736764158587383,0.319434907277167,
3.10609354911359));
#46996=CARTESIAN_POINT('Ctrl Pts',(0.730851239620766,0.636309800095206,
3.03193920640198));
#46997=CARTESIAN_POINT('Ctrl Pts',(0.732075357025827,0.79477268400084,2.97800571764298));
#46998=CARTESIAN_POINT('Ctrl Pts',(0.735457044102352,1.06847604194528,2.83902298122212));
#46999=CARTESIAN_POINT('Ctrl Pts',(0.738012470505655,1.18514270861212,2.76605409464577));
#47000=CARTESIAN_POINT('Ctrl Pts',(0.741659516280687,1.30000000000051,2.68027679827178));
#47001=CARTESIAN_POINT('Ctrl Pts',(0.936125406440075,-1.3,2.71650429950101));
#47002=CARTESIAN_POINT('Ctrl Pts',(0.909492919286401,-1.18514270861178,
2.79800958197493));
#47003=CARTESIAN_POINT('Ctrl Pts',(0.885532801701865,-1.06847604194512,
2.86699266749452));
#47004=CARTESIAN_POINT('Ctrl Pts',(0.836353845186883,-0.794772684000851,
2.99742861504232));
#47005=CARTESIAN_POINT('Ctrl Pts',(0.813383183475108,-0.636309800095197,
3.04725124007732));
#47006=CARTESIAN_POINT('Ctrl Pts',(0.77596280188267,-0.319434907277159,
3.11333278083123));
#47007=CARTESIAN_POINT('Ctrl Pts',(0.761169784372621,-0.158333333333332,
3.12751912120358));
#47008=CARTESIAN_POINT('Ctrl Pts',(0.74101228662764,0.158333333333334,3.12378496929258));
#47009=CARTESIAN_POINT('Ctrl Pts',(0.736764158587383,0.319434907277167,
3.10609354911359));
#47010=CARTESIAN_POINT('Ctrl Pts',(0.730851239620766,0.636309800095206,
3.03193920640198));
#47011=CARTESIAN_POINT('Ctrl Pts',(0.732075357025827,0.79477268400084,2.97800571764298));
#47012=CARTESIAN_POINT('Ctrl Pts',(0.73545704410235,1.06847604194511,2.8390229812222));
#47013=CARTESIAN_POINT('Ctrl Pts',(0.738012470505647,1.18514270861178,2.76605409464598));
#47014=CARTESIAN_POINT('Ctrl Pts',(0.74165951628067,1.3,2.68027679827216));
#47015=CARTESIAN_POINT('',(0.819062040271282,-1.2,2.31823419506971));
#47016=CARTESIAN_POINT('Ctrl Pts',(0.819062040271282,-1.2,2.31823419506971));
#47017=CARTESIAN_POINT('Ctrl Pts',(0.826817460709897,-1.21221394250375,
2.33192005968323));
#47018=CARTESIAN_POINT('Ctrl Pts',(0.839321576150835,-1.2301813580624,2.35228839172571));
#47019=CARTESIAN_POINT('Ctrl Pts',(0.860218448319171,-1.26364575297284,
2.38993774624693));
#47020=CARTESIAN_POINT('Ctrl Pts',(0.87185017021258,-1.2816915450181,2.41037451072659));
#47021=CARTESIAN_POINT('Ctrl Pts',(0.882693729841481,-1.30000000000349,
2.43100096673687));
#47022=CARTESIAN_POINT('',(0.664237964398142,-0.653834841336346,2.29476932996546));
#47023=CARTESIAN_POINT('Ctrl Pts',(0.664237964461389,-0.653834841321562,
2.29476932993277));
#47024=CARTESIAN_POINT('Ctrl Pts',(0.680825402116955,-0.719831522668225,
2.29701550479488));
#47025=CARTESIAN_POINT('Ctrl Pts',(0.694147737514797,-0.767178700652001,
2.2988870429438));
#47026=CARTESIAN_POINT('Ctrl Pts',(0.744612933014617,-0.949587838682991,
2.30619873464169));
#47027=CARTESIAN_POINT('Ctrl Pts',(0.774822021425007,-1.05662877212074,
2.31081161038503));
#47028=CARTESIAN_POINT('Ctrl Pts',(0.819062040271282,-1.2,2.31823419506971));
#47029=CARTESIAN_POINT('',(0.525742999964552,0.653834841531101,2.27799895388184));
#47030=CARTESIAN_POINT('Ctrl Pts',(0.525742999964552,0.6538348415311,2.27799895388184));
#47031=CARTESIAN_POINT('Ctrl Pts',(0.539185395144359,0.575762922599882,
2.31746185242062));
#47032=CARTESIAN_POINT('Ctrl Pts',(0.551466169169658,0.4937141636101,2.35040598822811));
#47033=CARTESIAN_POINT('Ctrl Pts',(0.571107869262371,0.337918064895967,
2.39711660814527));
#47034=CARTESIAN_POINT('Ctrl Pts',(0.579212684940256,0.265429240963003,
2.41309282046306));
#47035=CARTESIAN_POINT('Ctrl Pts',(0.593808443755668,0.129513007362985,
2.43255632813054));
#47036=CARTESIAN_POINT('Ctrl Pts',(0.600326349577118,0.0665349388579791,
2.43753385439801));
#47037=CARTESIAN_POINT('Ctrl Pts',(0.613439021868735,-0.0594336898450758,
2.4394973403484));
#47038=CARTESIAN_POINT('Ctrl Pts',(0.620111209962176,-0.122553013099034,
2.43651084370931));
#47039=CARTESIAN_POINT('Ctrl Pts',(0.633872071790792,-0.259894286834156,
2.42107710019218));
#47040=CARTESIAN_POINT('Ctrl Pts',(0.64081030202418,-0.333782902442558,
2.40697833921996));
#47041=CARTESIAN_POINT('Ctrl Pts',(0.653754957792595,-0.491517546675328,
2.36393127566722));
#47042=CARTESIAN_POINT('Ctrl Pts',(0.65977017879487,-0.574921333471004,
2.33273270890711));
#47043=CARTESIAN_POINT('Ctrl Pts',(0.664237964504258,-0.653834841358084,
2.29476933002314));
#47044=CARTESIAN_POINT('',(0.59761333344196,1.2,2.28620734018087));
#47045=CARTESIAN_POINT('Ctrl Pts',(0.597613333441959,1.2,2.28620734018087));
#47046=CARTESIAN_POINT('Ctrl Pts',(0.578803584943033,1.09907813786244,2.28391970672137));
#47047=CARTESIAN_POINT('Ctrl Pts',(0.563616863067985,0.997456289320577,
2.28217371941591));
#47048=CARTESIAN_POINT('Ctrl Pts',(0.53349441673388,0.766998566051729,2.27880400694723));
#47049=CARTESIAN_POINT('Ctrl Pts',(0.529155746207933,0.699729784093127,
2.27836348599618));
#47050=CARTESIAN_POINT('Ctrl Pts',(0.525742999964552,0.653834841531101,
2.27799895388184));
#47051=CARTESIAN_POINT('Ctrl Pts',(0.659051978146154,1.3,2.39498694173454));
#47052=CARTESIAN_POINT('Ctrl Pts',(0.649466552315287,1.28312826533509,2.37664251562972));
#47053=CARTESIAN_POINT('Ctrl Pts',(0.639075664739576,1.26651241391695,2.35849331479684));
#47054=CARTESIAN_POINT('Ctrl Pts',(0.622309019792689,1.23888116128521,2.32846173095479));
#47055=CARTESIAN_POINT('Ctrl Pts',(0.620849725903724,1.23596041607477,2.325331181624));
#47056=CARTESIAN_POINT('Ctrl Pts',(0.608663819665247,1.21698970713212,2.30467956529489));
#47057=CARTESIAN_POINT('Ctrl Pts',(0.603301253934286,1.20843659167084,2.29539785940356));
#47058=CARTESIAN_POINT('Ctrl Pts',(0.597613333441959,1.2,2.28620734018087));
#47059=CARTESIAN_POINT('Ctrl Pts',(0.936125406440075,-1.3,2.71650429950101));
#47060=CARTESIAN_POINT('Ctrl Pts',(0.909492919286401,-1.18514270861178,
2.79800958197493));
#47061=CARTESIAN_POINT('Ctrl Pts',(0.885532801701865,-1.06847604194512,
2.86699266749452));
#47062=CARTESIAN_POINT('Ctrl Pts',(0.836353845186883,-0.794772684000851,
2.99742861504232));
#47063=CARTESIAN_POINT('Ctrl Pts',(0.813383183475108,-0.636309800095197,
3.04725124007732));
#47064=CARTESIAN_POINT('Ctrl Pts',(0.77596280188267,-0.319434907277159,
3.11333278083123));
#47065=CARTESIAN_POINT('Ctrl Pts',(0.761169784372622,-0.158333333333332,
3.12751912120358));
#47066=CARTESIAN_POINT('Ctrl Pts',(0.74101228662764,0.158333333333335,3.12378496929258));
#47067=CARTESIAN_POINT('Ctrl Pts',(0.736764158587383,0.319434907277167,
3.10609354911359));
#47068=CARTESIAN_POINT('Ctrl Pts',(0.730851239620766,0.636309800095206,
3.03193920640198));
#47069=CARTESIAN_POINT('Ctrl Pts',(0.732075357025826,0.79477268400084,2.97800571764298));
#47070=CARTESIAN_POINT('Ctrl Pts',(0.73545704410235,1.06847604194511,2.83902298122221));
#47071=CARTESIAN_POINT('Ctrl Pts',(0.738012470505647,1.18514270861178,2.76605409464599));
#47072=CARTESIAN_POINT('Ctrl Pts',(0.74165951628067,1.3,2.68027679827216));
#47073=CARTESIAN_POINT('Ctrl Pts',(1.01101605778904,-1.3,2.73412529876815));
#47074=CARTESIAN_POINT('Ctrl Pts',(0.982742057194053,-1.18514270861178,
2.81507710262639));
#47075=CARTESIAN_POINT('Ctrl Pts',(0.95765377154039,-1.06847604194512,2.88363241978539));
#47076=CARTESIAN_POINT('Ctrl Pts',(0.90705445160062,-0.794772684000851,
3.01337055268305));
#47077=CARTESIAN_POINT('Ctrl Pts',(0.884801197368707,-0.636309800095197,
3.06317516506461));
#47078=CARTESIAN_POINT('Ctrl Pts',(0.847999940077956,-0.319434907277159,
3.12900897961302));
#47079=CARTESIAN_POINT('Ctrl Pts',(0.834445726094755,-0.158333333333332,
3.14327788892968));
#47080=CARTESIAN_POINT('Ctrl Pts',(0.814362858626306,0.158333333333335,
3.13919262917263));
#47081=CARTESIAN_POINT('Ctrl Pts',(0.808949443435951,0.319434907277167,
3.12107277268973));
#47082=CARTESIAN_POINT('Ctrl Pts',(0.802571685601039,0.636309800095206,
3.04644030028823));
#47083=CARTESIAN_POINT('Ctrl Pts',(0.803147745067787,0.79477268400084,2.99219856024142));
#47084=CARTESIAN_POINT('Ctrl Pts',(0.808110825487516,1.06847604194511,2.85315605226807));
#47085=CARTESIAN_POINT('Ctrl Pts',(0.811870873772817,1.18514270861178,2.78025524714239));
#47086=CARTESIAN_POINT('Ctrl Pts',(0.817242636729975,1.3,2.69463998655998));
#47087=CARTESIAN_POINT('Ctrl Pts',(1.08590670913801,-1.3,2.7517462980353));
#47088=CARTESIAN_POINT('Ctrl Pts',(1.05599119510171,-1.18514270861178,2.83214462327784));
#47089=CARTESIAN_POINT('Ctrl Pts',(1.02977474137891,-1.06847604194512,2.90027217207626));
#47090=CARTESIAN_POINT('Ctrl Pts',(0.977755058014356,-0.794772684000851,
3.02931249032378));
#47091=CARTESIAN_POINT('Ctrl Pts',(0.956219211262305,-0.636309800095197,
3.07909909005189));
#47092=CARTESIAN_POINT('Ctrl Pts',(0.920037078273242,-0.319434907277159,
3.1446851783948));
#47093=CARTESIAN_POINT('Ctrl Pts',(0.907721667816889,-0.158333333333332,
3.15903665665579));
#47094=CARTESIAN_POINT('Ctrl Pts',(0.887713430624972,0.158333333333335,
3.15460028905268));
#47095=CARTESIAN_POINT('Ctrl Pts',(0.881134728284519,0.319434907277167,
3.13605199626586));
#47096=CARTESIAN_POINT('Ctrl Pts',(0.874292131581311,0.636309800095206,
3.06094139417447));
#47097=CARTESIAN_POINT('Ctrl Pts',(0.874220133109747,0.79477268400084,3.00639140283986));
#47098=CARTESIAN_POINT('Ctrl Pts',(0.880764606872681,1.06847604194511,2.86728912331394));
#47099=CARTESIAN_POINT('Ctrl Pts',(0.885729277039987,1.18514270861178,2.79445639963879));
#47100=CARTESIAN_POINT('Ctrl Pts',(0.892825757179279,1.3,2.70900317484779));
#47101=CARTESIAN_POINT('Ctrl Pts',(1.16079736048698,-1.3,2.76936729730244));
#47102=CARTESIAN_POINT('Ctrl Pts',(1.12924033300936,-1.18514270861178,2.84921214392929));
#47103=CARTESIAN_POINT('Ctrl Pts',(1.10189571121744,-1.06847604194512,2.91691192436713));
#47104=CARTESIAN_POINT('Ctrl Pts',(1.04845566442809,-0.794772684000851,
3.04525442796451));
#47105=CARTESIAN_POINT('Ctrl Pts',(1.0276372251559,-0.636309800095197,3.09502301503918));
#47106=CARTESIAN_POINT('Ctrl Pts',(0.992074216468528,-0.319434907277159,
3.16036137717659));
#47107=CARTESIAN_POINT('Ctrl Pts',(0.980997609539022,-0.158333333333332,
3.17479542438189));
#47108=CARTESIAN_POINT('Ctrl Pts',(0.961064002623638,0.158333333333335,
3.17000794893274));
#47109=CARTESIAN_POINT('Ctrl Pts',(0.953320013133087,0.319434907277167,
3.151031219842));
#47110=CARTESIAN_POINT('Ctrl Pts',(0.946012577561583,0.636309800095206,
3.07544248806072));
#47111=CARTESIAN_POINT('Ctrl Pts',(0.945292521151707,0.79477268400084,3.02058424543829));
#47112=CARTESIAN_POINT('Ctrl Pts',(0.953418388257846,1.06847604194511,2.88142219435981));
#47113=CARTESIAN_POINT('Ctrl Pts',(0.959587680307157,1.18514270861178,2.80865755213519));
#47114=CARTESIAN_POINT('Ctrl Pts',(0.968408877628583,1.3,2.72336636313561));
#47115=CARTESIAN_POINT('Ctrl Pts',(1.16079736048698,-1.3,2.76936729730244));
#47116=CARTESIAN_POINT('Ctrl Pts',(1.12924033300936,-1.18514270861178,2.84921214392929));
#47117=CARTESIAN_POINT('Ctrl Pts',(1.10189571121744,-1.06847604194512,2.91691192436713));
#47118=CARTESIAN_POINT('Ctrl Pts',(1.04845566442809,-0.794772684000851,
3.0452544279645));
#47119=CARTESIAN_POINT('Ctrl Pts',(1.0276372251559,-0.636309800095197,3.09502301503918));
#47120=CARTESIAN_POINT('Ctrl Pts',(0.992074216468527,-0.319434907277159,
3.16036137717659));
#47121=CARTESIAN_POINT('Ctrl Pts',(0.980997609539022,-0.158333333333332,
3.17479542438189));
#47122=CARTESIAN_POINT('Ctrl Pts',(0.961064002623638,0.158333333333334,
3.17000794893273));
#47123=CARTESIAN_POINT('Ctrl Pts',(0.953320013133086,0.319434907277167,
3.151031219842));
#47124=CARTESIAN_POINT('Ctrl Pts',(0.946012577561583,0.636309800095206,
3.07544248806072));
#47125=CARTESIAN_POINT('Ctrl Pts',(0.945292521151707,0.79477268400084,3.02058424543829));
#47126=CARTESIAN_POINT('Ctrl Pts',(0.953418388257846,1.06847604194511,2.88142219435981));
#47127=CARTESIAN_POINT('Ctrl Pts',(0.959587680307157,1.18514270861178,2.80865755213519));
#47128=CARTESIAN_POINT('Ctrl Pts',(0.968408877628583,1.3,2.72336636313561));
#47129=CARTESIAN_POINT('Ctrl Pts',(1.16079736048841,-1.30000000000522,2.76936729729881));
#47130=CARTESIAN_POINT('Ctrl Pts',(1.12924033301019,-1.18514270861532,2.84921214392724));
#47131=CARTESIAN_POINT('Ctrl Pts',(1.10189571121779,-1.06847604194691,2.91691192436629));
#47132=CARTESIAN_POINT('Ctrl Pts',(1.04845566442809,-0.794772684000851,
3.04525442796451));
#47133=CARTESIAN_POINT('Ctrl Pts',(1.0276372251559,-0.636309800095197,3.09502301503918));
#47134=CARTESIAN_POINT('Ctrl Pts',(0.992074216468527,-0.319434907277159,
3.16036137717659));
#47135=CARTESIAN_POINT('Ctrl Pts',(0.980997609539023,-0.158333333333332,
3.17479542438189));
#47136=CARTESIAN_POINT('Ctrl Pts',(0.961064002623638,0.158333333333334,
3.17000794893273));
#47137=CARTESIAN_POINT('Ctrl Pts',(0.953320013133086,0.319434907277167,
3.151031219842));
#47138=CARTESIAN_POINT('Ctrl Pts',(0.946012577561583,0.636309800095206,
3.07544248806072));
#47139=CARTESIAN_POINT('Ctrl Pts',(0.945292521151708,0.79477268400084,3.02058424543829));
#47140=CARTESIAN_POINT('Ctrl Pts',(0.953418388257849,1.06847604194517,2.88142219435978));
#47141=CARTESIAN_POINT('Ctrl Pts',(0.959587680307164,1.1851427086119,2.80865755213511));
#47142=CARTESIAN_POINT('Ctrl Pts',(0.968408877628597,1.30000000000018,2.72336636313548));
#47143=CARTESIAN_POINT('Ctrl Pts',(1.16756547281118,-1.30000000000522,2.76381882356482));
#47144=CARTESIAN_POINT('Ctrl Pts',(1.13532397902447,-1.18514270861532,2.84362042453195));
#47145=CARTESIAN_POINT('Ctrl Pts',(1.10785601152185,-1.06847604194691,2.91149068883335));
#47146=CARTESIAN_POINT('Ctrl Pts',(1.05542731230007,-0.794772684000851,
3.04072080221479));
#47147=CARTESIAN_POINT('Ctrl Pts',(1.03785006786609,-0.636309800095197,
3.09216605877564));
#47148=CARTESIAN_POINT('Ctrl Pts',(1.00385002391232,-0.319434907277159,
3.15835068498378));
#47149=CARTESIAN_POINT('Ctrl Pts',(0.992336747169056,-0.158333333333332,
3.17245788747789));
#47150=CARTESIAN_POINT('Ctrl Pts',(0.972209900186261,0.158333333333334,
3.16753349823253));
#47151=CARTESIAN_POINT('Ctrl Pts',(0.964465402249313,0.319434907277167,
3.14860911297925));
#47152=CARTESIAN_POINT('Ctrl Pts',(0.955698270375131,0.636309800095206,
3.07217548855289));
#47153=CARTESIAN_POINT('Ctrl Pts',(0.952709891127438,0.79477268400084,3.01611817350183));
#47154=CARTESIAN_POINT('Ctrl Pts',(0.959681817340558,1.06847604194517,2.87601139810055));
#47155=CARTESIAN_POINT('Ctrl Pts',(0.965682205206479,1.1851427086119,2.80294609445152));
#47156=CARTESIAN_POINT('Ctrl Pts',(0.974665092415987,1.30000000000018,2.717462518757));
#47157=CARTESIAN_POINT('Ctrl Pts',(1.17429750653259,-1.30000000000522,2.75357268161649));
#47158=CARTESIAN_POINT('Ctrl Pts',(1.14162650151079,-1.18514270861532,2.8305066317218));
#47159=CARTESIAN_POINT('Ctrl Pts',(1.11441651150372,-1.06847604194691,2.89657751787525));
#47160=CARTESIAN_POINT('Ctrl Pts',(1.0641720284043,-0.794772684000852,3.02411863144687));
#47161=CARTESIAN_POINT('Ctrl Pts',(1.05131458055589,-0.636309800095196,
3.07846805658878));
#47162=CARTESIAN_POINT('Ctrl Pts',(1.0198646696171,-0.319434907277158,3.14599143412024));
#47163=CARTESIAN_POINT('Ctrl Pts',(1.00780392282228,-0.158333333333332,
3.16091515929002));
#47164=CARTESIAN_POINT('Ctrl Pts',(0.987525874605585,0.158333333333335,
3.15590178731436));
#47165=CARTESIAN_POINT('Ctrl Pts',(0.980318225717366,0.319434907277168,
3.13605041188448));
#47166=CARTESIAN_POINT('Ctrl Pts',(0.968406622993036,0.636309800095207,
3.0581405476509));
#47167=CARTESIAN_POINT('Ctrl Pts',(0.959600753467649,0.794772684000839,
2.99910157701068));
#47168=CARTESIAN_POINT('Ctrl Pts',(0.964457436413564,1.06847604194517,2.86069580646051));
#47169=CARTESIAN_POINT('Ctrl Pts',(0.970516793992365,1.18514270861189,2.78946635876449));
#47170=CARTESIAN_POINT('Ctrl Pts',(0.980533231060517,1.30000000000018,2.70691819300439));
#47171=CARTESIAN_POINT('Ctrl Pts',(1.18440293491058,-1.30000000000522,2.73864158445463));
#47172=CARTESIAN_POINT('Ctrl Pts',(1.15281893584074,-1.18514270861532,2.8120698416044));
#47173=CARTESIAN_POINT('Ctrl Pts',(1.12660451412146,-1.06847604194691,2.87562143340008));
#47174=CARTESIAN_POINT('Ctrl Pts',(1.07844875363333,-0.794772684000853,
2.99962125111139));
#47175=CARTESIAN_POINT('Ctrl Pts',(1.06684517117874,-0.636309800095195,
3.05491694960946));
#47176=CARTESIAN_POINT('Ctrl Pts',(1.03666116289866,-0.319434907277157,
3.12266967613995));
#47177=CARTESIAN_POINT('Ctrl Pts',(1.02482746060559,-0.158333333333332,
3.13902915190023));
#47178=CARTESIAN_POINT('Ctrl Pts',(1.00444286620191,0.158333333333334,3.13400464966217));
#47179=CARTESIAN_POINT('Ctrl Pts',(0.997213961942221,0.319434907277168,
3.11282604408903));
#47180=CARTESIAN_POINT('Ctrl Pts',(0.983183225095408,0.636309800095206,
3.03442043943294));
#47181=CARTESIAN_POINT('Ctrl Pts',(0.97133893520286,0.794772684000838,2.97384041811216));
#47182=CARTESIAN_POINT('Ctrl Pts',(0.973945325811959,1.06847604194517,2.83886592421529));
#47183=CARTESIAN_POINT('Ctrl Pts',(0.979334457355884,1.18514270861189,2.77022574197491));
#47184=CARTESIAN_POINT('Ctrl Pts',(0.988984510525345,1.30000000000018,2.69137083460419));
#47185=CARTESIAN_POINT('Ctrl Pts',(1.19282025714432,-1.30000000000522,2.72628875413115));
#47186=CARTESIAN_POINT('Ctrl Pts',(1.16240804411813,-1.18514270861532,2.79721826438278));
#47187=CARTESIAN_POINT('Ctrl Pts',(1.13692060833745,-1.06847604194691,2.85890943556789));
#47188=CARTESIAN_POINT('Ctrl Pts',(1.08941675357591,-0.794772684000851,
2.98008597091395));
#47189=CARTESIAN_POINT('Ctrl Pts',(1.0761430165978,-0.636309800095196,3.03543477422358));
#47190=CARTESIAN_POINT('Ctrl Pts',(1.04619263381479,-0.319434907277158,
3.10325000382581));
#47191=CARTESIAN_POINT('Ctrl Pts',(1.03574336889857,-0.158333333333332,
3.12107111876852));
#47192=CARTESIAN_POINT('Ctrl Pts',(1.0159100403865,0.158333333333334,3.11624401321292));
#47193=CARTESIAN_POINT('Ctrl Pts',(1.00867847609951,0.319434907277168,3.09407856463005));
#47194=CARTESIAN_POINT('Ctrl Pts',(0.993845310643403,0.636309800095207,
3.01544749694316));
#47195=CARTESIAN_POINT('Ctrl Pts',(0.980641741294821,0.794772684000839,
2.95384890499302));
#47196=CARTESIAN_POINT('Ctrl Pts',(0.982193099836836,1.06847604194517,2.82152975406996));
#47197=CARTESIAN_POINT('Ctrl Pts',(0.987236437588956,1.18514270861189,2.7548438908858));
#47198=CARTESIAN_POINT('Ctrl Pts',(0.996651587463857,1.30000000000018,2.67874822204431));
#47199=CARTESIAN_POINT('Ctrl Pts',(1.20387629867497,-1.30000000000522,2.71172082726954));
#47200=CARTESIAN_POINT('Ctrl Pts',(1.17507593415048,-1.18514270861532,2.77943672157987));
#47201=CARTESIAN_POINT('Ctrl Pts',(1.15053427987609,-1.06847604194691,2.83869134085797));
#47202=CARTESIAN_POINT('Ctrl Pts',(1.10367662159133,-0.794772684000853,
2.95603412723863));
#47203=CARTESIAN_POINT('Ctrl Pts',(1.08806112252454,-0.636309800095197,
3.01122675713547));
#47204=CARTESIAN_POINT('Ctrl Pts',(1.05741252960008,-0.319434907277159,
3.07866763728465));
#47205=CARTESIAN_POINT('Ctrl Pts',(1.0479864980603,-0.158333333333333,3.09808593381759));
#47206=CARTESIAN_POINT('Ctrl Pts',(1.02708751229622,0.158333333333335,3.09295520022724));
#47207=CARTESIAN_POINT('Ctrl Pts',(1.0171674141675,0.319434907277168,3.06873742908771));
#47208=CARTESIAN_POINT('Ctrl Pts',(1.00208322181011,0.636309800095208,2.99017086334158));
#47209=CARTESIAN_POINT('Ctrl Pts',(0.991947200773414,0.794772684000841,
2.92887248736516));
#47210=CARTESIAN_POINT('Ctrl Pts',(0.993279089156325,1.06847604194517,2.80043861029839));
#47211=CARTESIAN_POINT('Ctrl Pts',(0.997608246281604,1.1851427086119,2.73622560903023));
#47212=CARTESIAN_POINT('Ctrl Pts',(1.00569003540253,1.30000000000018,2.66339387293194));
#47213=CARTESIAN_POINT('Ctrl Pts',(1.22295971290336,-1.30000000000522,2.68787251266138));
#47214=CARTESIAN_POINT('Ctrl Pts',(1.19654332358173,-1.18514270861532,2.75037736984417));
#47215=CARTESIAN_POINT('Ctrl Pts',(1.17336384415623,-1.06847604194692,2.80568737756851));
#47216=CARTESIAN_POINT('Ctrl Pts',(1.12729251904644,-0.794772684000856,
2.91684301856624));
#47217=CARTESIAN_POINT('Ctrl Pts',(1.10872908000617,-0.6363098000952,2.97210999709675));
#47218=CARTESIAN_POINT('Ctrl Pts',(1.07528657029111,-0.319434907277161,
3.03843051421032));
#47219=CARTESIAN_POINT('Ctrl Pts',(1.06327501252726,-0.158333333333333,
3.05900814238434));
#47220=CARTESIAN_POINT('Ctrl Pts',(1.04142330771059,0.158333333333335,3.05362555883336));
#47221=CARTESIAN_POINT('Ctrl Pts',(1.03274202089434,0.319434907277169,3.02792543173402));
#47222=CARTESIAN_POINT('Ctrl Pts',(1.01931366641166,0.63630980009521,2.95011120583023));
#47223=CARTESIAN_POINT('Ctrl Pts',(1.01228085109468,0.794772684000845,2.88869625988921));
#47224=CARTESIAN_POINT('Ctrl Pts',(1.01275044424827,1.06847604194518,2.7662681088466));
#47225=CARTESIAN_POINT('Ctrl Pts',(1.01575016411372,1.1851427086119,2.70592580887601));
#47226=CARTESIAN_POINT('Ctrl Pts',(1.02154633436856,1.30000000000019,2.63823581911109));
#47227=CARTESIAN_POINT('Ctrl Pts',(1.24182813440133,-1.30000000000522,2.66390221260576));
#47228=CARTESIAN_POINT('Ctrl Pts',(1.218725159562,-1.18514270861532,2.72147669928059));
#47229=CARTESIAN_POINT('Ctrl Pts',(1.19758527856108,-1.06847604194691,2.77303231271835));
#47230=CARTESIAN_POINT('Ctrl Pts',(1.15328306391294,-0.794772684000849,
2.87823129217475));
#47231=CARTESIAN_POINT('Ctrl Pts',(1.13124218605865,-0.636309800095196,
2.93328961063753));
#47232=CARTESIAN_POINT('Ctrl Pts',(1.09568620149555,-0.319434907277159,
2.99864424003564));
#47233=CARTESIAN_POINT('Ctrl Pts',(1.08232555204351,-0.158333333333332,
3.02082353147524));
#47234=CARTESIAN_POINT('Ctrl Pts',(1.05962125523247,0.158333333333334,3.01518360825578));
#47235=CARTESIAN_POINT('Ctrl Pts',(1.05131103637489,0.319434907277167,2.98763078916219));
#47236=CARTESIAN_POINT('Ctrl Pts',(1.03851498364947,0.636309800095206,2.91024541366821));
#47237=CARTESIAN_POINT('Ctrl Pts',(1.03363914893915,0.794772684000838,2.84845345753121));
#47238=CARTESIAN_POINT('Ctrl Pts',(1.03272231259024,1.06847604194517,2.73201465841564));
#47239=CARTESIAN_POINT('Ctrl Pts',(1.0343351888939,1.1851427086119,2.67561491464539));
#47240=CARTESIAN_POINT('Ctrl Pts',(1.03795780598451,1.30000000000018,2.6132174687593));
#47241=CARTESIAN_POINT('Ctrl Pts',(1.26205481118799,-1.30000000000522,2.6405729968505));
#47242=CARTESIAN_POINT('Ctrl Pts',(1.24207905433544,-1.18514270861532,2.69320565243503));
#47243=CARTESIAN_POINT('Ctrl Pts',(1.22293655530526,-1.06847604194691,2.74102898310266));
#47244=CARTESIAN_POINT('Ctrl Pts',(1.18063854536445,-0.794772684000849,
2.84039994130838));
#47245=CARTESIAN_POINT('Ctrl Pts',(1.15634659093339,-0.636309800095197,
2.89566365798084));
#47246=CARTESIAN_POINT('Ctrl Pts',(1.11824845891302,-0.319434907277159,
2.959865286098));
#47247=CARTESIAN_POINT('Ctrl Pts',(1.10145016334698,-0.158333333333332,
2.98284476091643));
#47248=CARTESIAN_POINT('Ctrl Pts',(1.07788761365085,0.158333333333334,2.9769227689399));
#47249=CARTESIAN_POINT('Ctrl Pts',(1.07184303038958,0.319434907277167,2.94821599520184));
#47250=CARTESIAN_POINT('Ctrl Pts',(1.06048002749707,0.636309800095206,2.87155512008751));
#47251=CARTESIAN_POINT('Ctrl Pts',(1.05776628174413,0.794772684000839,2.80942552455464));
#47252=CARTESIAN_POINT('Ctrl Pts',(1.05479561954693,1.06847604194517,2.69868648796352));
#47253=CARTESIAN_POINT('Ctrl Pts',(1.05450561934856,1.1851427086119,2.64600329499075));
#47254=CARTESIAN_POINT('Ctrl Pts',(1.05521150854311,1.30000000000018,2.58857173469979));
#47255=CARTESIAN_POINT('Ctrl Pts',(1.2776175603506,-1.30000000000522,2.62164579396498));
#47256=CARTESIAN_POINT('Ctrl Pts',(1.25999481688344,-1.18514270861532,2.67023889873838));
#47257=CARTESIAN_POINT('Ctrl Pts',(1.24245454125395,-1.06847604194691,2.71506046278283));
#47258=CARTESIAN_POINT('Ctrl Pts',(1.20212351283273,-0.794772684000848,
2.80989422866985));
#47259=CARTESIAN_POINT('Ctrl Pts',(1.17673956294012,-0.636309800095195,
2.86564566881686));
#47260=CARTESIAN_POINT('Ctrl Pts',(1.13757402022123,-0.319434907277158,
2.92927823955686));
#47261=CARTESIAN_POINT('Ctrl Pts',(1.11908596269311,-0.158333333333332,
2.9532378566013));
#47262=CARTESIAN_POINT('Ctrl Pts',(1.09474153850865,0.158333333333334,2.94703959578193));
#47263=CARTESIAN_POINT('Ctrl Pts',(1.08928741242003,0.319434907277168,2.91697547995212));
#47264=CARTESIAN_POINT('Ctrl Pts',(1.07804578085774,0.636309800095207,2.84052651170049));
#47265=CARTESIAN_POINT('Ctrl Pts',(1.07646188707476,0.794772684000837,2.77790287505706));
#47266=CARTESIAN_POINT('Ctrl Pts',(1.07156457759862,1.06847604194517,2.67164506778811));
#47267=CARTESIAN_POINT('Ctrl Pts',(1.06978486191151,1.1851427086119,2.62196362218695));
#47268=CARTESIAN_POINT('Ctrl Pts',(1.0683452943463,1.30000000000018,2.56859579851158));
#47269=CARTESIAN_POINT('Ctrl Pts',(1.29897751391511,-1.30000000000523,2.59886823472693));
#47270=CARTESIAN_POINT('Ctrl Pts',(1.28556771443465,-1.18514270861533,2.6430095662816));
#47271=CARTESIAN_POINT('Ctrl Pts',(1.27070247446087,-1.06847604194692,2.68439718474942));
#47272=CARTESIAN_POINT('Ctrl Pts',(1.23299843764119,-0.79477268400086,2.77364923486504));
#47273=CARTESIAN_POINT('Ctrl Pts',(1.2038834720301,-0.636309800095201,2.82891455501619));
#47274=CARTESIAN_POINT('Ctrl Pts',(1.16234242040859,-0.31943490727716,2.89136182815192));
#47275=CARTESIAN_POINT('Ctrl Pts',(1.14182485146547,-0.158333333333333,
2.91660410511155));
#47276=CARTESIAN_POINT('Ctrl Pts',(1.11654454161528,0.158333333333335,2.91006068713333));
#47277=CARTESIAN_POINT('Ctrl Pts',(1.11201924982408,0.319434907277169,2.87835454662367));
#47278=CARTESIAN_POINT('Ctrl Pts',(1.10158246377129,0.63630980009521,2.80241675556593));
#47279=CARTESIAN_POINT('Ctrl Pts',(1.10242798139847,0.794772684000843,2.73959979850215));
#47280=CARTESIAN_POINT('Ctrl Pts',(1.09531632657767,1.06847604194518,2.63899234578077));
#47281=CARTESIAN_POINT('Ctrl Pts',(1.09153908597683,1.18514270861191,2.59298824503687));
#47282=CARTESIAN_POINT('Ctrl Pts',(1.08706297663432,1.30000000000019,2.54452928195864));
#47283=CARTESIAN_POINT('Ctrl Pts',(1.32380250697462,-1.30000000000523,2.57121941147693));
#47284=CARTESIAN_POINT('Ctrl Pts',(1.31451069985451,-1.18514270861532,2.60959592800393));
#47285=CARTESIAN_POINT('Ctrl Pts',(1.30247132551968,-1.06847604194691,2.64668422653664));
#47286=CARTESIAN_POINT('Ctrl Pts',(1.26831053242304,-0.794772684000854,
2.72938957436126));
#47287=CARTESIAN_POINT('Ctrl Pts',(1.23745046376972,-0.636309800095198,
2.78527587837556));
#47288=CARTESIAN_POINT('Ctrl Pts',(1.19416076340524,-0.319434907277159,
2.84674169288415));
#47289=CARTESIAN_POINT('Ctrl Pts',(1.17034498851464,-0.158333333333333,
2.87309146320457));
#47290=CARTESIAN_POINT('Ctrl Pts',(1.14442378353678,0.158333333333335,2.86629821921497));
#47291=CARTESIAN_POINT('Ctrl Pts',(1.14248695695105,0.31943490727717,2.83323019655854));
#47292=CARTESIAN_POINT('Ctrl Pts',(1.13263359597151,0.63630980009521,2.75777428057413));
#47293=CARTESIAN_POINT('Ctrl Pts',(1.13439789288439,0.794772684000841,2.69394937050413));
#47294=CARTESIAN_POINT('Ctrl Pts',(1.12349975140898,1.06847604194517,2.59970003508306));
#47295=CARTESIAN_POINT('Ctrl Pts',(1.11701341685411,1.1851427086119,2.55799661174547));
#47296=CARTESIAN_POINT('Ctrl Pts',(1.10875814937315,1.30000000000018,2.515386810092));
#47297=CARTESIAN_POINT('Ctrl Pts',(1.34353479425786,-1.30000000000523,2.55103104359542));
#47298=CARTESIAN_POINT('Ctrl Pts',(1.33804312545896,-1.18514270861533,2.58543063651654));
#47299=CARTESIAN_POINT('Ctrl Pts',(1.32849265660278,-1.06847604194692,2.61947456860717));
#47300=CARTESIAN_POINT('Ctrl Pts',(1.29705252288802,-0.794772684000856,
2.69730121453301));
#47301=CARTESIAN_POINT('Ctrl Pts',(1.26322137201649,-0.636309800095202,
2.75286490573782));
#47302=CARTESIAN_POINT('Ctrl Pts',(1.21856519239577,-0.319434907277162,
2.81352802858837));
#47303=CARTESIAN_POINT('Ctrl Pts',(1.19370551790263,-0.158333333333333,
2.84130728407494));
#47304=CARTESIAN_POINT('Ctrl Pts',(1.1672572311677,0.158333333333336,2.83430539053762));
#47305=CARTESIAN_POINT('Ctrl Pts',(1.16583639205031,0.319434907277169,2.79963733920804));
#47306=CARTESIAN_POINT('Ctrl Pts',(1.15627757415748,0.63630980009521,2.72448149151503));
#47307=CARTESIAN_POINT('Ctrl Pts',(1.16001923508657,0.794772684000848,2.66042492911123));
#47308=CARTESIAN_POINT('Ctrl Pts',(1.14623297406581,1.06847604194518,2.57091255294235));
#47309=CARTESIAN_POINT('Ctrl Pts',(1.13744728375627,1.1851427086119,2.53231823294277));
#47310=CARTESIAN_POINT('Ctrl Pts',(1.12584346470176,1.30000000000018,2.4938761838267));
#47311=CARTESIAN_POINT('Ctrl Pts',(1.35705527879887,-1.30000000000523,2.53776290116183));
#47312=CARTESIAN_POINT('Ctrl Pts',(1.35380115355581,-1.18514270861533,2.56938305660187));
#47313=CARTESIAN_POINT('Ctrl Pts',(1.34584081416615,-1.06847604194692,2.60136950328211));
#47314=CARTESIAN_POINT('Ctrl Pts',(1.31657854156224,-0.794772684000857,
2.6761108000208));
#47315=CARTESIAN_POINT('Ctrl Pts',(1.28246012884012,-0.636309800095202,
2.73221828163434));
#47316=CARTESIAN_POINT('Ctrl Pts',(1.2366713883074,-0.319434907277162,2.7922420731235));
#47317=CARTESIAN_POINT('Ctrl Pts',(1.20915115452519,-0.158333333333333,
2.82009033602051));
#47318=CARTESIAN_POINT('Ctrl Pts',(1.18189193316008,0.158333333333336,2.81272748580012));
#47319=CARTESIAN_POINT('Ctrl Pts',(1.18192670079688,0.319434907277169,2.77746487924114));
#47320=CARTESIAN_POINT('Ctrl Pts',(1.17265121446526,0.636309800095211,2.70254838042864));
#47321=CARTESIAN_POINT('Ctrl Pts',(1.17696692154763,0.794772684000848,2.63804206835142));
#47322=CARTESIAN_POINT('Ctrl Pts',(1.16121360887195,1.06847604194518,2.55166730436085));
#47323=CARTESIAN_POINT('Ctrl Pts',(1.15100373070832,1.1851427086119,2.51518588101529));
#47324=CARTESIAN_POINT('Ctrl Pts',(1.13740299972059,1.30000000000018,2.47961146915524));
#47325=CARTESIAN_POINT('Ctrl Pts',(1.36521872532696,-1.30000000000523,2.52851742886439));
#47326=CARTESIAN_POINT('Ctrl Pts',(1.36336594929023,-1.18514270861533,2.55823334895911));
#47327=CARTESIAN_POINT('Ctrl Pts',(1.35639680598846,-1.06847604194692,2.58881179127426));
#47328=CARTESIAN_POINT('Ctrl Pts',(1.32847685888128,-0.794772684000858,
2.66144670909424));
#47329=CARTESIAN_POINT('Ctrl Pts',(1.29382137562031,-0.636309800095202,
2.71778507964574));
#47330=CARTESIAN_POINT('Ctrl Pts',(1.24792930699923,-0.319434907277162,
2.77768202334506));
#47331=CARTESIAN_POINT('Ctrl Pts',(1.21991426953575,-0.158333333333334,
2.80614264216758));
#47332=CARTESIAN_POINT('Ctrl Pts',(1.1928290090653,0.158333333333336,2.79885835339839));
#47333=CARTESIAN_POINT('Ctrl Pts',(1.19381822041475,0.319434907277169,2.76319030999829));
#47334=CARTESIAN_POINT('Ctrl Pts',(1.18441850015633,0.636309800095211,2.68829922773841));
#47335=CARTESIAN_POINT('Ctrl Pts',(1.18823577795932,0.794772684000848,2.62311338878884));
#47336=CARTESIAN_POINT('Ctrl Pts',(1.17093262167389,1.06847604194518,2.53872392163905));
#47337=CARTESIAN_POINT('Ctrl Pts',(1.15981958146128,1.1851427086119,2.50366856483175));
#47338=CARTESIAN_POINT('Ctrl Pts',(1.1450833962469,1.30000000000018,2.47008692460837));
#47339=CARTESIAN_POINT('Ctrl Pts',(1.38122654843761,-1.30000000000523,2.51318553227769));
#47340=CARTESIAN_POINT('Ctrl Pts',(1.38278099200282,-1.18514270861533,2.54005217521767));
#47341=CARTESIAN_POINT('Ctrl Pts',(1.37809806873369,-1.06847604194692,2.56844338335525));
#47342=CARTESIAN_POINT('Ctrl Pts',(1.35287001399835,-0.794772684000859,
2.63755480438889));
#47343=CARTESIAN_POINT('Ctrl Pts',(1.31627260802992,-0.636309800095202,
2.69375117495694));
#47344=CARTESIAN_POINT('Ctrl Pts',(1.26885276023804,-0.319434907277161,
2.75277362407299));
#47345=CARTESIAN_POINT('Ctrl Pts',(1.23884504163408,-0.158333333333334,
2.7817914624677));
#47346=CARTESIAN_POINT('Ctrl Pts',(1.21062406304607,0.158333333333336,2.77400047963829));
#47347=CARTESIAN_POINT('Ctrl Pts',(1.21188528420357,0.319434907277169,2.73703651047564));
#47348=CARTESIAN_POINT('Ctrl Pts',(1.20289147466563,0.636309800095211,2.6624604154852));
#47349=CARTESIAN_POINT('Ctrl Pts',(1.20908308624123,0.794772684000847,2.59748057087056));
#47350=CARTESIAN_POINT('Ctrl Pts',(1.18963859489542,1.06847604194518,2.51681692708733));
#47351=CARTESIAN_POINT('Ctrl Pts',(1.17662584357406,1.1851427086119,2.48412382801717));
#47352=CARTESIAN_POINT('Ctrl Pts',(1.15901714074552,1.30000000000018,2.45365393238805));
#47353=CARTESIAN_POINT('Ctrl Pts',(1.39929231839369,-1.30000000000524,2.49557601088206));
#47354=CARTESIAN_POINT('Ctrl Pts',(1.4043825297588,-1.18514270861533,2.51902603264737));
#47355=CARTESIAN_POINT('Ctrl Pts',(1.40209251391536,-1.06847604194692,2.54482000595124));
#47356=CARTESIAN_POINT('Ctrl Pts',(1.37975231793992,-0.794772684000858,
2.60982424130932));
#47357=CARTESIAN_POINT('Ctrl Pts',(1.34090487750289,-0.636309800095206,
2.66585079183438));
#47358=CARTESIAN_POINT('Ctrl Pts',(1.29277799309058,-0.319434907277165,
2.72434458679463));
#47359=CARTESIAN_POINT('Ctrl Pts',(1.26193437457079,-0.158333333333334,
2.75465054837699));
#47360=CARTESIAN_POINT('Ctrl Pts',(1.2337965541703,0.158333333333336,2.74689265505336));
#47361=CARTESIAN_POINT('Ctrl Pts',(1.23645399959435,0.319434907277168,2.70891052034103));
#47362=CARTESIAN_POINT('Ctrl Pts',(1.22736466079988,0.636309800095212,2.63444799711698));
#47363=CARTESIAN_POINT('Ctrl Pts',(1.23374892176809,0.794772684000854,2.56861469097783));
#47364=CARTESIAN_POINT('Ctrl Pts',(1.21088952787038,1.06847604194519,2.49177015120832));
#47365=CARTESIAN_POINT('Ctrl Pts',(1.19561848422943,1.18514270861191,2.46172586752891));
#47366=CARTESIAN_POINT('Ctrl Pts',(1.17497138154185,1.30000000000019,2.43490045406549));
#47367=CARTESIAN_POINT('Ctrl Pts',(1.41702750924289,-1.30000000000524,2.47782989780478));
#47368=CARTESIAN_POINT('Ctrl Pts',(1.42540170270334,-1.18514270861534,2.49774146295186));
#47369=CARTESIAN_POINT('Ctrl Pts',(1.42550258089223,-1.06847604194693,2.52093867861861));
#47370=CARTESIAN_POINT('Ctrl Pts',(1.40662261634099,-0.794772684000863,
2.58211939738794));
#47371=CARTESIAN_POINT('Ctrl Pts',(1.3674919546006,-0.636309800095208,2.63893967676586));
#47372=CARTESIAN_POINT('Ctrl Pts',(1.31859656767163,-0.319434907277165,
2.6968814494316));
#47373=CARTESIAN_POINT('Ctrl Pts',(1.28526603322289,-0.158333333333335,
2.72766636464627));
#47374=CARTESIAN_POINT('Ctrl Pts',(1.25601404650177,0.158333333333337,2.71937822426703));
#47375=CARTESIAN_POINT('Ctrl Pts',(1.25935949790364,0.31943490727717,2.68007583722304));
#47376=CARTESIAN_POINT('Ctrl Pts',(1.25016395852549,0.636309800095215,2.6057188510221));
#47377=CARTESIAN_POINT('Ctrl Pts',(1.25785622378767,0.794772684000856,2.53952562511162));
#47378=CARTESIAN_POINT('Ctrl Pts',(1.23205394370523,1.06847604194519,2.46670730026971));
#47379=CARTESIAN_POINT('Ctrl Pts',(1.21461736482249,1.18514270861192,2.43935205790224));
#47380=CARTESIAN_POINT('Ctrl Pts',(1.190913058036,1.3000000000002,2.41616192780651));
#47381=CARTESIAN_POINT('Ctrl Pts',(1.42889034239943,-1.30000000000524,2.4671347108158));
#47382=CARTESIAN_POINT('Ctrl Pts',(1.43959238218228,-1.18514270861534,2.48498799650351));
#47383=CARTESIAN_POINT('Ctrl Pts',(1.44129116148517,-1.06847604194693,2.50662397310923));
#47384=CARTESIAN_POINT('Ctrl Pts',(1.42441634870989,-0.794772684000864,
2.56534618007554));
#47385=CARTESIAN_POINT('Ctrl Pts',(1.38418283888682,-0.636309800095209,
2.62218715507073));
#47386=CARTESIAN_POINT('Ctrl Pts',(1.33453728210758,-0.319434907277165,
2.679638563251));
#47387=CARTESIAN_POINT('Ctrl Pts',(1.29984363043981,-0.158333333333335,
2.71081619697965));
#47388=CARTESIAN_POINT('Ctrl Pts',(1.27036017180119,0.158333333333337,2.70240606017764));
#47389=CARTESIAN_POINT('Ctrl Pts',(1.27482324691011,0.31943490727717,2.66259157303672));
#47390=CARTESIAN_POINT('Ctrl Pts',(1.2659349467312,0.636309800095216,2.58847112715167));
#47391=CARTESIAN_POINT('Ctrl Pts',(1.27444322061751,0.794772684000857,2.5220568277252));
#47392=CARTESIAN_POINT('Ctrl Pts',(1.24642615280947,1.06847604194519,2.45157978994058));
#47393=CARTESIAN_POINT('Ctrl Pts',(1.22735423829508,1.18514270861192,2.4257732250998));
#47394=CARTESIAN_POINT('Ctrl Pts',(1.20133795978574,1.3000000000002,2.40466699364358));
#47395=CARTESIAN_POINT('Ctrl Pts',(1.43805424294559,-1.30000000000524,2.45842477476555));
#47396=CARTESIAN_POINT('Ctrl Pts',(1.45052579669823,-1.18514270861534,2.47458154256932));
#47397=CARTESIAN_POINT('Ctrl Pts',(1.4534793455906,-1.06847604194693,2.4949549554672));
#47398=CARTESIAN_POINT('Ctrl Pts',(1.43831413908994,-0.794772684000866,
2.55176290865245));
#47399=CARTESIAN_POINT('Ctrl Pts',(1.39764596953041,-0.636309800095209,
2.60885128227389));
#47400=CARTESIAN_POINT('Ctrl Pts',(1.34745618703037,-0.319434907277166,
2.66594148200833));
#47401=CARTESIAN_POINT('Ctrl Pts',(1.31136635177083,-0.158333333333335,
2.69727833926731));
#47402=CARTESIAN_POINT('Ctrl Pts',(1.28158088407649,0.158333333333337,2.68871558444311));
#47403=CARTESIAN_POINT('Ctrl Pts',(1.286959737645,0.319434907277171,2.6485089972729));
#47404=CARTESIAN_POINT('Ctrl Pts',(1.27836387244858,0.636309800095217,2.57460236864966));
#47405=CARTESIAN_POINT('Ctrl Pts',(1.28763311239507,0.794772684000857,2.50806146259966));
#47406=CARTESIAN_POINT('Ctrl Pts',(1.25789371311807,1.06847604194519,2.4394775747014));
#47407=CARTESIAN_POINT('Ctrl Pts',(1.23752024547041,1.18514270861192,2.41491090455382));
#47408=CARTESIAN_POINT('Ctrl Pts',(1.20964639416876,1.3000000000002,2.39546498804632));
#47409=CARTESIAN_POINT('Ctrl Pts',(1.44524658952179,-1.30000000000524,2.45206126832144));
#47410=CARTESIAN_POINT('Ctrl Pts',(1.45922916135726,-1.18514270861534,2.46704874305171));
#47411=CARTESIAN_POINT('Ctrl Pts',(1.46320189478081,-1.06847604194693,2.486520269857));
#47412=CARTESIAN_POINT('Ctrl Pts',(1.44925497453907,-0.794772684000865,
2.54186244936722));
#47413=CARTESIAN_POINT('Ctrl Pts',(1.40764544713522,-0.636309800095209,
2.59880991679825));
#47414=CARTESIAN_POINT('Ctrl Pts',(1.35704382757086,-0.319434907277166,
2.65561612297188));
#47415=CARTESIAN_POINT('Ctrl Pts',(1.32050975053321,-0.158333333333335,
2.68736805486952));
#47416=CARTESIAN_POINT('Ctrl Pts',(1.29048989222242,0.158333333333337,2.67868800789844));
#47417=CARTESIAN_POINT('Ctrl Pts',(1.29612786258562,0.319434907277171,2.6379816075213));
#47418=CARTESIAN_POINT('Ctrl Pts',(1.28736604709719,0.636309800095217,2.56405374750536));
#47419=CARTESIAN_POINT('Ctrl Pts',(1.29683125017996,0.794772684000857,2.49724645076415));
#47420=CARTESIAN_POINT('Ctrl Pts',(1.26587042318278,1.06847604194519,2.43011340484364));
#47421=CARTESIAN_POINT('Ctrl Pts',(1.24467757393584,1.18514270861192,2.40654812886309));
#47422=CARTESIAN_POINT('Ctrl Pts',(1.21569367023734,1.3000000000002,2.38847698495646));
#47423=CARTESIAN_POINT('Ctrl Pts',(1.45125471048104,-1.30000000000525,2.44677151525934));
#47424=CARTESIAN_POINT('Ctrl Pts',(1.46657802915925,-1.18514270861534,2.46082699799967));
#47425=CARTESIAN_POINT('Ctrl Pts',(1.47145035971793,-1.06847604194693,2.47957310579907));
#47426=CARTESIAN_POINT('Ctrl Pts',(1.45856254474585,-0.794772684000865,
2.53371664720401));
#47427=CARTESIAN_POINT('Ctrl Pts',(1.41605853233152,-0.63630980009521,2.5904910869508));
#47428=CARTESIAN_POINT('Ctrl Pts',(1.36511105480377,-0.319434907277166,
2.64705620006073));
#47429=CARTESIAN_POINT('Ctrl Pts',(1.32826769120673,-0.158333333333335,
2.67917980570048));
#47430=CARTESIAN_POINT('Ctrl Pts',(1.2980787856736,0.158333333333337,2.67041270033892));
#47431=CARTESIAN_POINT('Ctrl Pts',(1.30394353688909,0.319434907277171,2.62929574596627));
#47432=CARTESIAN_POINT('Ctrl Pts',(1.29500696350862,0.636309800095217,2.55533351194471));
#47433=CARTESIAN_POINT('Ctrl Pts',(1.30456279045928,0.794772684000857,2.48827139801315));
#47434=CARTESIAN_POINT('Ctrl Pts',(1.27253343099669,1.06847604194519,2.42232284467321));
#47435=CARTESIAN_POINT('Ctrl Pts',(1.25064238382091,1.18514270861192,2.39958405766975));
#47436=CARTESIAN_POINT('Ctrl Pts',(1.22072461237596,1.3000000000002,2.38265316876895));
#47437=CARTESIAN_POINT('Ctrl Pts',(1.45537244101042,-1.30000000000525,2.44302273583353));
#47438=CARTESIAN_POINT('Ctrl Pts',(1.47152458935058,-1.18514270861534,2.45636857978332));
#47439=CARTESIAN_POINT('Ctrl Pts',(1.47698039860248,-1.06847604194693,2.47458286929736));
#47440=CARTESIAN_POINT('Ctrl Pts',(1.46487372631624,-0.794772684000864,
2.52790860501314));
#47441=CARTESIAN_POINT('Ctrl Pts',(1.42209453125328,-0.636309800095209,
2.58474542793579));
#47442=CARTESIAN_POINT('Ctrl Pts',(1.37094607013501,-0.319434907277166,
2.64116469303645));
#47443=CARTESIAN_POINT('Ctrl Pts',(1.33362045532777,-0.158333333333335,
2.67341299515971));
#47444=CARTESIAN_POINT('Ctrl Pts',(1.30330856590516,0.158333333333337,2.66458056519826));
#47445=CARTESIAN_POINT('Ctrl Pts',(1.30949201144557,0.319434907277171,2.62325544072632));
#47446=CARTESIAN_POINT('Ctrl Pts',(1.30058855659897,0.636309800095217,2.54934296144613));
#47447=CARTESIAN_POINT('Ctrl Pts',(1.31039949309279,0.794772684000857,2.4821908922298));
#47448=CARTESIAN_POINT('Ctrl Pts',(1.27755379562326,1.06847604194519,2.41703947810683));
#47449=CARTESIAN_POINT('Ctrl Pts',(1.25507677437302,1.18514270861192,2.39483386454386));
#47450=CARTESIAN_POINT('Ctrl Pts',(1.22434041725408,1.3000000000002,2.37862427049395));
#47451=CARTESIAN_POINT('Ctrl Pts',(1.45770889761886,-1.30000000000525,2.44087227806979));
#47452=CARTESIAN_POINT('Ctrl Pts',(1.47431661684261,-1.18514270861534,2.4538032152612));
#47453=CARTESIAN_POINT('Ctrl Pts',(1.48009896655861,-1.06847604194693,2.47171005037934));
#47454=CARTESIAN_POINT('Ctrl Pts',(1.4684485819871,-0.794772684000865,2.52457374138764));
#47455=CARTESIAN_POINT('Ctrl Pts',(1.42557749616056,-0.636309800095209,
2.58148035505117));
#47456=CARTESIAN_POINT('Ctrl Pts',(1.37432090710934,-0.319434907277166,
2.63782004259088));
#47457=CARTESIAN_POINT('Ctrl Pts',(1.33666723192535,-0.158333333333335,
2.6701128498047));
#47458=CARTESIAN_POINT('Ctrl Pts',(1.30628393068094,0.158333333333337,2.66124204030451));
#47459=CARTESIAN_POINT('Ctrl Pts',(1.31268294514712,0.319434907277172,2.61981443073772));
#47460=CARTESIAN_POINT('Ctrl Pts',(1.3038258337411,0.636309800095217,2.5459432773986));
#47461=CARTESIAN_POINT('Ctrl Pts',(1.31381025086918,0.794772684000857,2.47875244019008));
#47462=CARTESIAN_POINT('Ctrl Pts',(1.28048713217962,1.06847604194519,2.41405118048533));
#47463=CARTESIAN_POINT('Ctrl Pts',(1.25766003214743,1.18514270861192,2.39214301276931));
#47464=CARTESIAN_POINT('Ctrl Pts',(1.22643017542054,1.3000000000002,2.37633345524551));
#47465=CARTESIAN_POINT('Ctrl Pts',(1.46814055446569,-1.30000000000524,2.43115338734429));
#47466=CARTESIAN_POINT('Ctrl Pts',(1.48673518636836,-1.18514270861534,2.44218454247932));
#47467=CARTESIAN_POINT('Ctrl Pts',(1.49396285394707,-1.06847604194693,2.45869541848749));
#47468=CARTESIAN_POINT('Ctrl Pts',(1.48440025040216,-0.794772684000863,
2.5094980964867));
#47469=CARTESIAN_POINT('Ctrl Pts',(1.44132034195163,-0.636309800095208,
2.56682530190243));
#47470=CARTESIAN_POINT('Ctrl Pts',(1.38964689881658,-0.319434907277165,
2.62284337703136));
#47471=CARTESIAN_POINT('Ctrl Pts',(1.35044030854968,-0.158333333333335,
2.65529734648699));
#47472=CARTESIAN_POINT('Ctrl Pts',(1.3197407819702,0.158333333333337,2.64625545093226));
#47473=CARTESIAN_POINT('Ctrl Pts',(1.3271147927352,0.31943490727717,2.60436881916562));
#47474=CARTESIAN_POINT('Ctrl Pts',(1.31856345788762,0.636309800095216,2.53072901757618));
#47475=CARTESIAN_POINT('Ctrl Pts',(1.32954725468782,0.794772684000856,2.46346697110161));
#47476=CARTESIAN_POINT('Ctrl Pts',(1.29403141650394,1.06847604194519,2.40076968330603));
#47477=CARTESIAN_POINT('Ctrl Pts',(1.26954793162237,1.18514270861192,2.38016129957916));
#47478=CARTESIAN_POINT('Ctrl Pts',(1.23595445221752,1.3000000000002,2.36608386484867));
#47479=CARTESIAN_POINT('Ctrl Pts',(1.48346539173413,-1.30000000000523,2.41811719874013));
#47480=CARTESIAN_POINT('Ctrl Pts',(1.50537195826871,-1.18514270861532,2.42681832126565));
#47481=CARTESIAN_POINT('Ctrl Pts',(1.51488511192707,-1.06847604194692,2.44154812472289));
#47482=CARTESIAN_POINT('Ctrl Pts',(1.50823113694001,-0.794772684000855,
2.48950437638155));
#47483=CARTESIAN_POINT('Ctrl Pts',(1.46354339745113,-0.6363098000952,2.54671340487404));
#47484=CARTESIAN_POINT('Ctrl Pts',(1.411125321792,-0.319434907277161,2.60217481893685));
#47485=CARTESIAN_POINT('Ctrl Pts',(1.37071656390568,-0.158333333333333,
2.63531459468677));
#47486=CARTESIAN_POINT('Ctrl Pts',(1.33947123938326,0.158333333333335,2.62597631962764));
#47487=CARTESIAN_POINT('Ctrl Pts',(1.3476753188231,0.31943490727717,2.58319881968591));
#47488=CARTESIAN_POINT('Ctrl Pts',(1.33840305303561,0.636309800095211,2.509325968028));
#47489=CARTESIAN_POINT('Ctrl Pts',(1.34865735229928,0.794772684000845,2.44096986906576));
#47490=CARTESIAN_POINT('Ctrl Pts',(1.31073523642226,1.06847604194518,2.3813193857751));
#47491=CARTESIAN_POINT('Ctrl Pts',(1.28489309106389,1.1851427086119,2.36293639782752));
#47492=CARTESIAN_POINT('Ctrl Pts',(1.24962387915744,1.30000000000019,2.35199090588064));
#47493=CARTESIAN_POINT('Ctrl Pts',(1.50232800365894,-1.30000000000523,2.40107596869255));
#47494=CARTESIAN_POINT('Ctrl Pts',(1.52841317350604,-1.18514270861532,2.40677102458424));
#47495=CARTESIAN_POINT('Ctrl Pts',(1.54083972280061,-1.06847604194691,2.41921947995603));
#47496=CARTESIAN_POINT('Ctrl Pts',(1.53799339171977,-0.794772684000854,
2.46357960598144));
#47497=CARTESIAN_POINT('Ctrl Pts',(1.49159331440414,-0.636309800095201,
2.52080060706813));
#47498=CARTESIAN_POINT('Ctrl Pts',(1.43822367291136,-0.319434907277162,
2.57555728417339));
#47499=CARTESIAN_POINT('Ctrl Pts',(1.39576077015877,-0.158333333333333,
2.6093349919864));
#47500=CARTESIAN_POINT('Ctrl Pts',(1.36412134633887,0.158333333333335,2.59977366191929));
#47501=CARTESIAN_POINT('Ctrl Pts',(1.37380619390945,0.319434907277167,2.55606276684382));
#47502=CARTESIAN_POINT('Ctrl Pts',(1.36504791729566,0.636309800095209,2.48258779516276));
#47503=CARTESIAN_POINT('Ctrl Pts',(1.37741843250096,0.794772684000847,2.41426910879833));
#47504=CARTESIAN_POINT('Ctrl Pts',(1.335210658048,1.06847604194518,2.35798863023809));
#47505=CARTESIAN_POINT('Ctrl Pts',(1.30610774767455,1.1851427086119,2.34176005044349));
#47506=CARTESIAN_POINT('Ctrl Pts',(1.26617210853617,1.30000000000018,2.33366462462575));
#47507=CARTESIAN_POINT('Ctrl Pts',(1.51240241427739,-1.30000000000522,2.39289301592785));
#47508=CARTESIAN_POINT('Ctrl Pts',(1.54036079622412,-1.18514270861532,2.39698352052958));
#47509=CARTESIAN_POINT('Ctrl Pts',(1.5541361931653,-1.06847604194691,2.40824395634222));
#47510=CARTESIAN_POINT('Ctrl Pts',(1.55319458319893,-0.794772684000851,
2.45082179114856));
#47511=CARTESIAN_POINT('Ctrl Pts',(1.50638430478293,-0.636309800095197,
2.50829316388192));
#47512=CARTESIAN_POINT('Ctrl Pts',(1.45275981718469,-0.319434907277159,
2.56280057377912));
#47513=CARTESIAN_POINT('Ctrl Pts',(1.40945018590222,-0.158333333333332,
2.596952544446));
#47514=CARTESIAN_POINT('Ctrl Pts',(1.37727481249132,0.158333333333334,2.5870955960286));
#47515=CARTESIAN_POINT('Ctrl Pts',(1.38703062157811,0.319434907277167,2.54259045047355));
#47516=CARTESIAN_POINT('Ctrl Pts',(1.37792399116514,0.636309800095206,2.46901592396535));
#47517=CARTESIAN_POINT('Ctrl Pts',(1.39070615145891,0.79477268400084,2.4004245622768));
#47518=CARTESIAN_POINT('Ctrl Pts',(1.34687223012689,1.06847604194517,2.34604685839021));
#47519=CARTESIAN_POINT('Ctrl Pts',(1.3166617592273,1.1851427086119,2.33112379976082));
#47520=CARTESIAN_POINT('Ctrl Pts',(1.27521489776589,1.30000000000018,2.32481577562205));
#47521=CARTESIAN_POINT('Ctrl Pts',(1.5174122737698,-1.30000000000522,2.38879014525548));
#47522=CARTESIAN_POINT('Ctrl Pts',(1.54630261814547,-1.18514270861532,2.39207685648064));
#47523=CARTESIAN_POINT('Ctrl Pts',(1.56074958986041,-1.06847604194691,2.40274235366977));
#47524=CARTESIAN_POINT('Ctrl Pts',(1.56075790439564,-0.794772684000851,
2.44442825749958));
#47525=CARTESIAN_POINT('Ctrl Pts',(1.51378858280601,-0.636309800095197,
2.50204658614368));
#47526=CARTESIAN_POINT('Ctrl Pts',(1.45995892423166,-0.319434907277159,
2.55639080502906));
#47527=CARTESIAN_POINT('Ctrl Pts',(1.41600270611002,-0.158333333333332,
2.5906195818553));
#47528=CARTESIAN_POINT('Ctrl Pts',(1.38362278588542,0.158333333333334,2.58064707201732));
#47529=CARTESIAN_POINT('Ctrl Pts',(1.39375448302884,0.319434907277167,2.53591491365547));
#47530=CARTESIAN_POINT('Ctrl Pts',(1.38457112325773,0.636309800095206,2.4623387576987));
#47531=CARTESIAN_POINT('Ctrl Pts',(1.39741805963303,0.79477268400084,2.39353727747146));
#47532=CARTESIAN_POINT('Ctrl Pts',(1.3526706067805,1.06847604194517,2.34006403730454));
#47533=CARTESIAN_POINT('Ctrl Pts',(1.32185850051434,1.1851427086119,2.32577266001673));
#47534=CARTESIAN_POINT('Ctrl Pts',(1.27960380226534,1.30000000000018,2.32033648973054));
#47535=CARTESIAN_POINT('',(1.23744427200895,1.2,2.40716872050849));
#47536=CARTESIAN_POINT('Ctrl Pts',(1.23744427200895,1.2,2.40716872050849));
#47537=CARTESIAN_POINT('Ctrl Pts',(1.21265992951091,1.22410027197493,2.42566031732214));
#47538=CARTESIAN_POINT('Ctrl Pts',(1.18821929348464,1.24663669298873,2.44278295325562));
#47539=CARTESIAN_POINT('Ctrl Pts',(1.16764034544656,1.26665794013823,2.45828850243014));
#47540=CARTESIAN_POINT('Ctrl Pts',(1.15325920879695,1.28043540591626,2.46894367010376));
#47541=CARTESIAN_POINT('Ctrl Pts',(1.13357773502981,1.30000000000018,2.48433445644807));
#47542=CARTESIAN_POINT('',(1.38832548123549,0.653834841342252,2.44867888290427));
#47543=CARTESIAN_POINT('Ctrl Pts',(1.38832548119236,0.653834841327917,2.44867888285037));
#47544=CARTESIAN_POINT('Ctrl Pts',(1.37454923404638,0.710422285467849,2.44465349402137));
#47545=CARTESIAN_POINT('Ctrl Pts',(1.35937799661829,0.767445708967689,2.44028939546552));
#47546=CARTESIAN_POINT('Ctrl Pts',(1.32837715554167,0.881873342563316,2.43154329000569));
#47547=CARTESIAN_POINT('Ctrl Pts',(1.31343556545719,0.939380857891816,2.42739657917695));
#47548=CARTESIAN_POINT('Ctrl Pts',(1.28543018260622,1.03763475213985,2.41980418590468));
#47549=CARTESIAN_POINT('Ctrl Pts',(1.28390944537373,1.04222967121286,2.41937301107199));
#47550=CARTESIAN_POINT('Ctrl Pts',(1.25550432481215,1.13919581836279,2.41185397080366));
#47551=CARTESIAN_POINT('Ctrl Pts',(1.24774191689618,1.16589029126337,2.40982743326882));
#47552=CARTESIAN_POINT('Ctrl Pts',(1.23744427200895,1.2,2.40716872050849));
#47553=CARTESIAN_POINT('',(1.52166805320966,-0.653834841531101,2.48968935888076));
#47554=CARTESIAN_POINT('Ctrl Pts',(1.52166805320965,-0.653834841531103,
2.48968935888076));
#47555=CARTESIAN_POINT('Ctrl Pts',(1.49334294437536,-0.575779834472804,
2.5202663708974));
#47556=CARTESIAN_POINT('Ctrl Pts',(1.46876645094377,-0.493711163709688,
2.54538047219522));
#47557=CARTESIAN_POINT('Ctrl Pts',(1.43180311244362,-0.338122820387436,
2.58001286451235));
#47558=CARTESIAN_POINT('Ctrl Pts',(1.41789173110139,-0.265674896964429,
2.59130979717286));
#47559=CARTESIAN_POINT('Ctrl Pts',(1.39652617980709,-0.129743851517951,
2.60315463078574));
#47560=CARTESIAN_POINT('Ctrl Pts',(1.38848883722884,-0.066666048842503,
2.60504789056344));
#47561=CARTESIAN_POINT('Ctrl Pts',(1.37568467463284,0.0595072959430674,
2.60150288534975));
#47562=CARTESIAN_POINT('Ctrl Pts',(1.3708331957342,0.122731095105783,2.59605943341458));
#47563=CARTESIAN_POINT('Ctrl Pts',(1.36465986011061,0.260115581078158,2.57636314119223));
#47564=CARTESIAN_POINT('Ctrl Pts',(1.36408862584207,0.333988073947148,2.5606638868716));
#47565=CARTESIAN_POINT('Ctrl Pts',(1.36979927568344,0.491535585046963,2.51611859105072));
#47566=CARTESIAN_POINT('Ctrl Pts',(1.37696799146085,0.574935557742433,2.48517079865281));
#47567=CARTESIAN_POINT('Ctrl Pts',(1.38832548111874,0.653834841363331,2.44867888291351));
#47568=CARTESIAN_POINT('',(1.45278841576471,-1.2,2.46799135471839));
#47569=CARTESIAN_POINT('Ctrl Pts',(1.45278841576471,-1.2,2.46799135471839));
#47570=CARTESIAN_POINT('Ctrl Pts',(1.46425358638865,-1.13668704506502,2.47151131174211));
#47571=CARTESIAN_POINT('Ctrl Pts',(1.48060714938815,-1.03615749185349,2.47658610316088));
#47572=CARTESIAN_POINT('Ctrl Pts',(1.51314428743919,-0.775105528038972,
2.48691778855522));
#47573=CARTESIAN_POINT('Ctrl Pts',(1.51686893334905,-0.721274379078139,
2.48813900096771));
#47574=CARTESIAN_POINT('Ctrl Pts',(1.52166805320965,-0.653834841531101,
2.48968935888076));
#47575=CARTESIAN_POINT('Ctrl Pts',(1.3523706033532,-1.30000000000523,2.54236178400089));
#47576=CARTESIAN_POINT('Ctrl Pts',(1.35337714919034,-1.2989997171284,2.54161244521808));
#47577=CARTESIAN_POINT('Ctrl Pts',(1.35437680901242,-1.29799915645057,2.54086100403259));
#47578=CARTESIAN_POINT('Ctrl Pts',(1.37100486089963,-1.2810069371636,2.52800100315971));
#47579=CARTESIAN_POINT('Ctrl Pts',(1.38698908584542,-1.26515051009269,2.5161817713799));
#47580=CARTESIAN_POINT('Ctrl Pts',(1.41422895348329,-1.23763938663058,2.49560680488971));
#47581=CARTESIAN_POINT('Ctrl Pts',(1.43177461776686,-1.21964479809685,2.48208962741353));
#47582=CARTESIAN_POINT('Ctrl Pts',(1.45278841576471,-1.2,2.4679913547184));
#47583=CARTESIAN_POINT('Origin',(0.,1.25,7.2));
#47584=CARTESIAN_POINT('Origin',(0.,1.2,7.2));
#47585=CARTESIAN_POINT('Origin',(0.,0.92691742076555,7.2));
#47586=CARTESIAN_POINT('Origin',(0.,0.653834841531101,7.2));
#47587=CARTESIAN_POINT('Origin',(0.,0.,7.2));
#47588=CARTESIAN_POINT('Origin',(0.,-0.653834841531101,7.2));
#47589=CARTESIAN_POINT('Origin',(0.,-0.926917420765551,7.2));
#47590=CARTESIAN_POINT('Origin',(0.,-1.2,7.2));
#47591=CARTESIAN_POINT('Origin',(0.,-1.25,7.2));
#47592=CARTESIAN_POINT('Ctrl Pts',(1.83297302538932,-1.30000000000158,2.50013704960828));
#47593=CARTESIAN_POINT('Ctrl Pts',(1.79559295569107,-1.18514270861285,2.47969831528161));
#47594=CARTESIAN_POINT('Ctrl Pts',(1.76226517728476,-1.06847604194566,2.47314938072437));
#47595=CARTESIAN_POINT('Ctrl Pts',(1.69463294550958,-0.794772684000851,
2.49010824789955));
#47596=CARTESIAN_POINT('Ctrl Pts',(1.66458583994784,-0.636309800095196,
2.55332105438372));
#47597=CARTESIAN_POINT('Ctrl Pts',(1.61390936643532,-0.319434907277159,
2.60744757149477));
#47598=CARTESIAN_POINT('Ctrl Pts',(1.59581317861836,-0.158333333333332,
2.64959190996504));
#47599=CARTESIAN_POINT('Ctrl Pts',(1.56375557866912,0.158333333333334,2.63862740032203));
#47600=CARTESIAN_POINT('Ctrl Pts',(1.54831342142296,0.319434907277167,2.58509892141403));
#47601=CARTESIAN_POINT('Ctrl Pts',(1.53670704324243,0.636309800095206,2.50949324534551));
#47602=CARTESIAN_POINT('Ctrl Pts',(1.53257526769918,0.79477268400084,2.43527116374883));
#47603=CARTESIAN_POINT('Ctrl Pts',(1.55708435379909,1.06847604194523,2.40155144628542));
#47604=CARTESIAN_POINT('Ctrl Pts',(1.57504122138999,1.18514270861202,2.40141459471864));
#47605=CARTESIAN_POINT('Ctrl Pts',(1.60034588135027,1.30000000000036,2.41573690783635));
#47606=CARTESIAN_POINT('Ctrl Pts',(1.83480870568655,-1.30000000000158,2.51254415305696));
#47607=CARTESIAN_POINT('Ctrl Pts',(1.79771081770392,-1.18514270861285,2.49446577697444));
#47608=CARTESIAN_POINT('Ctrl Pts',(1.7646139198211,-1.06847604194566,2.48964618907725));
#47609=CARTESIAN_POINT('Ctrl Pts',(1.69739655222609,-0.794772684000851,
2.50914242999906));
#47610=CARTESIAN_POINT('Ctrl Pts',(1.66749164590163,-0.636309800095196,
2.57193910873708));
#47611=CARTESIAN_POINT('Ctrl Pts',(1.61694123862426,-0.319434907277159,
2.62615319012968));
#47612=CARTESIAN_POINT('Ctrl Pts',(1.59850372071989,-0.158333333333332,
2.66748833124109));
#47613=CARTESIAN_POINT('Ctrl Pts',(1.56691293506486,0.158333333333334,2.65657729849294));
#47614=CARTESIAN_POINT('Ctrl Pts',(1.55242668624754,0.319434907277167,2.60393320297167));
#47615=CARTESIAN_POINT('Ctrl Pts',(1.54134412421265,0.636309800095206,2.52830467126513));
#47616=CARTESIAN_POINT('Ctrl Pts',(1.53729692887853,0.79477268400084,2.45450733583496));
#47617=CARTESIAN_POINT('Ctrl Pts',(1.5613175325965,1.06847604194523,2.41822774050965));
#47618=CARTESIAN_POINT('Ctrl Pts',(1.57888716167955,1.18514270861202,2.41633877452248));
#47619=CARTESIAN_POINT('Ctrl Pts',(1.60362879054724,1.30000000000036,2.42826493507295));
#47620=CARTESIAN_POINT('Ctrl Pts',(1.83708905662232,-1.30000000000159,2.53102448418581));
#47621=CARTESIAN_POINT('Ctrl Pts',(1.80136229993117,-1.18514270861286,2.51667909267183));
#47622=CARTESIAN_POINT('Ctrl Pts',(1.76913700894575,-1.06847604194566,2.51456415552258));
#47623=CARTESIAN_POINT('Ctrl Pts',(1.70277922636828,-0.79477268400085,2.53793302389257));
#47624=CARTESIAN_POINT('Ctrl Pts',(1.67135187920676,-0.636309800095195,
2.59978957685925));
#47625=CARTESIAN_POINT('Ctrl Pts',(1.62065406220172,-0.319434907277157,
2.65407625952769));
#47626=CARTESIAN_POINT('Ctrl Pts',(1.60262224066089,-0.158333333333332,
2.69434883567948));
#47627=CARTESIAN_POINT('Ctrl Pts',(1.57157649537649,0.158333333333334,2.68350638536189));
#47628=CARTESIAN_POINT('Ctrl Pts',(1.55748072036052,0.319434907277169,2.63204434634934));
#47629=CARTESIAN_POINT('Ctrl Pts',(1.54714424273508,0.636309800095207,2.55637921263097));
#47630=CARTESIAN_POINT('Ctrl Pts',(1.54431044423645,0.794772684000837,2.48337485439851));
#47631=CARTESIAN_POINT('Ctrl Pts',(1.56766279786463,1.06847604194523,2.44325716475985));
#47632=CARTESIAN_POINT('Ctrl Pts',(1.58448661498275,1.18514270861202,2.4387111168812));
#47633=CARTESIAN_POINT('Ctrl Pts',(1.60802588062332,1.30000000000036,2.44698448246157));
#47634=CARTESIAN_POINT('Ctrl Pts',(1.84208384966657,-1.30000000000158,2.56820316470835));
#47635=CARTESIAN_POINT('Ctrl Pts',(1.80706459881987,-1.18514270861285,2.5609412208685));
#47636=CARTESIAN_POINT('Ctrl Pts',(1.77543875409267,-1.06847604194566,2.5640181209671));
#47637=CARTESIAN_POINT('Ctrl Pts',(1.71021617302907,-0.794772684000848,
2.59501117350305));
#47638=CARTESIAN_POINT('Ctrl Pts',(1.67940607667781,-0.636309800095195,
2.65565089492229));
#47639=CARTESIAN_POINT('Ctrl Pts',(1.62893197543394,-0.319434907277158,
2.71017957772096));
#47640=CARTESIAN_POINT('Ctrl Pts',(1.60964708250435,-0.158333333333332,
2.74796538391066));
#47641=CARTESIAN_POINT('Ctrl Pts',(1.57962478506506,0.158333333333334,2.73725048261268));
#47642=CARTESIAN_POINT('Ctrl Pts',(1.56789372642441,0.319434907277167,2.68842722179615));
#47643=CARTESIAN_POINT('Ctrl Pts',(1.55923857138086,0.636309800095206,2.61273007445824));
#47644=CARTESIAN_POINT('Ctrl Pts',(1.55766344329217,0.794772684000837,2.54114139165139));
#47645=CARTESIAN_POINT('Ctrl Pts',(1.57949120126525,1.06847604194523,2.49328676282195));
#47646=CARTESIAN_POINT('Ctrl Pts',(1.5949086741531,1.18514270861202,2.4834158670341));
#47647=CARTESIAN_POINT('Ctrl Pts',(1.61629519230038,1.30000000000036,2.48438857108989));
#47648=CARTESIAN_POINT('Ctrl Pts',(1.84604424837343,-1.30000000000159,2.60515943272698));
#47649=CARTESIAN_POINT('Ctrl Pts',(1.81265507118371,-1.18514270861286,2.60519420663172));
#47650=CARTESIAN_POINT('Ctrl Pts',(1.7820979101349,-1.06847604194566,2.61358217824961));
#47651=CARTESIAN_POINT('Ctrl Pts',(1.71804727900156,-0.794772684000849,
2.65225762846366));
#47652=CARTESIAN_POINT('Ctrl Pts',(1.68577242078289,-0.636309800095195,
2.71129624843233));
#47653=CARTESIAN_POINT('Ctrl Pts',(1.63510774945675,-0.319434907277157,
2.76600019642908));
#47654=CARTESIAN_POINT('Ctrl Pts',(1.61578764048504,-0.158333333333332,
2.80150232629752));
#47655=CARTESIAN_POINT('Ctrl Pts',(1.58658890630827,0.158333333333334,2.79090471741053));
#47656=CARTESIAN_POINT('Ctrl Pts',(1.5757909659052,0.319434907277168,2.74451319525997));
#47657=CARTESIAN_POINT('Ctrl Pts',(1.56885249695731,0.636309800095206,2.66881702278035));
#47658=CARTESIAN_POINT('Ctrl Pts',(1.56982933223661,0.794772684000836,2.59888504417254));
#47659=CARTESIAN_POINT('Ctrl Pts',(1.59088502566213,1.06847604194523,2.54339135656419));
#47660=CARTESIAN_POINT('Ctrl Pts',(1.60513301753012,1.18514270861202,2.52820947633891));
#47661=CARTESIAN_POINT('Ctrl Pts',(1.62451477177252,1.30000000000036,2.52186687701023));
#47662=CARTESIAN_POINT('Ctrl Pts',(1.84998087442497,-1.30000000000158,2.64821750022589));
#47663=CARTESIAN_POINT('Ctrl Pts',(1.81753200576564,-1.18514270861285,2.65660597517614));
#47664=CARTESIAN_POINT('Ctrl Pts',(1.78756580934509,-1.06847604194566,2.67108144134482));
#47665=CARTESIAN_POINT('Ctrl Pts',(1.72407337042516,-0.794772684000847,
2.71858483141443));
#47666=CARTESIAN_POINT('Ctrl Pts',(1.69097357813135,-0.636309800095194,
2.77590746151336));
#47667=CARTESIAN_POINT('Ctrl Pts',(1.6396390517662,-0.319434907277157,2.8307265598103));
#47668=CARTESIAN_POINT('Ctrl Pts',(1.61879549410128,-0.158333333333332,
2.8632678771389));
#47669=CARTESIAN_POINT('Ctrl Pts',(1.59100525666869,0.158333333333334,2.85291518025025));
#47670=CARTESIAN_POINT('Ctrl Pts',(1.58380273704812,0.319434907277168,2.80987293931332));
#47671=CARTESIAN_POINT('Ctrl Pts',(1.57905167808586,0.636309800095206,2.7342680700284));
#47672=CARTESIAN_POINT('Ctrl Pts',(1.58039437267368,0.794772684000836,2.66585860404003));
#47673=CARTESIAN_POINT('Ctrl Pts',(1.60065206700527,1.06847604194523,2.60143225534537));
#47674=CARTESIAN_POINT('Ctrl Pts',(1.61409160529326,1.18514270861202,2.58011164689002));
#47675=CARTESIAN_POINT('Ctrl Pts',(1.63220187661463,1.30000000000036,2.56535820909775));
#47676=CARTESIAN_POINT('Ctrl Pts',(1.85283044901602,-1.30000000000159,2.68504538799601));
#47677=CARTESIAN_POINT('Ctrl Pts',(1.82102164246291,-1.18514270861286,2.70057949214545));
#47678=CARTESIAN_POINT('Ctrl Pts',(1.79142664860177,-1.06847604194566,2.72025750609338));
#47679=CARTESIAN_POINT('Ctrl Pts',(1.72817064251467,-0.794772684000851,
2.77529091550702));
#47680=CARTESIAN_POINT('Ctrl Pts',(1.69393483689088,-0.636309800095194,
2.83103592248963));
#47681=CARTESIAN_POINT('Ctrl Pts',(1.64263881365639,-0.319434907277156,
2.88607524331724));
#47682=CARTESIAN_POINT('Ctrl Pts',(1.62241952480379,-0.158333333333332,
2.91646130213644));
#47683=CARTESIAN_POINT('Ctrl Pts',(1.59539294034557,0.158333333333334,2.90625956285633));
#47684=CARTESIAN_POINT('Ctrl Pts',(1.58827489522903,0.319434907277167,2.86554585249684));
#47685=CARTESIAN_POINT('Ctrl Pts',(1.58515268627984,0.636309800095205,2.7899827975132));
#47686=CARTESIAN_POINT('Ctrl Pts',(1.58941187234875,0.794772684000835,2.7233635989376));
#47687=CARTESIAN_POINT('Ctrl Pts',(1.60959927129965,1.06847604194523,2.65137578211948));
#47688=CARTESIAN_POINT('Ctrl Pts',(1.62226556377947,1.18514270861202,2.62476489268611));
#47689=CARTESIAN_POINT('Ctrl Pts',(1.63885977175013,1.30000000000036,2.60270397230846));
#47690=CARTESIAN_POINT('Ctrl Pts',(1.85568448251895,-1.30000000000158,2.72795645097212));
#47691=CARTESIAN_POINT('Ctrl Pts',(1.82400623592181,-1.18514270861285,2.75170204140675));
#47692=CARTESIAN_POINT('Ctrl Pts',(1.79437245874033,-1.06847604194566,2.7773548944478));
#47693=CARTESIAN_POINT('Ctrl Pts',(1.73063563857937,-0.794772684000848,
2.84102427497556));
#47694=CARTESIAN_POINT('Ctrl Pts',(1.69534203274488,-0.636309800095195,
2.89499257118523));
#47695=CARTESIAN_POINT('Ctrl Pts',(1.64333947637977,-0.319434907277158,
2.95013761791124));
#47696=CARTESIAN_POINT('Ctrl Pts',(1.62231051404587,-0.158333333333332,
2.97767872212522));
#47697=CARTESIAN_POINT('Ctrl Pts',(1.59665261097123,0.158333333333334,2.96776928219619));
#47698=CARTESIAN_POINT('Ctrl Pts',(1.59219559290535,0.319434907277166,2.9303281940625));
#47699=CARTESIAN_POINT('Ctrl Pts',(1.59158465402795,0.636309800095205,2.85497907049425));
#47700=CARTESIAN_POINT('Ctrl Pts',(1.59748032345738,0.794772684000837,2.79013949145928));
#47701=CARTESIAN_POINT('Ctrl Pts',(1.6176228019188,1.06847604194523,2.70931450316173));
#47702=CARTESIAN_POINT('Ctrl Pts',(1.62969374557501,1.18514270861202,2.67656520456593));
#47703=CARTESIAN_POINT('Ctrl Pts',(1.64511670031386,1.30000000000037,2.64605274994738));
#47704=CARTESIAN_POINT('Ctrl Pts',(1.85622336316529,-1.30000000000159,2.76429054728891));
#47705=CARTESIAN_POINT('Ctrl Pts',(1.82459438932158,-1.18514270861286,2.79509037064409));
#47706=CARTESIAN_POINT('Ctrl Pts',(1.79488348319445,-1.06847604194566,2.82587338111097));
#47707=CARTESIAN_POINT('Ctrl Pts',(1.73067646652796,-0.794772684000851,
2.89694945227406));
#47708=CARTESIAN_POINT('Ctrl Pts',(1.6944354202499,-0.636309800095195,2.94935338210611));
#47709=CARTESIAN_POINT('Ctrl Pts',(1.64196761075382,-0.319434907277157,
3.00461008517178));
#47710=CARTESIAN_POINT('Ctrl Pts',(1.62068829545789,-0.158333333333332,
3.02979545220595));
#47711=CARTESIAN_POINT('Ctrl Pts',(1.59599470275176,0.158333333333334,3.02012457153028));
#47712=CARTESIAN_POINT('Ctrl Pts',(1.59284709103715,0.319434907277166,2.9853361056183));
#47713=CARTESIAN_POINT('Ctrl Pts',(1.59447265136719,0.636309800095204,2.91024244830098));
#47714=CARTESIAN_POINT('Ctrl Pts',(1.60259838285294,0.794772684000836,2.84714880964597));
#47715=CARTESIAN_POINT('Ctrl Pts',(1.62359037912186,1.06847604194523,2.75892429854575));
#47716=CARTESIAN_POINT('Ctrl Pts',(1.63556204596999,1.18514270861202,2.72097797593921));
#47717=CARTESIAN_POINT('Ctrl Pts',(1.65041872231155,1.30000000000036,2.6832744525411));
#47718=CARTESIAN_POINT('Ctrl Pts',(1.857207086575,-1.30000000000158,2.79473457766695));
#47719=CARTESIAN_POINT('Ctrl Pts',(1.82542798871702,-1.18514270861285,2.8313660125812));
#47720=CARTESIAN_POINT('Ctrl Pts',(1.79546058671256,-1.06847604194566,2.86637726826988));
#47721=CARTESIAN_POINT('Ctrl Pts',(1.73041527297429,-0.79477268400085,2.94351733476144));
#47722=CARTESIAN_POINT('Ctrl Pts',(1.69314276881944,-0.636309800095195,
2.99456124033277));
#47723=CARTESIAN_POINT('Ctrl Pts',(1.6397571931075,-0.319434907277157,3.04978086545143));
#47724=CARTESIAN_POINT('Ctrl Pts',(1.61779302863138,-0.158333333333332,
3.0728752244211));
#47725=CARTESIAN_POINT('Ctrl Pts',(1.59373174494822,0.158333333333334,3.06337604168251));
#47726=CARTESIAN_POINT('Ctrl Pts',(1.5920538524928,0.319434907277168,3.0309169560778));
#47727=CARTESIAN_POINT('Ctrl Pts',(1.59557439110431,0.636309800095206,2.95607430228268));
#47728=CARTESIAN_POINT('Ctrl Pts',(1.60528194200455,0.794772684000837,2.89439692122911));
#47729=CARTESIAN_POINT('Ctrl Pts',(1.6270284050152,1.06847604194523,2.80001408481769));
#47730=CARTESIAN_POINT('Ctrl Pts',(1.63899835050215,1.18514270861202,2.75774584268978));
#47731=CARTESIAN_POINT('Ctrl Pts',(1.65352500342459,1.30000000000036,2.7140641910877));
#47732=CARTESIAN_POINT('Ctrl Pts',(1.85717700294372,-1.30000000000158,2.82191251964817));
#47733=CARTESIAN_POINT('Ctrl Pts',(1.82467587459935,-1.18514270861285,2.86364814232314));
#47734=CARTESIAN_POINT('Ctrl Pts',(1.79409818749479,-1.06847604194566,2.90237027513821));
#47735=CARTESIAN_POINT('Ctrl Pts',(1.72790114728519,-0.794772684000848,
2.984864383854));
#47736=CARTESIAN_POINT('Ctrl Pts',(1.69002123908542,-0.636309800095195,
3.03475059042299));
#47737=CARTESIAN_POINT('Ctrl Pts',(1.63639307143117,-0.319434907277158,
3.09007880359328));
#47738=CARTESIAN_POINT('Ctrl Pts',(1.61478134544028,-0.158333333333332,
3.11153331731544));
#47739=CARTESIAN_POINT('Ctrl Pts',(1.59142418067489,0.158333333333334,3.10223802430183));
#47740=CARTESIAN_POINT('Ctrl Pts',(1.59008685968969,0.319434907277168,3.07165441116577));
#47741=CARTESIAN_POINT('Ctrl Pts',(1.59530685793716,0.636309800095207,2.99705383101375));
#47742=CARTESIAN_POINT('Ctrl Pts',(1.60699177532695,0.794772684000838,2.93680522299654));
#47743=CARTESIAN_POINT('Ctrl Pts',(1.63015295398593,1.06847604194523,2.83703937527365));
#47744=CARTESIAN_POINT('Ctrl Pts',(1.64249491695268,1.18514270861202,2.79095403592265));
#47745=CARTESIAN_POINT('Ctrl Pts',(1.65715322685094,1.30000000000036,2.74196829601092));
#47746=CARTESIAN_POINT('Ctrl Pts',(1.85685021732899,-1.30000000000159,2.8459911937542));
#47747=CARTESIAN_POINT('Ctrl Pts',(1.82383248374052,-1.18514270861286,2.89229117867176));
#47748=CARTESIAN_POINT('Ctrl Pts',(1.79276864095702,-1.06847604194566,2.93432330112572));
#47749=CARTESIAN_POINT('Ctrl Pts',(1.7255188284608,-0.794772684000849,3.02156629641757));
#47750=CARTESIAN_POINT('Ctrl Pts',(1.68687937034418,-0.636309800095198,
3.07036965871352));
#47751=CARTESIAN_POINT('Ctrl Pts',(1.63270555281764,-0.31943490727716,3.12571658143093));
#47752=CARTESIAN_POINT('Ctrl Pts',(1.61095676665338,-0.158333333333332,
3.14560901566983));
#47753=CARTESIAN_POINT('Ctrl Pts',(1.58829227266957,0.158333333333335,3.13651452669914));
#47754=CARTESIAN_POINT('Ctrl Pts',(1.58800405119919,0.319434907277168,3.10777322024674));
#47755=CARTESIAN_POINT('Ctrl Pts',(1.59473378186573,0.636309800095208,3.03340117467158));
#47756=CARTESIAN_POINT('Ctrl Pts',(1.60757909381203,0.794772684000842,2.97429514916649));
#47757=CARTESIAN_POINT('Ctrl Pts',(1.63156930313847,1.06847604194524,2.86966720804095));
#47758=CARTESIAN_POINT('Ctrl Pts',(1.64407815725073,1.18514270861202,2.82016190187009));
#47759=CARTESIAN_POINT('Ctrl Pts',(1.65871139278271,1.30000000000037,2.76644084839432));
#47760=CARTESIAN_POINT('Ctrl Pts',(1.85632123702933,-1.30000000000158,2.87004577464627));
#47761=CARTESIAN_POINT('Ctrl Pts',(1.82289752895431,-1.18514270861285,2.92096474537703));
#47762=CARTESIAN_POINT('Ctrl Pts',(1.79130358243341,-1.06847604194566,2.96630756421251));
#47763=CARTESIAN_POINT('Ctrl Pts',(1.7225423608555,-0.79477268400085,3.05817652013863));
#47764=CARTESIAN_POINT('Ctrl Pts',(1.68217109548419,-0.636309800095197,
3.10558863656927));
#47765=CARTESIAN_POINT('Ctrl Pts',(1.62677583236554,-0.319434907277159,
3.16074074995168));
#47766=CARTESIAN_POINT('Ctrl Pts',(1.60463331238041,-0.158333333333332,
3.17896989237942));
#47767=CARTESIAN_POINT('Ctrl Pts',(1.58286022960558,0.158333333333334,3.17015830327284));
#47768=CARTESIAN_POINT('Ctrl Pts',(1.58429600192276,0.319434907277167,3.14352493427863));
#47769=CARTESIAN_POINT('Ctrl Pts',(1.59316901530902,0.636309800095206,3.0695944801784));
#47770=CARTESIAN_POINT('Ctrl Pts',(1.60733848366096,0.794772684000841,3.0116791930089));
#47771=CARTESIAN_POINT('Ctrl Pts',(1.63271777493486,1.06847604194523,2.90230191173186));
#47772=CARTESIAN_POINT('Ctrl Pts',(1.64566487291264,1.18514270861202,2.84941986813064));
#47773=CARTESIAN_POINT('Ctrl Pts',(1.66057331407115,1.30000000000036,2.79100115316534));
#47774=CARTESIAN_POINT('Ctrl Pts',(1.85516825338194,-1.30000000000158,2.89087649958971));
#47775=CARTESIAN_POINT('Ctrl Pts',(1.82087595531089,-1.18514270861286,2.94566041516319));
#47776=CARTESIAN_POINT('Ctrl Pts',(1.78858547647656,-1.06847604194566,2.99381213551726));
#47777=CARTESIAN_POINT('Ctrl Pts',(1.71861261358064,-0.794772684000852,
3.08973054453065));
#47778=CARTESIAN_POINT('Ctrl Pts',(1.67807038790798,-0.636309800095199,
3.13632039877109));
#47779=CARTESIAN_POINT('Ctrl Pts',(1.62205182879722,-0.31943490727716,3.19142725953791));
#47780=CARTESIAN_POINT('Ctrl Pts',(1.59928535208654,-0.158333333333333,
3.20812244832611));
#47781=CARTESIAN_POINT('Ctrl Pts',(1.57795197742068,0.158333333333335,3.19946181817398));
#47782=CARTESIAN_POINT('Ctrl Pts',(1.58027056397191,0.319434907277167,3.17449190967688));
#47783=CARTESIAN_POINT('Ctrl Pts',(1.59103090675974,0.636309800095207,3.10095789708986));
#47784=CARTESIAN_POINT('Ctrl Pts',(1.60701735092504,0.794772684000845,3.04427403233974));
#47785=CARTESIAN_POINT('Ctrl Pts',(1.63400377214994,1.06847604194524,2.93087831801372));
#47786=CARTESIAN_POINT('Ctrl Pts',(1.64746113010348,1.18514270861202,2.87509346701162));
#47787=CARTESIAN_POINT('Ctrl Pts',(1.66269442420776,1.30000000000036,2.81260856801387));
#47788=CARTESIAN_POINT('Ctrl Pts',(1.85462998338906,-1.30000000000158,2.91496806145136));
#47789=CARTESIAN_POINT('Ctrl Pts',(1.81953039247779,-1.18514270861285,2.97428674730439));
#47790=CARTESIAN_POINT('Ctrl Pts',(1.78634444060864,-1.06847604194566,3.02566290057692));
#47791=CARTESIAN_POINT('Ctrl Pts',(1.71409914197363,-0.794772684000847,
3.1260032532413));
#47792=CARTESIAN_POINT('Ctrl Pts',(1.67107866881396,-0.636309800095196,
3.17094188573005));
#47793=CARTESIAN_POINT('Ctrl Pts',(1.61397295051063,-0.319434907277159,
3.22588933174316));
#47794=CARTESIAN_POINT('Ctrl Pts',(1.592195308861,-0.158333333333332,3.2413322754696));
#47795=CARTESIAN_POINT('Ctrl Pts',(1.57169749085167,0.158333333333334,3.23296778748139));
#47796=CARTESIAN_POINT('Ctrl Pts',(1.57436968834082,0.319434907277168,3.20974009366222));
#47797=CARTESIAN_POINT('Ctrl Pts',(1.5868866619752,0.636309800095207,3.13657390352965));
#47798=CARTESIAN_POINT('Ctrl Pts',(1.60481301503526,0.79477268400084,3.08129510338653));
#47799=CARTESIAN_POINT('Ctrl Pts',(1.63333994150167,1.06847604194523,2.96318319881582));
#47800=CARTESIAN_POINT('Ctrl Pts',(1.64725309423382,1.18514270861202,2.90400893539306));
#47801=CARTESIAN_POINT('Ctrl Pts',(1.66273115025762,1.30000000000036,2.83678667555881));
#47802=CARTESIAN_POINT('Ctrl Pts',(1.85283789437504,-1.30000000000158,2.93865027657442));
#47803=CARTESIAN_POINT('Ctrl Pts',(1.81651535992032,-1.18514270861285,3.00230228436277));
#47804=CARTESIAN_POINT('Ctrl Pts',(1.78225631473781,-1.06847604194566,3.05678785253886));
#47805=CARTESIAN_POINT('Ctrl Pts',(1.7078781398863,-0.794772684000851,3.16148410558165));
#47806=CARTESIAN_POINT('Ctrl Pts',(1.66383344619413,-0.636309800095199,
3.20518100870501));
#47807=CARTESIAN_POINT('Ctrl Pts',(1.60550325438214,-0.319434907277161,
3.25989184272619));
#47808=CARTESIAN_POINT('Ctrl Pts',(1.58317021770743,-0.158333333333333,
3.27362635495152));
#47809=CARTESIAN_POINT('Ctrl Pts',(1.56321488157999,0.158333333333335,3.2654805698432));
#47810=CARTESIAN_POINT('Ctrl Pts',(1.56698735291969,0.319434907277167,3.24422596096697));
#47811=CARTESIAN_POINT('Ctrl Pts',(1.5818289141946,0.636309800095207,3.17164826685943));
#47812=CARTESIAN_POINT('Ctrl Pts',(1.60165137239488,0.794772684000844,3.11781961864775));
#47813=CARTESIAN_POINT('Ctrl Pts',(1.63273513266472,1.06847604194524,2.99535467018597));
#47814=CARTESIAN_POINT('Ctrl Pts',(1.64772022370997,1.18514270861202,2.93299760235517));
#47815=CARTESIAN_POINT('Ctrl Pts',(1.66423539774648,1.30000000000037,2.86129400510915));
#47816=CARTESIAN_POINT('Ctrl Pts',(1.85121289296214,-1.30000000000158,2.95640735550508));
#47817=CARTESIAN_POINT('Ctrl Pts',(1.81413477572799,-1.18514270861286,3.0235044952298));
#47818=CARTESIAN_POINT('Ctrl Pts',(1.77903315218445,-1.06847604194566,3.08041661645333));
#47819=CARTESIAN_POINT('Ctrl Pts',(1.70250747556487,-0.794772684000852,
3.18836557146659));
#47820=CARTESIAN_POINT('Ctrl Pts',(1.6555293296576,-0.636309800095198,3.23041432047932));
#47821=CARTESIAN_POINT('Ctrl Pts',(1.59729653296459,-0.31943490727716,3.28530599267342));
#47822=CARTESIAN_POINT('Ctrl Pts',(1.57846605784173,-0.158333333333333,
3.29900685886699));
#47823=CARTESIAN_POINT('Ctrl Pts',(1.55960322480628,0.158333333333335,3.29126031404149));
#47824=CARTESIAN_POINT('Ctrl Pts',(1.56162134457333,0.319434907277168,3.27069541427598));
#47825=CARTESIAN_POINT('Ctrl Pts',(1.577255233148,0.636309800095208,3.19822697616151));
#47826=CARTESIAN_POINT('Ctrl Pts',(1.59906096221992,0.794772684000844,3.14564581967966));
#47827=CARTESIAN_POINT('Ctrl Pts',(1.63183545096121,1.06847604194524,3.01969470358375));
#47828=CARTESIAN_POINT('Ctrl Pts',(1.6474613512956,1.18514270861202,2.95480772724551));
#47829=CARTESIAN_POINT('Ctrl Pts',(1.66452629020275,1.30000000000036,2.87955334577817));
#47830=CARTESIAN_POINT('Ctrl Pts',(1.84997378187141,-1.30000000000158,2.971121535271));
#47831=CARTESIAN_POINT('Ctrl Pts',(1.81142637195795,-1.18514270861286,3.04058194767826));
#47832=CARTESIAN_POINT('Ctrl Pts',(1.77544026524582,-1.06847604194566,3.09927690703692));
#47833=CARTESIAN_POINT('Ctrl Pts',(1.69822228252699,-0.794772684000854,
3.21000365487782));
#47834=CARTESIAN_POINT('Ctrl Pts',(1.6530599183159,-0.636309800095197,3.25206334932354));
#47835=CARTESIAN_POINT('Ctrl Pts',(1.5956337929535,-0.319434907277159,3.30725099401256));
#47836=CARTESIAN_POINT('Ctrl Pts',(1.57732859396373,-0.158333333333332,
3.32013355742912));
#47837=CARTESIAN_POINT('Ctrl Pts',(1.55787980380818,0.158333333333335,3.31221462904587));
#47838=CARTESIAN_POINT('Ctrl Pts',(1.55791689148717,0.319434907277168,3.2920206154993));
#47839=CARTESIAN_POINT('Ctrl Pts',(1.57332227386698,0.636309800095207,3.21946529441339));
#47840=CARTESIAN_POINT('Ctrl Pts',(1.59644561705645,0.794772684000841,3.16791019272484));
#47841=CARTESIAN_POINT('Ctrl Pts',(1.63037248672539,1.06847604194523,3.03929244319824));
#47842=CARTESIAN_POINT('Ctrl Pts',(1.64651775933953,1.18514270861202,2.97247319594244));
#47843=CARTESIAN_POINT('Ctrl Pts',(1.66412261980254,1.30000000000036,2.89450855944361));
#47844=CARTESIAN_POINT('Ctrl Pts',(1.84769026538624,-1.30000000000158,2.98867205329444));
#47845=CARTESIAN_POINT('Ctrl Pts',(1.80728079128909,-1.18514270861285,3.06133928403981));
#47846=CARTESIAN_POINT('Ctrl Pts',(1.77031963716493,-1.06847604194566,3.12252412237443));
#47847=CARTESIAN_POINT('Ctrl Pts',(1.6928982860564,-0.794772684000852,3.23734671539853));
#47848=CARTESIAN_POINT('Ctrl Pts',(1.65105800544677,-0.636309800095197,
3.27993182337879));
#47849=CARTESIAN_POINT('Ctrl Pts',(1.59562625196975,-0.319434907277159,
3.3359607193907));
#47850=CARTESIAN_POINT('Ctrl Pts',(1.57813532525437,-0.158333333333332,
3.34778863471165));
#47851=CARTESIAN_POINT('Ctrl Pts',(1.55878655683849,0.158333333333335,3.33992605458163));
#47852=CARTESIAN_POINT('Ctrl Pts',(1.55779869358718,0.319434907277167,3.32076037305399));
#47853=CARTESIAN_POINT('Ctrl Pts',(1.57204631549811,0.636309800095207,3.24764695926783));
#47854=CARTESIAN_POINT('Ctrl Pts',(1.59359769213642,0.794772684000841,3.19612014661867));
#47855=CARTESIAN_POINT('Ctrl Pts',(1.62791108705985,1.06847604194523,3.06340873206302));
#47856=CARTESIAN_POINT('Ctrl Pts',(1.64472849376649,1.18514270861202,2.99396552178466));
#47857=CARTESIAN_POINT('Ctrl Pts',(1.66351030995401,1.30000000000036,2.91252495514655));
#47858=CARTESIAN_POINT('Ctrl Pts',(1.84624880074941,-1.30000000000158,3.00065723247174));
#47859=CARTESIAN_POINT('Ctrl Pts',(1.80327012405171,-1.18514270861285,3.07509490657786));
#47860=CARTESIAN_POINT('Ctrl Pts',(1.76517783186741,-1.06847604194566,3.13773291842763));
#47861=CARTESIAN_POINT('Ctrl Pts',(1.68846554232873,-0.794772684000851,
3.2551796761652));
#47862=CARTESIAN_POINT('Ctrl Pts',(1.65309822965784,-0.636309800095196,
3.29877447145925));
#47863=CARTESIAN_POINT('Ctrl Pts',(1.60107891377445,-0.319434907277159,
3.35545738171415));
#47864=CARTESIAN_POINT('Ctrl Pts',(1.58369000879615,-0.158333333333332,
3.3662154292582));
#47865=CARTESIAN_POINT('Ctrl Pts',(1.56451256417064,0.158333333333334,3.35836908000967));
#47866=CARTESIAN_POINT('Ctrl Pts',(1.56349013317765,0.319434907277167,3.34018877922963));
#47867=CARTESIAN_POINT('Ctrl Pts',(1.57488586701371,0.636309800095206,3.26665956746972));
#47868=CARTESIAN_POINT('Ctrl Pts',(1.59090434066293,0.79477268400084,3.21470783556925));
#47869=CARTESIAN_POINT('Ctrl Pts',(1.6244481867995,1.06847604194523,3.07934166145306));
#47870=CARTESIAN_POINT('Ctrl Pts',(1.64211927471603,1.18514270861202,3.00828819800809));
#47871=CARTESIAN_POINT('Ctrl Pts',(1.66294156247856,1.30000000000036,2.924776272082));
#47872=CARTESIAN_POINT('Ctrl Pts',(1.84783999216081,-1.30000000000158,3.00911085372598));
#47873=CARTESIAN_POINT('Ctrl Pts',(1.80484358765989,-1.18514270861285,3.08329784479062));
#47874=CARTESIAN_POINT('Ctrl Pts',(1.76706466618288,-1.06847604194566,3.14579189582396));
#47875=CARTESIAN_POINT('Ctrl Pts',(1.69184122946293,-0.794772684000851,
3.26315262496583));
#47876=CARTESIAN_POINT('Ctrl Pts',(1.65901382561028,-0.636309800095196,
3.30711063699039));
#47877=CARTESIAN_POINT('Ctrl Pts',(1.6086720442671,-0.319434907277159,3.36396800272369));
#47878=CARTESIAN_POINT('Ctrl Pts',(1.59125278366871,-0.158333333333332,
3.37476869623928));
#47879=CARTESIAN_POINT('Ctrl Pts',(1.57231214945024,0.158333333333334,3.36692516506795));
#47880=CARTESIAN_POINT('Ctrl Pts',(1.57183510628243,0.319434907277167,3.34873710938264));
#47881=CARTESIAN_POINT('Ctrl Pts',(1.58146895355656,0.636309800095206,3.27497385199526));
#47882=CARTESIAN_POINT('Ctrl Pts',(1.59387972389892,0.79477268400084,3.22247344768589));
#47883=CARTESIAN_POINT('Ctrl Pts',(1.62608364872299,1.06847604194523,3.08723090979032));
#47884=CARTESIAN_POINT('Ctrl Pts',(1.6437543175134,1.18514270861202,3.01638787148176));
#47885=CARTESIAN_POINT('Ctrl Pts',(1.66515576931089,1.30000000000036,2.93324327828973));
#47886=CARTESIAN_POINT('Ctrl Pts',(1.84783999216022,-1.3,3.009110853727));
#47887=CARTESIAN_POINT('Ctrl Pts',(1.80484358765954,-1.18514270861178,3.08329784479119));
#47888=CARTESIAN_POINT('Ctrl Pts',(1.76706466618273,-1.06847604194512,3.1457918958242));
#47889=CARTESIAN_POINT('Ctrl Pts',(1.69184122946293,-0.794772684000851,
3.26315262496584));
#47890=CARTESIAN_POINT('Ctrl Pts',(1.65901382561028,-0.636309800095197,
3.30711063699039));
#47891=CARTESIAN_POINT('Ctrl Pts',(1.6086720442671,-0.319434907277159,3.36396800272368));
#47892=CARTESIAN_POINT('Ctrl Pts',(1.59125278366871,-0.158333333333332,
3.37476869623928));
#47893=CARTESIAN_POINT('Ctrl Pts',(1.57231214945024,0.158333333333334,3.36692516506795));
#47894=CARTESIAN_POINT('Ctrl Pts',(1.57183510628243,0.319434907277167,3.34873710938264));
#47895=CARTESIAN_POINT('Ctrl Pts',(1.58146895355656,0.636309800095206,3.27497385199526));
#47896=CARTESIAN_POINT('Ctrl Pts',(1.59387972389891,0.79477268400084,3.22247344768589));
#47897=CARTESIAN_POINT('Ctrl Pts',(1.62608364872297,1.06847604194511,3.08723090979038));
#47898=CARTESIAN_POINT('Ctrl Pts',(1.64375431751336,1.18514270861178,3.01638787148191));
#47899=CARTESIAN_POINT('Ctrl Pts',(1.66515576931082,1.3,2.93324327828999));
#47900=CARTESIAN_POINT('',(1.8162121882396,-1.2,2.59523363379966));
#47901=CARTESIAN_POINT('Ctrl Pts',(1.8162121882396,-1.2,2.59523363379966));
#47902=CARTESIAN_POINT('Ctrl Pts',(1.82366382114832,-1.21762172383529,2.6171155864293));
#47903=CARTESIAN_POINT('Ctrl Pts',(1.83047749029892,-1.23476275836489,2.63830479398897));
#47904=CARTESIAN_POINT('Ctrl Pts',(1.84184377598764,-1.26421553765088,2.67466690339845));
#47905=CARTESIAN_POINT('Ctrl Pts',(1.84966377084331,-1.28493282003519,2.70024848455808));
#47906=CARTESIAN_POINT('Ctrl Pts',(1.85487686289296,-1.30000000000158,2.71871315094771));
#47907=CARTESIAN_POINT('',(1.66957758855468,-0.653834841386366,2.54006323267476));
#47908=CARTESIAN_POINT('Ctrl Pts',(1.66957758857006,-0.653834841385217,
2.54006323264526));
#47909=CARTESIAN_POINT('Ctrl Pts',(1.6873947828161,-0.728434665160969,2.54644683604794));
#47910=CARTESIAN_POINT('Ctrl Pts',(1.6996738894343,-0.774162846424616,2.55093543968267));
#47911=CARTESIAN_POINT('Ctrl Pts',(1.73768103151109,-0.918719140441923,
2.56495158387815));
#47912=CARTESIAN_POINT('Ctrl Pts',(1.7680361736811,-1.0361514204072,2.57623204764662));
#47913=CARTESIAN_POINT('Ctrl Pts',(1.8162121882396,-1.2,2.59523363379966));
#47914=CARTESIAN_POINT('',(1.53759581372313,0.653834841531101,2.49486460198847));
#47915=CARTESIAN_POINT('Ctrl Pts',(1.53759581372313,0.653834841531102,2.49486460198847));
#47916=CARTESIAN_POINT('Ctrl Pts',(1.54253080068449,0.575902863726212,2.53618577289924));
#47917=CARTESIAN_POINT('Ctrl Pts',(1.54736388103037,0.493640201102665,2.57092573760444));
#47918=CARTESIAN_POINT('Ctrl Pts',(1.55686464232257,0.338190864746863,2.62063165073203));
#47919=CARTESIAN_POINT('Ctrl Pts',(1.56146483259355,0.265716392874933,2.63794716225927));
#47920=CARTESIAN_POINT('Ctrl Pts',(1.57177149979286,0.12975615835201,2.66008608934449));
#47921=CARTESIAN_POINT('Ctrl Pts',(1.57719261268522,0.066649891557159,2.6663551854814));
#47922=CARTESIAN_POINT('Ctrl Pts',(1.58968313431103,-0.0595495593502237,
2.67102603384143));
#47923=CARTESIAN_POINT('Ctrl Pts',(1.59684415233489,-0.122807792517795,
2.66948042211137));
#47924=CARTESIAN_POINT('Ctrl Pts',(1.61355162359461,-0.260168353259011,
2.65721880712717));
#47925=CARTESIAN_POINT('Ctrl Pts',(1.62329765128691,-0.333963506589111,
2.64488766435628));
#47926=CARTESIAN_POINT('Ctrl Pts',(1.6449620096927,-0.49120546185675,2.60562844753539));
#47927=CARTESIAN_POINT('Ctrl Pts',(1.65723414657175,-0.574385269905671,
2.57651514903598));
#47928=CARTESIAN_POINT('Ctrl Pts',(1.66957758858473,-0.65383484140123,2.54006323271733));
#47929=CARTESIAN_POINT('',(1.60611193089494,1.2,2.51780986445051));
#47930=CARTESIAN_POINT('Ctrl Pts',(1.60611193089494,1.2,2.51780986445051));
#47931=CARTESIAN_POINT('Ctrl Pts',(1.58805485708337,1.09750097238566,2.5116158225927));
#47932=CARTESIAN_POINT('Ctrl Pts',(1.57349326241228,0.998393154633832,2.50672903384865));
#47933=CARTESIAN_POINT('Ctrl Pts',(1.55103395914313,0.813752614838904,2.49926560256432));
#47934=CARTESIAN_POINT('Ctrl Pts',(1.5447079032333,0.753887267506067,2.49718876869838));
#47935=CARTESIAN_POINT('Ctrl Pts',(1.53759581372313,0.653834841531101,2.49486460198847));
#47936=CARTESIAN_POINT('Ctrl Pts',(1.6438117816117,1.3,2.63706423159009));
#47937=CARTESIAN_POINT('Ctrl Pts',(1.63803607995104,1.28318156972391,2.61710700275808));
#47938=CARTESIAN_POINT('Ctrl Pts',(1.63190962613203,1.26645607930026,2.59717136778684));
#47939=CARTESIAN_POINT('Ctrl Pts',(1.61573517002289,1.22418846120041,2.54667912684929));
#47940=CARTESIAN_POINT('Ctrl Pts',(1.61410323990346,1.2192547094459,2.54090712136841));
#47941=CARTESIAN_POINT('Ctrl Pts',(1.60611193089494,1.2,2.51780986445051));
#47942=CARTESIAN_POINT('Ctrl Pts',(1.84783999216022,-1.3,3.009110853727));
#47943=CARTESIAN_POINT('Ctrl Pts',(1.80484358765954,-1.18514270861178,3.08329784479119));
#47944=CARTESIAN_POINT('Ctrl Pts',(1.76706466618273,-1.06847604194512,3.1457918958242));
#47945=CARTESIAN_POINT('Ctrl Pts',(1.69184122946293,-0.794772684000851,
3.26315262496583));
#47946=CARTESIAN_POINT('Ctrl Pts',(1.65901382561028,-0.636309800095197,
3.30711063699039));
#47947=CARTESIAN_POINT('Ctrl Pts',(1.6086720442671,-0.319434907277159,3.36396800272369));
#47948=CARTESIAN_POINT('Ctrl Pts',(1.59125278366871,-0.158333333333332,
3.37476869623928));
#47949=CARTESIAN_POINT('Ctrl Pts',(1.57231214945024,0.158333333333334,3.36692516506795));
#47950=CARTESIAN_POINT('Ctrl Pts',(1.57183510628243,0.319434907277167,3.34873710938264));
#47951=CARTESIAN_POINT('Ctrl Pts',(1.58146895355656,0.636309800095206,3.27497385199526));
#47952=CARTESIAN_POINT('Ctrl Pts',(1.59387972389891,0.79477268400084,3.22247344768589));
#47953=CARTESIAN_POINT('Ctrl Pts',(1.62608364872297,1.06847604194511,3.08723090979038));
#47954=CARTESIAN_POINT('Ctrl Pts',(1.64375431751336,1.18514270861178,3.01638787148191));
#47955=CARTESIAN_POINT('Ctrl Pts',(1.66515576931082,1.3,2.93324327828999));
#47956=CARTESIAN_POINT('Ctrl Pts',(1.91743049134307,-1.3,3.04191743383109));
#47957=CARTESIAN_POINT('Ctrl Pts',(1.87294351908302,-1.18514270861178,3.11522175128021));
#47958=CARTESIAN_POINT('Ctrl Pts',(1.83415002075929,-1.06847604194512,3.17706282238686));
#47959=CARTESIAN_POINT('Ctrl Pts',(1.75768234278715,-0.794772684000851,
3.29344567564148));
#47960=CARTESIAN_POINT('Ctrl Pts',(1.72556041438091,-0.636309800095197,
3.33753522603443));
#47961=CARTESIAN_POINT('Ctrl Pts',(1.67587573316224,-0.319434907277159,
3.39427900215457));
#47962=CARTESIAN_POINT('Ctrl Pts',(1.65965103821258,-0.158333333333332,
3.40541802202081));
#47963=CARTESIAN_POINT('Ctrl Pts',(1.64085640284598,0.158333333333334,3.39724657205924));
#47964=CARTESIAN_POINT('Ctrl Pts',(1.6393286137645,0.319434907277167,3.37839716560952));
#47965=CARTESIAN_POINT('Ctrl Pts',(1.64860718876712,0.636309800095206,3.30406958137807));
#47966=CARTESIAN_POINT('Ctrl Pts',(1.66044815183843,0.79477268400084,3.25113292298941));
#47967=CARTESIAN_POINT('Ctrl Pts',(1.69421133997152,1.06847604194511,3.116160709857));
#47968=CARTESIAN_POINT('Ctrl Pts',(1.71304615183609,1.18514270861178,3.0456347202283));
#47969=CARTESIAN_POINT('Ctrl Pts',(1.73610094247183,1.3,2.96300721082251));
#47970=CARTESIAN_POINT('Ctrl Pts',(1.98702099052592,-1.3,3.07472401393519));
#47971=CARTESIAN_POINT('Ctrl Pts',(1.9410434505065,-1.18514270861178,3.14714565776922));
#47972=CARTESIAN_POINT('Ctrl Pts',(1.90123537533586,-1.06847604194512,3.20833374894953));
#47973=CARTESIAN_POINT('Ctrl Pts',(1.82352345611138,-0.794772684000851,
3.32373872631713));
#47974=CARTESIAN_POINT('Ctrl Pts',(1.79210700315155,-0.636309800095197,
3.36795981507847));
#47975=CARTESIAN_POINT('Ctrl Pts',(1.74307942205737,-0.319434907277159,
3.42459000158545));
#47976=CARTESIAN_POINT('Ctrl Pts',(1.72804929275646,-0.158333333333332,
3.43606734780233));
#47977=CARTESIAN_POINT('Ctrl Pts',(1.70940065624172,0.158333333333334,3.42756797905052));
#47978=CARTESIAN_POINT('Ctrl Pts',(1.70682212124656,0.319434907277167,3.4080572218364));
#47979=CARTESIAN_POINT('Ctrl Pts',(1.71574542397769,0.636309800095206,3.33316531076089));
#47980=CARTESIAN_POINT('Ctrl Pts',(1.72701657977794,0.79477268400084,3.27979239829292));
#47981=CARTESIAN_POINT('Ctrl Pts',(1.76233903122006,1.06847604194511,3.14509050992361));
#47982=CARTESIAN_POINT('Ctrl Pts',(1.78233798615881,1.18514270861178,3.07488156897468));
#47983=CARTESIAN_POINT('Ctrl Pts',(1.80704611563284,1.3,2.99277114335502));
#47984=CARTESIAN_POINT('Ctrl Pts',(2.05661148970878,-1.3,3.10753059403929));
#47985=CARTESIAN_POINT('Ctrl Pts',(2.00914338192998,-1.18514270861178,3.17906956425824));
#47986=CARTESIAN_POINT('Ctrl Pts',(1.96832072991242,-1.06847604194512,3.23960467551219));
#47987=CARTESIAN_POINT('Ctrl Pts',(1.8893645694356,-0.794772684000851,3.35403177699278));
#47988=CARTESIAN_POINT('Ctrl Pts',(1.85865359192219,-0.636309800095197,
3.39838440412252));
#47989=CARTESIAN_POINT('Ctrl Pts',(1.8102831109525,-0.319434907277159,3.45490100101634));
#47990=CARTESIAN_POINT('Ctrl Pts',(1.79644754730034,-0.158333333333332,
3.46671667358385));
#47991=CARTESIAN_POINT('Ctrl Pts',(1.77794490963746,0.158333333333334,3.45788938604181));
#47992=CARTESIAN_POINT('Ctrl Pts',(1.77431562872862,0.319434907277167,3.43771727806328));
#47993=CARTESIAN_POINT('Ctrl Pts',(1.78288365918825,0.636309800095206,3.3622610401437));
#47994=CARTESIAN_POINT('Ctrl Pts',(1.79358500771746,0.79477268400084,3.30845187359643));
#47995=CARTESIAN_POINT('Ctrl Pts',(1.8304667224686,1.06847604194511,3.17402030999022));
#47996=CARTESIAN_POINT('Ctrl Pts',(1.85162982048153,1.18514270861178,3.10412841772107));
#47997=CARTESIAN_POINT('Ctrl Pts',(1.87799128879385,1.3,3.02253507588753));
#47998=CARTESIAN_POINT('Ctrl Pts',(2.05661148970878,-1.3,3.10753059403928));
#47999=CARTESIAN_POINT('Ctrl Pts',(2.00914338192998,-1.18514270861178,3.17906956425824));
#48000=CARTESIAN_POINT('Ctrl Pts',(1.96832072991242,-1.06847604194512,3.23960467551219));
#48001=CARTESIAN_POINT('Ctrl Pts',(1.8893645694356,-0.794772684000851,3.35403177699278));
#48002=CARTESIAN_POINT('Ctrl Pts',(1.85865359192218,-0.636309800095197,
3.39838440412251));
#48003=CARTESIAN_POINT('Ctrl Pts',(1.8102831109525,-0.319434907277159,3.45490100101634));
#48004=CARTESIAN_POINT('Ctrl Pts',(1.79644754730033,-0.158333333333332,
3.46671667358385));
#48005=CARTESIAN_POINT('Ctrl Pts',(1.77794490963746,0.158333333333334,3.45788938604181));
#48006=CARTESIAN_POINT('Ctrl Pts',(1.77431562872862,0.319434907277167,3.43771727806327));
#48007=CARTESIAN_POINT('Ctrl Pts',(1.78288365918825,0.636309800095206,3.36226104014369));
#48008=CARTESIAN_POINT('Ctrl Pts',(1.79358500771746,0.79477268400084,3.30845187359643));
#48009=CARTESIAN_POINT('Ctrl Pts',(1.8304667224686,1.06847604194511,3.17402030999022));
#48010=CARTESIAN_POINT('Ctrl Pts',(1.85162982048153,1.18514270861178,3.10412841772107));
#48011=CARTESIAN_POINT('Ctrl Pts',(1.87799128879385,1.3,3.02253507588753));
#48012=CARTESIAN_POINT('Ctrl Pts',(2.05661148970879,-1.30000000000002,3.10753059403927));
#48013=CARTESIAN_POINT('Ctrl Pts',(2.00914338192999,-1.18514270861179,3.17906956425823));
#48014=CARTESIAN_POINT('Ctrl Pts',(1.96832072991242,-1.06847604194512,3.23960467551219));
#48015=CARTESIAN_POINT('Ctrl Pts',(1.8893645694356,-0.794772684000851,3.35403177699278));
#48016=CARTESIAN_POINT('Ctrl Pts',(1.85865359192218,-0.636309800095197,
3.39838440412251));
#48017=CARTESIAN_POINT('Ctrl Pts',(1.8102831109525,-0.319434907277159,3.45490100101634));
#48018=CARTESIAN_POINT('Ctrl Pts',(1.79644754730034,-0.158333333333332,
3.46671667358385));
#48019=CARTESIAN_POINT('Ctrl Pts',(1.77794490963746,0.158333333333334,3.45788938604181));
#48020=CARTESIAN_POINT('Ctrl Pts',(1.77431562872862,0.319434907277167,3.43771727806328));
#48021=CARTESIAN_POINT('Ctrl Pts',(1.78288365918825,0.636309800095206,3.36226104014369));
#48022=CARTESIAN_POINT('Ctrl Pts',(1.79358500771746,0.79477268400084,3.30845187359643));
#48023=CARTESIAN_POINT('Ctrl Pts',(1.83046672246867,1.06847604194558,3.17402030998999));
#48024=CARTESIAN_POINT('Ctrl Pts',(1.8516298204817,1.1851427086127,3.10412841772051));
#48025=CARTESIAN_POINT('Ctrl Pts',(1.87799128879416,1.30000000000137,3.02253507588656));
#48026=CARTESIAN_POINT('Ctrl Pts',(2.06438529509424,-1.30000000000002,3.10351053744534));
#48027=CARTESIAN_POINT('Ctrl Pts',(2.0162566695166,-1.18514270861179,3.17486489847698));
#48028=CARTESIAN_POINT('Ctrl Pts',(1.97527792160046,-1.06847604194512,3.23554112309669));
#48029=CARTESIAN_POINT('Ctrl Pts',(1.89712646386989,-0.794772684000851,
3.35104670893996));
#48030=CARTESIAN_POINT('Ctrl Pts',(1.86923725412317,-0.636309800095197,
3.39771324860388));
#48031=CARTESIAN_POINT('Ctrl Pts',(1.82221963516387,-0.319434907277159,
3.45538257530852));
#48032=CARTESIAN_POINT('Ctrl Pts',(1.80802489881759,-0.158333333333332,
3.46678775674664));
#48033=CARTESIAN_POINT('Ctrl Pts',(1.78936170982528,0.158333333333334,3.45778637043419));
#48034=CARTESIAN_POINT('Ctrl Pts',(1.78572104868507,0.319434907277167,3.43766535674272));
#48035=CARTESIAN_POINT('Ctrl Pts',(1.79303694376684,0.636309800095206,3.36107920118311));
#48036=CARTESIAN_POINT('Ctrl Pts',(1.80176883893061,0.79477268400084,3.30562555398019));
#48037=CARTESIAN_POINT('Ctrl Pts',(1.83771824839722,1.06847604194558,3.17002999274191));
#48038=CARTESIAN_POINT('Ctrl Pts',(1.85877864421361,1.1851427086127,3.0998088920672));
#48039=CARTESIAN_POINT('Ctrl Pts',(1.88533826854518,1.30000000000137,3.01806098486724));
#48040=CARTESIAN_POINT('Ctrl Pts',(2.07311117400897,-1.30000000000002,3.09489607890757));
#48041=CARTESIAN_POINT('Ctrl Pts',(2.02516501665969,-1.1851427086118,3.16336132721032));
#48042=CARTESIAN_POINT('Ctrl Pts',(1.98481640679923,-1.06847604194512,3.22233412436262));
#48043=CARTESIAN_POINT('Ctrl Pts',(1.90915490089316,-0.794772684000852,
3.33664362213621));
#48044=CARTESIAN_POINT('Ctrl Pts',(1.88527241428737,-0.636309800095199,
3.38712679647839));
#48045=CARTESIAN_POINT('Ctrl Pts',(1.8404608163555,-0.31943490727716,3.44662850647972));
#48046=CARTESIAN_POINT('Ctrl Pts',(1.82554655027699,-0.158333333333333,
3.45870878172653));
#48047=CARTESIAN_POINT('Ctrl Pts',(1.8067527003081,0.158333333333335,3.44958823116425));
#48048=CARTESIAN_POINT('Ctrl Pts',(1.80384120716332,0.319434907277167,3.4286804811146));
#48049=CARTESIAN_POINT('Ctrl Pts',(1.80839915476674,0.636309800095207,3.35000389209952));
#48050=CARTESIAN_POINT('Ctrl Pts',(1.81207064732138,0.794772684000844,3.29043038686903));
#48051=CARTESIAN_POINT('Ctrl Pts',(1.84559920552924,1.06847604194558,3.15605953551499));
#48052=CARTESIAN_POINT('Ctrl Pts',(1.86633375488223,1.18514270861271,3.08764494368963));
#48053=CARTESIAN_POINT('Ctrl Pts',(1.89328958309553,1.30000000000137,3.00897992265948));
#48054=CARTESIAN_POINT('Ctrl Pts',(2.08606699867076,-1.30000000000002,3.0823702408846));
#48055=CARTESIAN_POINT('Ctrl Pts',(2.0399225376305,-1.1851427086118,3.14764008196292));
#48056=CARTESIAN_POINT('Ctrl Pts',(2.00108022081302,-1.06847604194512,3.20436220961664));
#48057=CARTESIAN_POINT('Ctrl Pts',(1.92821611252933,-0.794772684000853,
3.31565474374453));
#48058=CARTESIAN_POINT('Ctrl Pts',(1.90537613625137,-0.636309800095198,
3.36733137652309));
#48059=CARTESIAN_POINT('Ctrl Pts',(1.861761274782,-0.319434907277159,3.42732370528723));
#48060=CARTESIAN_POINT('Ctrl Pts',(1.84676876171031,-0.158333333333332,
3.44085260987035));
#48061=CARTESIAN_POINT('Ctrl Pts',(1.82785767731739,0.158333333333335,3.43169011688178));
#48062=CARTESIAN_POINT('Ctrl Pts',(1.82516531181488,0.319434907277167,3.40946043194975));
#48063=CARTESIAN_POINT('Ctrl Pts',(1.82776196305616,0.636309800095207,3.32986428928672));
#48064=CARTESIAN_POINT('Ctrl Pts',(1.82884049859466,0.794772684000843,3.26818649332466));
#48065=CARTESIAN_POINT('Ctrl Pts',(1.8594648678336,1.06847604194558,3.13670945384053));
#48066=CARTESIAN_POINT('Ctrl Pts',(1.87900001879695,1.1851427086127,3.07068436435281));
#48067=CARTESIAN_POINT('Ctrl Pts',(1.90481416602479,1.30000000000137,2.99554572406571));
#48068=CARTESIAN_POINT('Ctrl Pts',(2.09696957937698,-1.30000000000002,3.07210722196282));
#48069=CARTESIAN_POINT('Ctrl Pts',(2.05247729144278,-1.1851427086118,3.13516734031299));
#48070=CARTESIAN_POINT('Ctrl Pts',(2.01471700122407,-1.06847604194512,3.19021030643424));
#48071=CARTESIAN_POINT('Ctrl Pts',(1.94303543835297,-0.794772684000852,
3.29884934400734));
#48072=CARTESIAN_POINT('Ctrl Pts',(1.91850752763247,-0.636309800095198,
3.350202946425));
#48073=CARTESIAN_POINT('Ctrl Pts',(1.87507551772266,-0.31943490727716,3.41028477353073));
#48074=CARTESIAN_POINT('Ctrl Pts',(1.86111460420306,-0.158333333333332,
3.42552196248209));
#48075=CARTESIAN_POINT('Ctrl Pts',(1.84273788650679,0.158333333333335,3.4166882437844));
#48076=CARTESIAN_POINT('Ctrl Pts',(1.84035616299712,0.319434907277167,3.39355506649829));
#48077=CARTESIAN_POINT('Ctrl Pts',(1.84221284626722,0.636309800095207,3.31356950122377));
#48078=CARTESIAN_POINT('Ctrl Pts',(1.84204629899775,0.794772684000843,3.25053778242636));
#48079=CARTESIAN_POINT('Ctrl Pts',(1.87106471889265,1.06847604194558,3.12142528052509));
#48080=CARTESIAN_POINT('Ctrl Pts',(1.88986591440082,1.18514270861271,3.05724590643982));
#48081=CARTESIAN_POINT('Ctrl Pts',(1.91490730668305,1.30000000000137,2.98477517625274));
#48082=CARTESIAN_POINT('Ctrl Pts',(2.11058813200125,-1.30000000000002,3.06000397880413));
#48083=CARTESIAN_POINT('Ctrl Pts',(2.06838975835484,-1.1851427086118,3.12029349547214));
#48084=CARTESIAN_POINT('Ctrl Pts',(2.03210944478524,-1.06847604194513,3.17318478598011));
#48085=CARTESIAN_POINT('Ctrl Pts',(1.96196656526888,-0.794772684000854,
3.27828286548025));
#48086=CARTESIAN_POINT('Ctrl Pts',(1.93527184700814,-0.636309800095199,
3.32905154023907));
#48087=CARTESIAN_POINT('Ctrl Pts',(1.89129063602831,-0.31943490727716,3.38865386231255));
#48088=CARTESIAN_POINT('Ctrl Pts',(1.87801052102755,-0.158333333333333,
3.40566442232698));
#48089=CARTESIAN_POINT('Ctrl Pts',(1.85856089011937,0.158333333333335,3.39625770136831));
#48090=CARTESIAN_POINT('Ctrl Pts',(1.85373294313904,0.319434907277168,3.37042335719926));
#48091=CARTESIAN_POINT('Ctrl Pts',(1.85536397707056,0.636309800095208,3.29047282154238));
#48092=CARTESIAN_POINT('Ctrl Pts',(1.85848213792874,0.794772684000844,3.22857764871937));
#48093=CARTESIAN_POINT('Ctrl Pts',(1.88653846927129,1.06847604194558,3.10325347243792));
#48094=CARTESIAN_POINT('Ctrl Pts',(1.90409579177865,1.18514270861271,3.04132415698621));
#48095=CARTESIAN_POINT('Ctrl Pts',(1.92706589054469,1.30000000000137,2.97171371827676));
#48096=CARTESIAN_POINT('Ctrl Pts',(2.12535537170441,-1.30000000000002,3.0487948012942));
#48097=CARTESIAN_POINT('Ctrl Pts',(2.08510457409783,-1.1851427086118,3.10624984240559));
#48098=CARTESIAN_POINT('Ctrl Pts',(2.05000694414467,-1.06847604194513,3.15692071284892));
#48099=CARTESIAN_POINT('Ctrl Pts',(1.98082924586306,-0.794772684000853,
3.25830776883402));
#48100=CARTESIAN_POINT('Ctrl Pts',(1.9521414637683,-0.636309800095201,3.30859414238913));
#48101=CARTESIAN_POINT('Ctrl Pts',(1.9064880593285,-0.319434907277162,3.36708715701643));
#48102=CARTESIAN_POINT('Ctrl Pts',(1.89147447751587,-0.158333333333333,
3.38442963319047));
#48103=CARTESIAN_POINT('Ctrl Pts',(1.87173028908309,0.158333333333335,3.37489183848399));
#48104=CARTESIAN_POINT('Ctrl Pts',(1.86845863131722,0.319434907277168,3.34870687052084));
#48105=CARTESIAN_POINT('Ctrl Pts',(1.8709227717798,0.636309800095209,3.26936977284123));
#48106=CARTESIAN_POINT('Ctrl Pts',(1.87504632164862,0.794772684000847,3.20730369839696));
#48107=CARTESIAN_POINT('Ctrl Pts',(1.90170503351283,1.06847604194559,3.08531301579748));
#48108=CARTESIAN_POINT('Ctrl Pts',(1.91807197012133,1.18514270861271,3.02553340502337));
#48109=CARTESIAN_POINT('Ctrl Pts',(1.93926627477494,1.30000000000138,2.95877942977227));
#48110=CARTESIAN_POINT('Ctrl Pts',(2.14303983420993,-1.30000000000002,3.03242748668085));
#48111=CARTESIAN_POINT('Ctrl Pts',(2.10599477948638,-1.1851427086118,3.0864351878073));
#48112=CARTESIAN_POINT('Ctrl Pts',(2.07304606191122,-1.06847604194513,3.13446164902164));
#48113=CARTESIAN_POINT('Ctrl Pts',(2.00639129122644,-0.794772684000854,
3.23159452134748));
#48114=CARTESIAN_POINT('Ctrl Pts',(1.97578443836247,-0.6363098000952,3.28167480323916));
#48115=CARTESIAN_POINT('Ctrl Pts',(1.92883104153055,-0.319434907277161,
3.33921641080584));
#48116=CARTESIAN_POINT('Ctrl Pts',(1.91222223148185,-0.158333333333333,
3.35741115879828));
#48117=CARTESIAN_POINT('Ctrl Pts',(1.89156185596208,0.158333333333336,3.34736990639073));
#48118=CARTESIAN_POINT('Ctrl Pts',(1.88832568148489,0.319434907277169,3.31948156388352));
#48119=CARTESIAN_POINT('Ctrl Pts',(1.89153448823503,0.63630980009521,3.24077849406139));
#48120=CARTESIAN_POINT('Ctrl Pts',(1.89861717655721,0.794772684000847,3.17947682954823));
#48121=CARTESIAN_POINT('Ctrl Pts',(1.92358245481021,1.06847604194559,3.06216339058198));
#48122=CARTESIAN_POINT('Ctrl Pts',(1.93819516873417,1.18514270861271,3.00522745510929));
#48123=CARTESIAN_POINT('Ctrl Pts',(1.95661405268106,1.30000000000137,2.94213622500118));
#48124=CARTESIAN_POINT('Ctrl Pts',(2.16828207977002,-1.30000000000003,3.01421432900304));
#48125=CARTESIAN_POINT('Ctrl Pts',(2.13543077770946,-1.18514270861181,3.06412297603415));
#48126=CARTESIAN_POINT('Ctrl Pts',(2.10509779364543,-1.06847604194513,3.10885397352754));
#48127=CARTESIAN_POINT('Ctrl Pts',(2.04084035072463,-0.794772684000861,
3.20023011992529));
#48128=CARTESIAN_POINT('Ctrl Pts',(2.0062449787379,-0.636309800095203,3.24892252893296));
#48129=CARTESIAN_POINT('Ctrl Pts',(1.95650440827287,-0.319434907277161,
3.30449298344116));
#48130=CARTESIAN_POINT('Ctrl Pts',(1.93721902666464,-0.158333333333334,
3.32334251722877));
#48131=CARTESIAN_POINT('Ctrl Pts',(1.91605012504035,0.158333333333336,3.31304233970309));
#48132=CARTESIAN_POINT('Ctrl Pts',(1.9152582443003,0.319434907277173,3.28448329445562));
#48133=CARTESIAN_POINT('Ctrl Pts',(1.91965569576352,0.636309800095215,3.20672897571828));
#48134=CARTESIAN_POINT('Ctrl Pts',(1.92845845189327,0.794772684000848,3.14523263031291));
#48135=CARTESIAN_POINT('Ctrl Pts',(1.95058534406668,1.06847604194559,3.03324878049766));
#48136=CARTESIAN_POINT('Ctrl Pts',(1.96289276371449,1.18514270861272,2.9797377029536));
#48137=CARTESIAN_POINT('Ctrl Pts',(1.97792969127037,1.30000000000138,2.92118920704003));
#48138=CARTESIAN_POINT('Ctrl Pts',(2.19672991623476,-1.30000000000003,2.99108833318567));
#48139=CARTESIAN_POINT('Ctrl Pts',(2.16869424276217,-1.18514270861181,3.03588762958137));
#48140=CARTESIAN_POINT('Ctrl Pts',(2.14173379281298,-1.06847604194513,3.07677957866654));
#48141=CARTESIAN_POINT('Ctrl Pts',(2.08193374144757,-0.794772684000858,
3.16222140751015));
#48142=CARTESIAN_POINT('Ctrl Pts',(2.04588339614435,-0.636309800095203,
3.21145553758907));
#48143=CARTESIAN_POINT('Ctrl Pts',(1.99433386989076,-0.319434907277162,
3.26559008542051));
#48144=CARTESIAN_POINT('Ctrl Pts',(1.97120200673784,-0.158333333333334,
3.28468906039049));
#48145=CARTESIAN_POINT('Ctrl Pts',(1.94875210217719,0.158333333333337,3.27360352254155));
#48146=CARTESIAN_POINT('Ctrl Pts',(1.94973138469771,0.319434907277174,3.24353820867032));
#48147=CARTESIAN_POINT('Ctrl Pts',(1.95494644437421,0.636309800095217,3.16658041875194));
#48148=CARTESIAN_POINT('Ctrl Pts',(1.96652411484811,0.794772684000849,3.10532686289807));
#48149=CARTESIAN_POINT('Ctrl Pts',(1.98460432652983,1.06847604194559,2.99942775676767));
#48150=CARTESIAN_POINT('Ctrl Pts',(1.99364914302969,1.18514270861272,2.94976483985142));
#48151=CARTESIAN_POINT('Ctrl Pts',(2.00391252233024,1.30000000000138,2.89627880511424));
#48152=CARTESIAN_POINT('Ctrl Pts',(2.22228736155764,-1.30000000000004,2.97318805622785));
#48153=CARTESIAN_POINT('Ctrl Pts',(2.19878628984836,-1.18514270861181,3.01411939305874));
#48154=CARTESIAN_POINT('Ctrl Pts',(2.17483352473068,-1.06847604194514,3.05196497398288));
#48155=CARTESIAN_POINT('Ctrl Pts',(2.11845434344017,-0.794772684000864,
3.13226712345224));
#48156=CARTESIAN_POINT('Ctrl Pts',(2.07921732493002,-0.636309800095207,
3.18056046380941));
#48157=CARTESIAN_POINT('Ctrl Pts',(2.02610306617644,-0.319434907277164,
3.23340259317279));
#48158=CARTESIAN_POINT('Ctrl Pts',(2.00139690559124,-0.158333333333335,
3.25376618423287));
#48159=CARTESIAN_POINT('Ctrl Pts',(1.97837829254599,0.158333333333337,3.24233776287423));
#48160=CARTESIAN_POINT('Ctrl Pts',(1.98052143462657,0.319434907277174,3.21081772473499));
#48161=CARTESIAN_POINT('Ctrl Pts',(1.98582042272674,0.636309800095218,3.13414273191321));
#48162=CARTESIAN_POINT('Ctrl Pts',(1.99860964659895,0.794772684000852,3.07240526593313));
#48163=CARTESIAN_POINT('Ctrl Pts',(2.01319306797143,1.0684760419456,2.97147652148233));
#48164=CARTESIAN_POINT('Ctrl Pts',(2.01971052024537,1.18514270861273,2.92512583728176));
#48165=CARTESIAN_POINT('Ctrl Pts',(2.02643280205011,1.3000000000014,2.87611278257491));
#48166=CARTESIAN_POINT('Ctrl Pts',(2.24737536599506,-1.30000000000005,2.95499905098216));
#48167=CARTESIAN_POINT('Ctrl Pts',(2.2286045590397,-1.18514270861182,2.99223335401397));
#48168=CARTESIAN_POINT('Ctrl Pts',(2.20792711755062,-1.06847604194515,3.02723798283389));
#48169=CARTESIAN_POINT('Ctrl Pts',(2.15575338400896,-0.79477268400087,3.10295468458563));
#48170=CARTESIAN_POINT('Ctrl Pts',(2.11462868360512,-0.636309800095211,
3.15115911964104));
#48171=CARTESIAN_POINT('Ctrl Pts',(2.05987426195789,-0.319434907277165,
3.20261922855258));
#48172=CARTESIAN_POINT('Ctrl Pts',(2.03202581413481,-0.158333333333336,
3.22314257767777));
#48173=CARTESIAN_POINT('Ctrl Pts',(2.00803959240179,0.158333333333338,3.21106609562426));
#48174=CARTESIAN_POINT('Ctrl Pts',(2.01188908814568,0.319434907277175,3.17845166474377));
#48175=CARTESIAN_POINT('Ctrl Pts',(2.01781123398656,0.636309800095221,3.10242236996614));
#48176=CARTESIAN_POINT('Ctrl Pts',(2.03278417415428,0.794772684000857,3.04086896994047));
#48177=CARTESIAN_POINT('Ctrl Pts',(2.04347808426441,1.0684760419456,2.94466595306606));
#48178=CARTESIAN_POINT('Ctrl Pts',(2.04696960309575,1.18514270861273,2.90130214713938));
#48179=CARTESIAN_POINT('Ctrl Pts',(2.04932364332018,1.3000000000014,2.85621725661796));
#48180=CARTESIAN_POINT('Ctrl Pts',(2.26798132103125,-1.30000000000005,2.9408473417646));
#48181=CARTESIAN_POINT('Ctrl Pts',(2.25255110305297,-1.18514270861183,2.97478060009054));
#48182=CARTESIAN_POINT('Ctrl Pts',(2.23415159110123,-1.06847604194515,3.00725190803789));
#48183=CARTESIAN_POINT('Ctrl Pts',(2.18478537459899,-0.794772684000873,
3.07888972742241));
#48184=CARTESIAN_POINT('Ctrl Pts',(2.14170408572716,-0.636309800095214,
3.1267431070186));
#48185=CARTESIAN_POINT('Ctrl Pts',(2.08629851241369,-0.319434907277168,
3.17757100674675));
#48186=CARTESIAN_POINT('Ctrl Pts',(2.05739580921471,-0.158333333333336,
3.19924659455908));
#48187=CARTESIAN_POINT('Ctrl Pts',(2.03368395533952,0.158333333333339,3.18738275794237));
#48188=CARTESIAN_POINT('Ctrl Pts',(2.03937689580979,0.319434907277175,3.15421146313419));
#48189=CARTESIAN_POINT('Ctrl Pts',(2.04546040657606,0.636309800095223,3.07846792891086));
#48190=CARTESIAN_POINT('Ctrl Pts',(2.06060576749126,0.794772684000864,3.01599273531813));
#48191=CARTESIAN_POINT('Ctrl Pts',(2.0678307030203,1.06847604194561,2.9233141761816));
#48192=CARTESIAN_POINT('Ctrl Pts',(2.06900714824849,1.18514270861274,2.88240299534151));
#48193=CARTESIAN_POINT('Ctrl Pts',(2.0682326318246,1.3000000000014,2.84069774783254));
#48194=CARTESIAN_POINT('Ctrl Pts',(2.28890432978042,-1.30000000000006,2.92700191529698));
#48195=CARTESIAN_POINT('Ctrl Pts',(2.27802478124005,-1.18514270861183,2.95858349693434));
#48196=CARTESIAN_POINT('Ctrl Pts',(2.26275140213339,-1.06847604194516,2.98917562005717));
#48197=CARTESIAN_POINT('Ctrl Pts',(2.21731621337705,-0.794772684000877,
3.05756369729516));
#48198=CARTESIAN_POINT('Ctrl Pts',(2.17220848809185,-0.636309800095215,
3.10489338359369));
#48199=CARTESIAN_POINT('Ctrl Pts',(2.11513145228693,-0.319434907277167,
3.1542889853963));
#48200=CARTESIAN_POINT('Ctrl Pts',(2.08349683499688,-0.158333333333337,
3.17588196355153));
#48201=CARTESIAN_POINT('Ctrl Pts',(2.05842347363757,0.158333333333339,3.16306052982064));
#48202=CARTESIAN_POINT('Ctrl Pts',(2.06475605343639,0.319434907277179,3.12853903953918));
#48203=CARTESIAN_POINT('Ctrl Pts',(2.07122625430981,0.636309800095227,3.05324521138199));
#48204=CARTESIAN_POINT('Ctrl Pts',(2.08909517719549,0.794772684000863,2.99160015978278));
#48205=CARTESIAN_POINT('Ctrl Pts',(2.09300977471158,1.06847604194561,2.90256984400533));
#48206=CARTESIAN_POINT('Ctrl Pts',(2.09145710151166,1.18514270861274,2.86383573850736));
#48207=CARTESIAN_POINT('Ctrl Pts',(2.08665727089726,1.30000000000141,2.82490545231324));
#48208=CARTESIAN_POINT('Ctrl Pts',(2.30431755283692,-1.30000000000007,2.91638984227385));
#48209=CARTESIAN_POINT('Ctrl Pts',(2.29571829012651,-1.18514270861184,2.94533448550776));
#48210=CARTESIAN_POINT('Ctrl Pts',(2.28213591612243,-1.06847604194516,2.9740169693766));
#48211=CARTESIAN_POINT('Ctrl Pts',(2.23924593107205,-0.79477268400088,3.03967360444674));
#48212=CARTESIAN_POINT('Ctrl Pts',(2.19413283193249,-0.63630980009522,3.087819634541));
#48213=CARTESIAN_POINT('Ctrl Pts',(2.13677609077595,-0.319434907277171,
3.13688315664733));
#48214=CARTESIAN_POINT('Ctrl Pts',(2.10328576819757,-0.158333333333338,
3.15853623876091));
#48215=CARTESIAN_POINT('Ctrl Pts',(2.07816984202021,0.15833333333334,3.14567657626547));
#48216=CARTESIAN_POINT('Ctrl Pts',(2.08643904656091,0.319434907277178,3.11113745708857));
#48217=CARTESIAN_POINT('Ctrl Pts',(2.09285072274629,0.636309800095229,3.0359334515012));
#48218=CARTESIAN_POINT('Ctrl Pts',(2.11011916058644,0.79477268400087,2.97309367718847));
#48219=CARTESIAN_POINT('Ctrl Pts',(2.11124730556027,1.06847604194562,2.88656806265442));
#48220=CARTESIAN_POINT('Ctrl Pts',(2.10799714327054,1.18514270861275,2.84969292888836));
#48221=CARTESIAN_POINT('Ctrl Pts',(2.1010084865338,1.30000000000142,2.81339639379812));
#48222=CARTESIAN_POINT('Ctrl Pts',(2.31848178810538,-1.30000000000007,2.90674308074662));
#48223=CARTESIAN_POINT('Ctrl Pts',(2.31330948407002,-1.18514270861184,2.93431605064516));
#48224=CARTESIAN_POINT('Ctrl Pts',(2.30203462419369,-1.06847604194517,2.96183803201959));
#48225=CARTESIAN_POINT('Ctrl Pts',(2.26188931754665,-0.794772684000884,
3.02530152105712));
#48226=CARTESIAN_POINT('Ctrl Pts',(2.21458477884655,-0.636309800095223,
3.07247131282959));
#48227=CARTESIAN_POINT('Ctrl Pts',(2.15632375272408,-0.319434907277172,
3.1207021557373));
#48228=CARTESIAN_POINT('Ctrl Pts',(2.12186104592459,-0.158333333333339,
3.14294161679127));
#48229=CARTESIAN_POINT('Ctrl Pts',(2.09638240425404,0.158333333333341,3.12982658281625));
#48230=CARTESIAN_POINT('Ctrl Pts',(2.10526842822162,0.319434907277182,3.0944851345404));
#48231=CARTESIAN_POINT('Ctrl Pts',(2.11183099857077,0.636309800095233,3.01951333644257));
#48232=CARTESIAN_POINT('Ctrl Pts',(2.13034374854833,0.794772684000874,2.95681777120825));
#48233=CARTESIAN_POINT('Ctrl Pts',(2.12900406616482,1.06847604194562,2.87265018646151));
#48234=CARTESIAN_POINT('Ctrl Pts',(2.12388559097138,1.18514270861275,2.83726416304824));
#48235=CARTESIAN_POINT('Ctrl Pts',(2.1142285394482,1.30000000000142,2.80292514494225));
#48236=CARTESIAN_POINT('Ctrl Pts',(2.33500443641727,-1.30000000000007,2.89700892416184));
#48237=CARTESIAN_POINT('Ctrl Pts',(2.33230791385509,-1.18514270861185,2.92211467057017));
#48238=CARTESIAN_POINT('Ctrl Pts',(2.32283266395042,-1.06847604194517,2.94782140171622));
#48239=CARTESIAN_POINT('Ctrl Pts',(2.28528272491246,-0.794772684000888,
3.00859748824829));
#48240=CARTESIAN_POINT('Ctrl Pts',(2.23767755759602,-0.636309800095224,
3.05633197853381));
#48241=CARTESIAN_POINT('Ctrl Pts',(2.17894957675327,-0.319434907277171,
3.10406117509063));
#48242=CARTESIAN_POINT('Ctrl Pts',(2.14287631687027,-0.158333333333339,
3.12650800835465));
#48243=CARTESIAN_POINT('Ctrl Pts',(2.1166387623548,0.158333333333341,3.11282772068504));
#48244=CARTESIAN_POINT('Ctrl Pts',(2.12582711643291,0.319434907277181,3.07631724695481));
#48245=CARTESIAN_POINT('Ctrl Pts',(2.13242969586,0.636309800095233,3.00150315147276));
#48246=CARTESIAN_POINT('Ctrl Pts',(2.15256245994101,0.794772684000874,2.93918498086401));
#48247=CARTESIAN_POINT('Ctrl Pts',(2.14865882357122,1.06847604194562,2.85768077878978));
#48248=CARTESIAN_POINT('Ctrl Pts',(2.14154726099493,1.18514270861275,2.82394538145764));
#48249=CARTESIAN_POINT('Ctrl Pts',(2.12901387538286,1.30000000000142,2.79175473584303));
#48250=CARTESIAN_POINT('Ctrl Pts',(2.35046299219406,-1.30000000000009,2.88651938390127));
#48251=CARTESIAN_POINT('Ctrl Pts',(2.35145434254997,-1.18514270861186,2.91010471870674));
#48252=CARTESIAN_POINT('Ctrl Pts',(2.3444785009304,-1.06847604194518,2.93454070194135));
#48253=CARTESIAN_POINT('Ctrl Pts',(2.30995710398222,-0.794772684000892,
2.99295787965795));
#48254=CARTESIAN_POINT('Ctrl Pts',(2.25996266540508,-0.636309800095232,
3.0396171500443));
#48255=CARTESIAN_POINT('Ctrl Pts',(2.20065327861454,-0.319434907277177,
3.08672816750844));
#48256=CARTESIAN_POINT('Ctrl Pts',(2.16393187965731,-0.158333333333341,
3.11011708054026));
#48257=CARTESIAN_POINT('Ctrl Pts',(2.13799717022496,0.158333333333343,3.09665644543285));
#48258=CARTESIAN_POINT('Ctrl Pts',(2.1487758192993,0.319434907277185,3.05991842617207));
#48259=CARTESIAN_POINT('Ctrl Pts',(2.15527444815603,0.636309800095241,2.98516188789695));
#48260=CARTESIAN_POINT('Ctrl Pts',(2.17518339819993,0.794772684000885,2.9218796799385));
#48261=CARTESIAN_POINT('Ctrl Pts',(2.16799220827574,1.06847604194564,2.84250895998002));
#48262=CARTESIAN_POINT('Ctrl Pts',(2.15878722815583,1.18514270861277,2.81034848034886));
#48263=CARTESIAN_POINT('Ctrl Pts',(2.14349006757434,1.30000000000144,2.78038416478162));
#48264=CARTESIAN_POINT('Ctrl Pts',(2.36783505325599,-1.3000000000001,2.87561679699127));
#48265=CARTESIAN_POINT('Ctrl Pts',(2.37177397284949,-1.18514270861187,2.89674501502257));
#48266=CARTESIAN_POINT('Ctrl Pts',(2.36698852169671,-1.06847604194519,2.9194078754243));
#48267=CARTESIAN_POINT('Ctrl Pts',(2.3357781304793,-0.794772684000901,2.97530894752189));
#48268=CARTESIAN_POINT('Ctrl Pts',(2.28588906471611,-0.636309800095238,
3.02291294353573));
#48269=CARTESIAN_POINT('Ctrl Pts',(2.22609023343301,-0.319434907277179,
3.06948140221203));
#48270=CARTESIAN_POINT('Ctrl Pts',(2.18708241423167,-0.158333333333342,
3.09265489349129));
#48271=CARTESIAN_POINT('Ctrl Pts',(2.16014363050186,0.158333333333345,3.07842918311708));
#48272=CARTESIAN_POINT('Ctrl Pts',(2.17147580504844,0.319434907277187,3.04060014268787));
#48273=CARTESIAN_POINT('Ctrl Pts',(2.17790320617912,0.636309800095247,2.96593048690121));
#48274=CARTESIAN_POINT('Ctrl Pts',(2.19924803217963,0.794772684000892,2.90282809369987));
#48275=CARTESIAN_POINT('Ctrl Pts',(2.18916697066081,1.06847604194565,2.82625170081662));
#48276=CARTESIAN_POINT('Ctrl Pts',(2.17780279283653,1.18514270861278,2.79587273566341));
#48277=CARTESIAN_POINT('Ctrl Pts',(2.15943815517932,1.30000000000145,2.76826188840121));
#48278=CARTESIAN_POINT('Ctrl Pts',(2.38159818278248,-1.30000000000011,2.86757732560228));
#48279=CARTESIAN_POINT('Ctrl Pts',(2.38835803633944,-1.18514270861188,2.88726709648415));
#48280=CARTESIAN_POINT('Ctrl Pts',(2.3855241128328,-1.0684760419452,2.90878487398856));
#48281=CARTESIAN_POINT('Ctrl Pts',(2.35681363836256,-0.794772684000908,
2.96271830562995));
#48282=CARTESIAN_POINT('Ctrl Pts',(2.30561969519472,-0.636309800095244,
3.00993767690273));
#48283=CARTESIAN_POINT('Ctrl Pts',(2.2451591336905,-0.319434907277183,3.0558452560672));
#48284=CARTESIAN_POINT('Ctrl Pts',(2.20483064420271,-0.158333333333344,
3.07919353570339));
#48285=CARTESIAN_POINT('Ctrl Pts',(2.17777050754538,0.158333333333346,3.06486001802799));
#48286=CARTESIAN_POINT('Ctrl Pts',(2.19038774253737,0.31943490727719,3.02682434733364));
#48287=CARTESIAN_POINT('Ctrl Pts',(2.19705503421999,0.636309800095253,2.95244123931286));
#48288=CARTESIAN_POINT('Ctrl Pts',(2.21911081285458,0.7947726840009,2.88919402976588));
#48289=CARTESIAN_POINT('Ctrl Pts',(2.20633210372423,1.06847604194566,2.81441474453547));
#48290=CARTESIAN_POINT('Ctrl Pts',(2.19304428398507,1.18514270861279,2.78520929392479));
#48291=CARTESIAN_POINT('Ctrl Pts',(2.17200007419145,1.30000000000147,2.75916757443416));
#48292=CARTESIAN_POINT('Ctrl Pts',(2.39241281507888,-1.30000000000012,2.86099299160901));
#48293=CARTESIAN_POINT('Ctrl Pts',(2.40123064389783,-1.18514270861188,2.87937186881187));
#48294=CARTESIAN_POINT('Ctrl Pts',(2.39987122314209,-1.0684760419452,2.89990398789257));
#48295=CARTESIAN_POINT('Ctrl Pts',(2.3732192067758,-0.794772684000911,2.95231170989772));
#48296=CARTESIAN_POINT('Ctrl Pts',(2.32158734929061,-0.636309800095245,
2.99971220851892));
#48297=CARTESIAN_POINT('Ctrl Pts',(2.26067097336819,-0.319434907277183,
3.0451546597403));
#48298=CARTESIAN_POINT('Ctrl Pts',(2.21892702187026,-0.158333333333344,
3.06835588462233));
#48299=CARTESIAN_POINT('Ctrl Pts',(2.19158252580981,0.158333333333347,3.05379481700059));
#48300=CARTESIAN_POINT('Ctrl Pts',(2.20515161001715,0.319434907277191,3.01554709154152));
#48301=CARTESIAN_POINT('Ctrl Pts',(2.21206062274055,0.636309800095254,2.94143358598389));
#48302=CARTESIAN_POINT('Ctrl Pts',(2.23491733512154,0.794772684000901,2.87824270878038));
#48303=CARTESIAN_POINT('Ctrl Pts',(2.22007525929973,1.06847604194566,2.80496768584344));
#48304=CARTESIAN_POINT('Ctrl Pts',(2.20526040309828,1.18514270861279,2.7767071039221));
#48305=CARTESIAN_POINT('Ctrl Pts',(2.18205527536554,1.30000000000147,2.75190398240171));
#48306=CARTESIAN_POINT('Ctrl Pts',(2.40075906139621,-1.30000000000012,2.85625494698041));
#48307=CARTESIAN_POINT('Ctrl Pts',(2.41130761398963,-1.18514270861189,2.87381149743691));
#48308=CARTESIAN_POINT('Ctrl Pts',(2.41113847876893,-1.0684760419452,2.89367775466536));
#48309=CARTESIAN_POINT('Ctrl Pts',(2.38598773965703,-0.794772684000912,
2.94490866779268));
#48310=CARTESIAN_POINT('Ctrl Pts',(2.33345265229072,-0.636309800095246,
2.99196672747374));
#48311=CARTESIAN_POINT('Ctrl Pts',(2.27218838688196,-0.319434907277184,
3.03704260315317));
#48312=CARTESIAN_POINT('Ctrl Pts',(2.22992098264959,-0.158333333333345,
3.06055543823259));
#48313=CARTESIAN_POINT('Ctrl Pts',(2.20237774376518,0.158333333333347,3.04583547575045));
#48314=CARTESIAN_POINT('Ctrl Pts',(2.21631914337816,0.319434907277191,3.00716395179031));
#48315=CARTESIAN_POINT('Ctrl Pts',(2.22307425179954,0.636309800095255,2.93299822649179));
#48316=CARTESIAN_POINT('Ctrl Pts',(2.24616935156192,0.794772684000903,2.86958107124942));
#48317=CARTESIAN_POINT('Ctrl Pts',(2.22982669049922,1.06847604194566,2.79746816906829));
#48318=CARTESIAN_POINT('Ctrl Pts',(2.21400070184457,1.1851427086128,2.77001568706186));
#48319=CARTESIAN_POINT('Ctrl Pts',(2.18942285695403,1.30000000000147,2.74632572635692));
#48320=CARTESIAN_POINT('Ctrl Pts',(2.40704602554912,-1.30000000000012,2.85272853528918));
#48321=CARTESIAN_POINT('Ctrl Pts',(2.41894744732919,-1.18514270861189,2.86971428113638));
#48322=CARTESIAN_POINT('Ctrl Pts',(2.41970481574944,-1.06847604194521,2.88910946594559));
#48323=CARTESIAN_POINT('Ctrl Pts',(2.39570949568987,-0.794772684000916,
2.93948250885712));
#48324=CARTESIAN_POINT('Ctrl Pts',(2.34242210867447,-0.636309800095249,
2.98622271392694));
#48325=CARTESIAN_POINT('Ctrl Pts',(2.2808968417526,-0.319434907277185,3.03102043769811));
#48326=CARTESIAN_POINT('Ctrl Pts',(2.23828433805704,-0.158333333333345,
3.05480036444708));
#48327=CARTESIAN_POINT('Ctrl Pts',(2.21060493512933,0.158333333333347,3.03996945789718));
#48328=CARTESIAN_POINT('Ctrl Pts',(2.22481883476239,0.319434907277193,3.00097592096811));
#48329=CARTESIAN_POINT('Ctrl Pts',(2.23142811183105,0.636309800095258,2.92674824815461));
#48330=CARTESIAN_POINT('Ctrl Pts',(2.25465858662683,0.794772684000906,2.86312947009923));
#48331=CARTESIAN_POINT('Ctrl Pts',(2.23715641304854,1.06847604194567,2.791861217171));
#48332=CARTESIAN_POINT('Ctrl Pts',(2.2205612568082,1.1851427086128,2.76500566347436));
#48333=CARTESIAN_POINT('Ctrl Pts',(2.19494698675012,1.30000000000148,2.74214394202474));
#48334=CARTESIAN_POINT('Ctrl Pts',(2.41117858829815,-1.30000000000012,2.85032932948442));
#48335=CARTESIAN_POINT('Ctrl Pts',(2.42391523248741,-1.18514270861189,2.86687924818083));
#48336=CARTESIAN_POINT('Ctrl Pts',(2.42526239159974,-1.06847604194521,2.88593731788189));
#48337=CARTESIAN_POINT('Ctrl Pts',(2.40206260966107,-0.794772684000917,
2.93575960201975));
#48338=CARTESIAN_POINT('Ctrl Pts',(2.34848943910999,-0.63630980009525,2.98246672345806));
#48339=CARTESIAN_POINT('Ctrl Pts',(2.28681527120289,-0.319434907277185,
3.02710086613297));
#48340=CARTESIAN_POINT('Ctrl Pts',(2.24380722851281,-0.158333333333345,
3.05092454534281));
#48341=CARTESIAN_POINT('Ctrl Pts',(2.21603686091174,0.158333333333348,3.03601765840459));
#48342=CARTESIAN_POINT('Ctrl Pts',(2.23053779170613,0.319434907277193,2.99689268376164));
#48343=CARTESIAN_POINT('Ctrl Pts',(2.23714641542351,0.636309800095258,2.92269766743079));
#48344=CARTESIAN_POINT('Ctrl Pts',(2.26057947518346,0.794772684000906,2.85902842483262));
#48345=CARTESIAN_POINT('Ctrl Pts',(2.24225976029705,1.06847604194567,2.78828978216868));
#48346=CARTESIAN_POINT('Ctrl Pts',(2.22509138163621,1.1851427086128,2.76178669639393));
#48347=CARTESIAN_POINT('Ctrl Pts',(2.19868455007652,1.30000000000148,2.73940066212868));
#48348=CARTESIAN_POINT('Ctrl Pts',(2.41323520827443,-1.30000000000012,2.84912189739511));
#48349=CARTESIAN_POINT('Ctrl Pts',(2.42637973947482,-1.18514270861189,2.86544585475509));
#48350=CARTESIAN_POINT('Ctrl Pts',(2.42801799749355,-1.06847604194521,2.88433223279753));
#48351=CARTESIAN_POINT('Ctrl Pts',(2.40522090837747,-0.794772684000917,
2.93388324866955));
#48352=CARTESIAN_POINT('Ctrl Pts',(2.35153877693122,-0.63630980009525,2.98060189844466));
#48353=CARTESIAN_POINT('Ctrl Pts',(2.28979444325212,-0.319434907277186,
3.02515797836937));
#48354=CARTESIAN_POINT('Ctrl Pts',(2.24656293042211,-0.158333333333345,
3.04898273817961));
#48355=CARTESIAN_POINT('Ctrl Pts',(2.21874670178875,0.158333333333348,3.03403728268168));
#48356=CARTESIAN_POINT('Ctrl Pts',(2.23340643548609,0.319434907277193,2.99485864798279));
#48357=CARTESIAN_POINT('Ctrl Pts',(2.24003011623958,0.636309800095259,2.92069167220904));
#48358=CARTESIAN_POINT('Ctrl Pts',(2.26358389234128,0.794772684000907,2.85701171734795));
#48359=CARTESIAN_POINT('Ctrl Pts',(2.2448487877729,1.06847604194567,2.78653279237346));
#48360=CARTESIAN_POINT('Ctrl Pts',(2.22738418251441,1.1851427086128,2.76019864061975));
#48361=CARTESIAN_POINT('Ctrl Pts',(2.20056470456104,1.30000000000148,2.73803805223228));
#48362=CARTESIAN_POINT('Ctrl Pts',(2.4149416938484,-1.30000000000013,2.84810972283032));
#48363=CARTESIAN_POINT('Ctrl Pts',(2.42841761794733,-1.18514270861189,2.86423837624598));
#48364=CARTESIAN_POINT('Ctrl Pts',(2.43029499764378,-1.06847604194521,2.8829788474371));
#48365=CARTESIAN_POINT('Ctrl Pts',(2.40783716246048,-0.794772684000917,
2.93230690646064));
#48366=CARTESIAN_POINT('Ctrl Pts',(2.35409241215596,-0.63630980009525,2.979058445274));
#48367=CARTESIAN_POINT('Ctrl Pts',(2.29229354863594,-0.319434907277186,
3.02355285427215));
#48368=CARTESIAN_POINT('Ctrl Pts',(2.24885541735091,-0.158333333333345,
3.04736198846237));
#48369=CARTESIAN_POINT('Ctrl Pts',(2.22100066370134,0.158333333333348,3.03238391154703));
#48370=CARTESIAN_POINT('Ctrl Pts',(2.23580464062873,0.319434907277193,2.99316995187068));
#48371=CARTESIAN_POINT('Ctrl Pts',(2.24245295969698,0.636309800095259,2.91903553476513));
#48372=CARTESIAN_POINT('Ctrl Pts',(2.26612261002616,0.794772684000907,2.8553580721882));
#48373=CARTESIAN_POINT('Ctrl Pts',(2.24703633876835,1.06847604194567,2.78509170502467));
#48374=CARTESIAN_POINT('Ctrl Pts',(2.22931744509398,1.1851427086128,2.75889267576204));
#48375=CARTESIAN_POINT('Ctrl Pts',(2.20214139735672,1.30000000000148,2.73691032395644));
#48376=CARTESIAN_POINT('Ctrl Pts',(2.41613364838208,-1.30000000000013,2.84739916316315));
#48377=CARTESIAN_POINT('Ctrl Pts',(2.42983902368031,-1.18514270861189,2.86338905532675));
#48378=CARTESIAN_POINT('Ctrl Pts',(2.43188288087058,-1.06847604194521,2.88202666611246));
#48379=CARTESIAN_POINT('Ctrl Pts',(2.40966416014421,-0.794772684000917,
2.93120003516014));
#48380=CARTESIAN_POINT('Ctrl Pts',(2.35588459500443,-0.63630980009525,2.9779820160423));
#48381=CARTESIAN_POINT('Ctrl Pts',(2.29404984138118,-0.319434907277186,
3.02243513731673));
#48382=CARTESIAN_POINT('Ctrl Pts',(2.25046223374693,-0.158333333333345,
3.04622938508356));
#48383=CARTESIAN_POINT('Ctrl Pts',(2.22258049616417,0.158333333333348,3.03122837281821));
#48384=CARTESIAN_POINT('Ctrl Pts',(2.23748735745911,0.319434907277193,2.99199117955593));
#48385=CARTESIAN_POINT('Ctrl Pts',(2.24415654248457,0.636309800095259,2.91788226257516));
#48386=CARTESIAN_POINT('Ctrl Pts',(2.26791354297215,0.794772684000907,2.85421125792459));
#48387=CARTESIAN_POINT('Ctrl Pts',(2.24858007637575,1.06847604194567,2.78409253961979));
#48388=CARTESIAN_POINT('Ctrl Pts',(2.23068071130597,1.1851427086128,2.75798616747606));
#48389=CARTESIAN_POINT('Ctrl Pts',(2.20325072248047,1.30000000000148,2.73612521818825));
#48390=CARTESIAN_POINT('Ctrl Pts',(2.41681457200604,-1.30000000000013,2.84699299207084));
#48391=CARTESIAN_POINT('Ctrl Pts',(2.43065041876023,-1.18514270861189,2.86290307521796));
#48392=CARTESIAN_POINT('Ctrl Pts',(2.43278914516079,-1.06847604194521,2.88148170329692));
#48393=CARTESIAN_POINT('Ctrl Pts',(2.41070734297901,-0.794772684000917,
2.93056692343428));
#48394=CARTESIAN_POINT('Ctrl Pts',(2.35691009009076,-0.63630980009525,2.97736811556787));
#48395=CARTESIAN_POINT('Ctrl Pts',(2.29505499304316,-0.319434907277186,
3.02179777530637));
#48396=CARTESIAN_POINT('Ctrl Pts',(2.25138012750943,-0.158333333333345,
3.04558200006546));
#48397=CARTESIAN_POINT('Ctrl Pts',(2.22348289215596,0.158333333333348,3.03056778556771));
#48398=CARTESIAN_POINT('Ctrl Pts',(2.2384498897554,0.319434907277193,2.99131837933657));
#48399=CARTESIAN_POINT('Ctrl Pts',(2.2451315272552,0.636309800095259,2.91722443298138));
#48400=CARTESIAN_POINT('Ctrl Pts',(2.26893823935086,0.794772684000907,2.85355694387179));
#48401=CARTESIAN_POINT('Ctrl Pts',(2.24946333436203,1.06847604194567,2.78352243917053));
#48402=CARTESIAN_POINT('Ctrl Pts',(2.23146070973882,1.1851427086128,2.75746890576994));
#48403=CARTESIAN_POINT('Ctrl Pts',(2.20388542524573,1.30000000000148,2.73567718101984));
#48404=CARTESIAN_POINT('Ctrl Pts',(2.42803368628124,-1.30000000000011,2.84027846919267));
#48405=CARTESIAN_POINT('Ctrl Pts',(2.44402065915128,-1.18514270861188,2.85487052201608));
#48406=CARTESIAN_POINT('Ctrl Pts',(2.44772572745999,-1.0684760419452,2.872476855943));
#48407=CARTESIAN_POINT('Ctrl Pts',(2.42791151992621,-0.794772684000911,
2.92011460180321));
#48408=CARTESIAN_POINT('Ctrl Pts',(2.37383452031449,-0.636309800095245,
2.9672424416972));
#48409=CARTESIAN_POINT('Ctrl Pts',(2.31166562520256,-0.319434907277183,
3.01130282976078));
#48410=CARTESIAN_POINT('Ctrl Pts',(2.26657616089764,-0.158333333333344,
3.03494229696348));
#48411=CARTESIAN_POINT('Ctrl Pts',(2.23842584648046,0.158333333333346,3.01971249569558));
#48412=CARTESIAN_POINT('Ctrl Pts',(2.25434823525271,0.31943490727719,2.98023224163553));
#48413=CARTESIAN_POINT('Ctrl Pts',(2.26124803596978,0.636309800095253,2.90639437862457));
#48414=CARTESIAN_POINT('Ctrl Pts',(2.28594188468099,0.7947726840009,2.84283632170469));
#48415=CARTESIAN_POINT('Ctrl Pts',(2.26412910545058,1.06847604194566,2.77418730483049));
#48416=CARTESIAN_POINT('Ctrl Pts',(2.24440574900138,1.18514270861279,2.74899209209798));
#48417=CARTESIAN_POINT('Ctrl Pts',(2.21440097998873,1.30000000000147,2.72831728234109));
#48418=CARTESIAN_POINT('Ctrl Pts',(2.44524045743472,-1.30000000000006,2.8310296558097));
#48419=CARTESIAN_POINT('Ctrl Pts',(2.46485368041197,-1.18514270861183,2.84409064111044));
#48420=CARTESIAN_POINT('Ctrl Pts',(2.47109329270799,-1.06847604194516,2.86047382708478));
#48421=CARTESIAN_POINT('Ctrl Pts',(2.45461232928673,-0.794772684000878,
2.90599721229061));
#48422=CARTESIAN_POINT('Ctrl Pts',(2.39901041965485,-0.636309800095217,
2.95266860365645));
#48423=CARTESIAN_POINT('Ctrl Pts',(2.33621994369784,-0.319434907277169,
2.99602953340761));
#48424=CARTESIAN_POINT('Ctrl Pts',(2.28982481036253,-0.158333333333337,
3.02005838856858));
#48425=CARTESIAN_POINT('Ctrl Pts',(2.26120820172365,0.158333333333339,3.00443113808546));
#48426=CARTESIAN_POINT('Ctrl Pts',(2.27811655282629,0.319434907277176,2.96428675721951));
#48427=CARTESIAN_POINT('Ctrl Pts',(2.28438953840607,0.636309800095226,2.89008882490359));
#48428=CARTESIAN_POINT('Ctrl Pts',(2.3086092844839,0.794772684000866,2.8253422315068));
#48429=CARTESIAN_POINT('Ctrl Pts',(2.28391313972469,1.06847604194561,2.75910807960274));
#48430=CARTESIAN_POINT('Ctrl Pts',(2.26246063338278,1.18514270861274,2.73575643566054));
#48431=CARTESIAN_POINT('Ctrl Pts',(2.23024566668289,1.30000000000141,2.71772345791827));
#48432=CARTESIAN_POINT('Ctrl Pts',(2.46723566498124,-1.30000000000004,2.81828368411535));
#48433=CARTESIAN_POINT('Ctrl Pts',(2.49156132565254,-1.18514270861182,2.82927316502905));
#48434=CARTESIAN_POINT('Ctrl Pts',(2.50112533947257,-1.06847604194514,2.84403085533445));
#48435=CARTESIAN_POINT('Ctrl Pts',(2.48911776738753,-0.794772684000865,
2.88682938972833));
#48436=CARTESIAN_POINT('Ctrl Pts',(2.4318418165874,-0.636309800095211,2.93315911961345));
#48437=CARTESIAN_POINT('Ctrl Pts',(2.36826535756389,-0.319434907277168,
2.97563179632322));
#48438=CARTESIAN_POINT('Ctrl Pts',(2.31972158902228,-0.158333333333336,
2.99985276530071));
#48439=CARTESIAN_POINT('Ctrl Pts',(2.29076505790789,0.158333333333338,2.98392483559399));
#48440=CARTESIAN_POINT('Ctrl Pts',(2.30931783037278,0.319434907277172,2.94317659647188));
#48441=CARTESIAN_POINT('Ctrl Pts',(2.31601905110005,0.636309800095219,2.86948068711656));
#48442=CARTESIAN_POINT('Ctrl Pts',(2.34231658966155,0.794772684000861,2.80522231166917));
#48443=CARTESIAN_POINT('Ctrl Pts',(2.31272733666762,1.06847604194561,2.74139292904049));
#48444=CARTESIAN_POINT('Ctrl Pts',(2.28763326817312,1.18514270861273,2.71946745101114));
#48445=CARTESIAN_POINT('Ctrl Pts',(2.25025322241536,1.3000000000014,2.70324586958073));
#48446=CARTESIAN_POINT('Ctrl Pts',(2.47880653387094,-1.30000000000002,2.81238598020883));
#48447=CARTESIAN_POINT('Ctrl Pts',(2.50530349436362,-1.18514270861179,2.82219997193384));
#48448=CARTESIAN_POINT('Ctrl Pts',(2.51643668958125,-1.06847604194512,2.83607840627677));
#48449=CARTESIAN_POINT('Ctrl Pts',(2.50666322642594,-0.794772684000851,
2.87753004151657));
#48450=CARTESIAN_POINT('Ctrl Pts',(2.44892689462503,-0.636309800095197,
2.92401312273345));
#48451=CARTESIAN_POINT('Ctrl Pts',(2.38514150298642,-0.319434907277159,
2.96618025706083));
#48452=CARTESIAN_POINT('Ctrl Pts',(2.33567769709269,-0.158333333333332,
2.99058134656035));
#48453=CARTESIAN_POINT('Ctrl Pts',(2.30625480759988,0.158333333333334,2.97425015982675));
#48454=CARTESIAN_POINT('Ctrl Pts',(2.32505056891378,0.319434907277167,2.93274590524431));
#48455=CARTESIAN_POINT('Ctrl Pts',(2.33143994443199,0.636309800095206,2.85888578373837));
#48456=CARTESIAN_POINT('Ctrl Pts',(2.35820372983969,0.79477268400084,2.79445086843063));
#48457=CARTESIAN_POINT('Ctrl Pts',(2.32663344521582,1.06847604194558,2.73214786314114));
#48458=CARTESIAN_POINT('Ctrl Pts',(2.30018582394002,1.1851427086127,2.71126979906201));
#48459=CARTESIAN_POINT('Ctrl Pts',(2.26095618780779,1.30000000000137,2.69648233333975));
#48460=CARTESIAN_POINT('Ctrl Pts',(2.48455995069221,-1.30000000000002,2.80941437546233));
#48461=CARTESIAN_POINT('Ctrl Pts',(2.5121356260387,-1.18514270861179,2.81863590450896));
#48462=CARTESIAN_POINT('Ctrl Pts',(2.52404941520512,-1.06847604194512,2.83207202931145));
#48463=CARTESIAN_POINT('Ctrl Pts',(2.51539056129934,-0.794772684000851,
2.87284872481581));
#48464=CARTESIAN_POINT('Ctrl Pts',(2.45746810794786,-0.636309800095197,
2.91944248366907));
#48465=CARTESIAN_POINT('Ctrl Pts',(2.39351595813041,-0.319434907277159,
2.96140733565522));
#48466=CARTESIAN_POINT('Ctrl Pts',(2.34340372597283,-0.158333333333332,
2.98574911995223));
#48467=CARTESIAN_POINT('Ctrl Pts',(2.3138047860753,0.158333333333334,2.96926236941848));
#48468=CARTESIAN_POINT('Ctrl Pts',(2.33301542000643,0.319434907277167,2.92761421432513));
#48469=CARTESIAN_POINT('Ctrl Pts',(2.33933008166849,0.636309800095206,2.85373654604741));
#48470=CARTESIAN_POINT('Ctrl Pts',(2.36620091374558,0.79477268400084,2.78910957149981));
#48471=CARTESIAN_POINT('Ctrl Pts',(2.33354901187549,1.06847604194558,2.72750133134463));
#48472=CARTESIAN_POINT('Ctrl Pts',(2.30638156847357,1.1851427086127,2.70711605782787));
#48473=CARTESIAN_POINT('Ctrl Pts',(2.26618048011713,1.30000000000137,2.6930134351473));
#48474=CARTESIAN_POINT('',(2.20678870418117,1.2,2.7691328596878));
#48475=CARTESIAN_POINT('Ctrl Pts',(2.20678870418117,1.2,2.7691328596878));
#48476=CARTESIAN_POINT('Ctrl Pts',(2.18719042940982,1.21681100185863,2.77815258574768));
#48477=CARTESIAN_POINT('Ctrl Pts',(2.16682870549213,1.23316343936831,2.78634864439441));
#48478=CARTESIAN_POINT('Ctrl Pts',(2.13772436433275,1.25820872625497,2.80002267851674));
#48479=CARTESIAN_POINT('Ctrl Pts',(2.128098436078,1.26641397694272,2.80447330095078));
#48480=CARTESIAN_POINT('Ctrl Pts',(2.10695042735038,1.28440270834969,2.81424329862363));
#48481=CARTESIAN_POINT('Ctrl Pts',(2.09638038403599,1.29362818749432,2.81941082472892));
#48482=CARTESIAN_POINT('Ctrl Pts',(2.08911835446463,1.30000000000141,2.82300508327628));
#48483=CARTESIAN_POINT('',(2.34584244529745,0.653834841330817,2.8411557470558));
#48484=CARTESIAN_POINT('Ctrl Pts',(2.34584244526459,0.653834841315613,2.84115574699037));
#48485=CARTESIAN_POINT('Ctrl Pts',(2.33291982688079,0.711695067402296,2.83420105328051));
#48486=CARTESIAN_POINT('Ctrl Pts',(2.3192544465607,0.767440337243871,2.82692182047546));
#48487=CARTESIAN_POINT('Ctrl Pts',(2.2907904144071,0.881611845231268,2.81194318081469));
#48488=CARTESIAN_POINT('Ctrl Pts',(2.27698326702507,0.939285575122016,2.80475197710374));
#48489=CARTESIAN_POINT('Ctrl Pts',(2.25126333376498,1.03699756658839,2.79155206652874));
#48490=CARTESIAN_POINT('Ctrl Pts',(2.24987672470583,1.04154831766055,2.79081882997294));
#48491=CARTESIAN_POINT('Ctrl Pts',(2.22388678607746,1.13769836768628,2.77767579297531));
#48492=CARTESIAN_POINT('Ctrl Pts',(2.21630665873191,1.16589155301464,2.77387326690931));
#48493=CARTESIAN_POINT('Ctrl Pts',(2.20678870418117,1.2,2.7691328596878));
#48494=CARTESIAN_POINT('',(2.46774460503229,-0.653834841531101,2.90899352548449));
#48495=CARTESIAN_POINT('Ctrl Pts',(2.46774460503229,-0.653834841531101,
2.90899352548449));
#48496=CARTESIAN_POINT('Ctrl Pts',(2.43367040187115,-0.575755206684555,
2.93302081381537));
#48497=CARTESIAN_POINT('Ctrl Pts',(2.40440703109882,-0.49371053352102,2.95246212356931));
#48498=CARTESIAN_POINT('Ctrl Pts',(2.36105525320677,-0.338116463230631,
2.9786559138965));
#48499=CARTESIAN_POINT('Ctrl Pts',(2.34510580758702,-0.265668632538642,
2.98681711169481));
#48500=CARTESIAN_POINT('Ctrl Pts',(2.32175237490573,-0.129739525092484,
2.99396435195135));
#48501=CARTESIAN_POINT('Ctrl Pts',(2.31349848432192,-0.0666632460451577,
2.99414569446904));
#48502=CARTESIAN_POINT('Ctrl Pts',(2.30171267766772,0.0595076176857795,
2.9880167192894));
#48503=CARTESIAN_POINT('Ctrl Pts',(2.29809985009213,0.122729100378534,2.98168411333372));
#48504=CARTESIAN_POINT('Ctrl Pts',(2.29615407501564,0.260112555578735,2.96113399532689));
#48505=CARTESIAN_POINT('Ctrl Pts',(2.29885574957816,0.333987313117584,2.94565663983887));
#48506=CARTESIAN_POINT('Ctrl Pts',(2.31369679496233,0.49152811065413,2.90327079369133));
#48507=CARTESIAN_POINT('Ctrl Pts',(2.32714321918519,0.5749238686812,2.8744937786279));
#48508=CARTESIAN_POINT('Ctrl Pts',(2.3458424451743,0.653834841353173,2.84115574703964));
#48509=CARTESIAN_POINT('',(2.40480387199025,-1.2,2.87340568838946));
#48510=CARTESIAN_POINT('Ctrl Pts',(2.40480387199025,-1.2,2.87340568838946));
#48511=CARTESIAN_POINT('Ctrl Pts',(2.41517135482326,-1.13733527587012,2.87916813364408));
#48512=CARTESIAN_POINT('Ctrl Pts',(2.43005872934456,-1.03725368999983,2.88749973076383));
#48513=CARTESIAN_POINT('Ctrl Pts',(2.4603247499497,-0.771923993714115,2.90470411541019));
#48514=CARTESIAN_POINT('Ctrl Pts',(2.46348281431209,-0.719575717376282,
2.90654258276977));
#48515=CARTESIAN_POINT('Ctrl Pts',(2.46774460503229,-0.653834841531101,
2.90899352548449));
#48516=CARTESIAN_POINT('Ctrl Pts',(2.2912494730135,-1.30000000000006,2.92534494345862));
#48517=CARTESIAN_POINT('Ctrl Pts',(2.30303220569663,-1.289337655596,2.91956314586749));
#48518=CARTESIAN_POINT('Ctrl Pts',(2.3078497420404,-1.28460982232617,2.91678630959235));
#48519=CARTESIAN_POINT('Ctrl Pts',(2.32967167705473,-1.26566188389439,2.90704899985406));
#48520=CARTESIAN_POINT('Ctrl Pts',(2.3390344571774,-1.25743246251566,2.90277167327097));
#48521=CARTESIAN_POINT('Ctrl Pts',(2.35866194984038,-1.23987895240838,2.8934877174126));
#48522=CARTESIAN_POINT('Ctrl Pts',(2.38088284032858,-1.22001152618653,2.8830048470048));
#48523=CARTESIAN_POINT('Ctrl Pts',(2.40480387199025,-1.2,2.87340568838946));
#48524=CARTESIAN_POINT('Origin',(0.,1.25,7.2));
#48525=CARTESIAN_POINT('Origin',(0.,1.2,7.2));
#48526=CARTESIAN_POINT('Origin',(0.,0.92691742076555,7.2));
#48527=CARTESIAN_POINT('Origin',(0.,0.653834841531101,7.2));
#48528=CARTESIAN_POINT('Origin',(0.,0.,7.2));
#48529=CARTESIAN_POINT('Origin',(0.,-0.653834841531101,7.2));
#48530=CARTESIAN_POINT('Origin',(0.,-0.926917420765551,7.2));
#48531=CARTESIAN_POINT('Origin',(0.,-1.2,7.2));
#48532=CARTESIAN_POINT('Origin',(0.,-1.25,7.2));
#48533=CARTESIAN_POINT('Ctrl Pts',(2.77007461962236,-1.30000000000274,2.98393685222895));
#48534=CARTESIAN_POINT('Ctrl Pts',(2.73776084594367,-1.18514270861364,2.95617299979124));
#48535=CARTESIAN_POINT('Ctrl Pts',(2.70652295951449,-1.06847604194606,2.94283794040697));
#48536=CARTESIAN_POINT('Ctrl Pts',(2.63684270752248,-0.794772684000851,
2.94536468398338));
#48537=CARTESIAN_POINT('Ctrl Pts',(2.59430952183081,-0.636309800095197,
3.00094899446));
#48538=CARTESIAN_POINT('Ctrl Pts',(2.53348691516025,-0.319434907277159,
3.04335648601559));
#48539=CARTESIAN_POINT('Ctrl Pts',(2.50702387179492,-0.158333333333332,
3.08081746056841));
#48540=CARTESIAN_POINT('Ctrl Pts',(2.47794645705815,0.158333333333334,3.06342740195888));
#48541=CARTESIAN_POINT('Ctrl Pts',(2.47397094455433,0.319434907277167,3.00785804372116));
#48542=CARTESIAN_POINT('Ctrl Pts',(2.47833749753066,0.636309800095206,2.93149143136109));
#48543=CARTESIAN_POINT('Ctrl Pts',(2.48972764967703,0.79477268400084,2.85803223588656));
#48544=CARTESIAN_POINT('Ctrl Pts',(2.52071187691362,1.0684760419458,2.83014510068367));
#48545=CARTESIAN_POINT('Ctrl Pts',(2.5383047969051,1.18514270861315,2.83374468235468));
#48546=CARTESIAN_POINT('Ctrl Pts',(2.56007871299605,1.30000000000202,2.85301515320588));
#48547=CARTESIAN_POINT('Ctrl Pts',(2.76929060404465,-1.30000000000274,2.99645449009369));
#48548=CARTESIAN_POINT('Ctrl Pts',(2.73676209966059,-1.18514270861363,2.971058085287));
#48549=CARTESIAN_POINT('Ctrl Pts',(2.70539049707342,-1.06847604194605,2.95946258494912));
#48550=CARTESIAN_POINT('Ctrl Pts',(2.63558849381797,-0.794772684000847,
2.96455750968112));
#48551=CARTESIAN_POINT('Ctrl Pts',(2.59328091779236,-0.636309800095194,
3.01976435068509));
#48552=CARTESIAN_POINT('Ctrl Pts',(2.53256341686942,-0.319434907277157,
3.06228370367669));
#48553=CARTESIAN_POINT('Ctrl Pts',(2.50593474388911,-0.158333333333332,
3.09888219725884));
#48554=CARTESIAN_POINT('Ctrl Pts',(2.47730282396258,0.158333333333334,3.08164150309493));
#48555=CARTESIAN_POINT('Ctrl Pts',(2.47407845734968,0.319434907277168,3.02713594688277));
#48556=CARTESIAN_POINT('Ctrl Pts',(2.47896213178644,0.636309800095205,2.95085588583574));
#48557=CARTESIAN_POINT('Ctrl Pts',(2.49034670616782,0.794772684000836,2.87782974001919));
#48558=CARTESIAN_POINT('Ctrl Pts',(2.52138535406906,1.0684760419458,2.84733710522955));
#48559=CARTESIAN_POINT('Ctrl Pts',(2.53896378271483,1.18514270861314,2.8491423489711));
#48560=CARTESIAN_POINT('Ctrl Pts',(2.56068515942512,1.30000000000202,2.8659519681912));
#48561=CARTESIAN_POINT('Ctrl Pts',(2.76721848791142,-1.30000000000265,3.02121331325036));
#48562=CARTESIAN_POINT('Ctrl Pts',(2.73578637353955,-1.18514270861355,3.00121583992818));
#48563=CARTESIAN_POINT('Ctrl Pts',(2.70501257943525,-1.06847604194598,2.99348304482396));
#48564=CARTESIAN_POINT('Ctrl Pts',(2.63543981029279,-0.794772684000797,
3.00395260141672));
#48565=CARTESIAN_POINT('Ctrl Pts',(2.59106724941863,-0.636309800095158,
3.05737222262203));
#48566=CARTESIAN_POINT('Ctrl Pts',(2.5298731250399,-0.319434907277142,3.09983687965061));
#48567=CARTESIAN_POINT('Ctrl Pts',(2.50382283511936,-0.158333333333323,
3.13505529858875));
#48568=CARTESIAN_POINT('Ctrl Pts',(2.47579477399916,0.158333333333325,3.11801831865943));
#48569=CARTESIAN_POINT('Ctrl Pts',(2.47299997278668,0.319434907277146,3.06526604657375));
#48570=CARTESIAN_POINT('Ctrl Pts',(2.47876718605892,0.636309800095166,2.98911038310189));
#48571=CARTESIAN_POINT('Ctrl Pts',(2.49114624673536,0.794772684000794,2.91731837360279));
#48572=CARTESIAN_POINT('Ctrl Pts',(2.52227539906165,1.06847604194574,2.88158743177373));
#48573=CARTESIAN_POINT('Ctrl Pts',(2.53963249089368,1.18514270861308,2.87971951368484));
#48574=CARTESIAN_POINT('Ctrl Pts',(2.56087201796442,1.30000000000195,2.89145027826303));
#48575=CARTESIAN_POINT('Ctrl Pts',(2.7652185811479,-1.30000000000256,3.04654629607291));
#48576=CARTESIAN_POINT('Ctrl Pts',(2.73243126387775,-1.18514270861348,3.03098812080502));
#48577=CARTESIAN_POINT('Ctrl Pts',(2.70083628138072,-1.06847604194591,3.02656997753292));
#48578=CARTESIAN_POINT('Ctrl Pts',(2.63060008310996,-0.794772684000746,
3.04209888519379));
#48579=CARTESIAN_POINT('Ctrl Pts',(2.58791270220426,-0.636309800095112,
3.09526306562633));
#48580=CARTESIAN_POINT('Ctrl Pts',(2.52733228412459,-0.319434907277116,
3.13812521055095));
#48581=CARTESIAN_POINT('Ctrl Pts',(2.50092370254775,-0.158333333333311,
3.17156613975076));
#48582=CARTESIAN_POINT('Ctrl Pts',(2.47354491525794,0.158333333333314,3.15475538318367));
#48583=CARTESIAN_POINT('Ctrl Pts',(2.47144943768543,0.319434907277126,3.10389195667189));
#48584=CARTESIAN_POINT('Ctrl Pts',(2.4785533351495,0.636309800095123,3.02803358288528));
#48585=CARTESIAN_POINT('Ctrl Pts',(2.49247060842304,0.794772684000734,2.95770033352747));
#48586=CARTESIAN_POINT('Ctrl Pts',(2.52383408752185,1.06847604194566,2.91668889036367));
#48587=CARTESIAN_POINT('Ctrl Pts',(2.54091340125602,1.18514270861299,2.91105954495111));
#48588=CARTESIAN_POINT('Ctrl Pts',(2.56149594075389,1.30000000000185,2.91755318824791));
#48589=CARTESIAN_POINT('Ctrl Pts',(2.76408253126439,-1.30000000000255,3.05972730575715));
#48590=CARTESIAN_POINT('Ctrl Pts',(2.73152836524454,-1.18514270861346,3.04690234069982));
#48591=CARTESIAN_POINT('Ctrl Pts',(2.70004026601005,-1.0684760419459,3.0444554800774));
#48592=CARTESIAN_POINT('Ctrl Pts',(2.62975928514619,-0.794772684000735,
3.06277823992411));
#48593=CARTESIAN_POINT('Ctrl Pts',(2.58653525785172,-0.636309800095103,
3.11521585093284));
#48594=CARTESIAN_POINT('Ctrl Pts',(2.52563186823559,-0.319434907277112,
3.15802247013646));
#48595=CARTESIAN_POINT('Ctrl Pts',(2.49895903018375,-0.158333333333309,
3.19050025120487));
#48596=CARTESIAN_POINT('Ctrl Pts',(2.47190832759045,0.158333333333311,3.17380577933224));
#48597=CARTESIAN_POINT('Ctrl Pts',(2.47065441609167,0.319434907277121,3.12412270606223));
#48598=CARTESIAN_POINT('Ctrl Pts',(2.47824191681505,0.636309800095114,3.04835115392578));
#48599=CARTESIAN_POINT('Ctrl Pts',(2.49200957451927,0.794772684000723,2.97843587612576));
#48600=CARTESIAN_POINT('Ctrl Pts',(2.52349875362235,1.06847604194565,2.93465689948966));
#48601=CARTESIAN_POINT('Ctrl Pts',(2.54064141214415,1.18514270861297,2.92713029039323));
#48602=CARTESIAN_POINT('Ctrl Pts',(2.56129623034307,1.30000000000184,2.93102736901523));
#48603=CARTESIAN_POINT('Ctrl Pts',(2.76393671495793,-1.30000000000255,3.06127271886912));
#48604=CARTESIAN_POINT('Ctrl Pts',(2.73140696766947,-1.18514270861346,3.0487683078493));
#48605=CARTESIAN_POINT('Ctrl Pts',(2.6999301212694,-1.0684760419459,3.04655299023555));
#48606=CARTESIAN_POINT('Ctrl Pts',(2.62964472084827,-0.794772684000736,
3.06520502746905));
#48607=CARTESIAN_POINT('Ctrl Pts',(2.58636702198853,-0.636309800095104,
3.11756090521599));
#48608=CARTESIAN_POINT('Ctrl Pts',(2.52542602591945,-0.319434907277112,
3.16036129461213));
#48609=CARTESIAN_POINT('Ctrl Pts',(2.49871387963128,-0.158333333333309,
3.19272260274774));
#48610=CARTESIAN_POINT('Ctrl Pts',(2.4717012207635,0.158333333333311,3.17604171343888));
#48611=CARTESIAN_POINT('Ctrl Pts',(2.47055032595736,0.319434907277121,3.12649920803476));
#48612=CARTESIAN_POINT('Ctrl Pts',(2.47820064825465,0.636309800095114,3.05074013947077));
#48613=CARTESIAN_POINT('Ctrl Pts',(2.49195786235389,0.794772684000724,2.98087660648409));
#48614=CARTESIAN_POINT('Ctrl Pts',(2.52346380679981,1.06847604194565,2.93677266582891));
#48615=CARTESIAN_POINT('Ctrl Pts',(2.54061323305724,1.18514270861297,2.92902253581192));
#48616=CARTESIAN_POINT('Ctrl Pts',(2.56127432963171,1.30000000000184,2.93261323747555));
#48617=CARTESIAN_POINT('Ctrl Pts',(2.76367479421307,-1.30000000000255,3.06397452733984));
#48618=CARTESIAN_POINT('Ctrl Pts',(2.73117783714647,-1.18514270861346,3.0520268287371));
#48619=CARTESIAN_POINT('Ctrl Pts',(2.69971468392264,-1.0684760419459,3.0502141552986));
#48620=CARTESIAN_POINT('Ctrl Pts',(2.62941679948215,-0.794772684000736,
3.06944045266576));
#48621=CARTESIAN_POINT('Ctrl Pts',(2.58605487221752,-0.636309800095104,
3.12165763870706));
#48622=CARTESIAN_POINT('Ctrl Pts',(2.5250583247634,-0.319434907277112,3.16445140478554));
#48623=CARTESIAN_POINT('Ctrl Pts',(2.49829077627368,-0.158333333333309,
3.19661413676455));
#48624=CARTESIAN_POINT('Ctrl Pts',(2.47134447132379,0.158333333333311,3.17995702806293));
#48625=CARTESIAN_POINT('Ctrl Pts',(2.47035394045193,0.319434907277122,3.13065281472957));
#48626=CARTESIAN_POINT('Ctrl Pts',(2.47811633094835,0.636309800095115,3.05491634979516));
#48627=CARTESIAN_POINT('Ctrl Pts',(2.49187936704538,0.794772684000724,2.9851525184675));
#48628=CARTESIAN_POINT('Ctrl Pts',(2.52341791795381,1.06847604194565,2.94048112062575));
#48629=CARTESIAN_POINT('Ctrl Pts',(2.54057643155836,1.18514270861297,2.93233878096298));
#48630=CARTESIAN_POINT('Ctrl Pts',(2.56124158869765,1.30000000000184,2.93539069452477));
#48631=CARTESIAN_POINT('Ctrl Pts',(2.76309866457954,-1.30000000000255,3.0693569772583));
#48632=CARTESIAN_POINT('Ctrl Pts',(2.73060852771944,-1.18514270861347,3.05849815921093));
#48633=CARTESIAN_POINT('Ctrl Pts',(2.69913847631771,-1.0684760419459,3.05747652440161));
#48634=CARTESIAN_POINT('Ctrl Pts',(2.62879296349401,-0.794772684000738,
3.07784220481634));
#48635=CARTESIAN_POINT('Ctrl Pts',(2.58533532606946,-0.636309800095105,
3.1298130289063));
#48636=CARTESIAN_POINT('Ctrl Pts',(2.52428188718962,-0.319434907277113,
3.17261639434202));
#48637=CARTESIAN_POINT('Ctrl Pts',(2.4974530801566,-0.15833333333331,3.20440186989524));
#48638=CARTESIAN_POINT('Ctrl Pts',(2.47063810417917,0.158333333333312,3.1877925966685));
#48639=CARTESIAN_POINT('Ctrl Pts',(2.46987895907201,0.319434907277122,3.13893071555855));
#48640=CARTESIAN_POINT('Ctrl Pts',(2.47788671941555,0.636309800095115,3.06324697138882));
#48641=CARTESIAN_POINT('Ctrl Pts',(2.49179054834725,0.794772684000726,2.99373052952472));
#48642=CARTESIAN_POINT('Ctrl Pts',(2.52341492440155,1.06847604194565,2.94793175812201));
#48643=CARTESIAN_POINT('Ctrl Pts',(2.54057789787682,1.18514270861298,2.93899986355282));
#48644=CARTESIAN_POINT('Ctrl Pts',(2.56121482423204,1.30000000000184,2.94096066554301));
#48645=CARTESIAN_POINT('Ctrl Pts',(2.7621442995113,-1.30000000000256,3.07699590637945));
#48646=CARTESIAN_POINT('Ctrl Pts',(2.72942903075446,-1.18514270861347,3.06759261633828));
#48647=CARTESIAN_POINT('Ctrl Pts',(2.69781041332261,-1.06847604194591,3.06764199419852));
#48648=CARTESIAN_POINT('Ctrl Pts',(2.62729856571769,-0.794772684000742,
3.0895936207856));
#48649=CARTESIAN_POINT('Ctrl Pts',(2.58397375681921,-0.636309800095108,
3.14132870240152));
#48650=CARTESIAN_POINT('Ctrl Pts',(2.52306333846313,-0.319434907277114,
3.18423899962697));
#48651=CARTESIAN_POINT('Ctrl Pts',(2.49638657956733,-0.15833333333331,3.21558026331581));
#48652=CARTESIAN_POINT('Ctrl Pts',(2.4697476139746,0.158333333333313,3.19903735811405));
#48653=CARTESIAN_POINT('Ctrl Pts',(2.46891703047776,0.319434907277124,3.15065303364791));
#48654=CARTESIAN_POINT('Ctrl Pts',(2.47733461500681,0.636309800095119,3.07506481055014));
#48655=CARTESIAN_POINT('Ctrl Pts',(2.49196724242051,0.79477268400073,3.00609836528132));
#48656=CARTESIAN_POINT('Ctrl Pts',(2.52377377005411,1.06847604194566,2.9587108102807));
#48657=CARTESIAN_POINT('Ctrl Pts',(2.5408736807323,1.18514270861298,2.94862501569126));
#48658=CARTESIAN_POINT('Ctrl Pts',(2.56130563482408,1.30000000000184,2.94896574319025));
#48659=CARTESIAN_POINT('Ctrl Pts',(2.76100115701359,-1.30000000000257,3.08616759468416));
#48660=CARTESIAN_POINT('Ctrl Pts',(2.72800130695223,-1.18514270861348,3.07850646772044));
#48661=CARTESIAN_POINT('Ctrl Pts',(2.69618309389375,-1.06847604194592,3.07983308091253));
#48662=CARTESIAN_POINT('Ctrl Pts',(2.6254064743796,-0.794772684000749,3.10366130052537));
#48663=CARTESIAN_POINT('Ctrl Pts',(2.58215216274572,-0.636309800095113,
3.15507420908088));
#48664=CARTESIAN_POINT('Ctrl Pts',(2.52137305231519,-0.319434907277116,
3.19809534748637));
#48665=CARTESIAN_POINT('Ctrl Pts',(2.49490004610859,-0.158333333333311,
3.22891175502433));
#48666=CARTESIAN_POINT('Ctrl Pts',(2.46850828493044,0.158333333333314,3.21246574523192));
#48667=CARTESIAN_POINT('Ctrl Pts',(2.46766473902188,0.319434907277126,3.16468858611461));
#48668=CARTESIAN_POINT('Ctrl Pts',(2.47656946475392,0.636309800095123,3.08921660187131));
#48669=CARTESIAN_POINT('Ctrl Pts',(2.49193592041559,0.794772684000735,3.02085499815659));
#48670=CARTESIAN_POINT('Ctrl Pts',(2.52402010645754,1.06847604194566,2.97158305391625));
#48671=CARTESIAN_POINT('Ctrl Pts',(2.54111071189665,1.18514270861299,2.96013759686987));
#48672=CARTESIAN_POINT('Ctrl Pts',(2.56140386747354,1.30000000000185,2.95857468173336));
#48673=CARTESIAN_POINT('Ctrl Pts',(2.75973043404253,-1.30000000000257,3.09850296312576));
#48674=CARTESIAN_POINT('Ctrl Pts',(2.72673344694344,-1.18514270861349,3.09332988253571));
#48675=CARTESIAN_POINT('Ctrl Pts',(2.69486206402682,-1.06847604194592,3.09645179355735));
#48676=CARTESIAN_POINT('Ctrl Pts',(2.62383316447927,-0.794772684000754,
3.12282712258378));
#48677=CARTESIAN_POINT('Ctrl Pts',(2.58018454086766,-0.636309800095117,
3.17359946802657));
#48678=CARTESIAN_POINT('Ctrl Pts',(2.5190510459393,-0.319434907277118,3.21654618894011));
#48679=CARTESIAN_POINT('Ctrl Pts',(2.49224201902599,-0.158333333333313,
3.2464126972753));
#48680=CARTESIAN_POINT('Ctrl Pts',(2.46615483373219,0.158333333333315,3.2300839140066));
#48681=CARTESIAN_POINT('Ctrl Pts',(2.46611897094408,0.319434907277128,3.18344725658337));
#48682=CARTESIAN_POINT('Ctrl Pts',(2.47565813709047,0.636309800095127,3.10813901025747));
#48683=CARTESIAN_POINT('Ctrl Pts',(2.4911520371447,0.79477268400074,3.04027505419037));
#48684=CARTESIAN_POINT('Ctrl Pts',(2.52351148979463,1.06847604194567,2.98845100941886));
#48685=CARTESIAN_POINT('Ctrl Pts',(2.54069441470553,1.185142708613,2.97522591670852));
#48686=CARTESIAN_POINT('Ctrl Pts',(2.56105305651101,1.30000000000186,2.97120843999939));
#48687=CARTESIAN_POINT('Ctrl Pts',(2.75818571536233,-1.30000000000258,3.11395382493746));
#48688=CARTESIAN_POINT('Ctrl Pts',(2.72516881337955,-1.1851427086135,3.11188529650836));
#48689=CARTESIAN_POINT('Ctrl Pts',(2.69322800104665,-1.06847604194593,3.11725314803314));
#48690=CARTESIAN_POINT('Ctrl Pts',(2.62192431718254,-0.79477268400076,3.14683348422645));
#48691=CARTESIAN_POINT('Ctrl Pts',(2.57789912794509,-0.636309800095122,
3.1968538353808));
#48692=CARTESIAN_POINT('Ctrl Pts',(2.51639218605445,-0.31943490727712,3.23973300172921));
#48693=CARTESIAN_POINT('Ctrl Pts',(2.4892276348165,-0.158333333333314,3.26842989090202));
#48694=CARTESIAN_POINT('Ctrl Pts',(2.46340122882819,0.158333333333316,3.25219748804885));
#48695=CARTESIAN_POINT('Ctrl Pts',(2.46399403849527,0.319434907277131,3.20684119605487));
#48696=CARTESIAN_POINT('Ctrl Pts',(2.47441264586635,0.636309800095132,3.13176756205614));
#48697=CARTESIAN_POINT('Ctrl Pts',(2.49063108383278,0.794772684000745,3.0647364067299));
#48698=CARTESIAN_POINT('Ctrl Pts',(2.52348977741813,1.06847604194568,3.00978306948002));
#48699=CARTESIAN_POINT('Ctrl Pts',(2.54077114129557,1.18514270861301,2.99432928211294));
#48700=CARTESIAN_POINT('Ctrl Pts',(2.5611105581319,1.30000000000187,2.98720897085252));
#48701=CARTESIAN_POINT('Ctrl Pts',(2.7549023177279,-1.30000000000261,3.13832627815554));
#48702=CARTESIAN_POINT('Ctrl Pts',(2.72120577726823,-1.18514270861352,3.14095019256061));
#48703=CARTESIAN_POINT('Ctrl Pts',(2.68871288765401,-1.06847604194595,3.14972442523763));
#48704=CARTESIAN_POINT('Ctrl Pts',(2.61642848670769,-0.794772684000774,
3.18420312357576));
#48705=CARTESIAN_POINT('Ctrl Pts',(2.57194172056141,-0.636309800095132,
3.23307614933181));
#48706=CARTESIAN_POINT('Ctrl Pts',(2.51044675909465,-0.319434907277125,
3.27611316803085));
#48707=CARTESIAN_POINT('Ctrl Pts',(2.48372887214136,-0.158333333333316,
3.30338169611771));
#48708=CARTESIAN_POINT('Ctrl Pts',(2.45894850607955,0.158333333333319,3.28758166575951));
#48709=CARTESIAN_POINT('Ctrl Pts',(2.46072295196821,0.319434907277137,3.2443405872588));
#48710=CARTESIAN_POINT('Ctrl Pts',(2.47207426405154,0.636309800095144,3.16947145529152));
#48711=CARTESIAN_POINT('Ctrl Pts',(2.48810766360199,0.794772684000758,3.10327100058628));
#48712=CARTESIAN_POINT('Ctrl Pts',(2.52147144464212,1.0684760419457,3.04318070445959));
#48713=CARTESIAN_POINT('Ctrl Pts',(2.53902642198244,1.18514270861303,3.02419036799466));
#48714=CARTESIAN_POINT('Ctrl Pts',(2.55969443210068,1.3000000000019,3.0122205576932));
#48715=CARTESIAN_POINT('Ctrl Pts',(2.75184888476579,-1.30000000000264,3.16283396361858));
#48716=CARTESIAN_POINT('Ctrl Pts',(2.71746663127512,-1.18514270861355,3.17014743557151));
#48717=CARTESIAN_POINT('Ctrl Pts',(2.68448012602566,-1.06847604194598,3.18235462632914));
#48718=CARTESIAN_POINT('Ctrl Pts',(2.61149915762758,-0.794772684000793,
3.2218611484432));
#48719=CARTESIAN_POINT('Ctrl Pts',(2.56724671660987,-0.636309800095148,
3.26990395622154));
#48720=CARTESIAN_POINT('Ctrl Pts',(2.50568271389788,-0.319434907277134,
3.31306241579418));
#48721=CARTESIAN_POINT('Ctrl Pts',(2.47891175269111,-0.15833333333332,3.33865996146269));
#48722=CARTESIAN_POINT('Ctrl Pts',(2.4542701656467,0.158333333333322,3.32291066839621));
#48723=CARTESIAN_POINT('Ctrl Pts',(2.45598525678049,0.319434907277142,3.28129641508887));
#48724=CARTESIAN_POINT('Ctrl Pts',(2.46819998563599,0.636309800095157,3.20660248375591));
#48725=CARTESIAN_POINT('Ctrl Pts',(2.48531425849309,0.794772684000779,3.1417362377766));
#48726=CARTESIAN_POINT('Ctrl Pts',(2.51991043860404,1.06847604194572,3.07680171724122));
#48727=CARTESIAN_POINT('Ctrl Pts',(2.53797508303648,1.18514270861305,3.0543711466414));
#48728=CARTESIAN_POINT('Ctrl Pts',(2.55912896744609,1.30000000000192,3.03761775332049));
#48729=CARTESIAN_POINT('Ctrl Pts',(2.7483447845198,-1.30000000000265,3.18713448216638));
#48730=CARTESIAN_POINT('Ctrl Pts',(2.71346030506721,-1.18514270861355,3.19924195415874));
#48731=CARTESIAN_POINT('Ctrl Pts',(2.67991284763775,-1.06847604194598,3.21486580077584));
#48732=CARTESIAN_POINT('Ctrl Pts',(2.60550029817392,-0.794772684000795,
3.25908354083241));
#48733=CARTESIAN_POINT('Ctrl Pts',(2.55953575074245,-0.63630980009515,3.30539306082358));
#48734=CARTESIAN_POINT('Ctrl Pts',(2.49755111095438,-0.319434907277134,
3.34851999863704));
#48735=CARTESIAN_POINT('Ctrl Pts',(2.47177474429291,-0.158333333333321,
3.37294177377652));
#48736=CARTESIAN_POINT('Ctrl Pts',(2.44821621172272,0.158333333333323,3.35767651489293));
#48737=CARTESIAN_POINT('Ctrl Pts',(2.45050291347272,0.319434907277145,3.31796779184588));
#48738=CARTESIAN_POINT('Ctrl Pts',(2.46436024022379,0.636309800095161,3.24379079980185));
#48739=CARTESIAN_POINT('Ctrl Pts',(2.48315961503444,0.79477268400078,3.18051374342521));
#48740=CARTESIAN_POINT('Ctrl Pts',(2.51868068943466,1.06847604194573,3.1105959175308));
#48741=CARTESIAN_POINT('Ctrl Pts',(2.53685981385929,1.18514270861306,3.08455098390633));
#48742=CARTESIAN_POINT('Ctrl Pts',(2.55784230578616,1.30000000000193,3.06272595277639));
#48743=CARTESIAN_POINT('Ctrl Pts',(2.74574091063359,-1.30000000000266,3.20541339922365));
#48744=CARTESIAN_POINT('Ctrl Pts',(2.70964371406839,-1.18514270861356,3.22071934176333));
#48745=CARTESIAN_POINT('Ctrl Pts',(2.67533364623634,-1.06847604194599,3.23874024204124));
#48746=CARTESIAN_POINT('Ctrl Pts',(2.60019915072659,-0.794772684000802,
3.28664422225255));
#48747=CARTESIAN_POINT('Ctrl Pts',(2.55576917040971,-0.636309800095156,
3.332964495603));
#48748=CARTESIAN_POINT('Ctrl Pts',(2.49371487414238,-0.319434907277137,
3.37617641007381));
#48749=CARTESIAN_POINT('Ctrl Pts',(2.46683846697507,-0.158333333333322,
3.39884683891698));
#48750=CARTESIAN_POINT('Ctrl Pts',(2.44311848446409,0.158333333333324,3.3835033720173));
#48751=CARTESIAN_POINT('Ctrl Pts',(2.44600440432415,0.319434907277148,3.34531201998123));
#48752=CARTESIAN_POINT('Ctrl Pts',(2.46029380290506,0.636309800095166,3.27120803389401));
#48753=CARTESIAN_POINT('Ctrl Pts',(2.47879230060294,0.794772684000788,3.2085085373939));
#48754=CARTESIAN_POINT('Ctrl Pts',(2.51544085880915,1.06847604194574,3.13503668909042));
#48755=CARTESIAN_POINT('Ctrl Pts',(2.53437207462858,1.18514270861307,3.10655120032261));
#48756=CARTESIAN_POINT('Ctrl Pts',(2.55637070338285,1.30000000000194,3.08138346351737));
#48757=CARTESIAN_POINT('Ctrl Pts',(2.74195814600123,-1.30000000000267,3.22308002651805));
#48758=CARTESIAN_POINT('Ctrl Pts',(2.70557844442503,-1.18514270861357,3.24204765563099));
#48759=CARTESIAN_POINT('Ctrl Pts',(2.67088384859235,-1.068476041946,3.2626624023393));
#48760=CARTESIAN_POINT('Ctrl Pts',(2.59462532296085,-0.794772684000805,
3.31409176235129));
#48761=CARTESIAN_POINT('Ctrl Pts',(2.54860492617569,-0.63630980009516,3.35894703121784));
#48762=CARTESIAN_POINT('Ctrl Pts',(2.48613821236498,-0.319434907277141,
3.40208923138921));
#48763=CARTESIAN_POINT('Ctrl Pts',(2.45985076920911,-0.158333333333323,
3.42381119065622));
#48764=CARTESIAN_POINT('Ctrl Pts',(2.4375060132358,0.158333333333325,3.40910176479674));
#48765=CARTESIAN_POINT('Ctrl Pts',(2.4419033528333,0.31943490727715,3.37285105163994));
#48766=CARTESIAN_POINT('Ctrl Pts',(2.457929313369,0.636309800095171,3.29937879431315));
#48767=CARTESIAN_POINT('Ctrl Pts',(2.47738511628924,0.794772684000794,3.23773539497539));
#48768=CARTESIAN_POINT('Ctrl Pts',(2.51452673106549,1.06847604194574,3.16043120584603));
#48769=CARTESIAN_POINT('Ctrl Pts',(2.53342242175017,1.18514270861308,3.12917523589806));
#48770=CARTESIAN_POINT('Ctrl Pts',(2.55513657431532,1.30000000000195,3.1001254150738));
#48771=CARTESIAN_POINT('Ctrl Pts',(2.7396711808232,-1.30000000000267,3.2415292971106));
#48772=CARTESIAN_POINT('Ctrl Pts',(2.70247389906199,-1.18514270861358,3.26389070858423));
#48773=CARTESIAN_POINT('Ctrl Pts',(2.66713585044611,-1.06847604194601,3.28696483524763));
#48774=CARTESIAN_POINT('Ctrl Pts',(2.58979308929543,-0.794772684000814,
3.34191719846965));
#48775=CARTESIAN_POINT('Ctrl Pts',(2.54362204572139,-0.636309800095166,
3.38598362134397));
#48776=CARTESIAN_POINT('Ctrl Pts',(2.4807969499755,-0.319434907277143,3.4290724767243));
#48777=CARTESIAN_POINT('Ctrl Pts',(2.45461066784083,-0.158333333333325,
3.44959903115181));
#48778=CARTESIAN_POINT('Ctrl Pts',(2.43210511511045,0.158333333333327,3.43482545787348));
#48779=CARTESIAN_POINT('Ctrl Pts',(2.43594690083246,0.319434907277153,3.39958946421165));
#48780=CARTESIAN_POINT('Ctrl Pts',(2.45260174599739,0.636309800095177,3.32627726736606));
#48781=CARTESIAN_POINT('Ctrl Pts',(2.47315200888497,0.794772684000802,3.26581631617366));
#48782=CARTESIAN_POINT('Ctrl Pts',(2.51186915916835,1.06847604194575,3.18514950803714));
#48783=CARTESIAN_POINT('Ctrl Pts',(2.531519170011,1.18514270861309,3.15145192925572));
#48784=CARTESIAN_POINT('Ctrl Pts',(2.55405997195039,1.30000000000196,3.11897444393546));
#48785=CARTESIAN_POINT('Ctrl Pts',(2.73578893667187,-1.30000000000268,3.25590696673737));
#48786=CARTESIAN_POINT('Ctrl Pts',(2.69783422254653,-1.18514270861358,3.28107360162963));
#48787=CARTESIAN_POINT('Ctrl Pts',(2.66195064570056,-1.06847604194601,3.30620396777811));
#48788=CARTESIAN_POINT('Ctrl Pts',(2.58383714614665,-0.794772684000814,
3.3641763528397));
#48789=CARTESIAN_POINT('Ctrl Pts',(2.5379334691619,-0.636309800095167,3.4077814403611));
#48790=CARTESIAN_POINT('Ctrl Pts',(2.47500953345229,-0.319434907277144,
3.45092863049741));
#48791=CARTESIAN_POINT('Ctrl Pts',(2.44858806405404,-0.158333333333325,
3.47030416649335));
#48792=CARTESIAN_POINT('Ctrl Pts',(2.42648735108728,0.158333333333327,3.45572989129672));
#48793=CARTESIAN_POINT('Ctrl Pts',(2.4309471764933,0.319434907277153,3.42184459057));
#48794=CARTESIAN_POINT('Ctrl Pts',(2.44857027770594,0.636309800095178,3.34887924806674));
#48795=CARTESIAN_POINT('Ctrl Pts',(2.46970583260632,0.794772684000805,3.2892548202756));
#48796=CARTESIAN_POINT('Ctrl Pts',(2.50937611640074,1.06847604194575,3.2056317008609));
#48797=CARTESIAN_POINT('Ctrl Pts',(2.52943926998928,1.18514270861309,3.16980658619545));
#48798=CARTESIAN_POINT('Ctrl Pts',(2.55239378124058,1.30000000000196,3.13435370671735));
#48799=CARTESIAN_POINT('Ctrl Pts',(2.73421818102398,-1.30000000000268,3.2681977674749));
#48800=CARTESIAN_POINT('Ctrl Pts',(2.69571278637597,-1.18514270861358,3.29563003990244));
#48801=CARTESIAN_POINT('Ctrl Pts',(2.65934320270405,-1.06847604194601,3.322376510302));
#48802=CARTESIAN_POINT('Ctrl Pts',(2.58025633933426,-0.794772684000817,
3.38258186765897));
#48803=CARTESIAN_POINT('Ctrl Pts',(2.53384358370785,-0.636309800095168,
3.42546239955407));
#48804=CARTESIAN_POINT('Ctrl Pts',(2.47040513289856,-0.319434907277144,
3.46843740070974));
#48805=CARTESIAN_POINT('Ctrl Pts',(2.44383015879977,-0.158333333333325,
3.48690345475855));
#48806=CARTESIAN_POINT('Ctrl Pts',(2.42202544186461,0.158333333333327,3.4724760370481));
#48807=CARTESIAN_POINT('Ctrl Pts',(2.42704753007698,0.319434907277154,3.4397164682609));
#48808=CARTESIAN_POINT('Ctrl Pts',(2.44555838076725,0.636309800095179,3.36708110532485));
#48809=CARTESIAN_POINT('Ctrl Pts',(2.46742269085271,0.794772684000805,3.30823367937151));
#48810=CARTESIAN_POINT('Ctrl Pts',(2.50770768141108,1.06847604194576,3.22217370120946));
#48811=CARTESIAN_POINT('Ctrl Pts',(2.52794304634436,1.18514270861309,3.18457353925629));
#48812=CARTESIAN_POINT('Ctrl Pts',(2.55097589650418,1.30000000000196,3.14662539105996));
#48813=CARTESIAN_POINT('Ctrl Pts',(2.72948351347113,-1.30000000000268,3.29195966295096));
#48814=CARTESIAN_POINT('Ctrl Pts',(2.68991926187795,-1.18514270861358,3.32394588125519));
#48815=CARTESIAN_POINT('Ctrl Pts',(2.65266915533746,-1.06847604194601,3.35397123658253));
#48816=CARTESIAN_POINT('Ctrl Pts',(2.57196009538581,-0.794772684000816,
3.41880582819428));
#48817=CARTESIAN_POINT('Ctrl Pts',(2.52487679177749,-0.63630980009517,3.46040937964688));
#48818=CARTESIAN_POINT('Ctrl Pts',(2.46094514261025,-0.319434907277145,
3.50330855480773));
#48819=CARTESIAN_POINT('Ctrl Pts',(2.43467027355434,-0.158333333333326,
3.52025618121959));
#48820=CARTESIAN_POINT('Ctrl Pts',(2.41332137892381,0.158333333333328,3.50606492220678));
#48821=CARTESIAN_POINT('Ctrl Pts',(2.41857837798631,0.319434907277154,3.47512095010223));
#48822=CARTESIAN_POINT('Ctrl Pts',(2.43834959261132,0.63630980009518,3.402918177738));
#48823=CARTESIAN_POINT('Ctrl Pts',(2.46111398918522,0.794772684000808,3.34541583863585));
#48824=CARTESIAN_POINT('Ctrl Pts',(2.50354324361101,1.06847604194576,3.25490000136031));
#48825=CARTESIAN_POINT('Ctrl Pts',(2.52487969584024,1.18514270861309,3.2140856974905));
#48826=CARTESIAN_POINT('Ctrl Pts',(2.54918654821652,1.30000000000196,3.17163804176526));
#48827=CARTESIAN_POINT('Ctrl Pts',(2.72369170179333,-1.3000000000027,3.31849454912433));
#48828=CARTESIAN_POINT('Ctrl Pts',(2.68211479421324,-1.18514270861361,3.35520246504919));
#48829=CARTESIAN_POINT('Ctrl Pts',(2.64332497335363,-1.06847604194603,3.38864640930431));
#48830=CARTESIAN_POINT('Ctrl Pts',(2.56015145517037,-0.794772684000832,
3.45836818345907));
#48831=CARTESIAN_POINT('Ctrl Pts',(2.5128150583507,-0.636309800095181,3.49875698222628));
#48832=CARTESIAN_POINT('Ctrl Pts',(2.44867383136127,-0.319434907277151,
3.54174909975053));
#48833=CARTESIAN_POINT('Ctrl Pts',(2.42314097812259,-0.158333333333328,
3.55722010290175));
#48834=CARTESIAN_POINT('Ctrl Pts',(2.40257018414566,0.15833333333333,3.54344456141889));
#48835=CARTESIAN_POINT('Ctrl Pts',(2.4078959153891,0.319434907277158,3.51444953593751));
#48836=CARTESIAN_POINT('Ctrl Pts',(2.42939514255243,0.636309800095189,3.44288530588052));
#48837=CARTESIAN_POINT('Ctrl Pts',(2.45410708551317,0.794772684000823,3.38732971658239));
#48838=CARTESIAN_POINT('Ctrl Pts',(2.49855328806516,1.06847604194578,3.29162722367303));
#48839=CARTESIAN_POINT('Ctrl Pts',(2.5206580533214,1.18514270861311,3.24698429416533));
#48840=CARTESIAN_POINT('Ctrl Pts',(2.54562846964318,1.30000000000198,3.19912449820366));
#48841=CARTESIAN_POINT('Ctrl Pts',(2.71438902447655,-1.30000000000271,3.35633531279331));
#48842=CARTESIAN_POINT('Ctrl Pts',(2.67060459789709,-1.18514270861361,3.40019886347495));
#48843=CARTESIAN_POINT('Ctrl Pts',(2.62994469888926,-1.06847604194604,3.43874235686978));
#48844=CARTESIAN_POINT('Ctrl Pts',(2.54323048194666,-0.794772684000838,
3.51549514060459));
#48845=CARTESIAN_POINT('Ctrl Pts',(2.49451201224887,-0.636309800095185,
3.5536067747533));
#48846=CARTESIAN_POINT('Ctrl Pts',(2.42861015874721,-0.319434907277153,
3.59593822555784));
#48847=CARTESIAN_POINT('Ctrl Pts',(2.40230917701206,-0.158333333333329,
3.60824880302406));
#48848=CARTESIAN_POINT('Ctrl Pts',(2.38278887602257,0.158333333333331,3.59506410414001));
#48849=CARTESIAN_POINT('Ctrl Pts',(2.39033055985627,0.31943490727716,3.57007363504647));
#48850=CARTESIAN_POINT('Ctrl Pts',(2.41492085725434,0.636309800095193,3.49985764591031));
#48851=CARTESIAN_POINT('Ctrl Pts',(2.44086394794052,0.794772684000828,3.44643060171251));
#48852=CARTESIAN_POINT('Ctrl Pts',(2.48924552311111,1.06847604194578,3.34375288445897));
#48853=CARTESIAN_POINT('Ctrl Pts',(2.51337592653575,1.18514270861312,3.29400773222963));
#48854=CARTESIAN_POINT('Ctrl Pts',(2.54069414220766,1.30000000000199,3.23896280698576));
#48855=CARTESIAN_POINT('Ctrl Pts',(2.70713559815903,-1.30000000000272,3.38544760191281));
#48856=CARTESIAN_POINT('Ctrl Pts',(2.66108666670748,-1.18514270861363,3.43457778468442));
#48857=CARTESIAN_POINT('Ctrl Pts',(2.61851679459819,-1.06847604194605,3.47683322532625));
#48858=CARTESIAN_POINT('Ctrl Pts',(2.52820919701641,-0.794772684000844,
3.55856971677326));
#48859=CARTESIAN_POINT('Ctrl Pts',(2.47766951391152,-0.63630980009519,3.5944422383161));
#48860=CARTESIAN_POINT('Ctrl Pts',(2.41092519018967,-0.319434907277155,
3.63654891312596));
#48861=CARTESIAN_POINT('Ctrl Pts',(2.38612507388147,-0.158333333333331,
3.64759825207347));
#48862=CARTESIAN_POINT('Ctrl Pts',(2.36753152447389,0.158333333333333,3.63497645717648));
#48863=CARTESIAN_POINT('Ctrl Pts',(2.37474937021344,0.319434907277166,3.61201925378152));
#48864=CARTESIAN_POINT('Ctrl Pts',(2.40156007039164,0.636309800095202,3.54274866664481));
#48865=CARTESIAN_POINT('Ctrl Pts',(2.43021686726533,0.794772684000834,3.49184456180963));
#48866=CARTESIAN_POINT('Ctrl Pts',(2.48166834545503,1.06847604194579,3.38378694257873));
#48867=CARTESIAN_POINT('Ctrl Pts',(2.50705731805605,1.18514270861313,3.32994473516944));
#48868=CARTESIAN_POINT('Ctrl Pts',(2.53556382481485,1.300000000002,3.26903445978667));
#48869=CARTESIAN_POINT('Ctrl Pts',(2.69935280611515,-1.30000000000273,3.4142463597142));
#48870=CARTESIAN_POINT('Ctrl Pts',(2.65091913730647,-1.18514270861363,3.46848708019251));
#48871=CARTESIAN_POINT('Ctrl Pts',(2.60632467787954,-1.06847604194605,3.51431952016311));
#48872=CARTESIAN_POINT('Ctrl Pts',(2.51217189721573,-0.794772684000848,
3.6007768151995));
#48873=CARTESIAN_POINT('Ctrl Pts',(2.45996887884519,-0.636309800095194,
3.63447452807947));
#48874=CARTESIAN_POINT('Ctrl Pts',(2.39156773297291,-0.319434907277157,
3.67585824322938));
#48875=CARTESIAN_POINT('Ctrl Pts',(2.36677677594353,-0.158333333333331,
3.68480618023814));
#48876=CARTESIAN_POINT('Ctrl Pts',(2.34892395383732,0.158333333333334,3.67266358137842));
#48877=CARTESIAN_POINT('Ctrl Pts',(2.35719358301814,0.319434907277165,3.65251724971171));
#48878=CARTESIAN_POINT('Ctrl Pts',(2.38651765777384,0.636309800095202,3.58447665900661));
#48879=CARTESIAN_POINT('Ctrl Pts',(2.41666791960658,0.794772684000837,3.53559913548754));
#48880=CARTESIAN_POINT('Ctrl Pts',(2.47198053053757,1.0684760419458,3.42268260092749));
#48881=CARTESIAN_POINT('Ctrl Pts',(2.49935282260984,1.18514270861314,3.36515185339334));
#48882=CARTESIAN_POINT('Ctrl Pts',(2.53015462701651,1.30000000000201,3.29896774216626));
#48883=CARTESIAN_POINT('Ctrl Pts',(2.69303318688899,-1.30000000000273,3.43401667925717));
#48884=CARTESIAN_POINT('Ctrl Pts',(2.64282935584548,-1.18514270861363,3.49194305826096));
#48885=CARTESIAN_POINT('Ctrl Pts',(2.59667057889062,-1.06847604194605,3.54031522326202));
#48886=CARTESIAN_POINT('Ctrl Pts',(2.49937945424869,-0.79477268400085,3.62999245557226));
#48887=CARTESIAN_POINT('Ctrl Pts',(2.44467031211378,-0.636309800095196,
3.66134362032266));
#48888=CARTESIAN_POINT('Ctrl Pts',(2.37628184723862,-0.319434907277159,
3.70291872218279));
#48889=CARTESIAN_POINT('Ctrl Pts',(2.35498741875346,-0.158333333333332,
3.71239366789374));
#48890=CARTESIAN_POINT('Ctrl Pts',(2.33816277204694,0.158333333333334,3.70090332782829));
#48891=CARTESIAN_POINT('Ctrl Pts',(2.34446568277421,0.319434907277166,3.68123393892042));
#48892=CARTESIAN_POINT('Ctrl Pts',(2.37484960204422,0.636309800095205,3.61361419306542));
#48893=CARTESIAN_POINT('Ctrl Pts',(2.4070943212819,0.794772684000841,3.56670915350597));
#48894=CARTESIAN_POINT('Ctrl Pts',(2.46534344402644,1.0684760419458,3.45033103710803));
#48895=CARTESIAN_POINT('Ctrl Pts',(2.49412215195454,1.18514270861314,3.39011485922067));
#48896=CARTESIAN_POINT('Ctrl Pts',(2.52646568091726,1.30000000000202,3.32005827780055));
#48897=CARTESIAN_POINT('Ctrl Pts',(2.68881095174143,-1.30000000000273,3.44818305017374));
#48898=CARTESIAN_POINT('Ctrl Pts',(2.63669007242356,-1.18514270861363,3.50812985442003));
#48899=CARTESIAN_POINT('Ctrl Pts',(2.58929489284264,-1.06847604194606,3.55806783061209));
#48900=CARTESIAN_POINT('Ctrl Pts',(2.49071985840326,-0.794772684000852,
3.65031215060882));
#48901=CARTESIAN_POINT('Ctrl Pts',(2.43767831743658,-0.636309800095195,
3.68199369795424));
#48902=CARTESIAN_POINT('Ctrl Pts',(2.37003893525433,-0.319434907277157,
3.72404063399689));
#48903=CARTESIAN_POINT('Ctrl Pts',(2.34957190091252,-0.158333333333332,
3.73290265012859));
#48904=CARTESIAN_POINT('Ctrl Pts',(2.33223463491217,0.158333333333334,3.72113567254182));
#48905=CARTESIAN_POINT('Ctrl Pts',(2.33644686910212,0.319434907277166,3.70137589803932));
#48906=CARTESIAN_POINT('Ctrl Pts',(2.36656658377296,0.636309800095204,3.63358993894587));
#48907=CARTESIAN_POINT('Ctrl Pts',(2.39985803922327,0.794772684000837,3.5879471723796));
#48908=CARTESIAN_POINT('Ctrl Pts',(2.45974497985535,1.0684760419458,3.46916916360371));
#48909=CARTESIAN_POINT('Ctrl Pts',(2.48941623434979,1.18514270861314,3.40715690064001));
#48910=CARTESIAN_POINT('Ctrl Pts',(2.52283590576881,1.30000000000202,3.33454697355289));
#48911=CARTESIAN_POINT('Ctrl Pts',(2.6829039520614,-1.30000000000273,3.4648600390468));
#48912=CARTESIAN_POINT('Ctrl Pts',(2.6282815105453,-1.18514270861363,3.52754575513347));
#48913=CARTESIAN_POINT('Ctrl Pts',(2.5794116548837,-1.06847604194606,3.57971224017919));
#48914=CARTESIAN_POINT('Ctrl Pts',(2.47980213604945,-0.794772684000851,
3.67592572843441));
#48915=CARTESIAN_POINT('Ctrl Pts',(2.42997521426678,-0.636309800095196,
3.70885360105528));
#48916=CARTESIAN_POINT('Ctrl Pts',(2.36410441800568,-0.319434907277158,
3.75213277591685));
#48917=CARTESIAN_POINT('Ctrl Pts',(2.34457233682742,-0.158333333333332,
3.76008693715092));
#48918=CARTESIAN_POINT('Ctrl Pts',(2.32729940694406,0.158333333333334,3.74838365192667));
#48919=CARTESIAN_POINT('Ctrl Pts',(2.33032257384052,0.319434907277166,3.72943266456022));
#48920=CARTESIAN_POINT('Ctrl Pts',(2.35945341085199,0.636309800095205,3.66087573405795));
#48921=CARTESIAN_POINT('Ctrl Pts',(2.3912258713284,0.794772684000838,3.61494599460186));
#48922=CARTESIAN_POINT('Ctrl Pts',(2.45236846246531,1.0684760419458,3.49226103554975));
#48923=CARTESIAN_POINT('Ctrl Pts',(2.48325251042926,1.18514270861314,3.42782901639173));
#48924=CARTESIAN_POINT('Ctrl Pts',(2.5185542442102,1.30000000000202,3.35207075092373));
#48925=CARTESIAN_POINT('Ctrl Pts',(2.67899628993141,-1.30000000000274,3.47627965711681));
#48926=CARTESIAN_POINT('Ctrl Pts',(2.62148033775266,-1.18514270861364,3.54015492010688));
#48927=CARTESIAN_POINT('Ctrl Pts',(2.57119727859278,-1.06847604194606,3.59350430823753));
#48928=CARTESIAN_POINT('Ctrl Pts',(2.47174278265131,-0.794772684000851,
3.69243519070814));
#48929=CARTESIAN_POINT('Ctrl Pts',(2.42808446301743,-0.636309800095197,
3.72772405735239));
#48930=CARTESIAN_POINT('Ctrl Pts',(2.36541685428271,-0.319434907277159,
3.77235288610033));
#48931=CARTESIAN_POINT('Ctrl Pts',(2.346171214744,-0.158333333333332,3.77926048785863));
#48932=CARTESIAN_POINT('Ctrl Pts',(2.32904419103436,0.158333333333334,3.76759838522902));
#48933=CARTESIAN_POINT('Ctrl Pts',(2.33182399968641,0.319434907277167,3.74960279228391));
#48934=CARTESIAN_POINT('Ctrl Pts',(2.35825829213827,0.636309800095206,3.68004967650707));
#48935=CARTESIAN_POINT('Ctrl Pts',(2.38472809612599,0.79477268400084,3.63256364253536));
#48936=CARTESIAN_POINT('Ctrl Pts',(2.44568313888403,1.0684760419458,3.5071297018696));
#48937=CARTESIAN_POINT('Ctrl Pts',(2.47774091685542,1.18514270861315,3.44130295284402));
#48938=CARTESIAN_POINT('Ctrl Pts',(2.51547129339511,1.30000000000202,3.36394515992168));
#48939=CARTESIAN_POINT('Ctrl Pts',(2.67879510330428,-1.30000000000274,3.4848793737609));
#48940=CARTESIAN_POINT('Ctrl Pts',(2.62131393065235,-1.18514270861364,3.54850574591786));
#48941=CARTESIAN_POINT('Ctrl Pts',(2.57136732543471,-1.06847604194606,3.60177947255492));
#48942=CARTESIAN_POINT('Ctrl Pts',(2.4733870336565,-0.794772684000851,3.70093575626798));
#48943=CARTESIAN_POINT('Ctrl Pts',(2.4321376027347,-0.636309800095197,3.73710797922267));
#48944=CARTESIAN_POINT('Ctrl Pts',(2.37107459905216,-0.319434907277159,
3.7822562302209));
#48945=CARTESIAN_POINT('Ctrl Pts',(2.35179040064045,-0.158333333333332,
3.78919923474563));
#48946=CARTESIAN_POINT('Ctrl Pts',(2.33489442655109,0.158333333333334,3.77758912426359));
#48947=CARTESIAN_POINT('Ctrl Pts',(2.33820931733128,0.319434907277167,3.75969933838138));
#48948=CARTESIAN_POINT('Ctrl Pts',(2.36296888549193,0.636309800095206,3.68955097462145));
#48949=CARTESIAN_POINT('Ctrl Pts',(2.38602389855414,0.79477268400084,3.64077817435492));
#48950=CARTESIAN_POINT('Ctrl Pts',(2.4456425950795,1.0684760419458,3.5151865828561));
#48951=CARTESIAN_POINT('Ctrl Pts',(2.47765621323778,1.18514270861315,3.44956557353161));
#48952=CARTESIAN_POINT('Ctrl Pts',(2.51587672491888,1.30000000000202,3.37268750121553));
#48953=CARTESIAN_POINT('Ctrl Pts',(2.67879510330291,-1.3,3.48487937376242));
#48954=CARTESIAN_POINT('Ctrl Pts',(2.62131393065155,-1.18514270861178,3.54850574591871));
#48955=CARTESIAN_POINT('Ctrl Pts',(2.57136732543437,-1.06847604194512,3.60177947255526));
#48956=CARTESIAN_POINT('Ctrl Pts',(2.4733870336565,-0.794772684000851,3.70093575626798));
#48957=CARTESIAN_POINT('Ctrl Pts',(2.4321376027347,-0.636309800095197,3.73710797922267));
#48958=CARTESIAN_POINT('Ctrl Pts',(2.37107459905216,-0.319434907277159,
3.7822562302209));
#48959=CARTESIAN_POINT('Ctrl Pts',(2.35179040064045,-0.158333333333332,
3.78919923474563));
#48960=CARTESIAN_POINT('Ctrl Pts',(2.33489442655109,0.158333333333334,3.77758912426359));
#48961=CARTESIAN_POINT('Ctrl Pts',(2.33820931733128,0.319434907277167,3.75969933838138));
#48962=CARTESIAN_POINT('Ctrl Pts',(2.36296888549193,0.636309800095206,3.68955097462145));
#48963=CARTESIAN_POINT('Ctrl Pts',(2.38602389855414,0.79477268400084,3.64077817435492));
#48964=CARTESIAN_POINT('Ctrl Pts',(2.44564259507935,1.06847604194511,3.51518658285641));
#48965=CARTESIAN_POINT('Ctrl Pts',(2.47765621323741,1.18514270861178,3.44956557353238));
#48966=CARTESIAN_POINT('Ctrl Pts',(2.5158767249182,1.3,3.37268750121688));
#48967=CARTESIAN_POINT('',(2.73378250710872,-1.2,3.07338719967255));
#48968=CARTESIAN_POINT('Ctrl Pts',(2.73378250710872,-1.2,3.07338719967255));
#48969=CARTESIAN_POINT('Ctrl Pts',(2.7357577738517,-1.2168297082725,3.09488352363361));
#48970=CARTESIAN_POINT('Ctrl Pts',(2.73868491450415,-1.23325632720283,3.1165994859212));
#48971=CARTESIAN_POINT('Ctrl Pts',(2.7416199046039,-1.25866340409469,3.14922928548443));
#48972=CARTESIAN_POINT('Ctrl Pts',(2.74261161481058,-1.26676846238795,3.15969392154395));
#48973=CARTESIAN_POINT('Ctrl Pts',(2.74425212505128,-1.28145222431456,3.17857382838032));
#48974=CARTESIAN_POINT('Ctrl Pts',(2.74535078767749,-1.29188212206828,3.19196062087639));
#48975=CARTESIAN_POINT('Ctrl Pts',(2.74593693625412,-1.29845800981103,3.20033871480917));
#48976=CARTESIAN_POINT('Ctrl Pts',(2.74600242614502,-1.29922960688975,3.20131966196731));
#48977=CARTESIAN_POINT('Ctrl Pts',(2.74606318243978,-1.30000000000266,3.20229603421878));
#48978=CARTESIAN_POINT('',(2.60194865074806,-0.653834841416699,2.98901873447389));
#48979=CARTESIAN_POINT('Ctrl Pts',(2.60194865076408,-0.653834841416013,
2.9890187344531));
#48980=CARTESIAN_POINT('Ctrl Pts',(2.61576784735542,-0.717856062975954,
2.99755756131031));
#48981=CARTESIAN_POINT('Ctrl Pts',(2.62702784454639,-0.763802346224156,
3.00458546056376));
#48982=CARTESIAN_POINT('Ctrl Pts',(2.6708664756529,-0.949540328209464,3.03224190415644));
#48983=CARTESIAN_POINT('Ctrl Pts',(2.69381959728105,-1.04583430085205,3.04691272554419));
#48984=CARTESIAN_POINT('Ctrl Pts',(2.73378250710872,-1.2,3.07338719967255));
#48985=CARTESIAN_POINT('',(2.48224831221869,0.653834841531101,2.91736724473281));
#48986=CARTESIAN_POINT('Ctrl Pts',(2.48224831221869,0.6538348415311,2.91736724473281));
#48987=CARTESIAN_POINT('Ctrl Pts',(2.47847890444284,0.57579108168247,2.95887093612136));
#48988=CARTESIAN_POINT('Ctrl Pts',(2.47600131421347,0.493921151117629,2.99371026845236));
#48989=CARTESIAN_POINT('Ctrl Pts',(2.47494821893025,0.338203801397658,3.04438967831501));
#48990=CARTESIAN_POINT('Ctrl Pts',(2.47583991291864,0.265715671510878,3.06228273998636));
#48991=CARTESIAN_POINT('Ctrl Pts',(2.48131031772334,0.129742783470322,3.08607547669105));
#48992=CARTESIAN_POINT('Ctrl Pts',(2.48530809277579,0.0666420753572764,
3.09333289107435));
#48993=CARTESIAN_POINT('Ctrl Pts',(2.49656212049516,-0.0595517108187469,
3.10050296874366));
#48994=CARTESIAN_POINT('Ctrl Pts',(2.5038959934916,-0.122800467221057,3.10048501116942));
#48995=CARTESIAN_POINT('Ctrl Pts',(2.52282604869386,-0.260148767886255,
3.0919924718622));
#48996=CARTESIAN_POINT('Ctrl Pts',(2.53495894889212,-0.333947398986749,
3.08197900091245));
#48997=CARTESIAN_POINT('Ctrl Pts',(2.56433428307125,-0.491233239064203,
3.04808483264696));
#48998=CARTESIAN_POINT('Ctrl Pts',(2.58224468806056,-0.574172289671449,
3.02219719078165));
#48999=CARTESIAN_POINT('Ctrl Pts',(2.60194865076353,-0.653834841428418,
2.98901873451122));
#49000=CARTESIAN_POINT('',(2.54446987687431,1.2,2.95404038576917));
#49001=CARTESIAN_POINT('Ctrl Pts',(2.54446987687431,1.2,2.95404038576917));
#49002=CARTESIAN_POINT('Ctrl Pts',(2.53342410082955,1.13191853104164,2.94742100005518));
#49003=CARTESIAN_POINT('Ctrl Pts',(2.51940373078794,1.03495910820303,2.93908009495677));
#49004=CARTESIAN_POINT('Ctrl Pts',(2.49230898042137,0.795381693602028,2.9231940999664));
#49005=CARTESIAN_POINT('Ctrl Pts',(2.48794042596448,0.741811055998074,2.92066643953794));
#49006=CARTESIAN_POINT('Ctrl Pts',(2.48224831221869,0.653834841531101,2.91736724473281));
#49007=CARTESIAN_POINT('Ctrl Pts',(2.55661739137893,1.29999999999998,3.07856729836589));
#49008=CARTESIAN_POINT('Ctrl Pts',(2.55522672776558,1.28313639696102,3.05785996776105));
#49009=CARTESIAN_POINT('Ctrl Pts',(2.55298386248016,1.26654349104865,3.03699927317881));
#49010=CARTESIAN_POINT('Ctrl Pts',(2.54970999277994,1.23742205883468,3.0008947194452));
#49011=CARTESIAN_POINT('Ctrl Pts',(2.54814390762507,1.2200626218235,2.97963140604976));
#49012=CARTESIAN_POINT('Ctrl Pts',(2.54446987687431,1.2,2.95404038576917));
#49013=CARTESIAN_POINT('Ctrl Pts',(2.67879510330291,-1.3,3.48487937376242));
#49014=CARTESIAN_POINT('Ctrl Pts',(2.62131393065155,-1.18514270861178,3.54850574591871));
#49015=CARTESIAN_POINT('Ctrl Pts',(2.57136732543437,-1.06847604194512,3.60177947255526));
#49016=CARTESIAN_POINT('Ctrl Pts',(2.4733870336565,-0.794772684000851,3.70093575626798));
#49017=CARTESIAN_POINT('Ctrl Pts',(2.43213760273471,-0.636309800095197,
3.73710797922267));
#49018=CARTESIAN_POINT('Ctrl Pts',(2.37107459905216,-0.319434907277159,
3.7822562302209));
#49019=CARTESIAN_POINT('Ctrl Pts',(2.35179040064045,-0.158333333333332,
3.78919923474564));
#49020=CARTESIAN_POINT('Ctrl Pts',(2.33489442655109,0.158333333333334,3.77758912426359));
#49021=CARTESIAN_POINT('Ctrl Pts',(2.33820931733128,0.319434907277167,3.75969933838138));
#49022=CARTESIAN_POINT('Ctrl Pts',(2.36296888549193,0.636309800095206,3.68955097462145));
#49023=CARTESIAN_POINT('Ctrl Pts',(2.38602389855414,0.79477268400084,3.64077817435492));
#49024=CARTESIAN_POINT('Ctrl Pts',(2.44564259507935,1.06847604194511,3.51518658285641));
#49025=CARTESIAN_POINT('Ctrl Pts',(2.47765621323741,1.18514270861178,3.44956557353238));
#49026=CARTESIAN_POINT('Ctrl Pts',(2.5158767249182,1.3,3.37268750121688));
#49027=CARTESIAN_POINT('Ctrl Pts',(2.74004401157309,-1.3,3.53143772972948));
#49028=CARTESIAN_POINT('Ctrl Pts',(2.68128836180793,-1.18514270861178,3.59389081034382));
#49029=CARTESIAN_POINT('Ctrl Pts',(2.63048511284273,-1.06847604194512,3.64631488384437));
#49030=CARTESIAN_POINT('Ctrl Pts',(2.53149108129824,-0.794772684000851,
3.74425596830184));
#49031=CARTESIAN_POINT('Ctrl Pts',(2.49090436112714,-0.636309800095197,
3.78070353178887));
#49032=CARTESIAN_POINT('Ctrl Pts',(2.43050771496334,-0.319434907277159,
3.82587729417744));
#49033=CARTESIAN_POINT('Ctrl Pts',(2.41232163607126,-0.158333333333332,
3.83339959597414));
#49034=CARTESIAN_POINT('Ctrl Pts',(2.3956366485587,0.158333333333334,3.82149908738234));
#49035=CARTESIAN_POINT('Ctrl Pts',(2.39806125730008,0.319434907277167,3.80274394047715));
#49036=CARTESIAN_POINT('Ctrl Pts',(2.42259064688909,0.636309800095206,3.73196971651));
#49037=CARTESIAN_POINT('Ctrl Pts',(2.4451790066595,0.79477268400084,3.68265172576932));
#49038=CARTESIAN_POINT('Ctrl Pts',(2.50626668917078,1.06847604194511,3.55764874086027));
#49039=CARTESIAN_POINT('Ctrl Pts',(2.53935309295667,1.18514270861178,3.49257989089658));
#49040=CARTESIAN_POINT('Ctrl Pts',(2.57908330629107,1.3,3.41655135131922));
#49041=CARTESIAN_POINT('Ctrl Pts',(2.80129291984328,-1.3,3.57799608569655));
#49042=CARTESIAN_POINT('Ctrl Pts',(2.7412627929643,-1.18514270861178,3.63927587476892));
#49043=CARTESIAN_POINT('Ctrl Pts',(2.68960290025109,-1.06847604194512,3.69085029513349));
#49044=CARTESIAN_POINT('Ctrl Pts',(2.58959512893997,-0.794772684000851,
3.7875761803357));
#49045=CARTESIAN_POINT('Ctrl Pts',(2.54967111951957,-0.636309800095197,
3.82429908435506));
#49046=CARTESIAN_POINT('Ctrl Pts',(2.48994083087453,-0.319434907277159,
3.86949835813398));
#49047=CARTESIAN_POINT('Ctrl Pts',(2.47285287150207,-0.158333333333332,
3.87759995720265));
#49048=CARTESIAN_POINT('Ctrl Pts',(2.4563788705663,0.158333333333334,3.86540905050109));
#49049=CARTESIAN_POINT('Ctrl Pts',(2.45791319726889,0.319434907277167,3.84578854257292));
#49050=CARTESIAN_POINT('Ctrl Pts',(2.48221240828625,0.636309800095206,3.77438845839854));
#49051=CARTESIAN_POINT('Ctrl Pts',(2.50433411476485,0.79477268400084,3.72452527718373));
#49052=CARTESIAN_POINT('Ctrl Pts',(2.5668907832622,1.06847604194511,3.60011089886413));
#49053=CARTESIAN_POINT('Ctrl Pts',(2.60104997267594,1.18514270861178,3.53559420826078));
#49054=CARTESIAN_POINT('Ctrl Pts',(2.64228988766393,1.3,3.46041520142157));
#49055=CARTESIAN_POINT('Ctrl Pts',(2.86254182811346,-1.3,3.62455444166361));
#49056=CARTESIAN_POINT('Ctrl Pts',(2.80123722412067,-1.18514270861178,3.68466093919403));
#49057=CARTESIAN_POINT('Ctrl Pts',(2.74872068765945,-1.06847604194512,3.73538570642261));
#49058=CARTESIAN_POINT('Ctrl Pts',(2.6476991765817,-0.794772684000851,3.83089639236955));
#49059=CARTESIAN_POINT('Ctrl Pts',(2.60843787791201,-0.636309800095197,
3.86789463692126));
#49060=CARTESIAN_POINT('Ctrl Pts',(2.54937394678571,-0.319434907277159,
3.91311942209052));
#49061=CARTESIAN_POINT('Ctrl Pts',(2.53338410693289,-0.158333333333332,
3.92180031843115));
#49062=CARTESIAN_POINT('Ctrl Pts',(2.5171210925739,0.158333333333334,3.90931901361984));
#49063=CARTESIAN_POINT('Ctrl Pts',(2.5177651372377,0.319434907277167,3.88883314466868));
#49064=CARTESIAN_POINT('Ctrl Pts',(2.54183416968341,0.636309800095206,3.81680720028709));
#49065=CARTESIAN_POINT('Ctrl Pts',(2.56348922287021,0.79477268400084,3.76639882859814));
#49066=CARTESIAN_POINT('Ctrl Pts',(2.62751487735363,1.06847604194511,3.64257305686799));
#49067=CARTESIAN_POINT('Ctrl Pts',(2.6627468523952,1.18514270861178,3.57860852562499));
#49068=CARTESIAN_POINT('Ctrl Pts',(2.70549646903679,1.3,3.50427905152391));
#49069=CARTESIAN_POINT('Ctrl Pts',(2.86254182811346,-1.3,3.62455444166361));
#49070=CARTESIAN_POINT('Ctrl Pts',(2.80123722412067,-1.18514270861178,3.68466093919403));
#49071=CARTESIAN_POINT('Ctrl Pts',(2.74872068765946,-1.06847604194512,3.73538570642261));
#49072=CARTESIAN_POINT('Ctrl Pts',(2.6476991765817,-0.794772684000851,3.83089639236955));
#49073=CARTESIAN_POINT('Ctrl Pts',(2.60843787791201,-0.636309800095197,
3.86789463692126));
#49074=CARTESIAN_POINT('Ctrl Pts',(2.54937394678571,-0.319434907277159,
3.91311942209052));
#49075=CARTESIAN_POINT('Ctrl Pts',(2.53338410693288,-0.158333333333332,
3.92180031843115));
#49076=CARTESIAN_POINT('Ctrl Pts',(2.5171210925739,0.158333333333334,3.90931901361984));
#49077=CARTESIAN_POINT('Ctrl Pts',(2.5177651372377,0.319434907277167,3.88883314466868));
#49078=CARTESIAN_POINT('Ctrl Pts',(2.54183416968341,0.636309800095206,3.81680720028709));
#49079=CARTESIAN_POINT('Ctrl Pts',(2.5634892228702,0.79477268400084,3.76639882859813));
#49080=CARTESIAN_POINT('Ctrl Pts',(2.62751487735363,1.06847604194511,3.64257305686799));
#49081=CARTESIAN_POINT('Ctrl Pts',(2.6627468523952,1.18514270861178,3.57860852562499));
#49082=CARTESIAN_POINT('Ctrl Pts',(2.70549646903679,1.3,3.50427905152391));
#49083=CARTESIAN_POINT('Ctrl Pts',(2.86254182811642,-1.30000000000554,3.62455444166071));
#49084=CARTESIAN_POINT('Ctrl Pts',(2.80123722412236,-1.18514270861553,3.6846609391924));
#49085=CARTESIAN_POINT('Ctrl Pts',(2.74872068766016,-1.06847604194702,3.73538570642194));
#49086=CARTESIAN_POINT('Ctrl Pts',(2.6476991765817,-0.794772684000851,3.83089639236955));
#49087=CARTESIAN_POINT('Ctrl Pts',(2.60843787791201,-0.636309800095197,
3.86789463692126));
#49088=CARTESIAN_POINT('Ctrl Pts',(2.54937394678571,-0.319434907277159,
3.91311942209052));
#49089=CARTESIAN_POINT('Ctrl Pts',(2.53338410693289,-0.158333333333332,
3.92180031843115));
#49090=CARTESIAN_POINT('Ctrl Pts',(2.5171210925739,0.158333333333334,3.90931901361984));
#49091=CARTESIAN_POINT('Ctrl Pts',(2.5177651372377,0.319434907277167,3.88883314466868));
#49092=CARTESIAN_POINT('Ctrl Pts',(2.54183416968341,0.636309800095206,3.81680720028709));
#49093=CARTESIAN_POINT('Ctrl Pts',(2.56348922287021,0.79477268400084,3.76639882859813));
#49094=CARTESIAN_POINT('Ctrl Pts',(2.62751487735364,1.06847604194517,3.64257305686796));
#49095=CARTESIAN_POINT('Ctrl Pts',(2.66274685239524,1.18514270861189,3.57860852562492));
#49096=CARTESIAN_POINT('Ctrl Pts',(2.70549646903686,1.30000000000017,3.5042790515238));
#49097=CARTESIAN_POINT('Ctrl Pts',(2.87098157396645,-1.30000000000554,3.62223849797031));
#49098=CARTESIAN_POINT('Ctrl Pts',(2.80906926848047,-1.18514270861553,3.68202709109595));
#49099=CARTESIAN_POINT('Ctrl Pts',(2.7563707080711,-1.06847604194702,3.73285743386342));
#49100=CARTESIAN_POINT('Ctrl Pts',(2.65591208554583,-0.794772684000851,
3.8295903438114));
#49101=CARTESIAN_POINT('Ctrl Pts',(2.61892980277957,-0.636309800095197,
3.86943861486421));
#49102=CARTESIAN_POINT('Ctrl Pts',(2.56094950437883,-0.319434907277159,
3.91607221576025));
#49103=CARTESIAN_POINT('Ctrl Pts',(2.54469368652178,-0.158333333333332,
3.92427691498543));
#49104=CARTESIAN_POINT('Ctrl Pts',(2.52830982643484,0.158333333333334,3.91159193538119));
#49105=CARTESIAN_POINT('Ctrl Pts',(2.52893211645302,0.319434907277167,3.89115367810119));
#49106=CARTESIAN_POINT('Ctrl Pts',(2.55201129877011,0.636309800095206,3.81776217390742));
#49107=CARTESIAN_POINT('Ctrl Pts',(2.57208184262637,0.79477268400084,3.76533578503149));
#49108=CARTESIAN_POINT('Ctrl Pts',(2.63543757364827,1.06847604194517,3.64017761464239));
#49109=CARTESIAN_POINT('Ctrl Pts',(2.67063753705879,1.18514270861189,3.57586971600027));
#49110=CARTESIAN_POINT('Ctrl Pts',(2.71361311548166,1.30000000000017,3.5014302531102));
#49111=CARTESIAN_POINT('Ctrl Pts',(2.88130082125157,-1.30000000000553,3.61561587076792));
#49112=CARTESIAN_POINT('Ctrl Pts',(2.82016066715714,-1.18514270861553,3.67260438117326));
#49113=CARTESIAN_POINT('Ctrl Pts',(2.76842861614806,-1.06847604194701,3.72189205592847));
#49114=CARTESIAN_POINT('Ctrl Pts',(2.6706518295684,-0.794772684000848,3.817965973679));
#49115=CARTESIAN_POINT('Ctrl Pts',(2.63680341206716,-0.636309800095194,
3.86239125090444));
#49116=CARTESIAN_POINT('Ctrl Pts',(2.58060872343043,-0.319434907277157,
3.91128594284546));
#49117=CARTESIAN_POINT('Ctrl Pts',(2.56351725959355,-0.158333333333332,
3.92001259183717));
#49118=CARTESIAN_POINT('Ctrl Pts',(2.5470343810601,0.158333333333334,3.90718754649781));
#49119=CARTESIAN_POINT('Ctrl Pts',(2.54853327574153,0.319434907277167,3.88612733727331));
#49120=CARTESIAN_POINT('Ctrl Pts',(2.56934003151366,0.636309800095205,3.81010783163589));
#49121=CARTESIAN_POINT('Ctrl Pts',(2.58529810153918,0.794772684000837,3.75258095831877));
#49122=CARTESIAN_POINT('Ctrl Pts',(2.64602744646709,1.06847604194516,3.62811825223073));
#49123=CARTESIAN_POINT('Ctrl Pts',(2.68053526324991,1.18514270861188,3.5655147599639));
#49124=CARTESIAN_POINT('Ctrl Pts',(2.72326341364027,1.30000000000016,3.49418306909796));
#49125=CARTESIAN_POINT('Ctrl Pts',(2.89657701929988,-1.30000000000553,3.60605436272481));
#49126=CARTESIAN_POINT('Ctrl Pts',(2.83785983129768,-1.18514270861553,3.66028459218314));
#49127=CARTESIAN_POINT('Ctrl Pts',(2.78806648256914,-1.06847604194702,3.70767886828241));
#49128=CARTESIAN_POINT('Ctrl Pts',(2.69364973981185,-0.794772684000849,
3.80137670747613));
#49129=CARTESIAN_POINT('Ctrl Pts',(2.66057259609715,-0.636309800095194,
3.84718746245279));
#49130=CARTESIAN_POINT('Ctrl Pts',(2.60545054146012,-0.319434907277157,
3.89681571822015));
#49131=CARTESIAN_POINT('Ctrl Pts',(2.58798683559333,-0.158333333333332,
3.90695072166245));
#49132=CARTESIAN_POINT('Ctrl Pts',(2.57140695597793,0.158333333333334,3.89406819926671));
#49133=CARTESIAN_POINT('Ctrl Pts',(2.57340807017908,0.319434907277166,3.87176905961988));
#49134=CARTESIAN_POINT('Ctrl Pts',(2.59248226872427,0.636309800095204,3.79443673235879));
#49135=CARTESIAN_POINT('Ctrl Pts',(2.60631386943291,0.794772684000837,3.73428739218371));
#49136=CARTESIAN_POINT('Ctrl Pts',(2.66359704128096,1.06847604194516,3.61205146082038));
#49137=CARTESIAN_POINT('Ctrl Pts',(2.69643828805896,1.18514270861188,3.55154131212699));
#49138=CARTESIAN_POINT('Ctrl Pts',(2.73732501907265,1.30000000000016,3.48343242013976));
#49139=CARTESIAN_POINT('Ctrl Pts',(2.90936639791106,-1.30000000000553,3.59827482203786));
#49140=CARTESIAN_POINT('Ctrl Pts',(2.85272180916184,-1.18514270861552,3.65068715009277));
#49141=CARTESIAN_POINT('Ctrl Pts',(2.80433520504782,-1.06847604194701,3.69666533731781));
#49142=CARTESIAN_POINT('Ctrl Pts',(2.71163006634977,-0.794772684000845,
3.78801999524921));
#49143=CARTESIAN_POINT('Ctrl Pts',(2.67698192370522,-0.636309800095192,
3.83317642236382));
#49144=CARTESIAN_POINT('Ctrl Pts',(2.62202362155589,-0.319434907277156,
3.88293393740567));
#49145=CARTESIAN_POINT('Ctrl Pts',(2.60521467878967,-0.158333333333331,
3.894953219045));
#49146=CARTESIAN_POINT('Ctrl Pts',(2.58907353697783,0.158333333333333,3.88248974574418));
#49147=CARTESIAN_POINT('Ctrl Pts',(2.59153304544427,0.319434907277166,3.85934407438143));
#49148=CARTESIAN_POINT('Ctrl Pts',(2.60996342472877,0.636309800095202,3.78147581865173));
#49149=CARTESIAN_POINT('Ctrl Pts',(2.62289827165848,0.794772684000833,3.71977755633891));
#49150=CARTESIAN_POINT('Ctrl Pts',(2.67812342430724,1.06847604194516,3.59952069917244));
#49151=CARTESIAN_POINT('Ctrl Pts',(2.70985831899148,1.18514270861188,3.54065686063037));
#49152=CARTESIAN_POINT('Ctrl Pts',(2.7494231860719,1.30000000000016,3.47498392105788));
#49153=CARTESIAN_POINT('Ctrl Pts',(2.92520978215932,-1.30000000000552,3.58926377761781));
#49154=CARTESIAN_POINT('Ctrl Pts',(2.87137430883562,-1.18514270861552,3.63941583633585));
#49155=CARTESIAN_POINT('Ctrl Pts',(2.82487387978676,-1.06847604194701,3.68357671893372));
#49156=CARTESIAN_POINT('Ctrl Pts',(2.73439400595118,-0.794772684000843,
3.77175637672006));
#49157=CARTESIAN_POINT('Ctrl Pts',(2.6977337833005,-0.636309800095191,3.81588237558861));
#49158=CARTESIAN_POINT('Ctrl Pts',(2.64234943531422,-0.319434907277156,
3.86507084612856));
#49159=CARTESIAN_POINT('Ctrl Pts',(2.62585700317256,-0.158333333333331,
3.87899578028677));
#49160=CARTESIAN_POINT('Ctrl Pts',(2.60883450413301,0.158333333333333,3.86579195045199));
#49161=CARTESIAN_POINT('Ctrl Pts',(2.60954505347175,0.319434907277164,3.83955505545891));
#49162=CARTESIAN_POINT('Ctrl Pts',(2.62772875062843,0.6363098000952,3.7616546613167));
#49163=CARTESIAN_POINT('Ctrl Pts',(2.64349737435505,0.794772684000833,3.70162336321975));
#49164=CARTESIAN_POINT('Ctrl Pts',(2.69697512145966,1.06847604194516,3.58487210094493));
#49165=CARTESIAN_POINT('Ctrl Pts',(2.72704288094852,1.18514270861188,3.52797730830442));
#49166=CARTESIAN_POINT('Ctrl Pts',(2.76402986475048,1.30000000000015,3.46472501840155));
#49167=CARTESIAN_POINT('Ctrl Pts',(2.94195211702088,-1.30000000000551,3.58135635188366));
#49168=CARTESIAN_POINT('Ctrl Pts',(2.89061465528179,-1.18514270861551,3.62917911126257));
#49169=CARTESIAN_POINT('Ctrl Pts',(2.84574056684063,-1.068476041947,3.67144661144475));
#49170=CARTESIAN_POINT('Ctrl Pts',(2.75700413082334,-0.794772684000838,
3.75625923237902));
#49171=CARTESIAN_POINT('Ctrl Pts',(2.71855109018231,-0.636309800095188,
3.79954530516389));
#49172=CARTESIAN_POINT('Ctrl Pts',(2.66175505497251,-0.319434907277155,
3.84729132613465));
#49173=CARTESIAN_POINT('Ctrl Pts',(2.64347546109041,-0.15833333333333,3.86113639964704));
#49174=CARTESIAN_POINT('Ctrl Pts',(2.62607723464659,0.158333333333332,3.84764227098316));
#49175=CARTESIAN_POINT('Ctrl Pts',(2.62816708666822,0.319434907277163,3.82122097164442));
#49176=CARTESIAN_POINT('Ctrl Pts',(2.64706259124335,0.636309800095198,3.74411868020596));
#49177=CARTESIAN_POINT('Ctrl Pts',(2.6641715349787,0.794772684000831,3.68441341960523));
#49178=CARTESIAN_POINT('Ctrl Pts',(2.71563003021196,1.06847604194515,3.57063049673968));
#49179=CARTESIAN_POINT('Ctrl Pts',(2.74404835952103,1.18514270861187,3.51553217123244));
#49180=CARTESIAN_POINT('Ctrl Pts',(2.77861054227786,1.30000000000015,3.45458793145365));
#49181=CARTESIAN_POINT('Ctrl Pts',(2.96275287236147,-1.30000000000551,3.56912187057325));
#49182=CARTESIAN_POINT('Ctrl Pts',(2.9152380089655,-1.18514270861551,3.61419539427489));
#49183=CARTESIAN_POINT('Ctrl Pts',(2.8729820087517,-1.068476041947,3.65428018094039));
#49184=CARTESIAN_POINT('Ctrl Pts',(2.78751122095751,-0.794772684000838,
3.73535907652415));
#49185=CARTESIAN_POINT('Ctrl Pts',(2.74712712559485,-0.636309800095189,
3.7779565913181));
#49186=CARTESIAN_POINT('Ctrl Pts',(2.68921555700873,-0.319434907277157,
3.82446702635131));
#49187=CARTESIAN_POINT('Ctrl Pts',(2.6692019677842,-0.15833333333333,3.83883345347065));
#49188=CARTESIAN_POINT('Ctrl Pts',(2.65111542605734,0.158333333333332,3.82474985461491));
#49189=CARTESIAN_POINT('Ctrl Pts',(2.65381112051842,0.319434907277161,3.79685030737055));
#49190=CARTESIAN_POINT('Ctrl Pts',(2.67331602736107,0.636309800095197,3.72053130998223));
#49191=CARTESIAN_POINT('Ctrl Pts',(2.69291357929012,0.794772684000833,3.66196882305464));
#49192=CARTESIAN_POINT('Ctrl Pts',(2.74171634204975,1.06847604194515,3.55239654305779));
#49193=CARTESIAN_POINT('Ctrl Pts',(2.76785669428666,1.18514270861187,3.49974892305915));
#49194=CARTESIAN_POINT('Ctrl Pts',(2.79901249108243,1.30000000000015,3.44188346301939));
#49195=CARTESIAN_POINT('Ctrl Pts',(2.99103081011791,-1.3000000000055,3.55633083166487));
#49196=CARTESIAN_POINT('Ctrl Pts',(2.94848803293486,-1.1851427086155,3.59827269681306));
#49197=CARTESIAN_POINT('Ctrl Pts',(2.90950880187268,-1.06847604194699,3.63570253211179));
#49198=CARTESIAN_POINT('Ctrl Pts',(2.82769148477546,-0.794772684000828,
3.71174924788332));
#49199=CARTESIAN_POINT('Ctrl Pts',(2.78383232077458,-0.636309800095179,
3.75230485190503));
#49200=CARTESIAN_POINT('Ctrl Pts',(2.72373721633015,-0.31943490727715,3.79643645488893));
#49201=CARTESIAN_POINT('Ctrl Pts',(2.70106719923632,-0.158333333333328,
3.81097609762809));
#49202=CARTESIAN_POINT('Ctrl Pts',(2.68248021019993,0.15833333333333,3.79647629815684));
#49203=CARTESIAN_POINT('Ctrl Pts',(2.68747839337143,0.319434907277157,3.76820790883034));
#49204=CARTESIAN_POINT('Ctrl Pts',(2.70784903438241,0.636309800095187,3.69297067913685));
#49205=CARTESIAN_POINT('Ctrl Pts',(2.72924338216426,0.79477268400082,3.63464523256112));
#49206=CARTESIAN_POINT('Ctrl Pts',(2.77415286444821,1.06847604194513,3.52970451359164));
#49207=CARTESIAN_POINT('Ctrl Pts',(2.7973159748855,1.18514270861185,3.47992887819828));
#49208=CARTESIAN_POINT('Ctrl Pts',(2.82420254493968,1.30000000000012,3.42580255621658));
#49209=CARTESIAN_POINT('Ctrl Pts',(3.02374000248281,-1.30000000000548,3.53970490348622));
#49210=CARTESIAN_POINT('Ctrl Pts',(2.98688227510008,-1.18514270861548,3.57754592275709));
#49211=CARTESIAN_POINT('Ctrl Pts',(2.95194015891161,-1.06847604194698,3.61185076016537));
#49212=CARTESIAN_POINT('Ctrl Pts',(2.87564232544601,-0.79477268400082,3.68293250972372));
#49213=CARTESIAN_POINT('Ctrl Pts',(2.83029179168419,-0.636309800095175,
3.72376888730158));
#49214=CARTESIAN_POINT('Ctrl Pts',(2.76875349594478,-0.31943490727715,3.76615824891994));
#49215=CARTESIAN_POINT('Ctrl Pts',(2.74231322500643,-0.158333333333327,
3.78020127492504));
#49216=CARTESIAN_POINT('Ctrl Pts',(2.72265100687055,0.158333333333329,3.76468932346359));
#49217=CARTESIAN_POINT('Ctrl Pts',(2.7297147732218,0.319434907277155,3.73533386827454));
#49218=CARTESIAN_POINT('Ctrl Pts',(2.7506205684183,0.636309800095184,3.6609413659136));
#49219=CARTESIAN_POINT('Ctrl Pts',(2.77445372491561,0.794772684000816,3.6031922735046));
#49220=CARTESIAN_POINT('Ctrl Pts',(2.81412306654961,1.06847604194513,3.50334462000068));
#49221=CARTESIAN_POINT('Ctrl Pts',(2.83333729156544,1.18514270861185,3.45669992867096));
#49222=CARTESIAN_POINT('Ctrl Pts',(2.8545943534977,1.30000000000012,3.40663089549319));
#49223=CARTESIAN_POINT('Ctrl Pts',(3.05811345181906,-1.30000000000546,3.52497819970161));
#49224=CARTESIAN_POINT('Ctrl Pts',(3.02784713000013,-1.18514270861546,3.55976796518647));
#49225=CARTESIAN_POINT('Ctrl Pts',(2.99739814779495,-1.06847604194695,3.59148490966405));
#49226=CARTESIAN_POINT('Ctrl Pts',(2.92663292557024,-0.7947726840008,3.65765856511712));
#49227=CARTESIAN_POINT('Ctrl Pts',(2.87762423700182,-0.636309800095158,
3.696400314332));
#49228=CARTESIAN_POINT('Ctrl Pts',(2.81437264477428,-0.31943490727714,3.73665586758347));
#49229=CARTESIAN_POINT('Ctrl Pts',(2.7854988204527,-0.158333333333323,3.75149817535916));
#49230=CARTESIAN_POINT('Ctrl Pts',(2.76506258419809,0.158333333333324,3.73523024002701));
#49231=CARTESIAN_POINT('Ctrl Pts',(2.77370832229935,0.319434907277146,3.70430476682064));
#49232=CARTESIAN_POINT('Ctrl Pts',(2.79490878610156,0.636309800095165,3.63053623764237));
#49233=CARTESIAN_POINT('Ctrl Pts',(2.82105731392976,0.794772684000791,3.57332185604792));
#49234=CARTESIAN_POINT('Ctrl Pts',(2.85545611566572,1.0684760419451,3.47850624606086));
#49235=CARTESIAN_POINT('Ctrl Pts',(2.87074934203554,1.18514270861182,3.4349825522203));
#49236=CARTESIAN_POINT('Ctrl Pts',(2.8864458281049,1.30000000000009,3.38897732883797));
#49237=CARTESIAN_POINT('Ctrl Pts',(3.09205625616862,-1.30000000000543,3.50984328348391));
#49238=CARTESIAN_POINT('Ctrl Pts',(3.06800478826141,-1.18514270861544,3.54116922813601));
#49239=CARTESIAN_POINT('Ctrl Pts',(3.04195194514736,-1.06847604194693,3.57018503742081));
#49240=CARTESIAN_POINT('Ctrl Pts',(2.97714108859957,-0.794772684000788,
3.63188048662145));
#49241=CARTESIAN_POINT('Ctrl Pts',(2.92620087283072,-0.636309800095147,
3.67036357934875));
#49242=CARTESIAN_POINT('Ctrl Pts',(2.86161204481792,-0.319434907277135,
3.70886469308564));
#49243=CARTESIAN_POINT('Ctrl Pts',(2.82907770173351,-0.15833333333332,3.72319103898903));
#49244=CARTESIAN_POINT('Ctrl Pts',(2.80811545785615,0.158333333333322,3.7063924783893));
#49245=CARTESIAN_POINT('Ctrl Pts',(2.81978347874688,0.31943490727714,3.67537519627519));
#49246=CARTESIAN_POINT('Ctrl Pts',(2.84147833975011,0.636309800095155,3.60243740100193));
#49247=CARTESIAN_POINT('Ctrl Pts',(2.86909110561065,0.794772684000779,3.54488893058255));
#49248=CARTESIAN_POINT('Ctrl Pts',(2.89748472667741,1.06847604194508,3.45437721046725));
#49249=CARTESIAN_POINT('Ctrl Pts',(2.90852267843929,1.1851427086118,3.41364721031541));
#49250=CARTESIAN_POINT('Ctrl Pts',(2.9183080354906,1.30000000000007,3.37136637985989));
#49251=CARTESIAN_POINT('Ctrl Pts',(3.11687629317787,-1.30000000000541,3.50004924215962));
#49252=CARTESIAN_POINT('Ctrl Pts',(3.09754542267603,-1.18514270861542,3.52930518627741));
#49253=CARTESIAN_POINT('Ctrl Pts',(3.0747546067079,-1.06847604194692,3.55658817309006));
#49254=CARTESIAN_POINT('Ctrl Pts',(3.01411009634812,-0.794772684000775,
3.61505940450598));
#49255=CARTESIAN_POINT('Ctrl Pts',(2.96079261695772,-0.636309800095137,
3.65220373194291));
#49256=CARTESIAN_POINT('Ctrl Pts',(2.89540151624588,-0.319434907277129,
3.68956165600955));
#49257=CARTESIAN_POINT('Ctrl Pts',(2.86150434657455,-0.158333333333317,
3.7048038980158));
#49258=CARTESIAN_POINT('Ctrl Pts',(2.84019968751387,0.158333333333319,3.68765515484666));
#49259=CARTESIAN_POINT('Ctrl Pts',(2.85289391107185,0.319434907277135,3.6554224140808));
#49260=CARTESIAN_POINT('Ctrl Pts',(2.87468177331336,0.636309800095144,3.58281140246088));
#49261=CARTESIAN_POINT('Ctrl Pts',(2.90400762976015,0.794772684000765,3.52574151485857));
#49262=CARTESIAN_POINT('Ctrl Pts',(2.92809977392654,1.06847604194507,3.43821719621443));
#49263=CARTESIAN_POINT('Ctrl Pts',(2.9359865228172,1.18514270861178,3.39931308160935));
#49264=CARTESIAN_POINT('Ctrl Pts',(2.94133142409081,1.30000000000005,3.35939088684461));
#49265=CARTESIAN_POINT('Ctrl Pts',(3.13158353443155,-1.30000000000541,3.49443635111853));
#49266=CARTESIAN_POINT('Ctrl Pts',(3.11498108231661,-1.18514270861541,3.52243016001803));
#49267=CARTESIAN_POINT('Ctrl Pts',(3.09414544753145,-1.06847604194691,3.54873997504398));
#49268=CARTESIAN_POINT('Ctrl Pts',(3.03623146421028,-0.794772684000773,
3.60563054828418));
#49269=CARTESIAN_POINT('Ctrl Pts',(2.98236769368786,-0.636309800095134,
3.64292466044221));
#49270=CARTESIAN_POINT('Ctrl Pts',(2.91631142052615,-0.319434907277128,
3.67938965362454));
#49271=CARTESIAN_POINT('Ctrl Pts',(2.88044270014575,-0.158333333333317,
3.69387287687065));
#49272=CARTESIAN_POINT('Ctrl Pts',(2.85865085934877,0.158333333333318,3.67618650762719));
#49273=CARTESIAN_POINT('Ctrl Pts',(2.87260183512496,0.319434907277134,3.64393871473653));
#49274=CARTESIAN_POINT('Ctrl Pts',(2.89452615463776,0.636309800095142,3.57160714945251));
#49275=CARTESIAN_POINT('Ctrl Pts',(2.92450780919669,0.794772684000762,3.51445504771415));
#49276=CARTESIAN_POINT('Ctrl Pts',(2.94602178220094,1.06847604194506,3.42863571906366));
#49277=CARTESIAN_POINT('Ctrl Pts',(2.95208385538883,1.18514270861177,3.39083350140881));
#49278=CARTESIAN_POINT('Ctrl Pts',(2.95489540002235,1.30000000000004,3.35237707355236));
#49279=CARTESIAN_POINT('Ctrl Pts',(3.13747310944787,-1.30000000000541,3.49219508269092));
#49280=CARTESIAN_POINT('Ctrl Pts',(3.12186406304511,-1.18514270861541,3.51956831209898));
#49281=CARTESIAN_POINT('Ctrl Pts',(3.10174684277267,-1.06847604194691,3.54541437692169));
#49282=CARTESIAN_POINT('Ctrl Pts',(3.04485725601163,-0.794772684000771,
3.60159590144885));
#49283=CARTESIAN_POINT('Ctrl Pts',(2.99082346793244,-0.636309800095134,
3.6390167161116));
#49284=CARTESIAN_POINT('Ctrl Pts',(2.9246017824391,-0.319434907277128,3.67523948609918));
#49285=CARTESIAN_POINT('Ctrl Pts',(2.88807824804091,-0.158333333333317,
3.68956399077605));
#49286=CARTESIAN_POINT('Ctrl Pts',(2.86619353667346,0.158333333333318,3.67177298542));
#49287=CARTESIAN_POINT('Ctrl Pts',(2.880683819517,0.319434907277135,3.63955575270664));
#49288=CARTESIAN_POINT('Ctrl Pts',(2.9026304893724,0.636309800095142,3.5673011875794));
#49289=CARTESIAN_POINT('Ctrl Pts',(2.93271554483,0.794772684000762,3.50994922438559));
#49290=CARTESIAN_POINT('Ctrl Pts',(2.95319450356583,1.06847604194506,3.42480511734035));
#49291=CARTESIAN_POINT('Ctrl Pts',(2.95855830491183,1.18514270861177,3.38747509513212));
#49292=CARTESIAN_POINT('Ctrl Pts',(2.9604213251873,1.30000000000004,3.34967077975544));
#49293=CARTESIAN_POINT('Ctrl Pts',(3.14724612156393,-1.3000000000054,3.48766330278961));
#49294=CARTESIAN_POINT('Ctrl Pts',(3.13348128227247,-1.18514270861541,3.5140676492899));
#49295=CARTESIAN_POINT('Ctrl Pts',(3.11468903259007,-1.06847604194691,3.53917782727463));
#49296=CARTESIAN_POINT('Ctrl Pts',(3.05966085271442,-0.794772684000766,
3.59419757352424));
#49297=CARTESIAN_POINT('Ctrl Pts',(3.00509682848601,-0.63630980009513,3.63158621209596));
#49298=CARTESIAN_POINT('Ctrl Pts',(2.93881145735945,-0.319434907277126,
3.66764063632057));
#49299=CARTESIAN_POINT('Ctrl Pts',(2.90163688889582,-0.158333333333316,
3.68223796966319));
#49300=CARTESIAN_POINT('Ctrl Pts',(2.87983121837161,0.158333333333317,3.66453734208435));
#49301=CARTESIAN_POINT('Ctrl Pts',(2.89521422951983,0.319434907277132,3.63232151937108));
#49302=CARTESIAN_POINT('Ctrl Pts',(2.9170542722588,0.636309800095138,3.56004488163989));
#49303=CARTESIAN_POINT('Ctrl Pts',(2.94702340432198,0.794772684000757,3.50201390974382));
#49304=CARTESIAN_POINT('Ctrl Pts',(2.96554943465532,1.06847604194505,3.41789800082923));
#49305=CARTESIAN_POINT('Ctrl Pts',(2.96967079764774,1.18514270861176,3.38137354255371));
#49306=CARTESIAN_POINT('Ctrl Pts',(2.96989429155835,1.30000000000003,3.34473528617021));
#49307=CARTESIAN_POINT('Ctrl Pts',(3.16813308791021,-1.3000000000054,3.4801976087041));
#49308=CARTESIAN_POINT('Ctrl Pts',(3.15861104087973,-1.1851427086154,3.50535118787714));
#49309=CARTESIAN_POINT('Ctrl Pts',(3.14277726544515,-1.0684760419469,3.52937024792866));
#49310=CARTESIAN_POINT('Ctrl Pts',(3.09161672138539,-0.794772684000766,
3.58223811551322));
#49311=CARTESIAN_POINT('Ctrl Pts',(3.03534693789403,-0.636309800095129,
3.6187218270644));
#49312=CARTESIAN_POINT('Ctrl Pts',(2.96803742254168,-0.319434907277126,
3.65337423047707));
#49313=CARTESIAN_POINT('Ctrl Pts',(2.92883858231923,-0.158333333333316,
3.66769464217141));
#49314=CARTESIAN_POINT('Ctrl Pts',(2.90622356807653,0.158333333333318,3.64909280244314));
#49315=CARTESIAN_POINT('Ctrl Pts',(2.92239523057836,0.319434907277134,3.61581692172046));
#49316=CARTESIAN_POINT('Ctrl Pts',(2.94447913758118,0.636309800095139,3.54399422758025));
#49317=CARTESIAN_POINT('Ctrl Pts',(2.97650667690471,0.794772684000756,3.48708945195852));
#49318=CARTESIAN_POINT('Ctrl Pts',(2.9915670013947,1.06847604194505,3.40551175333258));
#49319=CARTESIAN_POINT('Ctrl Pts',(2.99300105055347,1.18514270861176,3.37038148369381));
#49320=CARTESIAN_POINT('Ctrl Pts',(2.98935009243932,1.30000000000003,3.3354329073998));
#49321=CARTESIAN_POINT('Ctrl Pts',(3.19179194785933,-1.30000000000532,3.47145281285552));
#49322=CARTESIAN_POINT('Ctrl Pts',(3.18689867313708,-1.18514270861533,3.49493494775585));
#49323=CARTESIAN_POINT('Ctrl Pts',(3.17431550602839,-1.06847604194684,3.51756498343844));
#49324=CARTESIAN_POINT('Ctrl Pts',(3.12748068298343,-0.794772684000715,
3.56787637333307));
#49325=CARTESIAN_POINT('Ctrl Pts',(3.06924355582359,-0.636309800095087,
3.60331146965924));
#49326=CARTESIAN_POINT('Ctrl Pts',(3.00149505536153,-0.319434907277103,
3.63718459141884));
#49327=CARTESIAN_POINT('Ctrl Pts',(2.96098140760044,-0.158333333333305,
3.6523108758059));
#49328=CARTESIAN_POINT('Ctrl Pts',(2.93839872540465,0.158333333333307,3.63373857487706));
#49329=CARTESIAN_POINT('Ctrl Pts',(2.95623380536833,0.319434907277111,3.60007094708565));
#49330=CARTESIAN_POINT('Ctrl Pts',(2.97817832027118,0.636309800095095,3.52830432733564));
#49331=CARTESIAN_POINT('Ctrl Pts',(3.01075035598527,0.794772684000702,3.47071903367215));
#49332=CARTESIAN_POINT('Ctrl Pts',(3.02115660837694,1.06847604194498,3.39126100268221));
#49333=CARTESIAN_POINT('Ctrl Pts',(3.01945905835154,1.18514270861168,3.3576417212101));
#49334=CARTESIAN_POINT('Ctrl Pts',(3.01155947723004,1.29999999999994,3.32479759567122));
#49335=CARTESIAN_POINT('Ctrl Pts',(3.21522080882871,-1.30000000000528,3.46246711081863));
#49336=CARTESIAN_POINT('Ctrl Pts',(3.21478036472508,-1.1851427086153,3.48407010925375));
#49337=CARTESIAN_POINT('Ctrl Pts',(3.2054431767628,-1.06847604194681,3.50530808615156));
#49338=CARTESIAN_POINT('Ctrl Pts',(3.16331914657126,-0.794772684000694,
3.55352878865432));
#49339=CARTESIAN_POINT('Ctrl Pts',(3.10445481574066,-0.636309800095072,
3.58951896614683));
#49340=CARTESIAN_POINT('Ctrl Pts',(3.03622583171377,-0.319434907277096,
3.62257076628785));
#49341=CARTESIAN_POINT('Ctrl Pts',(2.99327478607966,-0.158333333333301,
3.63715677864556));
#49342=CARTESIAN_POINT('Ctrl Pts',(2.96991053877903,0.158333333333303,3.61766975016863));
#49343=CARTESIAN_POINT('Ctrl Pts',(2.98892675674291,0.319434907277103,3.58309285692305));
#49344=CARTESIAN_POINT('Ctrl Pts',(3.01072668242984,0.63630980009508,3.51137369396961));
#49345=CARTESIAN_POINT('Ctrl Pts',(3.04460510772446,0.794772684000685,3.45395272792116));
#49346=CARTESIAN_POINT('Ctrl Pts',(3.05068074461062,1.06847604194496,3.3769694383871));
#49347=CARTESIAN_POINT('Ctrl Pts',(3.04591541965882,1.18514270861165,3.34492984949011));
#49348=CARTESIAN_POINT('Ctrl Pts',(3.03375485167175,1.29999999999991,3.31417388522341));
#49349=CARTESIAN_POINT('Ctrl Pts',(3.23043539172048,-1.30000000000525,3.45755404152851));
#49350=CARTESIAN_POINT('Ctrl Pts',(3.2329405320919,-1.18514270861527,3.47820324486245));
#49351=CARTESIAN_POINT('Ctrl Pts',(3.22568713974405,-1.06847604194679,3.4986527219145));
#49352=CARTESIAN_POINT('Ctrl Pts',(3.18638618961544,-0.794772684000677,
3.54543369714194));
#49353=CARTESIAN_POINT('Ctrl Pts',(3.12652860387767,-0.636309800095058,
3.58102011372498));
#49354=CARTESIAN_POINT('Ctrl Pts',(3.05782286067161,-0.319434907277089,
3.6133293068439));
#49355=CARTESIAN_POINT('Ctrl Pts',(3.01347626991863,-0.158333333333298,
3.62773044976816));
#49356=CARTESIAN_POINT('Ctrl Pts',(2.98993339731732,0.158333333333299,3.60801834881184));
#49357=CARTESIAN_POINT('Ctrl Pts',(3.01013999760652,0.319434907277096,3.57338353464544));
#49358=CARTESIAN_POINT('Ctrl Pts',(3.03210689055872,0.636309800095065,3.50198461231473));
#49359=CARTESIAN_POINT('Ctrl Pts',(3.06682651501897,0.794772684000667,3.44469950089005));
#49360=CARTESIAN_POINT('Ctrl Pts',(3.06994197699543,1.06847604194493,3.3689708590629));
#49361=CARTESIAN_POINT('Ctrl Pts',(3.06306346665119,1.18514270861163,3.33769266444407));
#49362=CARTESIAN_POINT('Ctrl Pts',(3.04795787791233,1.29999999999988,3.30791639823066));
#49363=CARTESIAN_POINT('Ctrl Pts',(3.24236037790981,-1.30000000000524,3.45333727526057));
#49364=CARTESIAN_POINT('Ctrl Pts',(3.24716949580118,-1.18514270861526,3.47315376125293));
#49365=CARTESIAN_POINT('Ctrl Pts',(3.24157375609316,-1.06847604194678,3.49295791273523));
#49366=CARTESIAN_POINT('Ctrl Pts',(3.20460917540481,-0.79477268400067,3.53868096928009));
#49367=CARTESIAN_POINT('Ctrl Pts',(3.14425046756847,-0.636309800095053,
3.574312076442));
#49368=CARTESIAN_POINT('Ctrl Pts',(3.0751964674596,-0.319434907277087,3.60607199428668));
#49369=CARTESIAN_POINT('Ctrl Pts',(3.02951884639692,-0.158333333333296,
3.62006145448726));
#49370=CARTESIAN_POINT('Ctrl Pts',(3.00576205606805,0.158333333333298,3.60008675760718));
#49371=CARTESIAN_POINT('Ctrl Pts',(3.02695727830684,0.319434907277093,3.56545728113027));
#49372=CARTESIAN_POINT('Ctrl Pts',(3.04909841932032,0.63630980009506,3.49436555167233));
#49373=CARTESIAN_POINT('Ctrl Pts',(3.08455863757736,0.794772684000662,3.43726743726676));
#49374=CARTESIAN_POINT('Ctrl Pts',(3.08533390700979,1.06847604194492,3.36257119443522));
#49375=CARTESIAN_POINT('Ctrl Pts',(3.07676594735122,1.18514270861162,3.33190059891139));
#49376=CARTESIAN_POINT('Ctrl Pts',(3.05929444262332,1.29999999999987,3.30289264361694));
#49377=CARTESIAN_POINT('Ctrl Pts',(3.25151506053727,-1.30000000000523,3.45044442082133));
#49378=CARTESIAN_POINT('Ctrl Pts',(3.25818052889986,-1.18514270861526,3.46980749709816));
#49379=CARTESIAN_POINT('Ctrl Pts',(3.25388329241467,-1.06847604194677,3.48920286726995));
#49380=CARTESIAN_POINT('Ctrl Pts',(3.21862977519508,-0.794772684000666,
3.53408465775458));
#49381=CARTESIAN_POINT('Ctrl Pts',(3.15747235989514,-0.63630980009505,3.56920933418693));
#49382=CARTESIAN_POINT('Ctrl Pts',(3.08815646817621,-0.319434907277086,
3.60054108442575));
#49383=CARTESIAN_POINT('Ctrl Pts',(3.04189754295722,-0.158333333333296,
3.61472107209399));
#49384=CARTESIAN_POINT('Ctrl Pts',(3.01797372470983,0.158333333333297,3.5945431182307));
#49385=CARTESIAN_POINT('Ctrl Pts',(3.03961372085166,0.319434907277091,3.55956805127921));
#49386=CARTESIAN_POINT('Ctrl Pts',(3.06161440808337,0.636309800095057,3.48839230192767));
#49387=CARTESIAN_POINT('Ctrl Pts',(3.09736224761959,0.794772684000659,3.43113070515455));
#49388=CARTESIAN_POINT('Ctrl Pts',(3.09643186938066,1.06847604194492,3.35726335515356));
#49389=CARTESIAN_POINT('Ctrl Pts',(3.08670795795583,1.18514270861161,3.32717417292955));
#49390=CARTESIAN_POINT('Ctrl Pts',(3.06766286137189,1.29999999999986,3.29897024724187));
#49391=CARTESIAN_POINT('Ctrl Pts',(3.25839374116323,-1.30000000000522,3.44829774143665));
#49392=CARTESIAN_POINT('Ctrl Pts',(3.26650238174667,-1.18514270861524,3.4673851188094));
#49393=CARTESIAN_POINT('Ctrl Pts',(3.26321007457816,-1.06847604194676,3.48651319165782));
#49394=CARTESIAN_POINT('Ctrl Pts',(3.22926571633663,-0.794772684000659,
3.53079688118505));
#49395=CARTESIAN_POINT('Ctrl Pts',(3.16743555483022,-0.636309800095044,
3.56545105153254));
#49396=CARTESIAN_POINT('Ctrl Pts',(3.09792478855041,-0.319434907277083,
3.59645939042958));
#49397=CARTESIAN_POINT('Ctrl Pts',(3.05127922196103,-0.158333333333294,
3.61083604519458));
#49398=CARTESIAN_POINT('Ctrl Pts',(3.02724725143658,0.158333333333296,3.59052331406926));
#49399=CARTESIAN_POINT('Ctrl Pts',(3.04921905371466,0.319434907277089,3.55528782026933));
#49400=CARTESIAN_POINT('Ctrl Pts',(3.07108571412861,0.636309800095052,3.48401629312595));
#49401=CARTESIAN_POINT('Ctrl Pts',(3.10699976074015,0.794772684000652,3.42657662119549));
#49402=CARTESIAN_POINT('Ctrl Pts',(3.10475968117388,1.06847604194491,3.35329452560483));
#49403=CARTESIAN_POINT('Ctrl Pts',(3.09416135764752,1.1851427086116,3.32363162846848));
#49404=CARTESIAN_POINT('Ctrl Pts',(3.07393435803593,1.29999999999985,3.29602693800773));
#49405=CARTESIAN_POINT('Ctrl Pts',(3.2629351555692,-1.30000000000522,3.44681055730694));
#49406=CARTESIAN_POINT('Ctrl Pts',(3.27195063283112,-1.18514270861524,3.46564439602566));
#49407=CARTESIAN_POINT('Ctrl Pts',(3.26930490564037,-1.06847604194676,3.48456486026918));
#49408=CARTESIAN_POINT('Ctrl Pts',(3.23625303145248,-0.794772684000657,
3.52847503998891));
#49409=CARTESIAN_POINT('Ctrl Pts',(3.17415149607227,-0.636309800095043,
3.56303901281693));
#49410=CARTESIAN_POINT('Ctrl Pts',(3.10452955844486,-0.319434907277082,
3.59385694153619));
#49411=CARTESIAN_POINT('Ctrl Pts',(3.05748804064638,-0.158333333333294,
3.60819414683819));
#49412=CARTESIAN_POINT('Ctrl Pts',(3.03338240007983,0.158333333333296,3.58778759734221));
#49413=CARTESIAN_POINT('Ctrl Pts',(3.05566128091489,0.319434907277088,3.5524820616037));
#49414=CARTESIAN_POINT('Ctrl Pts',(3.07752001872709,0.636309800095051,3.48124176820776));
#49415=CARTESIAN_POINT('Ctrl Pts',(3.11364277148084,0.79477268400065,3.42379492402245));
#49416=CARTESIAN_POINT('Ctrl Pts',(3.11049337442213,1.06847604194491,3.35086141207141));
#49417=CARTESIAN_POINT('Ctrl Pts',(3.09926141795675,1.1851427086116,3.32142448566816));
#49418=CARTESIAN_POINT('Ctrl Pts',(3.07816076231604,1.29999999999985,3.2941208477323));
#49419=CARTESIAN_POINT('Ctrl Pts',(3.2651977655983,-1.30000000000522,3.4460570044894));
#49420=CARTESIAN_POINT('Ctrl Pts',(3.27465921485341,-1.18514270861524,3.46475464341014));
#49421=CARTESIAN_POINT('Ctrl Pts',(3.27233393696745,-1.06847604194676,3.48356770879022));
#49422=CARTESIAN_POINT('Ctrl Pts',(3.2397323822584,-0.794772684000657,3.52729631157071));
#49423=CARTESIAN_POINT('Ctrl Pts',(3.17752178562626,-0.636309800095043,
3.56184883363791));
#49424=CARTESIAN_POINT('Ctrl Pts',(3.1078476368185,-0.319434907277082,3.5925760349404));
#49425=CARTESIAN_POINT('Ctrl Pts',(3.06058772743218,-0.158333333333294,
3.60686829725747));
#49426=CARTESIAN_POINT('Ctrl Pts',(3.03644527364713,0.158333333333296,3.58641449742714));
#49427=CARTESIAN_POINT('Ctrl Pts',(3.05889036651009,0.319434907277088,3.5510891556183));
#49428=CARTESIAN_POINT('Ctrl Pts',(3.08075762975828,0.63630980009505,3.47987898774469));
#49429=CARTESIAN_POINT('Ctrl Pts',(3.11700012148815,0.794772684000649,3.42244613527154));
#49430=CARTESIAN_POINT('Ctrl Pts',(3.11339055039977,1.06847604194491,3.34968045295409));
#49431=CARTESIAN_POINT('Ctrl Pts',(3.10183395340449,1.1851427086116,3.32034744392509));
#49432=CARTESIAN_POINT('Ctrl Pts',(3.08028320899029,1.29999999999985,3.29317899350803));
#49433=CARTESIAN_POINT('Ctrl Pts',(3.2670773572165,-1.30000000000522,3.4454216913974));
#49434=CARTESIAN_POINT('Ctrl Pts',(3.27690346099998,-1.18514270861524,3.46399707135251));
#49435=CARTESIAN_POINT('Ctrl Pts',(3.27484235905761,-1.06847604194676,3.48271706772866));
#49436=CARTESIAN_POINT('Ctrl Pts',(3.24261897799492,-0.794772684000656,
3.52629809714264));
#49437=CARTESIAN_POINT('Ctrl Pts',(3.18034046996167,-0.636309800095042,
3.56086999118983));
#49438=CARTESIAN_POINT('Ctrl Pts',(3.11062587849898,-0.319434907277082,
3.59152561799046));
#49439=CARTESIAN_POINT('Ctrl Pts',(3.06316711554304,-0.158333333333294,
3.60575962620988));
#49440=CARTESIAN_POINT('Ctrl Pts',(3.03899373624695,0.158333333333295,3.58526587749418));
#49441=CARTESIAN_POINT('Ctrl Pts',(3.06158720505367,0.319434907277087,3.54993590984734));
#49442=CARTESIAN_POINT('Ctrl Pts',(3.08347174416763,0.63630980009505,3.47876265237086));
#49443=CARTESIAN_POINT('Ctrl Pts',(3.11982701814721,0.794772684000649,3.42135628234749));
#49444=CARTESIAN_POINT('Ctrl Pts',(3.11582977098446,1.06847604194491,3.34872551469281));
#49445=CARTESIAN_POINT('Ctrl Pts',(3.10399636889382,1.1851427086116,3.31947182962008));
#49446=CARTESIAN_POINT('Ctrl Pts',(3.08205982489668,1.29999999999985,3.29240362755716));
#49447=CARTESIAN_POINT('Ctrl Pts',(3.26839113242907,-1.30000000000522,3.4449746547755));
#49448=CARTESIAN_POINT('Ctrl Pts',(3.27847045351117,-1.18514270861524,3.46346192886595));
#49449=CARTESIAN_POINT('Ctrl Pts',(3.27659354100122,-1.06847604194676,3.48211588468545));
#49450=CARTESIAN_POINT('Ctrl Pts',(3.24463620619448,-0.794772684000656,
3.52559532247786));
#49451=CARTESIAN_POINT('Ctrl Pts',(3.18231740566533,-0.636309800095042,
3.56018988379013));
#49452=CARTESIAN_POINT('Ctrl Pts',(3.11257644655851,-0.319434907277082,
3.59079784181469));
#49453=CARTESIAN_POINT('Ctrl Pts',(3.06497484078213,-0.158333333333294,
3.60498650919207));
#49454=CARTESIAN_POINT('Ctrl Pts',(3.04077972177938,0.158333333333295,3.58446456585854));
#49455=CARTESIAN_POINT('Ctrl Pts',(3.06347824714969,0.319434907277088,3.54913277272834));
#49456=CARTESIAN_POINT('Ctrl Pts',(3.0853775573579,0.63630980009505,3.47798839762382));
#49457=CARTESIAN_POINT('Ctrl Pts',(3.12181659359161,0.794772684000649,3.42060613391417));
#49458=CARTESIAN_POINT('Ctrl Pts',(3.11754710088519,1.06847604194491,3.34806866304846));
#49459=CARTESIAN_POINT('Ctrl Pts',(3.10551816588902,1.1851427086116,3.31886837560809));
#49460=CARTESIAN_POINT('Ctrl Pts',(3.083308401089,1.29999999999985,3.29186658408691));
#49461=CARTESIAN_POINT('Ctrl Pts',(3.26914141517851,-1.30000000000522,3.44471866630091));
#49462=CARTESIAN_POINT('Ctrl Pts',(3.27936503375922,-1.18514270861524,3.46315510004237));
#49463=CARTESIAN_POINT('Ctrl Pts',(3.27759322408484,-1.06847604194676,3.48177113502083));
#49464=CARTESIAN_POINT('Ctrl Pts',(3.24578815034159,-0.794772684000656,
3.52519281473233));
#49465=CARTESIAN_POINT('Ctrl Pts',(3.18344794709283,-0.636309800095042,
3.55980233955652));
#49466=CARTESIAN_POINT('Ctrl Pts',(3.11369178556253,-0.319434907277082,
3.59038290776075));
#49467=CARTESIAN_POINT('Ctrl Pts',(3.06600657894605,-0.158333333333294,
3.60454325978532));
#49468=CARTESIAN_POINT('Ctrl Pts',(3.04179920469789,0.158333333333295,3.58400538652966));
#49469=CARTESIAN_POINT('Ctrl Pts',(3.0645596308527,0.319434907277087,3.54867479637399));
#49470=CARTESIAN_POINT('Ctrl Pts',(3.08646841883026,0.636309800095049,3.47754814084337));
#49471=CARTESIAN_POINT('Ctrl Pts',(3.12295571757344,0.794772684000649,3.42018005651234));
#49472=CARTESIAN_POINT('Ctrl Pts',(3.1185300450144,1.06847604194491,3.34769519918457));
#49473=CARTESIAN_POINT('Ctrl Pts',(3.10638879801904,1.1851427086116,3.3185247695525));
#49474=CARTESIAN_POINT('Ctrl Pts',(3.08402201369178,1.29999999999985,3.29155991919689));
#49475=CARTESIAN_POINT('Ctrl Pts',(3.2815192757435,-1.30000000000524,3.44049349245556));
#49476=CARTESIAN_POINT('Ctrl Pts',(3.29411750209666,-1.18514270861526,3.45808378517407));
#49477=CARTESIAN_POINT('Ctrl Pts',(3.29407811160572,-1.06847604194678,3.47607236336675));
#49478=CARTESIAN_POINT('Ctrl Pts',(3.26479168863541,-0.794772684000672,
3.51854969671626));
#49479=CARTESIAN_POINT('Ctrl Pts',(3.20211463122718,-0.636309800095055,
3.55342708072927));
#49480=CARTESIAN_POINT('Ctrl Pts',(3.13213552189026,-0.319434907277088,
3.58358960599319));
#49481=CARTESIAN_POINT('Ctrl Pts',(3.08310955670434,-0.158333333333297,
3.59732839724589));
#49482=CARTESIAN_POINT('Ctrl Pts',(3.05869326203224,0.158333333333299,3.57651899659488));
#49483=CARTESIAN_POINT('Ctrl Pts',(3.08241532664736,0.319434907277094,3.54113626936939));
#49484=CARTESIAN_POINT('Ctrl Pts',(3.10446819107465,0.636309800095062,3.47028638166786));
#49485=CARTESIAN_POINT('Ctrl Pts',(3.14178581750134,0.794772684000664,3.4131936241766));
#49486=CARTESIAN_POINT('Ctrl Pts',(3.13479782110837,1.06847604194493,3.34159159469494));
#49487=CARTESIAN_POINT('Ctrl Pts',(3.12080760531913,1.18514270861162,3.31291693254506));
#49488=CARTESIAN_POINT('Ctrl Pts',(3.09585201844837,1.29999999999987,3.28656147369124));
#49489=CARTESIAN_POINT('Ctrl Pts',(3.30633337300009,-1.30000000000539,3.43306487095043));
#49490=CARTESIAN_POINT('Ctrl Pts',(3.32406547015772,-1.1851427086154,3.44965584374711));
#49491=CARTESIAN_POINT('Ctrl Pts',(3.32765731547434,-1.0684760419469,3.46674748844742));
#49492=CARTESIAN_POINT('Ctrl Pts',(3.30328838620176,-0.794772684000765,
3.50738925913304));
#49493=CARTESIAN_POINT('Ctrl Pts',(3.23879682294951,-0.636309800095127,
3.54130171876271));
#49494=CARTESIAN_POINT('Ctrl Pts',(3.16813786468817,-0.319434907277124,
3.57030559004538));
#49495=CARTESIAN_POINT('Ctrl Pts',(3.11710951207744,-0.158333333333315,
3.58395650927749));
#49496=CARTESIAN_POINT('Ctrl Pts',(3.09226299934626,0.158333333333317,3.56258450769254));
#49497=CARTESIAN_POINT('Ctrl Pts',(3.11774095891631,0.319434907277132,3.52696166627474));
#49498=CARTESIAN_POINT('Ctrl Pts',(3.13922311326188,0.636309800095137,3.45564656166672));
#49499=CARTESIAN_POINT('Ctrl Pts',(3.17628812002097,0.794772684000752,3.3969085309373));
#49500=CARTESIAN_POINT('Ctrl Pts',(3.16473749775489,1.06847604194505,3.32749488900432));
#49501=CARTESIAN_POINT('Ctrl Pts',(3.14787282716488,1.18514270861176,3.3006149624431));
#49502=CARTESIAN_POINT('Ctrl Pts',(3.1191433223711,1.30000000000003,3.27690170288451));
#49503=CARTESIAN_POINT('Ctrl Pts',(3.33062939107151,-1.30000000000554,3.42534919669555));
#49504=CARTESIAN_POINT('Ctrl Pts',(3.35332856352848,-1.18514270861553,3.44081299553099));
#49505=CARTESIAN_POINT('Ctrl Pts',(3.36047748554674,-1.06847604194702,3.45697322363563));
#49506=CARTESIAN_POINT('Ctrl Pts',(3.34106873621573,-0.794772684000851,
3.49591547433162));
#49507=CARTESIAN_POINT('Ctrl Pts',(3.27513477130193,-0.636309800095197,
3.52930916811412));
#49508=CARTESIAN_POINT('Ctrl Pts',(3.20409726056275,-0.319434907277159,
3.55752565372287));
#49509=CARTESIAN_POINT('Ctrl Pts',(3.15126301207831,-0.158333333333332,
3.57130224199688));
#49510=CARTESIAN_POINT('Ctrl Pts',(3.12601838770936,0.158333333333334,3.54939933546828));
#49511=CARTESIAN_POINT('Ctrl Pts',(3.15259691103518,0.319434907277167,3.51276440601536));
#49512=CARTESIAN_POINT('Ctrl Pts',(3.17427247911497,0.636309800095206,3.44187942845857));
#49513=CARTESIAN_POINT('Ctrl Pts',(3.2137035449833,0.79477268400084,3.38458268055424));
#49514=CARTESIAN_POINT('Ctrl Pts',(3.19697910110487,1.06847604194517,3.31662261217747));
#49515=CARTESIAN_POINT('Ctrl Pts',(3.17625676661729,1.18514270861189,3.2903696517621));
#49516=CARTESIAN_POINT('Ctrl Pts',(3.14205148969539,1.30000000000017,3.26728112636297));
#49517=CARTESIAN_POINT('Ctrl Pts',(3.34312043552546,-1.30000000000554,3.42192826582793));
#49518=CARTESIAN_POINT('Ctrl Pts',(3.36817625250915,-1.18514270861553,3.43668158762693));
#49519=CARTESIAN_POINT('Ctrl Pts',(3.37703616937261,-1.06847604194702,3.45230111691552));
#49520=CARTESIAN_POINT('Ctrl Pts',(3.36008858049118,-0.794772684000851,
3.49038646683314));
#49521=CARTESIAN_POINT('Ctrl Pts',(3.29374448453208,-0.636309800095197,
3.523919285052));
#49522=CARTESIAN_POINT('Ctrl Pts',(3.22246485929501,-0.319434907277159,
3.55167070473743));
#49523=CARTESIAN_POINT('Ctrl Pts',(3.16838675811195,-0.158333333333332,
3.56506164372659));
#49524=CARTESIAN_POINT('Ctrl Pts',(3.14286241424647,0.158333333333334,3.5427812026076));
#49525=CARTESIAN_POINT('Ctrl Pts',(3.17031238807969,0.319434907277167,3.50603727501036));
#49526=CARTESIAN_POINT('Ctrl Pts',(3.19184909015917,0.636309800095206,3.43508690301979));
#49527=CARTESIAN_POINT('Ctrl Pts',(3.23156943363573,0.79477268400084,3.3774589430542));
#49528=CARTESIAN_POINT('Ctrl Pts',(3.21244012754109,1.06847604194517,3.31040827863485));
#49529=CARTESIAN_POINT('Ctrl Pts',(3.19010469464422,1.18514270861189,3.28482004316132));
#49530=CARTESIAN_POINT('Ctrl Pts',(3.15371419664818,1.30000000000017,3.26266732036942));
#49531=CARTESIAN_POINT('',(3.07985616677633,1.2,3.32482439211205));
#49532=CARTESIAN_POINT('Ctrl Pts',(3.07985616677633,1.2,3.32482439211205));
#49533=CARTESIAN_POINT('Ctrl Pts',(3.05014647401839,1.22374741355226,3.33154618210707));
#49534=CARTESIAN_POINT('Ctrl Pts',(3.02045877557164,1.24661638075374,3.3373574996142));
#49535=CARTESIAN_POINT('Ctrl Pts',(3.00582299008617,1.2582899439244,3.34073830904269));
#49536=CARTESIAN_POINT('Ctrl Pts',(2.99588832002411,1.26618999194865,3.34301915383334));
#49537=CARTESIAN_POINT('Ctrl Pts',(2.97463599570754,1.28302939977084,3.34785885555862));
#49538=CARTESIAN_POINT('Ctrl Pts',(2.96409046681166,1.29150679485646,3.35043257954748));
#49539=CARTESIAN_POINT('Ctrl Pts',(2.95357407118872,1.30000000000004,3.3530661292399));
#49540=CARTESIAN_POINT('',(3.20083482135393,0.653834841418549,3.42413500689526));
#49541=CARTESIAN_POINT('Ctrl Pts',(3.20083482136852,0.653834841417875,3.42413500687395));
#49542=CARTESIAN_POINT('Ctrl Pts',(3.18838633393975,0.718152197254491,3.41358231176756));
#49543=CARTESIAN_POINT('Ctrl Pts',(3.17833113418676,0.763624982037616,3.40513577897662));
#49544=CARTESIAN_POINT('Ctrl Pts',(3.13840443789891,0.949782885938845,3.37192609991964));
#49545=CARTESIAN_POINT('Ctrl Pts',(3.11710083982675,1.04698696039931,3.35442517607146));
#49546=CARTESIAN_POINT('Ctrl Pts',(3.07985616677634,1.2,3.32482439211205));
#49547=CARTESIAN_POINT('',(3.3059688760626,-0.653834841531101,3.5158352655581));
#49548=CARTESIAN_POINT('Ctrl Pts',(3.3059688760626,-0.6538348415311,3.5158352655581));
#49549=CARTESIAN_POINT('Ctrl Pts',(3.26766469767615,-0.575797940622744,
3.53224408913098));
#49550=CARTESIAN_POINT('Ctrl Pts',(3.23528548386165,-0.49392132436527,3.54536167683063));
#49551=CARTESIAN_POINT('Ctrl Pts',(3.18740430810065,-0.338200813941495,
3.56201786612114));
#49552=CARTESIAN_POINT('Ctrl Pts',(3.17011432354766,-0.265716187090828,
3.566700550714));
#49553=CARTESIAN_POINT('Ctrl Pts',(3.14580106413494,-0.129745742366583,
3.56885504483666));
#49554=CARTESIAN_POINT('Ctrl Pts',(3.1376655006151,-0.066643296824382,3.56729763532479));
#49555=CARTESIAN_POINT('Ctrl Pts',(3.12737068196028,0.059553431415733,3.55881191132792));
#49556=CARTESIAN_POINT('Ctrl Pts',(3.12512315151907,0.12280156340828,3.55183285058316));
#49557=CARTESIAN_POINT('Ctrl Pts',(3.12735984298063,0.260160697362436,3.53121091709078));
#49558=CARTESIAN_POINT('Ctrl Pts',(3.13314355351978,0.333962939326844,3.51658347201579));
#49559=CARTESIAN_POINT('Ctrl Pts',(3.15628677742229,0.491153916066733,3.47819158431581));
#49560=CARTESIAN_POINT('Ctrl Pts',(3.1753971249946,0.574259753110387,3.45309552551028));
#49561=CARTESIAN_POINT('Ctrl Pts',(3.20083482131431,0.65383484143008,3.42413500689214));
#49562=CARTESIAN_POINT('',(3.25193073118135,-1.2,3.46805057381556));
#49563=CARTESIAN_POINT('Ctrl Pts',(3.25193073118135,-1.2,3.46805057381556));
#49564=CARTESIAN_POINT('Ctrl Pts',(3.2611441147676,-1.13542851615971,3.47607889408488));
#49565=CARTESIAN_POINT('Ctrl Pts',(3.27351847074519,-1.03917466802095,3.4869248101128));
#49566=CARTESIAN_POINT('Ctrl Pts',(3.29732029958888,-0.795561890270455,
3.50806949716737));
#49567=CARTESIAN_POINT('Ctrl Pts',(3.30108969495973,-0.741496651508692,
3.51145695404667));
#49568=CARTESIAN_POINT('Ctrl Pts',(3.3059688760626,-0.653834841531101,3.5158352655581));
#49569=CARTESIAN_POINT('Ctrl Pts',(3.12987662697833,-1.30000000000541,3.49508808473909));
#49570=CARTESIAN_POINT('Ctrl Pts',(3.13109823331778,-1.29899972592073,3.49481065515237));
#49571=CARTESIAN_POINT('Ctrl Pts',(3.13232167623714,-1.29800069349213,3.49453663626624));
#49572=CARTESIAN_POINT('Ctrl Pts',(3.15283006555946,-1.28106822770405,3.48970374150241));
#49573=CARTESIAN_POINT('Ctrl Pts',(3.17216112258937,-1.26515575976258,3.48526789140061));
#49574=CARTESIAN_POINT('Ctrl Pts',(3.2036719906995,-1.23909634935026,3.47796888024456));
#49575=CARTESIAN_POINT('Ctrl Pts',(3.22760791802916,-1.21917023077842,3.47228335861269));
#49576=CARTESIAN_POINT('Ctrl Pts',(3.25193073118135,-1.2,3.46805057381556));
#49577=CARTESIAN_POINT('Origin',(0.,1.25,7.2));
#49578=CARTESIAN_POINT('Origin',(0.,1.2,7.2));
#49579=CARTESIAN_POINT('Origin',(0.,0.92691742076555,7.2));
#49580=CARTESIAN_POINT('Origin',(0.,0.653834841531101,7.2));
#49581=CARTESIAN_POINT('Origin',(0.,0.,7.2));
#49582=CARTESIAN_POINT('Origin',(0.,-0.653834841531101,7.2));
#49583=CARTESIAN_POINT('Origin',(0.,-0.926917420765551,7.2));
#49584=CARTESIAN_POINT('Origin',(0.,-1.2,7.2));
#49585=CARTESIAN_POINT('Origin',(0.,-1.25,7.2));
#49586=CARTESIAN_POINT('Ctrl Pts',(3.58611066068443,-1.30000000000134,3.65199884532217));
#49587=CARTESIAN_POINT('Ctrl Pts',(3.56027544999399,-1.18514270861269,3.61812328835111));
#49588=CARTESIAN_POINT('Ctrl Pts',(3.53249270107514,-1.06847604194558,3.59858491022381));
#49589=CARTESIAN_POINT('Ctrl Pts',(3.46380979024152,-0.794772684000851,
3.58656909938251));
#49590=CARTESIAN_POINT('Ctrl Pts',(3.41064942873151,-0.636309800095197,
3.63209561276063));
#49591=CARTESIAN_POINT('Ctrl Pts',(3.34233892867367,-0.319434907277159,
3.66093066788605));
#49592=CARTESIAN_POINT('Ctrl Pts',(3.30866559173879,-0.158333333333332,
3.69207105417578));
#49593=CARTESIAN_POINT('Ctrl Pts',(3.2838391847674,0.158333333333334,3.66901547560771));
#49594=CARTESIAN_POINT('Ctrl Pts',(3.29150406597897,0.319434907277167,3.61383388564663));
#49595=CARTESIAN_POINT('Ctrl Pts',(3.31165271079405,0.636309800095206,3.54004392440282));
#49596=CARTESIAN_POINT('Ctrl Pts',(3.33806698632524,0.79477268400084,3.47055813438899));
#49597=CARTESIAN_POINT('Ctrl Pts',(3.37417869140185,1.06852528713347,3.4497186342675));
#49598=CARTESIAN_POINT('Ctrl Pts',(3.39064595623598,1.18523969452324,3.456907049513));
#49599=CARTESIAN_POINT('Ctrl Pts',(3.407945382661,1.30014322216931,3.48030665351317));
#49600=CARTESIAN_POINT('Ctrl Pts',(3.58274121447463,-1.30000000000134,3.66407993676206));
#49601=CARTESIAN_POINT('Ctrl Pts',(3.55620374542005,-1.18514270861269,3.6324754479871));
#49602=CARTESIAN_POINT('Ctrl Pts',(3.52792852769947,-1.06847604194558,3.61461081421486));
#49603=CARTESIAN_POINT('Ctrl Pts',(3.45859257127325,-0.794772684000851,
3.60508175009811));
#49604=CARTESIAN_POINT('Ctrl Pts',(3.40573136963311,-0.636309800095197,
3.65028594950435));
#49605=CARTESIAN_POINT('Ctrl Pts',(3.33750042120983,-0.319434907277159,
3.67925227433872));
#49606=CARTESIAN_POINT('Ctrl Pts',(3.30384439394135,-0.158333333333332,
3.70951459060301));
#49607=CARTESIAN_POINT('Ctrl Pts',(3.2794226920353,0.158333333333334,3.6866977360883));
#49608=CARTESIAN_POINT('Ctrl Pts',(3.28760112792004,0.319434907277167,3.63271287353839));
#49609=CARTESIAN_POINT('Ctrl Pts',(3.30823759882109,0.636309800095206,3.55911508785096));
#49610=CARTESIAN_POINT('Ctrl Pts',(3.33455638238822,0.794772684000839,3.49005172463855));
#49611=CARTESIAN_POINT('Ctrl Pts',(3.37126313977548,1.06852528713347,3.46667451953378));
#49612=CARTESIAN_POINT('Ctrl Pts',(3.38808948508963,1.18523969452324,3.47210378935024));
#49613=CARTESIAN_POINT('Ctrl Pts',(3.40584943566987,1.30014322216931,3.49308383984994));
#49614=CARTESIAN_POINT('Ctrl Pts',(3.57557006138374,-1.30000000000134,3.68788375928115));
#49615=CARTESIAN_POINT('Ctrl Pts',(3.54871468730387,-1.18514270861269,3.66160123862957));
#49616=CARTESIAN_POINT('Ctrl Pts',(3.52006039654804,-1.06847604194558,3.64752641016531));
#49617=CARTESIAN_POINT('Ctrl Pts',(3.44970739523745,-0.794772684000851,
3.64321295184625));
#49618=CARTESIAN_POINT('Ctrl Pts',(3.39554233222154,-0.636309800095199,
3.68647457548047));
#49619=CARTESIAN_POINT('Ctrl Pts',(3.32698774364401,-0.319434907277161,
3.71537815626217));
#49620=CARTESIAN_POINT('Ctrl Pts',(3.29412717751249,-0.158333333333332,
3.74437727537379));
#49621=CARTESIAN_POINT('Ctrl Pts',(3.27036429293828,0.158333333333334,3.7219560698061));
#49622=CARTESIAN_POINT('Ctrl Pts',(3.27878216535924,0.319434907277165,3.66988801420742));
#49623=CARTESIAN_POINT('Ctrl Pts',(3.30031819130643,0.636309800095206,3.59663343330932));
#49624=CARTESIAN_POINT('Ctrl Pts',(3.32721809087927,0.794772684000843,3.52889942146027));
#49625=CARTESIAN_POINT('Ctrl Pts',(3.36511136767073,1.06852528713347,3.50042325914989));
#49626=CARTESIAN_POINT('Ctrl Pts',(3.38251100926453,1.18523969452324,3.50222876615767));
#49627=CARTESIAN_POINT('Ctrl Pts',(3.40090383106788,1.30014322216931,3.51816896088486));
#49628=CARTESIAN_POINT('Ctrl Pts',(3.56833827722676,-1.30000000000135,3.71222778574955));
#49629=CARTESIAN_POINT('Ctrl Pts',(3.53951368675864,-1.1851427086127,3.69020412855297));
#49630=CARTESIAN_POINT('Ctrl Pts',(3.50953174671455,-1.06847604194559,3.67931834756835));
#49631=CARTESIAN_POINT('Ctrl Pts',(3.43759375829876,-0.79477268400086,3.67990073797496));
#49632=CARTESIAN_POINT('Ctrl Pts',(3.38473957204787,-0.636309800095202,
3.72298966139289));
#49633=CARTESIAN_POINT('Ctrl Pts',(3.31656863253884,-0.31943490727716,3.75231856887475));
#49634=CARTESIAN_POINT('Ctrl Pts',(3.28381112398346,-0.158333333333333,
3.77956240396853));
#49635=CARTESIAN_POINT('Ctrl Pts',(3.26055576646907,0.158333333333335,3.75744897779247));
#49636=CARTESIAN_POINT('Ctrl Pts',(3.26911907660334,0.319434907277167,3.70728528593329));
#49637=CARTESIAN_POINT('Ctrl Pts',(3.2918328786251,0.636309800095209,3.63455556259583));
#49638=CARTESIAN_POINT('Ctrl Pts',(3.32000435343564,0.794772684000844,3.56860834600287));
#49639=CARTESIAN_POINT('Ctrl Pts',(3.35920572172797,1.06852528713348,3.53499777280326));
#49640=CARTESIAN_POINT('Ctrl Pts',(3.37709638055073,1.18523969452325,3.53304948152668));
#49641=CARTESIAN_POINT('Ctrl Pts',(3.39590487901678,1.30014322216932,3.54370509973294));
#49642=CARTESIAN_POINT('Ctrl Pts',(3.56451873103144,-1.30000000000135,3.72490745184346));
#49643=CARTESIAN_POINT('Ctrl Pts',(3.53537269284097,-1.1851427086127,3.70561850550658));
#49644=CARTESIAN_POINT('Ctrl Pts',(3.50509427141749,-1.06847604194559,3.6966891013083));
#49645=CARTESIAN_POINT('Ctrl Pts',(3.43252902895124,-0.794772684000859,
3.69999300604859));
#49646=CARTESIAN_POINT('Ctrl Pts',(3.37924708572632,-0.636309800095202,
3.74222270265255));
#49647=CARTESIAN_POINT('Ctrl Pts',(3.3107713763284,-0.319434907277161,3.77142952113616));
#49648=CARTESIAN_POINT('Ctrl Pts',(3.2780046005121,-0.158333333333333,3.79770928059227));
#49649=CARTESIAN_POINT('Ctrl Pts',(3.25504948205071,0.158333333333335,3.77578028795297));
#49650=CARTESIAN_POINT('Ctrl Pts',(3.26416085675191,0.319434907277167,3.72692636513837));
#49651=CARTESIAN_POINT('Ctrl Pts',(3.28730506801098,0.636309800095209,3.65436593388957));
#49652=CARTESIAN_POINT('Ctrl Pts',(3.31522477600129,0.794772684000845,3.58878455992508));
#49653=CARTESIAN_POINT('Ctrl Pts',(3.35512040885107,1.06852528713348,3.55248950013008));
#49654=CARTESIAN_POINT('Ctrl Pts',(3.37347102058355,1.18523969452325,3.54869942253555));
#49655=CARTESIAN_POINT('Ctrl Pts',(3.39289883263694,1.30014322216932,3.55683375675957));
#49656=CARTESIAN_POINT('Ctrl Pts',(3.56405407843926,-1.30000000000135,3.72638825584007));
#49657=CARTESIAN_POINT('Ctrl Pts',(3.53486512075411,-1.1851427086127,3.70741783545932));
#49658=CARTESIAN_POINT('Ctrl Pts',(3.50454957210363,-1.06847604194559,3.69871726394456));
#49659=CARTESIAN_POINT('Ctrl Pts',(3.43191193961276,-0.79477268400086,3.70234260855873));
#49660=CARTESIAN_POINT('Ctrl Pts',(3.37859610411269,-0.636309800095202,
3.74448229810159));
#49661=CARTESIAN_POINT('Ctrl Pts',(3.3100842727485,-0.319434907277161,3.77367477472895));
#49662=CARTESIAN_POINT('Ctrl Pts',(3.27730053746247,-0.158333333333333,
3.79983058246958));
#49663=CARTESIAN_POINT('Ctrl Pts',(3.25437940413007,0.158333333333335,3.77792249528188));
#49664=CARTESIAN_POINT('Ctrl Pts',(3.26356406444697,0.319434907277167,3.72922864376837));
#49665=CARTESIAN_POINT('Ctrl Pts',(3.28676811589004,0.636309800095209,3.65669414717994));
#49666=CARTESIAN_POINT('Ctrl Pts',(3.31466720209241,0.794772684000845,3.5911614685024));
#49667=CARTESIAN_POINT('Ctrl Pts',(3.35464687355412,1.06852528713348,3.55455203426073));
#49668=CARTESIAN_POINT('Ctrl Pts',(3.37305048040543,1.18523969452325,3.5505445273049));
#49669=CARTESIAN_POINT('Ctrl Pts',(3.39254789692153,1.30014322216932,3.55838011592867));
#49670=CARTESIAN_POINT('Ctrl Pts',(3.56323412079071,-1.30000000000135,3.72897518027144));
#49671=CARTESIAN_POINT('Ctrl Pts',(3.53395858234347,-1.1851427086127,3.71055407799477));
#49672=CARTESIAN_POINT('Ctrl Pts',(3.50357082351767,-1.06847604194559,3.70224886594239));
#49673=CARTESIAN_POINT('Ctrl Pts',(3.43079957000651,-0.794772684000859,
3.70643189474446));
#49674=CARTESIAN_POINT('Ctrl Pts',(3.37743097835824,-0.636309800095202,
3.74841896020542));
#49675=CARTESIAN_POINT('Ctrl Pts',(3.30887043014344,-0.319434907277161,
3.77759635709755));
#49676=CARTESIAN_POINT('Ctrl Pts',(3.27608132292629,-0.158333333333333,
3.80355163191065));
#49677=CARTESIAN_POINT('Ctrl Pts',(3.25322209667042,0.158333333333335,3.78168201958454));
#49678=CARTESIAN_POINT('Ctrl Pts',(3.26250887851396,0.319434907277167,3.73325114933835));
#49679=CARTESIAN_POINT('Ctrl Pts',(3.28581677536265,0.636309800095209,3.66076127075894));
#49680=CARTESIAN_POINT('Ctrl Pts',(3.31370301444247,0.794772684000845,3.59532856098206));
#49681=CARTESIAN_POINT('Ctrl Pts',(3.35383280469244,1.06852528713348,3.55817086313435));
#49682=CARTESIAN_POINT('Ctrl Pts',(3.37232671642551,1.18523969452325,3.55378129974125));
#49683=CARTESIAN_POINT('Ctrl Pts',(3.39193974652874,1.30014322216932,3.56109015442525));
#49684=CARTESIAN_POINT('Ctrl Pts',(3.56156582974602,-1.30000000000135,3.73412995924475));
#49685=CARTESIAN_POINT('Ctrl Pts',(3.53209133194118,-1.1851427086127,3.71678998648117));
#49686=CARTESIAN_POINT('Ctrl Pts',(3.50154526127351,-1.06847604194559,3.70926618595618));
#49687=CARTESIAN_POINT('Ctrl Pts',(3.42850217963027,-0.794772684000859,
3.71456202320195));
#49688=CARTESIAN_POINT('Ctrl Pts',(3.37507654568519,-0.636309800095203,
3.75627781946126));
#49689=CARTESIAN_POINT('Ctrl Pts',(3.30643358005453,-0.319434907277161,
3.78543555203506));
#49690=CARTESIAN_POINT('Ctrl Pts',(3.2736276039743,-0.158333333333333,3.81098472065163));
#49691=CARTESIAN_POINT('Ctrl Pts',(3.25087704757571,0.158333333333335,3.7891821210627));
#49692=CARTESIAN_POINT('Ctrl Pts',(3.26032456276067,0.319434907277167,3.74124947997401));
#49693=CARTESIAN_POINT('Ctrl Pts',(3.28386454079099,0.636309800095209,3.66886461811563));
#49694=CARTESIAN_POINT('Ctrl Pts',(3.31182178754529,0.794772684000846,3.60369418477127));
#49695=CARTESIAN_POINT('Ctrl Pts',(3.35226734248451,1.06852528713348,3.5654497474108));
#49696=CARTESIAN_POINT('Ctrl Pts',(3.37093080265433,1.18523969452325,3.56028878987513));
#49697=CARTESIAN_POINT('Ctrl Pts',(3.39074621458239,1.30014322216932,3.56652537641267));
#49698=CARTESIAN_POINT('Ctrl Pts',(3.55795146928502,-1.30000000000135,3.74425510241154));
#49699=CARTESIAN_POINT('Ctrl Pts',(3.5276397670157,-1.1851427086127,3.72876901708838));
#49700=CARTESIAN_POINT('Ctrl Pts',(3.4965130841671,-1.06847604194559,3.72262266645001));
#49701=CARTESIAN_POINT('Ctrl Pts',(3.422721451741,-0.79477268400086,3.73000002243147));
#49702=CARTESIAN_POINT('Ctrl Pts',(3.36961874311334,-0.636309800095203,
3.77148182779834));
#49703=CARTESIAN_POINT('Ctrl Pts',(3.30126931674964,-0.319434907277161,
3.80091734639357));
#49704=CARTESIAN_POINT('Ctrl Pts',(3.26898601617818,-0.158333333333333,
3.82603122146535));
#49705=CARTESIAN_POINT('Ctrl Pts',(3.2465114457038,0.158333333333335,3.80441018268777));
#49706=CARTESIAN_POINT('Ctrl Pts',(3.25558832361884,0.319434907277168,3.75702201836801));
#49707=CARTESIAN_POINT('Ctrl Pts',(3.27964939834871,0.636309800095209,3.6848766247219));
#49708=CARTESIAN_POINT('Ctrl Pts',(3.30852724093942,0.794772684000846,3.62071968257323));
#49709=CARTESIAN_POINT('Ctrl Pts',(3.34969625632022,1.06852528713348,3.58035913324092));
#49710=CARTESIAN_POINT('Ctrl Pts',(3.36860193479976,1.18523969452325,3.57359493601362));
#49711=CARTESIAN_POINT('Ctrl Pts',(3.38858855032014,1.30014322216932,3.57754124552071));
#49712=CARTESIAN_POINT('Ctrl Pts',(3.55125760872384,-1.30000000000135,3.76488742240349));
#49713=CARTESIAN_POINT('Ctrl Pts',(3.51994370793949,-1.1851427086127,3.75358829971908));
#49714=CARTESIAN_POINT('Ctrl Pts',(3.48803104416294,-1.06847604194559,3.75046543253572));
#49715=CARTESIAN_POINT('Ctrl Pts',(3.41292314443867,-0.794772684000858,
3.76213977047639));
#49716=CARTESIAN_POINT('Ctrl Pts',(3.35964999376592,-0.636309800095202,
3.80257521452938));
#49717=CARTESIAN_POINT('Ctrl Pts',(3.29088986736577,-0.319434907277161,
3.8318703722204));
#49718=CARTESIAN_POINT('Ctrl Pts',(3.25849766059209,-0.158333333333334,
3.85531320792739));
#49719=CARTESIAN_POINT('Ctrl Pts',(3.23636220474763,0.158333333333336,3.83390613421074));
#49720=CARTESIAN_POINT('Ctrl Pts',(3.24588861328513,0.319434907277171,3.78841736816753));
#49721=CARTESIAN_POINT('Ctrl Pts',(3.27104806480137,0.636309800095212,3.71681884761097));
#49722=CARTESIAN_POINT('Ctrl Pts',(3.30067777372572,0.794772684000843,3.65401339492102));
#49723=CARTESIAN_POINT('Ctrl Pts',(3.34336407352903,1.06852528713348,3.60946500285551));
#49724=CARTESIAN_POINT('Ctrl Pts',(3.36300630369808,1.18523969452325,3.59964787807733));
#49725=CARTESIAN_POINT('Ctrl Pts',(3.38380909159561,1.30014322216933,3.59930152167878));
#49726=CARTESIAN_POINT('Ctrl Pts',(3.54143697371732,-1.30000000000136,3.79420796713043));
#49727=CARTESIAN_POINT('Ctrl Pts',(3.50854073084844,-1.1851427086127,3.78880121095158));
#49728=CARTESIAN_POINT('Ctrl Pts',(3.47534451349436,-1.06847604194558,3.78989510533326));
#49729=CARTESIAN_POINT('Ctrl Pts',(3.39796160945554,-0.794772684000852,
3.80744002343325));
#49730=CARTESIAN_POINT('Ctrl Pts',(3.34389786299372,-0.636309800095203,
3.84597495349244));
#49731=CARTESIAN_POINT('Ctrl Pts',(3.27464436116271,-0.319434907277163,
3.87513301512672));
#49732=CARTESIAN_POINT('Ctrl Pts',(3.2426752008845,-0.158333333333334,3.89660192235794));
#49733=CARTESIAN_POINT('Ctrl Pts',(3.22166096247914,0.158333333333336,3.87595595768556));
#49734=CARTESIAN_POINT('Ctrl Pts',(3.23257771150001,0.319434907277168,3.83369951488959));
#49735=CARTESIAN_POINT('Ctrl Pts',(3.25910447812562,0.636309800095211,3.76277547949074));
#49736=CARTESIAN_POINT('Ctrl Pts',(3.28834676493135,0.794772684000847,3.70095602241445));
#49737=CARTESIAN_POINT('Ctrl Pts',(3.3330176648565,1.06852528713348,3.65028482032406));
#49738=CARTESIAN_POINT('Ctrl Pts',(3.35389657654681,1.18523969452325,3.63620894075663));
#49739=CARTESIAN_POINT('Ctrl Pts',(3.37631346515805,1.30014322216933,3.62999603702785));
#49740=CARTESIAN_POINT('Ctrl Pts',(3.5308494554429,-1.30000000000135,3.82301235750127));
#49741=CARTESIAN_POINT('Ctrl Pts',(3.49565379721992,-1.1851427086127,3.82299168397096));
#49742=CARTESIAN_POINT('Ctrl Pts',(3.46082623482376,-1.06847604194559,3.82805987493514));
#49743=CARTESIAN_POINT('Ctrl Pts',(3.38121797345607,-0.79477268400086,3.85152470495659));
#49744=CARTESIAN_POINT('Ctrl Pts',(3.3279576869809,-0.636309800095204,3.88931306817055));
#49745=CARTESIAN_POINT('Ctrl Pts',(3.25892586967109,-0.319434907277163,
3.9188460358497));
#49746=CARTESIAN_POINT('Ctrl Pts',(3.22769302712512,-0.158333333333334,
3.93853026895662));
#49747=CARTESIAN_POINT('Ctrl Pts',(3.20691438908692,0.158333333333336,3.91804349652783));
#49748=CARTESIAN_POINT('Ctrl Pts',(3.21706206652025,0.319434907277172,3.87755908286915));
#49749=CARTESIAN_POINT('Ctrl Pts',(3.24439366783777,0.636309800095215,3.80693442462951));
#49750=CARTESIAN_POINT('Ctrl Pts',(3.27458119135646,0.79477268400085,3.7470230193912));
#49751=CARTESIAN_POINT('Ctrl Pts',(3.32176363692496,1.06852528713348,3.6905707095344));
#49752=CARTESIAN_POINT('Ctrl Pts',(3.34402017306192,1.18523969452325,3.67231724709913));
#49753=CARTESIAN_POINT('Ctrl Pts',(3.36810489928664,1.30014322216932,3.66025219477543));
#49754=CARTESIAN_POINT('Ctrl Pts',(3.52371537962296,-1.30000000000135,3.84339604055803));
#49755=CARTESIAN_POINT('Ctrl Pts',(3.48731301665105,-1.1851427086127,3.84745493965236));
#49756=CARTESIAN_POINT('Ctrl Pts',(3.45142165013046,-1.06847604194559,3.85537158057938));
#49757=CARTESIAN_POINT('Ctrl Pts',(3.36968591745182,-0.79477268400086,3.88257276021143));
#49758=CARTESIAN_POINT('Ctrl Pts',(3.31503821404233,-0.636309800095207,
3.91839227977945));
#49759=CARTESIAN_POINT('Ctrl Pts',(3.24543711991941,-0.319434907277165,
3.94766351942526));
#49760=CARTESIAN_POINT('Ctrl Pts',(3.21504596931657,-0.158333333333335,
3.96635996650926));
#49761=CARTESIAN_POINT('Ctrl Pts',(3.19521296665219,0.158333333333337,3.94655979247265));
#49762=CARTESIAN_POINT('Ctrl Pts',(3.20589244968541,0.31943490727717,3.90809629468899));
#49763=CARTESIAN_POINT('Ctrl Pts',(3.23484799455299,0.636309800095215,3.83842605633801));
#49764=CARTESIAN_POINT('Ctrl Pts',(3.2663336670866,0.794772684000854,3.78025792039953));
#49765=CARTESIAN_POINT('Ctrl Pts',(3.31526112888122,1.06852528713349,3.71973885925459));
#49766=CARTESIAN_POINT('Ctrl Pts',(3.3382448472766,1.18523969452325,3.69839512736118));
#49767=CARTESIAN_POINT('Ctrl Pts',(3.36302840712315,1.30014322216933,3.68191029696368));
#49768=CARTESIAN_POINT('Ctrl Pts',(3.51979390028975,-1.30000000000136,3.85333145849074));
#49769=CARTESIAN_POINT('Ctrl Pts',(3.48238428396745,-1.1851427086127,3.85912832344819));
#49770=CARTESIAN_POINT('Ctrl Pts',(3.44581182126015,-1.06847604194559,3.86835725545699));
#49771=CARTESIAN_POINT('Ctrl Pts',(3.36325610843303,-0.794772684000859,
3.89760669611004));
#49772=CARTESIAN_POINT('Ctrl Pts',(3.30933112338547,-0.636309800095206,
3.93349727704609));
#49773=CARTESIAN_POINT('Ctrl Pts',(3.23978280683933,-0.319434907277165,
3.96288649231997));
#49774=CARTESIAN_POINT('Ctrl Pts',(3.20930922997601,-0.158333333333335,
3.98070348680371));
#49775=CARTESIAN_POINT('Ctrl Pts',(3.1893653703264,0.158333333333337,3.96082437654682));
#49776=CARTESIAN_POINT('Ctrl Pts',(3.19981109945215,0.319434907277172,3.9230136476974));
#49777=CARTESIAN_POINT('Ctrl Pts',(3.22890628758542,0.636309800095216,3.85336559723001));
#49778=CARTESIAN_POINT('Ctrl Pts',(3.26044354591702,0.794772684000854,3.79569967042955));
#49779=CARTESIAN_POINT('Ctrl Pts',(3.31033911162144,1.06852528713349,3.73321313335938));
#49780=CARTESIAN_POINT('Ctrl Pts',(3.33393151120473,1.18523969452325,3.71048413390068));
#49781=CARTESIAN_POINT('Ctrl Pts',(3.35951327834847,1.30014322216933,3.69208061652413));
#49782=CARTESIAN_POINT('Ctrl Pts',(3.5179290077231,-1.30000000000135,3.85837468584765));
#49783=CARTESIAN_POINT('Ctrl Pts',(3.48005403549629,-1.1851427086127,3.86506852730633));
#49784=CARTESIAN_POINT('Ctrl Pts',(3.44314187351344,-1.06847604194559,3.87495403837134));
#49785=CARTESIAN_POINT('Ctrl Pts',(3.36009167935358,-0.794772684000861,
3.90516494180309));
#49786=CARTESIAN_POINT('Ctrl Pts',(3.30629219032297,-0.636309800095207,
3.94091742287119));
#49787=CARTESIAN_POINT('Ctrl Pts',(3.23666675631854,-0.319434907277165,
3.97028826328755));
#49788=CARTESIAN_POINT('Ctrl Pts',(3.20612698068171,-0.158333333333335,
3.98764668534676));
#49789=CARTESIAN_POINT('Ctrl Pts',(3.18630624078372,0.158333333333337,3.96785644620198));
#49790=CARTESIAN_POINT('Ctrl Pts',(3.19698046189018,0.319434907277171,3.9306236218399));
#49791=CARTESIAN_POINT('Ctrl Pts',(3.22632376004245,0.636309800095215,3.86111292352323));
#49792=CARTESIAN_POINT('Ctrl Pts',(3.25777655973932,0.794772684000855,3.80361188830843));
#49793=CARTESIAN_POINT('Ctrl Pts',(3.30817850266376,1.06852528713349,3.74015681273327));
#49794=CARTESIAN_POINT('Ctrl Pts',(3.33209361724937,1.18523969452325,3.71674937395376));
#49795=CARTESIAN_POINT('Ctrl Pts',(3.35810157080076,1.30014322216933,3.69740832117871));
#49796=CARTESIAN_POINT('Ctrl Pts',(3.51685348631722,-1.30000000000135,3.86124902200402));
#49797=CARTESIAN_POINT('Ctrl Pts',(3.47871524848394,-1.1851427086127,3.86845787734754));
#49798=CARTESIAN_POINT('Ctrl Pts',(3.44161058451423,-1.06847604194559,3.87872010796917));
#49799=CARTESIAN_POINT('Ctrl Pts',(3.35827915037236,-0.794772684000861,
3.90948182137531));
#49800=CARTESIAN_POINT('Ctrl Pts',(3.30454936288267,-0.636309800095207,
3.94515362384163));
#49801=CARTESIAN_POINT('Ctrl Pts',(3.23487623129755,-0.319434907277165,
3.97451120451713));
#49802=CARTESIAN_POINT('Ctrl Pts',(3.20429173341362,-0.158333333333335,
3.99160236582141));
#49803=CARTESIAN_POINT('Ctrl Pts',(3.18454347805265,0.158333333333337,3.97186450496687));
#49804=CARTESIAN_POINT('Ctrl Pts',(3.19535519874992,0.319434907277171,3.93496742549603));
#49805=CARTESIAN_POINT('Ctrl Pts',(3.22485250527958,0.636309800095216,3.86554387127726));
#49806=CARTESIAN_POINT('Ctrl Pts',(3.25627421268125,0.794772684000854,3.80814857075943));
#49807=CARTESIAN_POINT('Ctrl Pts',(3.30696480236959,1.06852528713349,3.74413943949904));
#49808=CARTESIAN_POINT('Ctrl Pts',(3.33105931371092,1.18523969452325,3.72034083223412));
#49809=CARTESIAN_POINT('Ctrl Pts',(3.3573010868368,1.30014322216933,3.70045732919041));
#49810=CARTESIAN_POINT('Ctrl Pts',(3.51180487015753,-1.30000000000136,3.87401110494669));
#49811=CARTESIAN_POINT('Ctrl Pts',(3.47264024281404,-1.1851427086127,3.88366306949258));
#49812=CARTESIAN_POINT('Ctrl Pts',(3.43474217778609,-1.06847604194559,3.89567950440077));
#49813=CARTESIAN_POINT('Ctrl Pts',(3.35011607841354,-0.794772684000859,
3.92890227246578));
#49814=CARTESIAN_POINT('Ctrl Pts',(3.2962603770796,-0.636309800095206,3.9638733351931));
#49815=CARTESIAN_POINT('Ctrl Pts',(3.22630686737986,-0.319434907277165,
3.99312184883118));
#49816=CARTESIAN_POINT('Ctrl Pts',(3.19568831864123,-0.158333333333335,
4.00914097268011));
#49817=CARTESIAN_POINT('Ctrl Pts',(3.17652657558406,0.158333333333337,3.98983366734609));
#49818=CARTESIAN_POINT('Ctrl Pts',(3.18823486903591,0.319434907277171,3.95465441538546));
#49819=CARTESIAN_POINT('Ctrl Pts',(3.2186450253389,0.636309800095215,3.88577852154938));
#49820=CARTESIAN_POINT('Ctrl Pts',(3.25004744052039,0.794772684000853,3.82892797482705));
#49821=CARTESIAN_POINT('Ctrl Pts',(3.30185451104873,1.06852528713349,3.76229555265933));
#49822=CARTESIAN_POINT('Ctrl Pts',(3.32659192685424,1.18523969452325,3.73662293940689));
#49823=CARTESIAN_POINT('Ctrl Pts',(3.35363611181697,1.30014322216933,3.71412721745266));
#49824=CARTESIAN_POINT('Ctrl Pts',(3.50259650582532,-1.30000000000136,3.89746406347487));
#49825=CARTESIAN_POINT('Ctrl Pts',(3.46154999817241,-1.1851427086127,3.91159800414215));
#49826=CARTESIAN_POINT('Ctrl Pts',(3.42218167181803,-1.06847604194559,3.92682005562182));
#49827=CARTESIAN_POINT('Ctrl Pts',(3.33510989685151,-0.794772684000861,
3.9644997933532));
#49828=CARTESIAN_POINT('Ctrl Pts',(3.28073758681194,-0.636309800095206,
3.9979602998355));
#49829=CARTESIAN_POINT('Ctrl Pts',(3.21051363500489,-0.319434907277164,
4.02719485174671));
#49830=CARTESIAN_POINT('Ctrl Pts',(3.18100004367731,-0.158333333333335,
4.04212537242215));
#49831=CARTESIAN_POINT('Ctrl Pts',(3.16212607813994,0.158333333333337,4.02304941802012));
#49832=CARTESIAN_POINT('Ctrl Pts',(3.17290244559924,0.31943490727717,3.9891388498205));
#49833=CARTESIAN_POINT('Ctrl Pts',(3.20440295564305,0.636309800095215,3.92085259690198));
#49834=CARTESIAN_POINT('Ctrl Pts',(3.23732532390392,0.794772684000853,3.86615764113347));
#49835=CARTESIAN_POINT('Ctrl Pts',(3.29193397918288,1.06852528713349,3.79525519905378));
#49836=CARTESIAN_POINT('Ctrl Pts',(3.31809858178777,1.18523969452325,3.76631546584324));
#49837=CARTESIAN_POINT('Ctrl Pts',(3.34678415229658,1.30014322216933,3.73913427300855));
#49838=CARTESIAN_POINT('Ctrl Pts',(3.49089583575975,-1.30000000000135,3.92550201961658));
#49839=CARTESIAN_POINT('Ctrl Pts',(3.44736236322143,-1.1851427086127,3.94492906119646));
#49840=CARTESIAN_POINT('Ctrl Pts',(3.40609555172084,-1.06847604194558,3.96395922057786));
#49841=CARTESIAN_POINT('Ctrl Pts',(3.31599740219843,-0.794772684000857,
4.00700581844465));
#49842=CARTESIAN_POINT('Ctrl Pts',(3.26166161224019,-0.636309800095204,
4.03913026138824));
#49843=CARTESIAN_POINT('Ctrl Pts',(3.1905759569815,-0.319434907277163,4.06792484823472));
#49844=CARTESIAN_POINT('Ctrl Pts',(3.16068882050753,-0.158333333333334,
4.08020066157171));
#49845=CARTESIAN_POINT('Ctrl Pts',(3.14236254451807,0.158333333333336,4.06156050213763));
#49846=CARTESIAN_POINT('Ctrl Pts',(3.1541827888424,0.319434907277169,4.03086642678733));
#49847=CARTESIAN_POINT('Ctrl Pts',(3.18741079324074,0.636309800095212,3.96365118824068));
#49848=CARTESIAN_POINT('Ctrl Pts',(3.22079758656425,0.79477268400085,3.91058590082593));
#49849=CARTESIAN_POINT('Ctrl Pts',(3.2784066018515,1.06852528713348,3.83421419732015));
#49850=CARTESIAN_POINT('Ctrl Pts',(3.3062703620255,1.18523969452325,3.80127839118273));
#49851=CARTESIAN_POINT('Ctrl Pts',(3.33705519689666,1.30014322216932,3.76847305109419));
#49852=CARTESIAN_POINT('Ctrl Pts',(3.47625432854937,-1.30000000000135,3.95868777960396));
#49853=CARTESIAN_POINT('Ctrl Pts',(3.42911187370096,-1.1851427086127,3.98396161926474));
#49854=CARTESIAN_POINT('Ctrl Pts',(3.38511464244507,-1.06847604194558,4.00719727209129));
#49855=CARTESIAN_POINT('Ctrl Pts',(3.29073833232675,-0.794772684000857,
4.056167659072));
#49856=CARTESIAN_POINT('Ctrl Pts',(3.23624777135572,-0.636309800095203,
4.08654859182015));
#49857=CARTESIAN_POINT('Ctrl Pts',(3.16482158835148,-0.319434907277162,
4.11536321774138));
#49858=CARTESIAN_POINT('Ctrl Pts',(3.13634639591439,-0.158333333333334,
4.12589756673083));
#49859=CARTESIAN_POINT('Ctrl Pts',(3.11868364739977,0.158333333333336,4.10781157269918));
#49860=CARTESIAN_POINT('Ctrl Pts',(3.12966022013018,0.319434907277171,4.07938414633349));
#49861=CARTESIAN_POINT('Ctrl Pts',(3.16477433760615,0.636309800095214,4.01333669546797));
#49862=CARTESIAN_POINT('Ctrl Pts',(3.20002198057908,0.794772684000849,3.96326008053157));
#49863=CARTESIAN_POINT('Ctrl Pts',(3.26221817393558,1.06852528713348,3.88106524589728));
#49864=CARTESIAN_POINT('Ctrl Pts',(3.29253078212396,1.18523969452325,3.84362847782292));
#49865=CARTESIAN_POINT('Ctrl Pts',(3.32622722561664,1.30014322216932,3.80434242564489));
#49866=CARTESIAN_POINT('Ctrl Pts',(3.46117898356208,-1.30000000000135,3.99157311770267));
#49867=CARTESIAN_POINT('Ctrl Pts',(3.41076491298548,-1.1851427086127,4.023001957923));
#49868=CARTESIAN_POINT('Ctrl Pts',(3.36415720577044,-1.06847604194558,4.05056023207062));
#49869=CARTESIAN_POINT('Ctrl Pts',(3.26527753908959,-0.794772684000856,
4.1052835764333));
#49870=CARTESIAN_POINT('Ctrl Pts',(3.20964019318071,-0.636309800095204,
4.13305481307774));
#49871=CARTESIAN_POINT('Ctrl Pts',(3.13712088711537,-0.319434907277164,
4.16127738694213));
#49872=CARTESIAN_POINT('Ctrl Pts',(3.10939958819912,-0.158333333333334,
4.16957122426424));
#49873=CARTESIAN_POINT('Ctrl Pts',(3.09289608996282,0.158333333333336,4.15246771284705));
#49874=CARTESIAN_POINT('Ctrl Pts',(3.10494510744031,0.31943490727717,4.12785984948249));
#49875=CARTESIAN_POINT('Ctrl Pts',(3.14215484712265,0.636309800095213,4.06319052949148));
#49876=CARTESIAN_POINT('Ctrl Pts',(3.1777260399402,0.794772684000852,4.01491400155314));
#49877=CARTESIAN_POINT('Ctrl Pts',(3.24388341852259,1.06852528713348,3.92641073195946));
#49878=CARTESIAN_POINT('Ctrl Pts',(3.27651390845349,1.18523969452325,3.88436610441899));
#49879=CARTESIAN_POINT('Ctrl Pts',(3.31313106099549,1.30014322216932,3.83859566465085));
#49880=CARTESIAN_POINT('Ctrl Pts',(3.44485221849218,-1.30000000000135,4.02343367468143));
#49881=CARTESIAN_POINT('Ctrl Pts',(3.3904531107521,-1.1851427086127,4.06041041072846));
#49882=CARTESIAN_POINT('Ctrl Pts',(3.34077120931611,-1.06847604194558,4.09188873350675));
#49883=CARTESIAN_POINT('Ctrl Pts',(3.23689376840521,-0.794772684000859,
4.15190752173675));
#49884=CARTESIAN_POINT('Ctrl Pts',(3.18091387827706,-0.636309800095201,
4.1776973988966));
#49885=CARTESIAN_POINT('Ctrl Pts',(3.10714605361911,-0.319434907277161,
4.20514333036985));
#49886=CARTESIAN_POINT('Ctrl Pts',(3.07968331606346,-0.158333333333333,
4.21070967621743));
#49887=CARTESIAN_POINT('Ctrl Pts',(3.06375590315938,0.158333333333335,4.19416442293091));
#49888=CARTESIAN_POINT('Ctrl Pts',(3.07589901910471,0.319434907277169,4.17273488913912));
#49889=CARTESIAN_POINT('Ctrl Pts',(3.11598582338588,0.63630980009521,4.11019815002703));
#49890=CARTESIAN_POINT('Ctrl Pts',(3.15393758156696,0.794772684000845,4.06545604734486));
#49891=CARTESIAN_POINT('Ctrl Pts',(3.22569455534372,1.06852528713348,3.97196316158908));
#49892=CARTESIAN_POINT('Ctrl Pts',(3.26123632842328,1.18523969452324,3.92576064732784));
#49893=CARTESIAN_POINT('Ctrl Pts',(3.30125161870687,1.30014322216932,3.87383476312156));
#49894=CARTESIAN_POINT('Ctrl Pts',(3.43445482759663,-1.30000000000135,4.04512352187352));
#49895=CARTESIAN_POINT('Ctrl Pts',(3.37739310683949,-1.1851427086127,4.08582511462002));
#49896=CARTESIAN_POINT('Ctrl Pts',(3.32553252350525,-1.06847604194558,4.11982694886549));
#49897=CARTESIAN_POINT('Ctrl Pts',(3.2177398692601,-0.794772684000855,4.18290020559656));
#49898=CARTESIAN_POINT('Ctrl Pts',(3.1602717043156,-0.636309800095199,4.2062596545617));
#49899=CARTESIAN_POINT('Ctrl Pts',(3.08559934474851,-0.31943490727716,4.23313249169756));
#49900=CARTESIAN_POINT('Ctrl Pts',(3.05951170294829,-0.158333333333333,
4.23793047763546));
#49901=CARTESIAN_POINT('Ctrl Pts',(3.04424337809605,0.158333333333335,4.22200977856802));
#49902=CARTESIAN_POINT('Ctrl Pts',(3.05606999883945,0.31943490727717,4.20236614100586));
#49903=CARTESIAN_POINT('Ctrl Pts',(3.09759007473543,0.63630980009521,4.14087419196223));
#49904=CARTESIAN_POINT('Ctrl Pts',(3.13660284781725,0.794772684000843,4.09810486373787));
#49905=CARTESIAN_POINT('Ctrl Pts',(3.21170591764102,1.06852528713347,4.0009754697502));
#49906=CARTESIAN_POINT('Ctrl Pts',(3.24908590504518,1.18523969452324,3.95191024741244));
#49907=CARTESIAN_POINT('Ctrl Pts',(3.29132888160908,1.30014322216931,3.89583342772439));
#49908=CARTESIAN_POINT('Ctrl Pts',(3.42583540128219,-1.30000000000135,4.06067213536237));
#49909=CARTESIAN_POINT('Ctrl Pts',(3.36661288013924,-1.1851427086127,4.10398359613909));
#49910=CARTESIAN_POINT('Ctrl Pts',(3.31307522218595,-1.06847604194558,4.13980302109888));
#49911=CARTESIAN_POINT('Ctrl Pts',(3.20252569336342,-0.794772684000855,
4.2052449568935));
#49912=CARTESIAN_POINT('Ctrl Pts',(3.1448199300957,-0.636309800095199,4.22749548355176));
#49913=CARTESIAN_POINT('Ctrl Pts',(3.06936510190686,-0.319434907277159,
4.25380950454983));
#49914=CARTESIAN_POINT('Ctrl Pts',(3.04329844177634,-0.158333333333333,
4.25715800894188));
#49915=CARTESIAN_POINT('Ctrl Pts',(3.02831998681033,0.158333333333335,4.241544528057));
#49916=CARTESIAN_POINT('Ctrl Pts',(3.04035721885161,0.319434907277168,4.22365522892132));
#49917=CARTESIAN_POINT('Ctrl Pts',(3.08336891334343,0.636309800095208,4.16335268713494));
#49918=CARTESIAN_POINT('Ctrl Pts',(3.12328012705945,0.794772684000842,4.12220188537788));
#49919=CARTESIAN_POINT('Ctrl Pts',(3.20157995038045,1.06852528713347,4.02295034772459));
#49920=CARTESIAN_POINT('Ctrl Pts',(3.24072639992362,1.18523969452324,3.97206638214448));
#49921=CARTESIAN_POINT('Ctrl Pts',(3.28511821848901,1.30014322216931,3.91327088983663));
#49922=CARTESIAN_POINT('Ctrl Pts',(3.41867497750123,-1.30000000000135,4.07366642162037));
#49923=CARTESIAN_POINT('Ctrl Pts',(3.35786428909695,-1.1851427086127,4.11939666182868));
#49924=CARTESIAN_POINT('Ctrl Pts',(3.30294497738628,-1.06847604194559,4.15678994545929));
#49925=CARTESIAN_POINT('Ctrl Pts',(3.1896806394923,-0.794772684000859,4.22391587364973));
#49926=CARTESIAN_POINT('Ctrl Pts',(3.12999634180018,-0.6363098000952,4.24366964123252));
#49927=CARTESIAN_POINT('Ctrl Pts',(3.05446827144717,-0.319434907277159,
4.27009294864879));
#49928=CARTESIAN_POINT('Ctrl Pts',(3.03115588594621,-0.158333333333333,
4.27472361324213));
#49929=CARTESIAN_POINT('Ctrl Pts',(3.01693050365394,0.158333333333335,4.25983509121364));
#49930=CARTESIAN_POINT('Ctrl Pts',(3.02744853280611,0.31943490727717,4.2418711520045));
#49931=CARTESIAN_POINT('Ctrl Pts',(3.07108562688173,0.63630980009521,4.18195307022728));
#49932=CARTESIAN_POINT('Ctrl Pts',(3.11216848002771,0.794772684000844,4.14246168042456));
#49933=CARTESIAN_POINT('Ctrl Pts',(3.19285610432454,1.06852528713347,4.04114397801849));
#49934=CARTESIAN_POINT('Ctrl Pts',(3.23327308090119,1.18523969452324,3.98854953307814));
#49935=CARTESIAN_POINT('Ctrl Pts',(3.27917211935977,1.30014322216931,3.92722765900645));
#49936=CARTESIAN_POINT('Ctrl Pts',(3.41288009340851,-1.30000000000134,4.0840369854531));
#49937=CARTESIAN_POINT('Ctrl Pts',(3.3501085556977,-1.18514270861269,4.13109309512308));
#49938=CARTESIAN_POINT('Ctrl Pts',(3.2938516684092,-1.06847604194558,4.1695359618191));
#49939=CARTESIAN_POINT('Ctrl Pts',(3.17893715034814,-0.794772684000856,
4.2384483600127));
#49940=CARTESIAN_POINT('Ctrl Pts',(3.12033039179534,-0.636309800095199,
4.25855232243253));
#49941=CARTESIAN_POINT('Ctrl Pts',(3.04531401376896,-0.31943490727716,4.28547323290277));
#49942=CARTESIAN_POINT('Ctrl Pts',(3.0229656380322,-0.158333333333333,4.2898835348833));
#49943=CARTESIAN_POINT('Ctrl Pts',(3.00852261298693,0.158333333333335,4.27481928527001));
#49944=CARTESIAN_POINT('Ctrl Pts',(3.0174471831594,0.319434907277169,4.25653778583326));
#49945=CARTESIAN_POINT('Ctrl Pts',(3.06096808240439,0.636309800095209,4.19650192222135));
#49946=CARTESIAN_POINT('Ctrl Pts',(3.1026006996025,0.794772684000843,4.1581458150171));
#49947=CARTESIAN_POINT('Ctrl Pts',(3.18512170256247,1.06852528713347,4.05516397331139));
#49948=CARTESIAN_POINT('Ctrl Pts',(3.22664119150678,1.18523969452324,4.00127326457945));
#49949=CARTESIAN_POINT('Ctrl Pts',(3.27395146596591,1.30014322216931,3.93807937694368));
#49950=CARTESIAN_POINT('Ctrl Pts',(3.4085543132438,-1.30000000000134,4.09168377759149));
#49951=CARTESIAN_POINT('Ctrl Pts',(3.34467845415707,-1.18514270861269,4.13986232556471));
#49952=CARTESIAN_POINT('Ctrl Pts',(3.28766192706407,-1.06847604194558,4.17917206071897));
#49953=CARTESIAN_POINT('Ctrl Pts',(3.1717887724725,-0.794772684000855,4.24949668099906));
#49954=CARTESIAN_POINT('Ctrl Pts',(3.11371826607727,-0.636309800095199,
4.26970423515541));
#49955=CARTESIAN_POINT('Ctrl Pts',(3.03899940900825,-0.319434907277159,
4.29698286659211));
#49956=CARTESIAN_POINT('Ctrl Pts',(3.01725958678558,-0.158333333333333,
4.30125685881936));
#49957=CARTESIAN_POINT('Ctrl Pts',(3.00276096947443,0.158333333333335,4.28616267948842));
#49958=CARTESIAN_POINT('Ctrl Pts',(3.01082965053031,0.319434907277169,4.26783367352206));
#49959=CARTESIAN_POINT('Ctrl Pts',(3.05433035874579,0.636309800095209,4.20769258011705));
#49960=CARTESIAN_POINT('Ctrl Pts',(3.09623103923164,0.794772684000843,4.16992322245467));
#49961=CARTESIAN_POINT('Ctrl Pts',(3.17988110680528,1.06852528713347,4.06564020803105));
#49962=CARTESIAN_POINT('Ctrl Pts',(3.22208818472508,1.18523969452324,4.01079574450038));
#49963=CARTESIAN_POINT('Ctrl Pts',(3.27028479171056,1.30014322216931,3.94625770947172));
#49964=CARTESIAN_POINT('Ctrl Pts',(3.40082388779475,-1.30000000000134,4.10430824537168));
#49965=CARTESIAN_POINT('Ctrl Pts',(3.33423500616368,-1.18514270861269,4.15421179357926));
#49966=CARTESIAN_POINT('Ctrl Pts',(3.27551973015998,-1.06847604194558,4.19505922110236));
#49967=CARTESIAN_POINT('Ctrl Pts',(3.15806530074953,-0.794772684000855,
4.26850349972861));
#49968=CARTESIAN_POINT('Ctrl Pts',(3.10273257509845,-0.636309800095199,
4.29056591942227));
#49969=CARTESIAN_POINT('Ctrl Pts',(3.02937307405698,-0.31943490727716,4.3192570837257));
#49970=CARTESIAN_POINT('Ctrl Pts',(3.00855323477179,-0.158333333333333,
4.32288342726441));
#49971=CARTESIAN_POINT('Ctrl Pts',(2.99403405178878,0.158333333333335,4.30779225194209));
#49972=CARTESIAN_POINT('Ctrl Pts',(3.00087337772276,0.319434907277168,4.28986623407122));
#49973=CARTESIAN_POINT('Ctrl Pts',(3.04356111718931,0.636309800095208,4.22882320170994));
#49974=CARTESIAN_POINT('Ctrl Pts',(3.08413237899026,0.794772684000843,4.1904766533688));
#49975=CARTESIAN_POINT('Ctrl Pts',(3.16950424792553,1.06852528713347,4.08314582629006));
#49976=CARTESIAN_POINT('Ctrl Pts',(3.21317507354939,1.18523969452324,4.02651144248977));
#49977=CARTESIAN_POINT('Ctrl Pts',(3.26355369627107,1.30014322216931,3.95971316303145));
#49978=CARTESIAN_POINT('Ctrl Pts',(3.39464917870745,-1.30000000000134,4.11466263946878));
#49979=CARTESIAN_POINT('Ctrl Pts',(3.32510507657478,-1.18514270861269,4.16518479880478));
#49980=CARTESIAN_POINT('Ctrl Pts',(3.26482642907165,-1.06847604194558,4.2069153131676));
#49981=CARTESIAN_POINT('Ctrl Pts',(3.1469757483796,-0.794772684000851,4.28301069085576));
#49982=CARTESIAN_POINT('Ctrl Pts',(3.09694274384213,-0.636309800095197,
4.30845659929));
#49983=CARTESIAN_POINT('Ctrl Pts',(3.02637005246077,-0.319434907277159,
4.33908386446847));
#49984=CARTESIAN_POINT('Ctrl Pts',(3.00610967573939,-0.158333333333332,
4.34183776787586));
#49985=CARTESIAN_POINT('Ctrl Pts',(2.99178190375838,0.158333333333334,4.32686979332697));
#49986=CARTESIAN_POINT('Ctrl Pts',(2.99824187046467,0.319434907277167,4.30984680666278));
#49987=CARTESIAN_POINT('Ctrl Pts',(3.03855572360122,0.636309800095206,4.24730726381801));
#49988=CARTESIAN_POINT('Ctrl Pts',(3.07431251187027,0.79477268400084,4.20635824741822));
#49989=CARTESIAN_POINT('Ctrl Pts',(3.16003068251616,1.06852528713347,4.09631458963396));
#49990=CARTESIAN_POINT('Ctrl Pts',(3.20509827163572,1.18523969452324,4.03856156651537));
#49991=CARTESIAN_POINT('Ctrl Pts',(3.2581204848396,1.30014322216931,3.97070056908081));
#49992=CARTESIAN_POINT('Ctrl Pts',(3.39266784164081,-1.30000000000134,4.12304256032365));
#49993=CARTESIAN_POINT('Ctrl Pts',(3.32321437844547,-1.18514270861269,4.17332679788356));
#49994=CARTESIAN_POINT('Ctrl Pts',(3.26328407460055,-1.06847604194558,4.21505186785088));
#49995=CARTESIAN_POINT('Ctrl Pts',(3.14683348690377,-0.794772684000851,
4.29167173715239));
#49996=CARTESIAN_POINT('Ctrl Pts',(3.09897158712509,-0.636309800095197,
4.31848151812622));
#49997=CARTESIAN_POINT('Ctrl Pts',(3.02986065695598,-0.319434907277159,
4.3499500784224));
#49998=CARTESIAN_POINT('Ctrl Pts',(3.00955419085523,-0.158333333333332,
4.35273203641936));
#49999=CARTESIAN_POINT('Ctrl Pts',(2.99544198242645,0.158333333333334,4.33786307216675));
#50000=CARTESIAN_POINT('Ctrl Pts',(3.00240549451288,0.319434907277167,4.32105409284838));
#50001=CARTESIAN_POINT('Ctrl Pts',(3.04120395637117,0.636309800095206,4.25758354584163));
#50002=CARTESIAN_POINT('Ctrl Pts',(3.07388603025902,0.79477268400084,4.21466382420666));
#50003=CARTESIAN_POINT('Ctrl Pts',(3.15832509141374,1.06852528713347,4.10419092108222));
#50004=CARTESIAN_POINT('Ctrl Pts',(3.20330442392552,1.18523969452324,4.04663254077152));
#50005=CARTESIAN_POINT('Ctrl Pts',(3.25670393351411,1.30014322216931,3.97934667714784));
#50006=CARTESIAN_POINT('Ctrl Pts',(3.39267401414619,-1.3,4.12301649229108));
#50007=CARTESIAN_POINT('Ctrl Pts',(3.32322027641429,-1.18514270861178,4.17330146776302));
#50008=CARTESIAN_POINT('Ctrl Pts',(3.26328889377514,-1.06847604194512,4.2150265525134));
#50009=CARTESIAN_POINT('Ctrl Pts',(3.1468339558515,-0.794772684000851,4.29164478539433));
#50010=CARTESIAN_POINT('Ctrl Pts',(3.09896529592856,-0.636309800095197,
4.31845031956243));
#50011=CARTESIAN_POINT('Ctrl Pts',(3.02984981618038,-0.319434907277159,
4.34991626061164));
#50012=CARTESIAN_POINT('Ctrl Pts',(3.00954349196179,-0.158333333333332,
4.35269813353154));
#50013=CARTESIAN_POINT('Ctrl Pts',(2.99543061314513,0.158333333333334,4.33782886127835));
#50014=CARTESIAN_POINT('Ctrl Pts',(3.0023925612396,0.319434907277167,4.321019214687));
#50015=CARTESIAN_POINT('Ctrl Pts',(3.04119573834858,0.636309800095206,4.25755156466003));
#50016=CARTESIAN_POINT('Ctrl Pts',(3.0738873794296,0.79477268400084,4.21463797384584));
#50017=CARTESIAN_POINT('Ctrl Pts',(3.15831522453555,1.06847604194511,4.10418628394815));
#50018=CARTESIAN_POINT('Ctrl Pts',(3.2032726433294,1.18514270861178,4.04665525660054));
#50019=CARTESIAN_POINT('Ctrl Pts',(3.25664179513071,1.3,3.97940364582358));
#50020=CARTESIAN_POINT('',(3.5320296967332,-1.2,3.73196507782941));
#50021=CARTESIAN_POINT('Ctrl Pts',(3.5320296967332,-1.2,3.73196507782941));
#50022=CARTESIAN_POINT('Ctrl Pts',(3.53028867930381,-1.21211429492071,3.74748292462223));
#50023=CARTESIAN_POINT('Ctrl Pts',(3.52932228775817,-1.22418007100414,3.76371958287565));
#50024=CARTESIAN_POINT('Ctrl Pts',(3.52404626292729,-1.25801070045455,3.80696300336817));
#50025=CARTESIAN_POINT('Ctrl Pts',(3.52267668202219,-1.26620635932822,3.81736245170488));
#50026=CARTESIAN_POINT('Ctrl Pts',(3.52019027398267,-1.28225243755813,3.83796696657072));
#50027=CARTESIAN_POINT('Ctrl Pts',(3.518816732318,-1.28996988102069,3.84770823323038));
#50028=CARTESIAN_POINT('Ctrl Pts',(3.51736191102066,-1.29864194176201,3.85876656793681));
#50029=CARTESIAN_POINT('Ctrl Pts',(3.51725750255116,-1.2992769549125,3.85957876048008));
#50030=CARTESIAN_POINT('Ctrl Pts',(3.51713261275492,-1.30000000000135,3.86049731482626));
#50031=CARTESIAN_POINT('',(3.42060206186096,-0.653834841369904,3.62201431891782));
#50032=CARTESIAN_POINT('Ctrl Pts',(3.42060206188991,-0.653834841368647,
3.62201431889471));
#50033=CARTESIAN_POINT('Ctrl Pts',(3.43224320734967,-0.717311520958095,
3.63314340931357));
#50034=CARTESIAN_POINT('Ctrl Pts',(3.44190785954811,-0.76493199155208,3.64246729321156));
#50035=CARTESIAN_POINT('Ctrl Pts',(3.47882511314388,-0.949616792156694,
3.67842212036166));
#50036=CARTESIAN_POINT('Ctrl Pts',(3.50217968247802,-1.06344427584388,3.70156424878262));
#50037=CARTESIAN_POINT('Ctrl Pts',(3.5320296967332,-1.2,3.73196507782941));
#50038=CARTESIAN_POINT('',(3.31841464832137,0.653834841531101,3.5270414892343));
#50039=CARTESIAN_POINT('Ctrl Pts',(3.31841464832137,0.653834841531103,3.52704148923431));
#50040=CARTESIAN_POINT('Ctrl Pts',(3.30612895695982,0.575984024643342,3.56675609404422));
#50041=CARTESIAN_POINT('Ctrl Pts',(3.29646327650278,0.493650097853836,3.60055643709482));
#50042=CARTESIAN_POINT('Ctrl Pts',(3.2849183733937,0.338156451488989,3.6498336491464));
#50043=CARTESIAN_POINT('Ctrl Pts',(3.28204499020856,0.265682397105468,3.66749131270142));
#50044=CARTESIAN_POINT('Ctrl Pts',(3.28241779428724,0.129732771186047,3.69186605780633));
#50045=CARTESIAN_POINT('Ctrl Pts',(3.28481237300939,0.0666332289558237,
3.69978892565048));
#50046=CARTESIAN_POINT('Ctrl Pts',(3.29431982878688,-0.0595523952111457,
3.70913249053805));
#50047=CARTESIAN_POINT('Ctrl Pts',(3.30149068665183,-0.122793824757702,
3.7106341531275));
#50048=CARTESIAN_POINT('Ctrl Pts',(3.32176361712298,-0.260152744154284,
3.70625373983926));
#50049=CARTESIAN_POINT('Ctrl Pts',(3.33571246492882,-0.333967683943717,
3.69897587089194));
#50050=CARTESIAN_POINT('Ctrl Pts',(3.37149324193757,-0.491223354642014,
3.6719351756202));
#50051=CARTESIAN_POINT('Ctrl Pts',(3.39449120914342,-0.57435899131098,3.65030401370791));
#50052=CARTESIAN_POINT('Ctrl Pts',(3.42060206187218,-0.653834841386456,
3.62201431897468));
#50053=CARTESIAN_POINT('',(3.37161559917284,1.2,3.57581619513933));
#50054=CARTESIAN_POINT('Ctrl Pts',(3.37161559917284,1.2,3.57581619513933));
#50055=CARTESIAN_POINT('Ctrl Pts',(3.36149720337276,1.12668871690934,3.56640294709369));
#50056=CARTESIAN_POINT('Ctrl Pts',(3.34983325017182,1.03142317896752,3.55563034886084));
#50057=CARTESIAN_POINT('Ctrl Pts',(3.32722135236781,0.796454095927989,3.53499453597592));
#50058=CARTESIAN_POINT('Ctrl Pts',(3.32317714215184,0.739661249859152,3.53134426838176));
#50059=CARTESIAN_POINT('Ctrl Pts',(3.31841464832137,0.653834841531101,3.52704148923431));
#50060=CARTESIAN_POINT('Ctrl Pts',(3.35740616785769,1.30000000000401,3.69995373973539));
#50061=CARTESIAN_POINT('Ctrl Pts',(3.35984187854911,1.28338139784583,3.67926185597637));
#50062=CARTESIAN_POINT('Ctrl Pts',(3.36202234317964,1.27060240530429,3.6636799898001));
#50063=CARTESIAN_POINT('Ctrl Pts',(3.36677577393269,1.23928230445676,3.62508321444296));
#50064=CARTESIAN_POINT('Ctrl Pts',(3.3675752148028,1.23365566836096,3.61811282666168));
#50065=CARTESIAN_POINT('Ctrl Pts',(3.36962079575489,1.21824133508529,3.59889874207068));
#50066=CARTESIAN_POINT('Ctrl Pts',(3.37086515981833,1.20824229626914,3.58637558604191));
#50067=CARTESIAN_POINT('Ctrl Pts',(3.37161559917284,1.2,3.57581619513933));
#50068=CARTESIAN_POINT('Ctrl Pts',(3.39267401414619,-1.3,4.12301649229108));
#50069=CARTESIAN_POINT('Ctrl Pts',(3.32322027641429,-1.18514270861178,4.17330146776302));
#50070=CARTESIAN_POINT('Ctrl Pts',(3.26328889377514,-1.06847604194512,4.2150265525134));
#50071=CARTESIAN_POINT('Ctrl Pts',(3.1468339558515,-0.794772684000851,4.29164478539432));
#50072=CARTESIAN_POINT('Ctrl Pts',(3.09896529592856,-0.636309800095196,
4.31845031956243));
#50073=CARTESIAN_POINT('Ctrl Pts',(3.02984981618038,-0.319434907277159,
4.34991626061163));
#50074=CARTESIAN_POINT('Ctrl Pts',(3.00954349196179,-0.158333333333332,
4.35269813353154));
#50075=CARTESIAN_POINT('Ctrl Pts',(2.99543061314513,0.158333333333334,4.33782886127834));
#50076=CARTESIAN_POINT('Ctrl Pts',(3.0023925612396,0.319434907277167,4.321019214687));
#50077=CARTESIAN_POINT('Ctrl Pts',(3.04119573834857,0.636309800095206,4.25755156466003));
#50078=CARTESIAN_POINT('Ctrl Pts',(3.0738873794296,0.79477268400084,4.21463797384584));
#50079=CARTESIAN_POINT('Ctrl Pts',(3.15831522453555,1.06847604194511,4.10418628394815));
#50080=CARTESIAN_POINT('Ctrl Pts',(3.20327264332939,1.18514270861178,4.04665525660054));
#50081=CARTESIAN_POINT('Ctrl Pts',(3.25664179513071,1.3,3.97940364582358));
#50082=CARTESIAN_POINT('Ctrl Pts',(3.44290446030743,-1.3,4.18129180055357));
#50083=CARTESIAN_POINT('Ctrl Pts',(3.37244803687278,-1.18514270861178,4.23016414502714));
#50084=CARTESIAN_POINT('Ctrl Pts',(3.31185538302694,-1.06847604194512,4.27088003735102));
#50085=CARTESIAN_POINT('Ctrl Pts',(3.19466151211464,-0.794772684000851,
4.34609885764707));
#50086=CARTESIAN_POINT('Ctrl Pts',(3.14738383460685,-0.636309800095196,
4.37331150080897));
#50087=CARTESIAN_POINT('Ctrl Pts',(3.07891484675056,-0.319434907277159,
4.40494093928184));
#50088=CARTESIAN_POINT('Ctrl Pts',(3.05956220283012,-0.158333333333332,
4.40851776232448));
#50089=CARTESIAN_POINT('Ctrl Pts',(3.04571607718934,0.158333333333334,4.39340830443289));
#50090=CARTESIAN_POINT('Ctrl Pts',(3.05198711671704,0.319434907277167,4.37556710698916));
#50091=CARTESIAN_POINT('Ctrl Pts',(3.09069526886232,0.636309800095206,4.31143941648607));
#50092=CARTESIAN_POINT('Ctrl Pts',(3.12304380561888,0.79477268400084,4.26789552624273));
#50093=CARTESIAN_POINT('Ctrl Pts',(3.20878615765139,1.06847604194511,4.15832499982844));
#50094=CARTESIAN_POINT('Ctrl Pts',(3.25467811874699,1.18514270861178,4.10155711050815));
#50095=CARTESIAN_POINT('Ctrl Pts',(3.3093473538106,1.3,4.03545035276417));
#50096=CARTESIAN_POINT('Ctrl Pts',(3.49313490646867,-1.3,4.23956710881606));
#50097=CARTESIAN_POINT('Ctrl Pts',(3.42167579733126,-1.18514270861178,4.28702682229127));
#50098=CARTESIAN_POINT('Ctrl Pts',(3.36042187227873,-1.06847604194512,4.32673352218864));
#50099=CARTESIAN_POINT('Ctrl Pts',(3.24248906837778,-0.794772684000851,
4.40055292989982));
#50100=CARTESIAN_POINT('Ctrl Pts',(3.19580237328514,-0.636309800095196,
4.42817268205552));
#50101=CARTESIAN_POINT('Ctrl Pts',(3.12797987732074,-0.319434907277159,
4.45996561795205));
#50102=CARTESIAN_POINT('Ctrl Pts',(3.10958091369845,-0.158333333333332,
4.46433739111742));
#50103=CARTESIAN_POINT('Ctrl Pts',(3.09600154123355,0.158333333333334,4.44898774758743));
#50104=CARTESIAN_POINT('Ctrl Pts',(3.10158167219449,0.319434907277167,4.43011499929131));
#50105=CARTESIAN_POINT('Ctrl Pts',(3.14019479937607,0.636309800095206,4.36532726831211));
#50106=CARTESIAN_POINT('Ctrl Pts',(3.17220023180817,0.79477268400084,4.32115307863963));
#50107=CARTESIAN_POINT('Ctrl Pts',(3.25925709076723,1.06847604194511,4.21246371570874));
#50108=CARTESIAN_POINT('Ctrl Pts',(3.30608359416459,1.18514270861178,4.15645896441577));
#50109=CARTESIAN_POINT('Ctrl Pts',(3.3620529124905,1.3,4.09149705970477));
#50110=CARTESIAN_POINT('Ctrl Pts',(3.54336535262991,-1.3,4.29784241707855));
#50111=CARTESIAN_POINT('Ctrl Pts',(3.47090355778975,-1.18514270861178,4.34388949955539));
#50112=CARTESIAN_POINT('Ctrl Pts',(3.40898836153053,-1.06847604194512,4.38258700702626));
#50113=CARTESIAN_POINT('Ctrl Pts',(3.29031662464092,-0.794772684000851,
4.45500700215256));
#50114=CARTESIAN_POINT('Ctrl Pts',(3.24422091196343,-0.636309800095196,
4.48303386330206));
#50115=CARTESIAN_POINT('Ctrl Pts',(3.17704490789093,-0.319434907277159,
4.51499029662226));
#50116=CARTESIAN_POINT('Ctrl Pts',(3.15959962456677,-0.158333333333332,
4.52015701991036));
#50117=CARTESIAN_POINT('Ctrl Pts',(3.14628700527777,0.158333333333334,4.50456719074197));
#50118=CARTESIAN_POINT('Ctrl Pts',(3.15117622767193,0.319434907277167,4.48466289159347));
#50119=CARTESIAN_POINT('Ctrl Pts',(3.18969432988981,0.636309800095206,4.41921512013816));
#50120=CARTESIAN_POINT('Ctrl Pts',(3.22135665799746,0.79477268400084,4.37441063103653));
#50121=CARTESIAN_POINT('Ctrl Pts',(3.30972802388306,1.06847604194511,4.26660243158904));
#50122=CARTESIAN_POINT('Ctrl Pts',(3.35748906958219,1.18514270861178,4.21136081832338));
#50123=CARTESIAN_POINT('Ctrl Pts',(3.4147584711704,1.3,4.14754376664537));
#50124=CARTESIAN_POINT('Ctrl Pts',(3.54336535262991,-1.3,4.29784241707854));
#50125=CARTESIAN_POINT('Ctrl Pts',(3.47090355778975,-1.18514270861178,4.34388949955539));
#50126=CARTESIAN_POINT('Ctrl Pts',(3.40898836153053,-1.06847604194512,4.38258700702626));
#50127=CARTESIAN_POINT('Ctrl Pts',(3.29031662464092,-0.794772684000851,
4.45500700215256));
#50128=CARTESIAN_POINT('Ctrl Pts',(3.24422091196343,-0.636309800095197,
4.48303386330206));
#50129=CARTESIAN_POINT('Ctrl Pts',(3.17704490789093,-0.319434907277159,
4.51499029662226));
#50130=CARTESIAN_POINT('Ctrl Pts',(3.15959962456678,-0.158333333333332,
4.52015701991036));
#50131=CARTESIAN_POINT('Ctrl Pts',(3.14628700527777,0.158333333333334,4.50456719074198));
#50132=CARTESIAN_POINT('Ctrl Pts',(3.15117622767193,0.319434907277167,4.48466289159347));
#50133=CARTESIAN_POINT('Ctrl Pts',(3.18969432988981,0.636309800095206,4.41921512013816));
#50134=CARTESIAN_POINT('Ctrl Pts',(3.22135665799746,0.79477268400084,4.37441063103653));
#50135=CARTESIAN_POINT('Ctrl Pts',(3.30972802388306,1.06847604194511,4.26660243158904));
#50136=CARTESIAN_POINT('Ctrl Pts',(3.35748906958219,1.18514270861178,4.21136081832338));
#50137=CARTESIAN_POINT('Ctrl Pts',(3.4147584711704,1.3,4.14754376664537));
#50138=CARTESIAN_POINT('Ctrl Pts',(3.5433653526303,-1.30000000000062,4.2978424170783));
#50139=CARTESIAN_POINT('Ctrl Pts',(3.47090355778997,-1.1851427086122,4.34388949955525));
#50140=CARTESIAN_POINT('Ctrl Pts',(3.40898836153062,-1.06847604194533,4.3825870070262));
#50141=CARTESIAN_POINT('Ctrl Pts',(3.29031662464092,-0.794772684000851,
4.45500700215256));
#50142=CARTESIAN_POINT('Ctrl Pts',(3.24422091196343,-0.636309800095197,
4.48303386330206));
#50143=CARTESIAN_POINT('Ctrl Pts',(3.17704490789093,-0.319434907277159,
4.51499029662226));
#50144=CARTESIAN_POINT('Ctrl Pts',(3.15959962456678,-0.158333333333332,
4.52015701991036));
#50145=CARTESIAN_POINT('Ctrl Pts',(3.14628700527777,0.158333333333334,4.50456719074198));
#50146=CARTESIAN_POINT('Ctrl Pts',(3.15117622767193,0.319434907277167,4.48466289159347));
#50147=CARTESIAN_POINT('Ctrl Pts',(3.18969432988981,0.636309800095206,4.41921512013816));
#50148=CARTESIAN_POINT('Ctrl Pts',(3.22135665799746,0.79477268400084,4.37441063103653));
#50149=CARTESIAN_POINT('Ctrl Pts',(3.30972802388322,1.0684760419456,4.26660243158885));
#50150=CARTESIAN_POINT('Ctrl Pts',(3.35748906958259,1.18514270861274,4.21136081832292));
#50151=CARTESIAN_POINT('Ctrl Pts',(3.41475847117111,1.30000000000142,4.14754376664458));
#50152=CARTESIAN_POINT('Ctrl Pts',(3.5521021815528,-1.30000000000062,4.29733180414384));
#50153=CARTESIAN_POINT('Ctrl Pts',(3.47911206099876,-1.1851427086122,4.34294158094407));
#50154=CARTESIAN_POINT('Ctrl Pts',(3.41699686806362,-1.06847604194533,4.38170451196752));
#50155=CARTESIAN_POINT('Ctrl Pts',(3.29862160460323,-0.794772684000851,
4.45543705367823));
#50156=CARTESIAN_POINT('Ctrl Pts',(3.25416255203503,-0.636309800095197,
4.48672549546171));
#50157=CARTESIAN_POINT('Ctrl Pts',(3.18775359145329,-0.319434907277159,
4.52028525841712));
#50158=CARTESIAN_POINT('Ctrl Pts',(3.17014714932986,-0.158333333333332,
4.52493089070268));
#50159=CARTESIAN_POINT('Ctrl Pts',(3.15675867145257,0.158333333333334,4.50911671228464));
#50160=CARTESIAN_POINT('Ctrl Pts',(3.1616167155693,0.319434907277167,4.48925446133289));
#50161=CARTESIAN_POINT('Ctrl Pts',(3.19945051410824,0.636309800095206,4.42226516940974));
#50162=CARTESIAN_POINT('Ctrl Pts',(3.22998252758132,0.79477268400084,4.37515732362437));
#50163=CARTESIAN_POINT('Ctrl Pts',(3.31797563069851,1.0684760419456,4.26590655670564));
#50164=CARTESIAN_POINT('Ctrl Pts',(3.36577675439426,1.18514270861274,4.2103224238498));
#50165=CARTESIAN_POINT('Ctrl Pts',(3.42329004791205,1.30000000000142,4.14644476699746));
#50166=CARTESIAN_POINT('Ctrl Pts',(3.56358560401321,-1.30000000000062,4.29301250933056));
#50167=CARTESIAN_POINT('Ctrl Pts',(3.49193405704469,-1.1851427086122,4.33603236797316));
#50168=CARTESIAN_POINT('Ctrl Pts',(3.43108544333025,-1.06847604194533,4.37347838998896));
#50169=CARTESIAN_POINT('Ctrl Pts',(3.31546990986285,-0.794772684000853,
4.44710951424628));
#50170=CARTESIAN_POINT('Ctrl Pts',(3.27311970557639,-0.636309800095198,
4.48352197486765));
#50171=CARTESIAN_POINT('Ctrl Pts',(3.20798893278061,-0.319434907277159,
4.51966840504823));
#50172=CARTESIAN_POINT('Ctrl Pts',(3.18945903340722,-0.158333333333333,
4.52466173920179));
#50173=CARTESIAN_POINT('Ctrl Pts',(3.17601420125164,0.158333333333335,4.50870622817952));
#50174=CARTESIAN_POINT('Ctrl Pts',(3.18188067369713,0.319434907277169,4.4884411098495));
#50175=CARTESIAN_POINT('Ctrl Pts',(3.21803362526629,0.636309800095209,4.41840175019651));
#50176=CARTESIAN_POINT('Ctrl Pts',(3.24556941817653,0.794772684000842,4.36540084563633));
#50177=CARTESIAN_POINT('Ctrl Pts',(3.33084078171532,1.0684760419456,4.25628551380435));
#50178=CARTESIAN_POINT('Ctrl Pts',(3.37761225073271,1.18514270861274,4.20223564636569));
#50179=CARTESIAN_POINT('Ctrl Pts',(3.43424437510688,1.30000000000142,4.14136789551703));
#50180=CARTESIAN_POINT('Ctrl Pts',(3.58056423090191,-1.30000000000062,4.28691857619095));
#50181=CARTESIAN_POINT('Ctrl Pts',(3.51184687283633,-1.1851427086122,4.32773477727964));
#50182=CARTESIAN_POINT('Ctrl Pts',(3.45327824423354,-1.06847604194533,4.36372030623571));
#50183=CARTESIAN_POINT('Ctrl Pts',(3.34141859085254,-0.794772684000853,
4.43569425800561));
#50184=CARTESIAN_POINT('Ctrl Pts',(3.29951533377265,-0.636309800095199,
4.47359261889896));
#50185=CARTESIAN_POINT('Ctrl Pts',(3.23525711070835,-0.319434907277161,
4.51064583822628));
#50186=CARTESIAN_POINT('Ctrl Pts',(3.21604851840059,-0.158333333333333,
4.51690915011358));
#50187=CARTESIAN_POINT('Ctrl Pts',(3.20253345039015,0.158333333333335,4.5008959554661));
#50188=CARTESIAN_POINT('Ctrl Pts',(3.20920278516287,0.319434907277168,4.47960149063721));
#50189=CARTESIAN_POINT('Ctrl Pts',(3.24394413212942,0.636309800095208,4.40793019855565));
#50190=CARTESIAN_POINT('Ctrl Pts',(3.26990464364179,0.794772684000844,4.35186295250137));
#50191=CARTESIAN_POINT('Ctrl Pts',(3.35133623487503,1.0684760419456,4.24419300944702));
#50192=CARTESIAN_POINT('Ctrl Pts',(3.39604531243483,1.18514270861274,4.19184388554515));
#50193=CARTESIAN_POINT('Ctrl Pts',(3.4502147490473,1.30000000000142,4.13375196652515));
#50194=CARTESIAN_POINT('Ctrl Pts',(3.59459177663741,-1.30000000000062,4.2817873486779));
#50195=CARTESIAN_POINT('Ctrl Pts',(3.52830294999471,-1.1851427086122,4.32126438957367));
#50196=CARTESIAN_POINT('Ctrl Pts',(3.47142888440619,-1.06847604194533,4.35617370605141));
#50197=CARTESIAN_POINT('Ctrl Pts',(3.36178839673057,-0.794772684000853,
4.42626885352393));
#50198=CARTESIAN_POINT('Ctrl Pts',(3.31852312824454,-0.636309800095198,
4.46326358015796));
#50199=CARTESIAN_POINT('Ctrl Pts',(3.2544599882222,-0.319434907277159,4.50056569204394));
#50200=CARTESIAN_POINT('Ctrl Pts',(3.2355596056058,-0.158333333333333,4.50890029393364));
#50201=CARTESIAN_POINT('Ctrl Pts',(3.22237306826455,0.158333333333335,4.49336746505154));
#50202=CARTESIAN_POINT('Ctrl Pts',(3.22956496962436,0.319434907277169,4.47118278232066));
#50203=CARTESIAN_POINT('Ctrl Pts',(3.2637573887239,0.636309800095208,4.39881377980514));
#50204=CARTESIAN_POINT('Ctrl Pts',(3.28921334598366,0.794772684000841,4.34112021976925));
#50205=CARTESIAN_POINT('Ctrl Pts',(3.36822517239961,1.0684760419456,4.23499892082117));
#50206=CARTESIAN_POINT('Ctrl Pts',(3.41150609894505,1.18514270861274,4.18404600643178));
#50207=CARTESIAN_POINT('Ctrl Pts',(3.46386666005709,1.30000000000143,4.12807615578604));
#50208=CARTESIAN_POINT('Ctrl Pts',(3.61517717129052,-1.30000000000062,4.27590496591519));
#50209=CARTESIAN_POINT('Ctrl Pts',(3.55257603072622,-1.18514270861221,4.31343443912465));
#50210=CARTESIAN_POINT('Ctrl Pts',(3.49822507367094,-1.06847604194533,4.34665935470873));
#50211=CARTESIAN_POINT('Ctrl Pts',(3.39172306435096,-0.794772684000854,
4.413471167091));
#50212=CARTESIAN_POINT('Ctrl Pts',(3.34628580744375,-0.6363098000952,4.44860492003066));
#50213=CARTESIAN_POINT('Ctrl Pts',(3.2817010387109,-0.319434907277161,4.48490921587586));
#50214=CARTESIAN_POINT('Ctrl Pts',(3.26253764798989,-0.158333333333333,
4.49525969638023));
#50215=CARTESIAN_POINT('Ctrl Pts',(3.24859414851813,0.158333333333335,4.47877122196578));
#50216=CARTESIAN_POINT('Ctrl Pts',(3.25488708647475,0.319434907277168,4.45314814577066));
#50217=CARTESIAN_POINT('Ctrl Pts',(3.28888423186795,0.636309800095209,4.38078135733872));
#50218=CARTESIAN_POINT('Ctrl Pts',(3.31693946370155,0.794772684000846,4.32534030247022));
#50219=CARTESIAN_POINT('Ctrl Pts',(3.39307595215939,1.0684760419456,4.22268003510549));
#50220=CARTESIAN_POINT('Ctrl Pts',(3.43399352685011,1.18514270861274,4.17354996578764));
#50221=CARTESIAN_POINT('Ctrl Pts',(3.48287201151301,1.30000000000142,4.11972765295644));
#50222=CARTESIAN_POINT('Ctrl Pts',(3.64437267289813,-1.30000000000062,4.26737943677028));
#50223=CARTESIAN_POINT('Ctrl Pts',(3.58678645305855,-1.18514270861221,4.30208784740518));
#50224=CARTESIAN_POINT('Ctrl Pts',(3.53590367424904,-1.06847604194533,4.33296392790851));
#50225=CARTESIAN_POINT('Ctrl Pts',(3.43384056593238,-0.794772684000854,
4.39544040135096));
#50226=CARTESIAN_POINT('Ctrl Pts',(3.38623061017473,-0.636309800095199,
4.42929823027561));
#50227=CARTESIAN_POINT('Ctrl Pts',(3.32015703785874,-0.31943490727716,4.46322634983303));
#50228=CARTESIAN_POINT('Ctrl Pts',(3.29807995641088,-0.158333333333333,
4.47281316602024));
#50229=CARTESIAN_POINT('Ctrl Pts',(3.28357941163567,0.158333333333335,4.45563258154672));
#50230=CARTESIAN_POINT('Ctrl Pts',(3.29196321705421,0.319434907277169,4.4297810809044));
#50231=CARTESIAN_POINT('Ctrl Pts',(3.32685587542683,0.636309800095209,4.35899172542706));
#50232=CARTESIAN_POINT('Ctrl Pts',(3.35725208631104,0.794772684000844,4.30498495279098));
#50233=CARTESIAN_POINT('Ctrl Pts',(3.42909951824085,1.0684760419456,4.20665305398618));
#50234=CARTESIAN_POINT('Ctrl Pts',(3.46667275064931,1.18514270861274,4.15991547309123));
#50235=CARTESIAN_POINT('Ctrl Pts',(3.51071912439348,1.30000000000142,4.10900454673807));
#50236=CARTESIAN_POINT('Ctrl Pts',(3.6737420698711,-1.30000000000063,4.25912999654594));
#50237=CARTESIAN_POINT('Ctrl Pts',(3.62184231618095,-1.18514270861221,4.29199543832869));
#50238=CARTESIAN_POINT('Ctrl Pts',(3.57489009921585,-1.06847604194534,4.32116332599509));
#50239=CARTESIAN_POINT('Ctrl Pts',(3.47785088485393,-0.794772684000862,
4.38000489181838));
#50240=CARTESIAN_POINT('Ctrl Pts',(3.4274789502663,-0.636309800095207,4.41148412633647));
#50241=CARTESIAN_POINT('Ctrl Pts',(3.36026164960747,-0.319434907277165,
4.44334903460234));
#50242=CARTESIAN_POINT('Ctrl Pts',(3.3362262356368,-0.158333333333335,4.45351730072373));
#50243=CARTESIAN_POINT('Ctrl Pts',(3.32106806187295,0.158333333333337,4.4354738147948));
#50244=CARTESIAN_POINT('Ctrl Pts',(3.33051057601067,0.31943490727717,4.40793856281615));
#50245=CARTESIAN_POINT('Ctrl Pts',(3.3657003458411,0.636309800095214,4.3379423909508));
#50246=CARTESIAN_POINT('Ctrl Pts',(3.3985296934135,0.794772684000856,4.2855346205433));
#50247=CARTESIAN_POINT('Ctrl Pts',(3.46578958001787,1.06847604194561,4.19129389020568));
#50248=CARTESIAN_POINT('Ctrl Pts',(3.49986477922429,1.18514270861275,4.14683941635537));
#50249=CARTESIAN_POINT('Ctrl Pts',(3.53890086495046,1.30000000000143,4.09872378885478));
#50250=CARTESIAN_POINT('Ctrl Pts',(3.71280539583414,-1.30000000000064,4.2499861281838));
#50251=CARTESIAN_POINT('Ctrl Pts',(3.66785373478321,-1.18514270861222,4.27984483444986));
#50252=CARTESIAN_POINT('Ctrl Pts',(3.62579800315821,-1.06847604194535,4.30652049503519));
#50253=CARTESIAN_POINT('Ctrl Pts',(3.53533102618688,-0.794772684000865,
4.36079313514626));
#50254=CARTESIAN_POINT('Ctrl Pts',(3.48270660238735,-0.636309800095211,
4.39125278842555));
#50255=CARTESIAN_POINT('Ctrl Pts',(3.4138032523265,-0.319434907277167,4.42014522530414));
#50256=CARTESIAN_POINT('Ctrl Pts',(3.38550575108799,-0.158333333333335,
4.42845155481182));
#50257=CARTESIAN_POINT('Ctrl Pts',(3.36962435074409,0.158333333333338,4.40938186290787));
#50258=CARTESIAN_POINT('Ctrl Pts',(3.38228202234426,0.319434907277171,4.38226570729989));
#50259=CARTESIAN_POINT('Ctrl Pts',(3.4183440412698,0.636309800095218,4.31400035314523));
#50260=CARTESIAN_POINT('Ctrl Pts',(3.45365007369846,0.794772684000861,4.26283591810305));
#50261=CARTESIAN_POINT('Ctrl Pts',(3.51432257080541,1.06847604194562,4.17291021015486));
#50262=CARTESIAN_POINT('Ctrl Pts',(3.54352829849691,1.18514270861276,4.13086142403693));
#50263=CARTESIAN_POINT('Ctrl Pts',(3.57567687801983,1.30000000000144,4.08568935869604));
#50264=CARTESIAN_POINT('Ctrl Pts',(3.73984169575366,-1.30000000000065,4.24369792702482));
#50265=CARTESIAN_POINT('Ctrl Pts',(3.70009029665069,-1.18514270861223,4.27212598516521));
#50266=CARTESIAN_POINT('Ctrl Pts',(3.66168668719453,-1.06847604194536,4.297501336716));
#50267=CARTESIAN_POINT('Ctrl Pts',(3.57608033044364,-0.794772684000877,
4.34907111220608));
#50268=CARTESIAN_POINT('Ctrl Pts',(3.5213729174716,-0.636309800095216,4.37791105023502));
#50269=CARTESIAN_POINT('Ctrl Pts',(3.45173005884871,-0.319434907277168,
4.40528139275286));
#50270=CARTESIAN_POINT('Ctrl Pts',(3.42160585925665,-0.158333333333336,
4.41391300952443));
#50271=CARTESIAN_POINT('Ctrl Pts',(3.40527212173098,0.158333333333338,4.39418531282052));
#50272=CARTESIAN_POINT('Ctrl Pts',(3.41928392621009,0.319434907277173,4.36612106135141));
#50273=CARTESIAN_POINT('Ctrl Pts',(3.45520527900381,0.636309800095221,4.29796580102719));
#50274=CARTESIAN_POINT('Ctrl Pts',(3.49165555094935,0.794772684000865,4.2467799582519));
#50275=CARTESIAN_POINT('Ctrl Pts',(3.5476576245798,1.06847604194563,4.1597157943461));
#50276=CARTESIAN_POINT('Ctrl Pts',(3.57360474182269,1.18514270861277,4.11952920202481));
#50277=CARTESIAN_POINT('Ctrl Pts',(3.60125775371514,1.30000000000145,4.07684286789193));
#50278=CARTESIAN_POINT('Ctrl Pts',(3.77057621024779,-1.30000000000065,4.2379879271015));
#50279=CARTESIAN_POINT('Ctrl Pts',(3.73643249224655,-1.18514270861224,4.2645649472371));
#50280=CARTESIAN_POINT('Ctrl Pts',(3.70200374773516,-1.06847604194536,4.28836838987465));
#50281=CARTESIAN_POINT('Ctrl Pts',(3.62180799220937,-0.794772684000879,
4.33695158535697));
#50282=CARTESIAN_POINT('Ctrl Pts',(3.56524355524324,-0.636309800095217,
4.3647082579409));
#50283=CARTESIAN_POINT('Ctrl Pts',(3.49478613174268,-0.319434907277169,
4.39037576030595));
#50284=CARTESIAN_POINT('Ctrl Pts',(3.46218066956914,-0.158333333333337,
4.39864161599536));
#50285=CARTESIAN_POINT('Ctrl Pts',(3.44541368781495,0.158333333333339,4.37824223121294));
#50286=CARTESIAN_POINT('Ctrl Pts',(3.46130343379324,0.319434907277174,4.34964902787133));
#50287=CARTESIAN_POINT('Ctrl Pts',(3.49750329847094,0.636309800095223,4.28228271306155));
#50288=CARTESIAN_POINT('Ctrl Pts',(3.5358199278298,0.794772684000867,4.23207070452443));
#50289=CARTESIAN_POINT('Ctrl Pts',(3.58639994847023,1.06847604194563,4.14781392326694));
#50290=CARTESIAN_POINT('Ctrl Pts',(3.60841589789106,1.18514270861277,4.10919379097405));
#50291=CARTESIAN_POINT('Ctrl Pts',(3.63055357997191,1.30000000000145,4.06842516497326));
#50292=CARTESIAN_POINT('Ctrl Pts',(3.79462037248655,-1.30000000000065,4.23248904186284));
#50293=CARTESIAN_POINT('Ctrl Pts',(3.76524282283804,-1.18514270861224,4.25807139147591));
#50294=CARTESIAN_POINT('Ctrl Pts',(3.73418925928466,-1.06847604194536,4.28095407868263));
#50295=CARTESIAN_POINT('Ctrl Pts',(3.65857738782657,-0.794772684000879,
4.32758090357173));
#50296=CARTESIAN_POINT('Ctrl Pts',(3.60040457910877,-0.636309800095218,
4.35423587023406));
#50297=CARTESIAN_POINT('Ctrl Pts',(3.52924851154402,-0.31943490727717,4.3784562060816));
#50298=CARTESIAN_POINT('Ctrl Pts',(3.49447968130587,-0.158333333333337,
4.38614777089569));
#50299=CARTESIAN_POINT('Ctrl Pts',(3.47750044519023,0.158333333333339,4.36542754016807));
#50300=CARTESIAN_POINT('Ctrl Pts',(3.49540412812361,0.319434907277176,4.33723169419255));
#50301=CARTESIAN_POINT('Ctrl Pts',(3.53174232357333,0.636309800095225,4.27036586654147));
#50302=CARTESIAN_POINT('Ctrl Pts',(3.57086134674376,0.794772684000868,4.2198267658269));
#50303=CARTESIAN_POINT('Ctrl Pts',(3.61691542379709,1.06847604194563,4.1375276664807));
#50304=CARTESIAN_POINT('Ctrl Pts',(3.6358059254883,1.18514270861278,4.10020016865909));
#50305=CARTESIAN_POINT('Ctrl Pts',(3.65365182538603,1.30000000000146,4.06116940364073));
#50306=CARTESIAN_POINT('Ctrl Pts',(3.82888894787332,-1.30000000000066,4.22716284196521));
#50307=CARTESIAN_POINT('Ctrl Pts',(3.80593264912406,-1.18514270861225,4.25121972230422));
#50308=CARTESIAN_POINT('Ctrl Pts',(3.77943693726649,-1.06847604194537,4.27273352877866));
#50309=CARTESIAN_POINT('Ctrl Pts',(3.71004979008918,-0.794772684000884,
4.31655971618947));
#50310=CARTESIAN_POINT('Ctrl Pts',(3.64977418033061,-0.636309800095223,
4.34181552019614));
#50311=CARTESIAN_POINT('Ctrl Pts',(3.57776768300628,-0.319434907277173,
4.3641282065308));
#50312=CARTESIAN_POINT('Ctrl Pts',(3.54032260485783,-0.158333333333338,
4.37139895676545));
#50313=CARTESIAN_POINT('Ctrl Pts',(3.52276007360683,0.15833333333334,4.34971852351405));
#50314=CARTESIAN_POINT('Ctrl Pts',(3.54254944263255,0.319434907277177,4.32070154415104));
#50315=CARTESIAN_POINT('Ctrl Pts',(3.57897212495849,0.63630980009523,4.25436139779018));
#50316=CARTESIAN_POINT('Ctrl Pts',(3.62013362735884,0.794772684000875,4.20488495138493));
#50317=CARTESIAN_POINT('Ctrl Pts',(3.6598731686715,1.06847604194564,4.12510137464479));
#50318=CARTESIAN_POINT('Ctrl Pts',(3.67423458806077,1.18514270861279,4.08915849505924));
#50319=CARTESIAN_POINT('Ctrl Pts',(3.68575565190016,1.30000000000147,4.05180808998614));
#50320=CARTESIAN_POINT('Ctrl Pts',(3.86578404397843,-1.30000000000068,4.22059393941875));
#50321=CARTESIAN_POINT('Ctrl Pts',(3.84991983243156,-1.18514270861226,4.24316430874856));
#50322=CARTESIAN_POINT('Ctrl Pts',(3.82853115116094,-1.06847604194538,4.26343685622839));
#50323=CARTESIAN_POINT('Ctrl Pts',(3.76635638840658,-0.794772684000894,
4.30496206826487));
#50324=CARTESIAN_POINT('Ctrl Pts',(3.70443753319059,-0.636309800095231,
4.32981945300887));
#50325=CARTESIAN_POINT('Ctrl Pts',(3.63164779125229,-0.319434907277176,
4.35026891636056));
#50326=CARTESIAN_POINT('Ctrl Pts',(3.59069310496552,-0.15833333333334,4.35601525622158));
#50327=CARTESIAN_POINT('Ctrl Pts',(3.57257645100268,0.158333333333342,4.33336461662472));
#50328=CARTESIAN_POINT('Ctrl Pts',(3.59513035178827,0.319434907277182,4.30460139098978));
#50329=CARTESIAN_POINT('Ctrl Pts',(3.63159652953213,0.636309800095238,4.23876022277154));
#50330=CARTESIAN_POINT('Ctrl Pts',(3.67409806878359,0.794772684000883,4.18905821311206));
#50331=CARTESIAN_POINT('Ctrl Pts',(3.70691792339081,1.06847604194565,4.11193558672093));
#50332=CARTESIAN_POINT('Ctrl Pts',(3.71649547878129,1.1851427086128,4.07772509165791));
#50333=CARTESIAN_POINT('Ctrl Pts',(3.72144409059821,1.30000000000149,4.04268762882171));
#50334=CARTESIAN_POINT('Ctrl Pts',(3.90344079132076,-1.3000000000007,4.21553163691707));
#50335=CARTESIAN_POINT('Ctrl Pts',(3.89499337632463,-1.18514270861227,4.23729060012759));
#50336=CARTESIAN_POINT('Ctrl Pts',(3.87886197620791,-1.0684760419454,4.25664495943046));
#50337=CARTESIAN_POINT('Ctrl Pts',(3.8238436720583,-0.794772684000903,4.29580228518037));
#50338=CARTESIAN_POINT('Ctrl Pts',(3.75921741940078,-0.636309800095236,
4.31824524376349));
#50339=CARTESIAN_POINT('Ctrl Pts',(3.68584534308364,-0.319434907277178,
4.33708131683519));
#50340=CARTESIAN_POINT('Ctrl Pts',(3.64266915085392,-0.158333333333342,
4.34349399923061));
#50341=CARTESIAN_POINT('Ctrl Pts',(3.62423560135531,0.158333333333344,4.32027591932134));
#50342=CARTESIAN_POINT('Ctrl Pts',(3.64873452700158,0.319434907277185,4.29042134256727));
#50343=CARTESIAN_POINT('Ctrl Pts',(3.68505522440327,0.636309800095243,4.22474760639587));
#50344=CARTESIAN_POINT('Ctrl Pts',(3.72945278009421,0.794772684000889,4.17570719036836));
#50345=CARTESIAN_POINT('Ctrl Pts',(3.75501039618448,1.06847604194566,4.10063722479461));
#50346=CARTESIAN_POINT('Ctrl Pts',(3.75949108194612,1.18514270861281,4.06762233632771));
#50347=CARTESIAN_POINT('Ctrl Pts',(3.75738950846692,1.3000000000015,4.0340875658745));
#50348=CARTESIAN_POINT('Ctrl Pts',(3.93147377616527,-1.30000000000071,4.21143726929199));
#50349=CARTESIAN_POINT('Ctrl Pts',(3.92840610329863,-1.18514270861229,4.23227712567801));
#50350=CARTESIAN_POINT('Ctrl Pts',(3.9161925755242,-1.06847604194541,4.2509169327825));
#50351=CARTESIAN_POINT('Ctrl Pts',(3.86684812859849,-0.794772684000911,
4.28889606211575));
#50352=CARTESIAN_POINT('Ctrl Pts',(3.80132675731271,-0.636309800095245,
4.3116279899647));
#50353=CARTESIAN_POINT('Ctrl Pts',(3.72756648851605,-0.319434907277184,
4.32934055793407));
#50354=CARTESIAN_POINT('Ctrl Pts',(3.68172597295035,-0.158333333333344,
4.33440289559836));
#50355=CARTESIAN_POINT('Ctrl Pts',(3.66280311231976,0.158333333333346,4.31025692903056));
#50356=CARTESIAN_POINT('Ctrl Pts',(3.68922480229359,0.319434907277191,4.28037607515652));
#50357=CARTESIAN_POINT('Ctrl Pts',(3.7254508113924,0.636309800095254,4.21484984705132));
#50358=CARTESIAN_POINT('Ctrl Pts',(3.77095851021474,0.794772684000901,4.16582082097937));
#50359=CARTESIAN_POINT('Ctrl Pts',(3.79103094672001,1.06847604194568,4.09219956202305));
#50360=CARTESIAN_POINT('Ctrl Pts',(3.79172296786206,1.18514270861283,4.06011405387389));
#50361=CARTESIAN_POINT('Ctrl Pts',(3.78441839614007,1.30000000000152,4.02781095264135));
#50362=CARTESIAN_POINT('Ctrl Pts',(3.95043864767117,-1.30000000000072,4.20925725898497));
#50363=CARTESIAN_POINT('Ctrl Pts',(3.95104583400332,-1.18514270861229,4.22967037753864));
#50364=CARTESIAN_POINT('Ctrl Pts',(3.94147292066165,-1.06847604194541,4.24790093097384));
#50365=CARTESIAN_POINT('Ctrl Pts',(3.89583950901916,-0.794772684000913,
4.28497499437453));
#50366=CARTESIAN_POINT('Ctrl Pts',(3.8293960455156,-0.636309800095246,4.3072798834843));
#50367=CARTESIAN_POINT('Ctrl Pts',(3.75525310382334,-0.319434907277183,
4.32399157087252));
#50368=CARTESIAN_POINT('Ctrl Pts',(3.70766249886697,-0.158333333333344,
4.32817377141168));
#50369=CARTESIAN_POINT('Ctrl Pts',(3.68856395072071,0.158333333333346,4.30367623710034));
#50370=CARTESIAN_POINT('Ctrl Pts',(3.71646988117644,0.319434907277191,4.27417450090621));
#50371=CARTESIAN_POINT('Ctrl Pts',(3.75290435261723,0.636309800095255,4.20923745755768));
#50372=CARTESIAN_POINT('Ctrl Pts',(3.79949284977158,0.794772684000901,4.16080347453736));
#50373=CARTESIAN_POINT('Ctrl Pts',(3.81577447298326,1.06847604194568,4.08790199358733));
#50374=CARTESIAN_POINT('Ctrl Pts',(3.81376017863368,1.18514270861283,4.05611279774224));
#50375=CARTESIAN_POINT('Ctrl Pts',(3.80268387853975,1.30000000000152,4.0240907558893));
#50376=CARTESIAN_POINT('Ctrl Pts',(3.9599652473406,-1.30000000000072,4.2082758133326));
#50377=CARTESIAN_POINT('Ctrl Pts',(3.96247373018997,-1.1851427086123,4.22861432199262));
#50378=CARTESIAN_POINT('Ctrl Pts',(3.95425317231514,-1.06847604194541,4.24670969468615));
#50379=CARTESIAN_POINT('Ctrl Pts',(3.91047580869722,-0.794772684000916,
4.28333153275462));
#50380=CARTESIAN_POINT('Ctrl Pts',(3.84339133338614,-0.636309800095249,
4.30504330605792));
#50381=CARTESIAN_POINT('Ctrl Pts',(3.76908987076134,-0.319434907277185,
4.32129971957743));
#50382=CARTESIAN_POINT('Ctrl Pts',(3.72087714150373,-0.158333333333345,
4.32552144672611));
#50383=CARTESIAN_POINT('Ctrl Pts',(3.70164568823774,0.158333333333347,4.30076892697359));
#50384=CARTESIAN_POINT('Ctrl Pts',(3.7300511581721,0.319434907277193,4.27100751547332));
#50385=CARTESIAN_POINT('Ctrl Pts',(3.76635241068391,0.636309800095258,4.20593539906908));
#50386=CARTESIAN_POINT('Ctrl Pts',(3.81323744935562,0.794772684000906,4.15736982750891));
#50387=CARTESIAN_POINT('Ctrl Pts',(3.82768797731427,1.06847604194568,4.08494046727559));
#50388=CARTESIAN_POINT('Ctrl Pts',(3.8244333521082,1.18514270861283,4.0534985246992));
#50389=CARTESIAN_POINT('Ctrl Pts',(3.81166900358756,1.30000000000153,4.02196662581921));
#50390=CARTESIAN_POINT('Ctrl Pts',(3.96795660160527,-1.30000000000072,4.20756810680955));
#50391=CARTESIAN_POINT('Ctrl Pts',(3.97209954742154,-1.1851427086123,4.22794665512002));
#50392=CARTESIAN_POINT('Ctrl Pts',(3.96503255625194,-1.06847604194542,4.24598437637122));
#50393=CARTESIAN_POINT('Ctrl Pts',(3.92280919592593,-0.794772684000918,
4.28224734210741));
#50394=CARTESIAN_POINT('Ctrl Pts',(3.85508341517208,-0.63630980009525,4.30325616298306));
#50395=CARTESIAN_POINT('Ctrl Pts',(3.78063937085281,-0.319434907277186,
4.31910554794975));
#50396=CARTESIAN_POINT('Ctrl Pts',(3.73196789195621,-0.158333333333345,
4.32346449797966));
#50397=CARTESIAN_POINT('Ctrl Pts',(3.71265745079205,0.158333333333347,4.29855353410026));
#50398=CARTESIAN_POINT('Ctrl Pts',(3.74149078519913,0.319434907277193,4.26859800790141));
#50399=CARTESIAN_POINT('Ctrl Pts',(3.77767574494274,0.636309800095259,4.20340332602937));
#50400=CARTESIAN_POINT('Ctrl Pts',(3.82478841406823,0.794772684000907,4.1546932186604));
#50401=CARTESIAN_POINT('Ctrl Pts',(3.83767602433403,1.06847604194569,4.08258873535245));
#50402=CARTESIAN_POINT('Ctrl Pts',(3.83336792724296,1.18514270861284,4.05139915651908));
#50403=CARTESIAN_POINT('Ctrl Pts',(3.81917316410977,1.30000000000153,4.02023135794197));
#50404=CARTESIAN_POINT('Ctrl Pts',(3.97348957508239,-1.30000000000072,4.20695237207222));
#50405=CARTESIAN_POINT('Ctrl Pts',(3.97871939465724,-1.1851427086123,4.22724269249007));
#50406=CARTESIAN_POINT('Ctrl Pts',(3.97243672548582,-1.06847604194542,4.24519268843738));
#50407=CARTESIAN_POINT('Ctrl Pts',(3.93132635078679,-0.794772684000919,
4.28125415225274));
#50408=CARTESIAN_POINT('Ctrl Pts',(3.86334433943363,-0.63630980009525,4.30215771288401));
#50409=CARTESIAN_POINT('Ctrl Pts',(3.78882281651341,-0.319434907277186,
4.31776997688037));
#50410=CARTESIAN_POINT('Ctrl Pts',(3.73968442782979,-0.158333333333346,
4.3219397055478));
#50411=CARTESIAN_POINT('Ctrl Pts',(3.7203114251934,0.158333333333348,4.29690084080081));
#50412=CARTESIAN_POINT('Ctrl Pts',(3.74952681995744,0.319434907277194,4.2669676940428));
#50413=CARTESIAN_POINT('Ctrl Pts',(3.78570722405296,0.636309800095259,4.20182892840625));
#50414=CARTESIAN_POINT('Ctrl Pts',(3.8330725899664,0.794772684000907,4.15318429705582));
#50415=CARTESIAN_POINT('Ctrl Pts',(3.84483294238354,1.06847604194569,4.08124764646214));
#50416=CARTESIAN_POINT('Ctrl Pts',(3.83973999715607,1.18514270861284,4.0501494404042));
#50417=CARTESIAN_POINT('Ctrl Pts',(3.82446348590374,1.30000000000153,4.01909173881478));
#50418=CARTESIAN_POINT('Ctrl Pts',(3.9762493453264,-1.30000000000072,4.20663124623647));
#50419=CARTESIAN_POINT('Ctrl Pts',(3.98201445584902,-1.1851427086123,4.22686110722728));
#50420=CARTESIAN_POINT('Ctrl Pts',(3.97612075762044,-1.06847604194542,4.24476089668994));
#50421=CARTESIAN_POINT('Ctrl Pts',(3.93557095513018,-0.794772684000919,
4.28073005983005));
#50422=CARTESIAN_POINT('Ctrl Pts',(3.86748860951078,-0.636309800095251,
4.30163715114415));
#50423=CARTESIAN_POINT('Ctrl Pts',(3.79293299943984,-0.319434907277186,
4.31714054172959));
#50424=CARTESIAN_POINT('Ctrl Pts',(3.74354167200372,-0.158333333333346,
4.32117722132424));
#50425=CARTESIAN_POINT('Ctrl Pts',(3.72413832370986,0.158333333333348,4.29607527301169));
#50426=CARTESIAN_POINT('Ctrl Pts',(3.75355646528761,0.319434907277193,4.26617542786185));
#50427=CARTESIAN_POINT('Ctrl Pts',(3.78974957006065,0.636309800095259,4.20109172067779));
#50428=CARTESIAN_POINT('Ctrl Pts',(3.83726280707289,0.794772684000908,4.15251844840692));
#50429=CARTESIAN_POINT('Ctrl Pts',(3.84845325322281,1.06847604194569,4.08065397088516));
#50430=CARTESIAN_POINT('Ctrl Pts',(3.84295812420178,1.18514270861284,4.04958360320056));
#50431=CARTESIAN_POINT('Ctrl Pts',(3.8271239366683,1.30000000000153,4.01855033730926));
#50432=CARTESIAN_POINT('Ctrl Pts',(3.9778242406541,-1.30000000000072,4.20644374584943));
#50433=CARTESIAN_POINT('Ctrl Pts',(3.98389358920159,-1.1851427086123,4.22663572625));
#50434=CARTESIAN_POINT('Ctrl Pts',(3.97822157650232,-1.06847604194542,4.24450561237847));
#50435=CARTESIAN_POINT('Ctrl Pts',(3.93799319915352,-0.794772684000919,
4.28042412189174));
#50436=CARTESIAN_POINT('Ctrl Pts',(3.869860199366,-0.636309800095251,4.30134643422922));
#50437=CARTESIAN_POINT('Ctrl Pts',(3.79528514884846,-0.319434907277186,
4.31678776143938));
#50438=CARTESIAN_POINT('Ctrl Pts',(3.74574263768344,-0.158333333333346,
4.32073550019824));
#50439=CARTESIAN_POINT('Ctrl Pts',(3.72632180662379,0.158333333333348,4.29559714436483));
#50440=CARTESIAN_POINT('Ctrl Pts',(3.75586079346121,0.319434907277193,4.26572593897617));
#50441=CARTESIAN_POINT('Ctrl Pts',(3.792063913688,0.636309800095259,4.20067880511743));
#50442=CARTESIAN_POINT('Ctrl Pts',(3.83966285207613,0.794772684000908,4.15214815192017));
#50443=CARTESIAN_POINT('Ctrl Pts',(3.85052627487336,1.06847604194569,4.08032247938029));
#50444=CARTESIAN_POINT('Ctrl Pts',(3.84479993025133,1.18514270861284,4.04926556481795));
#50445=CARTESIAN_POINT('Ctrl Pts',(3.82864486780783,1.30000000000153,4.01824240793237));
#50446=CARTESIAN_POINT('Ctrl Pts',(3.99120204265725,-1.30000000000072,4.20483258890774));
#50447=CARTESIAN_POINT('Ctrl Pts',(3.99984014572018,-1.18514270861229,4.22466990353234));
#50448=CARTESIAN_POINT('Ctrl Pts',(3.99604541110411,-1.06847604194541,4.24227305966425));
#50449=CARTESIAN_POINT('Ctrl Pts',(3.95855647278786,-0.794772684000913,
4.27777851876826));
#50450=CARTESIAN_POINT('Ctrl Pts',(3.89003289437388,-0.636309800095247,
4.29891255623496));
#50451=CARTESIAN_POINT('Ctrl Pts',(3.81533376908325,-0.319434907277184,
4.31390722216253));
#50452=CARTESIAN_POINT('Ctrl Pts',(3.76454564771665,-0.158333333333345,
4.31717238002423));
#50453=CARTESIAN_POINT('Ctrl Pts',(3.74497402444854,0.158333333333347,4.29171807813497));
#50454=CARTESIAN_POINT('Ctrl Pts',(3.77547356617403,0.319434907277191,4.26196114100903));
#50455=CARTESIAN_POINT('Ctrl Pts',(3.81176709258041,0.636309800095255,4.19723116161557));
#50456=CARTESIAN_POINT('Ctrl Pts',(3.86017384862098,0.794772684000903,4.14921298844651));
#50457=CARTESIAN_POINT('Ctrl Pts',(3.86826533404931,1.06847604194568,4.07772629020409));
#50458=CARTESIAN_POINT('Ctrl Pts',(3.8605627950136,1.18514270861283,4.0467599012596));
#50459=CARTESIAN_POINT('Ctrl Pts',(3.84165521271933,1.30000000000152,4.01577106619662));
#50460=CARTESIAN_POINT('Ctrl Pts',(4.01714771322487,-1.30000000000067,4.20256713842914));
#50461=CARTESIAN_POINT('Ctrl Pts',(4.0310716095307,-1.18514270861225,4.22252983978109));
#50462=CARTESIAN_POINT('Ctrl Pts',(4.03105144551193,-1.06847604194538,4.24002641390433));
#50463=CARTESIAN_POINT('Ctrl Pts',(3.99879129374527,-0.794772684000891,
4.27474975306124));
#50464=CARTESIAN_POINT('Ctrl Pts',(3.92862047411215,-0.636309800095223,
4.29442790699677));
#50465=CARTESIAN_POINT('Ctrl Pts',(3.85351966006039,-0.31943490727717,4.3081931331775));
#50466=CARTESIAN_POINT('Ctrl Pts',(3.80085515946744,-0.158333333333339,
4.31111896123164));
#50467=CARTESIAN_POINT('Ctrl Pts',(3.78103480159934,0.158333333333341,4.28513383912195));
#50468=CARTESIAN_POINT('Ctrl Pts',(3.81329874038641,0.319434907277181,4.25546850313326));
#50469=CARTESIAN_POINT('Ctrl Pts',(3.84920874621917,0.636309800095233,4.19031008381362));
#50470=CARTESIAN_POINT('Ctrl Pts',(3.89790985350236,0.79477268400087,4.14098496371114));
#50471=CARTESIAN_POINT('Ctrl Pts',(3.90097061500278,1.06847604194564,4.07056556841953));
#50472=CARTESIAN_POINT('Ctrl Pts',(3.8899631846853,1.18514270861279,4.04059238554448));
#50473=CARTESIAN_POINT('Ctrl Pts',(3.8666234338092,1.30000000000148,4.01112796672044));
#50474=CARTESIAN_POINT('Ctrl Pts',(4.04264117857254,-1.30000000000062,4.2003111613257));
#50475=CARTESIAN_POINT('Ctrl Pts',(4.06162921508691,-1.1851427086122,4.22015646238016));
#50476=CARTESIAN_POINT('Ctrl Pts',(4.06526201565741,-1.06847604194533,4.23744989519209));
#50477=CARTESIAN_POINT('Ctrl Pts',(4.03818084487976,-0.794772684000851,
4.27150585838726));
#50478=CARTESIAN_POINT('Ctrl Pts',(3.96674475595548,-0.636309800095197,
4.29046137771269));
#50479=CARTESIAN_POINT('Ctrl Pts',(3.891393048032,-0.319434907277159,4.30329173644276));
#50480=CARTESIAN_POINT('Ctrl Pts',(3.83684904087862,-0.158333333333332,
4.3057824152738));
#50481=CARTESIAN_POINT('Ctrl Pts',(3.81670994245089,0.158333333333334,4.27910948726714));
#50482=CARTESIAN_POINT('Ctrl Pts',(3.85032449139865,0.319434907277167,4.24880110464381));
#50483=CARTESIAN_POINT('Ctrl Pts',(3.88626421184786,0.636309800095206,4.18397173792747));
#50484=CARTESIAN_POINT('Ctrl Pts',(3.93674627805647,0.79477268400084,4.13612524101046));
#50485=CARTESIAN_POINT('Ctrl Pts',(3.93451699612749,1.0684760419456,4.06617305577716));
#50486=CARTESIAN_POINT('Ctrl Pts',(3.91970579175569,1.18514270861274,4.0361853699336));
#50487=CARTESIAN_POINT('Ctrl Pts',(3.89104835655611,1.30000000000142,4.00648970725012));
#50488=CARTESIAN_POINT('Ctrl Pts',(4.0555705152568,-1.30000000000062,4.19956202017773));
#50489=CARTESIAN_POINT('Ctrl Pts',(4.07701141444266,-1.1851427086122,4.21920234377182));
#50490=CARTESIAN_POINT('Ctrl Pts',(4.08243023812087,-1.06847604194533,4.23632262916535));
#50491=CARTESIAN_POINT('Ctrl Pts',(4.05793460522167,-0.794772684000851,
4.27005212095055));
#50492=CARTESIAN_POINT('Ctrl Pts',(3.98606842200265,-0.636309800095197,
4.28905845347054));
#50493=CARTESIAN_POINT('Ctrl Pts',(3.91057658300642,-0.319434907277159,
4.3013835706489));
#50494=CARTESIAN_POINT('Ctrl Pts',(3.85489608531509,-0.158333333333332,
4.30323841603954));
#50495=CARTESIAN_POINT('Ctrl Pts',(3.83456187378799,0.158333333333334,4.27613804652562));
#50496=CARTESIAN_POINT('Ctrl Pts',(3.86905149194718,0.319434907277167,4.24590423237741));
#50497=CARTESIAN_POINT('Ctrl Pts',(3.90486897721866,0.636309800095206,4.18098202838765));
#50498=CARTESIAN_POINT('Ctrl Pts',(3.95570286248539,0.79477268400084,4.13287170138419));
#50499=CARTESIAN_POINT('Ctrl Pts',(3.9509321946351,1.0684760419456,4.06330904848038));
#50500=CARTESIAN_POINT('Ctrl Pts',(3.9344049378379,1.18514270861274,4.03363617972609));
#50501=CARTESIAN_POINT('Ctrl Pts',(3.90341546958523,1.30000000000142,4.00440153710932));
#50502=CARTESIAN_POINT('',(3.81821165418158,1.2,4.04980004382707));
#50503=CARTESIAN_POINT('Ctrl Pts',(3.81821165418158,1.2,4.04980004382707));
#50504=CARTESIAN_POINT('Ctrl Pts',(3.79665007582074,1.21683809744007,4.05012443991704));
#50505=CARTESIAN_POINT('Ctrl Pts',(3.77476695290109,1.23326902184029,4.04951335763234));
#50506=CARTESIAN_POINT('Ctrl Pts',(3.72583131966217,1.27112366990156,4.05009292864458));
#50507=CARTESIAN_POINT('Ctrl Pts',(3.7087188599897,1.28439008066975,4.05044181113104));
#50508=CARTESIAN_POINT('Ctrl Pts',(3.68882920344064,1.30000000000147,4.05118449130007));
#50509=CARTESIAN_POINT('',(3.91593537809339,0.653834841369515,4.17213769893144));
#50510=CARTESIAN_POINT('Ctrl Pts',(3.91593537811947,0.653834841368255,4.172137698905));
#50511=CARTESIAN_POINT('Ctrl Pts',(3.90607125701142,0.717394112008443,4.15938042760931));
#50512=CARTESIAN_POINT('Ctrl Pts',(3.89801101167046,0.763835254644307,4.14905065629189));
#50513=CARTESIAN_POINT('Ctrl Pts',(3.86589991141364,0.949861807330393,4.10830966604798));
#50514=CARTESIAN_POINT('Ctrl Pts',(3.84603384758169,1.05921169948484,4.08352203753005));
#50515=CARTESIAN_POINT('Ctrl Pts',(3.81821165418158,1.2,4.04980004382707));
#50516=CARTESIAN_POINT('',(3.99970644341025,-0.653834841531101,4.28369268311062));
#50517=CARTESIAN_POINT('Ctrl Pts',(3.99970644341025,-0.653834841531099,
4.28369268311062));
#50518=CARTESIAN_POINT('Ctrl Pts',(3.9589217428953,-0.575977434761783,4.29176044842603));
#50519=CARTESIAN_POINT('Ctrl Pts',(3.92429750866062,-0.493637200227944,
4.29784498951834));
#50520=CARTESIAN_POINT('Ctrl Pts',(3.87408537207185,-0.338132850880589,
4.30417904451077));
#50521=CARTESIAN_POINT('Ctrl Pts',(3.85622396295216,-0.265656967148426,
4.30518930057354));
#50522=CARTESIAN_POINT('Ctrl Pts',(3.83202315778412,-0.129714373082854,
4.3022669066107));
#50523=CARTESIAN_POINT('Ctrl Pts',(3.82439467993068,-0.0666240349472378,
4.29905620930053));
#50524=CARTESIAN_POINT('Ctrl Pts',(3.81609664033849,0.0595432864754608,
4.28862474620457));
#50525=CARTESIAN_POINT('Ctrl Pts',(3.81535212458621,0.122776486830215,4.28133711266253));
#50526=CARTESIAN_POINT('Ctrl Pts',(3.82182272809368,0.260125347725809,4.26163282896374));
#50527=CARTESIAN_POINT('Ctrl Pts',(3.83051526302472,0.333941089025903,4.24851874359709));
#50528=CARTESIAN_POINT('Ctrl Pts',(3.86114742698447,0.491208851516981,4.2157592661589));
#50529=CARTESIAN_POINT('Ctrl Pts',(3.88506929628498,0.574353773592851,4.19514993653885));
#50530=CARTESIAN_POINT('Ctrl Pts',(3.91593537803789,0.653834841386106,4.17213769891429));
#50531=CARTESIAN_POINT('',(3.95671284637792,-1.2,4.2256221740828));
#50532=CARTESIAN_POINT('Ctrl Pts',(3.95671284637792,-1.2,4.2256221740828));
#50533=CARTESIAN_POINT('Ctrl Pts',(3.96497406598561,-1.12725969986381,4.23661179129406));
#50534=CARTESIAN_POINT('Ctrl Pts',(3.97450006409837,-1.03199076411307,4.24937898084558));
#50535=CARTESIAN_POINT('Ctrl Pts',(3.99271101970977,-0.796651282571319,
4.27409392899359));
#50536=CARTESIAN_POINT('Ctrl Pts',(3.99591651479174,-0.739855008065579,
4.27849480776061));
#50537=CARTESIAN_POINT('Ctrl Pts',(3.99970644341025,-0.653834841531101,
4.28369268311062));
#50538=CARTESIAN_POINT('Ctrl Pts',(3.83160559603087,-1.30000000000066,4.22656788265504));
#50539=CARTESIAN_POINT('Ctrl Pts',(3.85268755687877,-1.28300366105782,4.22601146009439));
#50540=CARTESIAN_POINT('Ctrl Pts',(3.87378621355538,-1.26602077773898,4.22557624381621));
#50541=CARTESIAN_POINT('Ctrl Pts',(3.92099711546401,-1.2283719856465,4.2253654510458));
#50542=CARTESIAN_POINT('Ctrl Pts',(3.93742292581801,-1.21501533405422,4.22495017710272));
#50543=CARTESIAN_POINT('Ctrl Pts',(3.95671284637792,-1.2,4.2256221740828));
#50544=CARTESIAN_POINT('Origin',(0.,1.25,7.2));
#50545=CARTESIAN_POINT('Origin',(0.,1.2,7.2));
#50546=CARTESIAN_POINT('Origin',(0.,0.92691742076555,7.2));
#50547=CARTESIAN_POINT('Origin',(0.,0.653834841531101,7.2));
#50548=CARTESIAN_POINT('Origin',(0.,0.,7.2));
#50549=CARTESIAN_POINT('Origin',(0.,-0.653834841531101,7.2));
#50550=CARTESIAN_POINT('Origin',(0.,-0.926917420765551,7.2));
#50551=CARTESIAN_POINT('Origin',(0.,-1.2,7.2));
#50552=CARTESIAN_POINT('Origin',(0.,-1.25,7.2));
#50553=CARTESIAN_POINT('Ctrl Pts',(4.24541645780685,-1.30000000000147,4.47512551407364));
#50554=CARTESIAN_POINT('Ctrl Pts',(4.22718893278279,-1.18514270861278,4.43661877696157));
#50555=CARTESIAN_POINT('Ctrl Pts',(4.2040755608183,-1.06847604194562,4.41173100097083));
#50556=CARTESIAN_POINT('Ctrl Pts',(4.13939176392353,-0.794772684000851,
4.38569778430383));
#50557=CARTESIAN_POINT('Ctrl Pts',(4.07792758948489,-0.636309800095197,
4.41917677348839));
#50558=CARTESIAN_POINT('Ctrl Pts',(4.00511469268244,-0.319434907277159,
4.43317916190871));
#50559=CARTESIAN_POINT('Ctrl Pts',(3.96570274858467,-0.158333333333332,
4.45663797562632));
#50560=CARTESIAN_POINT('Ctrl Pts',(3.94621238249364,0.158333333333334,4.42892451651608));
#50561=CARTESIAN_POINT('Ctrl Pts',(3.96518266533146,0.319434907277167,4.3765423951036));
#50562=CARTESIAN_POINT('Ctrl Pts',(4.00023280952294,0.636309800095206,4.3085540603659));
#50563=CARTESIAN_POINT('Ctrl Pts',(4.04051677784848,0.79477268400084,4.2460785382662));
#50564=CARTESIAN_POINT('Ctrl Pts',(4.08016499765644,1.06847604194569,4.23320479314945));
#50565=CARTESIAN_POINT('Ctrl Pts',(4.09477284803596,1.18514270861292,4.24364885985363));
#50566=CARTESIAN_POINT('Ctrl Pts',(4.10682630355144,1.30000000000169,4.27010956050376));
#50567=CARTESIAN_POINT('Ctrl Pts',(4.23960884193275,-1.30000000000147,4.48624205742122));
#50568=CARTESIAN_POINT('Ctrl Pts',(4.22022222294608,-1.18514270861278,4.44981075249239));
#50569=CARTESIAN_POINT('Ctrl Pts',(4.19627915278588,-1.06847604194562,4.42645775550554));
#50570=CARTESIAN_POINT('Ctrl Pts',(4.1304395571954,-0.794772684000851,4.40272116836744));
#50571=CARTESIAN_POINT('Ctrl Pts',(4.06933501810858,-0.636309800095197,
4.43594708574808));
#50572=CARTESIAN_POINT('Ctrl Pts',(3.99657264203947,-0.319434907277159,
4.45009441503412));
#50573=CARTESIAN_POINT('Ctrl Pts',(3.95736019037403,-0.158333333333332,
4.4726979455451));
#50574=CARTESIAN_POINT('Ctrl Pts',(3.9382160520501,0.158333333333334,4.44530213670932));
#50575=CARTESIAN_POINT('Ctrl Pts',(3.95743985353982,0.319434907277165,4.39419736536322));
#50576=CARTESIAN_POINT('Ctrl Pts',(3.992927208102,0.636309800095204,4.32649843143128));
#50577=CARTESIAN_POINT('Ctrl Pts',(4.03302994372149,0.794772684000841,4.26441625119816));
#50578=CARTESIAN_POINT('Ctrl Pts',(4.07378763143588,1.06847604194569,4.24918439864749));
#50579=CARTESIAN_POINT('Ctrl Pts',(4.08911206629833,1.18514270861292,4.25798336192542));
#50580=CARTESIAN_POINT('Ctrl Pts',(4.10211844323279,1.30000000000169,4.28217459305472));
#50581=CARTESIAN_POINT('Ctrl Pts',(4.22767543402957,-1.30000000000147,4.50806909203799));
#50582=CARTESIAN_POINT('Ctrl Pts',(4.20687971577468,-1.18514270861278,4.47678576931432));
#50583=CARTESIAN_POINT('Ctrl Pts',(4.18178147215414,-1.06847604194562,4.45706455756511));
#50584=CARTESIAN_POINT('Ctrl Pts',(4.11385981419251,-0.794772684000849,
4.43821540255297));
#50585=CARTESIAN_POINT('Ctrl Pts',(4.05186292446327,-0.636309800095195,
4.46924991849888));
#50586=CARTESIAN_POINT('Ctrl Pts',(3.97878311668032,-0.319434907277158,
4.48325358835845));
#50587=CARTESIAN_POINT('Ctrl Pts',(3.94060084469131,-0.158333333333332,
4.50477443631655));
#50588=CARTESIAN_POINT('Ctrl Pts',(3.92202810261724,0.158333333333334,4.47791014713781));
#50589=CARTESIAN_POINT('Ctrl Pts',(3.94113066143261,0.319434907277165,4.42877203439641));
#50590=CARTESIAN_POINT('Ctrl Pts',(3.97741179451921,0.636309800095203,4.36158149886323));
#50591=CARTESIAN_POINT('Ctrl Pts',(4.01772483256587,0.794772684000838,4.30084139570613));
#50592=CARTESIAN_POINT('Ctrl Pts',(4.06070253778891,1.06847604194569,4.28086982070652));
#50593=CARTESIAN_POINT('Ctrl Pts',(4.07735759975927,1.18514270861292,4.28626233727591));
#50594=CARTESIAN_POINT('Ctrl Pts',(4.0920642675898,1.30000000000169,4.30569232521228));
#50595=CARTESIAN_POINT('Ctrl Pts',(4.21536537138849,-1.30000000000148,4.53073018436133));
#50596=CARTESIAN_POINT('Ctrl Pts',(4.19171379454328,-1.18514270861278,4.50325264395899));
#50597=CARTESIAN_POINT('Ctrl Pts',(4.16462606938504,-1.06847604194563,4.48641597238428));
#50598=CARTESIAN_POINT('Ctrl Pts',(4.0941098153866,-0.794772684000856,4.47210242857244));
#50599=CARTESIAN_POINT('Ctrl Pts',(4.03346761141163,-0.636309800095198,
4.50326462824729));
#50600=CARTESIAN_POINT('Ctrl Pts',(3.96071008590311,-0.319434907277159,
4.51780391381332));
#50601=CARTESIAN_POINT('Ctrl Pts',(3.92306324501872,-0.158333333333333,
4.53766562651771));
#50602=CARTESIAN_POINT('Ctrl Pts',(3.90488012894027,0.158333333333334,4.51116354761295));
#50603=CARTESIAN_POINT('Ctrl Pts',(3.92354863114418,0.319434907277167,4.46376917352988));
#50604=CARTESIAN_POINT('Ctrl Pts',(3.96088826961113,0.636309800095206,4.39734628374278));
#50605=CARTESIAN_POINT('Ctrl Pts',(4.00230037561805,0.794772684000841,4.33885835941129));
#50606=CARTESIAN_POINT('Ctrl Pts',(4.04766438094242,1.06847604194569,4.31407344698293));
#50607=CARTESIAN_POINT('Ctrl Pts',(4.06555992346895,1.18514270861292,4.31580908798941));
#50608=CARTESIAN_POINT('Ctrl Pts',(4.08171461151912,1.30000000000169,4.33000884022113));
#50609=CARTESIAN_POINT('Ctrl Pts',(4.2085808450133,-1.30000000000148,4.54298047372179));
#50610=CARTESIAN_POINT('Ctrl Pts',(4.18398441102912,-1.18514270861278,4.51825502561577));
#50611=CARTESIAN_POINT('Ctrl Pts',(4.15615495420865,-1.06847604194563,4.50337578034686));
#50612=CARTESIAN_POINT('Ctrl Pts',(4.08439441217396,-0.794772684000854,
4.4917484454727));
#50613=CARTESIAN_POINT('Ctrl Pts',(4.02353939608196,-0.636309800095197,
4.5219690142106));
#50614=CARTESIAN_POINT('Ctrl Pts',(3.9504823383192,-0.319434907277158,4.53630419925681));
#50615=CARTESIAN_POINT('Ctrl Pts',(3.91297617665875,-0.158333333333332,
4.55510202742408));
#50616=CARTESIAN_POINT('Ctrl Pts',(3.89506471881218,0.158333333333334,4.5288581595896));
#50617=CARTESIAN_POINT('Ctrl Pts',(3.91406984960906,0.319434907277167,4.48299886281169));
#50618=CARTESIAN_POINT('Ctrl Pts',(3.95184347519112,0.636309800095206,4.41687220251966));
#50619=CARTESIAN_POINT('Ctrl Pts',(3.99290223892469,0.79477268400084,4.35869637636772));
#50620=CARTESIAN_POINT('Ctrl Pts',(4.03958051780275,1.06847604194569,4.33128930588467));
#50621=CARTESIAN_POINT('Ctrl Pts',(4.05836014539548,1.18514270861292,4.33122248868109));
#50622=CARTESIAN_POINT('Ctrl Pts',(4.07571410325526,1.30000000000169,4.34295235955402));
#50623=CARTESIAN_POINT('Ctrl Pts',(4.20704609201274,-1.30000000000148,4.54567370393651));
#50624=CARTESIAN_POINT('Ctrl Pts',(4.18222266565875,-1.18514270861278,4.52154229127531));
#50625=CARTESIAN_POINT('Ctrl Pts',(4.15421915538174,-1.06847604194563,4.50708863765698));
#50626=CARTESIAN_POINT('Ctrl Pts',(4.08217881452316,-0.794772684000854,
4.49605536577328));
#50627=CARTESIAN_POINT('Ctrl Pts',(4.02130604660735,-0.636309800095197,
4.52609789071604));
#50628=CARTESIAN_POINT('Ctrl Pts',(3.94819597380128,-0.319434907277158,
4.54040245096397));
#50629=CARTESIAN_POINT('Ctrl Pts',(3.91072278825904,-0.158333333333332,
4.55896581463651));
#50630=CARTESIAN_POINT('Ctrl Pts',(3.89286905623125,0.158333333333334,4.53277722495117));
#50631=CARTESIAN_POINT('Ctrl Pts',(3.91192915619521,0.319434907277167,4.48723963284581));
#50632=CARTESIAN_POINT('Ctrl Pts',(3.94981182527956,0.636309800095205,4.4211910906106));
#50633=CARTESIAN_POINT('Ctrl Pts',(3.99083691129868,0.794772684000839,4.36312830796479));
#50634=CARTESIAN_POINT('Ctrl Pts',(4.03781437771274,1.06847604194569,4.33514525823157));
#50635=CARTESIAN_POINT('Ctrl Pts',(4.05678516999129,1.18514270861292,4.33467258717553));
#50636=CARTESIAN_POINT('Ctrl Pts',(4.07439195002436,1.30000000000169,4.34584007041882));
#50637=CARTESIAN_POINT('Ctrl Pts',(4.20433936154425,-1.30000000000147,4.55036564872492));
#50638=CARTESIAN_POINT('Ctrl Pts',(4.17908965394546,-1.18514270861278,4.52724270221372));
#50639=CARTESIAN_POINT('Ctrl Pts',(4.15076399214117,-1.06847604194563,4.51351508747843));
#50640=CARTESIAN_POINT('Ctrl Pts',(4.07821997728699,-0.794772684000854,
4.50350664717199));
#50641=CARTESIAN_POINT('Ctrl Pts',(4.01734734138685,-0.636309800095197,
4.53327162429178));
#50642=CARTESIAN_POINT('Ctrl Pts',(3.94416815826401,-0.319434907277158,
4.54754774675137));
#50643=CARTESIAN_POINT('Ctrl Pts',(3.90677716273327,-0.158333333333332,
4.5657256039145));
#50644=CARTESIAN_POINT('Ctrl Pts',(3.88902354607648,0.158333333333334,4.53963347110758));
#50645=CARTESIAN_POINT('Ctrl Pts',(3.90813695298707,0.319434907277167,4.49461618985308));
#50646=CARTESIAN_POINT('Ctrl Pts',(3.94622059044497,0.636309800095206,4.42871445010138));
#50647=CARTESIAN_POINT('Ctrl Pts',(3.98724992174037,0.794772684000839,4.37091224759782));
#50648=CARTESIAN_POINT('Ctrl Pts',(4.03475881967035,1.06847604194569,4.34192866799764));
#50649=CARTESIAN_POINT('Ctrl Pts',(4.05405600820849,1.18514270861292,4.34073742432239));
#50650=CARTESIAN_POINT('Ctrl Pts',(4.07208554374899,1.30000000000169,4.35090085463336));
#50651=CARTESIAN_POINT('Ctrl Pts',(4.19873267755499,-1.30000000000147,4.55955506317463));
#50652=CARTESIAN_POINT('Ctrl Pts',(4.17231133494234,-1.18514270861278,4.53810655307788));
#50653=CARTESIAN_POINT('Ctrl Pts',(4.14315429278747,-1.06847604194562,4.52563026012046));
#50654=CARTESIAN_POINT('Ctrl Pts',(4.06947567934627,-0.794772684000854,
4.51753514399271));
#50655=CARTESIAN_POINT('Ctrl Pts',(4.00896929670049,-0.636309800095196,
4.54714109090363));
#50656=CARTESIAN_POINT('Ctrl Pts',(3.93598472360625,-0.319434907277158,
4.56171241723378));
#50657=CARTESIAN_POINT('Ctrl Pts',(3.89913110815116,-0.158333333333332,
4.57950311275997));
#50658=CARTESIAN_POINT('Ctrl Pts',(3.88156910106732,0.158333333333334,4.55360146623094));
#50659=CARTESIAN_POINT('Ctrl Pts',(3.90019959247597,0.319434907277167,4.50903198651371));
#50660=CARTESIAN_POINT('Ctrl Pts',(3.93875826929773,0.636309800095205,4.44348753744588));
#50661=CARTESIAN_POINT('Ctrl Pts',(3.98052794628395,0.794772684000839,4.3869195618298));
#50662=CARTESIAN_POINT('Ctrl Pts',(4.02920242948869,1.06847604194569,4.35603670625649));
#50663=CARTESIAN_POINT('Ctrl Pts',(4.04907016256394,1.18514270861292,4.35333003563285));
#50664=CARTESIAN_POINT('Ctrl Pts',(4.06773624850241,1.30000000000169,4.36128473824072));
#50665=CARTESIAN_POINT('Ctrl Pts',(4.19093136889261,-1.30000000000147,4.57290821024422));
#50666=CARTESIAN_POINT('Ctrl Pts',(4.16313154427205,-1.18514270861278,4.55417304171649));
#50667=CARTESIAN_POINT('Ctrl Pts',(4.13293331447271,-1.06847604194562,4.54364432926449));
#50668=CARTESIAN_POINT('Ctrl Pts',(4.05762856673893,-0.79477268400085,4.53827945246952));
#50669=CARTESIAN_POINT('Ctrl Pts',(3.99713251667256,-0.636309800095196,
4.56709991584869));
#50670=CARTESIAN_POINT('Ctrl Pts',(3.92391655521161,-0.319434907277159,
4.58155092634557));
#50671=CARTESIAN_POINT('Ctrl Pts',(3.8873086612351,-0.158333333333332,4.59824238789949));
#50672=CARTESIAN_POINT('Ctrl Pts',(3.87005884656604,0.158333333333334,4.57265595866863));
#50673=CARTESIAN_POINT('Ctrl Pts',(3.88886394919438,0.319434907277168,4.52962487744537));
#50674=CARTESIAN_POINT('Ctrl Pts',(3.92806965388208,0.636309800095206,4.46459034758097));
#50675=CARTESIAN_POINT('Ctrl Pts',(3.96991258425277,0.794772684000838,4.40882972731653));
#50676=CARTESIAN_POINT('Ctrl Pts',(4.02019691836951,1.06847604194569,4.37517252189455));
#50677=CARTESIAN_POINT('Ctrl Pts',(4.04103788752713,1.18514270861292,4.37044670215731));
#50678=CARTESIAN_POINT('Ctrl Pts',(4.0609536008214,1.3000000000017,4.37556401978768));
#50679=CARTESIAN_POINT('Ctrl Pts',(4.18172242510089,-1.30000000000147,4.58911913974467));
#50680=CARTESIAN_POINT('Ctrl Pts',(4.15242075783392,-1.18514270861278,4.57381508171145));
#50681=CARTESIAN_POINT('Ctrl Pts',(4.12106825076219,-1.06847604194562,4.56573360478442));
#50682=CARTESIAN_POINT('Ctrl Pts',(4.04389983716102,-0.794772684000853,
4.56374938361677));
#50683=CARTESIAN_POINT('Ctrl Pts',(3.98329099744489,-0.636309800095197,
4.59148869754783));
#50684=CARTESIAN_POINT('Ctrl Pts',(3.90966015561019,-0.319434907277159,
4.60564290670402));
#50685=CARTESIAN_POINT('Ctrl Pts',(3.87321187328493,-0.158333333333333,
4.6208588406351));
#50686=CARTESIAN_POINT('Ctrl Pts',(3.85621823674316,0.158333333333335,4.59552323915029));
#50687=CARTESIAN_POINT('Ctrl Pts',(3.87517408213286,0.319434907277169,4.55428904304731));
#50688=CARTESIAN_POINT('Ctrl Pts',(3.91520613040173,0.636309800095208,4.48991856855682));
#50689=CARTESIAN_POINT('Ctrl Pts',(3.95728363671029,0.79477268400084,4.43527185629106));
#50690=CARTESIAN_POINT('Ctrl Pts',(4.00964742619141,1.06847604194569,4.39843438524851));
#50691=CARTESIAN_POINT('Ctrl Pts',(4.03171928662598,1.18514270861292,4.39134954378234));
#50692=CARTESIAN_POINT('Ctrl Pts',(4.0531966632983,1.3000000000017,4.39312543710154));
#50693=CARTESIAN_POINT('Ctrl Pts',(4.16880507082559,-1.30000000000147,4.61004578002529));
#50694=CARTESIAN_POINT('Ctrl Pts',(4.13696503396582,-1.18514270861278,4.59874349674725));
#50695=CARTESIAN_POINT('Ctrl Pts',(4.10371802628018,-1.06847604194562,4.59354496739133));
#50696=CARTESIAN_POINT('Ctrl Pts',(4.02366040341415,-0.794772684000849,
4.59563621722879));
#50697=CARTESIAN_POINT('Ctrl Pts',(3.96311397001787,-0.636309800095195,
4.62215678944795));
#50698=CARTESIAN_POINT('Ctrl Pts',(3.88943653601152,-0.319434907277158,
4.63646741409111));
#50699=CARTESIAN_POINT('Ctrl Pts',(3.85397611191893,-0.158333333333332,
4.65056016494006));
#50700=CARTESIAN_POINT('Ctrl Pts',(3.83775883998639,0.158333333333334,4.62604196448687));
#50701=CARTESIAN_POINT('Ctrl Pts',(3.85692018103754,0.319434907277168,4.58720679960908));
#50702=CARTESIAN_POINT('Ctrl Pts',(3.89773084313788,0.636309800095206,4.5234110729215));
#50703=CARTESIAN_POINT('Ctrl Pts',(3.93934209301345,0.794772684000837,4.46948746060851));
#50704=CARTESIAN_POINT('Ctrl Pts',(3.99424963300068,1.06847604194569,4.42815357346725));
#50705=CARTESIAN_POINT('Ctrl Pts',(4.01799642861208,1.18514270861292,4.41793482658671));
#50706=CARTESIAN_POINT('Ctrl Pts',(4.04172258029922,1.30000000000169,4.41538924099766));
#50707=CARTESIAN_POINT('Ctrl Pts',(4.15604312001451,-1.30000000000148,4.63118777585926));
#50708=CARTESIAN_POINT('Ctrl Pts',(4.1216791626411,-1.18514270861278,4.62390281465639));
#50709=CARTESIAN_POINT('Ctrl Pts',(4.08658988648999,-1.06847604194563,4.62164593015606));
#50710=CARTESIAN_POINT('Ctrl Pts',(4.00385100751946,-0.794772684000854,
4.62804793851824));
#50711=CARTESIAN_POINT('Ctrl Pts',(3.94383336495263,-0.636309800095198,
4.65387812734365));
#50712=CARTESIAN_POINT('Ctrl Pts',(3.87003875709904,-0.319434907277159,
4.66826804374778));
#50713=CARTESIAN_POINT('Ctrl Pts',(3.8352167054639,-0.158333333333332,4.68082503182623));
#50714=CARTESIAN_POINT('Ctrl Pts',(3.81911560801986,0.158333333333334,4.65642088163312));
#50715=CARTESIAN_POINT('Ctrl Pts',(3.83758219438638,0.319434907277165,4.6190667059095));
#50716=CARTESIAN_POINT('Ctrl Pts',(3.87909815500753,0.636309800095204,4.5557678817093));
#50717=CARTESIAN_POINT('Ctrl Pts',(3.92109800041264,0.79477268400084,4.50344432729588));
#50718=CARTESIAN_POINT('Ctrl Pts',(3.97910646526714,1.06847604194569,4.45819029969242));
#50719=CARTESIAN_POINT('Ctrl Pts',(4.00473334786608,1.18514270861292,4.44505142981327));
#50720=CARTESIAN_POINT('Ctrl Pts',(4.03087739805383,1.30000000000169,4.43836248177756));
#50721=CARTESIAN_POINT('Ctrl Pts',(4.14297610782065,-1.30000000000148,4.65198541354976));
#50722=CARTESIAN_POINT('Ctrl Pts',(4.10620291401802,-1.18514270861278,4.64887574315513));
#50723=CARTESIAN_POINT('Ctrl Pts',(4.06921033438157,-1.06847604194563,4.64951097508102));
#50724=CARTESIAN_POINT('Ctrl Pts',(3.98324324991729,-0.794772684000855,
4.65962996143306));
#50725=CARTESIAN_POINT('Ctrl Pts',(3.92236141661275,-0.636309800095197,
4.68317313228162));
#50726=CARTESIAN_POINT('Ctrl Pts',(3.84818966802474,-0.319434907277158,
4.69735660219927));
#50727=CARTESIAN_POINT('Ctrl Pts',(3.81474932380975,-0.158333333333332,
4.7092392649545));
#50728=CARTESIAN_POINT('Ctrl Pts',(3.79944294976693,0.158333333333334,4.685720309876));
#50729=CARTESIAN_POINT('Ctrl Pts',(3.81766613437042,0.319434907277167,4.65034974776563));
#50730=CARTESIAN_POINT('Ctrl Pts',(3.86047817775576,0.636309800095206,4.58819660150164));
#50731=CARTESIAN_POINT('Ctrl Pts',(3.9033754919168,0.79477268400084,4.53801363871568));
#50732=CARTESIAN_POINT('Ctrl Pts',(3.96424901291745,1.06847604194569,4.48857485447331));
#50733=CARTESIAN_POINT('Ctrl Pts',(3.9914447211426,1.18514270861292,4.47217394456677));
#50734=CARTESIAN_POINT('Ctrl Pts',(4.01948624593792,1.30000000000169,4.46077234256479));
#50735=CARTESIAN_POINT('Ctrl Pts',(4.1331323253172,-1.30000000000148,4.66758769368662));
#50736=CARTESIAN_POINT('Ctrl Pts',(4.09395398214409,-1.18514270861279,4.66691172061687));
#50737=CARTESIAN_POINT('Ctrl Pts',(4.05529296241795,-1.06847604194563,4.66943087663154));
#50738=CARTESIAN_POINT('Ctrl Pts',(3.96717339339293,-0.794772684000856,
4.68263201834918));
#50739=CARTESIAN_POINT('Ctrl Pts',(3.90768874347606,-0.636309800095198,
4.70680805472394));
#50740=CARTESIAN_POINT('Ctrl Pts',(3.83342912388408,-0.319434907277158,
4.72105415210319));
#50741=CARTESIAN_POINT('Ctrl Pts',(3.79971225905942,-0.158333333333332,
4.73091072894089));
#50742=CARTESIAN_POINT('Ctrl Pts',(3.7842917854581,0.158333333333334,4.70725691348332));
#50743=CARTESIAN_POINT('Ctrl Pts',(3.80243447904911,0.319434907277167,4.67350146574777));
#50744=CARTESIAN_POINT('Ctrl Pts',(3.84559677523662,0.636309800095206,4.61157340969996));
#50745=CARTESIAN_POINT('Ctrl Pts',(3.88795953460117,0.794772684000839,4.56176937733571));
#50746=CARTESIAN_POINT('Ctrl Pts',(3.95131713811071,1.06847604194569,4.50955132448505));
#50747=CARTESIAN_POINT('Ctrl Pts',(3.98020441701305,1.18514270861292,4.49123939964216));
#50748=CARTESIAN_POINT('Ctrl Pts',(4.01055381588896,1.3000000000017,4.47721881016595));
#50749=CARTESIAN_POINT('Ctrl Pts',(4.12254789803899,-1.30000000000148,4.68226017949022));
#50750=CARTESIAN_POINT('Ctrl Pts',(4.08162160927235,-1.18514270861279,4.68481381781336));
#50751=CARTESIAN_POINT('Ctrl Pts',(4.04154893072778,-1.06847604194563,4.6895395859463));
#50752=CARTESIAN_POINT('Ctrl Pts',(3.95094503715524,-0.794772684000856,
4.70547511011371));
#50753=CARTESIAN_POINT('Ctrl Pts',(3.89055896161236,-0.636309800095199,
4.72761125572642));
#50754=CARTESIAN_POINT('Ctrl Pts',(3.81593662704533,-0.319434907277159,
4.7416081001466));
#50755=CARTESIAN_POINT('Ctrl Pts',(3.78316485350851,-0.158333333333333,
4.75086331769791));
#50756=CARTESIAN_POINT('Ctrl Pts',(3.76875250647682,0.158333333333335,4.72836052237739));
#50757=CARTESIAN_POINT('Ctrl Pts',(3.78748461749782,0.319434907277168,4.69699270366139));
#50758=CARTESIAN_POINT('Ctrl Pts',(3.83199090736013,0.636309800095208,4.63636448802781));
#50759=CARTESIAN_POINT('Ctrl Pts',(3.87485052625608,0.794772684000842,4.58796986865435));
#50760=CARTESIAN_POINT('Ctrl Pts',(3.94017354152225,1.06847604194569,4.5324020847612));
#50761=CARTESIAN_POINT('Ctrl Pts',(3.97011512822077,1.18514270861293,4.51150022929617));
#50762=CARTESIAN_POINT('Ctrl Pts',(4.00172238876529,1.3000000000017,4.49374975302422));
#50763=CARTESIAN_POINT('Ctrl Pts',(4.11277136635694,-1.30000000000148,4.69795681868002));
#50764=CARTESIAN_POINT('Ctrl Pts',(4.06972341382925,-1.18514270861279,4.70328683022413));
#50765=CARTESIAN_POINT('Ctrl Pts',(4.02807427462076,-1.06847604194563,4.71001290352959));
#50766=CARTESIAN_POINT('Ctrl Pts',(3.93508796976659,-0.794772684000856,
4.72877666036137));
#50767=CARTESIAN_POINT('Ctrl Pts',(3.87492859356411,-0.636309800095199,
4.75018115722892));
#50768=CARTESIAN_POINT('Ctrl Pts',(3.80006801748132,-0.319434907277159,
4.76406600863756));
#50769=CARTESIAN_POINT('Ctrl Pts',(3.7679477891152,-0.158333333333333,4.77236034151488));
#50770=CARTESIAN_POINT('Ctrl Pts',(3.75340490428175,0.158333333333335,4.7497246578718));
#50771=CARTESIAN_POINT('Ctrl Pts',(3.77112410984858,0.319434907277167,4.71894684138089));
#50772=CARTESIAN_POINT('Ctrl Pts',(3.81607291389888,0.636309800095207,4.65864471171329));
#50773=CARTESIAN_POINT('Ctrl Pts',(3.85938745500052,0.794772684000843,4.61170848166047));
#50774=CARTESIAN_POINT('Ctrl Pts',(3.92757055983804,1.06847604194569,4.55376900664564));
#50775=CARTESIAN_POINT('Ctrl Pts',(3.95924803712011,1.18514270861292,4.53100273925647));
#50776=CARTESIAN_POINT('Ctrl Pts',(3.99308905203305,1.30000000000169,4.51055005634297));
#50777=CARTESIAN_POINT('Ctrl Pts',(4.101856528153,-1.30000000000148,4.7122711116332));
#50778=CARTESIAN_POINT('Ctrl Pts',(4.05659542579174,-1.18514270861279,4.72028838079266));
#50779=CARTESIAN_POINT('Ctrl Pts',(4.01331820273123,-1.06847604194563,4.72896882822391));
#50780=CARTESIAN_POINT('Ctrl Pts',(3.91792231794129,-0.794772684000857,
4.75055447278382));
#50781=CARTESIAN_POINT('Ctrl Pts',(3.85817109968514,-0.6363098000952,4.77144910042573));
#50782=CARTESIAN_POINT('Ctrl Pts',(3.78305855782865,-0.31943490727716,4.78520903031956));
#50783=CARTESIAN_POINT('Ctrl Pts',(3.75116081181364,-0.158333333333333,
4.79202927430626));
#50784=CARTESIAN_POINT('Ctrl Pts',(3.73698370523568,0.158333333333335,4.76983140310512));
#50785=CARTESIAN_POINT('Ctrl Pts',(3.75484510432218,0.319434907277169,4.74098689183149));
#50786=CARTESIAN_POINT('Ctrl Pts',(3.80079318359405,0.636309800095209,4.68165787792731));
#50787=CARTESIAN_POINT('Ctrl Pts',(3.84450273988808,0.794772684000844,4.63609370377142));
#50788=CARTESIAN_POINT('Ctrl Pts',(3.9150270820872,1.0684760419457,4.5752130454864));
#50789=CARTESIAN_POINT('Ctrl Pts',(3.9480581762961,1.18514270861293,4.55016322717855));
#50790=CARTESIAN_POINT('Ctrl Pts',(3.98359299016023,1.3000000000017,4.52641657168378));
#50791=CARTESIAN_POINT('Ctrl Pts',(4.08853169252917,-1.30000000000148,4.73287853781556));
#50792=CARTESIAN_POINT('Ctrl Pts',(4.0404930763511,-1.18514270861278,4.74467643615338));
#50793=CARTESIAN_POINT('Ctrl Pts',(3.99507502628155,-1.06847604194563,4.75599153237031));
#50794=CARTESIAN_POINT('Ctrl Pts',(3.8962042767245,-0.794772684000854,4.78101629872514));
#50795=CARTESIAN_POINT('Ctrl Pts',(3.83610607894287,-0.636309800095199,
4.80017074373498));
#50796=CARTESIAN_POINT('Ctrl Pts',(3.76037354956376,-0.31943490727716,4.8134188260809));
#50797=CARTESIAN_POINT('Ctrl Pts',(3.7292573865684,-0.158333333333333,4.81883751778385));
#50798=CARTESIAN_POINT('Ctrl Pts',(3.71543660868739,0.158333333333335,4.79707715292213));
#50799=CARTESIAN_POINT('Ctrl Pts',(3.73301950557419,0.319434907277167,4.77027969434264));
#50800=CARTESIAN_POINT('Ctrl Pts',(3.78001446475977,0.636309800095207,4.71193002795179));
#50801=CARTESIAN_POINT('Ctrl Pts',(3.82401597092546,0.794772684000843,4.66795096043174));
#50802=CARTESIAN_POINT('Ctrl Pts',(3.89804389930781,1.06847604194569,4.60356088594938));
#50803=CARTESIAN_POINT('Ctrl Pts',(3.93320306627985,1.18514270861293,4.57581440871316));
#50804=CARTESIAN_POINT('Ctrl Pts',(3.97147745303223,1.3000000000017,4.54819353159681));
#50805=CARTESIAN_POINT('Ctrl Pts',(4.07049950580579,-1.30000000000147,4.75697072422884));
#50806=CARTESIAN_POINT('Ctrl Pts',(4.01840400164301,-1.18514270861278,4.77278304834912));
#50807=CARTESIAN_POINT('Ctrl Pts',(3.96997511063938,-1.06847604194562,4.78697882013429));
#50808=CARTESIAN_POINT('Ctrl Pts',(3.86656529415587,-0.794772684000852,
4.81603933352813));
#50809=CARTESIAN_POINT('Ctrl Pts',(3.80682492347781,-0.636309800095199,
4.83392412958058));
#50810=CARTESIAN_POINT('Ctrl Pts',(3.73085791651992,-0.319434907277161,
4.84718915136435));
#50811=CARTESIAN_POINT('Ctrl Pts',(3.70109773297182,-0.158333333333333,
4.85136434419625));
#50812=CARTESIAN_POINT('Ctrl Pts',(3.6877832654516,0.158333333333335,4.83026057386087));
#50813=CARTESIAN_POINT('Ctrl Pts',(3.70441500576368,0.319434907277169,4.80530409557185));
#50814=CARTESIAN_POINT('Ctrl Pts',(3.7528824829836,0.636309800095209,4.74839533465946));
#50815=CARTESIAN_POINT('Ctrl Pts',(3.79805031895221,0.794772684000843,4.70736492996899));
#50816=CARTESIAN_POINT('Ctrl Pts',(3.87672961928093,1.0684760419457,4.63893194866196));
#50817=CARTESIAN_POINT('Ctrl Pts',(3.91455463501092,1.18514270861293,4.60782998161182));
#50818=CARTESIAN_POINT('Ctrl Pts',(3.95614731271391,1.3000000000017,4.57524814942757));
#50819=CARTESIAN_POINT('Ctrl Pts',(4.04694899362265,-1.30000000000148,4.78821554320533));
#50820=CARTESIAN_POINT('Ctrl Pts',(3.98989123950318,-1.18514270861278,4.80967914782147));
#50821=CARTESIAN_POINT('Ctrl Pts',(3.93765915269118,-1.06847604194563,4.82779369545612));
#50822=CARTESIAN_POINT('Ctrl Pts',(3.82814084001427,-0.794772684000855,
4.86190493269116));
#50823=CARTESIAN_POINT('Ctrl Pts',(3.76801298829164,-0.636309800095199,
4.87711372021431));
#50824=CARTESIAN_POINT('Ctrl Pts',(3.69092186684021,-0.319434907277159,
4.88936263478558));
#50825=CARTESIAN_POINT('Ctrl Pts',(3.66216472084552,-0.158333333333333,
4.89086732377457));
#50826=CARTESIAN_POINT('Ctrl Pts',(3.64967259372367,0.158333333333335,4.87083435624963));
#50827=CARTESIAN_POINT('Ctrl Pts',(3.6665543296177,0.319434907277168,4.85020517031915));
#50828=CARTESIAN_POINT('Ctrl Pts',(3.71694367941793,0.636309800095208,4.79530005415465));
#50829=CARTESIAN_POINT('Ctrl Pts',(3.76196030831813,0.794772684000843,4.75620516222934));
#50830=CARTESIAN_POINT('Ctrl Pts',(3.84668046872571,1.06847604194569,4.68246710330853));
#50831=CARTESIAN_POINT('Ctrl Pts',(3.88829024992674,1.18514270861292,4.64732640905243));
#50832=CARTESIAN_POINT('Ctrl Pts',(3.93483759407961,1.30000000000169,4.60896349398276));
#50833=CARTESIAN_POINT('Ctrl Pts',(4.02820350434561,-1.30000000000148,4.81142487691947));
#50834=CARTESIAN_POINT('Ctrl Pts',(3.96711139186663,-1.18514270861278,4.83688576735673));
#50835=CARTESIAN_POINT('Ctrl Pts',(3.91175795323818,-1.06847604194562,4.85769236163318));
#50836=CARTESIAN_POINT('Ctrl Pts',(3.79713792120171,-0.794772684000852,
4.89500740153633));
#50837=CARTESIAN_POINT('Ctrl Pts',(3.73641632741839,-0.636309800095197,
4.90761088418304));
#50838=CARTESIAN_POINT('Ctrl Pts',(3.65836041920465,-0.319434907277159,
4.91891194253082));
#50839=CARTESIAN_POINT('Ctrl Pts',(3.63071576553046,-0.158333333333332,
4.91891982220856));
#50840=CARTESIAN_POINT('Ctrl Pts',(3.6187632745685,0.158333333333334,4.89969039499684));
#50841=CARTESIAN_POINT('Ctrl Pts',(3.63505260823184,0.319434907277167,4.88146360551658));
#50842=CARTESIAN_POINT('Ctrl Pts',(3.68754575873434,0.636309800095206,4.82893523730036));
#50843=CARTESIAN_POINT('Ctrl Pts',(3.73427465223176,0.794772684000839,4.79355980214051));
#50844=CARTESIAN_POINT('Ctrl Pts',(3.82428024392525,1.06847604194569,4.71663817608718));
#50845=CARTESIAN_POINT('Ctrl Pts',(3.8688015764165,1.18514270861292,4.67846105993602));
#50846=CARTESIAN_POINT('Ctrl Pts',(3.91888415579065,1.3000000000017,4.63540334932512));
#50847=CARTESIAN_POINT('Ctrl Pts',(4.01343459618057,-1.30000000000147,4.83038036764169));
#50848=CARTESIAN_POINT('Ctrl Pts',(3.94884952914959,-1.18514270861278,4.85880372193244));
#50849=CARTESIAN_POINT('Ctrl Pts',(3.89078431289497,-1.06847604194562,4.88156901137547));
#50850=CARTESIAN_POINT('Ctrl Pts',(3.77170420702538,-0.794772684000852,
4.92109012247909));
#50851=CARTESIAN_POINT('Ctrl Pts',(3.71031820055588,-0.636309800095198,
4.93138847019967));
#50852=CARTESIAN_POINT('Ctrl Pts',(3.63153238108231,-0.31943490727716,4.94197870250372));
#50853=CARTESIAN_POINT('Ctrl Pts',(3.60521842414231,-0.158333333333333,
4.94125686221945));
#50854=CARTESIAN_POINT('Ctrl Pts',(3.59372977080699,0.158333333333335,4.92270534040838));
#50855=CARTESIAN_POINT('Ctrl Pts',(3.60942918364311,0.319434907277167,4.90630002073989));
#50856=CARTESIAN_POINT('Ctrl Pts',(3.66303294591662,0.636309800095207,4.85502035171266));
#50857=CARTESIAN_POINT('Ctrl Pts',(3.71010928811268,0.794772684000843,4.82148032437692));
#50858=CARTESIAN_POINT('Ctrl Pts',(3.80424215552203,1.06847604194569,4.74179267501399));
#50859=CARTESIAN_POINT('Ctrl Pts',(3.85128182563464,1.18514270861292,4.70132919279899));
#50860=CARTESIAN_POINT('Ctrl Pts',(3.90461453552475,1.30000000000169,4.65489605905986));
#50861=CARTESIAN_POINT('Ctrl Pts',(4.00369573333263,-1.30000000000148,4.84150363158983));
#50862=CARTESIAN_POINT('Ctrl Pts',(3.9369331406498,-1.18514270861279,4.87168016066382));
#50863=CARTESIAN_POINT('Ctrl Pts',(3.87721261864588,-1.06847604194563,4.89563713118229));
#50864=CARTESIAN_POINT('Ctrl Pts',(3.75551485779726,-0.794772684000856,
4.93661410117369));
#50865=CARTESIAN_POINT('Ctrl Pts',(3.69414906548409,-0.636309800095199,
4.9460040068037));
#50866=CARTESIAN_POINT('Ctrl Pts',(3.61477395639173,-0.319434907277159,
4.95594238498443));
#50867=CARTESIAN_POINT('Ctrl Pts',(3.58861414097703,-0.158333333333333,
4.95391588925231));
#50868=CARTESIAN_POINT('Ctrl Pts',(3.57726781607701,0.158333333333335,4.93561307976536));
#50869=CARTESIAN_POINT('Ctrl Pts',(3.59283848397009,0.319434907277167,4.92066300742993));
#50870=CARTESIAN_POINT('Ctrl Pts',(3.64755963040239,0.636309800095207,4.87074166589155));
#50871=CARTESIAN_POINT('Ctrl Pts',(3.69529974618228,0.794772684000843,4.83892431680909));
#50872=CARTESIAN_POINT('Ctrl Pts',(3.79245733604709,1.06847604194569,4.75817145155974));
#50873=CARTESIAN_POINT('Ctrl Pts',(3.84123315554959,1.18514270861292,4.71654348050613));
#50874=CARTESIAN_POINT('Ctrl Pts',(3.89672887394551,1.30000000000169,4.6682424615769));
#50875=CARTESIAN_POINT('Ctrl Pts',(3.99200513405346,-1.30000000000148,4.85500476616359));
#50876=CARTESIAN_POINT('Ctrl Pts',(3.9225817040123,-1.18514270861278,4.88750892319406));
#50877=CARTESIAN_POINT('Ctrl Pts',(3.86073528255479,-1.06847604194562,4.91292369199203));
#50878=CARTESIAN_POINT('Ctrl Pts',(3.73536208225759,-0.794772684000853,
4.95525898707803));
#50879=CARTESIAN_POINT('Ctrl Pts',(3.67258109636451,-0.636309800095199,
4.96158478192644));
#50880=CARTESIAN_POINT('Ctrl Pts',(3.59320814768429,-0.31943490727716,4.97176932104344));
#50881=CARTESIAN_POINT('Ctrl Pts',(3.56997555784675,-0.158333333333333,
4.97186073258582));
#50882=CARTESIAN_POINT('Ctrl Pts',(3.55929280216314,0.158333333333335,4.95453826427217));
#50883=CARTESIAN_POINT('Ctrl Pts',(3.57301586257808,0.319434907277169,4.93908630245288));
#50884=CARTESIAN_POINT('Ctrl Pts',(3.62823902969615,0.636309800095209,4.88962085686202));
#50885=CARTESIAN_POINT('Ctrl Pts',(3.67674433586902,0.794772684000844,4.85984726567696));
#50886=CARTESIAN_POINT('Ctrl Pts',(3.77726226125242,1.06847604194569,4.77718005722317));
#50887=CARTESIAN_POINT('Ctrl Pts',(3.82803455991401,1.18514270861292,4.73385987707036));
#50888=CARTESIAN_POINT('Ctrl Pts',(3.88606867189482,1.30000000000169,4.6830030881825));
#50889=CARTESIAN_POINT('Ctrl Pts',(3.98232662500902,-1.30000000000148,4.86614166803579));
#50890=CARTESIAN_POINT('Ctrl Pts',(3.91032776155344,-1.18514270861278,4.89969217989033));
#50891=CARTESIAN_POINT('Ctrl Pts',(3.8467218346907,-1.06847604194563,4.92603065578664));
#50892=CARTESIAN_POINT('Ctrl Pts',(3.71916878184664,-0.794772684000855,
4.97021655827468));
#50893=CARTESIAN_POINT('Ctrl Pts',(3.65787869457123,-0.636309800095198,
4.97765410576821));
#50894=CARTESIAN_POINT('Ctrl Pts',(3.57897420566855,-0.319434907277158,
4.98853742307923));
#50895=CARTESIAN_POINT('Ctrl Pts',(3.55660206408478,-0.158333333333333,
4.98821755280578));
#50896=CARTESIAN_POINT('Ctrl Pts',(3.54553189689183,0.158333333333334,4.97039301587236));
#50897=CARTESIAN_POINT('Ctrl Pts',(3.55744003194949,0.319434907277168,4.95408557004192));
#50898=CARTESIAN_POINT('Ctrl Pts',(3.61256068172531,0.636309800095207,4.90445630177975));
#50899=CARTESIAN_POINT('Ctrl Pts',(3.661578762114,0.794772684000841,4.87634867301211));
#50900=CARTESIAN_POINT('Ctrl Pts',(3.76462577505384,1.06847604194569,4.79224273511056));
#50901=CARTESIAN_POINT('Ctrl Pts',(3.81696042431411,1.18514270861292,4.74767559603195));
#50902=CARTESIAN_POINT('Ctrl Pts',(3.87702448920102,1.30000000000169,4.69494766196028));
#50903=CARTESIAN_POINT('Ctrl Pts',(3.97017242189175,-1.30000000000147,4.8790119628149));
#50904=CARTESIAN_POINT('Ctrl Pts',(3.89477616791294,-1.18514270861278,4.91405759574364));
#50905=CARTESIAN_POINT('Ctrl Pts',(3.82891412524378,-1.06847604194562,4.9418349037975));
#50906=CARTESIAN_POINT('Ctrl Pts',(3.69878556645952,-0.794772684000853,
4.98921475774886));
#50907=CARTESIAN_POINT('Ctrl Pts',(3.63987925188336,-0.636309800095197,
4.99903821383355));
#50908=CARTESIAN_POINT('Ctrl Pts',(3.56209901489986,-0.319434907277159,
5.01178185899569));
#50909=CARTESIAN_POINT('Ctrl Pts',(3.54101295953038,-0.158333333333333,
5.01109473458552));
#50910=CARTESIAN_POINT('Ctrl Pts',(3.52999041709157,0.158333333333334,4.99337364465456));
#50911=CARTESIAN_POINT('Ctrl Pts',(3.54046028559251,0.319434907277167,4.97729034590911));
#50912=CARTESIAN_POINT('Ctrl Pts',(3.59496068023953,0.636309800095207,4.92651367674735));
#50913=CARTESIAN_POINT('Ctrl Pts',(3.64267540721733,0.79477268400084,4.8974863283316));
#50914=CARTESIAN_POINT('Ctrl Pts',(3.74843407961049,1.06847604194569,4.81028335055866));
#50915=CARTESIAN_POINT('Ctrl Pts',(3.8028541532843,1.18514270861292,4.76398549709187));
#50916=CARTESIAN_POINT('Ctrl Pts',(3.86591529009784,1.3000000000017,4.70913672804752));
#50917=CARTESIAN_POINT('Ctrl Pts',(3.96195840372475,-1.30000000000147,4.88785815300733));
#50918=CARTESIAN_POINT('Ctrl Pts',(3.88343455682606,-1.18514270861278,4.92281726405495));
#50919=CARTESIAN_POINT('Ctrl Pts',(3.81579954549607,-1.06847604194562,4.95110239256332));
#50920=CARTESIAN_POINT('Ctrl Pts',(3.68470452745418,-0.794772684000851,
5.00102846304682));
#50921=CARTESIAN_POINT('Ctrl Pts',(3.63046739270751,-0.636309800095197,
5.01550900850482));
#50922=CARTESIAN_POINT('Ctrl Pts',(3.55506550341723,-0.319434907277159,
5.03079025948107));
#50923=CARTESIAN_POINT('Ctrl Pts',(3.53467416208633,-0.158333333333332,
5.02927276087076));
#50924=CARTESIAN_POINT('Ctrl Pts',(3.52377125184822,0.158333333333334,5.01165271185736));
#50925=CARTESIAN_POINT('Ctrl Pts',(3.53363020048007,0.319434907277167,4.99634356970428));
#50926=CARTESIAN_POINT('Ctrl Pts',(3.58606892910199,0.636309800095206,4.94355543209541));
#50927=CARTESIAN_POINT('Ctrl Pts',(3.62956460835032,0.79477268400084,4.91094102067596));
#50928=CARTESIAN_POINT('Ctrl Pts',(3.73626839073644,1.06847604194569,4.82114406341654));
#50929=CARTESIAN_POINT('Ctrl Pts',(3.79232877910752,1.18514270861292,4.77404740884945));
#50930=CARTESIAN_POINT('Ctrl Pts',(3.85826144221939,1.30000000000169,4.71872387520778));
#50931=CARTESIAN_POINT('Ctrl Pts',(3.95827679071615,-1.30000000000147,4.89563255511119));
#50932=CARTESIAN_POINT('Ctrl Pts',(3.87988594951817,-1.18514270861278,4.93037843917678));
#50933=CARTESIAN_POINT('Ctrl Pts',(3.81258907846072,-1.06847604194562,4.95873129561837));
#50934=CARTESIAN_POINT('Ctrl Pts',(3.68274913399113,-0.794772684000851,
5.00946289323563));
#50935=CARTESIAN_POINT('Ctrl Pts',(3.630353335205,-0.636309800095197,5.0257302081468));
#50936=CARTESIAN_POINT('Ctrl Pts',(3.55620605750903,-0.319434907277159,
5.04213862663278));
#50937=CARTESIAN_POINT('Ctrl Pts',(3.53576509129249,-0.158333333333332,
5.04063778675236));
#50938=CARTESIAN_POINT('Ctrl Pts',(3.52505210827392,0.158333333333334,5.02315921127616));
#50939=CARTESIAN_POINT('Ctrl Pts',(3.53535684314381,0.319434907277167,5.00816436619336));
#50940=CARTESIAN_POINT('Ctrl Pts',(3.58650774416314,0.636309800095206,4.95415127075708));
#50941=CARTESIAN_POINT('Ctrl Pts',(3.62740723167583,0.79477268400084,4.91897241923608));
#50942=CARTESIAN_POINT('Ctrl Pts',(3.73295432340188,1.06847604194569,4.82848789979354));
#50943=CARTESIAN_POINT('Ctrl Pts',(3.78889068790091,1.18514270861292,4.78156123638169));
#50944=CARTESIAN_POINT('Ctrl Pts',(3.85507599179584,1.30000000000169,4.72687530524289));
#50945=CARTESIAN_POINT('Ctrl Pts',(3.95827679071515,-1.3,4.89563255511164));
#50946=CARTESIAN_POINT('Ctrl Pts',(3.8798859495176,-1.18514270861178,4.93037843917702));
#50947=CARTESIAN_POINT('Ctrl Pts',(3.81258907846048,-1.06847604194512,4.95873129561847));
#50948=CARTESIAN_POINT('Ctrl Pts',(3.68274913399113,-0.794772684000851,
5.00946289323563));
#50949=CARTESIAN_POINT('Ctrl Pts',(3.630353335205,-0.636309800095197,5.0257302081468));
#50950=CARTESIAN_POINT('Ctrl Pts',(3.55620605750903,-0.319434907277159,
5.04213862663278));
#50951=CARTESIAN_POINT('Ctrl Pts',(3.53576509129248,-0.158333333333332,
5.04063778675235));
#50952=CARTESIAN_POINT('Ctrl Pts',(3.52505210827392,0.158333333333334,5.02315921127615));
#50953=CARTESIAN_POINT('Ctrl Pts',(3.53535684314381,0.319434907277167,5.00816436619335));
#50954=CARTESIAN_POINT('Ctrl Pts',(3.58650774416314,0.636309800095206,4.95415127075708));
#50955=CARTESIAN_POINT('Ctrl Pts',(3.62740723167583,0.79477268400084,4.91897241923608));
#50956=CARTESIAN_POINT('Ctrl Pts',(3.73295432340165,1.06847604194511,4.82848789979373));
#50957=CARTESIAN_POINT('Ctrl Pts',(3.78889068790036,1.18514270861178,4.78156123638215));
#50958=CARTESIAN_POINT('Ctrl Pts',(3.85507599179487,1.3,4.7268753052437));
#50959=CARTESIAN_POINT('',(4.1759065994826,-1.2,4.54212414277912));
#50960=CARTESIAN_POINT('Ctrl Pts',(4.1759065994826,-1.2,4.54212414277912));
#50961=CARTESIAN_POINT('Ctrl Pts',(4.17214418520691,-1.20924463866719,4.55342996457554));
#50962=CARTESIAN_POINT('Ctrl Pts',(4.16875627541578,-1.21821443520797,4.56484907677502));
#50963=CARTESIAN_POINT('Ctrl Pts',(4.16201532047973,-1.23542515838613,4.58643092051385));
#50964=CARTESIAN_POINT('Ctrl Pts',(4.1614115775334,-1.23665315490756,4.5877694327218));
#50965=CARTESIAN_POINT('Ctrl Pts',(4.15027423165472,-1.26335624147386,4.62034316080045));
#50966=CARTESIAN_POINT('Ctrl Pts',(4.14011740706728,-1.28779025121432,4.65037203783849));
#50967=CARTESIAN_POINT('Ctrl Pts',(4.13470146325513,-1.3,4.66489767272486));
#50968=CARTESIAN_POINT('',(4.08975875278338,-0.653834841367117,4.41138504922928));
#50969=CARTESIAN_POINT('Ctrl Pts',(4.08975875281708,-0.653834841365838,
4.4113850492124));
#50970=CARTESIAN_POINT('Ctrl Pts',(4.09883612367009,-0.717342388655811,
4.42469784339655));
#50971=CARTESIAN_POINT('Ctrl Pts',(4.10644894485254,-0.765483511502256,
4.43597370734929));
#50972=CARTESIAN_POINT('Ctrl Pts',(4.13503526267317,-0.949592603242909,
4.47874631007404));
#50973=CARTESIAN_POINT('Ctrl Pts',(4.15182328757237,-1.05626431331092,4.50428578367362));
#50974=CARTESIAN_POINT('Ctrl Pts',(4.1759065994826,-1.2,4.54212414277912));
#50975=CARTESIAN_POINT('',(4.00955034077224,0.653834841531101,4.29724164546664));
#50976=CARTESIAN_POINT('Ctrl Pts',(4.00955034077224,0.653834841531101,4.29724164546664));
#50977=CARTESIAN_POINT('Ctrl Pts',(3.98927872982994,0.575994542894782,4.33352914862505));
#50978=CARTESIAN_POINT('Ctrl Pts',(3.97279875699981,0.493637872429252,4.36460185351157));
#50979=CARTESIAN_POINT('Ctrl Pts',(3.95126345212767,0.338127837060752,4.41040803616251));
#50980=CARTESIAN_POINT('Ctrl Pts',(3.94478094307397,0.265653872177931,4.42707925918047));
#50981=CARTESIAN_POINT('Ctrl Pts',(3.94007563669224,0.129712215371197,4.45098897808368));
#50982=CARTESIAN_POINT('Ctrl Pts',(3.94076895770888,0.0666227083564181,
4.45923189482429));
#50983=CARTESIAN_POINT('Ctrl Pts',(3.94812442420765,-0.0595436117189309,
4.47034568766396));
#50984=CARTESIAN_POINT('Ctrl Pts',(3.95482572321592,-0.122773201281119,
4.47330664288229));
#50985=CARTESIAN_POINT('Ctrl Pts',(3.97556620162042,-0.260125628448797,
4.47324337421401));
#50986=CARTESIAN_POINT('Ctrl Pts',(3.99072482510553,-0.333944860941934,
4.46902771026615));
#50987=CARTESIAN_POINT('Ctrl Pts',(4.03134314078074,-0.491205254633584,
4.45001447015766));
#50988=CARTESIAN_POINT('Ctrl Pts',(4.05833207591073,-0.574347106328157,
4.4336311917751));
#50989=CARTESIAN_POINT('Ctrl Pts',(4.08975875278252,-0.653834841383954,
4.41138504928823));
#50990=CARTESIAN_POINT('',(4.05150253593681,1.2,4.35608945265544));
#50991=CARTESIAN_POINT('Ctrl Pts',(4.05150253593681,1.2,4.35608945265544));
#50992=CARTESIAN_POINT('Ctrl Pts',(4.04575710139426,1.14657618383835,4.34790437009688));
#50993=CARTESIAN_POINT('Ctrl Pts',(4.03662031939464,1.06003819843532,4.3349237974889));
#50994=CARTESIAN_POINT('Ctrl Pts',(4.0161950566583,0.792700141885613,4.3064105960449));
#50995=CARTESIAN_POINT('Ctrl Pts',(4.01325274808858,0.738260770271576,4.30235574271615));
#50996=CARTESIAN_POINT('Ctrl Pts',(4.00955034077224,0.653834841531101,4.29724164546664));
#50997=CARTESIAN_POINT('Ctrl Pts',(4.01191463394249,1.3,4.47474020138297));
#50998=CARTESIAN_POINT('Ctrl Pts',(4.01997786089997,1.28107343755638,4.45292765725262));
#50999=CARTESIAN_POINT('Ctrl Pts',(4.02551045807113,1.26655089503634,4.43531292137856));
#51000=CARTESIAN_POINT('Ctrl Pts',(4.03894397720598,1.23311712142409,4.39592764313121));
#51001=CARTESIAN_POINT('Ctrl Pts',(4.04577421378828,1.21590150548676,4.37560629030699));
#51002=CARTESIAN_POINT('Ctrl Pts',(4.05150253593681,1.2,4.35608945265544));
#51003=CARTESIAN_POINT('Ctrl Pts',(3.95827679071515,-1.3,4.89563255511164));
#51004=CARTESIAN_POINT('Ctrl Pts',(3.8798859495176,-1.18514270861178,4.93037843917702));
#51005=CARTESIAN_POINT('Ctrl Pts',(3.81258907846048,-1.06847604194512,4.95873129561847));
#51006=CARTESIAN_POINT('Ctrl Pts',(3.68274913399113,-0.794772684000851,
5.00946289323563));
#51007=CARTESIAN_POINT('Ctrl Pts',(3.630353335205,-0.636309800095197,5.0257302081468));
#51008=CARTESIAN_POINT('Ctrl Pts',(3.55620605750904,-0.319434907277159,
5.04213862663278));
#51009=CARTESIAN_POINT('Ctrl Pts',(3.53576509129249,-0.158333333333332,
5.04063778675235));
#51010=CARTESIAN_POINT('Ctrl Pts',(3.52505210827392,0.158333333333334,5.02315921127615));
#51011=CARTESIAN_POINT('Ctrl Pts',(3.53535684314381,0.319434907277167,5.00816436619336));
#51012=CARTESIAN_POINT('Ctrl Pts',(3.58650774416314,0.636309800095206,4.95415127075708));
#51013=CARTESIAN_POINT('Ctrl Pts',(3.62740723167583,0.79477268400084,4.91897241923608));
#51014=CARTESIAN_POINT('Ctrl Pts',(3.73295432340165,1.06847604194511,4.82848789979373));
#51015=CARTESIAN_POINT('Ctrl Pts',(3.78889068790036,1.18514270861178,4.78156123638215));
#51016=CARTESIAN_POINT('Ctrl Pts',(3.85507599179487,1.3,4.7268753052437));
#51017=CARTESIAN_POINT('Ctrl Pts',(3.99529346323777,-1.3,4.96307790506253));
#51018=CARTESIAN_POINT('Ctrl Pts',(3.91621554992515,-1.18514270861178,4.99623355742632));
#51019=CARTESIAN_POINT('Ctrl Pts',(3.84848168092754,-1.06847604194512,5.02346178870243));
#51020=CARTESIAN_POINT('Ctrl Pts',(3.7182099051649,-0.794772684000851,5.07267092145019));
#51021=CARTESIAN_POINT('Ctrl Pts',(3.66630753169098,-0.636309800095197,
5.08945932120005));
#51022=CARTESIAN_POINT('Ctrl Pts',(3.59275862546217,-0.319434907277159,
5.10616207752106));
#51023=CARTESIAN_POINT('Ctrl Pts',(3.57308521991698,-0.158333333333332,
5.10563709747918));
#51024=CARTESIAN_POINT('Ctrl Pts',(3.56268309827958,0.158333333333334,5.08797904610088));
#51025=CARTESIAN_POINT('Ctrl Pts',(3.57252649407444,0.319434907277167,5.07183154405847));
#51026=CARTESIAN_POINT('Ctrl Pts',(3.62372167678492,0.636309800095206,5.01715307481322));
#51027=CARTESIAN_POINT('Ctrl Pts',(3.66441660424588,0.79477268400084,4.98128636201763));
#51028=CARTESIAN_POINT('Ctrl Pts',(3.77106627357833,1.06847604194511,4.89193705188011));
#51029=CARTESIAN_POINT('Ctrl Pts',(3.8277580930697,1.18514270861178,4.84595115236908));
#51030=CARTESIAN_POINT('Ctrl Pts',(3.89497704195816,1.3,4.7926553589873));
#51031=CARTESIAN_POINT('Ctrl Pts',(4.0323101357604,-1.3,5.03052325501342));
#51032=CARTESIAN_POINT('Ctrl Pts',(3.95254515033271,-1.18514270861178,5.06208867567562));
#51033=CARTESIAN_POINT('Ctrl Pts',(3.88437428339459,-1.06847604194512,5.08819228178639));
#51034=CARTESIAN_POINT('Ctrl Pts',(3.75367067633867,-0.794772684000851,
5.13587894966475));
#51035=CARTESIAN_POINT('Ctrl Pts',(3.70226172817696,-0.636309800095197,
5.15318843425331));
#51036=CARTESIAN_POINT('Ctrl Pts',(3.62931119341529,-0.319434907277159,
5.17018552840935));
#51037=CARTESIAN_POINT('Ctrl Pts',(3.61040534854147,-0.158333333333332,
5.170636408206));
#51038=CARTESIAN_POINT('Ctrl Pts',(3.60031408828524,0.158333333333334,5.1527988809256));
#51039=CARTESIAN_POINT('Ctrl Pts',(3.60969614500508,0.319434907277167,5.13549872192358));
#51040=CARTESIAN_POINT('Ctrl Pts',(3.6609356094067,0.636309800095206,5.08015487886937));
#51041=CARTESIAN_POINT('Ctrl Pts',(3.70142597681592,0.79477268400084,5.04360030479918));
#51042=CARTESIAN_POINT('Ctrl Pts',(3.80917822375501,1.06847604194511,4.9553862039665));
#51043=CARTESIAN_POINT('Ctrl Pts',(3.86662549823905,1.18514270861178,4.91034106835601));
#51044=CARTESIAN_POINT('Ctrl Pts',(3.93487809212145,1.3,4.85843541273091));
#51045=CARTESIAN_POINT('Ctrl Pts',(4.06932680828302,-1.3,5.09796860496431));
#51046=CARTESIAN_POINT('Ctrl Pts',(3.98887475074027,-1.18514270861178,5.12794379392492));
#51047=CARTESIAN_POINT('Ctrl Pts',(3.92026688586164,-1.06847604194512,5.15292277487036));
#51048=CARTESIAN_POINT('Ctrl Pts',(3.78913144751244,-0.794772684000851,
5.19908697787931));
#51049=CARTESIAN_POINT('Ctrl Pts',(3.73821592466294,-0.636309800095197,
5.21691754730656));
#51050=CARTESIAN_POINT('Ctrl Pts',(3.66586376136842,-0.319434907277159,
5.23420897929763));
#51051=CARTESIAN_POINT('Ctrl Pts',(3.64772547716597,-0.158333333333332,
5.23563571893282));
#51052=CARTESIAN_POINT('Ctrl Pts',(3.6379450782909,0.158333333333334,5.21761871575033));
#51053=CARTESIAN_POINT('Ctrl Pts',(3.64686579593571,0.319434907277167,5.19916589978869));
#51054=CARTESIAN_POINT('Ctrl Pts',(3.69814954202848,0.636309800095206,5.14315668292551));
#51055=CARTESIAN_POINT('Ctrl Pts',(3.73843534938597,0.79477268400084,5.10591424758073));
#51056=CARTESIAN_POINT('Ctrl Pts',(3.84729017393168,1.06847604194511,5.01883535605289));
#51057=CARTESIAN_POINT('Ctrl Pts',(3.90549290340839,1.18514270861178,4.97473098434294));
#51058=CARTESIAN_POINT('Ctrl Pts',(3.97477914228474,1.3,4.92421546647452));
#51059=CARTESIAN_POINT('Ctrl Pts',(4.06932680828302,-1.3,5.09796860496431));
#51060=CARTESIAN_POINT('Ctrl Pts',(3.98887475074027,-1.18514270861178,5.12794379392492));
#51061=CARTESIAN_POINT('Ctrl Pts',(3.92026688586165,-1.06847604194512,5.15292277487036));
#51062=CARTESIAN_POINT('Ctrl Pts',(3.78913144751244,-0.794772684000851,
5.19908697787931));
#51063=CARTESIAN_POINT('Ctrl Pts',(3.73821592466294,-0.636309800095197,
5.21691754730656));
#51064=CARTESIAN_POINT('Ctrl Pts',(3.66586376136842,-0.319434907277159,
5.23420897929763));
#51065=CARTESIAN_POINT('Ctrl Pts',(3.64772547716596,-0.158333333333332,
5.23563571893282));
#51066=CARTESIAN_POINT('Ctrl Pts',(3.6379450782909,0.158333333333334,5.21761871575033));
#51067=CARTESIAN_POINT('Ctrl Pts',(3.64686579593571,0.319434907277167,5.19916589978868));
#51068=CARTESIAN_POINT('Ctrl Pts',(3.69814954202848,0.636309800095206,5.14315668292551));
#51069=CARTESIAN_POINT('Ctrl Pts',(3.73843534938597,0.79477268400084,5.10591424758073));
#51070=CARTESIAN_POINT('Ctrl Pts',(3.84729017393168,1.06847604194511,5.01883535605289));
#51071=CARTESIAN_POINT('Ctrl Pts',(3.90549290340839,1.18514270861178,4.97473098434294));
#51072=CARTESIAN_POINT('Ctrl Pts',(3.97477914228473,1.3,4.92421546647452));
#51073=CARTESIAN_POINT('Ctrl Pts',(4.0693268082831,-1.30000000000011,5.09796860496428));
#51074=CARTESIAN_POINT('Ctrl Pts',(3.98887475074031,-1.18514270861186,5.1279437939249));
#51075=CARTESIAN_POINT('Ctrl Pts',(3.92026688586166,-1.06847604194515,5.15292277487035));
#51076=CARTESIAN_POINT('Ctrl Pts',(3.78913144751244,-0.794772684000851,
5.19908697787931));
#51077=CARTESIAN_POINT('Ctrl Pts',(3.73821592466294,-0.636309800095197,
5.21691754730656));
#51078=CARTESIAN_POINT('Ctrl Pts',(3.66586376136842,-0.319434907277159,
5.23420897929763));
#51079=CARTESIAN_POINT('Ctrl Pts',(3.64772547716596,-0.158333333333332,
5.23563571893282));
#51080=CARTESIAN_POINT('Ctrl Pts',(3.6379450782909,0.158333333333334,5.21761871575033));
#51081=CARTESIAN_POINT('Ctrl Pts',(3.64686579593571,0.319434907277167,5.19916589978868));
#51082=CARTESIAN_POINT('Ctrl Pts',(3.69814954202848,0.636309800095206,5.14315668292551));
#51083=CARTESIAN_POINT('Ctrl Pts',(3.73843534938597,0.79477268400084,5.10591424758073));
#51084=CARTESIAN_POINT('Ctrl Pts',(3.84729017393193,1.06847604194573,5.01883535605269));
#51085=CARTESIAN_POINT('Ctrl Pts',(3.905492903409,1.18514270861299,4.97473098434248));
#51086=CARTESIAN_POINT('Ctrl Pts',(3.97477914228582,1.3000000000018,4.92421546647373));
#51087=CARTESIAN_POINT('Ctrl Pts',(4.07797887893023,-1.30000000000011,5.09928563902119));
#51088=CARTESIAN_POINT('Ctrl Pts',(3.99710096182082,-1.18514270861186,5.12872323339091));
#51089=CARTESIAN_POINT('Ctrl Pts',(3.92828386835217,-1.06847604194515,5.15372462658026));
#51090=CARTESIAN_POINT('Ctrl Pts',(3.79716553099686,-0.794772684000851,
5.20123433417352));
#51091=CARTESIAN_POINT('Ctrl Pts',(3.74717278256209,-0.636309800095197,
5.2225954916431));
#51092=CARTESIAN_POINT('Ctrl Pts',(3.67523755004235,-0.319434907277159,
5.24161469397914));
#51093=CARTESIAN_POINT('Ctrl Pts',(3.65704996965851,-0.158333333333332,
5.24249822290199));
#51094=CARTESIAN_POINT('Ctrl Pts',(3.64724201471915,0.158333333333334,5.22424600115186));
#51095=CARTESIAN_POINT('Ctrl Pts',(3.65612349309497,0.319434907277167,5.2058278322046));
#51096=CARTESIAN_POINT('Ctrl Pts',(3.7070583893129,0.636309800095206,5.1481685060594));
#51097=CARTESIAN_POINT('Ctrl Pts',(3.7467174769052,0.79477268400084,5.10843804227397));
#51098=CARTESIAN_POINT('Ctrl Pts',(3.85550223127368,1.06847604194573,5.01986946158344));
#51099=CARTESIAN_POINT('Ctrl Pts',(3.91381537677383,1.18514270861299,4.97543838784214));
#51100=CARTESIAN_POINT('Ctrl Pts',(3.98335277848031,1.3000000000018,4.92491429715123));
#51101=CARTESIAN_POINT('Ctrl Pts',(4.09010264837502,-1.30000000000011,5.0974281824879));
#51102=CARTESIAN_POINT('Ctrl Pts',(4.01107193700271,-1.18514270861186,5.12460716309181));
#51103=CARTESIAN_POINT('Ctrl Pts',(3.94376817464231,-1.06847604194516,5.14858398387072));
#51104=CARTESIAN_POINT('Ctrl Pts',(3.81537461770386,-0.794772684000852,
5.19657760663093));
#51105=CARTESIAN_POINT('Ctrl Pts',(3.76638838416209,-0.636309800095198,
5.22341425512017));
#51106=CARTESIAN_POINT('Ctrl Pts',(3.69516960528746,-0.319434907277159,
5.24523969656485));
#51107=CARTESIAN_POINT('Ctrl Pts',(3.67600601086261,-0.158333333333333,
5.24626900813328));
#51108=CARTESIAN_POINT('Ctrl Pts',(3.66616720149152,0.158333333333335,5.22785505234343));
#51109=CARTESIAN_POINT('Ctrl Pts',(3.67610760976984,0.319434907277169,5.20922731970925));
#51110=CARTESIAN_POINT('Ctrl Pts',(3.72603146219124,0.636309800095208,5.14823279065688));
#51111=CARTESIAN_POINT('Ctrl Pts',(3.76399726034961,0.794772684000841,5.10214216240938));
#51112=CARTESIAN_POINT('Ctrl Pts',(3.87009225143811,1.06847604194573,5.01314284055789));
#51113=CARTESIAN_POINT('Ctrl Pts',(3.92707741387766,1.18514270861299,4.96999514155808));
#51114=CARTESIAN_POINT('Ctrl Pts',(3.9951231483213,1.3000000000018,4.92222425223821));
#51115=CARTESIAN_POINT('Ctrl Pts',(4.10794777737404,-1.30000000000012,5.09490870018085));
#51116=CARTESIAN_POINT('Ctrl Pts',(4.03225269306678,-1.18514270861186,5.12055373952318));
#51117=CARTESIAN_POINT('Ctrl Pts',(3.9674904650733,-1.06847604194516,5.14359000792102));
#51118=CARTESIAN_POINT('Ctrl Pts',(3.84313384796426,-0.794772684000854,
5.19078161354514));
#51119=CARTESIAN_POINT('Ctrl Pts',(3.79428998871027,-0.636309800095197,
5.21920069851044));
#51120=CARTESIAN_POINT('Ctrl Pts',(3.72375313872692,-0.319434907277158,
5.24213353045454));
#51121=CARTESIAN_POINT('Ctrl Pts',(3.70367705257536,-0.158333333333332,
5.24429872357439));
#51122=CARTESIAN_POINT('Ctrl Pts',(3.69377031090259,0.158333333333334,5.22578741725238));
#51123=CARTESIAN_POINT('Ctrl Pts',(3.70466740404922,0.319434907277167,5.20622006587942));
#51124=CARTESIAN_POINT('Ctrl Pts',(3.75354256291749,0.636309800095206,5.14332178106065));
#51125=CARTESIAN_POINT('Ctrl Pts',(3.79063989923004,0.79477268400084,5.09398573728429));
#51126=CARTESIAN_POINT('Ctrl Pts',(3.89268207298159,1.06847604194573,5.00562106515799));
#51127=CARTESIAN_POINT('Ctrl Pts',(3.94729257723669,1.18514270861299,4.96370624545236));
#51128=CARTESIAN_POINT('Ctrl Pts',(4.0123433097649,1.3000000000018,4.91812639837089));
#51129=CARTESIAN_POINT('Ctrl Pts',(4.12279848538878,-1.30000000000011,5.09299696544897));
#51130=CARTESIAN_POINT('Ctrl Pts',(4.04973737154303,-1.18514270861186,5.11780304214634));
#51131=CARTESIAN_POINT('Ctrl Pts',(3.98683773167486,-1.06847604194515,5.14010459239705));
#51132=CARTESIAN_POINT('Ctrl Pts',(3.86500201823367,-0.794772684000847,
5.18583967776539));
#51133=CARTESIAN_POINT('Ctrl Pts',(3.81499269883938,-0.636309800095196,
5.21304042894478));
#51134=CARTESIAN_POINT('Ctrl Pts',(3.74455865547157,-0.319434907277159,
5.23617576257593));
#51135=CARTESIAN_POINT('Ctrl Pts',(3.72431438160608,-0.158333333333332,
5.24034022241887));
#51136=CARTESIAN_POINT('Ctrl Pts',(3.71464909220497,0.158333333333334,5.22241426405417));
#51137=CARTESIAN_POINT('Ctrl Pts',(3.72633101530915,0.319434907277168,5.20229432941527));
#51138=CARTESIAN_POINT('Ctrl Pts',(3.77483095349572,0.636309800095206,5.13863137615708));
#51139=CARTESIAN_POINT('Ctrl Pts',(3.81170550975848,0.79477268400084,5.08744014969362));
#51140=CARTESIAN_POINT('Ctrl Pts',(3.91105160620998,1.06847604194572,5.0000431978649));
#51141=CARTESIAN_POINT('Ctrl Pts',(3.96398160966473,1.18514270861299,4.95919623757555));
#51142=CARTESIAN_POINT('Ctrl Pts',(4.02683837255595,1.30000000000179,4.91533321906738));
#51143=CARTESIAN_POINT('Ctrl Pts',(4.14093676471968,-1.30000000000012,5.09122327296693));
#51144=CARTESIAN_POINT('Ctrl Pts',(4.07136124135871,-1.18514270861186,5.11513023307149));
#51145=CARTESIAN_POINT('Ctrl Pts',(4.01092377079359,-1.06847604194515,5.13655462063614));
#51146=CARTESIAN_POINT('Ctrl Pts',(3.89241185333326,-0.794772684000849,
5.18031400264045));
#51147=CARTESIAN_POINT('Ctrl Pts',(3.84098475691061,-0.636309800095196,
5.20574733491462));
#51148=CARTESIAN_POINT('Ctrl Pts',(3.77038842401171,-0.319434907277158,
5.22817448647597));
#51149=CARTESIAN_POINT('Ctrl Pts',(3.74965933386978,-0.158333333333332,
5.23419883041956));
#51150=CARTESIAN_POINT('Ctrl Pts',(3.73946847381987,0.158333333333334,5.21519302180799));
#51151=CARTESIAN_POINT('Ctrl Pts',(3.75076522365139,0.319434907277166,5.19145759520968));
#51152=CARTESIAN_POINT('Ctrl Pts',(3.79905845830081,0.636309800095205,5.12767971641947));
#51153=CARTESIAN_POINT('Ctrl Pts',(3.83790641149878,0.79477268400084,5.07929867273251));
#51154=CARTESIAN_POINT('Ctrl Pts',(3.93424552319471,1.06847604194572,4.99440458049406));
#51155=CARTESIAN_POINT('Ctrl Pts',(3.98484885667692,1.18514270861299,4.95465795765977));
#51156=CARTESIAN_POINT('Ctrl Pts',(4.04435389190397,1.30000000000179,4.91191221888519));
#51157=CARTESIAN_POINT('Ctrl Pts',(4.15945674239667,-1.30000000000011,5.0907785324072));
#51158=CARTESIAN_POINT('Ctrl Pts',(4.09311080137659,-1.18514270861186,5.11348319756018));
#51159=CARTESIAN_POINT('Ctrl Pts',(4.0349310031657,-1.06847604194515,5.13378061450161));
#51160=CARTESIAN_POINT('Ctrl Pts',(3.91938945399031,-0.794772684000846,
5.17511048318358));
#51161=CARTESIAN_POINT('Ctrl Pts',(3.86667281998677,-0.636309800095196,
5.1991035673952));
#51162=CARTESIAN_POINT('Ctrl Pts',(3.79539589942942,-0.31943490727716,5.21970860197993));
#51163=CARTESIAN_POINT('Ctrl Pts',(3.77306755224646,-0.158333333333332,
5.22498077356131));
#51164=CARTESIAN_POINT('Ctrl Pts',(3.76271494571253,0.158333333333334,5.20569233878662));
#51165=CARTESIAN_POINT('Ctrl Pts',(3.77547192320316,0.319434907277168,5.18256501209488));
#51166=CARTESIAN_POINT('Ctrl Pts',(3.82407000646787,0.636309800095207,5.11975133721079));
#51167=CARTESIAN_POINT('Ctrl Pts',(3.86382586108813,0.794772684000841,5.07181087963962));
#51168=CARTESIAN_POINT('Ctrl Pts',(3.95706378536076,1.06847604194573,4.98878077345485));
#51169=CARTESIAN_POINT('Ctrl Pts',(4.00543525417068,1.18514270861299,4.95007068503404));
#51170=CARTESIAN_POINT('Ctrl Pts',(4.06181894917838,1.30000000000179,4.90859116459128));
#51171=CARTESIAN_POINT('Ctrl Pts',(4.18342557961076,-1.30000000000011,5.0880533237051));
#51172=CARTESIAN_POINT('Ctrl Pts',(4.12172043887367,-1.18514270861186,5.10991684623856));
#51173=CARTESIAN_POINT('Ctrl Pts',(4.06683983019807,-1.06847604194515,5.12935875501752));
#51174=CARTESIAN_POINT('Ctrl Pts',(3.95582067963427,-0.794772684000848,
5.16867904142233));
#51175=CARTESIAN_POINT('Ctrl Pts',(3.90159042509488,-0.636309800095196,
5.19114024563324));
#51176=CARTESIAN_POINT('Ctrl Pts',(3.82979124448239,-0.319434907277159,
5.21013150112414));
#51177=CARTESIAN_POINT('Ctrl Pts',(3.80569292631823,-0.158333333333333,
5.21522728291445));
#51178=CARTESIAN_POINT('Ctrl Pts',(3.79491029823192,0.158333333333334,5.19503577853373));
#51179=CARTESIAN_POINT('Ctrl Pts',(3.80871919091485,0.319434907277169,5.17060237547614));
#51180=CARTESIAN_POINT('Ctrl Pts',(3.85755031629569,0.636309800095207,5.10874318097783));
#51181=CARTESIAN_POINT('Ctrl Pts',(3.89921906501687,0.794772684000841,5.06307537622152));
#51182=CARTESIAN_POINT('Ctrl Pts',(3.988349596926,1.06847604194572,4.98286049811985));
#51183=CARTESIAN_POINT('Ctrl Pts',(4.033643981749,1.18514270861299,4.945453426566));
#51184=CARTESIAN_POINT('Ctrl Pts',(4.08565144674312,1.30000000000179,4.90536133193446));
#51185=CARTESIAN_POINT('Ctrl Pts',(4.22679133883142,-1.30000000000012,5.08754453791729));
#51186=CARTESIAN_POINT('Ctrl Pts',(4.17306496523607,-1.18514270861186,5.10773194716304));
#51187=CARTESIAN_POINT('Ctrl Pts',(4.12380529594997,-1.06847604194515,5.12539098632623));
#51188=CARTESIAN_POINT('Ctrl Pts',(4.02032458605148,-0.794772684000849,
5.1603458587825));
#51189=CARTESIAN_POINT('Ctrl Pts',(3.96318443294295,-0.636309800095198,
5.17933184465802));
#51190=CARTESIAN_POINT('Ctrl Pts',(3.89004562735247,-0.31943490727716,5.19434297850385));
#51191=CARTESIAN_POINT('Ctrl Pts',(3.86230316271858,-0.158333333333333,
5.19773408440576));
#51192=CARTESIAN_POINT('Ctrl Pts',(3.85110134256581,0.158333333333335,5.17666779739711));
#51193=CARTESIAN_POINT('Ctrl Pts',(3.86811858072083,0.319434907277172,5.15318648826755));
#51194=CARTESIAN_POINT('Ctrl Pts',(3.91746929822009,0.636309800095212,5.09327663222656));
#51195=CARTESIAN_POINT('Ctrl Pts',(3.9613474480484,0.794772684000842,5.04908300808404));
#51196=CARTESIAN_POINT('Ctrl Pts',(4.0427970212933,1.06847604194573,4.97242114815261));
#51197=CARTESIAN_POINT('Ctrl Pts',(4.08259446846774,1.185142708613,4.93685566114292));
#51198=CARTESIAN_POINT('Ctrl Pts',(4.12693286056292,1.3000000000018,4.89890876568608));
#51199=CARTESIAN_POINT('Ctrl Pts',(4.26662860959375,-1.30000000000012,5.08602638006158));
#51200=CARTESIAN_POINT('Ctrl Pts',(4.22064492887383,-1.18514270861187,5.10567179853889));
#51201=CARTESIAN_POINT('Ctrl Pts',(4.1769425473203,-1.06847604194516,5.1226133871387));
#51202=CARTESIAN_POINT('Ctrl Pts',(4.08125156074687,-0.79477268400086,5.15550545804108));
#51203=CARTESIAN_POINT('Ctrl Pts',(4.02203334074001,-0.636309800095201,
5.17254930925954));
#51204=CARTESIAN_POINT('Ctrl Pts',(3.9482250533704,-0.31943490727716,5.18500429751723));
#51205=CARTESIAN_POINT('Ctrl Pts',(3.91730131763066,-0.158333333333334,
5.18704892685074));
#51206=CARTESIAN_POINT('Ctrl Pts',(3.90552730303133,0.158333333333335,5.16460377015688));
#51207=CARTESIAN_POINT('Ctrl Pts',(3.9249029836412,0.319434907277171,5.14060546316211));
#51208=CARTESIAN_POINT('Ctrl Pts',(3.97426818785949,0.636309800095211,5.0814301994222));
#51209=CARTESIAN_POINT('Ctrl Pts',(4.02015060433034,0.794772684000846,5.03849229416171));
#51210=CARTESIAN_POINT('Ctrl Pts',(4.09419024093476,1.06847604194573,4.96458973189248));
#51211=CARTESIAN_POINT('Ctrl Pts',(4.12875752178953,1.185142708613,4.93050993642205));
#51212=CARTESIAN_POINT('Ctrl Pts',(4.16584306825184,1.3000000000018,4.89434002632783));
#51213=CARTESIAN_POINT('Ctrl Pts',(4.30412671312965,-1.30000000000013,5.08697688034835));
#51214=CARTESIAN_POINT('Ctrl Pts',(4.26520156315833,-1.18514270861187,5.10587992951633));
#51215=CARTESIAN_POINT('Ctrl Pts',(4.22656223259812,-1.06847604194517,5.12197699053405));
#51216=CARTESIAN_POINT('Ctrl Pts',(4.13795794925005,-0.794772684000862,
5.1526820277279));
#51217=CARTESIAN_POINT('Ctrl Pts',(4.07675900440676,-0.636309800095203,
5.16780866837543));
#51218=CARTESIAN_POINT('Ctrl Pts',(4.00244493151388,-0.31943490727716,5.17812328554403));
#51219=CARTESIAN_POINT('Ctrl Pts',(3.96881555197009,-0.158333333333333,
5.17941069446765));
#51220=CARTESIAN_POINT('Ctrl Pts',(3.956710122217,0.158333333333335,5.15609672050486));
#51221=CARTESIAN_POINT('Ctrl Pts',(3.97834621812703,0.319434907277169,5.13176330863161));
#51222=CARTESIAN_POINT('Ctrl Pts',(4.02777396866241,0.63630980009521,5.07341396750342));
#51223=CARTESIAN_POINT('Ctrl Pts',(4.07553836165738,0.794772684000846,5.03190523626189));
#51224=CARTESIAN_POINT('Ctrl Pts',(4.14251703231831,1.06847604194573,4.95996175355017));
#51225=CARTESIAN_POINT('Ctrl Pts',(4.17210106068191,1.185142708613,4.92680230509333));
#51226=CARTESIAN_POINT('Ctrl Pts',(4.20227653268427,1.30000000000181,4.89162507607687));
#51227=CARTESIAN_POINT('Ctrl Pts',(4.32877752354224,-1.30000000000013,5.08656709641375));
#51228=CARTESIAN_POINT('Ctrl Pts',(4.29471764204734,-1.18514270861187,5.10547876627365));
#51229=CARTESIAN_POINT('Ctrl Pts',(4.25957139147602,-1.06847604194517,5.12137741460555));
#51230=CARTESIAN_POINT('Ctrl Pts',(4.17586679177897,-0.794772684000861,
5.15114579028333));
#51231=CARTESIAN_POINT('Ctrl Pts',(4.11335372953131,-0.636309800095201,
5.16493876231558));
#51232=CARTESIAN_POINT('Ctrl Pts',(4.03865680925113,-0.319434907277159,
5.17369177464462));
#51233=CARTESIAN_POINT('Ctrl Pts',(4.00300143242074,-0.158333333333333,
5.17389121757444));
#51234=CARTESIAN_POINT('Ctrl Pts',(3.9907467253463,0.158333333333335,5.15019805216469));
#51235=CARTESIAN_POINT('Ctrl Pts',(4.01427473292349,0.319434907277171,5.12668534350072));
#51236=CARTESIAN_POINT('Ctrl Pts',(4.06375031928799,0.636309800095211,5.06889723091102));
#51237=CARTESIAN_POINT('Ctrl Pts',(4.11240127141197,0.794772684000843,5.02732095624963));
#51238=CARTESIAN_POINT('Ctrl Pts',(4.17454632702921,1.06847604194573,4.95635231974399));
#51239=CARTESIAN_POINT('Ctrl Pts',(4.20079656480992,1.185142708613,4.92378719688524));
#51240=CARTESIAN_POINT('Ctrl Pts',(4.22639674849581,1.3000000000018,4.88937664426398));
#51241=CARTESIAN_POINT('Ctrl Pts',(4.36338436399257,-1.30000000000013,5.0884218903031));
#51242=CARTESIAN_POINT('Ctrl Pts',(4.33592664886913,-1.18514270861187,5.10718352049792));
#51243=CARTESIAN_POINT('Ctrl Pts',(4.30552726312009,-1.06847604194517,5.12269850082007));
#51244=CARTESIAN_POINT('Ctrl Pts',(4.2285027530392,-0.794772684000863,5.15104079842947));
#51245=CARTESIAN_POINT('Ctrl Pts',(4.16422516240804,-0.636309800095203,
5.16303243823351));
#51246=CARTESIAN_POINT('Ctrl Pts',(4.08910985640763,-0.319434907277161,
5.16978297911069));
#51247=CARTESIAN_POINT('Ctrl Pts',(4.0509544209241,-0.158333333333334,5.16908627269049));
#51248=CARTESIAN_POINT('Ctrl Pts',(4.03832107969072,0.158333333333335,5.14431580914702));
#51249=CARTESIAN_POINT('Ctrl Pts',(4.06381919631585,0.319434907277169,5.12028774054229));
#51250=CARTESIAN_POINT('Ctrl Pts',(4.11325013655031,0.636309800095211,5.06298848473702));
#51251=CARTESIAN_POINT('Ctrl Pts',(4.16369137852978,0.794772684000846,5.02290141665623));
#51252=CARTESIAN_POINT('Ctrl Pts',(4.21914030658468,1.06847604194574,4.95309282287407));
#51253=CARTESIAN_POINT('Ctrl Pts',(4.24067397323001,1.185142708613,4.92094784529199));
#51254=CARTESIAN_POINT('Ctrl Pts',(4.25973952015092,1.30000000000181,4.88687544371288));
#51255=CARTESIAN_POINT('Ctrl Pts',(4.40081792825242,-1.30000000000013,5.08960668509033));
#51256=CARTESIAN_POINT('Ctrl Pts',(4.38060481916243,-1.18514270861188,5.10838195576156));
#51257=CARTESIAN_POINT('Ctrl Pts',(4.3554607296501,-1.06847604194517,5.12374749427031));
#51258=CARTESIAN_POINT('Ctrl Pts',(4.28598130160392,-0.794772684000866,
5.15136779868103));
#51259=CARTESIAN_POINT('Ctrl Pts',(4.22020498737131,-0.636309800095208,
5.16269876035965));
#51260=CARTESIAN_POINT('Ctrl Pts',(4.14472081457194,-0.319434907277165,
5.16748862079014));
#51261=CARTESIAN_POINT('Ctrl Pts',(4.10344384562433,-0.158333333333335,
5.16455139316179));
#51262=CARTESIAN_POINT('Ctrl Pts',(4.09045892148647,0.158333333333337,5.13868911700679));
#51263=CARTESIAN_POINT('Ctrl Pts',(4.11858576847778,0.319434907277171,5.11543355955347));
#51264=CARTESIAN_POINT('Ctrl Pts',(4.16795708181541,0.636309800095216,5.05863732762711));
#51265=CARTESIAN_POINT('Ctrl Pts',(4.21978800755112,0.794772684000854,5.01868454107607));
#51266=CARTESIAN_POINT('Ctrl Pts',(4.26791808824448,1.06847604194575,4.95004897516277));
#51267=CARTESIAN_POINT('Ctrl Pts',(4.28440774598148,1.18514270861301,4.9185943220005));
#51268=CARTESIAN_POINT('Ctrl Pts',(4.29655333291852,1.30000000000182,4.88539480896152));
#51269=CARTESIAN_POINT('Ctrl Pts',(4.43869075631515,-1.30000000000014,5.09244705574098));
#51270=CARTESIAN_POINT('Ctrl Pts',(4.4259039117771,-1.18514270861188,5.11197858778474));
#51271=CARTESIAN_POINT('Ctrl Pts',(4.40609614803908,-1.06847604194518,5.12754664347477));
#51272=CARTESIAN_POINT('Ctrl Pts',(4.34411652339266,-0.794772684000867,
5.1543555432298));
#51273=CARTESIAN_POINT('Ctrl Pts',(4.27619860307338,-0.636309800095207,
5.16276898456766));
#51274=CARTESIAN_POINT('Ctrl Pts',(4.20048954849266,-0.319434907277163,
5.16588018400511));
#51275=CARTESIAN_POINT('Ctrl Pts',(4.15691369948975,-0.158333333333335,
5.16316308628125));
#51276=CARTESIAN_POINT('Ctrl Pts',(4.14373089636936,0.158333333333337,5.13666783959865));
#51277=CARTESIAN_POINT('Ctrl Pts',(4.17396099819442,0.319434907277173,5.11269068694486));
#51278=CARTESIAN_POINT('Ctrl Pts',(4.22314953732488,0.636309800095217,5.05601593393405));
#51279=CARTESIAN_POINT('Ctrl Pts',(4.27671605343378,0.794772684000851,5.01714584195804));
#51280=CARTESIAN_POINT('Ctrl Pts',(4.31731758874883,1.06847604194574,4.94901350491504));
#51281=CARTESIAN_POINT('Ctrl Pts',(4.32857128559891,1.18514270861301,4.91766527313274));
#51282=CARTESIAN_POINT('Ctrl Pts',(4.33350377909629,1.30000000000182,4.88446077372224));
#51283=CARTESIAN_POINT('Ctrl Pts',(4.46694355687885,-1.30000000000014,5.09421253927619));
#51284=CARTESIAN_POINT('Ctrl Pts',(4.4596064259396,-1.18514270861189,5.11394876273183));
#51285=CARTESIAN_POINT('Ctrl Pts',(4.44377954862526,-1.06847604194518,5.12962974440685));
#51286=CARTESIAN_POINT('Ctrl Pts',(4.38760328337876,-0.794772684000872,
5.15648752928424));
#51287=CARTESIAN_POINT('Ctrl Pts',(4.3187730302285,-0.636309800095212,5.16507039195884));
#51288=CARTESIAN_POINT('Ctrl Pts',(4.24292776592144,-0.319434907277166,
5.16702937530694));
#51289=CARTESIAN_POINT('Ctrl Pts',(4.19702442005355,-0.158333333333336,
5.16242417342549));
#51290=CARTESIAN_POINT('Ctrl Pts',(4.18354609357958,0.158333333333338,5.13489369752115));
#51291=CARTESIAN_POINT('Ctrl Pts',(4.21564175361208,0.319434907277175,5.11124266511601));
#51292=CARTESIAN_POINT('Ctrl Pts',(4.26470351866793,0.636309800095221,5.05468440217912));
#51293=CARTESIAN_POINT('Ctrl Pts',(4.31937178111756,0.794772684000859,5.01609861444084));
#51294=CARTESIAN_POINT('Ctrl Pts',(4.35431037108749,1.06847604194575,4.94825399957144));
#51295=CARTESIAN_POINT('Ctrl Pts',(4.36166410385363,1.18514270861302,4.91702696257548));
#51296=CARTESIAN_POINT('Ctrl Pts',(4.36124794839026,1.30000000000182,4.88394030846984));
#51297=CARTESIAN_POINT('Ctrl Pts',(4.48436618663496,-1.30000000000014,5.09588490856402));
#51298=CARTESIAN_POINT('Ctrl Pts',(4.4804099567393,-1.18514270861189,5.11595623744478));
#51299=CARTESIAN_POINT('Ctrl Pts',(4.46703110461135,-1.06847604194518,5.1317821487358));
#51300=CARTESIAN_POINT('Ctrl Pts',(4.41435513741988,-0.794772684000872,
5.15853540585559));
#51301=CARTESIAN_POINT('Ctrl Pts',(4.34476889322958,-0.636309800095214,
5.16651743138278));
#51302=CARTESIAN_POINT('Ctrl Pts',(4.26877059680495,-0.319434907277168,
5.16749990384559));
#51303=CARTESIAN_POINT('Ctrl Pts',(4.22147324109189,-0.158333333333337,
5.16179550010107));
#51304=CARTESIAN_POINT('Ctrl Pts',(4.20790626770664,0.158333333333339,5.13392436678544));
#51305=CARTESIAN_POINT('Ctrl Pts',(4.24125663852064,0.319434907277176,5.11088979094392));
#51306=CARTESIAN_POINT('Ctrl Pts',(4.29039404310591,0.636309800095223,5.05490356707114));
#51307=CARTESIAN_POINT('Ctrl Pts',(4.34592397091069,0.794772684000863,5.01707090348525));
#51308=CARTESIAN_POINT('Ctrl Pts',(4.37732508768174,1.06847604194575,4.94914432789985));
#51309=CARTESIAN_POINT('Ctrl Pts',(4.38219364604858,1.18514270861302,4.91766097371381));
#51310=CARTESIAN_POINT('Ctrl Pts',(4.37833838285809,1.30000000000183,4.88409716298504));
#51311=CARTESIAN_POINT('Ctrl Pts',(4.49070400846268,-1.30000000000014,5.09652071259581));
#51312=CARTESIAN_POINT('Ctrl Pts',(4.48798825337379,-1.18514270861189,5.1167655310822));
#51313=CARTESIAN_POINT('Ctrl Pts',(4.47550560194655,-1.06847604194518,5.13267131386532));
#51314=CARTESIAN_POINT('Ctrl Pts',(4.42410469560128,-0.794772684000872,
5.15939281353954));
#51315=CARTESIAN_POINT('Ctrl Pts',(4.35421254555806,-0.636309800095214,
5.1670173368963));
#51316=CARTESIAN_POINT('Ctrl Pts',(4.27817340285055,-0.319434907277168,
5.16768424858849));
#51317=CARTESIAN_POINT('Ctrl Pts',(4.23043444623617,-0.158333333333337,
5.16181148227735));
#51318=CARTESIAN_POINT('Ctrl Pts',(4.21681702784594,0.158333333333338,5.13375826922441));
#51319=CARTESIAN_POINT('Ctrl Pts',(4.25055057292307,0.319434907277175,5.110698391497));
#51320=CARTESIAN_POINT('Ctrl Pts',(4.29964232896039,0.636309800095222,5.05468044231088));
#51321=CARTESIAN_POINT('Ctrl Pts',(4.35540993324731,0.794772684000862,5.0168849790298));
#51322=CARTESIAN_POINT('Ctrl Pts',(4.38554641430621,1.06847604194575,4.94899736917052));
#51323=CARTESIAN_POINT('Ctrl Pts',(4.38954737955112,1.18514270861302,4.9175353766224));
#51324=CARTESIAN_POINT('Ctrl Pts',(4.38450434405719,1.30000000000183,4.88399742235045));
#51325=CARTESIAN_POINT('Ctrl Pts',(4.49706625050769,-1.30000000000014,5.09725490143989));
#51326=CARTESIAN_POINT('Ctrl Pts',(4.49561313210597,-1.18514270861189,5.11776177368923));
#51327=CARTESIAN_POINT('Ctrl Pts',(4.48403718193686,-1.06847604194518,5.13379000112895));
#51328=CARTESIAN_POINT('Ctrl Pts',(4.43390865483705,-0.794772684000871,
5.16047184749054));
#51329=CARTESIAN_POINT('Ctrl Pts',(4.3636497831239,-0.636309800095214,5.16750626028728));
#51330=CARTESIAN_POINT('Ctrl Pts',(4.28756531497726,-0.319434907277168,
5.16783169026165));
#51331=CARTESIAN_POINT('Ctrl Pts',(4.23942987235426,-0.158333333333337,
5.16194741269489));
#51332=CARTESIAN_POINT('Ctrl Pts',(4.22577045208385,0.158333333333338,5.13373942688524));
#51333=CARTESIAN_POINT('Ctrl Pts',(4.25987060472629,0.319434907277175,5.11059656273882));
#51334=CARTESIAN_POINT('Ctrl Pts',(4.30889743682903,0.636309800095223,5.05448205830684));
#51335=CARTESIAN_POINT('Ctrl Pts',(4.36487767719341,0.794772684000863,5.01664278826843));
#51336=CARTESIAN_POINT('Ctrl Pts',(4.39374659513668,1.06847604194575,4.94878339216866));
#51337=CARTESIAN_POINT('Ctrl Pts',(4.39688482303203,1.18514270861302,4.9173578773307));
#51338=CARTESIAN_POINT('Ctrl Pts',(4.39066499394388,1.30000000000183,4.88388066578801));
#51339=CARTESIAN_POINT('Ctrl Pts',(4.50342826126824,-1.30000000000014,5.09799890728752));
#51340=CARTESIAN_POINT('Ctrl Pts',(4.5032420856426,-1.18514270861189,5.11878887146126));
#51341=CARTESIAN_POINT('Ctrl Pts',(4.49257623194904,-1.06847604194518,5.13495548473586));
#51342=CARTESIAN_POINT('Ctrl Pts',(4.44372582343088,-0.794772684000872,
5.16162273004491));
#51343=CARTESIAN_POINT('Ctrl Pts',(4.37309890724761,-0.636309800095214,
5.16806100431414));
#51344=CARTESIAN_POINT('Ctrl Pts',(4.29697528558695,-0.319434907277168,
5.16806105128099));
#51345=CARTESIAN_POINT('Ctrl Pts',(4.24845291887343,-0.158333333333336,
5.16218849036971));
#51346=CARTESIAN_POINT('Ctrl Pts',(4.23475258734916,0.158333333333338,5.13382616185956));
#51347=CARTESIAN_POINT('Ctrl Pts',(4.26921358881558,0.319434907277174,5.11058481137938));
#51348=CARTESIAN_POINT('Ctrl Pts',(4.31816602131599,0.636309800095222,5.05434366360625));
#51349=CARTESIAN_POINT('Ctrl Pts',(4.37434838324022,0.794772684000862,5.01642824211172));
#51350=CARTESIAN_POINT('Ctrl Pts',(4.40194351193221,1.06847604194575,4.94857304605718));
#51351=CARTESIAN_POINT('Ctrl Pts',(4.40421791446416,1.18514270861302,4.91717758007938));
#51352=CARTESIAN_POINT('Ctrl Pts',(4.39682181081755,1.30000000000183,4.88375864821306));
#51353=CARTESIAN_POINT('Ctrl Pts',(4.5089703151262,-1.30000000000014,5.09855433356514));
#51354=CARTESIAN_POINT('Ctrl Pts',(4.50986730449823,-1.18514270861189,5.1194902140667));
#51355=CARTESIAN_POINT('Ctrl Pts',(4.49998765777042,-1.06847604194518,5.13573692231672));
#51356=CARTESIAN_POINT('Ctrl Pts',(4.45226751216336,-0.794772684000871,
5.16243714255034));
#51357=CARTESIAN_POINT('Ctrl Pts',(4.38140730018764,-0.636309800095213,
5.1687021689243));
#51358=CARTESIAN_POINT('Ctrl Pts',(4.30525623160429,-0.319434907277168,
5.1684501436253));
#51359=CARTESIAN_POINT('Ctrl Pts',(4.25631839326472,-0.158333333333336,
5.16230199422985));
#51360=CARTESIAN_POINT('Ctrl Pts',(4.24258473667234,0.158333333333338,5.13380593151017));
#51361=CARTESIAN_POINT('Ctrl Pts',(4.2774154453425,0.319434907277175,5.11066851664683));
#51362=CARTESIAN_POINT('Ctrl Pts',(4.32635278207021,0.636309800095222,5.05448427175959));
#51363=CARTESIAN_POINT('Ctrl Pts',(4.38276986346915,0.794772684000862,5.01668834541608));
#51364=CARTESIAN_POINT('Ctrl Pts',(4.40922659624202,1.06847604194575,4.94876025066249));
#51365=CARTESIAN_POINT('Ctrl Pts',(4.4107134089054,1.18514270861302,4.91728834502899));
#51366=CARTESIAN_POINT('Ctrl Pts',(4.40223489493331,1.30000000000183,4.88374808899692));
#51367=CARTESIAN_POINT('Ctrl Pts',(4.51173593338493,-1.30000000000014,5.0988119602196));
#51368=CARTESIAN_POINT('Ctrl Pts',(4.51316878410743,-1.18514270861189,5.11979885946483));
#51369=CARTESIAN_POINT('Ctrl Pts',(4.50367993561254,-1.06847604194518,5.136076882354));
#51370=CARTESIAN_POINT('Ctrl Pts',(4.4565274872811,-0.794772684000871,5.16280392524531));
#51371=CARTESIAN_POINT('Ctrl Pts',(4.38556942968062,-0.636309800095214,
5.16905517158179));
#51372=CARTESIAN_POINT('Ctrl Pts',(4.30940797613757,-0.319434907277168,
5.16869064712411));
#51373=CARTESIAN_POINT('Ctrl Pts',(4.26025013011133,-0.158333333333336,
5.16235872701826));
#51374=CARTESIAN_POINT('Ctrl Pts',(4.24649955259772,0.158333333333338,5.13379357096223));
#51375=CARTESIAN_POINT('Ctrl Pts',(4.28152116181099,0.319434907277174,5.11072957108493));
#51376=CARTESIAN_POINT('Ctrl Pts',(4.33045923925767,0.636309800095221,5.0546011357185));
#51377=CARTESIAN_POINT('Ctrl Pts',(4.38700624373682,0.794772684000862,5.01690598005947));
#51378=CARTESIAN_POINT('Ctrl Pts',(4.41289071606697,1.06847604194575,4.94893059205468));
#51379=CARTESIAN_POINT('Ctrl Pts',(4.41397847476729,1.18514270861302,4.91740271407581));
#51380=CARTESIAN_POINT('Ctrl Pts',(4.40494956321041,1.30000000000183,4.88377098484906));
#51381=CARTESIAN_POINT('Ctrl Pts',(4.51331549988098,-1.30000000000014,5.09895634230767));
#51382=CARTESIAN_POINT('Ctrl Pts',(4.51505386685927,-1.18514270861189,5.11996963318523));
#51383=CARTESIAN_POINT('Ctrl Pts',(4.50578809552361,-1.06847604194518,5.13626457196588));
#51384=CARTESIAN_POINT('Ctrl Pts',(4.45896054925151,-0.794772684000871,
5.16300880309351));
#51385=CARTESIAN_POINT('Ctrl Pts',(4.38794960734779,-0.636309800095214,
5.16926379970333));
#51386=CARTESIAN_POINT('Ctrl Pts',(4.31178198849649,-0.319434907277168,
5.1688343464384));
#51387=CARTESIAN_POINT('Ctrl Pts',(4.26249479831643,-0.158333333333336,
5.1623841728602));
#51388=CARTESIAN_POINT('Ctrl Pts',(4.24873474873611,0.158333333333338,5.1337799496331));
#51389=CARTESIAN_POINT('Ctrl Pts',(4.28386868929949,0.319434907277174,5.11076930433508));
#51390=CARTESIAN_POINT('Ctrl Pts',(4.33280899807485,0.636309800095221,5.05467883811918));
#51391=CARTESIAN_POINT('Ctrl Pts',(4.38943094971871,0.794772684000862,5.01704314978778));
#51392=CARTESIAN_POINT('Ctrl Pts',(4.41498744433985,1.06847604194575,4.94903762837009));
#51393=CARTESIAN_POINT('Ctrl Pts',(4.41584622184238,1.18514270861302,4.91747476919486));
#51394=CARTESIAN_POINT('Ctrl Pts',(4.40650131728738,1.30000000000183,4.88378612121329));
#51395=CARTESIAN_POINT('Ctrl Pts',(4.52673420369595,-1.30000000000014,5.10015672069679));
#51396=CARTESIAN_POINT('Ctrl Pts',(4.53105886446733,-1.18514270861189,5.12135679964457));
#51397=CARTESIAN_POINT('Ctrl Pts',(4.52368495272715,-1.06847604194518,5.13778140892107));
#51398=CARTESIAN_POINT('Ctrl Pts',(4.47962369866828,-0.79477268400087,5.16469325181154));
#51399=CARTESIAN_POINT('Ctrl Pts',(4.40818825363879,-0.636309800095212,
5.17107852727311));
#51400=CARTESIAN_POINT('Ctrl Pts',(4.33199311210111,-0.319434907277167,
5.17018879965183));
#51401=CARTESIAN_POINT('Ctrl Pts',(4.28162985675607,-0.158333333333336,
5.16281249744401));
#51402=CARTESIAN_POINT('Ctrl Pts',(4.2677871536587,0.158333333333338,5.13386585357558));
#51403=CARTESIAN_POINT('Ctrl Pts',(4.30383451681207,0.319434907277172,5.11116134357201));
#51404=CARTESIAN_POINT('Ctrl Pts',(4.35279692096245,0.636309800095219,5.05539906111259));
#51405=CARTESIAN_POINT('Ctrl Pts',(4.41010452611587,0.79477268400086,5.01843725806858));
#51406=CARTESIAN_POINT('Ctrl Pts',(4.43287946120475,1.06847604194575,4.95018778605438));
#51407=CARTESIAN_POINT('Ctrl Pts',(4.43178623420622,1.18514270861302,4.91830230319173));
#51408=CARTESIAN_POINT('Ctrl Pts',(4.41974135470369,1.30000000000183,4.88407400500928));
#51409=CARTESIAN_POINT('Ctrl Pts',(4.55257517464123,-1.30000000000013,5.1033102584444));
#51410=CARTESIAN_POINT('Ctrl Pts',(4.56204421640626,-1.18514270861187,5.12573190702204));
#51411=CARTESIAN_POINT('Ctrl Pts',(4.55838559416382,-1.06847604194517,5.14283935276507));
#51412=CARTESIAN_POINT('Ctrl Pts',(4.5196059148415,-0.794772684000862,5.17008410311367));
#51413=CARTESIAN_POINT('Ctrl Pts',(4.44686892664056,-0.636309800095204,
5.17472119164269));
#51414=CARTESIAN_POINT('Ctrl Pts',(4.37054149862908,-0.319434907277161,
5.17255733923234));
#51415=CARTESIAN_POINT('Ctrl Pts',(4.31841632073828,-0.158333333333334,
5.16446413815593));
#51416=CARTESIAN_POINT('Ctrl Pts',(4.30443648682053,0.158333333333336,5.13493687844417));
#51417=CARTESIAN_POINT('Ctrl Pts',(4.342177815926,0.319434907277172,5.11266026279369));
#51418=CARTESIAN_POINT('Ctrl Pts',(4.39085227802371,0.636309800095214,5.05639544117813));
#51419=CARTESIAN_POINT('Ctrl Pts',(4.44873093967267,0.794772684000848,5.01824254835966));
#51420=CARTESIAN_POINT('Ctrl Pts',(4.46636449056368,1.06847604194574,4.94999476957805));
#51421=CARTESIAN_POINT('Ctrl Pts',(4.46183091987552,1.185142708613,4.91839135385537));
#51422=CARTESIAN_POINT('Ctrl Pts',(4.44513086770591,1.30000000000181,4.8847264570152));
#51423=CARTESIAN_POINT('Ctrl Pts',(4.57797014782441,-1.30000000000011,5.10637392230933));
#51424=CARTESIAN_POINT('Ctrl Pts',(4.59241718008651,-1.18514270861186,5.12973339069855));
#51425=CARTESIAN_POINT('Ctrl Pts',(4.5923750883925,-1.06847604194515,5.14740422222097));
#51426=CARTESIAN_POINT('Ctrl Pts',(4.55880507328097,-0.794772684000851,
5.17508548890529));
#51427=CARTESIAN_POINT('Ctrl Pts',(4.48498896022061,-0.636309800095197,
5.17877438662047));
#51428=CARTESIAN_POINT('Ctrl Pts',(4.40861628632669,-0.319434907277159,
5.17565787022847));
#51429=CARTESIAN_POINT('Ctrl Pts',(4.35474635534816,-0.158333333333332,
5.16675378500001));
#51430=CARTESIAN_POINT('Ctrl Pts',(4.34059295810105,0.158333333333334,5.1364765704601));
#51431=CARTESIAN_POINT('Ctrl Pts',(4.3797744155812,0.319434907277167,5.11381935642279));
#51432=CARTESIAN_POINT('Ctrl Pts',(4.42840755015826,0.636309800095206,5.05787895495823));
#51433=CARTESIAN_POINT('Ctrl Pts',(4.48773430817404,0.79477268400084,5.02157383053672));
#51434=CARTESIAN_POINT('Ctrl Pts',(4.50009761851211,1.06847604194573,4.95268677460948));
#51435=CARTESIAN_POINT('Ctrl Pts',(4.49184486495928,1.18514270861299,4.92027496910602));
#51436=CARTESIAN_POINT('Ctrl Pts',(4.46998773891406,1.3000000000018,4.88527001209309));
#51437=CARTESIAN_POINT('Ctrl Pts',(4.59077270268395,-1.30000000000011,5.10832931194405));
#51438=CARTESIAN_POINT('Ctrl Pts',(4.60766161389344,-1.18514270861186,5.13199826094758));
#51439=CARTESIAN_POINT('Ctrl Pts',(4.60940251578961,-1.06847604194515,5.14987106382229));
#51440=CARTESIAN_POINT('Ctrl Pts',(4.57842941557334,-0.794772684000851,
5.17777055683221));
#51441=CARTESIAN_POINT('Ctrl Pts',(4.50418204215329,-0.636309800095197,
5.1814197357197));
#51442=CARTESIAN_POINT('Ctrl Pts',(4.42777734501206,-0.319434907277159,
5.17777988362783));
#51443=CARTESIAN_POINT('Ctrl Pts',(4.37292795574625,-0.158333333333332,
5.16801756977584));
#51444=CARTESIAN_POINT('Ctrl Pts',(4.35867257917562,0.158333333333334,5.13728168805675));
#51445=CARTESIAN_POINT('Ctrl Pts',(4.39869447984769,0.319434907277167,5.11487935011378));
#51446=CARTESIAN_POINT('Ctrl Pts',(4.44722735233343,0.636309800095206,5.05882272597048));
#51447=CARTESIAN_POINT('Ctrl Pts',(4.50695309467615,0.79477268400084,5.02233268407818));
#51448=CARTESIAN_POINT('Ctrl Pts',(4.51674956614749,1.06847604194573,4.95329826442052));
#51449=CARTESIAN_POINT('Ctrl Pts',(4.50675280587869,1.18514270861299,4.9208376091363));
#51450=CARTESIAN_POINT('Ctrl Pts',(4.48251875583617,1.3000000000018,4.88579874086039));
#51451=CARTESIAN_POINT('',(4.3897288827106,1.2,4.91247287747308));
#51452=CARTESIAN_POINT('Ctrl Pts',(4.3897288827106,1.2,4.91247287747308));
#51453=CARTESIAN_POINT('Ctrl Pts',(4.36857135610553,1.21681573945508,4.90825963985616));
#51454=CARTESIAN_POINT('Ctrl Pts',(4.3473023706465,1.23325593210168,4.90314947462289));
#51455=CARTESIAN_POINT('Ctrl Pts',(4.2998391327148,1.27069836523098,4.89364883337151));
#51456=CARTESIAN_POINT('Ctrl Pts',(4.28243988954012,1.28442464637428,4.89030656849232));
#51457=CARTESIAN_POINT('Ctrl Pts',(4.26287719563543,1.30000000000181,4.88691158514987));
#51458=CARTESIAN_POINT('',(4.45989076534562,0.653834841370385,5.05247250056665));
#51459=CARTESIAN_POINT('Ctrl Pts',(4.45989076537646,0.653834841369131,5.05247250054632));
#51460=CARTESIAN_POINT('Ctrl Pts',(4.45288492245741,0.717482042443765,5.03792307375374));
#51461=CARTESIAN_POINT('Ctrl Pts',(4.44711302933054,0.764209734534401,5.02607170794616));
#51462=CARTESIAN_POINT('Ctrl Pts',(4.42420943059583,0.949856843367683,4.97961640082602));
#51463=CARTESIAN_POINT('Ctrl Pts',(4.41030972125718,1.0567232552086,4.95196718576286));
#51464=CARTESIAN_POINT('Ctrl Pts',(4.3897288827106,1.2,4.91247287747308));
#51465=CARTESIAN_POINT('',(4.51863764645995,-0.653834841531101,5.17900672440632));
#51466=CARTESIAN_POINT('Ctrl Pts',(4.51863764645995,-0.6538348415311,5.17900672440632));
#51467=CARTESIAN_POINT('Ctrl Pts',(4.47706947811755,-0.575982437876214,
5.17841861144383));
#51468=CARTESIAN_POINT('Ctrl Pts',(4.44193277695744,-0.493637398627582,
5.17716781668147));
#51469=CARTESIAN_POINT('Ctrl Pts',(4.39149855918852,-0.338135451747832,
5.17291766455466));
#51470=CARTESIAN_POINT('Ctrl Pts',(4.37381733731089,-0.265660868320344,
5.17019185540934));
#51471=CARTESIAN_POINT('Ctrl Pts',(4.35075353763555,-0.129717629145974,
5.16230413532239));
#51472=CARTESIAN_POINT('Ctrl Pts',(4.3439598574373,-0.0666258049312309,
5.15757923333407));
#51473=CARTESIAN_POINT('Ctrl Pts',(4.33801233342096,0.0595444162497744,
5.14565140581426));
#51474=CARTESIAN_POINT('Ctrl Pts',(4.33879948700794,0.122777977220077,5.13836852715898));
#51475=CARTESIAN_POINT('Ctrl Pts',(4.34922857416695,0.2601311288836,5.12044478424126));
#51476=CARTESIAN_POINT('Ctrl Pts',(4.36046089628691,0.333946038931111,5.10943059845951));
#51477=CARTESIAN_POINT('Ctrl Pts',(4.39723462068707,0.491209513290317,5.08375691479056));
#51478=CARTESIAN_POINT('Ctrl Pts',(4.42491373516359,0.574351626734296,5.06856490516704));
#51479=CARTESIAN_POINT('Ctrl Pts',(4.45989076529517,0.653834841386886,5.05247250053849));
#51480=CARTESIAN_POINT('',(4.48868816730329,-1.2,5.11333315148022));
#51481=CARTESIAN_POINT('Ctrl Pts',(4.48868816730329,-1.2,5.11333315148022));
#51482=CARTESIAN_POINT('Ctrl Pts',(4.49330354820273,-1.14227030646505,5.12326142807387));
#51483=CARTESIAN_POINT('Ctrl Pts',(4.49957148427282,-1.06120661874143,5.13679379880293));
#51484=CARTESIAN_POINT('Ctrl Pts',(4.51379468897461,-0.796649462481794,
5.16817211105445));
#51485=CARTESIAN_POINT('Ctrl Pts',(4.51601641408078,-0.739685413249303,
5.17314604221026));
#51486=CARTESIAN_POINT('Ctrl Pts',(4.51863764645995,-0.653834841531101,
5.17900672440632));
#51487=CARTESIAN_POINT('Ctrl Pts',(4.36619448174045,-1.30000000000001,5.08840208666064));
#51488=CARTESIAN_POINT('Ctrl Pts',(4.38689833577429,-1.28301364714831,5.09219695776369));
#51489=CARTESIAN_POINT('Ctrl Pts',(4.40759529208872,-1.26604667874466,5.0961307302198));
#51490=CARTESIAN_POINT('Ctrl Pts',(4.45484463189025,-1.22753397446419,5.10588976509139));
#51491=CARTESIAN_POINT('Ctrl Pts',(4.47022545323923,-1.21477226219745,5.10866030766466));
#51492=CARTESIAN_POINT('Ctrl Pts',(4.48868816730329,-1.2,5.11333315148022));
#51493=CARTESIAN_POINT('Origin',(0.,1.25,7.2));
#51494=CARTESIAN_POINT('Origin',(0.,1.2,7.2));
#51495=CARTESIAN_POINT('Origin',(0.,0.92691742076555,7.2));
#51496=CARTESIAN_POINT('Origin',(0.,0.653834841531101,7.2));
#51497=CARTESIAN_POINT('Origin',(0.,0.,7.2));
#51498=CARTESIAN_POINT('Origin',(0.,-0.653834841531101,7.2));
#51499=CARTESIAN_POINT('Origin',(0.,-0.926917420765551,7.2));
#51500=CARTESIAN_POINT('Origin',(0.,-1.2,7.2));
#51501=CARTESIAN_POINT('Origin',(0.,-1.25,7.2));
#51502=CARTESIAN_POINT('Ctrl Pts',(4.7191771839547,-1.30000000000134,5.41734227325848));
#51503=CARTESIAN_POINT('Ctrl Pts',(4.70935397490593,-1.18514270861269,5.37588728519308));
#51504=CARTESIAN_POINT('Ctrl Pts',(4.69192014516093,-1.06847604194558,5.34673782657451));
#51505=CARTESIAN_POINT('Ctrl Pts',(4.63406245451663,-0.794772684000851,
5.3078249805714));
#51506=CARTESIAN_POINT('Ctrl Pts',(4.56698074651016,-0.636309800095197,
5.32779325308501));
#51507=CARTESIAN_POINT('Ctrl Pts',(4.49284772594841,-0.319434907277159,
5.32635100323535));
#51508=CARTESIAN_POINT('Ctrl Pts',(4.44941966576432,-0.158333333333332,
5.34110298165352));
#51509=CARTESIAN_POINT('Ctrl Pts',(4.43611716307696,0.158333333333334,5.30994285314816));
#51510=CARTESIAN_POINT('Ctrl Pts',(4.46556375515151,0.319434907277167,5.26264955034729));
#51511=CARTESIAN_POINT('Ctrl Pts',(4.51398353922898,0.636309800095206,5.20343425858799));
#51512=CARTESIAN_POINT('Ctrl Pts',(4.56637659762912,0.79477268400084,5.15069948450899));
#51513=CARTESIAN_POINT('Ctrl Pts',(4.60783501082194,1.06847604194514,5.14635039002878));
#51514=CARTESIAN_POINT('Ctrl Pts',(4.61995220105504,1.18514270861184,5.15960337168886));
#51515=CARTESIAN_POINT('Ctrl Pts',(4.62624077063569,1.30000000000009,5.18799189685967));
#51516=CARTESIAN_POINT('Ctrl Pts',(4.71118521909801,-1.30000000000134,5.42700842222637));
#51517=CARTESIAN_POINT('Ctrl Pts',(4.69979673845632,-1.18514270861269,5.38734252398592));
#51518=CARTESIAN_POINT('Ctrl Pts',(4.68123224291413,-1.06847604194558,5.35952180181295));
#51519=CARTESIAN_POINT('Ctrl Pts',(4.62176651442015,-0.794772684000851,
5.32261509441226));
#51520=CARTESIAN_POINT('Ctrl Pts',(4.55508919945685,-0.636309800095197,
5.34241059774211));
#51521=CARTESIAN_POINT('Ctrl Pts',(4.48097546072873,-0.319434907277159,
5.34112062530357));
#51522=CARTESIAN_POINT('Ctrl Pts',(4.43792035696629,-0.158333333333332,
5.35507748731411));
#51523=CARTESIAN_POINT('Ctrl Pts',(4.42489047293298,0.158333333333334,5.32430005246305));
#51524=CARTESIAN_POINT('Ctrl Pts',(4.45431946765656,0.319434907277167,5.27830889605651));
#51525=CARTESIAN_POINT('Ctrl Pts',(4.5031067381983,0.636309800095206,5.21946758214842));
#51526=CARTESIAN_POINT('Ctrl Pts',(4.55524074388928,0.79477268400084,5.16707987407414));
#51527=CARTESIAN_POINT('Ctrl Pts',(4.59827465855659,1.06847604194514,5.16065487381351));
#51528=CARTESIAN_POINT('Ctrl Pts',(4.6114348104173,1.18514270861184,5.17244768779572));
#51529=CARTESIAN_POINT('Ctrl Pts',(4.61912732704296,1.30000000000009,5.19881446030323));
#51530=CARTESIAN_POINT('Ctrl Pts',(4.69494687124662,-1.3000000000016,5.445801977467));
#51531=CARTESIAN_POINT('Ctrl Pts',(4.68127539588664,-1.18514270861292,5.41115438741575));
#51532=CARTESIAN_POINT('Ctrl Pts',(4.66092526233145,-1.06847604194579,5.386812218893));
#51533=CARTESIAN_POINT('Ctrl Pts',(4.59848334629683,-0.794772684001002,
5.35438452529471));
#51534=CARTESIAN_POINT('Ctrl Pts',(4.53116973209331,-0.63630980009532,5.37149271969744));
#51535=CARTESIAN_POINT('Ctrl Pts',(4.45670596000581,-0.319434907277221,
5.36988490694989));
#51536=CARTESIAN_POINT('Ctrl Pts',(4.41494753063121,-0.158333333333363,
5.38309622210191));
#51537=CARTESIAN_POINT('Ctrl Pts',(4.40229724694797,0.158333333333365,5.35285740435751));
#51538=CARTESIAN_POINT('Ctrl Pts',(4.43104909968437,0.319434907277229,5.30854619488518));
#51539=CARTESIAN_POINT('Ctrl Pts',(4.48047089785509,0.63630980009533,5.25031366414003));
#51540=CARTESIAN_POINT('Ctrl Pts',(4.53265817182857,0.794772684000994,5.19946768138508));
#51541=CARTESIAN_POINT('Ctrl Pts',(4.57884238347787,1.06847604194535,5.18885484938565));
#51542=CARTESIAN_POINT('Ctrl Pts',(4.59398697743196,1.18514270861207,5.19755297456347));
#51543=CARTESIAN_POINT('Ctrl Pts',(4.60428473141087,1.30000000000035,5.21954312664747));
#51544=CARTESIAN_POINT('Ctrl Pts',(4.67855760031106,-1.30000000000186,5.46495686707269));
#51545=CARTESIAN_POINT('Ctrl Pts',(4.66120377365009,-1.18514270861316,5.43307420647752));
#51546=CARTESIAN_POINT('Ctrl Pts',(4.63825704955113,-1.068476041946,5.41090735290281));
#51547=CARTESIAN_POINT('Ctrl Pts',(4.57232481446913,-0.794772684001165,
5.38214294453913));
#51548=CARTESIAN_POINT('Ctrl Pts',(4.50650585290617,-0.63630980009545,5.40001639808124));
#51549=CARTESIAN_POINT('Ctrl Pts',(4.43231296648443,-0.319434907277286,
5.39910293902452));
#51550=CARTESIAN_POINT('Ctrl Pts',(4.39132670753068,-0.158333333333395,
5.41071813719325));
#51551=CARTESIAN_POINT('Ctrl Pts',(4.37907887492038,0.158333333333397,5.38106212502469));
#51552=CARTESIAN_POINT('Ctrl Pts',(4.40729214896405,0.319434907277294,5.33867722957612));
#51553=CARTESIAN_POINT('Ctrl Pts',(4.45760677965426,0.636309800095459,5.28145202353281));
#51554=CARTESIAN_POINT('Ctrl Pts',(4.51015579493688,0.794772684001156,5.23263852905263));
#51555=CARTESIAN_POINT('Ctrl Pts',(4.55960657769512,1.06847604194556,5.21792091386001));
#51556=CARTESIAN_POINT('Ctrl Pts',(4.57672612162891,1.18514270861231,5.22344389860329));
#51557=CARTESIAN_POINT('Ctrl Pts',(4.58955979797253,1.30000000000061,5.24086057836533));
#51558=CARTESIAN_POINT('Ctrl Pts',(4.67014172218832,-1.30000000000189,5.4746514904811));
#51559=CARTESIAN_POINT('Ctrl Pts',(4.65141061882585,-1.18514270861319,5.4450466677508));
#51560=CARTESIAN_POINT('Ctrl Pts',(4.62742281607529,-1.06847604194603,5.42448826836267));
#51561=CARTESIAN_POINT('Ctrl Pts',(4.5598621657925,-0.794772684001185,5.39789330073363));
#51562=CARTESIAN_POINT('Ctrl Pts',(4.49404072528191,-0.636309800095465,
5.41489649838808));
#51563=CARTESIAN_POINT('Ctrl Pts',(4.41962544439486,-0.319434907277294,
5.41375469060185));
#51564=CARTESIAN_POINT('Ctrl Pts',(4.37897528911165,-0.158333333333399,
5.42445428554484));
#51565=CARTESIAN_POINT('Ctrl Pts',(4.36691981565501,0.158333333333401,5.39507877025299));
#51566=CARTESIAN_POINT('Ctrl Pts',(4.39512779232409,0.319434907277302,5.35411223658114));
#51567=CARTESIAN_POINT('Ctrl Pts',(4.44577463236498,0.636309800095475,5.29723400018175));
#51568=CARTESIAN_POINT('Ctrl Pts',(4.49796376419975,0.794772684001176,5.24865657877164));
#51569=CARTESIAN_POINT('Ctrl Pts',(4.54909160096736,1.06847604194559,5.23183655050129));
#51570=CARTESIAN_POINT('Ctrl Pts',(4.56734349850341,1.18514270861234,5.23590627755165));
#51571=CARTESIAN_POINT('Ctrl Pts',(4.58171594751187,1.30000000000064,5.2513264986471));
#51572=CARTESIAN_POINT('Ctrl Pts',(4.66975770319508,-1.30000000000189,5.47508963792264));
#51573=CARTESIAN_POINT('Ctrl Pts',(4.6509638121167,-1.18514270861319,5.44558817224115));
#51574=CARTESIAN_POINT('Ctrl Pts',(4.62692864703389,-1.06847604194603,5.42510290197827));
#51575=CARTESIAN_POINT('Ctrl Pts',(4.55929421601096,-0.794772684001185,
5.39860704470745));
#51576=CARTESIAN_POINT('Ctrl Pts',(4.49347380603036,-0.636309800095465,
5.41557246512998));
#51577=CARTESIAN_POINT('Ctrl Pts',(4.41904815444869,-0.319434907277294,
5.41441990348809));
#51578=CARTESIAN_POINT('Ctrl Pts',(4.37841168271835,-0.158333333333399,
5.42507538042472));
#51579=CARTESIAN_POINT('Ctrl Pts',(4.36636475283526,0.158333333333401,5.39571233267948));
#51580=CARTESIAN_POINT('Ctrl Pts',(4.3945733925091,0.319434907277302,5.35481174037171));
#51581=CARTESIAN_POINT('Ctrl Pts',(4.44523618562804,0.636309800095475,5.2979505962091));
#51582=CARTESIAN_POINT('Ctrl Pts',(4.49740972306233,0.794772684001175,5.24938503158791));
#51583=CARTESIAN_POINT('Ctrl Pts',(4.54861403658599,1.06847604194559,5.2324697634132));
#51584=CARTESIAN_POINT('Ctrl Pts',(4.56691733345257,1.18514270861234,5.23647329586455));
#51585=CARTESIAN_POINT('Ctrl Pts',(4.58135947716816,1.30000000000064,5.2518023535876));
#51586=CARTESIAN_POINT('Ctrl Pts',(4.66937366746064,-1.30000000000189,5.47552778045089));
#51587=CARTESIAN_POINT('Ctrl Pts',(4.65051669169493,-1.18514270861319,5.44612915188768));
#51588=CARTESIAN_POINT('Ctrl Pts',(4.62643396503698,-1.06847604194603,5.42571666422186));
#51589=CARTESIAN_POINT('Ctrl Pts',(4.55872551875528,-0.794772684001185,
5.399319517354));
#51590=CARTESIAN_POINT('Ctrl Pts',(4.4929061657213,-0.636309800095465,5.41624725734922));
#51591=CARTESIAN_POINT('Ctrl Pts',(4.41847055766395,-0.319434907277293,
5.415084614726));
#51592=CARTESIAN_POINT('Ctrl Pts',(4.37784863172277,-0.158333333333399,
5.42569733153273));
#51593=CARTESIAN_POINT('Ctrl Pts',(4.3658103170721,0.158333333333401,5.39634687308374));
#51594=CARTESIAN_POINT('Ctrl Pts',(4.394018749592,0.319434907277302,5.35551085962946));
#51595=CARTESIAN_POINT('Ctrl Pts',(4.4446973896353,0.636309800095474,5.29866664025922));
#51596=CARTESIAN_POINT('Ctrl Pts',(4.49685595516693,0.794772684001175,5.25011389565956));
#51597=CARTESIAN_POINT('Ctrl Pts',(4.548136841441,1.06847604194559,5.23310354460809));
#51598=CARTESIAN_POINT('Ctrl Pts',(4.56649148995048,1.18514270861234,5.23704081452944));
#51599=CARTESIAN_POINT('Ctrl Pts',(4.58100319144551,1.30000000000064,5.25227850504666));
#51600=CARTESIAN_POINT('Ctrl Pts',(4.66860424610756,-1.30000000000189,5.47640181124463));
#51601=CARTESIAN_POINT('Ctrl Pts',(4.64962043429344,-1.18514270861319,5.4472078224012));
#51602=CARTESIAN_POINT('Ctrl Pts',(4.62544222348014,-1.06847604194603,5.4269403525071));
#51603=CARTESIAN_POINT('Ctrl Pts',(4.557585618843,-0.794772684001185,5.40074048707532));
#51604=CARTESIAN_POINT('Ctrl Pts',(4.49176959485631,-0.636309800095465,
5.41759484605104));
#51605=CARTESIAN_POINT('Ctrl Pts',(4.4173144942221,-0.319434907277294,5.41641276937917));
#51606=CARTESIAN_POINT('Ctrl Pts',(4.37672145967416,-0.158333333333399,
5.42693966204847));
#51607=CARTESIAN_POINT('Ctrl Pts',(4.36470027204301,0.158333333333401,5.39761426227359));
#51608=CARTESIAN_POINT('Ctrl Pts',(4.39290776017728,0.319434907277302,5.3569066287119));
#51609=CARTESIAN_POINT('Ctrl Pts',(4.44361873976636,0.636309800095475,5.30009724581093));
#51610=CARTESIAN_POINT('Ctrl Pts',(4.49574912285305,0.794772684001176,5.25157279731524));
#51611=CARTESIAN_POINT('Ctrl Pts',(4.54718351306965,1.06847604194559,5.23437279429459));
#51612=CARTESIAN_POINT('Ctrl Pts',(4.56564069312157,1.18514270861234,5.23817726141035));
#51613=CARTESIAN_POINT('Ctrl Pts',(4.58029101153264,1.30000000000064,5.25323143962657));
#51614=CARTESIAN_POINT('Ctrl Pts',(4.66693219276478,-1.30000000000189,5.47828738177555));
#51615=CARTESIAN_POINT('Ctrl Pts',(4.64766935794,-1.18514270861319,5.44952990506921));
#51616=CARTESIAN_POINT('Ctrl Pts',(4.62328180500171,-1.06847604194603,5.42957265493046));
#51617=CARTESIAN_POINT('Ctrl Pts',(4.55510255496264,-0.794772684001184,
5.4037976985262));
#51618=CARTESIAN_POINT('Ctrl Pts',(4.48929899212577,-0.636309800095464,
5.42050187043342));
#51619=CARTESIAN_POINT('Ctrl Pts',(4.41480542526063,-0.319434907277293,
5.41928396473858));
#51620=CARTESIAN_POINT('Ctrl Pts',(4.37427829715946,-0.158333333333399,
5.42963015579167));
#51621=CARTESIAN_POINT('Ctrl Pts',(4.36229409858572,0.158333333333401,5.40035906140909));
#51622=CARTESIAN_POINT('Ctrl Pts',(4.39049315721296,0.319434907277301,5.35991979077081));
#51623=CARTESIAN_POINT('Ctrl Pts',(4.44127621473851,0.636309800095473,5.30318890946986));
#51624=CARTESIAN_POINT('Ctrl Pts',(4.49335565797689,0.794772684001174,5.25474111672184));
#51625=CARTESIAN_POINT('Ctrl Pts',(4.5451243536289,1.06847604194559,5.23713274866849));
#51626=CARTESIAN_POINT('Ctrl Pts',(4.56380264041945,1.18514270861233,5.24064786127112));
#51627=CARTESIAN_POINT('Ctrl Pts',(4.57875046387201,1.30000000000064,5.25530009655232));
#51628=CARTESIAN_POINT('Ctrl Pts',(4.66433918992144,-1.30000000000188,5.48115537773742));
#51629=CARTESIAN_POINT('Ctrl Pts',(4.64462219001566,-1.18514270861318,5.45302835129213));
#51630=CARTESIAN_POINT('Ctrl Pts',(4.61989798918264,-1.06847604194602,5.43352436265774));
#51631=CARTESIAN_POINT('Ctrl Pts',(4.55121250337003,-0.794772684001181,
5.40838718952874));
#51632=CARTESIAN_POINT('Ctrl Pts',(4.48545813985766,-0.636309800095462,
5.42491067930126));
#51633=CARTESIAN_POINT('Ctrl Pts',(4.41092879968034,-0.319434907277292,
5.42367627998968));
#51634=CARTESIAN_POINT('Ctrl Pts',(4.37052608002569,-0.158333333333399,
5.43378096763672));
#51635=CARTESIAN_POINT('Ctrl Pts',(4.35859759217659,0.1583333333334,5.4045925269395));
#51636=CARTESIAN_POINT('Ctrl Pts',(4.38674242879302,0.3194349072773,5.36450256247766));
#51637=CARTESIAN_POINT('Ctrl Pts',(4.43764525238439,0.636309800095472,5.30790530752386));
#51638=CARTESIAN_POINT('Ctrl Pts',(4.48970501358236,0.794772684001172,5.25966391154349));
#51639=CARTESIAN_POINT('Ctrl Pts',(4.54199635107428,1.06847604194559,5.24143965836856));
#51640=CARTESIAN_POINT('Ctrl Pts',(4.561007966488,1.18514270861233,5.24449923967641));
#51641=CARTESIAN_POINT('Ctrl Pts',(4.5763962149002,1.30000000000063,5.25850700621639));
#51642=CARTESIAN_POINT('Ctrl Pts',(4.66172094582562,-1.30000000000188,5.48398442088032));
#51643=CARTESIAN_POINT('Ctrl Pts',(4.64150899348046,-1.18514270861318,5.45641999848686));
#51644=CARTESIAN_POINT('Ctrl Pts',(4.61642395834516,-1.06847604194602,5.43732907294139));
#51645=CARTESIAN_POINT('Ctrl Pts',(4.54721471283658,-0.794772684001179,
5.41280068864089));
#51646=CARTESIAN_POINT('Ctrl Pts',(4.48155516606521,-0.63630980009546,5.4292202247029));
#51647=CARTESIAN_POINT('Ctrl Pts',(4.40702933723865,-0.319434907277291,
5.42803369794112));
#51648=CARTESIAN_POINT('Ctrl Pts',(4.36679451875707,-0.158333333333398,
5.43796559955891));
#51649=CARTESIAN_POINT('Ctrl Pts',(4.35491993278884,0.1583333333334,5.40885853892069));
#51650=CARTESIAN_POINT('Ctrl Pts',(4.38293867732819,0.319434907277299,5.36900727587747));
#51651=CARTESIAN_POINT('Ctrl Pts',(4.43397241595115,0.63630980009547,5.31255941411302));
#51652=CARTESIAN_POINT('Ctrl Pts',(4.48610689373479,0.794772684001169,5.26466634500749));
#51653=CARTESIAN_POINT('Ctrl Pts',(4.53893316513018,1.06847604194558,5.24584450419028));
#51654=CARTESIAN_POINT('Ctrl Pts',(4.55826670494919,1.18514270861233,5.24843138609822));
#51655=CARTESIAN_POINT('Ctrl Pts',(4.57406724910643,1.30000000000063,5.26175242738594));
#51656=CARTESIAN_POINT('Ctrl Pts',(4.65961765599959,-1.30000000000188,5.4862348200152));
#51657=CARTESIAN_POINT('Ctrl Pts',(4.63899451884016,-1.18514270861318,5.45909535878768));
#51658=CARTESIAN_POINT('Ctrl Pts',(4.61361138707586,-1.06847604194602,5.44031933916282));
#51659=CARTESIAN_POINT('Ctrl Pts',(4.54397473505142,-0.794772684001178,
5.41626420090247));
#51660=CARTESIAN_POINT('Ctrl Pts',(4.47840478660175,-0.63630980009546,5.43262355317404));
#51661=CARTESIAN_POINT('Ctrl Pts',(4.40389466358109,-0.319434907277291,
5.43149635883522));
#51662=CARTESIAN_POINT('Ctrl Pts',(4.36381059902997,-0.158333333333398,
5.44131593587122));
#51663=CARTESIAN_POINT('Ctrl Pts',(4.35197931163416,0.1583333333334,5.41227511086386));
#51664=CARTESIAN_POINT('Ctrl Pts',(4.37987298285693,0.319434907277299,5.37257818907799));
#51665=CARTESIAN_POINT('Ctrl Pts',(4.43101509826136,0.636309800095469,5.31625524436967));
#51666=CARTESIAN_POINT('Ctrl Pts',(4.48323929908517,0.794772684001169,5.26868557276865));
#51667=CARTESIAN_POINT('Ctrl Pts',(4.53649974833629,1.06847604194558,5.24939489077834));
#51668=CARTESIAN_POINT('Ctrl Pts',(4.55608872115211,1.18514270861233,5.25160041987816));
#51669=CARTESIAN_POINT('Ctrl Pts',(4.57221219179707,1.30000000000063,5.26436169952119));
#51670=CARTESIAN_POINT('Ctrl Pts',(4.65645802341575,-1.30000000000188,5.48960367750286));
#51671=CARTESIAN_POINT('Ctrl Pts',(4.63520906889767,-1.18514270861318,5.46308670277238));
#51672=CARTESIAN_POINT('Ctrl Pts',(4.6093729641242,-1.06847604194601,5.44477340173828));
#51673=CARTESIAN_POINT('Ctrl Pts',(4.53908915885635,-0.794772684001175,
5.42141814016419));
#51674=CARTESIAN_POINT('Ctrl Pts',(4.47366052691697,-0.636309800095458,
5.43769880485434));
#51675=CARTESIAN_POINT('Ctrl Pts',(4.39917939959728,-0.31943490727729,5.43666934906166));
#51676=CARTESIAN_POINT('Ctrl Pts',(4.3593286810474,-0.158333333333397,5.4463314264387));
#51677=CARTESIAN_POINT('Ctrl Pts',(4.3475623901759,0.158333333333399,5.41739068141055));
#51678=CARTESIAN_POINT('Ctrl Pts',(4.37525716574878,0.319434907277298,5.37790894068853));
#51679=CARTESIAN_POINT('Ctrl Pts',(4.42656489904725,0.636309800095467,5.32177847598885));
#51680=CARTESIAN_POINT('Ctrl Pts',(4.47894022941081,0.794772684001166,5.27471890995798));
#51681=CARTESIAN_POINT('Ctrl Pts',(4.53285528563043,1.06847604194558,5.25472980658627));
#51682=CARTESIAN_POINT('Ctrl Pts',(4.55282607501066,1.18514270861232,5.25636110693174));
#51683=CARTESIAN_POINT('Ctrl Pts',(4.56942982368338,1.30000000000062,5.26827624980302));
#51684=CARTESIAN_POINT('Ctrl Pts',(4.65172118736733,-1.30000000000187,5.49466426294768));
#51685=CARTESIAN_POINT('Ctrl Pts',(4.62953530745722,-1.18514270861317,5.46908539104944));
#51686=CARTESIAN_POINT('Ctrl Pts',(4.60301728186944,-1.06847604194601,5.45146296630844));
#51687=CARTESIAN_POINT('Ctrl Pts',(4.53174721469078,-0.794772684001171,
5.42913262441784));
#51688=CARTESIAN_POINT('Ctrl Pts',(4.46649976982099,-0.636309800095454,
5.44524266254511));
#51689=CARTESIAN_POINT('Ctrl Pts',(4.39204489191104,-0.319434907277288,
5.44433103317628));
#51690=CARTESIAN_POINT('Ctrl Pts',(4.35254308403161,-0.158333333333397,
5.45375490248664));
#51691=CARTESIAN_POINT('Ctrl Pts',(4.340883637343,0.158333333333398,5.4249812631589));
#51692=CARTESIAN_POINT('Ctrl Pts',(4.36831059437072,0.319434907277296,5.38587428192443));
#51693=CARTESIAN_POINT('Ctrl Pts',(4.41986216725414,0.636309800095464,5.33002860994802));
#51694=CARTESIAN_POINT('Ctrl Pts',(4.47240823278967,0.794772684001162,5.28364794370393));
#51695=CARTESIAN_POINT('Ctrl Pts',(4.52732036069452,1.06847604194557,5.26263427823024));
#51696=CARTESIAN_POINT('Ctrl Pts',(4.54788509653285,1.18514270861232,5.26343644066977));
#51697=CARTESIAN_POINT('Ctrl Pts',(4.56524514273436,1.30000000000062,5.27413680269932));
#51698=CARTESIAN_POINT('Ctrl Pts',(4.64343731377181,-1.30000000000185,5.50388797998165));
#51699=CARTESIAN_POINT('Ctrl Pts',(4.61978873133986,-1.18514270861316,5.48031998362622));
#51700=CARTESIAN_POINT('Ctrl Pts',(4.59217046718998,-1.068476041946,5.46411584541671));
#51701=CARTESIAN_POINT('Ctrl Pts',(4.51919599308853,-0.794772684001161,
5.4436930299779));
#51702=CARTESIAN_POINT('Ctrl Pts',(4.45400261297904,-0.636309800095446,
5.45904661482441));
#51703=CARTESIAN_POINT('Ctrl Pts',(4.37931066061378,-0.319434907277284,
5.45787638034737));
#51704=CARTESIAN_POINT('Ctrl Pts',(4.34010869977133,-0.158333333333395,
5.46635690222688));
#51705=CARTESIAN_POINT('Ctrl Pts',(4.32863248605252,0.158333333333396,5.43786714965165));
#51706=CARTESIAN_POINT('Ctrl Pts',(4.35603805714203,0.319434907277293,5.40015099671855));
#51707=CARTESIAN_POINT('Ctrl Pts',(4.40800596400493,0.636309800095456,5.34480895728543));
#51708=CARTESIAN_POINT('Ctrl Pts',(4.46036003808239,0.794772684001151,5.29889952382618));
#51709=CARTESIAN_POINT('Ctrl Pts',(4.51699995807158,1.06847604194556,5.27599065917723));
#51710=CARTESIAN_POINT('Ctrl Pts',(4.5386892684419,1.1851427086123,5.27541374926672));
#51711=CARTESIAN_POINT('Ctrl Pts',(4.55755056653508,1.3000000000006,5.28417632809513));
#51712=CARTESIAN_POINT('Ctrl Pts',(4.63309485448232,-1.3000000000018,5.51545665194679));
#51713=CARTESIAN_POINT('Ctrl Pts',(4.60760364164271,-1.18514270861311,5.49438368210212));
#51714=CARTESIAN_POINT('Ctrl Pts',(4.57860822372549,-1.06847604194595,5.47995294952138));
#51715=CARTESIAN_POINT('Ctrl Pts',(4.50352759308024,-0.794772684001128,
5.46195996725641));
#51716=CARTESIAN_POINT('Ctrl Pts',(4.43847086903231,-0.63630980009542,5.47648406203382));
#51717=CARTESIAN_POINT('Ctrl Pts',(4.36352655275373,-0.319434907277271,
5.47505714380749));
#51718=CARTESIAN_POINT('Ctrl Pts',(4.32474324350625,-0.158333333333388,
5.48241472934437));
#51719=CARTESIAN_POINT('Ctrl Pts',(4.31342386194375,0.15833333333339,5.45416031427122));
#51720=CARTESIAN_POINT('Ctrl Pts',(4.34057405669332,0.319434907277279,5.41782832862097));
#51721=CARTESIAN_POINT('Ctrl Pts',(4.39310065915147,0.636309800095429,5.36316959541494));
#51722=CARTESIAN_POINT('Ctrl Pts',(4.44553030973306,0.794772684001119,5.31832839198243));
#51723=CARTESIAN_POINT('Ctrl Pts',(4.50441545219899,1.06847604194552,5.29318734209524));
#51724=CARTESIAN_POINT('Ctrl Pts',(4.52750125039646,1.18514270861225,5.29087758351447));
#51725=CARTESIAN_POINT('Ctrl Pts',(4.54818365052745,1.30000000000055,5.29714069528139));
#51726=CARTESIAN_POINT('Ctrl Pts',(4.6161176146744,-1.30000000000174,5.53325242217053));
#51727=CARTESIAN_POINT('Ctrl Pts',(4.58732595215133,-1.18514270861306,5.51558939620259));
#51728=CARTESIAN_POINT('Ctrl Pts',(4.55588209662729,-1.06847604194591,5.50359082894549));
#51729=CARTESIAN_POINT('Ctrl Pts',(4.47711340364355,-0.794772684001098,
5.48895777106956));
#51730=CARTESIAN_POINT('Ctrl Pts',(4.41230604183178,-0.636309800095395,
5.50219354548612));
#51731=CARTESIAN_POINT('Ctrl Pts',(4.33727355937462,-0.319434907277259,
5.50089227085189));
#51732=CARTESIAN_POINT('Ctrl Pts',(4.29971762482629,-0.158333333333382,
5.50740221834196));
#51733=CARTESIAN_POINT('Ctrl Pts',(4.28903017588411,0.158333333333384,5.48017967903576));
#51734=CARTESIAN_POINT('Ctrl Pts',(4.3159463033878,0.319434907277267,5.44634259540802));
#51735=CARTESIAN_POINT('Ctrl Pts',(4.36911217875662,0.636309800095405,5.39240657377784));
#51736=CARTESIAN_POINT('Ctrl Pts',(4.42082888974231,0.794772684001087,5.34800452472138));
#51737=CARTESIAN_POINT('Ctrl Pts',(4.48315348314286,1.06847604194547,5.31902371701114));
#51738=CARTESIAN_POINT('Ctrl Pts',(4.5085608872895,1.18514270861221,5.31404943712708));
#51739=CARTESIAN_POINT('Ctrl Pts',(4.53239768845348,1.3000000000005,5.31664559517197));
#51740=CARTESIAN_POINT('Ctrl Pts',(4.59914282463979,-1.30000000000162,5.5510909883858));
#51741=CARTESIAN_POINT('Ctrl Pts',(4.56702672616545,-1.18514270861294,5.53679389600347));
#51742=CARTESIAN_POINT('Ctrl Pts',(4.53317405091121,-1.0684760419458,5.52729541184619));
#51743=CARTESIAN_POINT('Ctrl Pts',(4.450955759107,-0.79477268400102,5.51643775823578));
#51744=CARTESIAN_POINT('Ctrl Pts',(4.38699771120582,-0.636309800095331,
5.52943437329957));
#51745=CARTESIAN_POINT('Ctrl Pts',(4.31187329989311,-0.319434907277225,
5.52825583955045));
#51746=CARTESIAN_POINT('Ctrl Pts',(4.27518623909131,-0.158333333333365,
5.53326785410993));
#51747=CARTESIAN_POINT('Ctrl Pts',(4.26446568816465,0.158333333333367,5.50597675500226));
#51748=CARTESIAN_POINT('Ctrl Pts',(4.29019729726968,0.319434907277233,5.47312013259392));
#51749=CARTESIAN_POINT('Ctrl Pts',(4.34396319420537,0.636309800095338,5.41983611993691));
#51750=CARTESIAN_POINT('Ctrl Pts',(4.3960664930059,0.794772684001007,5.37762997047923));
#51751=CARTESIAN_POINT('Ctrl Pts',(4.46218061828739,1.06847604194536,5.34536762855042));
#51752=CARTESIAN_POINT('Ctrl Pts',(4.48992864601964,1.18514270861209,5.33775927694476));
#51753=CARTESIAN_POINT('Ctrl Pts',(4.51680634641956,1.30000000000036,5.33650774611683));
#51754=CARTESIAN_POINT('Ctrl Pts',(4.58425706155024,-1.30000000000161,5.56666693784608));
#51755=CARTESIAN_POINT('Ctrl Pts',(4.54934641908668,-1.18514270861293,5.55555096597518));
#51756=CARTESIAN_POINT('Ctrl Pts',(4.51334321280132,-1.0684760419458,5.54818858475124));
#51757=CARTESIAN_POINT('Ctrl Pts',(4.42764456287057,-0.794772684001015,
5.53985155658237));
#51758=CARTESIAN_POINT('Ctrl Pts',(4.36323699882183,-0.636309800095328,
5.55051525689881));
#51759=CARTESIAN_POINT('Ctrl Pts',(4.28775589540894,-0.319434907277225,
5.54896405460372));
#51760=CARTESIAN_POINT('Ctrl Pts',(4.25232434093199,-0.158333333333365,
5.55356099824275));
#51761=CARTESIAN_POINT('Ctrl Pts',(4.24222446884936,0.158333333333367,5.52734280767035));
#51762=CARTESIAN_POINT('Ctrl Pts',(4.26761085002562,0.319434907277234,5.49652744853665));
#51763=CARTESIAN_POINT('Ctrl Pts',(4.32240782374077,0.636309800095338,5.44467454255857));
#51764=CARTESIAN_POINT('Ctrl Pts',(4.37485911402526,0.794772684001005,5.40439130860367));
#51765=CARTESIAN_POINT('Ctrl Pts',(4.44419613943937,1.06847604194536,5.36908451924072));
#51766=CARTESIAN_POINT('Ctrl Pts',(4.47387959944389,1.18514270861208,5.358972935203));
#51767=CARTESIAN_POINT('Ctrl Pts',(4.50323309034115,1.30000000000036,5.35403276799731));
#51768=CARTESIAN_POINT('Ctrl Pts',(4.57558856625113,-1.3000000000016,5.57530232637884));
#51769=CARTESIAN_POINT('Ctrl Pts',(4.53881326219513,-1.18514270861292,5.56552049733167));
#51770=CARTESIAN_POINT('Ctrl Pts',(4.50148536593342,-1.06847604194579,5.55920339728274));
#51771=CARTESIAN_POINT('Ctrl Pts',(4.41397385960811,-0.794772684001007,
5.5526138495408));
#51772=CARTESIAN_POINT('Ctrl Pts',(4.35029675070984,-0.636309800095322,
5.56370748004289));
#51773=CARTESIAN_POINT('Ctrl Pts',(4.2748039665828,-0.319434907277222,5.56228315938248));
#51774=CARTESIAN_POINT('Ctrl Pts',(4.23967479680681,-0.158333333333364,
5.56588570353577));
#51775=CARTESIAN_POINT('Ctrl Pts',(4.22947881187277,0.158333333333365,5.53950259976342));
#51776=CARTESIAN_POINT('Ctrl Pts',(4.25430888765728,0.31943490727723,5.50924503607498));
#51777=CARTESIAN_POINT('Ctrl Pts',(4.30924321033487,0.636309800095331,5.45748274682784));
#51778=CARTESIAN_POINT('Ctrl Pts',(4.36152013083792,0.794772684000997,5.41775682917475));
#51779=CARTESIAN_POINT('Ctrl Pts',(4.43281265088734,1.06847604194535,5.38089753337119));
#51780=CARTESIAN_POINT('Ctrl Pts',(4.46379355744217,1.18514270861207,5.36965480595422));
#51781=CARTESIAN_POINT('Ctrl Pts',(4.49489548027066,1.30000000000035,5.36312437450212));
#51782=CARTESIAN_POINT('Ctrl Pts',(4.56261230358745,-1.30000000000158,5.58829235114902));
#51783=CARTESIAN_POINT('Ctrl Pts',(4.5231919902109,-1.18514270861291,5.58079144907158));
#51784=CARTESIAN_POINT('Ctrl Pts',(4.48391086259223,-1.06847604194578,5.57610915203169));
#51785=CARTESIAN_POINT('Ctrl Pts',(4.39348514657536,-0.794772684001001,
5.57180365067601));
#51786=CARTESIAN_POINT('Ctrl Pts',(4.33020120361279,-0.636309800095317,
5.58229128160804));
#51787=CARTESIAN_POINT('Ctrl Pts',(4.25444104633124,-0.319434907277219,
5.58061017277558));
#51788=CARTESIAN_POINT('Ctrl Pts',(4.21974659764685,-0.158333333333363,
5.58269369541246));
#51789=CARTESIAN_POINT('Ctrl Pts',(4.20999271078741,0.158333333333364,5.55707577920068));
#51790=CARTESIAN_POINT('Ctrl Pts',(4.23503288483197,0.319434907277228,5.52947251411293));
#51791=CARTESIAN_POINT('Ctrl Pts',(4.29072217396501,0.636309800095328,5.47877179929094));
#51792=CARTESIAN_POINT('Ctrl Pts',(4.34248883596468,0.794772684000991,5.43939020400205));
#51793=CARTESIAN_POINT('Ctrl Pts',(4.41662435868359,1.06847604194534,5.40004809333104));
#51794=CARTESIAN_POINT('Ctrl Pts',(4.4494865285756,1.18514270861206,5.38701200335624));
#51795=CARTESIAN_POINT('Ctrl Pts',(4.48312034756644,1.30000000000033,5.37796956534724));
#51796=CARTESIAN_POINT('Ctrl Pts',(4.54301380784669,-1.30000000000155,5.60754561873799));
#51797=CARTESIAN_POINT('Ctrl Pts',(4.49979258745065,-1.18514270861288,5.60379481597793));
#51798=CARTESIAN_POINT('Ctrl Pts',(4.45765702292381,-1.06847604194574,5.60171611997361));
#51799=CARTESIAN_POINT('Ctrl Pts',(4.36282352191878,-0.794772684000976,
5.60077681747148));
#51800=CARTESIAN_POINT('Ctrl Pts',(4.29958263496403,-0.636309800095297,
5.60931453785102));
#51801=CARTESIAN_POINT('Ctrl Pts',(4.2234914941984,-0.319434907277209,5.60736584564812));
#51802=CARTESIAN_POINT('Ctrl Pts',(4.19031554805787,-0.158333333333357,
5.6087274109245));
#51803=CARTESIAN_POINT('Ctrl Pts',(4.1808176578041,0.158333333333359,5.58359711196709));
#51804=CARTESIAN_POINT('Ctrl Pts',(4.20454998114033,0.319434907277217,5.55719162544147));
#51805=CARTESIAN_POINT('Ctrl Pts',(4.26118406444266,0.636309800095306,5.50777576293752));
#51806=CARTESIAN_POINT('Ctrl Pts',(4.3135833993088,0.794772684000966,5.47132072006254));
#51807=CARTESIAN_POINT('Ctrl Pts',(4.39229505523178,1.06847604194531,5.42878365567674));
#51808=CARTESIAN_POINT('Ctrl Pts',(4.42792972501858,1.18514270861202,5.41296560669806));
#51809=CARTESIAN_POINT('Ctrl Pts',(4.46512770529741,1.3000000000003,5.39974222775972));
#51810=CARTESIAN_POINT('Ctrl Pts',(4.516298972992,-1.3000000000015,5.63216227364944));
#51811=CARTESIAN_POINT('Ctrl Pts',(4.46765342605821,-1.18514270861284,5.6327703562665));
#51812=CARTESIAN_POINT('Ctrl Pts',(4.42152401198595,-1.06847604194572,5.63383083869071));
#51813=CARTESIAN_POINT('Ctrl Pts',(4.32076860758239,-0.794772684000958,
5.63732589929622));
#51814=CARTESIAN_POINT('Ctrl Pts',(4.25845143957159,-0.636309800095281,
5.64488057483907));
#51815=CARTESIAN_POINT('Ctrl Pts',(4.18182204396956,-0.3194349072772,5.64240443057221));
#51816=CARTESIAN_POINT('Ctrl Pts',(4.14971614301137,-0.158333333333353,
5.64102184400878));
#51817=CARTESIAN_POINT('Ctrl Pts',(4.14053077540987,0.158333333333355,5.61649581157307));
#51818=CARTESIAN_POINT('Ctrl Pts',(4.16351040483269,0.319434907277211,5.59349208043877));
#51819=CARTESIAN_POINT('Ctrl Pts',(4.22130949356724,0.636309800095291,5.54572587370549));
#51820=CARTESIAN_POINT('Ctrl Pts',(4.27328072613241,0.794772684000945,5.51108618839217));
#51821=CARTESIAN_POINT('Ctrl Pts',(4.35813807793187,1.06847604194528,5.46435842093235));
#51822=CARTESIAN_POINT('Ctrl Pts',(4.3977545667793,1.18514270861199,5.44528778384203));
#51823=CARTESIAN_POINT('Ctrl Pts',(4.44025594115493,1.30000000000026,5.4273732287603));
#51824=CARTESIAN_POINT('Ctrl Pts',(4.4943385548838,-1.30000000000144,5.65331652551978));
#51825=CARTESIAN_POINT('Ctrl Pts',(4.44111925554601,-1.18514270861278,5.65742385386435));
#51826=CARTESIAN_POINT('Ctrl Pts',(4.39153931856661,-1.06847604194566,5.66084062336221));
#51827=CARTESIAN_POINT('Ctrl Pts',(4.28540740081183,-0.794772684000913,
5.66713871534291));
#51828=CARTESIAN_POINT('Ctrl Pts',(4.22308865148336,-0.636309800095247,
5.67239269145178));
#51829=CARTESIAN_POINT('Ctrl Pts',(4.14584564055604,-0.319434907277184,
5.66911903350957));
#51830=CARTESIAN_POINT('Ctrl Pts',(4.11518564330417,-0.158333333333345,
5.66644082444016));
#51831=CARTESIAN_POINT('Ctrl Pts',(4.10641616714155,0.158333333333347,5.64275210326189));
#51832=CARTESIAN_POINT('Ctrl Pts',(4.12836718487157,0.319434907277194,5.62197732139297));
#51833=CARTESIAN_POINT('Ctrl Pts',(4.18762417697754,0.636309800095258,5.57651859441387));
#51834=CARTESIAN_POINT('Ctrl Pts',(4.24049473217301,0.794772684000904,5.54559351084376));
#51835=CARTESIAN_POINT('Ctrl Pts',(4.33065336907891,1.06847604194522,5.495734264183));
#51836=CARTESIAN_POINT('Ctrl Pts',(4.3734134672318,1.18514270861193,5.47366901455216));
#51837=CARTESIAN_POINT('Ctrl Pts',(4.41990733032775,1.30000000000019,5.45112073570273));
#51838=CARTESIAN_POINT('Ctrl Pts',(4.47582949985432,-1.30000000000144,5.66843433384013));
#51839=CARTESIAN_POINT('Ctrl Pts',(4.41879406299081,-1.18514270861278,5.67510274423551));
#51840=CARTESIAN_POINT('Ctrl Pts',(4.36638556973584,-1.06847604194566,5.68031676220333));
#51841=CARTESIAN_POINT('Ctrl Pts',(4.25600063138655,-0.79477268400091,5.68900224931184));
#51842=CARTESIAN_POINT('Ctrl Pts',(4.19404971549608,-0.636309800095244,
5.6930639368886));
#51843=CARTESIAN_POINT('Ctrl Pts',(4.11659846569157,-0.319434907277182,
5.68972467519604));
#51844=CARTESIAN_POINT('Ctrl Pts',(4.08725497155438,-0.158333333333344,
5.68638447927321));
#51845=CARTESIAN_POINT('Ctrl Pts',(4.07885160595465,0.158333333333346,5.66346590183524));
#51846=CARTESIAN_POINT('Ctrl Pts',(4.09999152136496,0.319434907277193,5.64444220511035));
#51847=CARTESIAN_POINT('Ctrl Pts',(4.15991876903039,0.636309800095255,5.59996812177501));
#51848=CARTESIAN_POINT('Ctrl Pts',(4.2124157915973,0.794772684000898,5.57017371395485));
#51849=CARTESIAN_POINT('Ctrl Pts',(4.30687468477072,1.06847604194522,5.51787148695648));
#51850=CARTESIAN_POINT('Ctrl Pts',(4.35244962590473,1.18514270861193,5.49389380217444));
#51851=CARTESIAN_POINT('Ctrl Pts',(4.40271175336492,1.30000000000019,5.46857812868941));
#51852=CARTESIAN_POINT('Ctrl Pts',(4.45542493556607,-1.30000000000142,5.68625771326939));
#51853=CARTESIAN_POINT('Ctrl Pts',(4.39420635524456,-1.18514270861277,5.69596986392667));
#51854=CARTESIAN_POINT('Ctrl Pts',(4.33864496717878,-1.06847604194565,5.70322160418365));
#51855=CARTESIAN_POINT('Ctrl Pts',(4.22335629155764,-0.794772684000902,
5.71429053465481));
#51856=CARTESIAN_POINT('Ctrl Pts',(4.16157081915296,-0.636309800095236,
5.7165455055085));
#51857=CARTESIAN_POINT('Ctrl Pts',(4.08329064411361,-0.319434907277177,
5.71188878932228));
#51858=CARTESIAN_POINT('Ctrl Pts',(4.05463582269465,-0.158333333333342,
5.70610769473987));
#51859=CARTESIAN_POINT('Ctrl Pts',(4.0465228193423,0.158333333333344,5.68383506722709));
#51860=CARTESIAN_POINT('Ctrl Pts',(4.0673207203027,0.319434907277186,5.66808682426998));
#51861=CARTESIAN_POINT('Ctrl Pts',(4.12855366925288,0.636309800095244,5.6258617737382));
#51862=CARTESIAN_POINT('Ctrl Pts',(4.1810976527764,0.794772684000889,5.5981460706891));
#51863=CARTESIAN_POINT('Ctrl Pts',(4.28062148488611,1.0684760419452,5.54358048255127));
#51864=CARTESIAN_POINT('Ctrl Pts',(4.32936623029481,1.18514270861191,5.51749860208889));
#51865=CARTESIAN_POINT('Ctrl Pts',(4.38377554191335,1.30000000000016,5.48895426241469));
#51866=CARTESIAN_POINT('Ctrl Pts',(4.43225268787918,-1.30000000000137,5.70516072474127));
#51867=CARTESIAN_POINT('Ctrl Pts',(4.36613347470572,-1.18514270861272,5.71785619133634));
#51868=CARTESIAN_POINT('Ctrl Pts',(4.30686656640134,-1.06847604194561,5.72703108182496));
#51869=CARTESIAN_POINT('Ctrl Pts',(4.18577834696053,-0.794772684000878,
5.74009367918948));
#51870=CARTESIAN_POINT('Ctrl Pts',(4.12380303207223,-0.636309800095214,
5.73940093161573));
#51871=CARTESIAN_POINT('Ctrl Pts',(4.04506367699879,-0.319434907277166,
5.73425187114617));
#51872=CARTESIAN_POINT('Ctrl Pts',(4.01851537171127,-0.158333333333337,
5.72864632025602));
#51873=CARTESIAN_POINT('Ctrl Pts',(4.01088922296883,0.158333333333339,5.70750320497276));
#51874=CARTESIAN_POINT('Ctrl Pts',(4.03021207820231,0.319434907277177,5.69314302340603));
#51875=CARTESIAN_POINT('Ctrl Pts',(4.09260132301132,0.636309800095224,5.65282683635549));
#51876=CARTESIAN_POINT('Ctrl Pts',(4.14568293805015,0.794772684000862,5.62844713099643));
#51877=CARTESIAN_POINT('Ctrl Pts',(4.2508220265062,1.06847604194517,5.57127723847806));
#51878=CARTESIAN_POINT('Ctrl Pts',(4.30301548770747,1.18514270861186,5.54265797204684));
#51879=CARTESIAN_POINT('Ctrl Pts',(4.36189159450457,1.30000000000012,5.51016616730232));
#51880=CARTESIAN_POINT('Ctrl Pts',(4.4090851760024,-1.30000000000137,5.72400020051124));
#51881=CARTESIAN_POINT('Ctrl Pts',(4.33802134759834,-1.18514270861272,5.73940830788491));
#51882=CARTESIAN_POINT('Ctrl Pts',(4.27500476704778,-1.0684760419456,5.75027058921371));
#51883=CARTESIAN_POINT('Ctrl Pts',(4.14801461194053,-0.79477268400087,5.7648628645221));
#51884=CARTESIAN_POINT('Ctrl Pts',(4.08597965493875,-0.636309800095212,
5.76144969401772));
#51885=CARTESIAN_POINT('Ctrl Pts',(4.00629549513168,-0.319434907277166,
5.75468117423453));
#51886=CARTESIAN_POINT('Ctrl Pts',(3.98094327595155,-0.158333333333336,
5.74728069400309));
#51887=CARTESIAN_POINT('Ctrl Pts',(3.97361735282597,0.158333333333338,5.72692681989707));
#51888=CARTESIAN_POINT('Ctrl Pts',(3.99214944324806,0.319434907277175,5.71549125834631));
#51889=CARTESIAN_POINT('Ctrl Pts',(4.05588095842403,0.636309800095221,5.67770868694704));
#51890=CARTESIAN_POINT('Ctrl Pts',(4.10903941712925,0.794772684000858,5.65594961861467));
#51891=CARTESIAN_POINT('Ctrl Pts',(4.22016590033604,1.06847604194517,5.5971307493497));
#51892=CARTESIAN_POINT('Ctrl Pts',(4.27612221881426,1.18514270861187,5.56667518822238));
#51893=CARTESIAN_POINT('Ctrl Pts',(4.3399323188325,1.30000000000012,5.53122457501863));
#51894=CARTESIAN_POINT('Ctrl Pts',(4.39231891341342,-1.30000000000136,5.73621537749296));
#51895=CARTESIAN_POINT('Ctrl Pts',(4.31765942975983,-1.18514270861271,5.75357177533912));
#51896=CARTESIAN_POINT('Ctrl Pts',(4.25188676500677,-1.0684760419456,5.76557492280135));
#51897=CARTESIAN_POINT('Ctrl Pts',(4.12046908111323,-0.794772684000867,
5.78093751535959));
#51898=CARTESIAN_POINT('Ctrl Pts',(4.05778038283076,-0.636309800095208,
5.77414225579004));
#51899=CARTESIAN_POINT('Ctrl Pts',(3.97800859932127,-0.319434907277164,
5.76756567149917));
#51900=CARTESIAN_POINT('Ctrl Pts',(3.95520035708981,-0.158333333333335,
5.76269698499336));
#51901=CARTESIAN_POINT('Ctrl Pts',(3.94833518429538,0.158333333333337,5.74349827159986));
#51902=CARTESIAN_POINT('Ctrl Pts',(3.96499427116526,0.319434907277172,5.73128534480092));
#51903=CARTESIAN_POINT('Ctrl Pts',(4.02932371604558,0.636309800095216,5.69444315181794));
#51904=CARTESIAN_POINT('Ctrl Pts',(4.08299019926578,0.794772684000854,5.67546484354474));
#51905=CARTESIAN_POINT('Ctrl Pts',(4.19852158235783,1.06847604194516,5.61556027904465));
#51906=CARTESIAN_POINT('Ctrl Pts',(4.25719705724207,1.18514270861186,5.58376271007258));
#51907=CARTESIAN_POINT('Ctrl Pts',(4.32453875212963,1.30000000000011,5.54609803841764));
#51908=CARTESIAN_POINT('Ctrl Pts',(4.38057663395295,-1.30000000000135,5.74519668890432));
#51909=CARTESIAN_POINT('Ctrl Pts',(4.30317639524159,-1.1851427086127,5.76305837794972));
#51910=CARTESIAN_POINT('Ctrl Pts',(4.23548147494313,-1.06847604194559,5.77559986068481));
#51911=CARTESIAN_POINT('Ctrl Pts',(4.10151389380763,-0.794772684000863,
5.79228245383744));
#51912=CARTESIAN_POINT('Ctrl Pts',(4.03998121252943,-0.636309800095205,
5.7867372046775));
#51913=CARTESIAN_POINT('Ctrl Pts',(3.96053722377183,-0.319434907277163,
5.78098056510057));
#51914=CARTESIAN_POINT('Ctrl Pts',(3.93875704946889,-0.158333333333334,
5.77609714660842));
#51915=CARTESIAN_POINT('Ctrl Pts',(3.93163988064319,0.158333333333336,5.75637324885947));
#51916=CARTESIAN_POINT('Ctrl Pts',(3.9466618734353,0.319434907277171,5.7428622438365));
#51917=CARTESIAN_POINT('Ctrl Pts',(4.01087747043568,0.636309800095214,5.70573468057763));
#51918=CARTESIAN_POINT('Ctrl Pts',(4.06465181025686,0.794772684000851,5.6883983338919));
#51919=CARTESIAN_POINT('Ctrl Pts',(4.18291930551696,1.06847604194515,5.62751390936758));
#51920=CARTESIAN_POINT('Ctrl Pts',(4.24337208879345,1.18514270861185,5.59478575178472));
#51921=CARTESIAN_POINT('Ctrl Pts',(4.31308403889095,1.3000000000001,5.55568404800531));
#51922=CARTESIAN_POINT('Ctrl Pts',(4.36598759938401,-1.30000000000135,5.75520187083884));
#51923=CARTESIAN_POINT('Ctrl Pts',(4.28495371436841,-1.1851427086127,5.77380994737787));
#51924=CARTESIAN_POINT('Ctrl Pts',(4.2147559770505,-1.06847604194558,5.78728839633516));
#51925=CARTESIAN_POINT('Ctrl Pts',(4.07761882978273,-0.794772684000858,
5.80657584388858));
#51926=CARTESIAN_POINT('Ctrl Pts',(4.01795330178055,-0.636309800095201,
5.80392668218628));
#51927=CARTESIAN_POINT('Ctrl Pts',(3.93921907864403,-0.319434907277161,
5.80021298084493));
#51928=CARTESIAN_POINT('Ctrl Pts',(3.91873439854227,-0.158333333333333,
5.7951550993706));
#51929=CARTESIAN_POINT('Ctrl Pts',(3.91163478140379,0.158333333333335,5.77552597077783));
#51930=CARTESIAN_POINT('Ctrl Pts',(3.92521934381218,0.319434907277169,5.76196968775307));
#51931=CARTESIAN_POINT('Ctrl Pts',(3.98908579202181,0.63630980009521,5.72363285871615));
#51932=CARTESIAN_POINT('Ctrl Pts',(4.04179431355421,0.794772684000846,5.70516207961435));
#51933=CARTESIAN_POINT('Ctrl Pts',(4.16337291576826,1.06847604194515,5.64185200560908));
#51934=CARTESIAN_POINT('Ctrl Pts',(4.22622970877727,1.18514270861185,5.60787943748067));
#51935=CARTESIAN_POINT('Ctrl Pts',(4.29931642282803,1.3000000000001,5.56733888639128));
#51936=CARTESIAN_POINT('Ctrl Pts',(4.35610142762914,-1.30000000000134,5.76212147047595));
#51937=CARTESIAN_POINT('Ctrl Pts',(4.27202510729744,-1.18514270861269,5.77999061529273));
#51938=CARTESIAN_POINT('Ctrl Pts',(4.19998727434625,-1.06847604194558,5.79359553631554));
#51939=CARTESIAN_POINT('Ctrl Pts',(4.06137678325034,-0.794772684000851,
5.81517441551416));
#51940=CARTESIAN_POINT('Ctrl Pts',(4.00531418533707,-0.636309800095197,
5.81806199192094));
#51941=CARTESIAN_POINT('Ctrl Pts',(3.92838285750872,-0.319434907277159,
5.81733237660638));
#51942=CARTESIAN_POINT('Ctrl Pts',(3.90875262161207,-0.158333333333332,
5.81160844072743));
#51943=CARTESIAN_POINT('Ctrl Pts',(3.90175138030431,0.158333333333334,5.79210658955772));
#51944=CARTESIAN_POINT('Ctrl Pts',(3.91457783688431,0.319434907277167,5.77918177957112));
#51945=CARTESIAN_POINT('Ctrl Pts',(3.97684592441674,0.636309800095206,5.73844981415392));
#51946=CARTESIAN_POINT('Ctrl Pts',(4.02617203613902,0.79477268400084,5.71559136609044));
#51947=CARTESIAN_POINT('Ctrl Pts',(4.14921392208308,1.06847604194514,5.64994165160661));
#51948=CARTESIAN_POINT('Ctrl Pts',(4.213841201547,1.18514270861184,5.61552978207355));
#51949=CARTESIAN_POINT('Ctrl Pts',(4.28983548720086,1.30000000000009,5.57512337184579));
#51950=CARTESIAN_POINT('Ctrl Pts',(4.35088387761145,-1.30000000000134,5.76896053285544));
#51951=CARTESIAN_POINT('Ctrl Pts',(4.26698198886915,-1.18514270861269,5.78664876365145));
#51952=CARTESIAN_POINT('Ctrl Pts',(4.19526082558516,-1.06847604194558,5.80039023590544));
#51953=CARTESIAN_POINT('Ctrl Pts',(4.05771050318435,-0.794772684000851,
5.82301798400579));
#51954=CARTESIAN_POINT('Ctrl Pts',(4.00307751336492,-0.636309800095197,
5.82803611993916));
#51955=CARTESIAN_POINT('Ctrl Pts',(3.9271390295546,-0.319434907277159,5.82866988923775));
#51956=CARTESIAN_POINT('Ctrl Pts',(3.90745678965039,-0.158333333333332,
5.8229519304616));
#51957=CARTESIAN_POINT('Ctrl Pts',(3.90061191119441,0.158333333333334,5.80362794938222));
#51958=CARTESIAN_POINT('Ctrl Pts',(3.91380906647831,0.319434907277167,5.79110325249133));
#51959=CARTESIAN_POINT('Ctrl Pts',(3.97507215158419,0.636309800095206,5.74890534309992));
#51960=CARTESIAN_POINT('Ctrl Pts',(4.02239198166674,0.79477268400084,5.72299871549042));
#51961=CARTESIAN_POINT('Ctrl Pts',(4.14444540563289,1.06847604194514,5.65643597419594));
#51962=CARTESIAN_POINT('Ctrl Pts',(4.20891602829543,1.18514270861184,5.62216459509058));
#51963=CARTESIAN_POINT('Ctrl Pts',(4.28502486891064,1.30000000000009,5.58243438119359));
#51964=CARTESIAN_POINT('Ctrl Pts',(4.35088387761047,-1.3,5.76896053285564));
#51965=CARTESIAN_POINT('Ctrl Pts',(4.26698198886859,-1.18514270861178,5.78664876365156));
#51966=CARTESIAN_POINT('Ctrl Pts',(4.19526082558493,-1.06847604194512,5.80039023590548));
#51967=CARTESIAN_POINT('Ctrl Pts',(4.05771050318435,-0.794772684000851,
5.8230179840058));
#51968=CARTESIAN_POINT('Ctrl Pts',(4.00307751336492,-0.636309800095197,
5.82803611993916));
#51969=CARTESIAN_POINT('Ctrl Pts',(3.9271390295546,-0.319434907277159,5.82866988923776));
#51970=CARTESIAN_POINT('Ctrl Pts',(3.90745678965039,-0.158333333333332,
5.8229519304616));
#51971=CARTESIAN_POINT('Ctrl Pts',(3.90061191119441,0.158333333333334,5.80362794938222));
#51972=CARTESIAN_POINT('Ctrl Pts',(3.91380906647831,0.319434907277167,5.79110325249133));
#51973=CARTESIAN_POINT('Ctrl Pts',(3.9750721515842,0.636309800095206,5.74890534309992));
#51974=CARTESIAN_POINT('Ctrl Pts',(4.02239198166674,0.79477268400084,5.72299871549042));
#51975=CARTESIAN_POINT('Ctrl Pts',(4.14444540563287,1.06847604194511,5.65643597419595));
#51976=CARTESIAN_POINT('Ctrl Pts',(4.20891602829539,1.18514270861178,5.6221645950906));
#51977=CARTESIAN_POINT('Ctrl Pts',(4.28502486891058,1.3,5.58243438119362));
#51978=CARTESIAN_POINT('',(4.63722129958651,-1.2,5.46833068437959));
#51979=CARTESIAN_POINT('Ctrl Pts',(4.6372212995865,-1.2,5.4683306843796));
#51980=CARTESIAN_POINT('Ctrl Pts',(4.62750586065925,-1.21481068879262,5.48465035288688));
#51981=CARTESIAN_POINT('Ctrl Pts',(4.62725170851186,-1.21549275722123,5.48594687910636));
#51982=CARTESIAN_POINT('Ctrl Pts',(4.6149839274451,-1.23450984640621,5.50765759125053));
#51983=CARTESIAN_POINT('Ctrl Pts',(4.61396625404581,-1.23601256685819,5.50922612580931));
#51984=CARTESIAN_POINT('Ctrl Pts',(4.5936259721994,-1.26668179624999,5.54302123985939));
#51985=CARTESIAN_POINT('Ctrl Pts',(4.58460229424093,-1.28035635399065,5.55832572060974));
#51986=CARTESIAN_POINT('Ctrl Pts',(4.57129987359789,-1.30000000000159,5.57959342582533));
#51987=CARTESIAN_POINT('',(4.58017336234084,-0.65383484141843,5.32263163693194));
#51988=CARTESIAN_POINT('Ctrl Pts',(4.58017336236564,-0.653834841417755,
5.32263163692465));
#51989=CARTESIAN_POINT('Ctrl Pts',(4.58634999591384,-0.718019341709874,
5.33770063084345));
#51990=CARTESIAN_POINT('Ctrl Pts',(4.59130924624133,-0.763830568183498,
5.34995750755485));
#51991=CARTESIAN_POINT('Ctrl Pts',(4.6105027479006,-0.949554209366674,5.39805721041602));
#51992=CARTESIAN_POINT('Ctrl Pts',(4.62071098387629,-1.04816473166287,5.424117862114));
#51993=CARTESIAN_POINT('Ctrl Pts',(4.6372212995865,-1.2,5.46833068437959));
#51994=CARTESIAN_POINT('',(4.52544944337419,0.653834841531101,5.19430627077206));
#51995=CARTESIAN_POINT('Ctrl Pts',(4.52544944337418,0.6538348415311,5.19430627077206));
#51996=CARTESIAN_POINT('Ctrl Pts',(4.49800585333586,0.575794444672551,5.22566650872935));
#51997=CARTESIAN_POINT('Ctrl Pts',(4.47552348374572,0.493916456452013,5.2524053607931));
#51998=CARTESIAN_POINT('Ctrl Pts',(4.44488537421593,0.338192744373412,5.29279369503618));
#51999=CARTESIAN_POINT('Ctrl Pts',(4.43508928797886,0.265707177517069,5.30779049654904));
#52000=CARTESIAN_POINT('Ctrl Pts',(4.42552848990739,0.12973909330966,5.33024832219718));
#52001=CARTESIAN_POINT('Ctrl Pts',(4.42449620873789,0.0666398892825386,
5.33846719753409));
#52002=CARTESIAN_POINT('Ctrl Pts',(4.42938530227431,-0.0595502670510932,
5.35088018140976));
#52003=CARTESIAN_POINT('Ctrl Pts',(4.43532785702372,-0.122795603932536,
5.35517433332143));
#52004=CARTESIAN_POINT('Ctrl Pts',(4.4556310002044,-0.260150559875305,5.35942166735652));
#52005=CARTESIAN_POINT('Ctrl Pts',(4.4713300777237,-0.333952819465554,5.35844333383778));
#52006=CARTESIAN_POINT('Ctrl Pts',(4.51499497518982,-0.491148042392089,
5.34829752130936));
#52007=CARTESIAN_POINT('Ctrl Pts',(4.5447686026171,-0.574257524294844,5.33787546399782));
#52008=CARTESIAN_POINT('Ctrl Pts',(4.58017336233156,-0.653834841429973,
5.32263163697063));
#52009=CARTESIAN_POINT('',(4.55420717418533,1.2,5.26049052216833));
#52010=CARTESIAN_POINT('Ctrl Pts',(4.55420717418533,1.2,5.26049052216833));
#52011=CARTESIAN_POINT('Ctrl Pts',(4.54938384035087,1.13496897291812,5.24916474015826));
#52012=CARTESIAN_POINT('Ctrl Pts',(4.54290377805626,1.03871956312488,5.23407139532195));
#52013=CARTESIAN_POINT('Ctrl Pts',(4.5301510071915,0.795283719863686,5.20490499247069));
#52014=CARTESIAN_POINT('Ctrl Pts',(4.52810469686917,0.741463044907116,5.20029732278355));
#52015=CARTESIAN_POINT('Ctrl Pts',(4.52544944337418,0.653834841531101,5.19430627077206));
#52016=CARTESIAN_POINT('Ctrl Pts',(4.49080284932948,1.30000000000007,5.36828229018401));
#52017=CARTESIAN_POINT('Ctrl Pts',(4.49816830366447,1.2884795594474,5.35583641315607));
#52018=CARTESIAN_POINT('Ctrl Pts',(4.50506668818057,1.27813273296559,5.34541970920166));
#52019=CARTESIAN_POINT('Ctrl Pts',(4.51196371767097,1.26718805828393,5.33343091922482));
#52020=CARTESIAN_POINT('Ctrl Pts',(4.51743270817141,1.25854452828621,5.32405235793424));
#52021=CARTESIAN_POINT('Ctrl Pts',(4.52987929250229,1.23907155243216,5.30329891655241));
#52022=CARTESIAN_POINT('Ctrl Pts',(4.54268753971979,1.21913747525351,5.28228350697248));
#52023=CARTESIAN_POINT('Ctrl Pts',(4.55420717418533,1.2,5.26049052216833));
#52024=CARTESIAN_POINT('Ctrl Pts',(4.35088387761047,-1.3,5.76896053285564));
#52025=CARTESIAN_POINT('Ctrl Pts',(4.26698198886859,-1.18514270861178,5.78664876365156));
#52026=CARTESIAN_POINT('Ctrl Pts',(4.19526082558493,-1.06847604194512,5.80039023590548));
#52027=CARTESIAN_POINT('Ctrl Pts',(4.05771050318435,-0.794772684000851,
5.8230179840058));
#52028=CARTESIAN_POINT('Ctrl Pts',(4.00307751336492,-0.636309800095196,
5.82803611993916));
#52029=CARTESIAN_POINT('Ctrl Pts',(3.9271390295546,-0.319434907277159,5.82866988923776));
#52030=CARTESIAN_POINT('Ctrl Pts',(3.90745678965039,-0.158333333333332,
5.8229519304616));
#52031=CARTESIAN_POINT('Ctrl Pts',(3.90061191119441,0.158333333333335,5.80362794938222));
#52032=CARTESIAN_POINT('Ctrl Pts',(3.91380906647831,0.319434907277167,5.79110325249134));
#52033=CARTESIAN_POINT('Ctrl Pts',(3.9750721515842,0.636309800095206,5.74890534309992));
#52034=CARTESIAN_POINT('Ctrl Pts',(4.02239198166674,0.794772684000841,5.72299871549042));
#52035=CARTESIAN_POINT('Ctrl Pts',(4.14444540563287,1.06847604194511,5.65643597419595));
#52036=CARTESIAN_POINT('Ctrl Pts',(4.20891602829539,1.18514270861178,5.6221645950906));
#52037=CARTESIAN_POINT('Ctrl Pts',(4.28502486891058,1.3,5.58243438119362));
#52038=CARTESIAN_POINT('Ctrl Pts',(4.37306897027954,-1.3,5.84262823906338));
#52039=CARTESIAN_POINT('Ctrl Pts',(4.28882565135864,-1.18514270861178,5.85861813821062));
#52040=CARTESIAN_POINT('Ctrl Pts',(4.21691086230761,-1.06847604194512,5.87116870407665));
#52041=CARTESIAN_POINT('Ctrl Pts',(4.0792546834088,-0.794772684000851,5.89221747404342));
#52042=CARTESIAN_POINT('Ctrl Pts',(4.02499599674477,-0.636309800095196,
5.89784789675249));
#52043=CARTESIAN_POINT('Ctrl Pts',(3.94958161227244,-0.319434907277159,
5.8988939803217));
#52044=CARTESIAN_POINT('Ctrl Pts',(3.93044726732831,-0.158333333333332,
5.89429014134225));
#52045=CARTESIAN_POINT('Ctrl Pts',(3.92394377232475,0.158333333333335,5.87485523805521));
#52046=CARTESIAN_POINT('Ctrl Pts',(3.9369293207567,0.319434907277167,5.86110715473768));
#52047=CARTESIAN_POINT('Ctrl Pts',(3.99837405888618,0.636309800095206,5.81826761823271));
#52048=CARTESIAN_POINT('Ctrl Pts',(4.04563681344556,0.794772684000841,5.7916456303416));
#52049=CARTESIAN_POINT('Ctrl Pts',(4.16853269776624,1.06847604194511,5.72642253007944));
#52050=CARTESIAN_POINT('Ctrl Pts',(4.23354667110408,1.18514270861178,5.69322842485112));
#52051=CARTESIAN_POINT('Ctrl Pts',(4.31037754319865,1.3,5.65507287774392));
#52052=CARTESIAN_POINT('Ctrl Pts',(4.39525406294861,-1.3,5.91629594527112));
#52053=CARTESIAN_POINT('Ctrl Pts',(4.3106693138487,-1.18514270861178,5.93058751276968));
#52054=CARTESIAN_POINT('Ctrl Pts',(4.2385608990303,-1.06847604194512,5.94194717224782));
#52055=CARTESIAN_POINT('Ctrl Pts',(4.10079886363325,-0.794772684000851,
5.96141696408105));
#52056=CARTESIAN_POINT('Ctrl Pts',(4.04691448012462,-0.636309800095196,
5.96765967356582));
#52057=CARTESIAN_POINT('Ctrl Pts',(3.97202419499028,-0.319434907277159,
5.96911807140564));
#52058=CARTESIAN_POINT('Ctrl Pts',(3.95343774500623,-0.158333333333332,
5.9656283522229));
#52059=CARTESIAN_POINT('Ctrl Pts',(3.94727563345509,0.158333333333335,5.9460825267282));
#52060=CARTESIAN_POINT('Ctrl Pts',(3.96004957503508,0.319434907277167,5.93111105698402));
#52061=CARTESIAN_POINT('Ctrl Pts',(4.02167596618816,0.636309800095206,5.8876298933655));
#52062=CARTESIAN_POINT('Ctrl Pts',(4.06888164522438,0.794772684000841,5.86029254519278));
#52063=CARTESIAN_POINT('Ctrl Pts',(4.19261998989962,1.06847604194511,5.79640908596293));
#52064=CARTESIAN_POINT('Ctrl Pts',(4.25817731391276,1.18514270861178,5.76429225461164));
#52065=CARTESIAN_POINT('Ctrl Pts',(4.33573021748671,1.3,5.72771137429423));
#52066=CARTESIAN_POINT('Ctrl Pts',(4.41743915561768,-1.3,5.98996365147886));
#52067=CARTESIAN_POINT('Ctrl Pts',(4.33251297633875,-1.18514270861178,6.00255688732874));
#52068=CARTESIAN_POINT('Ctrl Pts',(4.26021093575299,-1.06847604194512,6.01272564041899));
#52069=CARTESIAN_POINT('Ctrl Pts',(4.12234304385769,-0.794772684000851,
6.03061645411867));
#52070=CARTESIAN_POINT('Ctrl Pts',(4.06883296350447,-0.636309800095196,
6.03747145037915));
#52071=CARTESIAN_POINT('Ctrl Pts',(3.99446677770813,-0.319434907277159,
6.03934216248958));
#52072=CARTESIAN_POINT('Ctrl Pts',(3.97642822268415,-0.158333333333332,
6.03696656310355));
#52073=CARTESIAN_POINT('Ctrl Pts',(3.97060749458543,0.158333333333335,6.01730981540119));
#52074=CARTESIAN_POINT('Ctrl Pts',(3.98316982931346,0.319434907277167,6.00111495923037));
#52075=CARTESIAN_POINT('Ctrl Pts',(4.04497787349015,0.636309800095206,5.95699216849829));
#52076=CARTESIAN_POINT('Ctrl Pts',(4.0921264770032,0.794772684000841,5.92893946004396));
#52077=CARTESIAN_POINT('Ctrl Pts',(4.21670728203299,1.06847604194511,5.86639564184641));
#52078=CARTESIAN_POINT('Ctrl Pts',(4.28280795672145,1.18514270861178,5.83535608437217));
#52079=CARTESIAN_POINT('Ctrl Pts',(4.36108289177478,1.3,5.80034987084453));
#52080=CARTESIAN_POINT('Ctrl Pts',(4.41743915561768,-1.3,5.98996365147886));
#52081=CARTESIAN_POINT('Ctrl Pts',(4.33251297633875,-1.18514270861178,6.00255688732874));
#52082=CARTESIAN_POINT('Ctrl Pts',(4.26021093575299,-1.06847604194512,6.01272564041899));
#52083=CARTESIAN_POINT('Ctrl Pts',(4.12234304385769,-0.794772684000851,
6.03061645411867));
#52084=CARTESIAN_POINT('Ctrl Pts',(4.06883296350448,-0.636309800095197,
6.03747145037915));
#52085=CARTESIAN_POINT('Ctrl Pts',(3.99446677770812,-0.319434907277159,
6.03934216248958));
#52086=CARTESIAN_POINT('Ctrl Pts',(3.97642822268415,-0.158333333333332,
6.03696656310355));
#52087=CARTESIAN_POINT('Ctrl Pts',(3.97060749458543,0.158333333333334,6.01730981540119));
#52088=CARTESIAN_POINT('Ctrl Pts',(3.98316982931346,0.319434907277167,6.00111495923037));
#52089=CARTESIAN_POINT('Ctrl Pts',(4.04497787349014,0.636309800095206,5.95699216849829));
#52090=CARTESIAN_POINT('Ctrl Pts',(4.0921264770032,0.79477268400084,5.92893946004396));
#52091=CARTESIAN_POINT('Ctrl Pts',(4.21670728203298,1.06847604194511,5.86639564184641));
#52092=CARTESIAN_POINT('Ctrl Pts',(4.28280795672145,1.18514270861178,5.83535608437217));
#52093=CARTESIAN_POINT('Ctrl Pts',(4.36108289177478,1.3,5.80034987084453));
#52094=CARTESIAN_POINT('Ctrl Pts',(4.41743915561997,-1.30000000000309,5.98996365147853));
#52095=CARTESIAN_POINT('Ctrl Pts',(4.33251297634005,-1.18514270861388,6.00255688732856));
#52096=CARTESIAN_POINT('Ctrl Pts',(4.26021093575352,-1.06847604194618,6.01272564041892));
#52097=CARTESIAN_POINT('Ctrl Pts',(4.12234304385769,-0.794772684000851,
6.03061645411867));
#52098=CARTESIAN_POINT('Ctrl Pts',(4.06883296350447,-0.636309800095196,
6.03747145037915));
#52099=CARTESIAN_POINT('Ctrl Pts',(3.99446677770812,-0.319434907277159,
6.03934216248958));
#52100=CARTESIAN_POINT('Ctrl Pts',(3.97642822268415,-0.158333333333332,
6.03696656310355));
#52101=CARTESIAN_POINT('Ctrl Pts',(3.97060749458543,0.158333333333334,6.01730981540119));
#52102=CARTESIAN_POINT('Ctrl Pts',(3.98316982931346,0.319434907277167,6.00111495923037));
#52103=CARTESIAN_POINT('Ctrl Pts',(4.04497787349015,0.636309800095206,5.95699216849829));
#52104=CARTESIAN_POINT('Ctrl Pts',(4.0921264770032,0.794772684000841,5.92893946004397));
#52105=CARTESIAN_POINT('Ctrl Pts',(4.21670728203357,1.0684760419464,5.86639564184612));
#52106=CARTESIAN_POINT('Ctrl Pts',(4.28280795672289,1.18514270861431,5.8353560843715));
#52107=CARTESIAN_POINT('Ctrl Pts',(4.36108289177733,1.30000000000375,5.80034987084339));
#52108=CARTESIAN_POINT('Ctrl Pts',(4.42562833098721,-1.30000000000309,5.99305077181872));
#52109=CARTESIAN_POINT('Ctrl Pts',(4.34039737039433,-1.18514270861388,6.00502961962694));
#52110=CARTESIAN_POINT('Ctrl Pts',(4.26788601359697,-1.06847604194618,6.01517679412997));
#52111=CARTESIAN_POINT('Ctrl Pts',(4.12975510286419,-0.794772684000851,
6.03438726540721));
#52112=CARTESIAN_POINT('Ctrl Pts',(4.07641358156132,-0.636309800095196,
6.04488755347926));
#52113=CARTESIAN_POINT('Ctrl Pts',(4.00209599194821,-0.319434907277159,
6.04853496478958));
#52114=CARTESIAN_POINT('Ctrl Pts',(3.98412215784035,-0.158333333333332,
6.04561777589617));
#52115=CARTESIAN_POINT('Ctrl Pts',(3.97832338053354,0.158333333333334,6.0257252204883));
#52116=CARTESIAN_POINT('Ctrl Pts',(3.99084012994539,0.319434907277167,6.0095560959087));
#52117=CARTESIAN_POINT('Ctrl Pts',(4.05265002446484,0.636309800095206,5.96374672477414));
#52118=CARTESIAN_POINT('Ctrl Pts',(4.09970289374315,0.794772684000841,5.93313005490399));
#52119=CARTESIAN_POINT('Ctrl Pts',(4.2245248835901,1.0684760419464,5.86911453241694));
#52120=CARTESIAN_POINT('Ctrl Pts',(4.29080148661917,1.18514270861431,5.8377783689165));
#52121=CARTESIAN_POINT('Ctrl Pts',(4.36932387838279,1.30000000000375,5.80281598959156));
#52122=CARTESIAN_POINT('Ctrl Pts',(4.43787121888944,-1.30000000000308,5.99376524194423));
#52123=CARTESIAN_POINT('Ctrl Pts',(4.35491096318019,-1.18514270861386,6.00391672292321));
#52124=CARTESIAN_POINT('Ctrl Pts',(4.2840885617701,-1.06847604194617,6.01337406538631));
#52125=CARTESIAN_POINT('Ctrl Pts',(4.14851551814112,-0.794772684000842,
6.03361881957726));
#52126=CARTESIAN_POINT('Ctrl Pts',(4.09501955407359,-0.636309800095189,
6.04967670444219));
#52127=CARTESIAN_POINT('Ctrl Pts',(4.02081949266675,-0.319434907277155,
6.0562190775837));
#52128=CARTESIAN_POINT('Ctrl Pts',(4.00186551766012,-0.15833333333333,6.05325499433251));
#52129=CARTESIAN_POINT('Ctrl Pts',(3.99606931639037,0.158333333333333,6.03319499170625));
#52130=CARTESIAN_POINT('Ctrl Pts',(4.00965920221954,0.319434907277164,6.01702438361));
#52131=CARTESIAN_POINT('Ctrl Pts',(4.07117263776139,0.636309800095199,5.9677364370366));
#52132=CARTESIAN_POINT('Ctrl Pts',(4.11789328435415,0.794772684000831,5.93055388199639));
#52133=CARTESIAN_POINT('Ctrl Pts',(4.24018002663975,1.06847604194638,5.86555700416122));
#52134=CARTESIAN_POINT('Ctrl Pts',(4.30489463524463,1.1851427086143,5.83519871970262));
#52135=CARTESIAN_POINT('Ctrl Pts',(4.38139045288901,1.30000000000373,5.80261689082876));
#52136=CARTESIAN_POINT('Ctrl Pts',(4.45585041430731,-1.30000000000307,5.99501197237341));
#52137=CARTESIAN_POINT('Ctrl Pts',(4.37647147135345,-1.18514270861386,6.00435238130437));
#52138=CARTESIAN_POINT('Ctrl Pts',(4.30833031726903,-1.06847604194617,6.01341501487799));
#52139=CARTESIAN_POINT('Ctrl Pts',(4.17687216014389,-0.794772684000842,
6.03370979476238));
#52140=CARTESIAN_POINT('Ctrl Pts',(4.12318598035631,-0.636309800095189,
6.051344155984));
#52141=CARTESIAN_POINT('Ctrl Pts',(4.04942280399533,-0.319434907277155,
6.05911325681098));
#52142=CARTESIAN_POINT('Ctrl Pts',(4.02934019274684,-0.15833333333333,6.05707345537754));
#52143=CARTESIAN_POINT('Ctrl Pts',(4.02349949763675,0.158333333333333,6.03691189730058));
#52144=CARTESIAN_POINT('Ctrl Pts',(4.0382239070047,0.319434907277164,6.02003355142058));
#52145=CARTESIAN_POINT('Ctrl Pts',(4.09910720400251,0.636309800095199,5.96866407027448));
#52146=CARTESIAN_POINT('Ctrl Pts',(4.14564853964763,0.794772684000832,5.92810673121632));
#52147=CARTESIAN_POINT('Ctrl Pts',(4.26383848145775,1.06847604194638,5.86288689468531));
#52148=CARTESIAN_POINT('Ctrl Pts',(4.32597451263342,1.1851427086143,5.83324406605495));
#52149=CARTESIAN_POINT('Ctrl Pts',(4.3990865285438,1.30000000000373,5.80218965939557));
#52150=CARTESIAN_POINT('Ctrl Pts',(4.47077112054955,-1.30000000000307,5.99624136741226));
#52151=CARTESIAN_POINT('Ctrl Pts',(4.3941367061776,-1.18514270861385,6.0053141056848));
#52152=CARTESIAN_POINT('Ctrl Pts',(4.3279655414052,-1.06847604194616,6.0140486726285));
#52153=CARTESIAN_POINT('Ctrl Pts',(4.19926911302636,-0.794772684000836,
6.03344602619192));
#52154=CARTESIAN_POINT('Ctrl Pts',(4.14469678620781,-0.636309800095183,
6.04964010753271));
#52155=CARTESIAN_POINT('Ctrl Pts',(4.07099239599207,-0.319434907277152,
6.05762788567868));
#52156=CARTESIAN_POINT('Ctrl Pts',(4.05033624387987,-0.158333333333329,
6.05752341512769));
#52157=CARTESIAN_POINT('Ctrl Pts',(4.04460429816785,0.158333333333331,6.0379605124523));
#52158=CARTESIAN_POINT('Ctrl Pts',(4.06019377913399,0.319434907277161,6.0206465745952));
#52159=CARTESIAN_POINT('Ctrl Pts',(4.12086749225863,0.636309800095193,5.96844239186139));
#52160=CARTESIAN_POINT('Ctrl Pts',(4.16759019757613,0.794772684000824,5.92608052888347));
#52161=CARTESIAN_POINT('Ctrl Pts',(4.28295080002241,1.06847604194637,5.86124858282267));
#52162=CARTESIAN_POINT('Ctrl Pts',(4.34322444403162,1.18514270861429,5.83229200346367));
#52163=CARTESIAN_POINT('Ctrl Pts',(4.41383640178237,1.30000000000372,5.80244219193521));
#52164=CARTESIAN_POINT('Ctrl Pts',(4.48888549481477,-1.30000000000306,5.99826902796289));
#52165=CARTESIAN_POINT('Ctrl Pts',(4.41585250305352,-1.18514270861385,6.00716604759878));
#52166=CARTESIAN_POINT('Ctrl Pts',(4.35227563785691,-1.06847604194615,6.01553951366496));
#52167=CARTESIAN_POINT('Ctrl Pts',(4.22724590480102,-0.794772684000832,
6.03367438190129));
#52168=CARTESIAN_POINT('Ctrl Pts',(4.17165190374168,-0.636309800095182,
6.04784773027761));
#52169=CARTESIAN_POINT('Ctrl Pts',(4.09793603477848,-0.319434907277151,
6.0551166088243));
#52170=CARTESIAN_POINT('Ctrl Pts',(4.07641255024289,-0.158333333333329,
6.05672669443841));
#52171=CARTESIAN_POINT('Ctrl Pts',(4.07040330877367,0.158333333333331,6.03605204947613));
#52172=CARTESIAN_POINT('Ctrl Pts',(4.08639823387368,0.31943490727716,6.01522745208349));
#52173=CARTESIAN_POINT('Ctrl Pts',(4.14689459595155,0.636309800095192,5.9628716242103));
#52174=CARTESIAN_POINT('Ctrl Pts',(4.19493228340675,0.794772684000823,5.9235372548977));
#52175=CARTESIAN_POINT('Ctrl Pts',(4.3068199206522,1.06847604194637,5.86052220641105));
#52176=CARTESIAN_POINT('Ctrl Pts',(4.36458750470472,1.18514270861428,5.83217938427488));
#52177=CARTESIAN_POINT('Ctrl Pts',(4.43169066049147,1.30000000000371,5.8027706195549));
#52178=CARTESIAN_POINT('Ctrl Pts',(4.5070805240044,-1.30000000000304,6.00172835399182));
#52179=CARTESIAN_POINT('Ctrl Pts',(4.43743267384654,-1.18514270861383,6.01016185167031));
#52180=CARTESIAN_POINT('Ctrl Pts',(4.37628118333525,-1.06847604194614,6.01793101980723));
#52181=CARTESIAN_POINT('Ctrl Pts',(4.25463729741546,-0.79477268400082,6.03434461828046));
#52182=CARTESIAN_POINT('Ctrl Pts',(4.19808657167185,-0.636309800095172,
6.04682497611925));
#52183=CARTESIAN_POINT('Ctrl Pts',(4.12408493576571,-0.319434907277146,
6.05216015227242));
#52184=CARTESIAN_POINT('Ctrl Pts',(4.10118108824753,-0.158333333333326,
6.05275179787127));
#52185=CARTESIAN_POINT('Ctrl Pts',(4.0950379936865,0.158333333333328,6.03161959587353));
#52186=CARTESIAN_POINT('Ctrl Pts',(4.11224098282643,0.319434907277155,6.01137027620302));
#52187=CARTESIAN_POINT('Ctrl Pts',(4.172828774167,0.636309800095181,5.95998681893364));
#52188=CARTESIAN_POINT('Ctrl Pts',(4.22174645187094,0.79477268400081,5.9216197443018));
#52189=CARTESIAN_POINT('Ctrl Pts',(4.33025333204167,1.06847604194635,5.85979788035525));
#52190=CARTESIAN_POINT('Ctrl Pts',(4.38563297633725,1.18514270861426,5.83195039824915));
#52191=CARTESIAN_POINT('Ctrl Pts',(4.44942365707838,1.30000000000369,5.80301582821375));
#52192=CARTESIAN_POINT('Ctrl Pts',(4.53109886254452,-1.30000000000303,6.00406302153179));
#52193=CARTESIAN_POINT('Ctrl Pts',(4.46616480243323,-1.18514270861382,6.01256767400805));
#52194=CARTESIAN_POINT('Ctrl Pts',(4.40841786727856,-1.06847604194613,6.02013682822857));
#52195=CARTESIAN_POINT('Ctrl Pts',(4.29161459126626,-0.794772684000815,
6.03546190056545));
#52196=CARTESIAN_POINT('Ctrl Pts',(4.23390801699434,-0.636309800095169,
6.0461976720324));
#52197=CARTESIAN_POINT('Ctrl Pts',(4.15971786921738,-0.319434907277146,
6.04979125214187));
#52198=CARTESIAN_POINT('Ctrl Pts',(4.13507614674857,-0.158333333333325,
6.04965079389733));
#52199=CARTESIAN_POINT('Ctrl Pts',(4.1287251135606,0.158333333333328,6.02765789882209));
#52200=CARTESIAN_POINT('Ctrl Pts',(4.14731388921087,0.319434907277154,6.00671206620468));
#52201=CARTESIAN_POINT('Ctrl Pts',(4.20796025920192,0.63630980009518,5.95647385486317));
#52202=CARTESIAN_POINT('Ctrl Pts',(4.25823946126208,0.794772684000807,5.92061942086322));
#52203=CARTESIAN_POINT('Ctrl Pts',(4.36212968709833,1.06847604194635,5.86069137778686));
#52204=CARTESIAN_POINT('Ctrl Pts',(4.41422395080956,1.18514270861426,5.83347966904655));
#52205=CARTESIAN_POINT('Ctrl Pts',(4.47344224897951,1.30000000000369,5.80499688086099));
#52206=CARTESIAN_POINT('Ctrl Pts',(4.55542077951101,-1.30000000000301,6.0091065818418));
#52207=CARTESIAN_POINT('Ctrl Pts',(4.49515867257234,-1.1851427086138,6.01776346089841));
#52208=CARTESIAN_POINT('Ctrl Pts',(4.44076843666203,-1.06847604194611,6.02506284513832));
#52209=CARTESIAN_POINT('Ctrl Pts',(4.32868130771967,-0.794772684000799,
6.03878979837678));
#52210=CARTESIAN_POINT('Ctrl Pts',(4.26968336791182,-0.636309800095154,
6.04672131813715));
#52211=CARTESIAN_POINT('Ctrl Pts',(4.19523270114734,-0.319434907277137,
6.04799361755878));
#52212=CARTESIAN_POINT('Ctrl Pts',(4.16886869472472,-0.158333333333322,
6.04709843557643));
#52213=CARTESIAN_POINT('Ctrl Pts',(4.1623841418559,0.158333333333324,6.02456257462145));
#52214=CARTESIAN_POINT('Ctrl Pts',(4.18256377673187,0.319434907277147,6.00407772113189));
#52215=CARTESIAN_POINT('Ctrl Pts',(4.24319442846635,0.636309800095165,5.95454716229398));
#52216=CARTESIAN_POINT('Ctrl Pts',(4.29447370823118,0.794772684000787,5.91935837850987));
#52217=CARTESIAN_POINT('Ctrl Pts',(4.39365357926063,1.06847604194633,5.86048505252226));
#52218=CARTESIAN_POINT('Ctrl Pts',(4.44247879492748,1.18514270861423,5.83376298909323));
#52219=CARTESIAN_POINT('Ctrl Pts',(4.49719793506867,1.30000000000366,5.80580294358365));
#52220=CARTESIAN_POINT('Ctrl Pts',(4.57961335592317,-1.30000000000298,6.01326169023633));
#52221=CARTESIAN_POINT('Ctrl Pts',(4.52404695564334,-1.18514270861378,6.02217753251362));
#52222=CARTESIAN_POINT('Ctrl Pts',(4.47306199948735,-1.06847604194609,6.02944633197147));
#52223=CARTESIAN_POINT('Ctrl Pts',(4.36586060370283,-0.794772684000784,
6.04243371443469));
#52224=CARTESIAN_POINT('Ctrl Pts',(4.30585581723244,-0.636309800095142,
6.04909462591785));
#52225=CARTESIAN_POINT('Ctrl Pts',(4.23121474878952,-0.319434907277131,
6.04828584773161));
#52226=CARTESIAN_POINT('Ctrl Pts',(4.2029207811322,-0.158333333333319,6.04532202205807));
#52227=CARTESIAN_POINT('Ctrl Pts',(4.19628041448162,0.158333333333321,6.02203922050159));
#52228=CARTESIAN_POINT('Ctrl Pts',(4.21813530655345,0.31943490727714,6.00249961225309));
#52229=CARTESIAN_POINT('Ctrl Pts',(4.27884041084526,0.636309800095152,5.95429548433113));
#52230=CARTESIAN_POINT('Ctrl Pts',(4.33126058845234,0.794772684000772,5.92069046234265));
#52231=CARTESIAN_POINT('Ctrl Pts',(4.42567265879968,1.06847604194631,5.86279094197079));
#52232=CARTESIAN_POINT('Ctrl Pts',(4.47115504984018,1.18514270861421,5.83626623457124));
#52233=CARTESIAN_POINT('Ctrl Pts',(4.52125234497956,1.30000000000364,5.8082793767526));
#52234=CARTESIAN_POINT('Ctrl Pts',(4.60381579105714,-1.30000000000298,6.01754841177121));
#52235=CARTESIAN_POINT('Ctrl Pts',(4.55290203223089,-1.18514270861378,6.02632358361635));
#52236=CARTESIAN_POINT('Ctrl Pts',(4.50530124431252,-1.06847604194609,6.03336789866386));
#52237=CARTESIAN_POINT('Ctrl Pts',(4.40298752727133,-0.794772684000784,
6.04564305017475));
#52238=CARTESIAN_POINT('Ctrl Pts',(4.34201232346892,-0.636309800095145,
6.05164736415331));
#52239=CARTESIAN_POINT('Ctrl Pts',(4.26733571815094,-0.319434907277134,
6.04969354682945));
#52240=CARTESIAN_POINT('Ctrl Pts',(4.23737292911869,-0.158333333333319,
6.04591398439182));
#52241=CARTESIAN_POINT('Ctrl Pts',(4.23058205335565,0.158333333333322,6.02181828848998));
#52242=CARTESIAN_POINT('Ctrl Pts',(4.25388869406487,0.319434907277141,6.00196886684759));
#52243=CARTESIAN_POINT('Ctrl Pts',(4.31445834431823,0.636309800095155,5.95389082819043));
#52244=CARTESIAN_POINT('Ctrl Pts',(4.36786778497214,0.794772684000777,5.92103100417116));
#52245=CARTESIAN_POINT('Ctrl Pts',(4.45743057115858,1.06847604194631,5.86363653008099));
#52246=CARTESIAN_POINT('Ctrl Pts',(4.49956711306004,1.18514270861421,5.83728451025261));
#52247=CARTESIAN_POINT('Ctrl Pts',(4.54507178535092,1.30000000000364,5.80942441175477));
#52248=CARTESIAN_POINT('Ctrl Pts',(4.62354611479265,-1.30000000000292,6.02187971789063));
#52249=CARTESIAN_POINT('Ctrl Pts',(4.57654041299366,-1.18514270861372,6.03190893581532));
#52250=CARTESIAN_POINT('Ctrl Pts',(4.53176285751006,-1.06847604194604,6.03955116088897));
#52251=CARTESIAN_POINT('Ctrl Pts',(4.43346521035186,-0.794772684000746,
6.05169179862876));
#52252=CARTESIAN_POINT('Ctrl Pts',(4.37152877982439,-0.636309800095112,
6.05516887015694));
#52253=CARTESIAN_POINT('Ctrl Pts',(4.29671435794294,-0.319434907277116,
6.05124212051647));
#52254=CARTESIAN_POINT('Ctrl Pts',(4.26531192771955,-0.158333333333311,
6.04636116710423));
#52255=CARTESIAN_POINT('Ctrl Pts',(4.25842001866299,0.158333333333313,6.02170035863254));
#52256=CARTESIAN_POINT('Ctrl Pts',(4.28302862982561,0.319434907277126,6.00238960620395));
#52257=CARTESIAN_POINT('Ctrl Pts',(4.34360492693411,0.636309800095123,5.9551285363422));
#52258=CARTESIAN_POINT('Ctrl Pts',(4.39787976032314,0.794772684000733,5.92328230146951));
#52259=CARTESIAN_POINT('Ctrl Pts',(4.48356835798253,1.06847604194626,5.86660248501926));
#52260=CARTESIAN_POINT('Ctrl Pts',(4.52300590752555,1.18514270861416,5.84043964376399));
#52261=CARTESIAN_POINT('Ctrl Pts',(4.56478958776009,1.30000000000358,5.81264855360073));
#52262=CARTESIAN_POINT('Ctrl Pts',(4.63874413860242,-1.30000000000292,6.02548249806497));
#52263=CARTESIAN_POINT('Ctrl Pts',(4.59465672471239,-1.18514270861372,6.03557603946561));
#52264=CARTESIAN_POINT('Ctrl Pts',(4.55200234525745,-1.06847604194603,6.04316523301098));
#52265=CARTESIAN_POINT('Ctrl Pts',(4.45677279196024,-0.794772684000744,
6.05491224377494));
#52266=CARTESIAN_POINT('Ctrl Pts',(4.39422085386997,-0.636309800095109,
6.05770680163088));
#52267=CARTESIAN_POINT('Ctrl Pts',(4.31940808634673,-0.319434907277114,
6.0530565082544));
#52268=CARTESIAN_POINT('Ctrl Pts',(4.28699461990195,-0.158333333333311,
6.04781261330039));
#52269=CARTESIAN_POINT('Ctrl Pts',(4.28003945825534,0.158333333333313,6.0227713625454));
#52270=CARTESIAN_POINT('Ctrl Pts',(4.30556805694205,0.319434907277125,6.00333617711307));
#52271=CARTESIAN_POINT('Ctrl Pts',(4.36607047738981,0.63630980009512,5.95624153076773));
#52272=CARTESIAN_POINT('Ctrl Pts',(4.4209775188318,0.79477268400073,5.92504094672903));
#52273=CARTESIAN_POINT('Ctrl Pts',(4.5035970151742,1.06847604194625,5.86842779829152));
#52274=CARTESIAN_POINT('Ctrl Pts',(4.54091462698009,1.18514270861415,5.84216667581498));
#52275=CARTESIAN_POINT('Ctrl Pts',(4.57978693197907,1.30000000000357,5.81415016509678));
#52276=CARTESIAN_POINT('Ctrl Pts',(4.64482079169386,-1.30000000000291,6.02690740127364));
#52277=CARTESIAN_POINT('Ctrl Pts',(4.60191504159934,-1.18514270861371,6.03716613059751));
#52278=CARTESIAN_POINT('Ctrl Pts',(4.56011944211076,-1.06847604194603,6.04482333556412));
#52279=CARTESIAN_POINT('Ctrl Pts',(4.46612791609618,-0.794772684000742,
6.0565029691571));
#52280=CARTESIAN_POINT('Ctrl Pts',(4.40332274652645,-0.636309800095109,
6.05891824706142));
#52281=CARTESIAN_POINT('Ctrl Pts',(4.32849953478007,-0.319434907277114,
6.0538798088146));
#52282=CARTESIAN_POINT('Ctrl Pts',(4.29565827532708,-0.158333333333311,
6.04833685913728));
#52283=CARTESIAN_POINT('Ctrl Pts',(4.28868341905821,0.158333333333313,6.02317300087302));
#52284=CARTESIAN_POINT('Ctrl Pts',(4.31460773806686,0.319434907277124,6.00386949195305));
#52285=CARTESIAN_POINT('Ctrl Pts',(4.37510569943537,0.63630980009512,5.95700444250547));
#52286=CARTESIAN_POINT('Ctrl Pts',(4.43028166958698,0.794772684000729,5.92617200183776));
#52287=CARTESIAN_POINT('Ctrl Pts',(4.51167910779437,1.06847604194625,5.86961587904899));
#52288=CARTESIAN_POINT('Ctrl Pts',(4.54814679444583,1.18514270861415,5.84329781936374));
#52289=CARTESIAN_POINT('Ctrl Pts',(4.5858482328209,1.30000000000357,5.81514274993776));
#52290=CARTESIAN_POINT('Ctrl Pts',(4.65541484816498,-1.30000000000291,6.02904115986957));
#52291=CARTESIAN_POINT('Ctrl Pts',(4.61460498496626,-1.18514270861371,6.0399105177876));
#52292=CARTESIAN_POINT('Ctrl Pts',(4.5743320538263,-1.06847604194603,6.04790675769232));
#52293=CARTESIAN_POINT('Ctrl Pts',(4.48253394678982,-0.794772684000739,
6.05974219413844));
#52294=CARTESIAN_POINT('Ctrl Pts',(4.41928383318675,-0.636309800095105,
6.06137265385868));
#52295=CARTESIAN_POINT('Ctrl Pts',(4.34442306225996,-0.319434907277113,
6.05547552036877));
#52296=CARTESIAN_POINT('Ctrl Pts',(4.31079257432893,-0.15833333333331,6.04910982007256));
#52297=CARTESIAN_POINT('Ctrl Pts',(4.30376503396204,0.158333333333312,6.02357447304307));
#52298=CARTESIAN_POINT('Ctrl Pts',(4.33039479005563,0.319434907277123,6.00457287561657));
#52299=CARTESIAN_POINT('Ctrl Pts',(4.39088636021054,0.636309800095117,5.95811404147546));
#52300=CARTESIAN_POINT('Ctrl Pts',(4.44652348451578,0.794772684000725,5.92788673225629));
#52301=CARTESIAN_POINT('Ctrl Pts',(4.52579694767258,1.06847604194624,5.87152878984834));
#52302=CARTESIAN_POINT('Ctrl Pts',(4.56078851772166,1.18514270861415,5.84518250637771));
#52303=CARTESIAN_POINT('Ctrl Pts',(4.59645711299034,1.30000000000357,5.81688520443742));
#52304=CARTESIAN_POINT('Ctrl Pts',(4.6766367318432,-1.30000000000289,6.03366080550862));
#52305=CARTESIAN_POINT('Ctrl Pts',(4.63993747158105,-1.18514270861369,6.04487333679941));
#52306=CARTESIAN_POINT('Ctrl Pts',(4.60265480542224,-1.06847604194601,6.05297495110862));
#52307=CARTESIAN_POINT('Ctrl Pts',(4.51517660389278,-0.794772684000726,
6.06450446032101));
#52308=CARTESIAN_POINT('Ctrl Pts',(4.45105908241519,-0.636309800095095,
6.06509936357692));
#52309=CARTESIAN_POINT('Ctrl Pts',(4.37619392540727,-0.319434907277107,
6.05814915506877));
#52310=CARTESIAN_POINT('Ctrl Pts',(4.3410990948752,-0.158333333333307,6.05094393173563));
#52311=CARTESIAN_POINT('Ctrl Pts',(4.3340396043192,0.158333333333309,6.02527429564328));
#52312=CARTESIAN_POINT('Ctrl Pts',(4.36212647356014,0.319434907277117,6.00728440154909));
#52313=CARTESIAN_POINT('Ctrl Pts',(4.42250699520338,0.636309800095105,5.96098084925809));
#52314=CARTESIAN_POINT('Ctrl Pts',(4.47882945207936,0.794772684000713,5.93021983262011));
#52315=CARTESIAN_POINT('Ctrl Pts',(4.55375622132621,1.06847604194623,5.87358000316449));
#52316=CARTESIAN_POINT('Ctrl Pts',(4.58578679647162,1.18514270861412,5.84713790028093));
#52317=CARTESIAN_POINT('Ctrl Pts',(4.61741492466572,1.30000000000354,5.81877097797278));
#52318=CARTESIAN_POINT('Ctrl Pts',(4.70094536200485,-1.30000000000283,6.040011863196));
#52319=CARTESIAN_POINT('Ctrl Pts',(4.66902133675282,-1.18514270861363,6.05279341445746));
#52320=CARTESIAN_POINT('Ctrl Pts',(4.63520845163771,-1.06847604194596,6.0617460142815));
#52321=CARTESIAN_POINT('Ctrl Pts',(4.55273027862888,-0.794772684000688,
6.07358266703692));
#52322=CARTESIAN_POINT('Ctrl Pts',(4.48757147724743,-0.636309800095066,
6.07175891365129));
#52323=CARTESIAN_POINT('Ctrl Pts',(4.41268620746716,-0.319434907277093,
6.0629803630447));
#52324=CARTESIAN_POINT('Ctrl Pts',(4.37595562502286,-0.1583333333333,6.05490103609209));
#52325=CARTESIAN_POINT('Ctrl Pts',(4.36875227568137,0.158333333333302,6.0281015831388));
#52326=CARTESIAN_POINT('Ctrl Pts',(4.39823174652913,0.319434907277102,6.00933141895887));
#52327=CARTESIAN_POINT('Ctrl Pts',(4.45854160063371,0.636309800095077,5.96362333769257));
#52328=CARTESIAN_POINT('Ctrl Pts',(4.51608172583745,0.794772684000676,5.93551344003385));
#52329=CARTESIAN_POINT('Ctrl Pts',(4.58609921371453,1.06847604194618,5.87892679803689));
#52330=CARTESIAN_POINT('Ctrl Pts',(4.61469399881586,1.18514270861407,5.85194577731453));
#52331=CARTESIAN_POINT('Ctrl Pts',(4.64157559291995,1.30000000000348,5.8224779964487));
#52332=CARTESIAN_POINT('Ctrl Pts',(4.72069270328122,-1.3000000000028,6.04521039352825));
#52333=CARTESIAN_POINT('Ctrl Pts',(4.69257203670566,-1.18514270861361,6.05835663747547));
#52334=CARTESIAN_POINT('Ctrl Pts',(4.66154109137681,-1.06847604194594,6.06755884022885));
#52335=CARTESIAN_POINT('Ctrl Pts',(4.58313007382887,-0.794772684000672,
6.07970624532299));
#52336=CARTESIAN_POINT('Ctrl Pts',(4.51731897215768,-0.636309800095054,
6.07820763874449));
#52337=CARTESIAN_POINT('Ctrl Pts',(4.44244429505606,-0.319434907277088,
6.06831849035796));
#52338=CARTESIAN_POINT('Ctrl Pts',(4.40422789755839,-0.158333333333297,
6.05795366283987));
#52339=CARTESIAN_POINT('Ctrl Pts',(4.39695983770024,0.158333333333299,6.03050840572729));
#52340=CARTESIAN_POINT('Ctrl Pts',(4.42783577478779,0.319434907277095,6.01316697049685));
#52341=CARTESIAN_POINT('Ctrl Pts',(4.48805341198737,0.636309800095063,5.96768375595659));
#52342=CARTESIAN_POINT('Ctrl Pts',(4.5462177986737,0.794772684000664,5.93901571765619));
#52343=CARTESIAN_POINT('Ctrl Pts',(4.61221117101888,1.06847604194616,5.88213897831174));
#52344=CARTESIAN_POINT('Ctrl Pts',(4.63806563950542,1.18514270861405,5.85505464187112));
#52345=CARTESIAN_POINT('Ctrl Pts',(4.66120849088553,1.30000000000346,5.82550580196134));
#52346=CARTESIAN_POINT('Ctrl Pts',(4.73277983786844,-1.3000000000028,6.04774757720061));
#52347=CARTESIAN_POINT('Ctrl Pts',(4.70702828209547,-1.18514270861361,6.06144066240088));
#52348=CARTESIAN_POINT('Ctrl Pts',(4.67772380816164,-1.06847604194593,6.07096186531051));
#52349=CARTESIAN_POINT('Ctrl Pts',(4.60181665932455,-0.794772684000669,
6.08331986606822));
#52350=CARTESIAN_POINT('Ctrl Pts',(4.53551006683239,-0.636309800095052,
6.0810430560724));
#52351=CARTESIAN_POINT('Ctrl Pts',(4.46068656840018,-0.319434907277087,
6.0708469211743));
#52352=CARTESIAN_POINT('Ctrl Pts',(4.42170832034993,-0.158333333333296,
6.06048747780477));
#52353=CARTESIAN_POINT('Ctrl Pts',(4.41444165181559,0.158333333333298,6.03307259932769));
#52354=CARTESIAN_POINT('Ctrl Pts',(4.44609545841066,0.319434907277094,6.01595725300538));
#52355=CARTESIAN_POINT('Ctrl Pts',(4.50623495553593,0.636309800095061,5.97043328921319));
#52356=CARTESIAN_POINT('Ctrl Pts',(4.5648121875001,0.794772684000661,5.94159185355148));
#52357=CARTESIAN_POINT('Ctrl Pts',(4.62831581752182,1.06847604194616,5.88441441473242));
#52358=CARTESIAN_POINT('Ctrl Pts',(4.65247175398913,1.18514270861404,5.85717138499989));
#52359=CARTESIAN_POINT('Ctrl Pts',(4.6732952585286,1.30000000000345,5.82743532016684));
#52360=CARTESIAN_POINT('Ctrl Pts',(4.74494445621426,-1.30000000000275,6.05141731309816));
#52361=CARTESIAN_POINT('Ctrl Pts',(4.72159046772432,-1.18514270861356,6.06624105700331));
#52362=CARTESIAN_POINT('Ctrl Pts',(4.69402959774547,-1.0684760419459,6.07641364231617));
#52363=CARTESIAN_POINT('Ctrl Pts',(4.62063973673839,-0.794772684000642,
6.08916924259824));
#52364=CARTESIAN_POINT('Ctrl Pts',(4.55383037099021,-0.63630980009503,6.08549942988976));
#52365=CARTESIAN_POINT('Ctrl Pts',(4.47898769993957,-0.319434907277075,
6.074077080766));
#52366=CARTESIAN_POINT('Ctrl Pts',(4.43914810147163,-0.158333333333291,
6.06277640534756));
#52367=CARTESIAN_POINT('Ctrl Pts',(4.43180983029836,0.158333333333293,6.0346854767056));
#52368=CARTESIAN_POINT('Ctrl Pts',(4.46420681851606,0.319434907277083,6.01758245701524));
#52369=CARTESIAN_POINT('Ctrl Pts',(4.52431449074692,0.636309800095039,5.97242268988233));
#52370=CARTESIAN_POINT('Ctrl Pts',(4.5834589120997,0.794772684000632,5.94471142931503));
#52371=CARTESIAN_POINT('Ctrl Pts',(4.64450497239395,1.06847604194612,5.88749046259075));
#52372=CARTESIAN_POINT('Ctrl Pts',(4.66694884054746,1.185142708614,5.8599635463673));
#52373=CARTESIAN_POINT('Ctrl Pts',(4.68541199933239,1.30000000000341,5.82967855016972));
#52374=CARTESIAN_POINT('Ctrl Pts',(4.76168328182841,-1.30000000000272,6.05637407538914));
#52375=CARTESIAN_POINT('Ctrl Pts',(4.74151822683416,-1.18514270861354,6.07120642815316));
#52376=CARTESIAN_POINT('Ctrl Pts',(4.71629112175755,-1.06847604194587,6.08139554862026));
#52377=CARTESIAN_POINT('Ctrl Pts',(4.64631711401595,-0.794772684000621,
6.09420765974442));
#52378=CARTESIAN_POINT('Ctrl Pts',(4.5789340665717,-0.636309800095014,6.09077707494308));
#52379=CARTESIAN_POINT('Ctrl Pts',(4.50417819467794,-0.319434907277067,
6.07909088955251));
#52380=CARTESIAN_POINT('Ctrl Pts',(4.4632640376533,-0.158333333333287,6.06732493430611));
#52381=CARTESIAN_POINT('Ctrl Pts',(4.45587334963848,0.158333333333289,6.03864220529557));
#52382=CARTESIAN_POINT('Ctrl Pts',(4.48924849400527,0.319434907277077,6.02098088567907));
#52383=CARTESIAN_POINT('Ctrl Pts',(4.54925219317818,0.636309800095025,5.97575900359238));
#52384=CARTESIAN_POINT('Ctrl Pts',(4.60908633115064,0.794772684000613,5.94897774902275));
#52385=CARTESIAN_POINT('Ctrl Pts',(4.66673128287468,1.06847604194609,5.89150927474576));
#52386=CARTESIAN_POINT('Ctrl Pts',(4.68683018214767,1.18514270861397,5.86364625932992));
#52387=CARTESIAN_POINT('Ctrl Pts',(4.70207561704814,1.30000000000337,5.83279620159604));
#52388=CARTESIAN_POINT('Ctrl Pts',(4.7798379970422,-1.30000000000266,6.06110253687931));
#52389=CARTESIAN_POINT('Ctrl Pts',(4.76328097334858,-1.18514270861348,6.07786348671036));
#52390=CARTESIAN_POINT('Ctrl Pts',(4.74067709072031,-1.06847604194582,6.08918028975207));
#52391=CARTESIAN_POINT('Ctrl Pts',(4.67448814614907,-0.794772684000584,
6.10274730051581));
#52392=CARTESIAN_POINT('Ctrl Pts',(4.60630253549995,-0.636309800094985,
6.09662993565042));
#52393=CARTESIAN_POINT('Ctrl Pts',(4.53159424561923,-0.319434907277053,
6.0838013327509));
#52394=CARTESIAN_POINT('Ctrl Pts',(4.48951023736959,-0.15833333333328,6.07183198905575));
#52395=CARTESIAN_POINT('Ctrl Pts',(4.4821426868114,0.158333333333282,6.04335038428183));
#52396=CARTESIAN_POINT('Ctrl Pts',(4.51675951190241,0.319434907277061,6.02682073307529));
#52397=CARTESIAN_POINT('Ctrl Pts',(4.57666357621065,0.636309800094995,5.98166978023208));
#52398=CARTESIAN_POINT('Ctrl Pts',(4.63708456690679,0.794772684000577,5.95424377633781));
#52399=CARTESIAN_POINT('Ctrl Pts',(4.69095441782067,1.06847604194604,5.8958353667492));
#52400=CARTESIAN_POINT('Ctrl Pts',(4.70848363320909,1.18514270861392,5.86747665052283));
#52401=CARTESIAN_POINT('Ctrl Pts',(4.72022380159989,1.30000000000331,5.83604205433626));
#52402=CARTESIAN_POINT('Ctrl Pts',(4.79803929283521,-1.30000000000263,6.06614678322407));
#52403=CARTESIAN_POINT('Ctrl Pts',(4.78497732456114,-1.18514270861345,6.08322755623773));
#52404=CARTESIAN_POINT('Ctrl Pts',(4.76493629506773,-1.0684760419458,6.09485086245138));
#52405=CARTESIAN_POINT('Ctrl Pts',(4.702514480171,-0.794772684000566,6.10909518496873));
#52406=CARTESIAN_POINT('Ctrl Pts',(4.6337583158824,-0.636309800094968,6.10392234455836));
#52407=CARTESIAN_POINT('Ctrl Pts',(4.55913407892579,-0.319434907277044,
6.09061273470484));
#52408=CARTESIAN_POINT('Ctrl Pts',(4.51580190865141,-0.158333333333275,
6.07705069401337));
#52409=CARTESIAN_POINT('Ctrl Pts',(4.5083421663999,0.158333333333278,6.04742756797417));
#52410=CARTESIAN_POINT('Ctrl Pts',(4.544036612003,0.319434907277053,6.03047774157301));
#52411=CARTESIAN_POINT('Ctrl Pts',(4.60382842848645,0.636309800094978,5.98525747815496));
#52412=CARTESIAN_POINT('Ctrl Pts',(4.66500701574621,0.794772684000556,5.95889528869559));
#52413=CARTESIAN_POINT('Ctrl Pts',(4.71517494313533,1.06847604194601,5.90023635608127));
#52414=CARTESIAN_POINT('Ctrl Pts',(4.73015035970638,1.18514270861389,5.87151429963215));
#52415=CARTESIAN_POINT('Ctrl Pts',(4.73838535598652,1.30000000000328,5.83946146513514));
#52416=CARTESIAN_POINT('Ctrl Pts',(4.81094807828055,-1.30000000000258,6.07031856917121));
#52417=CARTESIAN_POINT('Ctrl Pts',(4.80040109501589,-1.18514270861341,6.08840887737886));
#52418=CARTESIAN_POINT('Ctrl Pts',(4.78219419594427,-1.06847604194576,6.10063671605705));
#52419=CARTESIAN_POINT('Ctrl Pts',(4.72243667893648,-0.794772684000535,
6.11534199217825));
#52420=CARTESIAN_POINT('Ctrl Pts',(4.65317658805189,-0.636309800094944,
6.10903162237028));
#52421=CARTESIAN_POINT('Ctrl Pts',(4.57859096384098,-0.319434907277032,
6.09488648935993));
#52422=CARTESIAN_POINT('Ctrl Pts',(4.53439696116877,-0.158333333333269,
6.08059548100309));
#52423=CARTESIAN_POINT('Ctrl Pts',(4.52693655107921,0.158333333333272,6.05083684999365));
#52424=CARTESIAN_POINT('Ctrl Pts',(4.56349429876338,0.319434907277041,6.03460096200745));
#52425=CARTESIAN_POINT('Ctrl Pts',(4.62324178818616,0.636309800094954,5.98969480751174));
#52426=CARTESIAN_POINT('Ctrl Pts',(4.68491393411039,0.794772684000524,5.96367396250213));
#52427=CARTESIAN_POINT('Ctrl Pts',(4.73241342899345,1.06847604194597,5.90433667604155));
#52428=CARTESIAN_POINT('Ctrl Pts',(4.74555459285911,1.18514270861384,5.87507424421135));
#52429=CARTESIAN_POINT('Ctrl Pts',(4.75127614928519,1.30000000000323,5.84223429319674));
#52430=CARTESIAN_POINT('Ctrl Pts',(4.8185298804356,-1.30000000000257,6.07259108813827));
#52431=CARTESIAN_POINT('Ctrl Pts',(4.80945416287109,-1.1851427086134,6.09110994876213));
#52432=CARTESIAN_POINT('Ctrl Pts',(4.79232260434384,-1.06847604194575,6.10361999370318));
#52433=CARTESIAN_POINT('Ctrl Pts',(4.73413467280032,-0.794772684000532,
6.11863913385612));
#52434=CARTESIAN_POINT('Ctrl Pts',(4.66460317470995,-0.636309800094941,
6.11214114341466));
#52435=CARTESIAN_POINT('Ctrl Pts',(4.5900426618142,-0.31943490727703,6.09758341926879));
#52436=CARTESIAN_POINT('Ctrl Pts',(4.54532685018444,-0.158333333333269,
6.08260397486844));
#52437=CARTESIAN_POINT('Ctrl Pts',(4.53785597458308,0.158333333333271,6.05264851354725));
#52438=CARTESIAN_POINT('Ctrl Pts',(4.57491371826594,0.319434907277039,6.03679573423671));
#52439=CARTESIAN_POINT('Ctrl Pts',(4.63463789281222,0.636309800094951,5.99212224239495));
#52440=CARTESIAN_POINT('Ctrl Pts',(4.69661644685499,0.794772684000521,5.96647342222013));
#52441=CARTESIAN_POINT('Ctrl Pts',(4.74255240611472,1.06847604194597,5.90679120314264));
#52442=CARTESIAN_POINT('Ctrl Pts',(4.75461520664285,1.18514270861384,5.87720825205933));
#52443=CARTESIAN_POINT('Ctrl Pts',(4.75885683303048,1.30000000000322,5.84387657108736));
#52444=CARTESIAN_POINT('Ctrl Pts',(4.82156335065102,-1.30000000000257,6.07351992691993));
#52445=CARTESIAN_POINT('Ctrl Pts',(4.81307603159707,-1.1851427086134,6.09221744319849));
#52446=CARTESIAN_POINT('Ctrl Pts',(4.79637446542063,-1.06847604194575,6.10484289962611));
#52447=CARTESIAN_POINT('Ctrl Pts',(4.73881395230902,-0.79477268400053,6.11998255672066));
#52448=CARTESIAN_POINT('Ctrl Pts',(4.669172937198,-0.63630980009494,6.11337925974468));
#52449=CARTESIAN_POINT('Ctrl Pts',(4.59462305158774,-0.31943490727703,6.09865712892641));
#52450=CARTESIAN_POINT('Ctrl Pts',(4.54970080024142,-0.158333333333268,
6.08343482517382));
#52451=CARTESIAN_POINT('Ctrl Pts',(4.54222563209188,0.158333333333271,6.05339961884823));
#52452=CARTESIAN_POINT('Ctrl Pts',(4.57948149923688,0.319434907277039,6.03767582519329));
#52453=CARTESIAN_POINT('Ctrl Pts',(4.63919449888597,0.63630980009495,5.9930738228806));
#52454=CARTESIAN_POINT('Ctrl Pts',(4.70129367065987,0.79477268400052,5.9675537403918));
#52455=CARTESIAN_POINT('Ctrl Pts',(4.7466045404738,1.06847604194597,5.90773699490193));
#52456=CARTESIAN_POINT('Ctrl Pts',(4.758236768349,1.18514270861383,5.87803411752938));
#52457=CARTESIAN_POINT('Ctrl Pts',(4.76188782749003,1.30000000000322,5.84452081547814));
#52458=CARTESIAN_POINT('Ctrl Pts',(4.82687180554659,-1.30000000000256,6.07516303402758));
#52459=CARTESIAN_POINT('Ctrl Pts',(4.81941366164088,-1.1851427086134,6.09418064141752));
#52460=CARTESIAN_POINT('Ctrl Pts',(4.80346422963748,-1.06847604194575,6.10701136017159));
#52461=CARTESIAN_POINT('Ctrl Pts',(4.74700127685497,-0.794772684000528,
6.12235993683822));
#52462=CARTESIAN_POINT('Ctrl Pts',(4.67716837738524,-0.636309800094938,
6.11554555143684));
#52463=CARTESIAN_POINT('Ctrl Pts',(4.60263831817618,-0.319434907277029,
6.10054193746771));
#52464=CARTESIAN_POINT('Ctrl Pts',(4.55735821474082,-0.158333333333268,
6.08493920424772));
#52465=CARTESIAN_POINT('Ctrl Pts',(4.54987431150987,0.15833333333327,6.05475127028888));
#52466=CARTESIAN_POINT('Ctrl Pts',(4.58747219868369,0.319434907277038,6.03919945093894));
#52467=CARTESIAN_POINT('Ctrl Pts',(4.64716203523448,0.636309800094948,5.99468134954926));
#52468=CARTESIAN_POINT('Ctrl Pts',(4.70946959676387,0.794772684000518,5.96935828691381));
#52469=CARTESIAN_POINT('Ctrl Pts',(4.75368817807476,1.06847604194596,5.90931968376478));
#52470=CARTESIAN_POINT('Ctrl Pts',(4.76456883971137,1.18514270861383,5.87942535681887));
#52471=CARTESIAN_POINT('Ctrl Pts',(4.76718957759493,1.30000000000322,5.84562518958093));
#52472=CARTESIAN_POINT('Ctrl Pts',(4.83294183153657,-1.30000000000255,6.07717547848024));
#52473=CARTESIAN_POINT('Ctrl Pts',(4.82666302720955,-1.18514270861339,6.09667934639319));
#52474=CARTESIAN_POINT('Ctrl Pts',(4.81157442383178,-1.06847604194574,6.10980130540581));
#52475=CARTESIAN_POINT('Ctrl Pts',(4.75636433336315,-0.794772684000522,
6.12537216950749));
#52476=CARTESIAN_POINT('Ctrl Pts',(4.68629888445387,-0.636309800094933,
6.11797637025502));
#52477=CARTESIAN_POINT('Ctrl Pts',(4.61179504573014,-0.319434907277026,
6.10263727675094));
#52478=CARTESIAN_POINT('Ctrl Pts',(4.56612601490908,-0.158333333333267,
6.0868969511743));
#52479=CARTESIAN_POINT('Ctrl Pts',(4.55863200153038,0.158333333333269,6.05653705639946));
#52480=CARTESIAN_POINT('Ctrl Pts',(4.59660638914432,0.319434907277035,6.0409884473164));
#52481=CARTESIAN_POINT('Ctrl Pts',(4.65625413071718,0.636309800094943,5.99637900850148));
#52482=CARTESIAN_POINT('Ctrl Pts',(4.71878104658324,0.794772684000511,5.97108276538689));
#52483=CARTESIAN_POINT('Ctrl Pts',(4.76175471078031,1.06847604194595,5.91081980006133));
#52484=CARTESIAN_POINT('Ctrl Pts',(4.77178386433909,1.18514270861382,5.88078275953025));
#52485=CARTESIAN_POINT('Ctrl Pts',(4.77324046455682,1.30000000000321,5.84679428319473));
#52486=CARTESIAN_POINT('Ctrl Pts',(4.8390112966445,-1.30000000000254,6.07922833436859));
#52487=CARTESIAN_POINT('Ctrl Pts',(4.8339135640654,-1.18514270861338,6.09927229604029));
#52488=CARTESIAN_POINT('Ctrl Pts',(4.81968675892488,-1.06847604194573,6.11271650145966));
#52489=CARTESIAN_POINT('Ctrl Pts',(4.76573000910636,-0.794772684000516,
6.12852854826283));
#52490=CARTESIAN_POINT('Ctrl Pts',(4.69542749616083,-0.636309800094927,
6.12045465101031));
#52491=CARTESIAN_POINT('Ctrl Pts',(4.62095209785004,-0.319434907277023,
6.10478117796908));
#52492=CARTESIAN_POINT('Ctrl Pts',(4.57490134636149,-0.158333333333265,
6.08897820923182));
#52493=CARTESIAN_POINT('Ctrl Pts',(4.56739926580259,0.158333333333267,6.05846060622671));
#52494=CARTESIAN_POINT('Ctrl Pts',(4.60574790329659,0.319434907277033,6.04289046439477));
#52495=CARTESIAN_POINT('Ctrl Pts',(4.66534955738218,0.636309800094938,5.99814438476442));
#52496=CARTESIAN_POINT('Ctrl Pts',(4.72808987051969,0.794772684000504,5.97281491664591));
#52497=CARTESIAN_POINT('Ctrl Pts',(4.7698168520734,1.06847604194594,5.91230119986894));
#52498=CARTESIAN_POINT('Ctrl Pts',(4.77899489585878,1.18514270861381,5.88212034815777));
#52499=CARTESIAN_POINT('Ctrl Pts',(4.77928891925188,1.3000000000032,5.84795279047415));
#52500=CARTESIAN_POINT('Ctrl Pts',(4.84356149439792,-1.30000000000254,6.08073619732913));
#52501=CARTESIAN_POINT('Ctrl Pts',(4.8393482645136,-1.18514270861337,6.1011533481644));
#52502=CARTESIAN_POINT('Ctrl Pts',(4.82576733162132,-1.06847604194572,6.11482793676999));
#52503=CARTESIAN_POINT('Ctrl Pts',(4.77275139183321,-0.794772684000512,
6.13084230444543));
#52504=CARTESIAN_POINT('Ctrl Pts',(4.70227599982204,-0.636309800094924,
6.12238275651382));
#52505=CARTESIAN_POINT('Ctrl Pts',(4.6278224045325,-0.319434907277022,6.10647297836777));
#52506=CARTESIAN_POINT('Ctrl Pts',(4.58148079102623,-0.158333333333265,
6.09052479916083));
#52507=CARTESIAN_POINT('Ctrl Pts',(4.57397362820661,0.158333333333267,6.0598899687823));
#52508=CARTESIAN_POINT('Ctrl Pts',(4.61260710790117,0.319434907277032,6.04436986604123));
#52509=CARTESIAN_POINT('Ctrl Pts',(4.67217851650135,0.636309800094935,5.99957638132379));
#52510=CARTESIAN_POINT('Ctrl Pts',(4.7350844771806,0.794772684000501,5.97428347733527));
#52511=CARTESIAN_POINT('Ctrl Pts',(4.77587357611191,1.06847604194594,5.91354819880508));
#52512=CARTESIAN_POINT('Ctrl Pts',(4.78440989833677,1.1851427086138,5.88322022759615));
#52513=CARTESIAN_POINT('Ctrl Pts',(4.78382645324408,1.30000000000319,5.84885433679028));
#52514=CARTESIAN_POINT('Ctrl Pts',(4.84735109619278,-1.30000000000253,6.08194736323051));
#52515=CARTESIAN_POINT('Ctrl Pts',(4.84387297711041,-1.18514270861336,6.10262734294782));
#52516=CARTESIAN_POINT('Ctrl Pts',(4.83082945738997,-1.06847604194572,6.11647464917));
#52517=CARTESIAN_POINT('Ctrl Pts',(4.77859832846308,-0.794772684000508,
6.13267985404193));
#52518=CARTESIAN_POINT('Ctrl Pts',(4.70798563528429,-0.63630980009492,6.12406340049069));
#52519=CARTESIAN_POINT('Ctrl Pts',(4.63355045458484,-0.31943490727702,6.10797546379102));
#52520=CARTESIAN_POINT('Ctrl Pts',(4.58695984285549,-0.158333333333264,
6.09177860752226));
#52521=CARTESIAN_POINT('Ctrl Pts',(4.57944918836609,0.158333333333266,6.06104441523148));
#52522=CARTESIAN_POINT('Ctrl Pts',(4.61832512952634,0.31943490727703,6.04564528896951));
#52523=CARTESIAN_POINT('Ctrl Pts',(4.67787721388067,0.636309800094931,6.000885293576));
#52524=CARTESIAN_POINT('Ctrl Pts',(4.74092911393698,0.794772684000496,5.97570879341499));
#52525=CARTESIAN_POINT('Ctrl Pts',(4.78093385702523,1.06847604194593,5.91475556026459));
#52526=CARTESIAN_POINT('Ctrl Pts',(4.78893147581347,1.1851427086138,5.88425932578742));
#52527=CARTESIAN_POINT('Ctrl Pts',(4.78761014242878,1.30000000000318,5.84965125292416));
#52528=CARTESIAN_POINT('Ctrl Pts',(4.84981335970265,-1.30000000000253,6.08271543673521));
#52529=CARTESIAN_POINT('Ctrl Pts',(4.84681216960126,-1.18514270861336,6.10354542857903));
#52530=CARTESIAN_POINT('Ctrl Pts',(4.83411760053641,-1.06847604194572,6.1174966921877));
#52531=CARTESIAN_POINT('Ctrl Pts',(4.78239696189765,-0.794772684000507,
6.13383566375637));
#52532=CARTESIAN_POINT('Ctrl Pts',(4.71169803130065,-0.63630980009492,6.12518762763234));
#52533=CARTESIAN_POINT('Ctrl Pts',(4.63727503230506,-0.319434907277019,
6.10899387850149));
#52534=CARTESIAN_POINT('Ctrl Pts',(4.59051985296273,-0.158333333333263,
6.09258456230556));
#52535=CARTESIAN_POINT('Ctrl Pts',(4.58300720612642,0.158333333333266,6.06178474597553));
#52536=CARTESIAN_POINT('Ctrl Pts',(4.6220426819302,0.319434907277029,6.04649333922819));
#52537=CARTESIAN_POINT('Ctrl Pts',(4.68158471984265,0.63630980009493,6.00178516205892));
#52538=CARTESIAN_POINT('Ctrl Pts',(4.74473500781343,0.794772684000495,5.97672300320449));
#52539=CARTESIAN_POINT('Ctrl Pts',(4.7842289634859,1.06847604194593,5.91561562779994));
#52540=CARTESIAN_POINT('Ctrl Pts',(4.79187486711119,1.1851427086138,5.88499139560751));
#52541=CARTESIAN_POINT('Ctrl Pts',(4.79007120434632,1.30000000000318,5.85019404978402));
#52542=CARTESIAN_POINT('Ctrl Pts',(4.85094964634893,-1.30000000000253,6.08306779187192));
#52543=CARTESIAN_POINT('Ctrl Pts',(4.84816846260519,-1.18514270861336,6.10396475566952));
#52544=CARTESIAN_POINT('Ctrl Pts',(4.83563490089031,-1.06847604194572,6.11796318511599));
#52545=CARTESIAN_POINT('Ctrl Pts',(4.78414992192894,-0.794772684000507,
6.13436536311531));
#52546=CARTESIAN_POINT('Ctrl Pts',(4.71341155752716,-0.63630980009492,6.1257109881841));
#52547=CARTESIAN_POINT('Ctrl Pts',(4.63899425350069,-0.319434907277019,
6.10947015908353));
#52548=CARTESIAN_POINT('Ctrl Pts',(4.59216286874051,-0.158333333333263,
6.09295777030185));
#52549=CARTESIAN_POINT('Ctrl Pts',(4.58464934874306,0.158333333333266,6.0621275986729));
#52550=CARTESIAN_POINT('Ctrl Pts',(4.62375862448146,0.319434907277029,6.0468883650167));
#52551=CARTESIAN_POINT('Ctrl Pts',(4.68329631008815,0.63630980009493,6.00220728330628));
#52552=CARTESIAN_POINT('Ctrl Pts',(4.74649242772978,0.794772684000495,5.97720262890682));
#52553=CARTESIAN_POINT('Ctrl Pts',(4.78575057188746,1.06847604194593,5.9160228008181));
#52554=CARTESIAN_POINT('Ctrl Pts',(4.79323399432667,1.1851427086138,5.88533740405829));
#52555=CARTESIAN_POINT('Ctrl Pts',(4.79120744325674,1.30000000000318,5.85044909118237));
#52556=CARTESIAN_POINT('Ctrl Pts',(4.85151776293019,-1.30000000000253,6.08324358479667));
#52557=CARTESIAN_POINT('Ctrl Pts',(4.84884655889996,-1.18514270861336,6.10417359305687));
#52558=CARTESIAN_POINT('Ctrl Pts',(4.8363934910204,-1.06847604194572,6.11819544663104));
#52559=CARTESIAN_POINT('Ctrl Pts',(4.78502635064411,-0.794772684000507,
6.13462951415317));
#52560=CARTESIAN_POINT('Ctrl Pts',(4.71426833995495,-0.63630980009492,6.12597354378368));
#52561=CARTESIAN_POINT('Ctrl Pts',(4.63985390202787,-0.319434907277019,
6.10970958088203));
#52562=CARTESIAN_POINT('Ctrl Pts',(4.59298437609572,-0.158333333333263,
6.09314483996833));
#52563=CARTESIAN_POINT('Ctrl Pts',(4.58547042767463,0.158333333333266,6.06229945950021));
#52564=CARTESIAN_POINT('Ctrl Pts',(4.62461662402917,0.319434907277029,6.04708659910565));
#52565=CARTESIAN_POINT('Ctrl Pts',(4.68415218438462,0.63630980009493,6.00241960966407));
#52566=CARTESIAN_POINT('Ctrl Pts',(4.74737129829366,0.794772684000495,5.97744465461301));
#52567=CARTESIAN_POINT('Ctrl Pts',(4.78651153236238,1.06847604194593,5.91622840739023));
#52568=CARTESIAN_POINT('Ctrl Pts',(4.7939136905355,1.1851427086138,5.88551206469203));
#52569=CARTESIAN_POINT('Ctrl Pts',(4.79177564984189,1.30000000000318,5.85057762443301));
#52570=CARTESIAN_POINT('Ctrl Pts',(4.85199117167453,-1.30000000000253,6.08338979720196));
#52571=CARTESIAN_POINT('Ctrl Pts',(4.8494116027254,-1.18514270861336,6.10434707702687));
#52572=CARTESIAN_POINT('Ctrl Pts',(4.83702560731203,-1.06847604194572,6.11838836417142));
#52573=CARTESIAN_POINT('Ctrl Pts',(4.78575667319626,-0.794772684000506,
6.13484921979393));
#52574=CARTESIAN_POINT('Ctrl Pts',(4.71498234069302,-0.636309800094919,
6.12619298053283));
#52575=CARTESIAN_POINT('Ctrl Pts',(4.64057029990235,-0.319434907277019,
6.10990994199582));
#52576=CARTESIAN_POINT('Ctrl Pts',(4.59366895218851,-0.158333333333263,
6.09330085972181));
#52577=CARTESIAN_POINT('Ctrl Pts',(4.58615465430625,0.158333333333266,6.06244281756089));
#52578=CARTESIAN_POINT('Ctrl Pts',(4.62533164690651,0.319434907277029,6.04725236075715));
#52579=CARTESIAN_POINT('Ctrl Pts',(4.68486547541404,0.63630980009493,6.0025975506947));
#52580=CARTESIAN_POINT('Ctrl Pts',(4.74810380440349,0.794772684000494,5.97764789769707));
#52581=CARTESIAN_POINT('Ctrl Pts',(4.78714577026928,1.06847604194593,5.91640110141059));
#52582=CARTESIAN_POINT('Ctrl Pts',(4.79448018794372,1.1851427086138,5.88565868956355));
#52583=CARTESIAN_POINT('Ctrl Pts',(4.79224920291661,1.30000000000318,5.85068533456457));
#52584=CARTESIAN_POINT('Ctrl Pts',(4.85232255024837,-1.30000000000253,6.08349210501827));
#52585=CARTESIAN_POINT('Ctrl Pts',(4.84980711534308,-1.18514270861336,6.10446835008361));
#52586=CARTESIAN_POINT('Ctrl Pts',(4.83746806547677,-1.06847604194572,6.11852320156077));
#52587=CARTESIAN_POINT('Ctrl Pts',(4.78626787610001,-0.794772684000506,
6.13500291632764));
#52588=CARTESIAN_POINT('Ctrl Pts',(4.71548213668488,-0.636309800094919,
6.1263468992948));
#52589=CARTESIAN_POINT('Ctrl Pts',(4.64107179257917,-0.319434907277019,
6.11005080784577));
#52590=CARTESIAN_POINT('Ctrl Pts',(4.59414818736665,-0.158333333333263,
6.0934108481001));
#52591=CARTESIAN_POINT('Ctrl Pts',(4.58663364693649,0.158333333333266,6.06254390033073));
#52592=CARTESIAN_POINT('Ctrl Pts',(4.62583217203044,0.319434907277029,6.04736874073722));
#52593=CARTESIAN_POINT('Ctrl Pts',(4.68536479253069,0.63630980009493,6.00272243929111));
#52594=CARTESIAN_POINT('Ctrl Pts',(4.74861659642694,0.794772684000494,5.97779085964576));
#52595=CARTESIAN_POINT('Ctrl Pts',(4.78758979248769,1.06847604194593,5.91652274959415));
#52596=CARTESIAN_POINT('Ctrl Pts',(4.79487679837593,1.1851427086138,5.88576206683842));
#52597=CARTESIAN_POINT('Ctrl Pts',(4.79258075767685,1.30000000000318,5.85076139596124));
#52598=CARTESIAN_POINT('Ctrl Pts',(4.85251190324314,-1.30000000000253,6.08355044596462));
#52599=CARTESIAN_POINT('Ctrl Pts',(4.85003311963239,-1.18514270861336,6.10453752533249));
#52600=CARTESIAN_POINT('Ctrl Pts',(4.83772089855381,-1.06847604194571,6.11860013226608));
#52601=CARTESIAN_POINT('Ctrl Pts',(4.78655999708807,-0.794772684000506,
6.13509065093837));
#52602=CARTESIAN_POINT('Ctrl Pts',(4.7157677494904,-0.636309800094919,6.12643492366188));
#52603=CARTESIAN_POINT('Ctrl Pts',(4.64135836161881,-0.319434907277019,
6.11013118911448));
#52604=CARTESIAN_POINT('Ctrl Pts',(4.59442199860524,-0.158333333333263,
6.09347303387878));
#52605=CARTESIAN_POINT('Ctrl Pts',(4.58690732254322,0.158333333333266,6.06260105720591));
#52606=CARTESIAN_POINT('Ctrl Pts',(4.62611819457161,0.319434907277029,6.047435271639));
#52607=CARTESIAN_POINT('Ctrl Pts',(4.68565014319882,0.63630980009493,6.00279409494844));
#52608=CARTESIAN_POINT('Ctrl Pts',(4.74890965125886,0.794772684000494,5.97787278285643));
#52609=CARTESIAN_POINT('Ctrl Pts',(4.78784352652163,1.06847604194593,5.91659230348755));
#52610=CARTESIAN_POINT('Ctrl Pts',(4.79510342179896,1.1851427086138,5.88582104180445));
#52611=CARTESIAN_POINT('Ctrl Pts',(4.79277018039452,1.30000000000318,5.85080456729165));
#52612=CARTESIAN_POINT('Ctrl Pts',(4.86472558979003,-1.30000000000256,6.08732701272415));
#52613=CARTESIAN_POINT('Ctrl Pts',(4.8646099437343,-1.18514270861339,6.1090082878518));
#52614=CARTESIAN_POINT('Ctrl Pts',(4.85402760574505,-1.06847604194574,6.12356913043093));
#52615=CARTESIAN_POINT('Ctrl Pts',(4.80540013577967,-0.794772684000528,
6.14075796605051));
#52616=CARTESIAN_POINT('Ctrl Pts',(4.73418764713308,-0.636309800094937,
6.13211774128059));
#52617=CARTESIAN_POINT('Ctrl Pts',(4.65984242997234,-0.319434907277028,
6.11535711134947));
#52618=CARTESIAN_POINT('Ctrl Pts',(4.61208889892998,-0.158333333333268,
6.09760172484103));
#52619=CARTESIAN_POINT('Ctrl Pts',(4.60456520912973,0.15833333333327,6.06639620794663));
#52620=CARTESIAN_POINT('Ctrl Pts',(4.64456604111084,0.319434907277037,6.05173924304811));
#52621=CARTESIAN_POINT('Ctrl Pts',(4.70405251924755,0.636309800094947,6.00739471694425));
#52622=CARTESIAN_POINT('Ctrl Pts',(4.76780941860996,0.794772684000517,5.98315811264259));
#52623=CARTESIAN_POINT('Ctrl Pts',(4.80421088102902,1.06847604194596,5.92110660856591));
#52624=CARTESIAN_POINT('Ctrl Pts',(4.80972472899935,1.18514270861383,5.88966949830968));
#52625=CARTESIAN_POINT('Ctrl Pts',(4.80499558066583,1.30000000000321,5.85365507467733));
#52626=CARTESIAN_POINT('Ctrl Pts',(4.88902711963931,-1.30000000000283,6.09588044237462));
#52627=CARTESIAN_POINT('Ctrl Pts',(4.89362272238644,-1.18514270861364,6.11974191404088));
#52628=CARTESIAN_POINT('Ctrl Pts',(4.88648376275866,-1.06847604194596,6.1356918865946));
#52629=CARTESIAN_POINT('Ctrl Pts',(4.84288215129751,-0.794772684000684,
6.15426236833479));
#52630=CARTESIAN_POINT('Ctrl Pts',(4.77077405342329,-0.636309800095067,
6.14378744785621));
#52631=CARTESIAN_POINT('Ctrl Pts',(4.69656033089538,-0.319434907277095,
6.12570668923954));
#52632=CARTESIAN_POINT('Ctrl Pts',(4.64725062312647,-0.1583333333333,6.10673167683751));
#52633=CARTESIAN_POINT('Ctrl Pts',(4.63971054859242,0.158333333333302,6.07482811089041));
#52634=CARTESIAN_POINT('Ctrl Pts',(4.68126272296262,0.319434907277101,6.06099583291417));
#52635=CARTESIAN_POINT('Ctrl Pts',(4.74056080461783,0.636309800095076,6.01593214642562));
#52636=CARTESIAN_POINT('Ctrl Pts',(4.80507337495969,0.794772684000679,5.99020181338789));
#52637=CARTESIAN_POINT('Ctrl Pts',(4.83652787897588,1.06847604194618,5.92725255822721));
#52638=CARTESIAN_POINT('Ctrl Pts',(4.83868267738028,1.18514270861407,5.89559025311695));
#52639=CARTESIAN_POINT('Ctrl Pts',(4.82937678490462,1.30000000000348,5.85951404295586));
#52640=CARTESIAN_POINT('Ctrl Pts',(4.91321985407802,-1.30000000000309,6.10393818921991));
#52641=CARTESIAN_POINT('Ctrl Pts',(4.92249447745382,-1.18514270861388,6.12979090408451));
#52642=CARTESIAN_POINT('Ctrl Pts',(4.9187793331044,-1.06847604194618,6.14706683418608));
#52643=CARTESIAN_POINT('Ctrl Pts',(4.88018764440598,-0.794772684000851,
6.16716360017606));
#52644=CARTESIAN_POINT('Ctrl Pts',(4.80721762555925,-0.636309800095196,
6.15542465374956));
#52645=CARTESIAN_POINT('Ctrl Pts',(4.73316183802081,-0.319434907277159,
6.13649746895652));
#52646=CARTESIAN_POINT('Ctrl Pts',(4.68232035769752,-0.158333333333332,
6.11658777091958));
#52647=CARTESIAN_POINT('Ctrl Pts',(4.67477123300628,0.158333333333334,6.08402952940802));
#52648=CARTESIAN_POINT('Ctrl Pts',(4.71780718131348,0.319434907277167,6.07001371293154));
#52649=CARTESIAN_POINT('Ctrl Pts',(4.77700822866973,0.636309800095206,6.02540714069458));
#52650=CARTESIAN_POINT('Ctrl Pts',(4.84258681448599,0.794772684000839,6.00223009691712));
#52651=CARTESIAN_POINT('Ctrl Pts',(4.86900238110365,1.0684760419464,5.93741886519659));
#52652=CARTESIAN_POINT('Ctrl Pts',(4.86766876330111,1.18514270861432,5.90399949146263));
#52653=CARTESIAN_POINT('Ctrl Pts',(4.85356720770038,1.30000000000375,5.86521512471389));
#52654=CARTESIAN_POINT('Ctrl Pts',(4.92533609403191,-1.30000000000309,6.10851264972719));
#52655=CARTESIAN_POINT('Ctrl Pts',(4.93693489080362,-1.18514270861388,6.1351757774929));
#52656=CARTESIAN_POINT('Ctrl Pts',(4.93492178515123,-1.06847604194618,6.1530199706002));
#52657=CARTESIAN_POINT('Ctrl Pts',(4.89882489072261,-0.794772684000851,
6.17387012311378));
#52658=CARTESIAN_POINT('Ctrl Pts',(4.82544129359841,-0.636309800095196,
6.16200266174069));
#52659=CARTESIAN_POINT('Ctrl Pts',(4.75146299020767,-0.319434907277159,
6.14255691938095));
#52660=CARTESIAN_POINT('Ctrl Pts',(4.69984189087486,-0.158333333333332,
6.12160410624644));
#52661=CARTESIAN_POINT('Ctrl Pts',(4.69228837762174,0.158333333333334,6.08857601784043));
#52662=CARTESIAN_POINT('Ctrl Pts',(4.73609341170092,0.319434907277167,6.07498424576916));
#52663=CARTESIAN_POINT('Ctrl Pts',(4.79522055198674,0.636309800095206,6.03024314493691));
#52664=CARTESIAN_POINT('Ctrl Pts',(4.86122784986915,0.794772684000841,6.0069681780851));
#52665=CARTESIAN_POINT('Ctrl Pts',(4.88516330785021,1.0684760419464,5.9414791270764));
#52666=CARTESIAN_POINT('Ctrl Pts',(4.88213395050327,1.18514270861431,5.90764937166149));
#52667=CARTESIAN_POINT('Ctrl Pts',(4.86571446294546,1.30000000000375,5.86833764440499));
#52668=CARTESIAN_POINT('',(4.76941883344573,1.2,5.87518152519931));
#52669=CARTESIAN_POINT('Ctrl Pts',(4.76941883344572,1.2,5.87518152519931));
#52670=CARTESIAN_POINT('Ctrl Pts',(4.74961204056679,1.21680461799894,5.86666410782715));
#52671=CARTESIAN_POINT('Ctrl Pts',(4.72990091069275,1.23316973561102,5.85707750905065));
#52672=CARTESIAN_POINT('Ctrl Pts',(4.70474620103762,1.25441876751169,5.84645216075377));
#52673=CARTESIAN_POINT('Ctrl Pts',(4.70038407444622,1.25810278200312,5.84461785213178));
#52674=CARTESIAN_POINT('Ctrl Pts',(4.68036604493196,1.27496667239558,5.83609863719043));
#52675=CARTESIAN_POINT('Ctrl Pts',(4.66554413690735,1.28742980080914,5.82982295251271));
#52676=CARTESIAN_POINT('Ctrl Pts',(4.65067750876737,1.30000000000347,5.82388274140186));
#52677=CARTESIAN_POINT('',(4.80892752422524,0.65383484141801,6.02666455499999));
#52678=CARTESIAN_POINT('Ctrl Pts',(4.80892752424968,0.653834841417331,6.02666455499128));
#52679=CARTESIAN_POINT('Ctrl Pts',(4.80506100115371,0.718122177489598,6.01081756986998));
#52680=CARTESIAN_POINT('Ctrl Pts',(4.80189346001836,0.763538358793002,5.99808354372755));
#52681=CARTESIAN_POINT('Ctrl Pts',(4.78910823433444,0.949783543739865,5.94773239137322));
#52682=CARTESIAN_POINT('Ctrl Pts',(4.78204164843337,1.04839967606025,5.92062434825642));
#52683=CARTESIAN_POINT('Ctrl Pts',(4.76941883344572,1.2,5.87518152519931));
#52684=CARTESIAN_POINT('',(4.84008270153026,-0.653834841531101,6.16264786964716));
#52685=CARTESIAN_POINT('Ctrl Pts',(4.84008270153025,-0.653834841531099,
6.16264786964715));
#52686=CARTESIAN_POINT('Ctrl Pts',(4.79944932185601,-0.575798355642387,
6.15340830475714));
#52687=CARTESIAN_POINT('Ctrl Pts',(4.76554358800515,-0.493918960588331,
6.14499354505786));
#52688=CARTESIAN_POINT('Ctrl Pts',(4.71701549206806,-0.338195044740467,
6.13032179136123));
#52689=CARTESIAN_POINT('Ctrl Pts',(4.70027425207649,-0.265709840048834,
6.12394244996249));
#52690=CARTESIAN_POINT('Ctrl Pts',(4.67933806233096,-0.129740191198744,
6.11139089035258));
#52691=CARTESIAN_POINT('Ctrl Pts',(4.67367217159743,-0.0666411092615673,
6.10534940426575));
#52692=CARTESIAN_POINT('Ctrl Pts',(4.6703311450012,0.059549413910394,6.09243289590055));
#52693=CARTESIAN_POINT('Ctrl Pts',(4.67261431641252,0.122794913999556,6.0854643527866));
#52694=CARTESIAN_POINT('Ctrl Pts',(4.68654341749057,0.260150718519473,6.07009424202348));
#52695=CARTESIAN_POINT('Ctrl Pts',(4.69981969456811,0.333951442794183,6.06166111874082));
#52696=CARTESIAN_POINT('Ctrl Pts',(4.74110964114528,0.491144733190181,6.04420974956465));
#52697=CARTESIAN_POINT('Ctrl Pts',(4.77132339271692,0.574255455836941,6.03514263513348));
#52698=CARTESIAN_POINT('Ctrl Pts',(4.80892752419487,0.653834841429595,6.02666455497405));
#52699=CARTESIAN_POINT('',(4.82444742165433,-1.2,6.09220621246874));
#52700=CARTESIAN_POINT('Ctrl Pts',(4.82444742165433,-1.2,6.09220621246874));
#52701=CARTESIAN_POINT('Ctrl Pts',(4.8272118332668,-1.1348197950149,6.10424523870834));
#52702=CARTESIAN_POINT('Ctrl Pts',(4.83083887049113,-1.03881930443303,6.12025722567746));
#52703=CARTESIAN_POINT('Ctrl Pts',(4.83765685676595,-0.795493170498027,
6.15131114758654));
#52704=CARTESIAN_POINT('Ctrl Pts',(4.83870897311039,-0.741489946887419,
6.15623832079));
#52705=CARTESIAN_POINT('Ctrl Pts',(4.84008270153025,-0.6538348415311,6.16264786964715));
#52706=CARTESIAN_POINT('Ctrl Pts',(4.7098133285389,-1.30000000000282,6.04234788891915));
#52707=CARTESIAN_POINT('Ctrl Pts',(4.72925071810808,-1.28307077053216,6.05050207742009));
#52708=CARTESIAN_POINT('Ctrl Pts',(4.74865938770459,-1.26613268536529,6.05870659013052));
#52709=CARTESIAN_POINT('Ctrl Pts',(4.78083864386518,-1.23799653492038,6.07242372484376));
#52710=CARTESIAN_POINT('Ctrl Pts',(4.8036210251056,-1.21801262437289,6.08199369402584));
#52711=CARTESIAN_POINT('Ctrl Pts',(4.82444742165433,-1.2,6.09220621246874));
#52712=CARTESIAN_POINT('Origin',(0.,1.25,7.2));
#52713=CARTESIAN_POINT('Origin',(0.,1.2,7.2));
#52714=CARTESIAN_POINT('Origin',(0.,0.92691742076555,7.2));
#52715=CARTESIAN_POINT('Origin',(0.,0.653834841531101,7.2));
#52716=CARTESIAN_POINT('Origin',(0.,0.,7.2));
#52717=CARTESIAN_POINT('Origin',(0.,-0.653834841531101,7.2));
#52718=CARTESIAN_POINT('Origin',(0.,-0.926917420765551,7.2));
#52719=CARTESIAN_POINT('Origin',(0.,-1.2,7.2));
#52720=CARTESIAN_POINT('Origin',(0.,-1.25,7.2));
#52721=CARTESIAN_POINT('Ctrl Pts',(4.98668722203916,-1.30000000000008,6.43746972924236));
#52722=CARTESIAN_POINT('Ctrl Pts',(4.98569765033805,-1.18514270861184,6.39487827212538));
#52723=CARTESIAN_POINT('Ctrl Pts',(4.97470530482918,-1.06847604194514,6.36274110209538));
#52724=CARTESIAN_POINT('Ctrl Pts',(4.92620237914858,-0.794772684000851,
6.31264930485112));
#52725=CARTESIAN_POINT('Ctrl Pts',(4.85643493010791,-0.636309800095196,
6.31823415136655));
#52726=CARTESIAN_POINT('Ctrl Pts',(4.7842217545151,-0.319434907277159,6.30141029648602));
#52727=CARTESIAN_POINT('Ctrl Pts',(4.73867559286568,-0.158333333333332,
6.30681070736002));
#52728=CARTESIAN_POINT('Ctrl Pts',(4.73214233678194,0.158333333333334,6.27356575659811));
#52729=CARTESIAN_POINT('Ctrl Pts',(4.77077828071913,0.319434907277167,6.2334282166797));
#52730=CARTESIAN_POINT('Ctrl Pts',(4.83045152777451,0.636309800095206,6.18557396029517));
#52731=CARTESIAN_POINT('Ctrl Pts',(4.89266384818737,0.79477268400084,6.14488469691364));
#52732=CARTESIAN_POINT('Ctrl Pts',(4.93412052316908,1.06847604194527,6.149250329368));
#52733=CARTESIAN_POINT('Ctrl Pts',(4.9432174738979,1.1851427086121,6.16473300709073));
#52734=CARTESIAN_POINT('Ctrl Pts',(4.94346631687715,1.30000000000048,6.19380864200933));
#52735=CARTESIAN_POINT('Ctrl Pts',(4.97686019541382,-1.30000000000008,6.44526302673736));
#52736=CARTESIAN_POINT('Ctrl Pts',(4.97396758436905,-1.18514270861184,6.40409612527667));
#52737=CARTESIAN_POINT('Ctrl Pts',(4.96159302098239,-1.06847604194514,6.37302357697528));
#52738=CARTESIAN_POINT('Ctrl Pts',(4.91110009726839,-0.794772684000851,
6.32455974952348));
#52739=CARTESIAN_POINT('Ctrl Pts',(4.84176412504578,-0.636309800095198,
6.33005968031769));
#52740=CARTESIAN_POINT('Ctrl Pts',(4.76953814967829,-0.319434907277161,
6.31338878414013));
#52741=CARTESIAN_POINT('Ctrl Pts',(4.72452210845459,-0.158333333333333,
6.31808899580793));
#52742=CARTESIAN_POINT('Ctrl Pts',(4.71817594716849,0.158333333333335,6.28527505653109));
#52743=CARTESIAN_POINT('Ctrl Pts',(4.75652394684051,0.319434907277168,6.24640754928909));
#52744=CARTESIAN_POINT('Ctrl Pts',(4.81647889553183,0.636309800095209,6.19899550317458));
#52745=CARTESIAN_POINT('Ctrl Pts',(4.8783656650789,0.794772684000845,6.15859186148608));
#52746=CARTESIAN_POINT('Ctrl Pts',(4.92179501812862,1.06847604194528,6.16125451685743));
#52747=CARTESIAN_POINT('Ctrl Pts',(4.93221572520193,1.1851427086121,6.17552577898485));
#52748=CARTESIAN_POINT('Ctrl Pts',(4.93425818162946,1.30000000000048,6.20291573839054));
#52749=CARTESIAN_POINT('Ctrl Pts',(4.95706874230453,-1.30000000000014,6.46030632993531));
#52750=CARTESIAN_POINT('Ctrl Pts',(4.95079122398016,-1.18514270861189,6.42325134866451));
#52751=CARTESIAN_POINT('Ctrl Pts',(4.93588292679964,-1.06847604194519,6.39501776655385));
#52752=CARTESIAN_POINT('Ctrl Pts',(4.88150295217893,-0.794772684000883,
6.3501717405442));
#52753=CARTESIAN_POINT('Ctrl Pts',(4.81225615197418,-0.636309800095221,
6.35334452626117));
#52754=CARTESIAN_POINT('Ctrl Pts',(4.73980482549258,-0.31943490727717,6.33642842109036));
#52755=CARTESIAN_POINT('Ctrl Pts',(4.696170859758,-0.158333333333338,6.34055762075764));
#52756=CARTESIAN_POINT('Ctrl Pts',(4.69012591704432,0.15833333333334,6.30845198515447));
#52757=CARTESIAN_POINT('Ctrl Pts',(4.72754383863126,0.319434907277177,6.27128669989665));
#52758=CARTESIAN_POINT('Ctrl Pts',(4.78803057335667,0.636309800095228,6.22470119665593));
#52759=CARTESIAN_POINT('Ctrl Pts',(4.84961397558834,0.794772684000868,6.18573688361928));
#52760=CARTESIAN_POINT('Ctrl Pts',(4.89700059988731,1.06847604194532,6.18498545886474));
#52761=CARTESIAN_POINT('Ctrl Pts',(4.91001220404317,1.18514270861215,6.19666573939433));
#52762=CARTESIAN_POINT('Ctrl Pts',(4.91552349854335,1.30000000000054,6.22035156438672));
#52763=CARTESIAN_POINT('Ctrl Pts',(4.93691061846834,-1.30000000000018,6.47575166451482));
#52764=CARTESIAN_POINT('Ctrl Pts',(4.92653611020849,-1.18514270861193,6.44097594222251));
#52765=CARTESIAN_POINT('Ctrl Pts',(4.90867909622876,-1.06847604194522,6.41453646114568));
#52766=CARTESIAN_POINT('Ctrl Pts',(4.85013973656912,-0.79477268400091,6.37271435552521));
#52767=CARTESIAN_POINT('Ctrl Pts',(4.78205759083351,-0.636309800095246,
6.37652947871845));
#52768=CARTESIAN_POINT('Ctrl Pts',(4.70966700916279,-0.319434907277184,
6.36018130843371));
#52769=CARTESIAN_POINT('Ctrl Pts',(4.66714547480156,-0.158333333333345,
6.36293868473051));
#52770=CARTESIAN_POINT('Ctrl Pts',(4.66133147057174,0.158333333333347,6.3313827263226));
#52771=CARTESIAN_POINT('Ctrl Pts',(4.69775031582757,0.319434907277193,6.29585311532871));
#52772=CARTESIAN_POINT('Ctrl Pts',(4.75888621980995,0.636309800095257,6.25040153766716));
#52773=CARTESIAN_POINT('Ctrl Pts',(4.82045415980186,0.794772684000902,6.21364759328796));
#52774=CARTESIAN_POINT('Ctrl Pts',(4.8719170783672,1.06847604194536,6.2095231014812));
#52775=CARTESIAN_POINT('Ctrl Pts',(4.88752980681081,1.18514270861219,6.21845908172245));
#52776=CARTESIAN_POINT('Ctrl Pts',(4.89647887314016,1.30000000000058,6.23811638188062));
#52777=CARTESIAN_POINT('Ctrl Pts',(4.92636805940448,-1.30000000000019,6.48376534470158));
#52778=CARTESIAN_POINT('Ctrl Pts',(4.91412619153649,-1.18514270861194,6.45101218262242));
#52779=CARTESIAN_POINT('Ctrl Pts',(4.89487951363381,-1.06847604194523,6.42598062912506));
#52780=CARTESIAN_POINT('Ctrl Pts',(4.83423332490632,-0.794772684000915,
6.38599119352752));
#52781=CARTESIAN_POINT('Ctrl Pts',(4.76631059477317,-0.636309800095249,
6.38886174607922));
#52782=CARTESIAN_POINT('Ctrl Pts',(4.69374505420487,-0.319434907277185,
6.37223471354738));
#52783=CARTESIAN_POINT('Ctrl Pts',(4.65178182810547,-0.158333333333345,
6.37420333831997));
#52784=CARTESIAN_POINT('Ctrl Pts',(4.64610231107768,0.158333333333348,6.34297281401876));
#52785=CARTESIAN_POINT('Ctrl Pts',(4.68219514209646,0.319434907277194,6.30882664971357));
#52786=CARTESIAN_POINT('Ctrl Pts',(4.74358072026792,0.63630980009526,6.26376835475518));
#52787=CARTESIAN_POINT('Ctrl Pts',(4.80473133823679,0.794772684000906,6.22716635240518));
#52788=CARTESIAN_POINT('Ctrl Pts',(4.85833367902391,1.06847604194536,6.22128074130118));
#52789=CARTESIAN_POINT('Ctrl Pts',(4.87540005304793,1.1851427086122,6.22899812669478));
#52790=CARTESIAN_POINT('Ctrl Pts',(4.88633033393167,1.30000000000059,6.24698056044553));
#52791=CARTESIAN_POINT('Ctrl Pts',(4.92512165412919,-1.30000000000019,6.48468994389186));
#52792=CARTESIAN_POINT('Ctrl Pts',(4.91265773749602,-1.18514270861194,6.45216897026815));
#52793=CARTESIAN_POINT('Ctrl Pts',(4.89324644872196,-1.06847604194523,6.42730053234831));
#52794=CARTESIAN_POINT('Ctrl Pts',(4.83235266897639,-0.794772684000915,
6.38752835419998));
#52795=CARTESIAN_POINT('Ctrl Pts',(4.76445543410879,-0.636309800095249,
6.39030617896606));
#52796=CARTESIAN_POINT('Ctrl Pts',(4.69186920163666,-0.319434907277185,
6.3736466176957));
#52797=CARTESIAN_POINT('Ctrl Pts',(4.64996529198419,-0.158333333333345,
6.37550554229197));
#52798=CARTESIAN_POINT('Ctrl Pts',(4.64430108817236,0.158333333333348,6.34431222881329));
#52799=CARTESIAN_POINT('Ctrl Pts',(4.68035913284604,0.319434907277194,6.31033866685585));
#52800=CARTESIAN_POINT('Ctrl Pts',(4.74177782070676,0.63630980009526,6.26533636497439));
#52801=CARTESIAN_POINT('Ctrl Pts',(4.80288296703754,0.794772684000907,6.22876118771136));
#52802=CARTESIAN_POINT('Ctrl Pts',(4.85673799241266,1.06847604194536,6.22267052237588));
#52803=CARTESIAN_POINT('Ctrl Pts',(4.87397495550491,1.1851427086122,6.23024323981494));
#52804=CARTESIAN_POINT('Ctrl Pts',(4.88513703672986,1.30000000000059,6.2480250980354));
#52805=CARTESIAN_POINT('Ctrl Pts',(4.92293833907504,-1.30000000000019,6.48630256823851));
#52806=CARTESIAN_POINT('Ctrl Pts',(4.91008208674477,-1.18514270861194,6.45417672305587));
#52807=CARTESIAN_POINT('Ctrl Pts',(4.89038039954413,-1.06847604194523,6.42958680601259));
#52808=CARTESIAN_POINT('Ctrl Pts',(4.82905123682654,-0.794772684000915,
6.39018868000574));
#52809=CARTESIAN_POINT('Ctrl Pts',(4.76120097554205,-0.636309800095249,
6.39281196796341));
#52810=CARTESIAN_POINT('Ctrl Pts',(4.68858360111441,-0.319434907277185,
6.37610978023243));
#52811=CARTESIAN_POINT('Ctrl Pts',(4.6467921652549,-0.158333333333345,6.37780010804488));
#52812=CARTESIAN_POINT('Ctrl Pts',(4.64115480296635,0.158333333333348,6.34667240984026));
#52813=CARTESIAN_POINT('Ctrl Pts',(4.67714081045394,0.319434907277194,6.31297145333446));
#52814=CARTESIAN_POINT('Ctrl Pts',(4.73861762231401,0.63630980009526,6.26806722692365));
#52815=CARTESIAN_POINT('Ctrl Pts',(4.7996545888502,0.794772684000906,6.23156801465449));
#52816=CARTESIAN_POINT('Ctrl Pts',(4.8539535036347,1.06847604194536,6.22512301388828));
#52817=CARTESIAN_POINT('Ctrl Pts',(4.87148787148143,1.1851427086122,6.23243986365501));
#52818=CARTESIAN_POINT('Ctrl Pts',(4.88305261893776,1.30000000000059,6.24986336520934));
#52819=CARTESIAN_POINT('Ctrl Pts',(4.91855575959217,-1.30000000000019,6.48948322463651));
#52820=CARTESIAN_POINT('Ctrl Pts',(4.90489971974153,-1.18514270861194,6.45810477885079));
#52821=CARTESIAN_POINT('Ctrl Pts',(4.88460837725371,-1.06847604194523,6.43404695026136));
#52822=CARTESIAN_POINT('Ctrl Pts',(4.82240244035806,-0.794772684000913,
6.39538064367556));
#52823=CARTESIAN_POINT('Ctrl Pts',(4.75466619892734,-0.636309800095248,
6.39775306830035));
#52824=CARTESIAN_POINT('Ctrl Pts',(4.6819970277539,-0.319434907277185,6.38099611983521));
#52825=CARTESIAN_POINT('Ctrl Pts',(4.64043601582692,-0.158333333333345,
6.38236366871908));
#52826=CARTESIAN_POINT('Ctrl Pts',(4.63485083995942,0.158333333333347,6.35136490007434));
#52827=CARTESIAN_POINT('Ctrl Pts',(4.67067489536199,0.319434907277194,6.31816401775939));
#52828=CARTESIAN_POINT('Ctrl Pts',(4.73227663170893,0.636309800095259,6.27347865485972));
#52829=CARTESIAN_POINT('Ctrl Pts',(4.79321242094628,0.794772684000905,6.23722144826176));
#52830=CARTESIAN_POINT('Ctrl Pts',(4.84840411962865,1.06847604194536,6.23007975932987));
#52831=CARTESIAN_POINT('Ctrl Pts',(4.86652887652838,1.1851427086122,6.23687296384654));
#52832=CARTESIAN_POINT('Ctrl Pts',(4.8788879490222,1.30000000000059,6.25355074539284));
#52833=CARTESIAN_POINT('Ctrl Pts',(4.90969678062161,-1.30000000000019,6.49559848148463));
#52834=CARTESIAN_POINT('Ctrl Pts',(4.89429034770527,-1.18514270861194,6.4652752091426));
#52835=CARTESIAN_POINT('Ctrl Pts',(4.87273109405207,-1.06847604194523,6.44202331212106));
#52836=CARTESIAN_POINT('Ctrl Pts',(4.80871065842956,-0.794772684000916,
6.40464307008932));
#52837=CARTESIAN_POINT('Ctrl Pts',(4.74137158253816,-0.636309800095248,
6.40701333983432));
#52838=CARTESIAN_POINT('Ctrl Pts',(4.66876019540481,-0.319434907277185,
6.39060475719409));
#52839=CARTESIAN_POINT('Ctrl Pts',(4.62784934778019,-0.158333333333345,
6.39184122976634));
#52840=CARTESIAN_POINT('Ctrl Pts',(4.62236214305987,0.158333333333347,6.36109576080471));
#52841=CARTESIAN_POINT('Ctrl Pts',(4.65756162412944,0.319434907277194,6.32810519387628));
#52842=CARTESIAN_POINT('Ctrl Pts',(4.71945257185647,0.636309800095259,6.28394196729414));
#52843=CARTESIAN_POINT('Ctrl Pts',(4.78056554749451,0.794772684000907,6.2491212948399));
#52844=CARTESIAN_POINT('Ctrl Pts',(4.83759362894242,1.06847604194536,6.24071710639619));
#52845=CARTESIAN_POINT('Ctrl Pts',(4.85685476193013,1.18514270861219,6.24635519381419));
#52846=CARTESIAN_POINT('Ctrl Pts',(4.87069168454543,1.30000000000058,6.26126923042159));
#52847=CARTESIAN_POINT('Ctrl Pts',(4.89713958049952,-1.30000000000017,6.50462396405601));
#52848=CARTESIAN_POINT('Ctrl Pts',(4.87937217586078,-1.18514270861192,6.47622076642019));
#52849=CARTESIAN_POINT('Ctrl Pts',(4.8560702776099,-1.06847604194522,6.45432379139764));
#52850=CARTESIAN_POINT('Ctrl Pts',(4.78945244370591,-0.794772684000906,
6.41876807442275));
#52851=CARTESIAN_POINT('Ctrl Pts',(4.7224340152446,-0.63630980009524,6.42040187127375));
#52852=CARTESIAN_POINT('Ctrl Pts',(4.6496605599142,-0.31943490727718,6.40378804953575));
#52853=CARTESIAN_POINT('Ctrl Pts',(4.60942850882551,-0.158333333333343,
6.40413794851151));
#52854=CARTESIAN_POINT('Ctrl Pts',(4.60410214916729,0.158333333333345,6.37381907547874));
#52855=CARTESIAN_POINT('Ctrl Pts',(4.63883571633811,0.31943490727719,6.34230925296491));
#52856=CARTESIAN_POINT('Ctrl Pts',(4.70111036527886,0.63630980009525,6.29887887268815));
#52857=CARTESIAN_POINT('Ctrl Pts',(4.76195747457999,0.794772684000895,6.26481378454199));
#52858=CARTESIAN_POINT('Ctrl Pts',(4.82158826959047,1.06847604194535,6.25454543594719));
#52859=CARTESIAN_POINT('Ctrl Pts',(4.84256297288892,1.18514270861218,6.25874685006882));
#52860=CARTESIAN_POINT('Ctrl Pts',(4.8587004178645,1.30000000000057,6.27159446593894));
#52861=CARTESIAN_POINT('Ctrl Pts',(4.88212929215244,-1.30000000000016,6.51567079219986));
#52862=CARTESIAN_POINT('Ctrl Pts',(4.86159707438084,-1.18514270861191,6.48979833670658));
#52863=CARTESIAN_POINT('Ctrl Pts',(4.83624723042465,-1.06847604194521,6.46967229640823));
#52864=CARTESIAN_POINT('Ctrl Pts',(4.76655433941777,-0.794772684000905,
6.43645248578523));
#52865=CARTESIAN_POINT('Ctrl Pts',(4.69987163509091,-0.636309800095237,
6.43704889500626));
#52866=CARTESIAN_POINT('Ctrl Pts',(4.62683906545535,-0.319434907277178,
6.41999118933009));
#52867=CARTESIAN_POINT('Ctrl Pts',(4.58735092903532,-0.158333333333342,
6.41905017668548));
#52868=CARTESIAN_POINT('Ctrl Pts',(4.58215666749824,0.158333333333344,6.38906625062512));
#52869=CARTESIAN_POINT('Ctrl Pts',(4.61629639064893,0.319434907277187,6.35926187789649));
#52870=CARTESIAN_POINT('Ctrl Pts',(4.67906261951202,0.636309800095246,6.31679552289548));
#52871=CARTESIAN_POINT('Ctrl Pts',(4.73968915183838,0.79477268400089,6.28389249252736));
#52872=CARTESIAN_POINT('Ctrl Pts',(4.80250707499649,1.06847604194534,6.27154949174964));
#52873=CARTESIAN_POINT('Ctrl Pts',(4.82555758093061,1.18514270861218,6.27407497603294));
#52874=CARTESIAN_POINT('Ctrl Pts',(4.84446704149716,1.30000000000056,6.28446877228295));
#52875=CARTESIAN_POINT('Ctrl Pts',(4.86182565717412,-1.30000000000016,6.52956179564368));
#52876=CARTESIAN_POINT('Ctrl Pts',(4.83734621833198,-1.18514270861191,6.50630411448896));
#52877=CARTESIAN_POINT('Ctrl Pts',(4.80909398668839,-1.06847604194521,6.48803936152431));
#52878=CARTESIAN_POINT('Ctrl Pts',(4.73510977363616,-0.794772684000899,
6.45737879127558));
#52879=CARTESIAN_POINT('Ctrl Pts',(4.66899789504025,-0.636309800095234,
6.45694585784103));
#52880=CARTESIAN_POINT('Ctrl Pts',(4.59585217179943,-0.319434907277178,
6.43999002672486));
#52881=CARTESIAN_POINT('Ctrl Pts',(4.55769689007927,-0.158333333333342,
6.43834269264524));
#52882=CARTESIAN_POINT('Ctrl Pts',(4.55286565414339,0.158333333333344,6.40937925847717));
#52883=CARTESIAN_POINT('Ctrl Pts',(4.5862140872802,0.319434907277186,6.38184240151));
#52884=CARTESIAN_POINT('Ctrl Pts',(4.64946925549905,0.636309800095244,6.34025146852919));
#52885=CARTESIAN_POINT('Ctrl Pts',(4.70941285168286,0.794772684000888,6.30792389975058));
#52886=CARTESIAN_POINT('Ctrl Pts',(4.77637892632758,1.06847604194534,6.29250110299389));
#52887=CARTESIAN_POINT('Ctrl Pts',(4.80222293614429,1.18514270861217,6.29281684556559));
#52888=CARTESIAN_POINT('Ctrl Pts',(4.82492382340163,1.30000000000056,6.30012428795403));
#52889=CARTESIAN_POINT('Ctrl Pts',(4.84154147293362,-1.30000000000014,6.54358302839007));
#52890=CARTESIAN_POINT('Ctrl Pts',(4.81313480855745,-1.1851427086119,6.52301053449656));
#52891=CARTESIAN_POINT('Ctrl Pts',(4.78201025093487,-1.0684760419452,6.50670714550205));
#52892=CARTESIAN_POINT('Ctrl Pts',(4.70382741926839,-0.79477268400089,6.47890554179115));
#52893=CARTESIAN_POINT('Ctrl Pts',(4.63845673257079,-0.636309800095226,
6.47797802085801));
#52894=CARTESIAN_POINT('Ctrl Pts',(4.5651715809394,-0.319434907277173,6.4610415223539));
#52895=CARTESIAN_POINT('Ctrl Pts',(4.52823440680283,-0.158333333333339,
6.4582792046978));
#52896=CARTESIAN_POINT('Ctrl Pts',(4.523479643894,0.158333333333342,6.42952429902268));
#52897=CARTESIAN_POINT('Ctrl Pts',(4.55560208671196,0.319434907277181,6.40310820853837));
#52898=CARTESIAN_POINT('Ctrl Pts',(4.61932427998526,0.636309800095235,6.36233567863279));
#52899=CARTESIAN_POINT('Ctrl Pts',(4.67901776100319,0.794772684000877,6.33174657323979));
#52900=CARTESIAN_POINT('Ctrl Pts',(4.75038445471543,1.06847604194532,6.31392860517125));
#52901=CARTESIAN_POINT('Ctrl Pts',(4.77910498021926,1.18514270861216,6.31226155035503));
#52902=CARTESIAN_POINT('Ctrl Pts',(4.80565403391551,1.30000000000054,6.3166401788787));
#52903=CARTESIAN_POINT('Ctrl Pts',(4.82116243215177,-1.30000000000014,6.55733558918724));
#52904=CARTESIAN_POINT('Ctrl Pts',(4.78883341287566,-1.18514270861189,6.53951145811885));
#52905=CARTESIAN_POINT('Ctrl Pts',(4.75478741066505,-1.06847604194519,6.52504768752977));
#52906=CARTESIAN_POINT('Ctrl Pts',(4.67216776061922,-0.794772684000887,
6.49939658894659));
#52907=CARTESIAN_POINT('Ctrl Pts',(4.60704322956664,-0.636309800095225,
6.49637469731541));
#52908=CARTESIAN_POINT('Ctrl Pts',(4.53351417304343,-0.319434907277172,
6.47915083859645));
#52909=CARTESIAN_POINT('Ctrl Pts',(4.49807225560928,-0.158333333333339,
6.47619891866663));
#52910=CARTESIAN_POINT('Ctrl Pts',(4.49360873628281,0.158333333333341,6.44834180152489));
#52911=CARTESIAN_POINT('Ctrl Pts',(4.52460924588721,0.319434907277181,6.42334992397671));
#52912=CARTESIAN_POINT('Ctrl Pts',(4.58900139539972,0.636309800095234,6.38400740246072));
#52913=CARTESIAN_POINT('Ctrl Pts',(4.64866261035791,0.794772684000875,6.35580900848947));
#52914=CARTESIAN_POINT('Ctrl Pts',(4.72438699513373,1.06847604194532,6.33545359086945));
#52915=CARTESIAN_POINT('Ctrl Pts',(4.7558936377855,1.18514270861215,6.33152370410616));
#52916=CARTESIAN_POINT('Ctrl Pts',(4.78612864278456,1.30000000000054,6.33247503662476));
#52917=CARTESIAN_POINT('Ctrl Pts',(4.80064499571522,-1.30000000000014,6.57074186966073));
#52918=CARTESIAN_POINT('Ctrl Pts',(4.76413166792447,-1.18514270861189,6.55480952312448));
#52919=CARTESIAN_POINT('Ctrl Pts',(4.72705540277594,-1.06847604194519,6.54182573186236));
#52920=CARTESIAN_POINT('Ctrl Pts',(4.64010131528972,-0.794772684000882,
6.51864232918802));
#52921=CARTESIAN_POINT('Ctrl Pts',(4.57609739480573,-0.63630980009522,6.51635936434249));
#52922=CARTESIAN_POINT('Ctrl Pts',(4.50238395474208,-0.31943490727717,6.49901640971187));
#52923=CARTESIAN_POINT('Ctrl Pts',(4.4677782557077,-0.158333333333338,6.49368883985741));
#52924=CARTESIAN_POINT('Ctrl Pts',(4.46341909854567,0.15833333333334,6.4661459081692));
#52925=CARTESIAN_POINT('Ctrl Pts',(4.4936600016079,0.319434907277179,6.44376797469062));
#52926=CARTESIAN_POINT('Ctrl Pts',(4.55850563825248,0.63630980009523,6.40533910736424));
#52927=CARTESIAN_POINT('Ctrl Pts',(4.61736729464155,0.794772684000869,6.37742243298241));
#52928=CARTESIAN_POINT('Ctrl Pts',(4.69750095462133,1.06847604194531,6.35465771123057));
#52929=CARTESIAN_POINT('Ctrl Pts',(4.73199779532328,1.18514270861215,6.34900925101938));
#52930=CARTESIAN_POINT('Ctrl Pts',(4.76630458456664,1.30000000000053,6.34756633512731));
#52931=CARTESIAN_POINT('Ctrl Pts',(4.77472662307008,-1.30000000000012,6.58645074781878));
#52932=CARTESIAN_POINT('Ctrl Pts',(4.73330827518786,-1.18514270861187,6.5740302963003));
#52933=CARTESIAN_POINT('Ctrl Pts',(4.69256680491827,-1.06847604194517,6.56335519378605));
#52934=CARTESIAN_POINT('Ctrl Pts',(4.60000958098637,-0.794772684000873,
6.54272567678683));
#52935=CARTESIAN_POINT('Ctrl Pts',(4.53619379013752,-0.636309800095217,
6.53733495387666));
#52936=CARTESIAN_POINT('Ctrl Pts',(4.46216853663192,-0.31943490727717,6.5196152407362));
#52937=CARTESIAN_POINT('Ctrl Pts',(4.42953403920399,-0.158333333333337,
6.5144177485044));
#52938=CARTESIAN_POINT('Ctrl Pts',(4.42559058451556,0.15833333333334,6.4882478384849));
#52939=CARTESIAN_POINT('Ctrl Pts',(4.45441449289897,0.319434907277177,6.4676825932433));
#52940=CARTESIAN_POINT('Ctrl Pts',(4.52013657539244,0.636309800095227,6.4312667028111));
#52941=CARTESIAN_POINT('Ctrl Pts',(4.5789001329555,0.794772684000868,6.4062686380822));
#52942=CARTESIAN_POINT('Ctrl Pts',(4.66470405570312,1.06847604194531,6.380980410857));
#52943=CARTESIAN_POINT('Ctrl Pts',(4.70283664676022,1.18514270861214,6.3729180923415));
#52944=CARTESIAN_POINT('Ctrl Pts',(4.74196049006563,1.30000000000052,6.36773979185513));
#52945=CARTESIAN_POINT('Ctrl Pts',(4.75153496462463,-1.30000000000011,6.60128956561562));
#52946=CARTESIAN_POINT('Ctrl Pts',(4.70542491577634,-1.18514270861187,6.59109134143449));
#52947=CARTESIAN_POINT('Ctrl Pts',(4.66124595282902,-1.06847604194517,6.58201508893444));
#52948=CARTESIAN_POINT('Ctrl Pts',(4.56364490519314,-0.794772684000872,
6.56363910899422));
#52949=CARTESIAN_POINT('Ctrl Pts',(4.50077518794686,-0.636309800095211,
6.55803052449013));
#52950=CARTESIAN_POINT('Ctrl Pts',(4.42634106799007,-0.319434907277165,
6.53945370326785));
#52951=CARTESIAN_POINT('Ctrl Pts',(4.39468669995836,-0.158333333333335,
6.53155092825692));
#52952=CARTESIAN_POINT('Ctrl Pts',(4.39076683331099,0.158333333333338,6.50551318054222));
#52953=CARTESIAN_POINT('Ctrl Pts',(4.41852656654882,0.319434907277173,6.48750688101309));
#52954=CARTESIAN_POINT('Ctrl Pts',(4.48492480491589,0.636309800095219,6.45278458692865));
#52955=CARTESIAN_POINT('Ctrl Pts',(4.54334400499924,0.794772684000856,6.42982150976879));
#52956=CARTESIAN_POINT('Ctrl Pts',(4.63422280032256,1.0684760419453,6.40216138117284));
#52957=CARTESIAN_POINT('Ctrl Pts',(4.67566990004589,1.18514270861213,6.39198737148927));
#52958=CARTESIAN_POINT('Ctrl Pts',(4.71922603638829,1.30000000000051,6.38361239688253));
#52959=CARTESIAN_POINT('Ctrl Pts',(4.73570235451822,-1.30000000000011,6.60979664855893));
#52960=CARTESIAN_POINT('Ctrl Pts',(4.68648240632083,-1.18514270861186,6.60116566063527));
#52961=CARTESIAN_POINT('Ctrl Pts',(4.64000788798049,-1.06847604194516,6.59316231854331));
#52962=CARTESIAN_POINT('Ctrl Pts',(4.53898494560996,-0.794772684000866,
6.57612298467915));
#52963=CARTESIAN_POINT('Ctrl Pts',(4.47648015595929,-0.636309800095209,
6.56945074464614));
#52964=CARTESIAN_POINT('Ctrl Pts',(4.40194285334807,-0.319434907277165,
6.55094083724988));
#52965=CARTESIAN_POINT('Ctrl Pts',(4.3714743653883,-0.158333333333335,6.54314363023759));
#52966=CARTESIAN_POINT('Ctrl Pts',(4.36771574607594,0.158333333333337,6.51772130069368));
#52967=CARTESIAN_POINT('Ctrl Pts',(4.39449091929033,0.319434907277172,6.5004228962701));
#52968=CARTESIAN_POINT('Ctrl Pts',(4.46123916429103,0.636309800095217,6.46648384759227));
#52969=CARTESIAN_POINT('Ctrl Pts',(4.51931896438363,0.794772684000856,6.44459016033573));
#52970=CARTESIAN_POINT('Ctrl Pts',(4.61378982530285,1.06847604194529,6.41598308369089));
#52971=CARTESIAN_POINT('Ctrl Pts',(4.65761426622038,1.18514270861212,6.40490552984303));
#52972=CARTESIAN_POINT('Ctrl Pts',(4.70437021285387,1.30000000000051,6.3951333656302));
#52973=CARTESIAN_POINT('Ctrl Pts',(4.7252393646867,-1.3000000000001,6.61586137002474));
#52974=CARTESIAN_POINT('Ctrl Pts',(4.67382252237325,-1.18514270861186,6.60782874010441));
#52975=CARTESIAN_POINT('Ctrl Pts',(4.62574478186383,-1.06847604194516,6.60027689400989));
#52976=CARTESIAN_POINT('Ctrl Pts',(4.52238957652034,-0.794772684000865,
6.58394132560799));
#52977=CARTESIAN_POINT('Ctrl Pts',(4.46034180597355,-0.636309800095209,
6.57733202806776));
#52978=CARTESIAN_POINT('Ctrl Pts',(4.38571589031662,-0.319434907277165,
6.55878086823184));
#52979=CARTESIAN_POINT('Ctrl Pts',(4.35586566462306,-0.158333333333335,
6.55040045163682));
#52980=CARTESIAN_POINT('Ctrl Pts',(4.35213895544039,0.158333333333337,6.52512591111799));
#52981=CARTESIAN_POINT('Ctrl Pts',(4.37827665702741,0.319434907277172,6.50841589181447));
#52982=CARTESIAN_POINT('Ctrl Pts',(4.44528264043256,0.636309800095217,6.4751096245853));
#52983=CARTESIAN_POINT('Ctrl Pts',(4.50321590295328,0.794772684000856,6.45419665430419));
#52984=CARTESIAN_POINT('Ctrl Pts',(4.60006593612573,1.0684760419453,6.42491863672633));
#52985=CARTESIAN_POINT('Ctrl Pts',(4.64544722920282,1.18514270861213,6.41314989514694));
#52986=CARTESIAN_POINT('Ctrl Pts',(4.69428702464404,1.30000000000051,6.40228578094015));
#52987=CARTESIAN_POINT('Ctrl Pts',(4.71234108790911,-1.30000000000011,6.62410664981093));
#52988=CARTESIAN_POINT('Ctrl Pts',(4.65836817745684,-1.18514270861186,6.61751085829036));
#52989=CARTESIAN_POINT('Ctrl Pts',(4.60837884174036,-1.06847604194516,6.61085327576169));
#52990=CARTESIAN_POINT('Ctrl Pts',(4.50209633045397,-0.794772684000865,
6.59533017868569));
#52991=CARTESIAN_POINT('Ctrl Pts',(4.4401961854101,-0.636309800095209,6.58721850187003));
#52992=CARTESIAN_POINT('Ctrl Pts',(4.3652774986666,-0.319434907277166,6.56794003407505));
#52993=CARTESIAN_POINT('Ctrl Pts',(4.33619889704844,-0.158333333333335,
6.5588500831238));
#52994=CARTESIAN_POINT('Ctrl Pts',(4.33261304783716,0.158333333333337,6.53412644399904));
#52995=CARTESIAN_POINT('Ctrl Pts',(4.35814120400026,0.319434907277172,6.51885093956372));
#52996=CARTESIAN_POINT('Ctrl Pts',(4.42568365918782,0.636309800095217,6.48703954013807));
#52997=CARTESIAN_POINT('Ctrl Pts',(4.48368809821893,0.794772684000856,6.46807029115539));
#52998=CARTESIAN_POINT('Ctrl Pts',(4.58339644619586,1.0684760419453,6.43758944376375));
#52999=CARTESIAN_POINT('Ctrl Pts',(4.63057769859682,1.18514270861212,6.42450991647051));
#53000=CARTESIAN_POINT('Ctrl Pts',(4.68178015411791,1.30000000000051,6.41154489129317));
#53001=CARTESIAN_POINT('Ctrl Pts',(4.69635329463591,-1.3000000000001,6.63210460558044));
#53002=CARTESIAN_POINT('Ctrl Pts',(4.63915551108548,-1.18514270861185,6.62668263242346));
#53003=CARTESIAN_POINT('Ctrl Pts',(4.58679981984083,-1.06847604194516,6.620852896027));
#53004=CARTESIAN_POINT('Ctrl Pts',(4.47703390122908,-0.794772684000863,
6.6064430240604));
#53005=CARTESIAN_POINT('Ctrl Pts',(4.41565432462298,-0.636309800095207,
6.59776964441761));
#53006=CARTESIAN_POINT('Ctrl Pts',(4.340636532308,-0.319434907277165,6.57857504094738));
#53007=CARTESIAN_POINT('Ctrl Pts',(4.31265878703245,-0.158333333333335,
6.56931862491168));
#53008=CARTESIAN_POINT('Ctrl Pts',(4.30919534601676,0.158333333333337,6.5451218747419));
#53009=CARTESIAN_POINT('Ctrl Pts',(4.33378623887568,0.319434907277173,6.53073886803835));
#53010=CARTESIAN_POINT('Ctrl Pts',(4.40159324575602,0.636309800095218,6.49951119778951));
#53011=CARTESIAN_POINT('Ctrl Pts',(4.45906063875119,0.794772684000854,6.48106534498985));
#53012=CARTESIAN_POINT('Ctrl Pts',(4.56234421467301,1.06847604194529,6.44960463262572));
#53013=CARTESIAN_POINT('Ctrl Pts',(4.6119386373717,1.18514270861212,6.43572580559705));
#53014=CARTESIAN_POINT('Ctrl Pts',(4.66641984978617,1.3000000000005,6.42158632818787));
#53015=CARTESIAN_POINT('Ctrl Pts',(4.672740123946,-1.3000000000001,6.64549193416045));
#53016=CARTESIAN_POINT('Ctrl Pts',(4.61083841229515,-1.18514270861186,6.64225703122094));
#53017=CARTESIAN_POINT('Ctrl Pts',(4.55498406308354,-1.06847604194516,6.63779961664745));
#53018=CARTESIAN_POINT('Ctrl Pts',(4.43991995978582,-0.794772684000864,
6.62467785084282));
#53019=CARTESIAN_POINT('Ctrl Pts',(4.37902881615403,-0.636309800095206,
6.6140804027378));
#53020=CARTESIAN_POINT('Ctrl Pts',(4.30343931027374,-0.319434907277164,
6.59329323836205));
#53021=CARTESIAN_POINT('Ctrl Pts',(4.27661637159808,-0.158333333333334,
6.58169995518562));
#53022=CARTESIAN_POINT('Ctrl Pts',(4.27331855534109,0.158333333333336,6.558253636353));
#53023=CARTESIAN_POINT('Ctrl Pts',(4.29694261300081,0.31943490727717,6.54718967402276));
#53024=CARTESIAN_POINT('Ctrl Pts',(4.36561318065384,0.636309800095214,6.51861108957765));
#53025=CARTESIAN_POINT('Ctrl Pts',(4.42276020605754,0.794772684000853,6.50239596111591));
#53026=CARTESIAN_POINT('Ctrl Pts',(4.53144245410637,1.06847604194529,6.46968503431283));
#53027=CARTESIAN_POINT('Ctrl Pts',(4.58453968076316,1.18514270861212,6.45429464940842));
#53028=CARTESIAN_POINT('Ctrl Pts',(4.64368961597056,1.3000000000005,6.43767322775339));
#53029=CARTESIAN_POINT('Ctrl Pts',(4.64616298310555,-1.30000000000009,6.65922290148753));
#53030=CARTESIAN_POINT('Ctrl Pts',(4.57884821129795,-1.18514270861185,6.65787295346516));
#53031=CARTESIAN_POINT('Ctrl Pts',(4.51897037773764,-1.06847604194515,6.65451742945261));
#53032=CARTESIAN_POINT('Ctrl Pts',(4.39782141879937,-0.794772684000858,
6.64213221596193));
#53033=CARTESIAN_POINT('Ctrl Pts',(4.33736029833944,-0.636309800095203,
6.62862782895121));
#53034=CARTESIAN_POINT('Ctrl Pts',(4.26142549421988,-0.319434907277163,
6.60727042170557));
#53035=CARTESIAN_POINT('Ctrl Pts',(4.23663037107786,-0.158333333333334,
6.59630683043));
#53036=CARTESIAN_POINT('Ctrl Pts',(4.23356409439211,0.158333333333336,6.57403153571279));
#53037=CARTESIAN_POINT('Ctrl Pts',(4.25543929850625,0.319434907277169,6.56394883342396));
#53038=CARTESIAN_POINT('Ctrl Pts',(4.32483019778521,0.636309800095212,6.53742968234783));
#53039=CARTESIAN_POINT('Ctrl Pts',(4.38179799022299,0.794772684000848,6.52455367094891));
#53040=CARTESIAN_POINT('Ctrl Pts',(4.49652643255578,1.06847604194529,6.49051542299507));
#53041=CARTESIAN_POINT('Ctrl Pts',(4.55353612285477,1.18514270861211,6.4734061804994));
#53042=CARTESIAN_POINT('Ctrl Pts',(4.61789381187462,1.3000000000005,6.4539215918059));
#53043=CARTESIAN_POINT('Ctrl Pts',(4.61959384082983,-1.30000000000009,6.67287273622477));
#53044=CARTESIAN_POINT('Ctrl Pts',(4.54688106239739,-1.18514270861185,6.67316414663884));
#53045=CARTESIAN_POINT('Ctrl Pts',(4.48298529463437,-1.06847604194515,6.67068658498385));
#53046=CARTESIAN_POINT('Ctrl Pts',(4.35574234728053,-0.794772684000856,
6.65856604251577));
#53047=CARTESIAN_POINT('Ctrl Pts',(4.29577879950244,-0.636309800095202,
6.64235039988357));
#53048=CARTESIAN_POINT('Ctrl Pts',(4.21924951501912,-0.319434907277163,
6.61918589916601));
#53049=CARTESIAN_POINT('Ctrl Pts',(4.19599251313008,-0.158333333333334,
6.60669429060777));
#53050=CARTESIAN_POINT('Ctrl Pts',(4.19305991900079,0.158333333333336,6.58526803818489));
#53051=CARTESIAN_POINT('Ctrl Pts',(4.21356435840231,0.319434907277169,6.57792549211187));
#53052=CARTESIAN_POINT('Ctrl Pts',(4.28375344830649,0.636309800095211,6.55420327081868));
#53053=CARTESIAN_POINT('Ctrl Pts',(4.34026573204614,0.79477268400085,6.54394750424994));
#53054=CARTESIAN_POINT('Ctrl Pts',(4.4611881714325,1.06847604194528,6.50951686686024));
#53055=CARTESIAN_POINT('Ctrl Pts',(4.52225280844087,1.18514270861211,6.49136607426142));
#53056=CARTESIAN_POINT('Ctrl Pts',(4.59203923906518,1.30000000000049,6.46996823620894));
#53057=CARTESIAN_POINT('Ctrl Pts',(4.60066248946871,-1.30000000000009,6.68136532610089));
#53058=CARTESIAN_POINT('Ctrl Pts',(4.52402803840086,-1.18514270861185,6.6828157790179));
#53059=CARTESIAN_POINT('Ctrl Pts',(4.45719926929767,-1.06847604194515,6.6808807938454));
#53060=CARTESIAN_POINT('Ctrl Pts',(4.32546453057817,-0.794772684000855,
6.66858955176316));
#53061=CARTESIAN_POINT('Ctrl Pts',(4.26556250120118,-0.636309800095201,
6.64892274713424));
#53062=CARTESIAN_POINT('Ctrl Pts',(4.18890570850718,-0.319434907277161,
6.62592093780954));
#53063=CARTESIAN_POINT('Ctrl Pts',(4.16761019334189,-0.158333333333333,
6.61643242376773));
#53064=CARTESIAN_POINT('Ctrl Pts',(4.16488682183599,0.158333333333335,6.59622710193004));
#53065=CARTESIAN_POINT('Ctrl Pts',(4.18371953328468,0.319434907277168,6.58773074716968));
#53066=CARTESIAN_POINT('Ctrl Pts',(4.25429825648514,0.636309800095209,6.56505286778703));
#53067=CARTESIAN_POINT('Ctrl Pts',(4.31073095914166,0.794772684000847,6.55762692818754));
#53068=CARTESIAN_POINT('Ctrl Pts',(4.43618954910262,1.06847604194528,6.52305558630728));
#53069=CARTESIAN_POINT('Ctrl Pts',(4.50019375550391,1.18514270861211,6.50416016967104));
#53070=CARTESIAN_POINT('Ctrl Pts',(4.5738957934113,1.30000000000049,6.48133398930408));
#53071=CARTESIAN_POINT('Ctrl Pts',(4.58731275561848,-1.30000000000009,6.68772391623227));
#53072=CARTESIAN_POINT('Ctrl Pts',(4.50789187753129,-1.18514270861184,6.68910077756878));
#53073=CARTESIAN_POINT('Ctrl Pts',(4.43907033323774,-1.06847604194515,6.68729338620038));
#53074=CARTESIAN_POINT('Ctrl Pts',(4.3045653796696,-0.794772684000855,6.67576168981605));
#53075=CARTESIAN_POINT('Ctrl Pts',(4.2455327159996,-0.636309800095199,6.6575524797122));
#53076=CARTESIAN_POINT('Ctrl Pts',(4.16902454304607,-0.319434907277159,
6.63541503524111));
#53077=CARTESIAN_POINT('Ctrl Pts',(4.14873681505423,-0.158333333333333,
6.62612005228647));
#53078=CARTESIAN_POINT('Ctrl Pts',(4.14587644666081,0.158333333333335,6.60534948552149));
#53079=CARTESIAN_POINT('Ctrl Pts',(4.16337892247362,0.319434907277168,6.59525003245809));
#53080=CARTESIAN_POINT('Ctrl Pts',(4.23390772464296,0.636309800095208,6.57227624871251));
#53081=CARTESIAN_POINT('Ctrl Pts',(4.2901072464585,0.794772684000843,6.56648684843127));
#53082=CARTESIAN_POINT('Ctrl Pts',(4.41844626576087,1.06847604194528,6.53152294131612));
#53083=CARTESIAN_POINT('Ctrl Pts',(4.48438193971655,1.1851427086121,6.51208260176214));
#53084=CARTESIAN_POINT('Ctrl Pts',(4.56070008160123,1.30000000000048,6.4883365025039));
#53085=CARTESIAN_POINT('Ctrl Pts',(4.5709651981178,-1.30000000000009,6.69448853267874));
#53086=CARTESIAN_POINT('Ctrl Pts',(4.48783488180397,-1.18514270861184,6.69584068605108));
#53087=CARTESIAN_POINT('Ctrl Pts',(4.41637026894378,-1.06847604194515,6.6944294937794));
#53088=CARTESIAN_POINT('Ctrl Pts',(4.27822282548381,-0.794772684000853,
6.68478547608066));
#53089=CARTESIAN_POINT('Ctrl Pts',(4.22041348676743,-0.636309800095197,
6.66979426696317));
#53090=CARTESIAN_POINT('Ctrl Pts',(4.14417396510687,-0.319434907277159,
6.64979950085998));
#53091=CARTESIAN_POINT('Ctrl Pts',(4.12518931827153,-0.158333333333332,
6.64060101194686));
#53092=CARTESIAN_POINT('Ctrl Pts',(4.12232618138738,0.158333333333335,6.61992583140733));
#53093=CARTESIAN_POINT('Ctrl Pts',(4.13843207228677,0.319434907277167,6.60948413798752));
#53094=CARTESIAN_POINT('Ctrl Pts',(4.20887140515095,0.636309800095207,6.58525683316955));
#53095=CARTESIAN_POINT('Ctrl Pts',(4.26426538681998,0.794772684000841,6.57813941511196));
#53096=CARTESIAN_POINT('Ctrl Pts',(4.39634797677891,1.06847604194528,6.54149178548603));
#53097=CARTESIAN_POINT('Ctrl Pts',(4.46489389934355,1.1851427086121,6.52133356456642));
#53098=CARTESIAN_POINT('Ctrl Pts',(4.54481208542189,1.30000000000048,6.49688052366376));
#53099=CARTESIAN_POINT('Ctrl Pts',(4.55986191625149,-1.30000000000008,6.69922697939143));
#53100=CARTESIAN_POINT('Ctrl Pts',(4.4739076611286,-1.18514270861184,6.69922519060322));
#53101=CARTESIAN_POINT('Ctrl Pts',(4.40061540553236,-1.06847604194514,6.69755530380812));
#53102=CARTESIAN_POINT('Ctrl Pts',(4.26054738497045,-0.794772684000851,
6.68984389115396));
#53103=CARTESIAN_POINT('Ctrl Pts',(4.20510952843759,-0.636309800095196,
6.6810122975644));
#53104=CARTESIAN_POINT('Ctrl Pts',(4.13001103025471,-0.319434907277159,
6.66430370364935));
#53105=CARTESIAN_POINT('Ctrl Pts',(4.11199983529727,-0.158333333333332,
6.65462349396618));
#53106=CARTESIAN_POINT('Ctrl Pts',(4.1092062507607,0.158333333333334,6.63409216511655));
#53107=CARTESIAN_POINT('Ctrl Pts',(4.12443963758816,0.319434907277167,6.62411656351297));
#53108=CARTESIAN_POINT('Ctrl Pts',(4.19381566981051,0.636309800095206,6.59722095262982));
#53109=CARTESIAN_POINT('Ctrl Pts',(4.24681642623153,0.79477268400084,6.58511749178966));
#53110=CARTESIAN_POINT('Ctrl Pts',(4.38081889489758,1.06847604194527,6.54648422762646));
#53111=CARTESIAN_POINT('Ctrl Pts',(4.45118854322608,1.1851427086121,6.52626110695219));
#53112=CARTESIAN_POINT('Ctrl Pts',(4.53392313647836,1.30000000000048,6.50253777415639));
#53113=CARTESIAN_POINT('Ctrl Pts',(4.55333646119707,-1.30000000000008,6.70483180220308));
#53114=CARTESIAN_POINT('Ctrl Pts',(4.46759044005478,-1.18514270861184,6.70468931916621));
#53115=CARTESIAN_POINT('Ctrl Pts',(4.39457954353637,-1.06847604194514,6.70321883895621));
#53116=CARTESIAN_POINT('Ctrl Pts',(4.25533045233314,-0.794772684000851,
6.69675379636771));
#53117=CARTESIAN_POINT('Ctrl Pts',(4.20084799529369,-0.636309800095196,
6.6903034367033));
#53118=CARTESIAN_POINT('Ctrl Pts',(4.1264371815048,-0.319434907277159,6.675134858055));
#53119=CARTESIAN_POINT('Ctrl Pts',(4.1083738762426,-0.158333333333332,6.66544968261944));
#53120=CARTESIAN_POINT('Ctrl Pts',(4.10569625638312,0.158333333333334,6.6451248466368));
#53121=CARTESIAN_POINT('Ctrl Pts',(4.12120905306814,0.319434907277167,6.63561768729212));
#53122=CARTESIAN_POINT('Ctrl Pts',(4.18990683146856,0.636309800095206,6.607079215074));
#53123=CARTESIAN_POINT('Ctrl Pts',(4.24157890048061,0.79477268400084,6.59157705531633));
#53124=CARTESIAN_POINT('Ctrl Pts',(4.37480433638251,1.06847604194527,6.55184520336775));
#53125=CARTESIAN_POINT('Ctrl Pts',(4.44499154163423,1.1851427086121,6.53172693228782));
#53126=CARTESIAN_POINT('Ctrl Pts',(4.52769759742463,1.30000000000048,6.50868883662629));
#53127=CARTESIAN_POINT('Ctrl Pts',(4.55333646119701,-1.3,6.70483180220308));
#53128=CARTESIAN_POINT('Ctrl Pts',(4.46759044005475,-1.18514270861178,6.70468931916621));
#53129=CARTESIAN_POINT('Ctrl Pts',(4.39457954353636,-1.06847604194512,6.70321883895621));
#53130=CARTESIAN_POINT('Ctrl Pts',(4.25533045233314,-0.794772684000851,
6.69675379636771));
#53131=CARTESIAN_POINT('Ctrl Pts',(4.20084799529369,-0.636309800095197,
6.6903034367033));
#53132=CARTESIAN_POINT('Ctrl Pts',(4.1264371815048,-0.319434907277159,6.675134858055));
#53133=CARTESIAN_POINT('Ctrl Pts',(4.1083738762426,-0.158333333333332,6.66544968261944));
#53134=CARTESIAN_POINT('Ctrl Pts',(4.10569625638312,0.158333333333334,6.6451248466368));
#53135=CARTESIAN_POINT('Ctrl Pts',(4.12120905306815,0.319434907277167,6.63561768729212));
#53136=CARTESIAN_POINT('Ctrl Pts',(4.18990683146856,0.636309800095206,6.607079215074));
#53137=CARTESIAN_POINT('Ctrl Pts',(4.24157890048061,0.79477268400084,6.59157705531633));
#53138=CARTESIAN_POINT('Ctrl Pts',(4.37480433638243,1.06847604194511,6.55184520336778));
#53139=CARTESIAN_POINT('Ctrl Pts',(4.44499154163404,1.18514270861178,6.53172693228788));
#53140=CARTESIAN_POINT('Ctrl Pts',(4.52769759742429,1.3,6.50868883662639));
#53141=CARTESIAN_POINT('',(4.89593598449868,-1.2,6.47040364879548));
#53142=CARTESIAN_POINT('Ctrl Pts',(4.89593598449868,-1.2,6.47040364879548));
#53143=CARTESIAN_POINT('Ctrl Pts',(4.88552007488463,-1.21198332754869,6.48180974294822));
#53144=CARTESIAN_POINT('Ctrl Pts',(4.86715275551669,-1.23320804299601,6.5029687954801));
#53145=CARTESIAN_POINT('Ctrl Pts',(4.83662477530882,-1.26800122851154,6.53578088853726));
#53146=CARTESIAN_POINT('Ctrl Pts',(4.8232775251527,-1.28318627910763,6.55035026134636));
#53147=CARTESIAN_POINT('Ctrl Pts',(4.80833879006001,-1.29999999996669,6.56566721641765));
#53148=CARTESIAN_POINT('',(4.87041241528844,-0.653834841370086,6.31592822427069));
#53149=CARTESIAN_POINT('Ctrl Pts',(4.87041241532541,-0.653834841368829,
6.31592822426901));
#53150=CARTESIAN_POINT('Ctrl Pts',(4.87328845860714,-0.717304357747199,
6.33177254516113));
#53151=CARTESIAN_POINT('Ctrl Pts',(4.87561663331839,-0.764718184626917,
6.34493691099469));
#53152=CARTESIAN_POINT('Ctrl Pts',(4.88435675347613,-0.949625201953965,
6.39576546853942));
#53153=CARTESIAN_POINT('Ctrl Pts',(4.88944388081821,-1.05881455110567,6.42683856795065));
#53154=CARTESIAN_POINT('Ctrl Pts',(4.89593598449868,-1.2,6.47040364879548));
#53155=CARTESIAN_POINT('',(4.84356468978495,0.653834841531101,6.17902933643107));
#53156=CARTESIAN_POINT('Ctrl Pts',(4.84356468978495,0.653834841531099,6.17902933643107));
#53157=CARTESIAN_POINT('Ctrl Pts',(4.81027480171635,0.575967894595913,6.20394293927447));
#53158=CARTESIAN_POINT('Ctrl Pts',(4.78258938258321,0.493633270675005,6.22560831669507));
#53159=CARTESIAN_POINT('Ctrl Pts',(4.74428430246563,0.338128732286169,6.25868470950295));
#53160=CARTESIAN_POINT('Ctrl Pts',(4.73158136615163,0.265653446049887,6.27127805152257));
#53161=CARTESIAN_POINT('Ctrl Pts',(4.71755921729924,0.129712949542664,6.2912135864992));
#53162=CARTESIAN_POINT('Ctrl Pts',(4.71484070144113,0.0666229865808594,
6.29903019023757));
#53163=CARTESIAN_POINT('Ctrl Pts',(4.71704007282426,-0.0595430897305052,
6.31217543572927));
#53164=CARTESIAN_POINT('Ctrl Pts',(4.72195733819667,-0.122775140765603,
6.31760388022771));
#53165=CARTESIAN_POINT('Ctrl Pts',(4.74092964991683,-0.260125061892429,
6.32597746664295));
#53166=CARTESIAN_POINT('Ctrl Pts',(4.75649191430833,-0.333942206836294,
6.32829157281983));
#53167=CARTESIAN_POINT('Ctrl Pts',(4.80133465609412,-0.491210015044957,
6.32745084093312));
#53168=CARTESIAN_POINT('Ctrl Pts',(4.83265724001896,-0.574353127738433,
6.32346804471193));
#53169=CARTESIAN_POINT('Ctrl Pts',(4.87041241526413,-0.653834841386618,
6.31592822432322));
#53170=CARTESIAN_POINT('',(4.85795990615321,1.2,6.24988129678031));
#53171=CARTESIAN_POINT('Ctrl Pts',(4.85795990615321,1.2,6.24988129678031));
#53172=CARTESIAN_POINT('Ctrl Pts',(4.85544249344361,1.13014930724506,6.23700975770938));
#53173=CARTESIAN_POINT('Ctrl Pts',(4.85277540338472,1.05323054854764,6.22352942609793));
#53174=CARTESIAN_POINT('Ctrl Pts',(4.84602121616902,0.796444496061531,6.19067038861466));
#53175=CARTESIAN_POINT('Ctrl Pts',(4.84489099862009,0.73982206670996,6.18532144929078));
#53176=CARTESIAN_POINT('Ctrl Pts',(4.84356468978495,0.653834841531101,6.17902933643107));
#53177=CARTESIAN_POINT('Ctrl Pts',(4.77352764767187,1.30000000000002,6.34213416147271));
#53178=CARTESIAN_POINT('Ctrl Pts',(4.78797295912602,1.28314836924958,6.32724218773947));
#53179=CARTESIAN_POINT('Ctrl Pts',(4.80202291543942,1.26652615695483,6.31171709974393));
#53180=CARTESIAN_POINT('Ctrl Pts',(4.83031567071051,1.23309342866822,6.28121078500142));
#53181=CARTESIAN_POINT('Ctrl Pts',(4.8447116454302,1.21600083823975,6.26550527072992));
#53182=CARTESIAN_POINT('Ctrl Pts',(4.85795990615321,1.2,6.24988129678031));
#53183=CARTESIAN_POINT('Ctrl Pts',(4.55333646119701,-1.3,6.70483180220308));
#53184=CARTESIAN_POINT('Ctrl Pts',(4.46759044005475,-1.18514270861178,6.70468931916621));
#53185=CARTESIAN_POINT('Ctrl Pts',(4.39457954353636,-1.06847604194512,6.70321883895621));
#53186=CARTESIAN_POINT('Ctrl Pts',(4.25533045233313,-0.794772684000851,
6.69675379636771));
#53187=CARTESIAN_POINT('Ctrl Pts',(4.20084799529369,-0.636309800095197,
6.6903034367033));
#53188=CARTESIAN_POINT('Ctrl Pts',(4.1264371815048,-0.319434907277159,6.675134858055));
#53189=CARTESIAN_POINT('Ctrl Pts',(4.1083738762426,-0.158333333333332,6.66544968261944));
#53190=CARTESIAN_POINT('Ctrl Pts',(4.10569625638312,0.158333333333334,6.6451248466368));
#53191=CARTESIAN_POINT('Ctrl Pts',(4.12120905306814,0.319434907277167,6.63561768729212));
#53192=CARTESIAN_POINT('Ctrl Pts',(4.18990683146856,0.636309800095206,6.607079215074));
#53193=CARTESIAN_POINT('Ctrl Pts',(4.24157890048061,0.79477268400084,6.59157705531633));
#53194=CARTESIAN_POINT('Ctrl Pts',(4.37480433638243,1.06847604194511,6.55184520336778));
#53195=CARTESIAN_POINT('Ctrl Pts',(4.44499154163404,1.18514270861178,6.53172693228788));
#53196=CARTESIAN_POINT('Ctrl Pts',(4.52769759742429,1.3,6.50868883662639));
#53197=CARTESIAN_POINT('Ctrl Pts',(4.559720379007,-1.3,6.78150223240952));
#53198=CARTESIAN_POINT('Ctrl Pts',(4.47399349175896,-1.18514270861178,6.77962754301943));
#53199=CARTESIAN_POINT('Ctrl Pts',(4.40104080402149,-1.06847604194512,6.77695192352273));
#53200=CARTESIAN_POINT('Ctrl Pts',(4.26201645755201,-0.794772684000851,
6.76892039845776));
#53201=CARTESIAN_POINT('Ctrl Pts',(4.20777282266716,-0.636309800095197,
6.76314676763589));
#53202=CARTESIAN_POINT('Ctrl Pts',(4.13378893043112,-0.319434907277159,
6.74849045958165));
#53203=CARTESIAN_POINT('Ctrl Pts',(4.11602990877888,-0.158333333333332,
6.74000897151971));
#53204=CARTESIAN_POINT('Ctrl Pts',(4.11370927434805,0.158333333333334,6.71964661485659));
#53205=CARTESIAN_POINT('Ctrl Pts',(4.12926944463902,0.319434907277167,6.70889880747554));
#53206=CARTESIAN_POINT('Ctrl Pts',(4.19827830828669,0.636309800095206,6.67977049702301));
#53207=CARTESIAN_POINT('Ctrl Pts',(4.25004328077839,0.79477268400084,6.6635567426537));
#53208=CARTESIAN_POINT('Ctrl Pts',(4.38381424022261,1.06847604194511,6.62531041472351));
#53209=CARTESIAN_POINT('Ctrl Pts',(4.45430894480039,1.18514270861178,6.60635884545937));
#53210=CARTESIAN_POINT('Ctrl Pts',(4.53739386231511,1.3,6.58501112512597));
#53211=CARTESIAN_POINT('Ctrl Pts',(4.56610429681699,-1.3,6.85817266261596));
#53212=CARTESIAN_POINT('Ctrl Pts',(4.48039654346318,-1.18514270861178,6.85456576687265));
#53213=CARTESIAN_POINT('Ctrl Pts',(4.40750206450663,-1.06847604194512,6.85068500808926));
#53214=CARTESIAN_POINT('Ctrl Pts',(4.26870246277088,-0.794772684000851,
6.84108700054782));
#53215=CARTESIAN_POINT('Ctrl Pts',(4.21469765004064,-0.636309800095197,
6.83599009856847));
#53216=CARTESIAN_POINT('Ctrl Pts',(4.14114067935745,-0.319434907277159,
6.8218460611083));
#53217=CARTESIAN_POINT('Ctrl Pts',(4.12368594131515,-0.158333333333332,
6.81456826041999));
#53218=CARTESIAN_POINT('Ctrl Pts',(4.12172229231298,0.158333333333334,6.79416838307638));
#53219=CARTESIAN_POINT('Ctrl Pts',(4.1373298362099,0.319434907277167,6.78217992765896));
#53220=CARTESIAN_POINT('Ctrl Pts',(4.20664978510482,0.636309800095206,6.75246177897202));
#53221=CARTESIAN_POINT('Ctrl Pts',(4.25850766107617,0.79477268400084,6.73553642999107));
#53222=CARTESIAN_POINT('Ctrl Pts',(4.39282414406279,1.06847604194511,6.69877562607923));
#53223=CARTESIAN_POINT('Ctrl Pts',(4.46362634796674,1.18514270861178,6.68099075863087));
#53224=CARTESIAN_POINT('Ctrl Pts',(4.54709012720593,1.3,6.66133341362554));
#53225=CARTESIAN_POINT('Ctrl Pts',(4.57248821462698,-1.3,6.9348430928224));
#53226=CARTESIAN_POINT('Ctrl Pts',(4.48679959516739,-1.18514270861178,6.92950399072586));
#53227=CARTESIAN_POINT('Ctrl Pts',(4.41396332499177,-1.06847604194512,6.92441809265578));
#53228=CARTESIAN_POINT('Ctrl Pts',(4.27538846798975,-0.794772684000851,
6.91325360263787));
#53229=CARTESIAN_POINT('Ctrl Pts',(4.22162247741411,-0.636309800095197,
6.90883342950106));
#53230=CARTESIAN_POINT('Ctrl Pts',(4.14849242828377,-0.319434907277159,
6.89520166263496));
#53231=CARTESIAN_POINT('Ctrl Pts',(4.13134197385142,-0.158333333333332,
6.88912754932026));
#53232=CARTESIAN_POINT('Ctrl Pts',(4.12973531027791,0.158333333333334,6.86869015129617));
#53233=CARTESIAN_POINT('Ctrl Pts',(4.14539022778078,0.319434907277167,6.85546104784238));
#53234=CARTESIAN_POINT('Ctrl Pts',(4.21502126192296,0.636309800095206,6.82515306092103));
#53235=CARTESIAN_POINT('Ctrl Pts',(4.26697204137396,0.79477268400084,6.80751611732844));
#53236=CARTESIAN_POINT('Ctrl Pts',(4.40183404790297,1.06847604194511,6.77224083743496));
#53237=CARTESIAN_POINT('Ctrl Pts',(4.47294375113309,1.18514270861178,6.75562267180236));
#53238=CARTESIAN_POINT('Ctrl Pts',(4.55678639209675,1.3,6.73765570212511));
#53239=CARTESIAN_POINT('Ctrl Pts',(4.57248821462698,-1.3,6.9348430928224));
#53240=CARTESIAN_POINT('Ctrl Pts',(4.48679959516739,-1.18514270861178,6.92950399072586));
#53241=CARTESIAN_POINT('Ctrl Pts',(4.41396332499177,-1.06847604194512,6.92441809265578));
#53242=CARTESIAN_POINT('Ctrl Pts',(4.27538846798975,-0.794772684000851,
6.91325360263787));
#53243=CARTESIAN_POINT('Ctrl Pts',(4.22162247741411,-0.636309800095197,
6.90883342950106));
#53244=CARTESIAN_POINT('Ctrl Pts',(4.14849242828377,-0.319434907277159,
6.89520166263496));
#53245=CARTESIAN_POINT('Ctrl Pts',(4.13134197385143,-0.158333333333332,
6.88912754932026));
#53246=CARTESIAN_POINT('Ctrl Pts',(4.12973531027791,0.158333333333334,6.86869015129617));
#53247=CARTESIAN_POINT('Ctrl Pts',(4.14539022778078,0.319434907277167,6.85546104784238));
#53248=CARTESIAN_POINT('Ctrl Pts',(4.21502126192295,0.636309800095206,6.82515306092103));
#53249=CARTESIAN_POINT('Ctrl Pts',(4.26697204137395,0.79477268400084,6.80751611732844));
#53250=CARTESIAN_POINT('Ctrl Pts',(4.40183404790297,1.06847604194511,6.77224083743496));
#53251=CARTESIAN_POINT('Ctrl Pts',(4.47294375113309,1.18514270861178,6.75562267180236));
#53252=CARTESIAN_POINT('Ctrl Pts',(4.55678639209675,1.3,6.73765570212511));
#53253=CARTESIAN_POINT('Ctrl Pts',(4.57248821462698,-1.3,6.9348430928224));
#53254=CARTESIAN_POINT('Ctrl Pts',(4.48679959516739,-1.18514270861178,6.92950399072586));
#53255=CARTESIAN_POINT('Ctrl Pts',(4.41396332499177,-1.06847604194512,6.92441809265578));
#53256=CARTESIAN_POINT('Ctrl Pts',(4.27538846798975,-0.794772684000851,
6.91325360263787));
#53257=CARTESIAN_POINT('Ctrl Pts',(4.22162247741411,-0.636309800095197,
6.90883342950106));
#53258=CARTESIAN_POINT('Ctrl Pts',(4.14849242828377,-0.319434907277159,
6.89520166263495));
#53259=CARTESIAN_POINT('Ctrl Pts',(4.13134197385142,-0.158333333333332,
6.88912754932025));
#53260=CARTESIAN_POINT('Ctrl Pts',(4.12973531027791,0.158333333333334,6.86869015129617));
#53261=CARTESIAN_POINT('Ctrl Pts',(4.14539022778078,0.319434907277167,6.85546104784237));
#53262=CARTESIAN_POINT('Ctrl Pts',(4.21502126192295,0.636309800095206,6.82515306092102));
#53263=CARTESIAN_POINT('Ctrl Pts',(4.26697204137396,0.79477268400084,6.80751611732844));
#53264=CARTESIAN_POINT('Ctrl Pts',(4.40183404790374,1.06847604194666,6.77224083743476));
#53265=CARTESIAN_POINT('Ctrl Pts',(4.47294375113495,1.18514270861482,6.75562267180193));
#53266=CARTESIAN_POINT('Ctrl Pts',(4.55678639210004,1.3000000000045,6.73765570212441));
#53267=CARTESIAN_POINT('Ctrl Pts',(4.57985658845472,-1.3,6.93956537747332));
#53268=CARTESIAN_POINT('Ctrl Pts',(4.4939975863417,-1.18514270861178,6.93356194558967));
#53269=CARTESIAN_POINT('Ctrl Pts',(4.42096106045723,-1.06847604194512,6.92841142118886));
#53270=CARTESIAN_POINT('Ctrl Pts',(4.28185455997266,-0.794772684000851,
6.91848306637304));
#53271=CARTESIAN_POINT('Ctrl Pts',(4.22749554624361,-0.636309800095197,
6.91766357207286));
#53272=CARTESIAN_POINT('Ctrl Pts',(4.1540436348186,-0.319434907277159,6.90577978298097));
#53273=CARTESIAN_POINT('Ctrl Pts',(4.13706908978531,-0.158333333333332,
6.89918937142415));
#53274=CARTESIAN_POINT('Ctrl Pts',(4.13553292450502,0.158333333333334,6.87852588248496));
#53275=CARTESIAN_POINT('Ctrl Pts',(4.1511379029416,0.319434907277167,6.86531247060522));
#53276=CARTESIAN_POINT('Ctrl Pts',(4.22112140677529,0.636309800095206,6.83335514381765));
#53277=CARTESIAN_POINT('Ctrl Pts',(4.27351162156741,0.79477268400084,6.81319036325118));
#53278=CARTESIAN_POINT('Ctrl Pts',(4.40891552697402,1.06847604194666,6.77652568448102));
#53279=CARTESIAN_POINT('Ctrl Pts',(4.48025898194898,1.18514270861482,6.75965397193426));
#53280=CARTESIAN_POINT('Ctrl Pts',(4.56433455845715,1.3000000000045,6.74178132772021));
#53281=CARTESIAN_POINT('Ctrl Pts',(4.59168572246724,-1.30000000000002,6.94280967669042));
#53282=CARTESIAN_POINT('Ctrl Pts',(4.50842963072979,-1.1851427086118,6.93550875066837));
#53283=CARTESIAN_POINT('Ctrl Pts',(4.437190204196,-1.06847604194513,6.93004561131568));
#53284=CARTESIAN_POINT('Ctrl Pts',(4.30037377805058,-0.794772684000862,
6.92167032136784));
#53285=CARTESIAN_POINT('Ctrl Pts',(4.24470982715029,-0.636309800095207,
6.92623862411642));
#53286=CARTESIAN_POINT('Ctrl Pts',(4.17077209362945,-0.319434907277164,
6.91719495861301));
#53287=CARTESIAN_POINT('Ctrl Pts',(4.15284748798856,-0.158333333333335,
6.91033447894196));
#53288=CARTESIAN_POINT('Ctrl Pts',(4.15134880332261,0.158333333333337,6.88950691599258));
#53289=CARTESIAN_POINT('Ctrl Pts',(4.16800480359992,0.319434907277172,6.87653626951492));
#53290=CARTESIAN_POINT('Ctrl Pts',(4.2384211693924,0.636309800095216,6.84112601890762));
#53291=CARTESIAN_POINT('Ctrl Pts',(4.29185181052877,0.794772684000852,6.8144698216443));
#53292=CARTESIAN_POINT('Ctrl Pts',(4.42497591024534,1.06847604194667,6.77632001966336));
#53293=CARTESIAN_POINT('Ctrl Pts',(4.49458557019052,1.18514270861484,6.76008017149172));
#53294=CARTESIAN_POINT('Ctrl Pts',(4.5761804000472,1.30000000000452,6.74411411083662));
#53295=CARTESIAN_POINT('Ctrl Pts',(4.60901351621805,-1.30000000000003,6.94776612680297));
#53296=CARTESIAN_POINT('Ctrl Pts',(4.52942942664903,-1.18514270861181,6.94042190776583));
#53297=CARTESIAN_POINT('Ctrl Pts',(4.46089500922349,-1.06847604194514,6.93513362968046));
#53298=CARTESIAN_POINT('Ctrl Pts',(4.32809374783802,-0.794772684000868,
6.92766628427501));
#53299=CARTESIAN_POINT('Ctrl Pts',(4.27191634453898,-0.636309800095211,
6.93373309324915));
#53300=CARTESIAN_POINT('Ctrl Pts',(4.1981511998046,-0.319434907277166,6.92597574477209));
#53301=CARTESIAN_POINT('Ctrl Pts',(4.1789303220762,-0.158333333333336,6.9197783105525));
#53302=CARTESIAN_POINT('Ctrl Pts',(4.17740932610982,0.158333333333338,6.8988415262861));
#53303=CARTESIAN_POINT('Ctrl Pts',(4.19532242039286,0.319434907277174,6.88542037767051));
#53304=CARTESIAN_POINT('Ctrl Pts',(4.26555510730558,0.63630980009522,6.84784592269368));
#53305=CARTESIAN_POINT('Ctrl Pts',(4.31951206683825,0.794772684000859,6.8178513996686));
#53306=CARTESIAN_POINT('Ctrl Pts',(4.44867433870729,1.06847604194668,6.77863163545275));
#53307=CARTESIAN_POINT('Ctrl Pts',(4.51561242266566,1.18514270861485,6.76255514417353));
#53308=CARTESIAN_POINT('Ctrl Pts',(4.59357902902374,1.30000000000453,6.74737894430877));
#53309=CARTESIAN_POINT('Ctrl Pts',(4.6233534298674,-1.30000000000005,6.95207556239594));
#53310=CARTESIAN_POINT('Ctrl Pts',(4.54651014232481,-1.18514270861182,6.94505581919046));
#53311=CARTESIAN_POINT('Ctrl Pts',(4.4799715641937,-1.06847604194515,6.93986541852847));
#53312=CARTESIAN_POINT('Ctrl Pts',(4.35006007790447,-0.794772684000877,
6.93210070189737));
#53313=CARTESIAN_POINT('Ctrl Pts',(4.29331731838996,-0.636309800095217,
6.9365561992288));
#53314=CARTESIAN_POINT('Ctrl Pts',(4.21956531577933,-0.319434907277168,
6.92900915459488));
#53315=CARTESIAN_POINT('Ctrl Pts',(4.19938038514094,-0.158333333333338,
6.92456854816355));
#53316=CARTESIAN_POINT('Ctrl Pts',(4.19784131139462,0.158333333333339,6.90424024601326));
#53317=CARTESIAN_POINT('Ctrl Pts',(4.21669151098746,0.319434907277178,6.89059198569614));
#53318=CARTESIAN_POINT('Ctrl Pts',(4.28689229982556,0.636309800095227,6.85217017386736));
#53319=CARTESIAN_POINT('Ctrl Pts',(4.34140188971318,0.794772684000865,6.82045193860963));
#53320=CARTESIAN_POINT('Ctrl Pts',(4.46771360256903,1.06847604194669,6.78102673047936));
#53321=CARTESIAN_POINT('Ctrl Pts',(4.53268578500315,1.18514270861486,6.76523453140521));
#53322=CARTESIAN_POINT('Ctrl Pts',(4.60795448968593,1.30000000000454,6.75071584500868));
#53323=CARTESIAN_POINT('Ctrl Pts',(4.64065212265408,-1.30000000000006,6.95781610440239));
#53324=CARTESIAN_POINT('Ctrl Pts',(4.56736875666192,-1.18514270861184,6.95137736045384));
#53325=CARTESIAN_POINT('Ctrl Pts',(4.50344330243136,-1.06847604194516,6.94637658530222));
#53326=CARTESIAN_POINT('Ctrl Pts',(4.37738136312857,-0.794772684000886,
6.93814578988592));
#53327=CARTESIAN_POINT('Ctrl Pts',(4.32005877814057,-0.636309800095224,
6.94041641143475));
#53328=CARTESIAN_POINT('Ctrl Pts',(4.24644502861887,-0.319434907277172,
6.93216354244808));
#53329=CARTESIAN_POINT('Ctrl Pts',(4.22505541355766,-0.158333333333339,
6.92921338110318));
#53330=CARTESIAN_POINT('Ctrl Pts',(4.22347657514697,0.158333333333341,6.90773716913098));
#53331=CARTESIAN_POINT('Ctrl Pts',(4.2434536947023,0.31943490727718,6.89074124728874));
#53332=CARTESIAN_POINT('Ctrl Pts',(4.3135126355416,0.636309800095232,6.85213185666438));
#53333=CARTESIAN_POINT('Ctrl Pts',(4.36867916688973,0.794772684000874,6.82364499201943));
#53334=CARTESIAN_POINT('Ctrl Pts',(4.49121503331224,1.0684760419467,6.78527105908375));
#53335=CARTESIAN_POINT('Ctrl Pts',(4.55360760784926,1.18514270861487,6.76955654046397));
#53336=CARTESIAN_POINT('Ctrl Pts',(4.62535152074995,1.30000000000456,6.75473815689801));
#53337=CARTESIAN_POINT('Ctrl Pts',(4.65772891567358,-1.3000000000001,6.9650122729636));
#53338=CARTESIAN_POINT('Ctrl Pts',(4.58785149243056,-1.18514270861187,6.95886872864369));
#53339=CARTESIAN_POINT('Ctrl Pts',(4.52642377891097,-1.06847604194519,6.95380579361821));
#53340=CARTESIAN_POINT('Ctrl Pts',(4.40403399192852,-0.794772684000904,
6.94460582451793));
#53341=CARTESIAN_POINT('Ctrl Pts',(4.34613524203725,-0.636309800095241,
6.94495603954721));
#53342=CARTESIAN_POINT('Ctrl Pts',(4.27264773874593,-0.319434907277181,
6.93470095333162));
#53343=CARTESIAN_POINT('Ctrl Pts',(4.25011864464721,-0.158333333333343,
6.93042203799672));
#53344=CARTESIAN_POINT('Ctrl Pts',(4.24850364252821,0.158333333333345,6.90847420714758));
#53345=CARTESIAN_POINT('Ctrl Pts',(4.26954211934693,0.319434907277189,6.89234795461961));
#53346=CARTESIAN_POINT('Ctrl Pts',(4.33948661664487,0.63630980009525,6.85475459626415));
#53347=CARTESIAN_POINT('Ctrl Pts',(4.39531220514294,0.794772684000897,6.82742116863333));
#53348=CARTESIAN_POINT('Ctrl Pts',(4.5142895898812,1.06847604194673,6.78952706502359));
#53349=CARTESIAN_POINT('Ctrl Pts',(4.57424140111991,1.18514270861491,6.77380152188313));
#53350=CARTESIAN_POINT('Ctrl Pts',(4.64264412229035,1.30000000000459,6.75875338894005));
#53351=CARTESIAN_POINT('Ctrl Pts',(4.68074462869342,-1.3000000000001,6.97223030803504));
#53352=CARTESIAN_POINT('Ctrl Pts',(4.61546701102458,-1.18514270861187,6.96711220410798));
#53353=CARTESIAN_POINT('Ctrl Pts',(4.55741287000154,-1.0684760419452,6.96255256638903));
#53354=CARTESIAN_POINT('Ctrl Pts',(4.43998386665053,-0.794772684000911,
6.95330905976739));
#53355=CARTESIAN_POINT('Ctrl Pts',(4.38130823543249,-0.636309800095243,
6.95178561930535));
#53356=CARTESIAN_POINT('Ctrl Pts',(4.307995220275,-0.319434907277182,6.93983193085731));
#53357=CARTESIAN_POINT('Ctrl Pts',(4.28392004501045,-0.158333333333344,
6.93449206360987));
#53358=CARTESIAN_POINT('Ctrl Pts',(4.28228212154936,0.158333333333346,6.91164478340126));
#53359=CARTESIAN_POINT('Ctrl Pts',(4.30482303330787,0.319434907277191,6.89508261334793));
#53360=CARTESIAN_POINT('Ctrl Pts',(4.37458856844489,0.636309800095253,6.85857264532631));
#53361=CARTESIAN_POINT('Ctrl Pts',(4.4312245980318,0.794772684000898,6.83394799296566));
#53362=CARTESIAN_POINT('Ctrl Pts',(4.54529186856434,1.06847604194673,6.79691837208924));
#53363=CARTESIAN_POINT('Ctrl Pts',(4.60189712594626,1.18514270861491,6.78112435439916));
#53364=CARTESIAN_POINT('Ctrl Pts',(4.66573214590514,1.3000000000046,6.76556506981383));
#53365=CARTESIAN_POINT('Ctrl Pts',(4.70347027821068,-1.30000000000016,6.9823724522687));
#53366=CARTESIAN_POINT('Ctrl Pts',(4.64271971394712,-1.18514270861193,6.97849915325402));
#53367=CARTESIAN_POINT('Ctrl Pts',(4.58800010266077,-1.06847604194524,6.9744350044508));
#53368=CARTESIAN_POINT('Ctrl Pts',(4.47551956183392,-0.794772684000947,
6.96460510649433));
#53369=CARTESIAN_POINT('Ctrl Pts',(4.41619320511171,-0.636309800095273,
6.95982737803518));
#53370=CARTESIAN_POINT('Ctrl Pts',(4.34312042184911,-0.319434907277197,
6.94537946334079));
#53371=CARTESIAN_POINT('Ctrl Pts',(4.31751409845567,-0.158333333333351,
6.93882991032973));
#53372=CARTESIAN_POINT('Ctrl Pts',(4.31585533458879,0.158333333333353,6.91545225315629));
#53373=CARTESIAN_POINT('Ctrl Pts',(4.33985068426229,0.319434907277205,6.89984296341105));
#53374=CARTESIAN_POINT('Ctrl Pts',(4.40944733987471,0.636309800095282,6.86418963648015));
#53375=CARTESIAN_POINT('Ctrl Pts',(4.4669199632229,0.794772684000936,6.84053040220008));
#53376=CARTESIAN_POINT('Ctrl Pts',(4.57615689899014,1.06847604194678,6.80362722765851));
#53377=CARTESIAN_POINT('Ctrl Pts',(4.62946163274559,1.18514270861497,6.7876436506777));
#53378=CARTESIAN_POINT('Ctrl Pts',(4.68878647838988,1.30000000000466,6.77165051357786));
#53379=CARTESIAN_POINT('Ctrl Pts',(4.73772090176179,-1.30000000000017,6.99560535184883));
#53380=CARTESIAN_POINT('Ctrl Pts',(4.68380518377452,-1.18514270861193,6.99338267515873));
#53381=CARTESIAN_POINT('Ctrl Pts',(4.63410339321969,-1.06847604194525,6.99025797323616));
#53382=CARTESIAN_POINT('Ctrl Pts',(4.52901732959112,-0.794772684000953,
6.98095542796402));
#53383=CARTESIAN_POINT('Ctrl Pts',(4.46854489566491,-0.636309800095279,
6.97453050087433));
#53384=CARTESIAN_POINT('Ctrl Pts',(4.39581782749983,-0.3194349072772,6.95729884977924));
#53385=CARTESIAN_POINT('Ctrl Pts',(4.36803658709379,-0.158333333333352,
6.94725609926108));
#53386=CARTESIAN_POINT('Ctrl Pts',(4.3663924659603,0.158333333333354,6.92263405197941));
#53387=CARTESIAN_POINT('Ctrl Pts',(4.39256517391286,0.319434907277205,6.90860399762272));
#53388=CARTESIAN_POINT('Ctrl Pts',(4.46187079413096,0.636309800095285,6.87456354401537));
#53389=CARTESIAN_POINT('Ctrl Pts',(4.52053080970807,0.794772684000943,6.8533649349418));
#53390=CARTESIAN_POINT('Ctrl Pts',(4.62246797863368,1.0684760419468,6.81620646621921));
#53391=CARTESIAN_POINT('Ctrl Pts',(4.67080332086836,1.18514270861498,6.79941891700058));
#53392=CARTESIAN_POINT('Ctrl Pts',(4.72334918205387,1.30000000000467,6.78192834281648));
#53393=CARTESIAN_POINT('Ctrl Pts',(4.77170045210599,-1.30000000000031,7.01099742213157));
#53394=CARTESIAN_POINT('Ctrl Pts',(4.72457989536022,-1.18514270861206,7.01054672126873));
#53395=CARTESIAN_POINT('Ctrl Pts',(4.67987505604944,-1.06847604194537,7.00838749823058));
#53396=CARTESIAN_POINT('Ctrl Pts',(4.5821787246065,-0.794772684001035,6.99945223304775));
#53397=CARTESIAN_POINT('Ctrl Pts',(4.52064605182507,-0.636309800095346,
6.9902351849925));
#53398=CARTESIAN_POINT('Ctrl Pts',(4.4482758509293,-0.319434907277234,6.97114789687891));
#53399=CARTESIAN_POINT('Ctrl Pts',(4.41826092950754,-0.15833333333337,6.96037904196055));
#53400=CARTESIAN_POINT('Ctrl Pts',(4.41663733815419,0.158333333333371,6.93485712386133));
#53401=CARTESIAN_POINT('Ctrl Pts',(4.44502504936253,0.319434907277241,6.92068169288381));
#53402=CARTESIAN_POINT('Ctrl Pts',(4.51409548293143,0.636309800095355,6.88660607626106));
#53403=CARTESIAN_POINT('Ctrl Pts',(4.57398757726845,0.794772684001026,6.86635219269857));
#53404=CARTESIAN_POINT('Ctrl Pts',(4.66867345823415,1.06847604194691,6.82852799893898));
#53405=CARTESIAN_POINT('Ctrl Pts',(4.71205687341492,1.18514270861511,6.81112568365538));
#53406=CARTESIAN_POINT('Ctrl Pts',(4.7578376943638,1.30000000000481,6.79269374504232));
#53407=CARTESIAN_POINT('Ctrl Pts',(4.80284656862992,-1.3000000000004,7.0246922001963));
#53408=CARTESIAN_POINT('Ctrl Pts',(4.76180440192939,-1.18514270861215,7.02714890150709));
#53409=CARTESIAN_POINT('Ctrl Pts',(4.7215804598047,-1.06847604194545,7.02680909351662));
#53410=CARTESIAN_POINT('Ctrl Pts',(4.6305453691801,-0.794772684001097,7.01956357315458));
#53411=CARTESIAN_POINT('Ctrl Pts',(4.56812621870751,-0.636309800095391,
7.0079220313082));
#53412=CARTESIAN_POINT('Ctrl Pts',(4.49617888379903,-0.319434907277255,
6.98635594713443));
#53413=CARTESIAN_POINT('Ctrl Pts',(4.46425646853839,-0.15833333333338,6.97271361979845));
#53414=CARTESIAN_POINT('Ctrl Pts',(4.46270091772386,0.158333333333382,6.94610378427663));
#53415=CARTESIAN_POINT('Ctrl Pts',(4.49305793527175,0.319434907277263,6.93331088443485));
#53416=CARTESIAN_POINT('Ctrl Pts',(4.56185678259714,0.636309800095399,6.9003189849978));
#53417=CARTESIAN_POINT('Ctrl Pts',(4.62279227031746,0.794772684001082,6.8820914801612));
#53418=CARTESIAN_POINT('Ctrl Pts',(4.71084723147589,1.06847604194698,6.84306730324731));
#53419=CARTESIAN_POINT('Ctrl Pts',(4.74972412878629,1.18514270861519,6.8243806532821));
#53420=CARTESIAN_POINT('Ctrl Pts',(4.78936219347922,1.3000000000049,6.80389947354956));
#53421=CARTESIAN_POINT('Ctrl Pts',(4.81971140125444,-1.30000000000041,7.03315528836703));
#53422=CARTESIAN_POINT('Ctrl Pts',(4.78205573170685,-1.18514270861216,7.03656810206538));
#53423=CARTESIAN_POINT('Ctrl Pts',(4.74432372331691,-1.06847604194546,7.03679188724867));
#53424=CARTESIAN_POINT('Ctrl Pts',(4.65697887767639,-0.794772684001105,
7.02994158195739));
#53425=CARTESIAN_POINT('Ctrl Pts',(4.59403847146914,-0.636309800095399,
7.01716029480937));
#53426=CARTESIAN_POINT('Ctrl Pts',(4.52228780611912,-0.319434907277259,
6.99474285236196));
#53427=CARTESIAN_POINT('Ctrl Pts',(4.48928384359097,-0.158333333333382,
6.98032903146902));
#53428=CARTESIAN_POINT('Ctrl Pts',(4.48772670483764,0.158333333333384,6.95368112889899));
#53429=CARTESIAN_POINT('Ctrl Pts',(4.51913133053022,0.319434907277267,6.9418614804413));
#53430=CARTESIAN_POINT('Ctrl Pts',(4.58779617081258,0.636309800095406,6.90915489343853));
#53431=CARTESIAN_POINT('Ctrl Pts',(4.64936530997947,0.794772684001091,6.89103472616041));
#53432=CARTESIAN_POINT('Ctrl Pts',(4.73382833875133,1.068476041947,6.85105551647746));
#53433=CARTESIAN_POINT('Ctrl Pts',(4.77024949270081,1.1851427086152,6.83169607364316));
#53434=CARTESIAN_POINT('Ctrl Pts',(4.80653088510784,1.30000000000491,6.8102827064707));
#53435=CARTESIAN_POINT('Ctrl Pts',(4.83096799856834,-1.30000000000042,7.03863230490359));
#53436=CARTESIAN_POINT('Ctrl Pts',(4.79552525970306,-1.18514270861216,7.04304197726479));
#53437=CARTESIAN_POINT('Ctrl Pts',(4.7594275305241,-1.06847604194546,7.04386721275325));
#53438=CARTESIAN_POINT('Ctrl Pts',(4.67452139613975,-0.794772684001107,
7.03749290557919));
#53439=CARTESIAN_POINT('Ctrl Pts',(4.61129369378158,-0.6363098000954,7.02353895100331));
#53440=CARTESIAN_POINT('Ctrl Pts',(4.53968737529017,-0.31943490727726,7.00048559153463));
#53441=CARTESIAN_POINT('Ctrl Pts',(4.50593463306667,-0.158333333333383,
6.98581607785175));
#53442=CARTESIAN_POINT('Ctrl Pts',(4.50439362104787,0.158333333333385,6.95890559981965));
#53443=CARTESIAN_POINT('Ctrl Pts',(4.5365515958803,0.319434907277268,6.94703279480892));
#53444=CARTESIAN_POINT('Ctrl Pts',(4.60512847966881,0.636309800095408,6.91452153408074));
#53445=CARTESIAN_POINT('Ctrl Pts',(4.66706162126644,0.794772684001093,6.89726615352155));
#53446=CARTESIAN_POINT('Ctrl Pts',(4.74911765294583,1.068476041947,6.85682604989947));
#53447=CARTESIAN_POINT('Ctrl Pts',(4.78390477172902,1.1851427086152,6.8369783580517));
#53448=CARTESIAN_POINT('Ctrl Pts',(4.81795999365678,1.30000000000492,6.81478799676077));
#53449=CARTESIAN_POINT('Ctrl Pts',(4.85064503155324,-1.30000000000048,7.04822977209989));
#53450=CARTESIAN_POINT('Ctrl Pts',(4.81903273181648,-1.18514270861222,7.05464112033737));
#53451=CARTESIAN_POINT('Ctrl Pts',(4.78575590538376,-1.06847604194551,7.05679631184695));
#53452=CARTESIAN_POINT('Ctrl Pts',(4.70503438966276,-0.794772684001141,
7.05194266189598));
#53453=CARTESIAN_POINT('Ctrl Pts',(4.64119241175957,-0.63630980009543,7.03711520378676));
#53454=CARTESIAN_POINT('Ctrl Pts',(4.569903924195,-0.319434907277277,7.01237065244096));
#53455=CARTESIAN_POINT('Ctrl Pts',(4.53507152662869,-0.15833333333339,6.99506602236045));
#53456=CARTESIAN_POINT('Ctrl Pts',(4.53364402719554,0.158333333333392,6.96692253685092));
#53457=CARTESIAN_POINT('Ctrl Pts',(4.56703024750014,0.31943490727728,6.95587817161925));
#53458=CARTESIAN_POINT('Ctrl Pts',(4.63544906689471,0.636309800095436,6.92371507805114));
#53459=CARTESIAN_POINT('Ctrl Pts',(4.69805011618501,0.794772684001133,6.90760418502399));
#53460=CARTESIAN_POINT('Ctrl Pts',(4.77591426929651,1.06847604194705,6.86601741539685));
#53461=CARTESIAN_POINT('Ctrl Pts',(4.80784953659453,1.18514270861526,6.84516416546964));
#53462=CARTESIAN_POINT('Ctrl Pts',(4.83801556445957,1.30000000000498,6.82145903724525));
#53463=CARTESIAN_POINT('Ctrl Pts',(4.87871671758069,-1.30000000000054,7.06204569683692));
#53464=CARTESIAN_POINT('Ctrl Pts',(4.85261429636222,-1.18514270861228,7.07091863093545));
#53465=CARTESIAN_POINT('Ctrl Pts',(4.82339622580947,-1.06847604194556,7.07467246919414));
#53466=CARTESIAN_POINT('Ctrl Pts',(4.74869886453194,-0.794772684001184,
7.07151845106283));
#53467=CARTESIAN_POINT('Ctrl Pts',(4.68402722643482,-0.636309800095464,
7.05490525161979));
#53468=CARTESIAN_POINT('Ctrl Pts',(4.61311119848741,-0.319434907277293,
7.02872583981344));
#53469=CARTESIAN_POINT('Ctrl Pts',(4.57655793236568,-0.158333333333399,
7.00971783538784));
#53470=CARTESIAN_POINT('Ctrl Pts',(4.57519716966948,0.1583333333334,6.98097470457716));
#53471=CARTESIAN_POINT('Ctrl Pts',(4.61036071493994,0.319434907277299,6.97097376742859));
#53472=CARTESIAN_POINT('Ctrl Pts',(4.6785639529302,0.636309800095471,6.93914692873393));
#53473=CARTESIAN_POINT('Ctrl Pts',(4.74215816227969,0.794772684001174,6.92381055693346));
#53474=CARTESIAN_POINT('Ctrl Pts',(4.81404997075486,1.06847604194711,6.88067792422925));
#53475=CARTESIAN_POINT('Ctrl Pts',(4.84191306424059,1.18514270861532,6.85863141173312));
#53476=CARTESIAN_POINT('Ctrl Pts',(4.86651995117699,1.30000000000505,6.8332089052171));
#53477=CARTESIAN_POINT('Ctrl Pts',(4.91215937291756,-1.30000000000072,7.08002716631402));
#53478=CARTESIAN_POINT('Ctrl Pts',(4.89251476135823,-1.18514270861244,7.09277168660335));
#53479=CARTESIAN_POINT('Ctrl Pts',(4.86807491003913,-1.0684760419457,7.09900844705983));
#53480=CARTESIAN_POINT('Ctrl Pts',(4.80053600118698,-0.794772684001288,
7.09838238428716));
#53481=CARTESIAN_POINT('Ctrl Pts',(4.73507778921139,-0.636309800095545,
7.07844833130014));
#53482=CARTESIAN_POINT('Ctrl Pts',(4.66466571408515,-0.319434907277332,
7.05037683229815));
#53483=CARTESIAN_POINT('Ctrl Pts',(4.62598644584666,-0.158333333333419,
7.02995740311529));
#53484=CARTESIAN_POINT('Ctrl Pts',(4.62473318702404,0.158333333333421,7.00024857509394));
#53485=CARTESIAN_POINT('Ctrl Pts',(4.66209924063571,0.319434907277341,6.99060220955304));
#53486=CARTESIAN_POINT('Ctrl Pts',(4.73008064343413,0.636309800095553,6.95888608045245));
#53487=CARTESIAN_POINT('Ctrl Pts',(4.79480850862359,0.794772684001275,6.94538259911256));
#53488=CARTESIAN_POINT('Ctrl Pts',(4.8596126378628,1.06847604194724,6.89966616634739));
#53489=CARTESIAN_POINT('Ctrl Pts',(4.88264845166585,1.18514270861547,6.87556527970286));
#53490=CARTESIAN_POINT('Ctrl Pts',(4.90066877295375,1.30000000000521,6.84715245619721));
#53491=CARTESIAN_POINT('Ctrl Pts',(4.93725468010072,-1.3000000000009,7.09313254193612));
#53492=CARTESIAN_POINT('Ctrl Pts',(4.92251910617382,-1.1851427086126,7.10818590821563));
#53493=CARTESIAN_POINT('Ctrl Pts',(4.90167952468772,-1.06847604194585,7.11607516844198));
#53494=CARTESIAN_POINT('Ctrl Pts',(4.83943444394655,-0.7947726840014,7.11775041964863));
#53495=CARTESIAN_POINT('Ctrl Pts',(4.77307358991183,-0.636309800095634,
7.09754354905514));
#53496=CARTESIAN_POINT('Ctrl Pts',(4.70299017031348,-0.319434907277378,
7.06849582648515));
#53497=CARTESIAN_POINT('Ctrl Pts',(4.66292407258137,-0.158333333333441,
7.0456896209772));
#53498=CARTESIAN_POINT('Ctrl Pts',(4.66180668659304,0.158333333333443,7.01506827046914));
#53499=CARTESIAN_POINT('Ctrl Pts',(4.70074790993159,0.319434907277388,7.0064583020073));
#53500=CARTESIAN_POINT('Ctrl Pts',(4.7685705480685,0.636309800095645,6.97475153656514));
#53501=CARTESIAN_POINT('Ctrl Pts',(4.83420160951624,0.794772684001386,6.96180863596743));
#53502=CARTESIAN_POINT('Ctrl Pts',(4.89371750845255,1.06847604194739,6.91403814004657));
#53503=CARTESIAN_POINT('Ctrl Pts',(4.91313980712197,1.18514270861564,6.88848593338276));
#53504=CARTESIAN_POINT('Ctrl Pts',(4.92622217709251,1.3000000000054,6.85805959766812));
#53505=CARTESIAN_POINT('Ctrl Pts',(4.95249061094029,-1.30000000000096,7.10174801877597));
#53506=CARTESIAN_POINT('Ctrl Pts',(4.94070585124906,-1.18514270861266,7.11849736921204));
#53507=CARTESIAN_POINT('Ctrl Pts',(4.9220425490444,-1.06847604194591,7.12752623178392));
#53508=CARTESIAN_POINT('Ctrl Pts',(4.8630357781171,-0.794772684001439,7.13054883909814));
#53509=CARTESIAN_POINT('Ctrl Pts',(4.79622705686757,-0.636309800095667,
7.10950393241955));
#53510=CARTESIAN_POINT('Ctrl Pts',(4.72640341159517,-0.319434907277394,
7.07947600393533));
#53511=CARTESIAN_POINT('Ctrl Pts',(4.68551672620583,-0.158333333333449,
7.05503452127875));
#53512=CARTESIAN_POINT('Ctrl Pts',(4.68445951073731,0.158333333333451,7.02403999448838));
#53513=CARTESIAN_POINT('Ctrl Pts',(4.72429471911312,0.319434907277403,7.01652446843246));
#53514=CARTESIAN_POINT('Ctrl Pts',(4.79195320377858,0.636309800095676,6.98537928389906));
#53515=CARTESIAN_POINT('Ctrl Pts',(4.85806437875647,0.794772684001427,6.97348302681867));
#53516=CARTESIAN_POINT('Ctrl Pts',(4.9143815398544,1.06847604194745,6.92419940749604));
#53517=CARTESIAN_POINT('Ctrl Pts',(4.93163769063275,1.1851427086157,6.89740020700775));
#53518=CARTESIAN_POINT('Ctrl Pts',(4.94177237990647,1.30000000000546,6.86513485869803));
#53519=CARTESIAN_POINT('Ctrl Pts',(4.95733067203265,-1.30000000000097,7.10451141794751));
#53520=CARTESIAN_POINT('Ctrl Pts',(4.94647610786229,-1.18514270861266,7.12183906008298));
#53521=CARTESIAN_POINT('Ctrl Pts',(4.92850102344608,-1.06847604194591,7.13124929539685));
#53522=CARTESIAN_POINT('Ctrl Pts',(4.87052515631817,-0.794772684001442,
7.13469802785336));
#53523=CARTESIAN_POINT('Ctrl Pts',(4.80359922661366,-0.636309800095668,
7.11325670664432));
#53524=CARTESIAN_POINT('Ctrl Pts',(4.73385490618067,-0.319434907277395,
7.0829648622029));
#53525=CARTESIAN_POINT('Ctrl Pts',(4.69267438292149,-0.15833333333345,7.05823840696025));
#53526=CARTESIAN_POINT('Ctrl Pts',(4.69164133602762,0.158333333333452,7.02708359220464));
#53527=CARTESIAN_POINT('Ctrl Pts',(4.73179205882609,0.319434907277404,7.01968331650939));
#53528=CARTESIAN_POINT('Ctrl Pts',(4.79942552436748,0.636309800095677,6.9884947697978));
#53529=CARTESIAN_POINT('Ctrl Pts',(4.86571380921929,0.794772684001429,6.976708471892));
#53530=CARTESIAN_POINT('Ctrl Pts',(4.92100610955694,1.06847604194745,6.92700584775463));
#53531=CARTESIAN_POINT('Ctrl Pts',(4.93756098960259,1.1851427086157,6.89991592312669));
#53532=CARTESIAN_POINT('Ctrl Pts',(4.94673676165919,1.30000000000546,6.8672504981963));
#53533=CARTESIAN_POINT('Ctrl Pts',(4.96008932255006,-1.30000000000097,7.10613091373259));
#53534=CARTESIAN_POINT('Ctrl Pts',(4.94975998138204,-1.18514270861267,7.1238253241681));
#53535=CARTESIAN_POINT('Ctrl Pts',(4.9321750309227,-1.06847604194591,7.13347119770518));
#53536=CARTESIAN_POINT('Ctrl Pts',(4.87478836856172,-0.794772684001444,
7.13716136488657));
#53537=CARTESIAN_POINT('Ctrl Pts',(4.80781052390886,-0.63630980009567,7.11540215248782));
#53538=CARTESIAN_POINT('Ctrl Pts',(4.73811441601435,-0.319434907277396,
7.08494616615572));
#53539=CARTESIAN_POINT('Ctrl Pts',(4.69675812744069,-0.15833333333345,7.06011197857061));
#53540=CARTESIAN_POINT('Ctrl Pts',(4.69573759385705,0.158333333333452,7.02887605276384));
#53541=CARTESIAN_POINT('Ctrl Pts',(4.73607110158677,0.319434907277405,7.02152412363642));
#53542=CARTESIAN_POINT('Ctrl Pts',(4.80369303355971,0.636309800095679,6.99029024862042));
#53543=CARTESIAN_POINT('Ctrl Pts',(4.87008576851561,0.794772684001431,6.97854073298898));
#53544=CARTESIAN_POINT('Ctrl Pts',(4.92479332431127,1.06847604194745,6.928592729483));
#53545=CARTESIAN_POINT('Ctrl Pts',(4.94094715647548,1.1851427086157,6.90133988204735));
#53546=CARTESIAN_POINT('Ctrl Pts',(4.9495739470145,1.30000000000547,6.86845482713801));
#53547=CARTESIAN_POINT('Ctrl Pts',(4.96284649527735,-1.30000000000097,7.1077561478983));
#53548=CARTESIAN_POINT('Ctrl Pts',(4.95304069625497,-1.18514270861267,7.12582630027899));
#53549=CARTESIAN_POINT('Ctrl Pts',(4.93584495681872,-1.06847604194592,7.13571277356245));
#53550=CARTESIAN_POINT('Ctrl Pts',(4.87904711801652,-0.794772684001446,
7.13964656877545));
#53551=CARTESIAN_POINT('Ctrl Pts',(4.81202080450033,-0.636309800095671,
7.11754979988703));
#53552=CARTESIAN_POINT('Ctrl Pts',(4.74237295771725,-0.319434907277396,
7.0869326009472));
#53553=CARTESIAN_POINT('Ctrl Pts',(4.70083792287829,-0.15833333333345,7.06201365483902));
#53554=CARTESIAN_POINT('Ctrl Pts',(4.69983004401309,0.158333333333452,7.03069623555303));
#53555=CARTESIAN_POINT('Ctrl Pts',(4.74034847566072,0.319434907277405,7.02337647020484));
#53556=CARTESIAN_POINT('Ctrl Pts',(4.80796111658925,0.636309800095681,6.99207894680393));
#53557=CARTESIAN_POINT('Ctrl Pts',(4.87446055457127,0.794772684001433,6.98034563087335));
#53558=CARTESIAN_POINT('Ctrl Pts',(4.92858340434634,1.06847604194745,6.93015259185655));
#53559=CARTESIAN_POINT('Ctrl Pts',(4.94433555464321,1.18514270861571,6.9027428538463));
#53560=CARTESIAN_POINT('Ctrl Pts',(4.95241207901841,1.30000000000547,6.86965008458096));
#53561=CARTESIAN_POINT('Ctrl Pts',(4.96629038502904,-1.30000000000098,7.10979928916033));
#53562=CARTESIAN_POINT('Ctrl Pts',(4.95713670065089,-1.18514270861268,7.12835135544506));
#53563=CARTESIAN_POINT('Ctrl Pts',(4.94042605295921,-1.06847604194592,7.13854596531376));
#53564=CARTESIAN_POINT('Ctrl Pts',(4.88436301681819,-0.794772684001452,
7.14279015731071));
#53565=CARTESIAN_POINT('Ctrl Pts',(4.81727907004437,-0.636309800095676,
7.12025291182898));
#53566=CARTESIAN_POINT('Ctrl Pts',(4.74769202939327,-0.319434907277399,
7.08943460009879));
#53567=CARTESIAN_POINT('Ctrl Pts',(4.70593253920081,-0.158333333333452,
7.06442226739939));
#53568=CARTESIAN_POINT('Ctrl Pts',(4.70494017607543,0.158333333333454,7.0330076981234));
#53569=CARTESIAN_POINT('Ctrl Pts',(4.74568956954566,0.319434907277408,7.02572793492377));
#53570=CARTESIAN_POINT('Ctrl Pts',(4.81329136002281,0.636309800095685,6.99434448950996));
#53571=CARTESIAN_POINT('Ctrl Pts',(4.87992526190969,0.794772684001439,6.98262174097569));
#53572=CARTESIAN_POINT('Ctrl Pts',(4.93331876013669,1.06847604194746,6.93211213018218));
#53573=CARTESIAN_POINT('Ctrl Pts',(4.94856952183904,1.18514270861572,6.90450207555735));
#53574=CARTESIAN_POINT('Ctrl Pts',(4.95595897828523,1.30000000000548,6.87114570525484));
#53575=CARTESIAN_POINT('Ctrl Pts',(4.97042752796124,-1.30000000000099,7.11222067280422));
#53576=CARTESIAN_POINT('Ctrl Pts',(4.96206120246261,-1.18514270861269,7.13132279160153));
#53577=CARTESIAN_POINT('Ctrl Pts',(4.94593429676918,-1.06847604194593,7.14187758047346));
#53578=CARTESIAN_POINT('Ctrl Pts',(4.89074942569216,-0.794772684001456,
7.14651521223085));
#53579=CARTESIAN_POINT('Ctrl Pts',(4.82357707335456,-0.63630980009568,7.1235618642295));
#53580=CARTESIAN_POINT('Ctrl Pts',(4.75406052371135,-0.319434907277401,
7.09251675749891));
#53581=CARTESIAN_POINT('Ctrl Pts',(4.71204634504394,-0.158333333333453,
7.06730418522112));
#53582=CARTESIAN_POINT('Ctrl Pts',(4.71107332656958,0.158333333333454,7.03577415975341));
#53583=CARTESIAN_POINT('Ctrl Pts',(4.75209106551394,0.319434907277409,7.02860172769455));
#53584=CARTESIAN_POINT('Ctrl Pts',(4.81967335398172,0.636309800095689,6.99716397318012));
#53585=CARTESIAN_POINT('Ctrl Pts',(4.88646202340049,0.794772684001444,6.98550864356446));
#53586=CARTESIAN_POINT('Ctrl Pts',(4.93898422941487,1.06847604194747,6.93458752317071));
#53587=CARTESIAN_POINT('Ctrl Pts',(4.95363781148886,1.18514270861572,6.90670098220033));
#53588=CARTESIAN_POINT('Ctrl Pts',(4.96021005879261,1.30000000000549,6.87296976646473));
#53589=CARTESIAN_POINT('Ctrl Pts',(4.97388248677194,-1.300000000001,7.11419330698134));
#53590=CARTESIAN_POINT('Ctrl Pts',(4.96618059363683,-1.1851427086127,7.13370484739741));
#53591=CARTESIAN_POINT('Ctrl Pts',(4.95054344986816,-1.06847604194594,7.1445400528125));
#53592=CARTESIAN_POINT('Ctrl Pts',(4.89608650315763,-0.794772684001463,
7.14952747534969));
#53593=CARTESIAN_POINT('Ctrl Pts',(4.82881225868493,-0.636309800095686,
7.12639344125074));
#53594=CARTESIAN_POINT('Ctrl Pts',(4.75935076571616,-0.319434907277404,
7.09517759987284));
#53595=CARTESIAN_POINT('Ctrl Pts',(4.71714499090967,-0.158333333333454,
7.06966810286072));
#53596=CARTESIAN_POINT('Ctrl Pts',(4.71618917228211,0.158333333333456,7.03804039880248));
#53597=CARTESIAN_POINT('Ctrl Pts',(4.75741862739402,0.319434907277412,7.03103876207293));
#53598=CARTESIAN_POINT('Ctrl Pts',(4.82497494583709,0.636309800095695,6.99963073021055));
#53599=CARTESIAN_POINT('Ctrl Pts',(4.89188220977964,0.794772684001451,6.98811958001273));
#53600=CARTESIAN_POINT('Ctrl Pts',(4.94368264879308,1.06847604194748,6.93682171039539));
#53601=CARTESIAN_POINT('Ctrl Pts',(4.95784437193867,1.18514270861573,6.9086581737759));
#53602=CARTESIAN_POINT('Ctrl Pts',(4.96374532757619,1.3000000000055,6.87453604752103));
#53603=CARTESIAN_POINT('Ctrl Pts',(4.97630421138477,-1.300000000001,7.11555377724202));
#53604=CARTESIAN_POINT('Ctrl Pts',(4.96907109514182,-1.1851427086127,7.13533017872965));
#53605=CARTESIAN_POINT('Ctrl Pts',(4.95377823876846,-1.06847604194594,7.1463530476813));
#53606=CARTESIAN_POINT('Ctrl Pts',(4.89982906917387,-0.794772684001465,
7.15159566878068));
#53607=CARTESIAN_POINT('Ctrl Pts',(4.83247110010632,-0.636309800095687,
7.12840880700605));
#53608=CARTESIAN_POINT('Ctrl Pts',(4.76304610150664,-0.319434907277404,
7.09708440442982));
#53609=CARTESIAN_POINT('Ctrl Pts',(4.72071445783629,-0.158333333333454,
7.0713148078593));
#53610=CARTESIAN_POINT('Ctrl Pts',(4.71977122477105,0.158333333333456,7.03961757193506));
#53611=CARTESIAN_POINT('Ctrl Pts',(4.76114467462826,0.319434907277413,7.03276470241732));
#53612=CARTESIAN_POINT('Ctrl Pts',(4.82867884935533,0.636309800095696,7.0014087449179));
#53613=CARTESIAN_POINT('Ctrl Pts',(4.89566416734629,0.794772684001452,6.9900399194674));
#53614=CARTESIAN_POINT('Ctrl Pts',(4.94696107898536,1.06847604194748,6.93846538579834));
#53615=CARTESIAN_POINT('Ctrl Pts',(4.96078097285189,1.18514270861574,6.91008837141033));
#53616=CARTESIAN_POINT('Ctrl Pts',(4.96621622827414,1.3000000000055,6.87565904723499));
#53617=CARTESIAN_POINT('Ctrl Pts',(4.97751550866759,-1.30000000000101,7.11623101982547));
#53618=CARTESIAN_POINT('Ctrl Pts',(4.97051729691734,-1.1851427086127,7.13613666114551));
#53619=CARTESIAN_POINT('Ctrl Pts',(4.95539676594355,-1.06847604194594,7.14725219990602));
#53620=CARTESIAN_POINT('Ctrl Pts',(4.90170113227145,-0.794772684001466,
7.15262442273227));
#53621=CARTESIAN_POINT('Ctrl Pts',(4.83429936465745,-0.636309800095687,
7.1294227924869));
#53622=CARTESIAN_POINT('Ctrl Pts',(4.764892248713,-0.319434907277404,7.09804621852923));
#53623=CARTESIAN_POINT('Ctrl Pts',(4.72249891275604,-0.158333333333454,
7.07213879181453));
#53624=CARTESIAN_POINT('Ctrl Pts',(4.72156205558291,0.158333333333456,7.04040671329765));
#53625=CARTESIAN_POINT('Ctrl Pts',(4.7630068896913,0.319434907277413,7.03363250408665));
#53626=CARTESIAN_POINT('Ctrl Pts',(4.83052941439548,0.636309800095697,7.00230729896226));
#53627=CARTESIAN_POINT('Ctrl Pts',(4.89755300497442,0.794772684001453,6.99101596247396));
#53628=CARTESIAN_POINT('Ctrl Pts',(4.94859845261492,1.06847604194748,6.93930114815657));
#53629=CARTESIAN_POINT('Ctrl Pts',(4.96224783122096,1.18514270861574,6.91081442761733));
#53630=CARTESIAN_POINT('Ctrl Pts',(4.96745090556956,1.3000000000055,6.87622641343428));
#53631=CARTESIAN_POINT('Ctrl Pts',(4.97812123381433,-1.30000000000101,7.1165690665992));
#53632=CARTESIAN_POINT('Ctrl Pts',(4.9712405789915,-1.1851427086127,7.13653863761121));
#53633=CARTESIAN_POINT('Ctrl Pts',(4.95620624288918,-1.06847604194594,7.14770027504741));
#53634=CARTESIAN_POINT('Ctrl Pts',(4.90263728399023,-0.794772684001466,
7.15313780182181));
#53635=CARTESIAN_POINT('Ctrl Pts',(4.83521322869637,-0.636309800095687,
7.12993111711226));
#53636=CARTESIAN_POINT('Ctrl Pts',(4.76581487589349,-0.319434907277404,
7.09852959461544));
#53637=CARTESIAN_POINT('Ctrl Pts',(4.72339074516187,-0.158333333333454,
7.07255305525712));
#53638=CARTESIAN_POINT('Ctrl Pts',(4.72245710661183,0.158333333333456,7.04080347291612));
#53639=CARTESIAN_POINT('Ctrl Pts',(4.76393775562899,0.319434907277413,7.03406779705712));
#53640=CARTESIAN_POINT('Ctrl Pts',(4.83145440374682,0.636309800095696,7.00275852022833));
#53641=CARTESIAN_POINT('Ctrl Pts',(4.89849685066599,0.794772684001453,6.99150802023193));
#53642=CARTESIAN_POINT('Ctrl Pts',(4.94941660947784,1.06847604194748,6.93972298463305));
#53643=CARTESIAN_POINT('Ctrl Pts',(4.96298081810854,1.18514270861574,6.91118089734209));
#53644=CARTESIAN_POINT('Ctrl Pts',(4.96806795854315,1.3000000000055,6.8765125458464));
#53645=CARTESIAN_POINT('Ctrl Pts',(4.97846737342916,-1.30000000000101,7.1167621372107));
#53646=CARTESIAN_POINT('Ctrl Pts',(4.97165389322874,-1.1851427086127,7.13676826564106));
#53647=CARTESIAN_POINT('Ctrl Pts',(4.95666881041786,-1.06847604194594,7.14795626906208));
#53648=CARTESIAN_POINT('Ctrl Pts',(4.9031722346155,-0.794772684001466,7.1534311622856));
#53649=CARTESIAN_POINT('Ctrl Pts',(4.83573539246057,-0.636309800095688,
7.13022194721542));
#53650=CARTESIAN_POINT('Ctrl Pts',(4.76634214031379,-0.319434907277405,
7.09880555346919));
#53651=CARTESIAN_POINT('Ctrl Pts',(4.72390064694252,-0.158333333333454,
7.07278793416587));
#53652=CARTESIAN_POINT('Ctrl Pts',(4.72296883574537,0.158333333333456,7.04102843310387));
#53653=CARTESIAN_POINT('Ctrl Pts',(4.76446968198849,0.319434907277413,7.03431659521749));
#53654=CARTESIAN_POINT('Ctrl Pts',(4.83198289997454,0.636309800095697,7.00301690285337));
#53655=CARTESIAN_POINT('Ctrl Pts',(4.89903625057841,0.794772684001453,6.99178893957758));
#53656=CARTESIAN_POINT('Ctrl Pts',(4.94988421697014,1.06847604194748,6.93996342244769));
#53657=CARTESIAN_POINT('Ctrl Pts',(4.96339975863266,1.18514270861574,6.91138957243487));
#53658=CARTESIAN_POINT('Ctrl Pts',(4.9684206414094,1.3000000000055,6.87667521845023));
#53659=CARTESIAN_POINT('Ctrl Pts',(4.98971731443253,-1.30000000000093,7.12303343632508));
#53660=CARTESIAN_POINT('Ctrl Pts',(4.98508891455217,-1.18514270861263,7.14421273284097));
#53661=CARTESIAN_POINT('Ctrl Pts',(4.97170506847732,-1.06847604194588,7.15625196709077));
#53662=CARTESIAN_POINT('Ctrl Pts',(4.92055887438486,-0.794772684001422,
7.16294963435057));
#53663=CARTESIAN_POINT('Ctrl Pts',(4.85270237754255,-0.636309800095653,
7.13967947678175));
#53664=CARTESIAN_POINT('Ctrl Pts',(4.78346413868162,-0.319434907277387,
7.10785049809407));
#53665=CARTESIAN_POINT('Ctrl Pts',(4.74044174664496,-0.158333333333446,
7.08061369858619));
#53666=CARTESIAN_POINT('Ctrl Pts',(4.73957082539452,0.158333333333448,7.04852441713683));
#53667=CARTESIAN_POINT('Ctrl Pts',(4.78175076018467,0.319434907277395,7.04243439289715));
#53668=CARTESIAN_POINT('Ctrl Pts',(4.84915701604034,0.636309800095661,7.01142060033288));
#53669=CARTESIAN_POINT('Ctrl Pts',(4.91654958673662,0.794772684001409,7.00102617359138));
#53670=CARTESIAN_POINT('Ctrl Pts',(4.96506311114736,1.06847604194742,6.94791011372403));
#53671=CARTESIAN_POINT('Ctrl Pts',(4.97699869546298,1.18514270861567,6.91830327291942));
#53672=CARTESIAN_POINT('Ctrl Pts',(4.97987015697993,1.30000000000543,6.88208156548295));
#53673=CARTESIAN_POINT('Ctrl Pts',(5.01178389861922,-1.3000000000005,7.13627644036779));
#53674=CARTESIAN_POINT('Ctrl Pts',(5.01131141371871,-1.18514270861224,7.16062282534453));
#53675=CARTESIAN_POINT('Ctrl Pts',(5.00100904105187,-1.06847604194552,7.17476947647352));
#53676=CARTESIAN_POINT('Ctrl Pts',(4.9544994920063,-0.794772684001155,7.18388764497125));
#53677=CARTESIAN_POINT('Ctrl Pts',(4.88616940395213,-0.636309800095441,
7.15851802196042));
#53678=CARTESIAN_POINT('Ctrl Pts',(4.81732321849579,-0.319434907277282,
7.12548645290095));
#53679=CARTESIAN_POINT('Ctrl Pts',(4.77299709493401,-0.158333333333393,
7.09689357667308));
#53680=CARTESIAN_POINT('Ctrl Pts',(4.77223561752897,0.158333333333395,7.06422913948137));
#53681=CARTESIAN_POINT('Ctrl Pts',(4.81577330570672,0.319434907277287,7.05922075284174));
#53682=CARTESIAN_POINT('Ctrl Pts',(4.88312332797933,0.636309800095447,7.02762546170713));
#53683=CARTESIAN_POINT('Ctrl Pts',(4.95151460519703,0.794772684001146,7.01634068080159));
#53684=CARTESIAN_POINT('Ctrl Pts',(4.99538366475049,1.06847604194707,6.96116272290421));
#53685=CARTESIAN_POINT('Ctrl Pts',(5.00409750598239,1.18514270861528,6.93043959360876));
#53686=CARTESIAN_POINT('Ctrl Pts',(5.00253589807423,1.300000000005,6.89287782844697));
#53687=CARTESIAN_POINT('Ctrl Pts',(5.03373827646428,-1.3,7.14940561675095));
#53688=CARTESIAN_POINT('Ctrl Pts',(5.03743514540704,-1.18514270861178,7.17662169039555));
#53689=CARTESIAN_POINT('Ctrl Pts',(5.03020931803737,-1.06847604194511,7.19274767803129));
#53690=CARTESIAN_POINT('Ctrl Pts',(4.98828259773197,-0.794772684000847,
7.20438161821808));
#53691=CARTESIAN_POINT('Ctrl Pts',(4.91934781307154,-0.636309800095196,
7.17772787593842));
#53692=CARTESIAN_POINT('Ctrl Pts',(4.85084550516311,-0.319434907277159,
7.14381723154251));
#53693=CARTESIAN_POINT('Ctrl Pts',(4.80525449214962,-0.158333333333332,
7.11377207003864));
#53694=CARTESIAN_POINT('Ctrl Pts',(4.80463957298797,0.158333333333334,7.08035575294124));
#53695=CARTESIAN_POINT('Ctrl Pts',(4.84964913467179,0.319434907277167,7.07559389246093));
#53696=CARTESIAN_POINT('Ctrl Pts',(4.91683072495962,0.636309800095206,7.04427067070441));
#53697=CARTESIAN_POINT('Ctrl Pts',(4.98579503969525,0.794772684000841,7.03523465559988));
#53698=CARTESIAN_POINT('Ctrl Pts',(5.02510837557537,1.06847604194666,6.97733180991118));
#53699=CARTESIAN_POINT('Ctrl Pts',(5.03075217902059,1.18514270861482,6.94436545494296));
#53700=CARTESIAN_POINT('Ctrl Pts',(5.02502249951107,1.3000000000045,6.90349674139346));
#53701=CARTESIAN_POINT('Ctrl Pts',(5.0446386636865,-1.3,7.15639922225603));
#53702=CARTESIAN_POINT('Ctrl Pts',(5.05044042294362,-1.18514270861178,7.18489122215592));
#53703=CARTESIAN_POINT('Ctrl Pts',(5.04476129211945,-1.06847604194512,7.20192692863061));
#53704=CARTESIAN_POINT('Ctrl Pts',(5.0051182109774,-0.794772684000851,7.21481648893273));
#53705=CARTESIAN_POINT('Ctrl Pts',(4.93580560547694,-0.636309800095197,
7.18795105230746));
#53706=CARTESIAN_POINT('Ctrl Pts',(4.86748690268215,-0.319434907277159,
7.15354929193199));
#53707=CARTESIAN_POINT('Ctrl Pts',(4.82135018302871,-0.158333333333332,
7.12232171799169));
#53708=CARTESIAN_POINT('Ctrl Pts',(4.82082865786803,0.158333333333334,7.08844490884846));
#53709=CARTESIAN_POINT('Ctrl Pts',(4.86650233516518,0.319434907277167,7.08425772830895));
#53710=CARTESIAN_POINT('Ctrl Pts',(4.93363960349709,0.636309800095206,7.05278755158574));
#53711=CARTESIAN_POINT('Ctrl Pts',(5.00304362126358,0.79477268400084,7.04374488751153));
#53712=CARTESIAN_POINT('Ctrl Pts',(5.04007197138552,1.06847604194666,6.98466339093232));
#53713=CARTESIAN_POINT('Ctrl Pts',(5.0441424144131,1.18514270861482,6.95094305803163));
#53714=CARTESIAN_POINT('Ctrl Pts',(5.03625509973595,1.3000000000045,6.90907658291435));
#53715=CARTESIAN_POINT('',(4.94063912830279,1.2,6.89572216005206));
#53716=CARTESIAN_POINT('Ctrl Pts',(4.94063912830279,1.2,6.89572216005206));
#53717=CARTESIAN_POINT('Ctrl Pts',(4.92390473453183,1.21597616111059,6.88390203159158));
#53718=CARTESIAN_POINT('Ctrl Pts',(4.90745111372174,1.23156175617616,6.87117277576754));
#53719=CARTESIAN_POINT('Ctrl Pts',(4.87600876742023,1.261382346883,6.84892960913813));
#53720=CARTESIAN_POINT('Ctrl Pts',(4.84864612923132,1.28723399810768,6.82956657428991));
#53721=CARTESIAN_POINT('Ctrl Pts',(4.83514898734333,1.30000000000497,6.82074511190421));
#53722=CARTESIAN_POINT('',(4.94779107629418,0.653834841369961,7.05213700604833));
#53723=CARTESIAN_POINT('Ctrl Pts',(4.94779107633072,0.653834841368704,7.05213700604228));
#53724=CARTESIAN_POINT('Ctrl Pts',(4.94730914812078,0.717423550067115,7.03601072567456));
#53725=CARTESIAN_POINT('Ctrl Pts',(4.9468618942627,0.763685300918966,7.02296808068869));
#53726=CARTESIAN_POINT('Ctrl Pts',(4.94482981071674,0.949868242106328,6.9711151806119));
#53727=CARTESIAN_POINT('Ctrl Pts',(4.94322281841657,1.06483235008049,6.93767421437741));
#53728=CARTESIAN_POINT('Ctrl Pts',(4.9406391283028,1.2,6.89572216005206));
#53729=CARTESIAN_POINT('',(4.94999291725008,-0.653834841531101,7.19162628075221));
#53730=CARTESIAN_POINT('Ctrl Pts',(4.94999291725008,-0.6538348415311,7.1916262807522));
#53731=CARTESIAN_POINT('Ctrl Pts',(4.91226053268323,-0.57598825529314,7.17418301909822));
#53732=CARTESIAN_POINT('Ctrl Pts',(4.88066779187612,-0.493638204898488,
7.15874635405016));
#53733=CARTESIAN_POINT('Ctrl Pts',(4.83632237990281,-0.338136439546806,
7.13434742800906));
#53734=CARTESIAN_POINT('Ctrl Pts',(4.82127841502355,-0.265661862329625,
7.12466561743286));
#53735=CARTESIAN_POINT('Ctrl Pts',(4.80341669336683,-0.129718290004032,
7.10807972575262));
#53736=CARTESIAN_POINT('Ctrl Pts',(4.79913211996351,-0.0666263115009711,
7.10100067551947));
#53737=CARTESIAN_POINT('Ctrl Pts',(4.79855022586424,0.0595444515987862,
7.0876845625097));
#53738=CARTESIAN_POINT('Ctrl Pts',(4.80223154791772,0.122778289585405,7.08135019967731));
#53739=CARTESIAN_POINT('Ctrl Pts',(4.81904908132387,0.260130845872543,7.06921455582952));
#53740=CARTESIAN_POINT('Ctrl Pts',(4.83379007158933,0.333945959033105,7.06371918300369));
#53741=CARTESIAN_POINT('Ctrl Pts',(4.87782753950601,0.491210667319418,7.05522657143219));
#53742=CARTESIAN_POINT('Ctrl Pts',(4.90929426434707,0.574355066564918,7.05261167566303));
#53743=CARTESIAN_POINT('Ctrl Pts',(4.94779107625945,0.653834841386506,7.05213700600196));
#53744=CARTESIAN_POINT('',(4.94934486610223,-1.2,7.11946804120388));
#53745=CARTESIAN_POINT('Ctrl Pts',(4.94934486610223,-1.2,7.11946804120388));
#53746=CARTESIAN_POINT('Ctrl Pts',(4.94954877297065,-1.13394982025349,7.13199977925508));
#53747=CARTESIAN_POINT('Ctrl Pts',(4.9497650894168,-1.03818575991279,7.14834426936692));
#53748=CARTESIAN_POINT('Ctrl Pts',(4.94997573806144,-0.796404165621293,
7.17980499094405));
#53749=CARTESIAN_POINT('Ctrl Pts',(4.94998207838412,-0.739512578337757,
7.18521905498287));
#53750=CARTESIAN_POINT('Ctrl Pts',(4.94999291725008,-0.653834841531101,
7.1916262807522));
#53751=CARTESIAN_POINT('Ctrl Pts',(4.84757809483801,-1.3,7.04674656791213));
#53752=CARTESIAN_POINT('Ctrl Pts',(4.86730712653357,-1.28070206600169,7.06007770157836));
#53753=CARTESIAN_POINT('Ctrl Pts',(4.88299831626126,-1.26532349056323,7.07130878936968));
#53754=CARTESIAN_POINT('Ctrl Pts',(4.92478995175362,-1.224253828607,7.10129971725897));
#53755=CARTESIAN_POINT('Ctrl Pts',(4.92948688426405,-1.21960121810543,7.10384727574809));
#53756=CARTESIAN_POINT('Ctrl Pts',(4.94934486610223,-1.2,7.11946804120388));
#53757=CARTESIAN_POINT('Origin',(0.,1.25,7.2));
#53758=CARTESIAN_POINT('Origin',(0.,1.2,7.2));
#53759=CARTESIAN_POINT('Origin',(0.,0.92691742076555,7.2));
#53760=CARTESIAN_POINT('Origin',(0.,0.653834841531101,7.2));
#53761=CARTESIAN_POINT('Origin',(0.,0.,7.2));
#53762=CARTESIAN_POINT('Origin',(0.,-0.653834841531101,7.2));
#53763=CARTESIAN_POINT('Origin',(0.,-0.926917420765551,7.2));
#53764=CARTESIAN_POINT('Origin',(0.,-1.2,7.2));
#53765=CARTESIAN_POINT('Origin',(0.,-1.25,7.2));
#53766=CARTESIAN_POINT('Ctrl Pts',(5.03625509974048,-1.30000000000004,7.49092341708498));
#53767=CARTESIAN_POINT('Ctrl Pts',(5.04414241441886,-1.18514270861181,7.44905694196869));
#53768=CARTESIAN_POINT('Ctrl Pts',(5.04007197139197,-1.06847604194513,7.41533660906868));
#53769=CARTESIAN_POINT('Ctrl Pts',(5.00304362127007,-0.794772684000851,
7.35625511248991));
#53770=CARTESIAN_POINT('Ctrl Pts',(4.93363960349964,-0.636309800095197,
7.34721244841535));
#53771=CARTESIAN_POINT('Ctrl Pts',(4.86650233516645,-0.319434907277159,
7.31574227169205));
#53772=CARTESIAN_POINT('Ctrl Pts',(4.82082865787052,-0.158333333333332,
7.31155509115263));
#53773=CARTESIAN_POINT('Ctrl Pts',(4.82135018303129,0.158333333333334,7.27767828200944));
#53774=CARTESIAN_POINT('Ctrl Pts',(4.86748690268524,0.319434907277167,7.24645070806922));
#53775=CARTESIAN_POINT('Ctrl Pts',(4.93580560547818,0.636309800095206,7.21204894769365));
#53776=CARTESIAN_POINT('Ctrl Pts',(5.00511821097388,0.79477268400084,7.18518351106812));
#53777=CARTESIAN_POINT('Ctrl Pts',(5.04476129211656,1.06847604194523,7.19807307137016));
#53778=CARTESIAN_POINT('Ctrl Pts',(5.05044042294223,1.18514270861202,7.21510877784489));
#53779=CARTESIAN_POINT('Ctrl Pts',(5.04463866368783,1.30000000000036,7.24360077774488));
#53780=CARTESIAN_POINT('Ctrl Pts',(5.0250224995653,-1.30000000000004,7.49650325861012));
#53781=CARTESIAN_POINT('Ctrl Pts',(5.03075217910044,-1.18514270861181,7.45563454506349));
#53782=CARTESIAN_POINT('Ctrl Pts',(5.02510837566901,-1.06847604194513,7.42266819009693));
#53783=CARTESIAN_POINT('Ctrl Pts',(4.98579503979313,-0.794772684000851,
7.36476534440886));
#53784=CARTESIAN_POINT('Ctrl Pts',(4.9168307250082,-0.636309800095197,7.35572932930014));
#53785=CARTESIAN_POINT('Ctrl Pts',(4.84964913470353,-0.319434907277159,
7.32440610754237));
#53786=CARTESIAN_POINT('Ctrl Pts',(4.80463957303099,-0.158333333333332,
7.31964424706344));
#53787=CARTESIAN_POINT('Ctrl Pts',(4.80525449219255,0.158333333333334,7.286227929966));
#53788=CARTESIAN_POINT('Ctrl Pts',(4.85084550521323,0.319434907277167,7.25618276846203));
#53789=CARTESIAN_POINT('Ctrl Pts',(4.91934781310058,0.636309800095206,7.22227212406456));
#53790=CARTESIAN_POINT('Ctrl Pts',(4.98828259770888,0.794772684000842,7.19561838178182));
#53791=CARTESIAN_POINT('Ctrl Pts',(5.03020931801556,1.06847604194523,7.20725232196856));
#53792=CARTESIAN_POINT('Ctrl Pts',(5.03743514539826,1.18514270861202,7.22337830960505));
#53793=CARTESIAN_POINT('Ctrl Pts',(5.03373827648099,1.30000000000036,7.25059438325115));
#53794=CARTESIAN_POINT('Ctrl Pts',(5.00253629492169,-1.30000000000007,7.5071180066086));
#53795=CARTESIAN_POINT('Ctrl Pts',(5.0041000765162,-1.18514270861184,7.46957409453477));
#53796=CARTESIAN_POINT('Ctrl Pts',(4.99538754505344,-1.06847604194516,7.43886314014003));
#53797=CARTESIAN_POINT('Ctrl Pts',(4.95151951550678,-0.79477268400087,7.38370019095));
#53798=CARTESIAN_POINT('Ctrl Pts',(4.88312596255923,-0.636309800095213,
7.37241107226535));
#53799=CARTESIAN_POINT('Ctrl Pts',(4.81577396602792,-0.319434907277168,
7.34080030142118));
#53800=CARTESIAN_POINT('Ctrl Pts',(4.77223465376658,-0.158333333333336,
7.33576655937609));
#53801=CARTESIAN_POINT('Ctrl Pts',(4.77299491001348,0.158333333333338,7.30308535487117));
#53802=CARTESIAN_POINT('Ctrl Pts',(4.81731919591816,0.319434907277172,7.27447936700617));
#53803=CARTESIAN_POINT('Ctrl Pts',(4.8861694321273,0.63630980009522,7.2414733246328));
#53804=CARTESIAN_POINT('Ctrl Pts',(4.95451014435092,0.794772684000861,7.21617408048259));
#53805=CARTESIAN_POINT('Ctrl Pts',(5.00102041438665,1.06847604194526,7.22530225004274));
#53806=CARTESIAN_POINT('Ctrl Pts',(5.01132079453024,1.18514270861205,7.23943924357551));
#53807=CARTESIAN_POINT('Ctrl Pts',(5.01178898229432,1.30000000000039,7.26376198427049));
#53808=CARTESIAN_POINT('Ctrl Pts',(4.97960768346775,-1.30000000000009,7.5180473284774));
#53809=CARTESIAN_POINT('Ctrl Pts',(4.9766898729321,-1.18514270861186,7.48188505323422));
#53810=CARTESIAN_POINT('Ctrl Pts',(4.96471982623668,-1.06847604194517,7.45231951336133));
#53811=CARTESIAN_POINT('Ctrl Pts',(4.91615414734792,-0.794772684000884,
7.39925698006668));
#53812=CARTESIAN_POINT('Ctrl Pts',(4.84876618885557,-0.636309800095224,
7.3888440607498));
#53813=CARTESIAN_POINT('Ctrl Pts',(4.78135491398204,-0.319434907277172,
7.35780243811579));
#53814=CARTESIAN_POINT('Ctrl Pts',(4.73918890339539,-0.158333333333339,
7.35165944877986));
#53815=CARTESIAN_POINT('Ctrl Pts',(4.74005905500855,0.158333333333341,7.31954667302313));
#53816=CARTESIAN_POINT('Ctrl Pts',(4.78306310332938,0.31943490727718,7.29230286563965));
#53817=CARTESIAN_POINT('Ctrl Pts',(4.85231222804514,0.636309800095233,7.26052816522222));
#53818=CARTESIAN_POINT('Ctrl Pts',(4.92018013385201,0.794772684000875,7.23739729695367));
#53819=CARTESIAN_POINT('Ctrl Pts',(4.97138152451334,1.06847604194528,7.24408340050477));
#53820=CARTESIAN_POINT('Ctrl Pts',(4.98479812888538,1.18514270861207,7.25608266977393));
#53821=CARTESIAN_POINT('Ctrl Pts',(4.98946815281066,1.30000000000041,7.27718704182951));
#53822=CARTESIAN_POINT('Ctrl Pts',(4.96762951206948,-1.3000000000001,7.52369694152733));
#53823=CARTESIAN_POINT('Ctrl Pts',(4.96246471251451,-1.18514270861186,7.48912650638533));
#53824=CARTESIAN_POINT('Ctrl Pts',(4.94884267675674,-1.06847604194518,7.46065043105714));
#53825=CARTESIAN_POINT('Ctrl Pts',(4.8978351415846,-0.794772684000887,7.40894419077206));
#53826=CARTESIAN_POINT('Ctrl Pts',(4.83079936287769,-0.636309800095225,
7.39764041936882));
#53827=CARTESIAN_POINT('Ctrl Pts',(4.76327466385806,-0.319434907277173,
7.36628860048776));
#53828=CARTESIAN_POINT('Ctrl Pts',(4.72181854707695,-0.158333333333339,
7.35948896452109));
#53829=CARTESIAN_POINT('Ctrl Pts',(4.72275225828287,0.158333333333341,7.32771916071371));
#53830=CARTESIAN_POINT('Ctrl Pts',(4.76514949861775,0.319434907277181,7.30175698426488));
#53831=CARTESIAN_POINT('Ctrl Pts',(4.83456100171557,0.636309800095235,7.27041665039979));
#53832=CARTESIAN_POINT('Ctrl Pts',(4.90198920287092,0.794772684000876,7.2473480172949));
#53833=CARTESIAN_POINT('Ctrl Pts',(4.95564985032951,1.06847604194528,7.25275781317528));
#53834=CARTESIAN_POINT('Ctrl Pts',(4.9707419647311,1.18514270861207,7.26386848383299));
#53835=CARTESIAN_POINT('Ctrl Pts',(4.97769848757239,1.30000000000041,7.28374812496449));
#53836=CARTESIAN_POINT('Ctrl Pts',(4.96621805807752,-1.3000000000001,7.52434179038395));
#53837=CARTESIAN_POINT('Ctrl Pts',(4.96078772625744,-1.18514270861186,7.48995179094868));
#53838=CARTESIAN_POINT('Ctrl Pts',(4.94697072767715,-1.06847604194518,7.46160074156553));
#53839=CARTESIAN_POINT('Ctrl Pts',(4.89567581891261,-0.794772684000887,
7.41005532859067));
#53840=CARTESIAN_POINT('Ctrl Pts',(4.82868432317164,-0.636309800095225,
7.39866670011986));
#53841=CARTESIAN_POINT('Ctrl Pts',(4.76114622750612,-0.319434907277173,
7.36727937712788));
#53842=CARTESIAN_POINT('Ctrl Pts',(4.71977103742867,-0.158333333333339,
7.36038548847363));
#53843=CARTESIAN_POINT('Ctrl Pts',(4.7207120039862,0.158333333333341,7.32865541212252));
#53844=CARTESIAN_POINT('Ctrl Pts',(4.76303921752189,0.319434907277181,7.30285410419705));
#53845=CARTESIAN_POINT('Ctrl Pts',(4.83247147220263,0.636309800095235,7.2715754267178));
#53846=CARTESIAN_POINT('Ctrl Pts',(4.89984974091479,0.794772684000876,7.24852423454693));
#53847=CARTESIAN_POINT('Ctrl Pts',(4.95380019818296,1.06847604194528,7.25378609204053));
#53848=CARTESIAN_POINT('Ctrl Pts',(4.96908923651688,1.18514270861207,7.26479066039715));
#53849=CARTESIAN_POINT('Ctrl Pts',(4.97631415929477,1.30000000000041,7.28452213397244));
#53850=CARTESIAN_POINT('Ctrl Pts',(4.9637474723205,-1.3000000000001,7.52546764988381));
#53851=CARTESIAN_POINT('Ctrl Pts',(4.9578515887148,-1.18514270861186,7.49138561279624));
#53852=CARTESIAN_POINT('Ctrl Pts',(4.94369283991791,-1.06847604194518,7.46324840340755));
#53853=CARTESIAN_POINT('Ctrl Pts',(4.89189442617697,-0.794772684000887,
7.41197956213334));
#53854=CARTESIAN_POINT('Ctrl Pts',(4.82498061700849,-0.636309800095225,
7.40044630641422));
#53855=CARTESIAN_POINT('Ctrl Pts',(4.75742044765574,-0.319434907277173,
7.36900715748394));
#53856=CARTESIAN_POINT('Ctrl Pts',(4.71618974295627,-0.158333333333339,
7.36196748723083));
#53857=CARTESIAN_POINT('Ctrl Pts',(4.7171432438584,0.158333333333341,7.33030631010084));
#53858=CARTESIAN_POINT('Ctrl Pts',(4.75934399763486,0.319434907277181,7.30476100870489));
#53859=CARTESIAN_POINT('Ctrl Pts',(4.82881267223018,0.636309800095235,7.27359032242174));
#53860=CARTESIAN_POINT('Ctrl Pts',(4.89610772436469,0.794772684000877,7.25059534316193));
#53861=CARTESIAN_POINT('Ctrl Pts',(4.95056595954635,1.06847604194528,7.25560230833908));
#53862=CARTESIAN_POINT('Ctrl Pts',(4.96619919450976,1.18514270861207,7.26641881217423));
#53863=CARTESIAN_POINT('Ctrl Pts',(4.9738927123029,1.30000000000042,7.28588449014569));
#53864=CARTESIAN_POINT('Ctrl Pts',(4.95879774516821,-1.3000000000001,7.5276563571909));
#53865=CARTESIAN_POINT('Ctrl Pts',(4.95196211656313,-1.18514270861186,7.49412296198952));
#53866=CARTESIAN_POINT('Ctrl Pts',(4.93711477351148,-1.06847604194518,7.46637434836761));
#53867=CARTESIAN_POINT('Ctrl Pts',(4.88430577775183,-0.794772684000886,
7.41563350249997));
#53868=CARTESIAN_POINT('Ctrl Pts',(4.81755779821641,-0.636309800095225,
7.40389731948821));
#53869=CARTESIAN_POINT('Ctrl Pts',(4.74996087059343,-0.319434907277173,
7.37241417162736));
#53870=CARTESIAN_POINT('Ctrl Pts',(4.70902588150169,-0.158333333333339,
7.36513038159391));
#53871=CARTESIAN_POINT('Ctrl Pts',(4.71000378351542,0.158333333333341,7.3336081834644));
#53872=CARTESIAN_POINT('Ctrl Pts',(4.7519379321394,0.319434907277181,7.3084896567254));
#53873=CARTESIAN_POINT('Ctrl Pts',(4.82148347571844,0.636309800095234,7.27755709497504));
#53874=CARTESIAN_POINT('Ctrl Pts',(4.88863357496422,0.794772684000876,7.25480084860166));
#53875=CARTESIAN_POINT('Ctrl Pts',(4.94411080355287,1.06847604194528,7.25931676866177));
#53876=CARTESIAN_POINT('Ctrl Pts',(4.96043010760253,1.18514270861207,7.26974266752768));
#53877=CARTESIAN_POINT('Ctrl Pts',(4.96905467907973,1.30000000000041,7.28863969079682));
#53878=CARTESIAN_POINT('Ctrl Pts',(4.95170655585734,-1.30000000000009,7.53066301974529));
#53879=CARTESIAN_POINT('Ctrl Pts',(4.94349922945896,-1.18514270861186,7.49767213261703));
#53880=CARTESIAN_POINT('Ctrl Pts',(4.92765097558884,-1.06847604194517,7.47033625580933));
#53881=CARTESIAN_POINT('Ctrl Pts',(4.87338626769454,-0.794772684000885,
7.42024911698156));
#53882=CARTESIAN_POINT('Ctrl Pts',(4.80690758119547,-0.636309800095224,
7.408498441716));
#53883=CARTESIAN_POINT('Ctrl Pts',(4.73928911609014,-0.319434907277173,
7.37718751125002));
#53884=CARTESIAN_POINT('Ctrl Pts',(4.69881519121616,-0.158333333333339,
7.36981610804418));
#53885=CARTESIAN_POINT('Ctrl Pts',(4.69982263937953,0.158333333333341,7.33847081935012));
#53886=CARTESIAN_POINT('Ctrl Pts',(4.74130467688739,0.31943490727718,7.31350778961374));
#53887=CARTESIAN_POINT('Ctrl Pts',(4.81097388788422,0.636309800095233,7.28298543955834));
#53888=CARTESIAN_POINT('Ctrl Pts',(4.87801805469122,0.794772684000875,7.26117165117431));
#53889=CARTESIAN_POINT('Ctrl Pts',(4.93496342103356,1.06847604194528,7.26506331349464));
#53890=CARTESIAN_POINT('Ctrl Pts',(4.9522499344413,1.18514270861207,7.27485794428191));
#53891=CARTESIAN_POINT('Ctrl Pts',(4.96217342220097,1.30000000000041,7.29276264943828));
#53892=CARTESIAN_POINT('Ctrl Pts',(4.94318957929729,-1.30000000000009,7.53423305499234));
#53893=CARTESIAN_POINT('Ctrl Pts',(4.93332953624159,-1.18514270861186,7.50185198254238));
#53894=CARTESIAN_POINT('Ctrl Pts',(4.91627433805312,-1.06847604194517,7.47497318322297));
#53895=CARTESIAN_POINT('Ctrl Pts',(4.8602511706145,-0.794772684000885,7.42558913136725));
#53896=CARTESIAN_POINT('Ctrl Pts',(4.79408885098585,-0.636309800095225,
7.41376001035497));
#53897=CARTESIAN_POINT('Ctrl Pts',(4.72644038716081,-0.319434907277173,
7.38262462152606));
#53898=CARTESIAN_POINT('Ctrl Pts',(4.68652131684815,-0.158333333333339,
7.37515634458014));
#53899=CARTESIAN_POINT('Ctrl Pts',(4.68756990475403,0.158333333333341,7.34408617678325));
#53900=CARTESIAN_POINT('Ctrl Pts',(4.72852508143549,0.319434907277181,7.31945437181908));
#53901=CARTESIAN_POINT('Ctrl Pts',(4.79833486731633,0.636309800095234,7.28939992686437));
#53902=CARTESIAN_POINT('Ctrl Pts',(4.86521212340213,0.794772684000876,7.2684628347598));
#53903=CARTESIAN_POINT('Ctrl Pts',(4.92392569863787,1.06847604194528,7.27163090554263));
#53904=CARTESIAN_POINT('Ctrl Pts',(4.94238557203983,1.18514270861207,7.28073645836866));
#53905=CARTESIAN_POINT('Ctrl Pts',(4.95389038767657,1.30000000000041,7.29757622356745));
#53906=CARTESIAN_POINT('Ctrl Pts',(4.92622393725722,-1.30000000000009,7.54194881348275));
#53907=CARTESIAN_POINT('Ctrl Pts',(4.91314484487837,-1.18514270861185,7.51153479287278));
#53908=CARTESIAN_POINT('Ctrl Pts',(4.89372426348806,-1.06847604194517,7.48599119980892));
#53909=CARTESIAN_POINT('Ctrl Pts',(4.8342087271754,-0.794772684000883,7.43823205181034));
#53910=CARTESIAN_POINT('Ctrl Pts',(4.76857066695711,-0.636309800095222,
7.42528661629812));
#53911=CARTESIAN_POINT('Ctrl Pts',(4.70074680043619,-0.319434907277171,
7.39357266963));
#53912=CARTESIAN_POINT('Ctrl Pts',(4.66180971695086,-0.158333333333338,
7.38496016242235));
#53913=CARTESIAN_POINT('Ctrl Pts',(4.66292672045037,0.15833333333334,7.35430893144978));
#53914=CARTESIAN_POINT('Ctrl Pts',(4.70298799249483,0.319434907277179,7.33144843630135));
#53915=CARTESIAN_POINT('Ctrl Pts',(4.77307247926823,0.636309800095231,7.30240192157892));
#53916=CARTESIAN_POINT('Ctrl Pts',(4.83944016939201,0.794772684000872,7.28225470268924));
#53917=CARTESIAN_POINT('Ctrl Pts',(4.90168661026715,1.06847604194527,7.2839604412694));
#53918=CARTESIAN_POINT('Ctrl Pts',(4.92252564715923,1.18514270861206,7.29185791074353));
#53919=CARTESIAN_POINT('Ctrl Pts',(4.93725954314648,1.30000000000041,7.30691449866427));
#53920=CARTESIAN_POINT('Ctrl Pts',(4.90065660867547,-1.30000000000008,7.55262755751749));
#53921=CARTESIAN_POINT('Ctrl Pts',(4.88263466293015,-1.18514270861185,7.52418493048915));
#53922=CARTESIAN_POINT('Ctrl Pts',(4.85959630730382,-1.06847604194516,7.50006003157311));
#53923=CARTESIAN_POINT('Ctrl Pts',(4.79478418664526,-0.794772684000876,
7.45430150460558));
#53924=CARTESIAN_POINT('Ctrl Pts',(4.7300403503272,-0.636309800095217,7.44075615110194));
#53925=CARTESIAN_POINT('Ctrl Pts',(4.66206323450965,-0.319434907277169,
7.40908706908356));
#53926=CARTESIAN_POINT('Ctrl Pts',(4.62471215024605,-0.158333333333337,
7.39950084206595));
#53927=CARTESIAN_POINT('Ctrl Pts',(4.62599014559949,0.158333333333339,7.36997551533005));
#53928=CARTESIAN_POINT('Ctrl Pts',(4.66470153449349,0.319434907277176,7.34982371775994));
#53929=CARTESIAN_POINT('Ctrl Pts',(4.73511417675659,0.636309800095225,7.32178508532075));
#53930=CARTESIAN_POINT('Ctrl Pts',(4.80053155068804,0.794772684000865,7.30156262702942));
#53931=CARTESIAN_POINT('Ctrl Pts',(4.86806019542745,1.06847604194527,7.30088393315434));
#53932=CARTESIAN_POINT('Ctrl Pts',(4.89250121694453,1.18514270861206,7.30713907296468));
#53933=CARTESIAN_POINT('Ctrl Pts',(4.91215261185388,1.30000000000041,7.31994313401581));
#53934=CARTESIAN_POINT('Ctrl Pts',(4.86653286362622,-1.30000000000007,7.56699602339097));
#53935=CARTESIAN_POINT('Ctrl Pts',(4.84193012512882,-1.18514270861184,7.54156815072991));
#53936=CARTESIAN_POINT('Ctrl Pts',(4.81406891318095,-1.06847604194516,7.51951951330367));
#53937=CARTESIAN_POINT('Ctrl Pts',(4.74217621443908,-0.794772684000874,
7.47638945944037));
#53938=CARTESIAN_POINT('Ctrl Pts',(4.67856929883686,-0.63630980009521,7.46107138749974));
#53939=CARTESIAN_POINT('Ctrl Pts',(4.61036610444347,-0.319434907277163,
7.42924713609238));
#53940=CARTESIAN_POINT('Ctrl Pts',(4.57522062589997,-0.158333333333335,
7.41932126812144));
#53941=CARTESIAN_POINT('Ctrl Pts',(4.57656999719294,0.158333333333337,7.39040121976789));
#53942=CARTESIAN_POINT('Ctrl Pts',(4.61308700479027,0.319434907277172,7.37101508989296));
#53943=CARTESIAN_POINT('Ctrl Pts',(4.68399363758603,0.636309800095217,7.34472965801132));
#53944=CARTESIAN_POINT('Ctrl Pts',(4.74868416146106,0.794772684000855,7.32832235074326));
#53945=CARTESIAN_POINT('Ctrl Pts',(4.82339340706111,1.06847604194525,7.32530219441606));
#53946=CARTESIAN_POINT('Ctrl Pts',(4.85261650093078,1.18514270861204,7.32911395995992));
#53947=CARTESIAN_POINT('Ctrl Pts',(4.87872382450021,1.30000000000039,7.33804480481385));
#53948=CARTESIAN_POINT('Ctrl Pts',(4.8322831212685,-1.30000000000007,7.58030962560515));
#53949=CARTESIAN_POINT('Ctrl Pts',(4.80099763659862,-1.18514270861183,7.556825992742));
#53950=CARTESIAN_POINT('Ctrl Pts',(4.76824497763037,-1.06847604194515,7.53617635724849));
#53951=CARTESIAN_POINT('Ctrl Pts',(4.68919031713033,-0.794772684000866,
7.49501866917608));
#53952=CARTESIAN_POINT('Ctrl Pts',(4.62681181703605,-0.636309800095206,
7.4792780833236));
#53953=CARTESIAN_POINT('Ctrl Pts',(4.55835898630226,-0.319434907277162,
7.44716273305618));
#53954=CARTESIAN_POINT('Ctrl Pts',(4.52530841472525,-0.158333333333334,
7.4354970781266));
#53955=CARTESIAN_POINT('Ctrl Pts',(4.52677534967624,0.158333333333336,7.40763889322388));
#53956=CARTESIAN_POINT('Ctrl Pts',(4.56133568964948,0.319434907277171,7.39136145828312));
#53957=CARTESIAN_POINT('Ctrl Pts',(4.63268931261174,0.636309800095214,7.36690463706524));
#53958=CARTESIAN_POINT('Ctrl Pts',(4.69626304790192,0.794772684000848,7.35165672911438));
#53959=CARTESIAN_POINT('Ctrl Pts',(4.77817412582395,1.06847604194525,7.34637870177531));
#53960=CARTESIAN_POINT('Ctrl Pts',(4.81227352272635,1.18514270861204,7.34830992636712));
#53961=CARTESIAN_POINT('Ctrl Pts',(4.84501604600325,1.30000000000038,7.35445703801565));
#53962=CARTESIAN_POINT('Ctrl Pts',(4.80369703210636,-1.30000000000006,7.59113993557896));
#53963=CARTESIAN_POINT('Ctrl Pts',(4.76686780308405,-1.18514270861182,7.56989617465925));
#53964=CARTESIAN_POINT('Ctrl Pts',(4.73004535157928,-1.06847604194514,7.55067186892));
#53965=CARTESIAN_POINT('Ctrl Pts',(4.64499377971837,-0.79477268400086,7.51092522231064));
#53966=CARTESIAN_POINT('Ctrl Pts',(4.58352304285331,-0.636309800095202,
7.4929261169799));
#53967=CARTESIAN_POINT('Ctrl Pts',(4.51483597746967,-0.31943490727716,7.46015120183153));
#53968=CARTESIAN_POINT('Ctrl Pts',(4.48360461045807,-0.158333333333334,
7.44800193996648));
#53969=CARTESIAN_POINT('Ctrl Pts',(4.48516732851818,0.158333333333336,7.42127916339769));
#53970=CARTESIAN_POINT('Ctrl Pts',(4.51800961074064,0.319434907277173,7.40706991303503));
#53971=CARTESIAN_POINT('Ctrl Pts',(4.58978164616749,0.636309800095214,7.38467047618168));
#53972=CARTESIAN_POINT('Ctrl Pts',(4.65258624879034,0.794772684000844,7.37171976821259));
#53973=CARTESIAN_POINT('Ctrl Pts',(4.74054992968274,1.06847604194524,7.36491717020787));
#53974=CARTESIAN_POINT('Ctrl Pts',(4.77871036700213,1.18514270861203,7.3652032319829));
#53975=CARTESIAN_POINT('Ctrl Pts',(4.81695502355821,1.30000000000037,7.36871994814812));
#53976=CARTESIAN_POINT('Ctrl Pts',(4.78072070206189,-1.30000000000005,7.59826996426713));
#53977=CARTESIAN_POINT('Ctrl Pts',(4.73939596944773,-1.18514270861182,7.57810409291054));
#53978=CARTESIAN_POINT('Ctrl Pts',(4.69928638575355,-1.06847604194514,7.55968520884557));
#53979=CARTESIAN_POINT('Ctrl Pts',(4.60943246062009,-0.794772684000857,
7.52116979209764));
#53980=CARTESIAN_POINT('Ctrl Pts',(4.54882050012122,-0.6363098000952,7.50324893132566));
#53981=CARTESIAN_POINT('Ctrl Pts',(4.47997038535647,-0.319434907277159,
7.47030730395309));
#53982=CARTESIAN_POINT('Ctrl Pts',(4.45015536348438,-0.158333333333333,
7.45697243813239));
#53983=CARTESIAN_POINT('Ctrl Pts',(4.45172513689568,0.158333333333335,7.4305333745949));
#53984=CARTESIAN_POINT('Ctrl Pts',(4.48311660067188,0.319434907277171,7.41751656523236));
#53985=CARTESIAN_POINT('Ctrl Pts',(4.55515064760831,0.636309800095212,7.39642572006936));
#53986=CARTESIAN_POINT('Ctrl Pts',(4.6172815010005,0.794772684000843,7.38520208752937));
#53987=CARTESIAN_POINT('Ctrl Pts',(4.71013514431173,1.06847604194524,7.37760971985347));
#53988=CARTESIAN_POINT('Ctrl Pts',(4.75159422184822,1.18514270861203,7.3769152536041));
#53989=CARTESIAN_POINT('Ctrl Pts',(4.79431947529833,1.30000000000037,7.37881277574731));
#53990=CARTESIAN_POINT('Ctrl Pts',(4.76786499505706,-1.30000000000005,7.60368176740185));
#53991=CARTESIAN_POINT('Ctrl Pts',(4.72403017506114,-1.18514270861182,7.58434250585805));
#53992=CARTESIAN_POINT('Ctrl Pts',(4.68207593127194,-1.06847604194514,7.56639781277273));
#53993=CARTESIAN_POINT('Ctrl Pts',(4.58949774244669,-0.794772684000855,
7.52816371404363));
#53994=CARTESIAN_POINT('Ctrl Pts',(4.52928725147374,-0.636309800095199,
7.50909410570766));
#53995=CARTESIAN_POINT('Ctrl Pts',(4.46031010843157,-0.319434907277159,
7.47547069309426));
#53996=CARTESIAN_POINT('Ctrl Pts',(4.43129639052106,-0.158333333333333,
7.46149895232343));
#53997=CARTESIAN_POINT('Ctrl Pts',(4.43290065961814,0.158333333333335,7.43554361832388));
#53998=CARTESIAN_POINT('Ctrl Pts',(4.46353033253678,0.31943490727717,7.42390395304713));
#53999=CARTESIAN_POINT('Ctrl Pts',(4.5357514528591,0.63630980009521,7.40395766267498));
#54000=CARTESIAN_POINT('Ctrl Pts',(4.59753036765001,0.794772684000841,7.39381410651702));
#54001=CARTESIAN_POINT('Ctrl Pts',(4.69310019596524,1.06847604194524,7.38543317330055));
#54002=CARTESIAN_POINT('Ctrl Pts',(4.73638310392889,1.18514270861202,7.3839008144956));
#54003=CARTESIAN_POINT('Ctrl Pts',(4.78158028238967,1.30000000000037,7.38446389233092));
#54004=CARTESIAN_POINT('Ctrl Pts',(4.75923927618336,-1.30000000000005,7.60624853723847));
#54005=CARTESIAN_POINT('Ctrl Pts',(4.71371888822517,-1.18514270861182,7.58733968665901));
#54006=CARTESIAN_POINT('Ctrl Pts',(4.67053009679902,-1.06847604194514,7.56968470619033));
#54007=CARTESIAN_POINT('Ctrl Pts',(4.5761418031398,-0.794772684000856,7.53179486023267));
#54008=CARTESIAN_POINT('Ctrl Pts',(4.51623070437183,-0.636309800095199,
7.51239178373076));
#54009=CARTESIAN_POINT('Ctrl Pts',(4.44719492422517,-0.319434907277159,
7.47876712691051));
#54010=CARTESIAN_POINT('Ctrl Pts',(4.41874093581131,-0.158333333333333,
7.46481603696944));
#54011=CARTESIAN_POINT('Ctrl Pts',(4.42035217695484,0.158333333333335,7.43907172064773));
#54012=CARTESIAN_POINT('Ctrl Pts',(4.45042291996238,0.31943490727717,7.42764711885315));
#54013=CARTESIAN_POINT('Ctrl Pts',(4.52272945180426,0.63630980009521,7.40808159523841));
#54014=CARTESIAN_POINT('Ctrl Pts',(4.58422871234628,0.794772684000842,7.39842119779554));
#54015=CARTESIAN_POINT('Ctrl Pts',(4.68165701495636,1.06847604194524,7.38997292819499));
#54016=CARTESIAN_POINT('Ctrl Pts',(4.72619958205877,1.18514270861203,7.38826513261078));
#54017=CARTESIAN_POINT('Ctrl Pts',(4.77311161413808,1.30000000000037,7.38850648431319));
#54018=CARTESIAN_POINT('Ctrl Pts',(4.75348070600748,-1.30000000000005,7.60784584718064));
#54019=CARTESIAN_POINT('Ctrl Pts',(4.70683011197265,-1.18514270861182,7.58912773525085));
#54020=CARTESIAN_POINT('Ctrl Pts',(4.66281435287995,-1.06847604194514,7.5716076021723));
#54021=CARTESIAN_POINT('Ctrl Pts',(4.56721613986662,-0.794772684000856,
7.53390016067141));
#54022=CARTESIAN_POINT('Ctrl Pts',(4.50751187293003,-0.636309800095199,
7.51438143784491));
#54023=CARTESIAN_POINT('Ctrl Pts',(4.43844157285354,-0.319434907277159,
7.48082496512931));
#54024=CARTESIAN_POINT('Ctrl Pts',(4.41036344576932,-0.158333333333333,
7.46692564018267));
#54025=CARTESIAN_POINT('Ctrl Pts',(4.41198144907926,0.158333333333335,7.441363506674));
#54026=CARTESIAN_POINT('Ctrl Pts',(4.44167897603494,0.31943490727717,7.43008701444388));
#54027=CARTESIAN_POINT('Ctrl Pts',(4.51404218765837,0.63630980009521,7.41078836318461));
#54028=CARTESIAN_POINT('Ctrl Pts',(4.57535476318257,0.794772684000841,7.40145625908929));
#54029=CARTESIAN_POINT('Ctrl Pts',(4.67402065827908,1.06847604194524,7.39295150913252));
#54030=CARTESIAN_POINT('Ctrl Pts',(4.71940216420826,1.18514270861202,7.39111669715767));
#54031=CARTESIAN_POINT('Ctrl Pts',(4.76745636601108,1.30000000000037,7.39112846433221));
#54032=CARTESIAN_POINT('Ctrl Pts',(4.74343057879297,-1.30000000000005,7.61127081391063));
#54033=CARTESIAN_POINT('Ctrl Pts',(4.69479529387935,-1.18514270861182,7.59271990632606));
#54034=CARTESIAN_POINT('Ctrl Pts',(4.64932744556142,-1.06847604194514,7.57531939333081));
#54035=CARTESIAN_POINT('Ctrl Pts',(4.55160503231467,-0.794772684000857,
7.53777836898805));
#54036=CARTESIAN_POINT('Ctrl Pts',(4.49227113018039,-0.6363098000952,7.51826466037316));
#54037=CARTESIAN_POINT('Ctrl Pts',(4.42312822731368,-0.319434907277159,
7.48458776204415));
#54038=CARTESIAN_POINT('Ctrl Pts',(4.39568514603662,-0.158333333333333,
7.47029425012699));
#54039=CARTESIAN_POINT('Ctrl Pts',(4.39730494690124,0.158333333333335,7.4448710587498));
#54040=CARTESIAN_POINT('Ctrl Pts',(4.42635287440999,0.31943490727717,7.4340199568158));
#54041=CARTESIAN_POINT('Ctrl Pts',(4.4988256565189,0.63630980009521,7.41534420247766));
#54042=CARTESIAN_POINT('Ctrl Pts',(4.55984006195317,0.794772684000842,7.40686093806267));
#54043=CARTESIAN_POINT('Ctrl Pts',(4.66066222458958,1.06847604194524,7.39819903766625));
#54044=CARTESIAN_POINT('Ctrl Pts',(4.70749909041594,1.18514270861203,7.39603518760888));
#54045=CARTESIAN_POINT('Ctrl Pts',(4.75753064369264,1.30000000000037,7.39545690322072));
#54046=CARTESIAN_POINT('Ctrl Pts',(4.72909269571893,-1.30000000000005,7.61656804117484));
#54047=CARTESIAN_POINT('Ctrl Pts',(4.67765262468082,-1.18514270861182,7.59884377256573));
#54048=CARTESIAN_POINT('Ctrl Pts',(4.63012539389608,-1.06847604194514,7.5818984556327));
#54049=CARTESIAN_POINT('Ctrl Pts',(4.52936742673965,-0.794772684000858,
7.54455091781885));
#54050=CARTESIAN_POINT('Ctrl Pts',(4.47049638455632,-0.6363098000952,7.52370599516994));
#54051=CARTESIAN_POINT('Ctrl Pts',(4.40122132489785,-0.319434907277159,
7.48931759022313));
#54052=CARTESIAN_POINT('Ctrl Pts',(4.37468286868284,-0.158333333333333,
7.47450898079698));
#54053=CARTESIAN_POINT('Ctrl Pts',(4.37632493538259,0.158333333333335,7.44964337104086));
#54054=CARTESIAN_POINT('Ctrl Pts',(4.40447438467914,0.31943490727717,7.44002129711005));
#54055=CARTESIAN_POINT('Ctrl Pts',(4.47715751069514,0.63630980009521,7.42287433160762));
#54056=CARTESIAN_POINT('Ctrl Pts',(4.53783231460736,0.794772684000843,7.41626767988291));
#54057=CARTESIAN_POINT('Ctrl Pts',(4.64170473749484,1.06847604194524,7.40702856231035));
#54058=CARTESIAN_POINT('Ctrl Pts',(4.69057892767158,1.18514270861202,7.40397220206445));
#54059=CARTESIAN_POINT('Ctrl Pts',(4.74336478500964,1.30000000000037,7.40185875322678));
#54060=CARTESIAN_POINT('Ctrl Pts',(4.71179724858884,-1.30000000000005,7.62108876395165));
#54061=CARTESIAN_POINT('Ctrl Pts',(4.65696649830876,-1.18514270861182,7.60388388473665));
#54062=CARTESIAN_POINT('Ctrl Pts',(4.60695810500404,-1.06847604194514,7.58727783427176));
#54063=CARTESIAN_POINT('Ctrl Pts',(4.5025693216476,-0.794772684000857,7.55029794987688));
#54064=CARTESIAN_POINT('Ctrl Pts',(4.44432282135363,-0.6363098000952,7.52893227478901));
#54065=CARTESIAN_POINT('Ctrl Pts',(4.37493188734826,-0.31943490727716,7.4945638321171));
#54066=CARTESIAN_POINT('Ctrl Pts',(4.34949958004939,-0.158333333333333,
7.47981019719062));
#54067=CARTESIAN_POINT('Ctrl Pts',(4.3511508890067,0.158333333333335,7.45549244158879));
#54068=CARTESIAN_POINT('Ctrl Pts',(4.3782011752311,0.319434907277169,7.44657555188257));
#54069=CARTESIAN_POINT('Ctrl Pts',(4.45102359755922,0.63630980009521,7.43009211444813));
#54070=CARTESIAN_POINT('Ctrl Pts',(4.51106842473165,0.794772684000843,7.42392158711869));
#54071=CARTESIAN_POINT('Ctrl Pts',(4.6186361277069,1.06847604194524,7.41448353620949));
#54072=CARTESIAN_POINT('Ctrl Pts',(4.67003232286398,1.18514270861203,7.41114697329846));
#54073=CARTESIAN_POINT('Ctrl Pts',(4.72626264033635,1.30000000000037,7.40855923000074));
#54074=CARTESIAN_POINT('Ctrl Pts',(4.68590468587279,-1.30000000000005,7.62938620214826));
#54075=CARTESIAN_POINT('Ctrl Pts',(4.62599255528755,-1.18514270861182,7.61324620206889));
#54076=CARTESIAN_POINT('Ctrl Pts',(4.57225708453609,-1.06847604194514,7.59720278860638));
#54077=CARTESIAN_POINT('Ctrl Pts',(4.46238671720871,-0.79477268400086,7.56036242844115));
#54078=CARTESIAN_POINT('Ctrl Pts',(4.40501323857521,-0.636309800095201,
7.53737430405052));
#54079=CARTESIAN_POINT('Ctrl Pts',(4.33539413439024,-0.31943490727716,7.50142300748779));
#54080=CARTESIAN_POINT('Ctrl Pts',(4.31159708863585,-0.158333333333333,
7.48469201207812));
#54081=CARTESIAN_POINT('Ctrl Pts',(4.31325645221777,0.158333333333335,7.46109374815198));
#54082=CARTESIAN_POINT('Ctrl Pts',(4.33865773735432,0.319434907277168,7.45508785741748));
#54083=CARTESIAN_POINT('Ctrl Pts',(4.41176912970336,0.636309800095209,7.44121662497348));
#54084=CARTESIAN_POINT('Ctrl Pts',(4.47102658985925,0.794772684000846,7.43704322311659));
#54085=CARTESIAN_POINT('Ctrl Pts',(4.58415795221862,1.06847604194524,7.42743491767402));
#54086=CARTESIAN_POINT('Ctrl Pts',(4.63931218712884,1.18514270861202,7.42334114155557));
#54087=CARTESIAN_POINT('Ctrl Pts',(4.70065028211401,1.30000000000036,7.41931266872195));
#54088=CARTESIAN_POINT('Ctrl Pts',(4.65997285225604,-1.30000000000004,7.63611399060629));
#54089=CARTESIAN_POINT('Ctrl Pts',(4.59502018717183,-1.18514270861181,7.62090823517882));
#54090=CARTESIAN_POINT('Ctrl Pts',(4.5375965812993,-1.06847604194514,7.60524155890487));
#54091=CARTESIAN_POINT('Ctrl Pts',(4.42233019714286,-0.794772684000858,
7.56798358324191));
#54092=CARTESIAN_POINT('Ctrl Pts',(4.36590065335152,-0.636309800095198,
7.54205387854712));
#54093=CARTESIAN_POINT('Ctrl Pts',(4.29608547850594,-0.319434907277158,
7.50531053618865));
#54094=CARTESIAN_POINT('Ctrl Pts',(4.27389244970255,-0.158333333333333,
7.48940950321921));
#54095=CARTESIAN_POINT('Ctrl Pts',(4.27552401124187,0.158333333333334,7.46700810106707));
#54096=CARTESIAN_POINT('Ctrl Pts',(4.29923520182961,0.319434907277168,7.46181003652398));
#54097=CARTESIAN_POINT('Ctrl Pts',(4.37260473719026,0.636309800095207,7.45027063487121));
#54098=CARTESIAN_POINT('Ctrl Pts',(4.43110737170687,0.794772684000841,7.44930808338118));
#54099=CARTESIAN_POINT('Ctrl Pts',(4.54974418748316,1.06847604194523,7.43989901659481));
#54100=CARTESIAN_POINT('Ctrl Pts',(4.60861517528759,1.18514270861202,7.43508138351226));
#54101=CARTESIAN_POINT('Ctrl Pts',(4.67500366927415,1.30000000000036,7.42951895371868));
#54102=CARTESIAN_POINT('Ctrl Pts',(4.63687848316797,-1.30000000000004,7.64278362359798));
#54103=CARTESIAN_POINT('Ctrl Pts',(4.56734946810552,-1.18514270861181,7.6277193111944));
#54104=CARTESIAN_POINT('Ctrl Pts',(4.50657400117256,-1.06847604194514,7.61194573999381));
#54105=CARTESIAN_POINT('Ctrl Pts',(4.38639296178727,-0.794772684000858,
7.57386710532048));
#54106=CARTESIAN_POINT('Ctrl Pts',(4.33078037996717,-0.636309800095198,
7.54632081086968));
#54107=CARTESIAN_POINT('Ctrl Pts',(4.26079711972564,-0.319434907277158,
7.5084122504634));
#54108=CARTESIAN_POINT('Ctrl Pts',(4.2401246124826,-0.158333333333332,7.49191187221995));
#54109=CARTESIAN_POINT('Ctrl Pts',(4.24173169812143,0.158333333333334,7.47008700208653));
#54110=CARTESIAN_POINT('Ctrl Pts',(4.26387907057827,0.319434907277167,7.4663085322291));
#54111=CARTESIAN_POINT('Ctrl Pts',(4.3374051720377,0.636309800095206,7.4566122680534));
#54112=CARTESIAN_POINT('Ctrl Pts',(4.39510148966059,0.79477268400084,7.45739853999331));
#54113=CARTESIAN_POINT('Ctrl Pts',(4.51872055606065,1.06847604194523,7.44840780746785));
#54114=CARTESIAN_POINT('Ctrl Pts',(4.58098662417127,1.18514270861202,7.44334161528439));
#54115=CARTESIAN_POINT('Ctrl Pts',(4.65200864708575,1.30000000000036,7.43710098588828));
#54116=CARTESIAN_POINT('Ctrl Pts',(4.62245430981321,-1.30000000000005,7.64588206265252));
#54117=CARTESIAN_POINT('Ctrl Pts',(4.55013160928749,-1.18514270861182,7.63120092471038));
#54118=CARTESIAN_POINT('Ctrl Pts',(4.48731630235014,-1.06847604194514,7.61551111620122));
#54119=CARTESIAN_POINT('Ctrl Pts',(4.36416435830239,-0.794772684000858,
7.57693428901595));
#54120=CARTESIAN_POINT('Ctrl Pts',(4.30911474602555,-0.636309800095199,
7.54764413863052));
#54121=CARTESIAN_POINT('Ctrl Pts',(4.23903212360004,-0.319434907277158,
7.50902218476997));
#54122=CARTESIAN_POINT('Ctrl Pts',(4.21922995277278,-0.158333333333333,
7.49271556413392));
#54123=CARTESIAN_POINT('Ctrl Pts',(4.22079997598892,0.158333333333335,7.47152050406351));
#54124=CARTESIAN_POINT('Ctrl Pts',(4.24199652951127,0.319434907277168,7.46836398924111));
#54125=CARTESIAN_POINT('Ctrl Pts',(4.31563494327749,0.636309800095207,7.4602853261014));
#54126=CARTESIAN_POINT('Ctrl Pts',(4.37286400473976,0.794772684000841,7.4629571255785));
#54127=CARTESIAN_POINT('Ctrl Pts',(4.49955541502258,1.06847604194524,7.45478068246077));
#54128=CARTESIAN_POINT('Ctrl Pts',(4.56390770899303,1.18514270861202,7.44972028485976));
#54129=CARTESIAN_POINT('Ctrl Pts',(4.6377722798019,1.30000000000036,7.44313876891631));
#54130=CARTESIAN_POINT('Ctrl Pts',(4.60795019531385,-1.30000000000005,7.6493488567498));
#54131=CARTESIAN_POINT('Ctrl Pts',(4.53267139934727,-1.18514270861182,7.63479518093068));
#54132=CARTESIAN_POINT('Ctrl Pts',(4.46769163127909,-1.06847604194514,7.6189806971343));
#54133=CARTESIAN_POINT('Ctrl Pts',(4.34136818264232,-0.794772684000858,
7.57953335723679));
#54134=CARTESIAN_POINT('Ctrl Pts',(4.28685816211639,-0.636309800095199,
7.54783991273211));
#54135=CARTESIAN_POINT('Ctrl Pts',(4.21665741811185,-0.319434907277158,
7.50944861440254));
#54136=CARTESIAN_POINT('Ctrl Pts',(4.19781321920072,-0.158333333333333,
7.49584497305017));
#54137=CARTESIAN_POINT('Ctrl Pts',(4.19935364590263,0.158333333333335,7.47552237467756));
#54138=CARTESIAN_POINT('Ctrl Pts',(4.219536137998,0.319434907277168,7.47106293288307));
#54139=CARTESIAN_POINT('Ctrl Pts',(4.29328635170139,0.636309800095207,7.46345609177895));
#54140=CARTESIAN_POINT('Ctrl Pts',(4.35002376194345,0.79477268400084,7.4678362313814));
#54141=CARTESIAN_POINT('Ctrl Pts',(4.47994147943138,1.06847604194523,7.4600160329351));
#54142=CARTESIAN_POINT('Ctrl Pts',(4.54648534280962,1.18514270861202,7.45480994003203));
#54143=CARTESIAN_POINT('Ctrl Pts',(4.62333650359142,1.30000000000037,7.4477828283664));
#54144=CARTESIAN_POINT('Ctrl Pts',(4.59357906309859,-1.30000000000004,7.65261768781226));
#54145=CARTESIAN_POINT('Ctrl Pts',(4.515613582606,-1.18514270861181,7.63746571967198));
#54146=CARTESIAN_POINT('Ctrl Pts',(4.44867658010229,-1.06847604194513,7.62139812597335));
#54147=CARTESIAN_POINT('Ctrl Pts',(4.31951670401105,-0.794772684000855,
7.58216349200832));
#54148=CARTESIAN_POINT('Ctrl Pts',(4.26556225269653,-0.636309800095198,
7.55207793454907));
#54149=CARTESIAN_POINT('Ctrl Pts',(4.19532952755911,-0.319434907277159,
7.51449404889587));
#54150=CARTESIAN_POINT('Ctrl Pts',(4.17741300812966,-0.158333333333333,
7.50113035871167));
#54151=CARTESIAN_POINT('Ctrl Pts',(4.17893351407558,0.158333333333335,7.48022729652089));
#54152=CARTESIAN_POINT('Ctrl Pts',(4.19815674351198,0.319434907277168,7.47404087090977));
#54153=CARTESIAN_POINT('Ctrl Pts',(4.27192211671505,0.636309800095207,7.46629086955863));
#54154=CARTESIAN_POINT('Ctrl Pts',(4.32809954591735,0.794772684000841,7.47235465402125));
#54155=CARTESIAN_POINT('Ctrl Pts',(4.46089760304215,1.06847604194523,7.46486667057211));
#54156=CARTESIAN_POINT('Ctrl Pts',(4.52942990010045,1.18514270861202,7.45956477448967));
#54157=CARTESIAN_POINT('Ctrl Pts',(4.60901113594068,1.30000000000036,7.45220225290278));
#54158=CARTESIAN_POINT('Ctrl Pts',(4.57617941896526,-1.30000000000004,7.65590048748505));
#54159=CARTESIAN_POINT('Ctrl Pts',(4.49458263105147,-1.18514270861181,7.6399348939217));
#54160=CARTESIAN_POINT('Ctrl Pts',(4.4249715844402,-1.06847604194513,7.62369292737989));
#54161=CARTESIAN_POINT('Ctrl Pts',(4.29184560127414,-0.794772684000854,
7.58553225860559));
#54162=CARTESIAN_POINT('Ctrl Pts',(4.23841576762044,-0.636309800095198,
7.55884844446226));
#54163=CARTESIAN_POINT('Ctrl Pts',(4.1679993993941,-0.319434907277159,7.52344207579474));
#54164=CARTESIAN_POINT('Ctrl Pts',(4.15134356171619,-0.158333333333332,
7.5105034367935));
#54165=CARTESIAN_POINT('Ctrl Pts',(4.15284239670344,0.158333333333334,7.48968966703876));
#54166=CARTESIAN_POINT('Ctrl Pts',(4.17076731329137,0.319434907277167,7.48282865376814));
#54167=CARTESIAN_POINT('Ctrl Pts',(4.24470469705338,0.636309800095206,7.47377318779266));
#54168=CARTESIAN_POINT('Ctrl Pts',(4.30036736809567,0.79477268400084,7.47832213150233));
#54169=CARTESIAN_POINT('Ctrl Pts',(4.43718403996299,1.06847604194523,7.46992576188581));
#54170=CARTESIAN_POINT('Ctrl Pts',(4.50842391007758,1.18514270861202,7.46445378067426));
#54171=CARTESIAN_POINT('Ctrl Pts',(4.59168078261271,1.30000000000037,7.457144295542));
#54172=CARTESIAN_POINT('Ctrl Pts',(4.56433455848947,-1.30000000000004,7.65821867228285));
#54173=CARTESIAN_POINT('Ctrl Pts',(4.48025898197814,-1.18514270861181,7.64034602806837));
#54174=CARTESIAN_POINT('Ctrl Pts',(4.40891552700136,-1.06847604194513,7.62347431552138));
#54175=CARTESIAN_POINT('Ctrl Pts',(4.27351162159271,-0.794772684000851,
7.58680963675092));
#54176=CARTESIAN_POINT('Ctrl Pts',(4.22112140679108,-0.636309800095197,
7.56664485618359));
#54177=CARTESIAN_POINT('Ctrl Pts',(4.15113790298686,-0.319434907277159,
7.53468752939888));
#54178=CARTESIAN_POINT('Ctrl Pts',(4.13553292461561,-0.158333333333332,
7.52147411752544));
#54179=CARTESIAN_POINT('Ctrl Pts',(4.13706908989959,0.158333333333334,7.50081062858686));
#54180=CARTESIAN_POINT('Ctrl Pts',(4.15404363487222,0.319434907277167,7.49422021702462));
#54181=CARTESIAN_POINT('Ctrl Pts',(4.22749554627325,0.636309800095206,7.48233642793057));
#54182=CARTESIAN_POINT('Ctrl Pts',(4.2818545600116,0.79477268400084,7.4815169336313));
#54183=CARTESIAN_POINT('Ctrl Pts',(4.42096106050366,1.06847604194523,7.47158857881567));
#54184=CARTESIAN_POINT('Ctrl Pts',(4.49399758639363,1.18514270861202,7.46643805441502));
#54185=CARTESIAN_POINT('Ctrl Pts',(4.57985658851437,1.30000000000036,7.4604346225316));
#54186=CARTESIAN_POINT('Ctrl Pts',(4.55678639209678,-1.30000000000004,7.66234429787489));
#54187=CARTESIAN_POINT('Ctrl Pts',(4.4729437511331,-1.18514270861181,7.64437732819764));
#54188=CARTESIAN_POINT('Ctrl Pts',(4.40183404790298,-1.06847604194513,7.62775916256505));
#54189=CARTESIAN_POINT('Ctrl Pts',(4.26697204137397,-0.794772684000851,
7.59248388267156));
#54190=CARTESIAN_POINT('Ctrl Pts',(4.21502126192296,-0.636309800095197,
7.57484693907898));
#54191=CARTESIAN_POINT('Ctrl Pts',(4.14539022778078,-0.319434907277159,
7.54453895215762));
#54192=CARTESIAN_POINT('Ctrl Pts',(4.12973531027791,-0.158333333333332,
7.53130984870383));
#54193=CARTESIAN_POINT('Ctrl Pts',(4.13134197385143,0.158333333333334,7.51087245067975));
#54194=CARTESIAN_POINT('Ctrl Pts',(4.14849242828378,0.319434907277167,7.50479833736505));
#54195=CARTESIAN_POINT('Ctrl Pts',(4.22162247741412,0.636309800095206,7.49116657049894));
#54196=CARTESIAN_POINT('Ctrl Pts',(4.27538846798974,0.79477268400084,7.48674639736213));
#54197=CARTESIAN_POINT('Ctrl Pts',(4.41396332499183,1.06847604194523,7.47558190734422));
#54198=CARTESIAN_POINT('Ctrl Pts',(4.48679959516754,1.18514270861202,7.47049600927413));
#54199=CARTESIAN_POINT('Ctrl Pts',(4.57248821462725,1.30000000000036,7.46515690717758));
#54200=CARTESIAN_POINT('Ctrl Pts',(4.55678639209675,-1.3,7.66234429787489));
#54201=CARTESIAN_POINT('Ctrl Pts',(4.47294375113309,-1.18514270861178,7.64437732819764));
#54202=CARTESIAN_POINT('Ctrl Pts',(4.40183404790297,-1.06847604194512,7.62775916256504));
#54203=CARTESIAN_POINT('Ctrl Pts',(4.26697204137396,-0.794772684000851,
7.59248388267156));
#54204=CARTESIAN_POINT('Ctrl Pts',(4.21502126192295,-0.636309800095197,
7.57484693907897));
#54205=CARTESIAN_POINT('Ctrl Pts',(4.14539022778078,-0.319434907277159,
7.54453895215762));
#54206=CARTESIAN_POINT('Ctrl Pts',(4.12973531027791,-0.158333333333332,
7.53130984870383));
#54207=CARTESIAN_POINT('Ctrl Pts',(4.13134197385143,0.158333333333334,7.51087245067974));
#54208=CARTESIAN_POINT('Ctrl Pts',(4.14849242828378,0.319434907277167,7.50479833736505));
#54209=CARTESIAN_POINT('Ctrl Pts',(4.22162247741411,0.636309800095206,7.49116657049894));
#54210=CARTESIAN_POINT('Ctrl Pts',(4.27538846798974,0.79477268400084,7.48674639736213));
#54211=CARTESIAN_POINT('Ctrl Pts',(4.41396332499177,1.06847604194511,7.47558190734422));
#54212=CARTESIAN_POINT('Ctrl Pts',(4.48679959516739,1.18514270861178,7.47049600927414));
#54213=CARTESIAN_POINT('Ctrl Pts',(4.57248821462698,1.3,7.4651569071776));
#54214=CARTESIAN_POINT('',(4.94063630726094,-1.2,7.50432364248438));
#54215=CARTESIAN_POINT('Ctrl Pts',(4.94063630726094,-1.2,7.50432364248438));
#54216=CARTESIAN_POINT('Ctrl Pts',(4.91543282814962,-1.22406366621288,7.52208787588012));
#54217=CARTESIAN_POINT('Ctrl Pts',(4.89161703542051,-1.24658722057704,7.53992231957329));
#54218=CARTESIAN_POINT('Ctrl Pts',(4.86706934907891,-1.2698559227574,7.55736574712289));
#54219=CARTESIAN_POINT('Ctrl Pts',(4.86506208885659,-1.27176577548985,7.55895005581378));
#54220=CARTESIAN_POINT('Ctrl Pts',(4.83515729345013,-1.30000000000007,7.57914897810145));
#54221=CARTESIAN_POINT('',(4.94779107628116,-0.653834841367199,7.34786299436625));
#54222=CARTESIAN_POINT('Ctrl Pts',(4.94779107631832,-0.653834841365921,
7.3478629943724));
#54223=CARTESIAN_POINT('Ctrl Pts',(4.94731087382852,-0.717195374693346,
7.36393152865268));
#54224=CARTESIAN_POINT('Ctrl Pts',(4.94685161325703,-0.764532971978773,
7.37728967122618));
#54225=CARTESIAN_POINT('Ctrl Pts',(4.94482900656359,-0.949610828965762,
7.42891509030179));
#54226=CARTESIAN_POINT('Ctrl Pts',(4.94332990982166,-1.05888885523217,7.46059351852754));
#54227=CARTESIAN_POINT('Ctrl Pts',(4.94063630726094,-1.2,7.50432364248438));
#54228=CARTESIAN_POINT('',(4.94999291725008,0.653834841531101,7.20837371924883));
#54229=CARTESIAN_POINT('Ctrl Pts',(4.94999291725008,0.653834841531103,7.20837371924884));
#54230=CARTESIAN_POINT('Ctrl Pts',(4.91225397924647,0.575974734740856,7.22582001049342));
#54231=CARTESIAN_POINT('Ctrl Pts',(4.88067089553362,0.493646300356214,7.2412455994813));
#54232=CARTESIAN_POINT('Ctrl Pts',(4.83632534903071,0.338148396013879,7.26563634685165));
#54233=CARTESIAN_POINT('Ctrl Pts',(4.82128042816978,0.265672258741385,7.27532070701134));
#54234=CARTESIAN_POINT('Ctrl Pts',(4.80341717712112,0.129723868038644,7.29191291738494));
#54235=CARTESIAN_POINT('Ctrl Pts',(4.79913221039573,0.066629300779875,7.29899463278343));
#54236=CARTESIAN_POINT('Ctrl Pts',(4.79855028835759,-0.0595469689982444,
7.31231323091239));
#54237=CARTESIAN_POINT('Ctrl Pts',(4.80223201689649,-0.122785107468493,
7.31864896555666));
#54238=CARTESIAN_POINT('Ctrl Pts',(4.81905000979055,-0.260135494715071,
7.33079046336944));
#54239=CARTESIAN_POINT('Ctrl Pts',(4.833790517691,-0.333948532118538,7.33629188943222));
#54240=CARTESIAN_POINT('Ctrl Pts',(4.87782657508354,-0.491208515200836,
7.34478416173381));
#54241=CARTESIAN_POINT('Ctrl Pts',(4.9092926136062,-0.574351663742094,7.34738838935052));
#54242=CARTESIAN_POINT('Ctrl Pts',(4.94779107624583,-0.653834841384027,
7.34786299441341));
#54243=CARTESIAN_POINT('',(4.94934267693687,1.2,7.28066638861011));
#54244=CARTESIAN_POINT('Ctrl Pts',(4.94934267693687,1.2,7.28066638861011));
#54245=CARTESIAN_POINT('Ctrl Pts',(4.94957987508122,1.12296364294518,7.26611293060881));
#54246=CARTESIAN_POINT('Ctrl Pts',(4.94977340107779,1.02715393518566,7.25038272030311));
#54247=CARTESIAN_POINT('Ctrl Pts',(4.9499755995156,0.796382219298827,7.22023948863579));
#54248=CARTESIAN_POINT('Ctrl Pts',(4.94998203044102,0.739891552765075,7.21480928582414));
#54249=CARTESIAN_POINT('Ctrl Pts',(4.94999291725008,0.6538348415311,7.20837371924884));
#54250=CARTESIAN_POINT('Ctrl Pts',(4.84757646506369,1.30000000000001,7.35330497500277));
#54251=CARTESIAN_POINT('Ctrl Pts',(4.86532490684006,1.28264531619758,7.34112851298703));
#54252=CARTESIAN_POINT('Ctrl Pts',(4.8829689846372,1.26535232528287,7.32871014390654));
#54253=CARTESIAN_POINT('Ctrl Pts',(4.92078898353074,1.22818637919983,7.3015438601204));
#54254=CARTESIAN_POINT('Ctrl Pts',(4.93221880462763,1.21690340343215,7.29405567061454));
#54255=CARTESIAN_POINT('Ctrl Pts',(4.94934267693687,1.2,7.28066638861011));
#54256=CARTESIAN_POINT('Ctrl Pts',(4.55678639209675,-1.3,7.66234429787489));
#54257=CARTESIAN_POINT('Ctrl Pts',(4.47294375113309,-1.18514270861178,7.64437732819764));
#54258=CARTESIAN_POINT('Ctrl Pts',(4.40183404790298,-1.06847604194512,7.62775916256505));
#54259=CARTESIAN_POINT('Ctrl Pts',(4.26697204137397,-0.794772684000851,
7.59248388267156));
#54260=CARTESIAN_POINT('Ctrl Pts',(4.21502126192295,-0.636309800095197,
7.57484693907897));
#54261=CARTESIAN_POINT('Ctrl Pts',(4.14539022778077,-0.319434907277159,
7.54453895215762));
#54262=CARTESIAN_POINT('Ctrl Pts',(4.12973531027791,-0.158333333333332,
7.53130984870382));
#54263=CARTESIAN_POINT('Ctrl Pts',(4.13134197385143,0.158333333333334,7.51087245067974));
#54264=CARTESIAN_POINT('Ctrl Pts',(4.14849242828378,0.319434907277167,7.50479833736504));
#54265=CARTESIAN_POINT('Ctrl Pts',(4.22162247741411,0.636309800095206,7.49116657049894));
#54266=CARTESIAN_POINT('Ctrl Pts',(4.27538846798974,0.79477268400084,7.48674639736213));
#54267=CARTESIAN_POINT('Ctrl Pts',(4.41396332499176,1.06847604194511,7.47558190734422));
#54268=CARTESIAN_POINT('Ctrl Pts',(4.48679959516739,1.18514270861178,7.47049600927414));
#54269=CARTESIAN_POINT('Ctrl Pts',(4.57248821462698,1.3,7.4651569071776));
#54270=CARTESIAN_POINT('Ctrl Pts',(4.54709012720593,-1.3,7.73866658637446));
#54271=CARTESIAN_POINT('Ctrl Pts',(4.46362634796674,-1.18514270861178,7.71900924136913));
#54272=CARTESIAN_POINT('Ctrl Pts',(4.39282414406279,-1.06847604194512,7.70122437392077));
#54273=CARTESIAN_POINT('Ctrl Pts',(4.25850766107618,-0.794772684000851,
7.66446357000893));
#54274=CARTESIAN_POINT('Ctrl Pts',(4.20664978510482,-0.636309800095197,
7.64753822102798));
#54275=CARTESIAN_POINT('Ctrl Pts',(4.1373298362099,-0.319434907277159,7.61782007234104));
#54276=CARTESIAN_POINT('Ctrl Pts',(4.12172229231298,-0.158333333333332,
7.60583161692362));
#54277=CARTESIAN_POINT('Ctrl Pts',(4.12368594131515,0.158333333333334,7.58543173958001));
#54278=CARTESIAN_POINT('Ctrl Pts',(4.14114067935745,0.319434907277167,7.5781539388917));
#54279=CARTESIAN_POINT('Ctrl Pts',(4.21469765004064,0.636309800095206,7.56400990143153));
#54280=CARTESIAN_POINT('Ctrl Pts',(4.26870246277087,0.79477268400084,7.55891299945219));
#54281=CARTESIAN_POINT('Ctrl Pts',(4.40750206450663,1.06847604194511,7.54931499191075));
#54282=CARTESIAN_POINT('Ctrl Pts',(4.48039654346318,1.18514270861178,7.54543423312736));
#54283=CARTESIAN_POINT('Ctrl Pts',(4.56610429681699,1.3,7.54182733738404));
#54284=CARTESIAN_POINT('Ctrl Pts',(4.53739386231511,-1.3,7.81498887487404));
#54285=CARTESIAN_POINT('Ctrl Pts',(4.45430894480039,-1.18514270861178,7.79364115454063));
#54286=CARTESIAN_POINT('Ctrl Pts',(4.38381424022261,-1.06847604194512,7.7746895852765));
#54287=CARTESIAN_POINT('Ctrl Pts',(4.2500432807784,-0.794772684000851,7.7364432573463));
#54288=CARTESIAN_POINT('Ctrl Pts',(4.19827830828669,-0.636309800095197,
7.72022950297699));
#54289=CARTESIAN_POINT('Ctrl Pts',(4.12926944463902,-0.319434907277159,
7.69110119252446));
#54290=CARTESIAN_POINT('Ctrl Pts',(4.11370927434805,-0.158333333333332,
7.68035338514341));
#54291=CARTESIAN_POINT('Ctrl Pts',(4.11602990877888,0.158333333333334,7.65999102848028));
#54292=CARTESIAN_POINT('Ctrl Pts',(4.13378893043113,0.319434907277167,7.65150954041835));
#54293=CARTESIAN_POINT('Ctrl Pts',(4.20777282266716,0.636309800095206,7.63685323236411));
#54294=CARTESIAN_POINT('Ctrl Pts',(4.262016457552,0.79477268400084,7.63107960154224));
#54295=CARTESIAN_POINT('Ctrl Pts',(4.40104080402149,1.06847604194511,7.62304807647727));
#54296=CARTESIAN_POINT('Ctrl Pts',(4.47399349175896,1.18514270861178,7.62037245698058));
#54297=CARTESIAN_POINT('Ctrl Pts',(4.559720379007,1.3,7.61849776759048));
#54298=CARTESIAN_POINT('Ctrl Pts',(4.52769759742428,-1.3,7.89131116337361));
#54299=CARTESIAN_POINT('Ctrl Pts',(4.44499154163403,-1.18514270861178,7.86827306771213));
#54300=CARTESIAN_POINT('Ctrl Pts',(4.37480433638243,-1.06847604194512,7.84815479663223));
#54301=CARTESIAN_POINT('Ctrl Pts',(4.24157890048062,-0.794772684000851,
7.80842294468367));
#54302=CARTESIAN_POINT('Ctrl Pts',(4.18990683146856,-0.636309800095197,
7.792920784926));
#54303=CARTESIAN_POINT('Ctrl Pts',(4.12120905306814,-0.319434907277159,
7.76438231270788));
#54304=CARTESIAN_POINT('Ctrl Pts',(4.10569625638312,-0.158333333333332,
7.7548751533632));
#54305=CARTESIAN_POINT('Ctrl Pts',(4.1083738762426,0.158333333333334,7.73455031738056));
#54306=CARTESIAN_POINT('Ctrl Pts',(4.1264371815048,0.319434907277167,7.724865141945));
#54307=CARTESIAN_POINT('Ctrl Pts',(4.20084799529369,0.636309800095206,7.7096965632967));
#54308=CARTESIAN_POINT('Ctrl Pts',(4.25533045233313,0.79477268400084,7.70324620363229));
#54309=CARTESIAN_POINT('Ctrl Pts',(4.39457954353636,1.06847604194511,7.69678116104379));
#54310=CARTESIAN_POINT('Ctrl Pts',(4.46759044005475,1.18514270861178,7.69531068083379));
#54311=CARTESIAN_POINT('Ctrl Pts',(4.55333646119701,1.3,7.69516819779692));
#54312=CARTESIAN_POINT('Ctrl Pts',(4.52769759742429,-1.3,7.89131116337361));
#54313=CARTESIAN_POINT('Ctrl Pts',(4.44499154163404,-1.18514270861178,7.86827306771213));
#54314=CARTESIAN_POINT('Ctrl Pts',(4.37480433638243,-1.06847604194512,7.84815479663222));
#54315=CARTESIAN_POINT('Ctrl Pts',(4.24157890048062,-0.794772684000851,
7.80842294468367));
#54316=CARTESIAN_POINT('Ctrl Pts',(4.18990683146856,-0.636309800095197,
7.792920784926));
#54317=CARTESIAN_POINT('Ctrl Pts',(4.12120905306814,-0.319434907277159,
7.76438231270788));
#54318=CARTESIAN_POINT('Ctrl Pts',(4.10569625638312,-0.158333333333332,
7.7548751533632));
#54319=CARTESIAN_POINT('Ctrl Pts',(4.1083738762426,0.158333333333334,7.73455031738056));
#54320=CARTESIAN_POINT('Ctrl Pts',(4.1264371815048,0.319434907277167,7.724865141945));
#54321=CARTESIAN_POINT('Ctrl Pts',(4.20084799529369,0.636309800095206,7.7096965632967));
#54322=CARTESIAN_POINT('Ctrl Pts',(4.25533045233313,0.79477268400084,7.70324620363229));
#54323=CARTESIAN_POINT('Ctrl Pts',(4.39457954353635,1.06847604194511,7.69678116104379));
#54324=CARTESIAN_POINT('Ctrl Pts',(4.46759044005475,1.18514270861178,7.69531068083379));
#54325=CARTESIAN_POINT('Ctrl Pts',(4.55333646119701,1.3,7.69516819779692));
#54326=CARTESIAN_POINT('Ctrl Pts',(4.52769759742604,-1.30000000000244,7.8913111633741));
#54327=CARTESIAN_POINT('Ctrl Pts',(4.44499154163503,-1.18514270861343,7.86827306771241));
#54328=CARTESIAN_POINT('Ctrl Pts',(4.37480433638284,-1.06847604194595,7.84815479663235));
#54329=CARTESIAN_POINT('Ctrl Pts',(4.24157890048062,-0.794772684000851,
7.80842294468367));
#54330=CARTESIAN_POINT('Ctrl Pts',(4.18990683146856,-0.636309800095196,
7.792920784926));
#54331=CARTESIAN_POINT('Ctrl Pts',(4.12120905306814,-0.319434907277159,
7.76438231270788));
#54332=CARTESIAN_POINT('Ctrl Pts',(4.10569625638312,-0.158333333333332,
7.7548751533632));
#54333=CARTESIAN_POINT('Ctrl Pts',(4.1083738762426,0.158333333333334,7.73455031738056));
#54334=CARTESIAN_POINT('Ctrl Pts',(4.1264371815048,0.319434907277167,7.72486514194501));
#54335=CARTESIAN_POINT('Ctrl Pts',(4.20084799529369,0.636309800095206,7.70969656329671));
#54336=CARTESIAN_POINT('Ctrl Pts',(4.25533045233313,0.79477268400084,7.7032462036323));
#54337=CARTESIAN_POINT('Ctrl Pts',(4.39457954353637,1.06847604194513,7.69678116104379));
#54338=CARTESIAN_POINT('Ctrl Pts',(4.46759044005478,1.18514270861182,7.69531068083379));
#54339=CARTESIAN_POINT('Ctrl Pts',(4.55333646119706,1.30000000000007,7.69516819779692));
#54340=CARTESIAN_POINT('Ctrl Pts',(4.53392313642068,-1.30000000000244,7.89746222583649));
#54341=CARTESIAN_POINT('Ctrl Pts',(4.45118854317531,-1.18514270861343,7.87373889304186));
#54342=CARTESIAN_POINT('Ctrl Pts',(4.38081889485167,-1.06847604194595,7.85351577236843));
#54343=CARTESIAN_POINT('Ctrl Pts',(4.24681642619259,-0.794772684000851,
7.81488250820649));
#54344=CARTESIAN_POINT('Ctrl Pts',(4.19381566978082,-0.636309800095196,
7.80277904736738));
#54345=CARTESIAN_POINT('Ctrl Pts',(4.12443963753454,-0.319434907277159,
7.77588343648135));
#54346=CARTESIAN_POINT('Ctrl Pts',(4.10920625064663,-0.158333333333332,
7.76590783487045));
#54347=CARTESIAN_POINT('Ctrl Pts',(4.11199983518693,0.158333333333334,7.74537650602099));
#54348=CARTESIAN_POINT('Ctrl Pts',(4.13001103020958,0.319434907277167,7.73569629634525));
#54349=CARTESIAN_POINT('Ctrl Pts',(4.20510952842189,0.636309800095206,7.71898770243354));
#54350=CARTESIAN_POINT('Ctrl Pts',(4.26054738494527,0.79477268400084,7.71015610884286));
#54351=CARTESIAN_POINT('Ctrl Pts',(4.40061540550434,1.06847604194513,7.70244469618862));
#54352=CARTESIAN_POINT('Ctrl Pts',(4.47390766109764,1.18514270861182,7.70077480939336));
#54353=CARTESIAN_POINT('Ctrl Pts',(4.5598619162159,1.30000000000007,7.70077302060486));
#54354=CARTESIAN_POINT('Ctrl Pts',(4.54480756132074,-1.30000000000244,7.9031313104298));
#54355=CARTESIAN_POINT('Ctrl Pts',(4.46489083553443,-1.18514270861343,7.87867015857436));
#54356=CARTESIAN_POINT('Ctrl Pts',(4.39634596099135,-1.06847604194595,7.85850593886263));
#54357=CARTESIAN_POINT('Ctrl Pts',(4.26426483974512,-0.794772684000851,
7.82184933034068));
#54358=CARTESIAN_POINT('Ctrl Pts',(4.20887006018204,-0.636309800095195,
7.81473397539683));
#54359=CARTESIAN_POINT('Ctrl Pts',(4.13843139653786,-0.319434907277158,
7.79050397880872));
#54360=CARTESIAN_POINT('Ctrl Pts',(4.12232754980889,-0.158333333333332,
7.78005767523933));
#54361=CARTESIAN_POINT('Ctrl Pts',(4.12518911467222,0.158333333333334,7.75938696584332));
#54362=CARTESIAN_POINT('Ctrl Pts',(4.14416864038823,0.319434907277167,7.75020180904442));
#54363=CARTESIAN_POINT('Ctrl Pts',(4.22040735616573,0.636309800095205,7.73021018349228));
#54364=CARTESIAN_POINT('Ctrl Pts',(4.27822012753513,0.794772684000839,7.71521033816527));
#54365=CARTESIAN_POINT('Ctrl Pts',(4.41636977068153,1.06847604194513,7.70556351793047));
#54366=CARTESIAN_POINT('Ctrl Pts',(4.48783523330211,1.18514270861182,7.7041518618103));
#54367=CARTESIAN_POINT('Ctrl Pts',(4.57096629697396,1.30000000000006,7.7055043005997));
#54368=CARTESIAN_POINT('Ctrl Pts',(4.56073300810824,-1.30000000000243,7.91156448348569));
#54369=CARTESIAN_POINT('Ctrl Pts',(4.48442324017247,-1.18514270861343,7.8878141720034));
#54370=CARTESIAN_POINT('Ctrl Pts',(4.41849168518471,-1.06847604194595,7.86837871921155));
#54371=CARTESIAN_POINT('Ctrl Pts',(4.29015235166538,-0.794772684000849,
7.83344712197293));
#54372=CARTESIAN_POINT('Ctrl Pts',(4.23393748623805,-0.636309800095195,
7.8277112028804));
#54373=CARTESIAN_POINT('Ctrl Pts',(4.16339507988998,-0.319434907277158,
7.804796401206));
#54374=CARTESIAN_POINT('Ctrl Pts',(4.14588138546196,-0.158333333333332,
7.7947403583322));
#54375=CARTESIAN_POINT('Ctrl Pts',(4.14874058420388,0.158333333333334,7.7739769333919));
#54376=CARTESIAN_POINT('Ctrl Pts',(4.16904183231081,0.319434907277167,7.76463591973765));
#54377=CARTESIAN_POINT('Ctrl Pts',(4.24555415646176,0.636309800095206,7.7424739257509));
#54378=CARTESIAN_POINT('Ctrl Pts',(4.30458812558598,0.794772684000839,7.72425389573271));
#54379=CARTESIAN_POINT('Ctrl Pts',(4.43908143338691,1.06847604194513,7.71273200536022));
#54380=CARTESIAN_POINT('Ctrl Pts',(4.50789470780772,1.18514270861182,7.71093554617766));
#54381=CARTESIAN_POINT('Ctrl Pts',(4.58730408717054,1.30000000000006,7.71233002722669));
#54382=CARTESIAN_POINT('Ctrl Pts',(4.57382741729863,-1.30000000000243,7.91886372538083));
#54383=CARTESIAN_POINT('Ctrl Pts',(4.50011834828894,-1.18514270861343,7.89601079220276));
#54384=CARTESIAN_POINT('Ctrl Pts',(4.43611194809718,-1.06847604194595,7.87708349177196));
#54385=CARTESIAN_POINT('Ctrl Pts',(4.31065946519988,-0.794772684000845,
7.84242663834982));
#54386=CARTESIAN_POINT('Ctrl Pts',(4.2542467506077,-0.636309800095193,7.83492820952284));
#54387=CARTESIAN_POINT('Ctrl Pts',(4.18369130649239,-0.319434907277157,
7.81215028741846));
#54388=CARTESIAN_POINT('Ctrl Pts',(4.16488401333284,-0.158333333333331,
7.80356975748878));
#54389=CARTESIAN_POINT('Ctrl Pts',(4.16760272647753,0.158333333333333,7.78337191057216));
#54390=CARTESIAN_POINT('Ctrl Pts',(4.18885680806588,0.319434907277164,7.77400698678823));
#54391=CARTESIAN_POINT('Ctrl Pts',(4.26550396617013,0.636309800095202,7.75105538623989));
#54392=CARTESIAN_POINT('Ctrl Pts',(4.32541781011878,0.794772684000836,7.73137058834162));
#54393=CARTESIAN_POINT('Ctrl Pts',(4.45717945460002,1.06847604194513,7.71905327456052));
#54394=CARTESIAN_POINT('Ctrl Pts',(4.52402445451157,1.18514270861182,7.71709979233987));
#54395=CARTESIAN_POINT('Ctrl Pts',(4.60067972068886,1.30000000000006,7.71852453663296));
#54396=CARTESIAN_POINT('Ctrl Pts',(4.58698548913814,-1.30000000000243,7.92639668444855));
#54397=CARTESIAN_POINT('Ctrl Pts',(4.51610702437853,-1.18514270861343,7.90459440423691));
#54398=CARTESIAN_POINT('Ctrl Pts',(4.4542148014283,-1.06847604194595,7.88626268544465));
#54399=CARTESIAN_POINT('Ctrl Pts',(4.33199140118815,-0.794772684000845,
7.85193043894911));
#54400=CARTESIAN_POINT('Ctrl Pts',(4.27544799960624,-0.636309800095193,
7.84267294551725));
#54401=CARTESIAN_POINT('Ctrl Pts',(4.20509654546967,-0.319434907277158,
7.81947012356536));
#54402=CARTESIAN_POINT('Ctrl Pts',(4.18502425031126,-0.158333333333331,
7.81196684122426));
#54403=CARTESIAN_POINT('Ctrl Pts',(4.18789652359372,0.158333333333334,7.79090500173329));
#54404=CARTESIAN_POINT('Ctrl Pts',(4.21065422441233,0.319434907277165,7.7790726717311));
#54405=CARTESIAN_POINT('Ctrl Pts',(4.28723692830633,0.636309800095203,7.75585784273532));
#54406=CARTESIAN_POINT('Ctrl Pts',(4.34717946538134,0.794772684000837,7.73863682367033));
#54407=CARTESIAN_POINT('Ctrl Pts',(4.47565859061765,1.06847604194513,7.72650961893564));
#54408=CARTESIAN_POINT('Ctrl Pts',(4.54036052502848,1.18514270861182,7.72422790455448));
#54409=CARTESIAN_POINT('Ctrl Pts',(4.61415054115615,1.30000000000006,7.7249138933646));
#54410=CARTESIAN_POINT('Ctrl Pts',(4.59965290246012,-1.30000000000243,7.9352726802013));
#54411=CARTESIAN_POINT('Ctrl Pts',(4.53148144844337,-1.18514270861343,7.91440595450751));
#54412=CARTESIAN_POINT('Ctrl Pts',(4.47163014578841,-1.06847604194595,7.89650759170913));
#54413=CARTESIAN_POINT('Ctrl Pts',(4.35258287753016,-0.794772684000846,
7.86201630519716));
#54414=CARTESIAN_POINT('Ctrl Pts',(4.29598055952938,-0.636309800095193,
7.85080058306915));
#54415=CARTESIAN_POINT('Ctrl Pts',(4.22608334988363,-0.319434907277157,
7.82600970215437));
#54416=CARTESIAN_POINT('Ctrl Pts',(4.20522035605998,-0.158333333333331,
7.8176557606092));
#54417=CARTESIAN_POINT('Ctrl Pts',(4.20818531124961,0.158333333333333,7.79597947196624));
#54418=CARTESIAN_POINT('Ctrl Pts',(4.23182022180882,0.319434907277164,7.78420148504121));
#54419=CARTESIAN_POINT('Ctrl Pts',(4.30815003712369,0.636309800095202,7.76169357626058));
#54420=CARTESIAN_POINT('Ctrl Pts',(4.36828391922503,0.794772684000836,7.74628043878177));
#54421=CARTESIAN_POINT('Ctrl Pts',(4.49374998194681,1.06847604194513,7.73402993457807));
#54422=CARTESIAN_POINT('Ctrl Pts',(4.55647188035704,1.18514270861181,7.7312467586804));
#54423=CARTESIAN_POINT('Ctrl Pts',(4.62760606760105,1.30000000000006,7.73098319622891));
#54424=CARTESIAN_POINT('Ctrl Pts',(4.62058857472608,-1.30000000000242,7.94740044967756));
#54425=CARTESIAN_POINT('Ctrl Pts',(4.55682246865916,-1.18514270861342,7.92810801062365));
#54426=CARTESIAN_POINT('Ctrl Pts',(4.50024585615088,-1.06847604194595,7.91113510616114));
#54427=CARTESIAN_POINT('Ctrl Pts',(4.38615173151841,-0.794772684000848,
7.87728289036243));
#54428=CARTESIAN_POINT('Ctrl Pts',(4.32908918141778,-0.636309800095194,
7.86428752440045));
#54429=CARTESIAN_POINT('Ctrl Pts',(4.25969428741779,-0.319434907277158,
7.83785273071171));
#54430=CARTESIAN_POINT('Ctrl Pts',(4.23756287865151,-0.158333333333331,
7.82795116092122));
#54431=CARTESIAN_POINT('Ctrl Pts',(4.24063325570311,0.158333333333333,7.80566477392697));
#54432=CARTESIAN_POINT('Ctrl Pts',(4.26568526094983,0.319434907277163,7.79454110809123));
#54433=CARTESIAN_POINT('Ctrl Pts',(4.34163938416832,0.636309800095201,7.77301126161501));
#54434=CARTESIAN_POINT('Ctrl Pts',(4.40223043329164,0.794772684000837,7.75938974055269));
#54435=CARTESIAN_POINT('Ctrl Pts',(4.52273003821343,1.06847604194513,7.7468944981955));
#54436=CARTESIAN_POINT('Ctrl Pts',(4.58215662922367,1.18514270861182,7.74350690324006));
#54437=CARTESIAN_POINT('Ctrl Pts',(4.64884999722391,1.30000000000006,7.74214044075126));
#54438=CARTESIAN_POINT('Ctrl Pts',(4.648594134421,-1.30000000000242,7.96634699489031));
#54439=CARTESIAN_POINT('Ctrl Pts',(4.590425503944,-1.18514270861342,7.95036965591271));
#54440=CARTESIAN_POINT('Ctrl Pts',(4.53808890713736,-1.06847604194595,7.93529776095));
#54441=CARTESIAN_POINT('Ctrl Pts',(4.43065406308698,-0.794772684000845,
7.90257042527186));
#54442=CARTESIAN_POINT('Ctrl Pts',(4.3736277410315,-0.636309800095188,7.88520288404559));
#54443=CARTESIAN_POINT('Ctrl Pts',(4.30526704996447,-0.319434907277153,
7.85555771503743));
#54444=CARTESIAN_POINT('Ctrl Pts',(4.28146640826412,-0.15833333333333,7.84357758256878));
#54445=CARTESIAN_POINT('Ctrl Pts',(4.28477232272335,0.158333333333332,7.82001009819072));
#54446=CARTESIAN_POINT('Ctrl Pts',(4.31173064007393,0.319434907277162,7.80929521920069));
#54447=CARTESIAN_POINT('Ctrl Pts',(4.38712719264106,0.636309800095196,7.78915795492929));
#54448=CARTESIAN_POINT('Ctrl Pts',(4.44813248358814,0.794772684000826,7.77910758672209));
#54449=CARTESIAN_POINT('Ctrl Pts',(4.5620254058037,1.06847604194512,7.76584719773633));
#54450=CARTESIAN_POINT('Ctrl Pts',(4.61711174649682,1.18514270861181,7.76112877184541));
#54451=CARTESIAN_POINT('Ctrl Pts',(4.67798440200465,1.30000000000006,7.75743185110967));
#54452=CARTESIAN_POINT('Ctrl Pts',(4.68165552287129,-1.30000000000242,7.98886506857474));
#54453=CARTESIAN_POINT('Ctrl Pts',(4.63044692290565,-1.18514270861342,7.9759028451139));
#54454=CARTESIAN_POINT('Ctrl Pts',(4.58326800846122,-1.06847604194594,7.96280091003532));
#54455=CARTESIAN_POINT('Ctrl Pts',(4.48358465767529,-0.794772684000843,
7.93221005718464));
#54456=CARTESIAN_POINT('Ctrl Pts',(4.4255974463165,-0.636309800095188,7.91320356677101));
#54457=CARTESIAN_POINT('Ctrl Pts',(4.3581626577691,-0.319434907277154,7.88096518691823));
#54458=CARTESIAN_POINT('Ctrl Pts',(4.33281031472247,-0.158333333333329,
7.86496806667059));
#54459=CARTESIAN_POINT('Ctrl Pts',(4.33640145193234,0.158333333333332,7.84022588101273));
#54460=CARTESIAN_POINT('Ctrl Pts',(4.36531510784172,0.31943490727716,7.8318139044389));
#54461=CARTESIAN_POINT('Ctrl Pts',(4.44012553436285,0.636309800095195,7.81297575562654));
#54462=CARTESIAN_POINT('Ctrl Pts',(4.50196696609397,0.794772684000829,7.80507489872517));
#54463=CARTESIAN_POINT('Ctrl Pts',(4.6082648302697,1.06847604194512,7.78952242190487));
#54464=CARTESIAN_POINT('Ctrl Pts',(4.65828629564362,1.1851427086118,7.78276118857335));
#54465=CARTESIAN_POINT('Ctrl Pts',(4.71231681971385,1.30000000000005,7.77597081284977));
#54466=CARTESIAN_POINT('Ctrl Pts',(4.70425563008758,-1.30000000000241,8.00520911535597));
#54467=CARTESIAN_POINT('Ctrl Pts',(4.65747659860534,-1.18514270861341,7.99545421885104));
#54468=CARTESIAN_POINT('Ctrl Pts',(4.61364357336526,-1.06847604194593,7.98435965147816));
#54469=CARTESIAN_POINT('Ctrl Pts',(4.51918638006031,-0.794772684000833,
7.95563407368116));
#54470=CARTESIAN_POINT('Ctrl Pts',(4.46117060216464,-0.636309800095182,
7.93352610681582));
#54471=CARTESIAN_POINT('Ctrl Pts',(4.3944737386267,-0.319434907277151,7.89939714677356));
#54472=CARTESIAN_POINT('Ctrl Pts',(4.36771834352831,-0.158333333333328,
7.88204658024336));
#54473=CARTESIAN_POINT('Ctrl Pts',(4.37150210807931,0.158333333333331,7.85651957051754));
#54474=CARTESIAN_POINT('Ctrl Pts',(4.40196138338493,0.319434907277159,7.8487048664006));
#54475=CARTESIAN_POINT('Ctrl Pts',(4.47652822152956,0.636309800095191,7.83010030917989));
#54476=CARTESIAN_POINT('Ctrl Pts',(4.53908134358413,0.794772684000821,7.82329415309885));
#54477=CARTESIAN_POINT('Ctrl Pts',(4.64012069704688,1.06847604194511,7.80627724109663));
#54478=CARTESIAN_POINT('Ctrl Pts',(4.68659362897972,1.1851427086118,7.79832390296704));
#54479=CARTESIAN_POINT('Ctrl Pts',(4.73580330060843,1.30000000000004,7.78978321737488));
#54480=CARTESIAN_POINT('Ctrl Pts',(4.71911478157206,-1.30000000000241,8.01670270298301));
#54481=CARTESIAN_POINT('Ctrl Pts',(4.67550859596122,-1.18514270861341,8.00842616314175));
#54482=CARTESIAN_POINT('Ctrl Pts',(4.63403254674509,-1.06847604194593,7.99829893819727));
#54483=CARTESIAN_POINT('Ctrl Pts',(4.54313561700505,-0.794772684000834,
7.97062756981452));
#54484=CARTESIAN_POINT('Ctrl Pts',(4.4847695101651,-0.63630980009518,7.94750775051987));
#54485=CARTESIAN_POINT('Ctrl Pts',(4.41844002242372,-0.31943490727715,7.91254580530321));
#54486=CARTESIAN_POINT('Ctrl Pts',(4.39079099009392,-0.158333333333328,
7.89416363326185));
#54487=CARTESIAN_POINT('Ctrl Pts',(4.39467503626453,0.15833333333333,7.86825657552279));
#54488=CARTESIAN_POINT('Ctrl Pts',(4.42614665727086,0.319434907277158,7.86098063695745));
#54489=CARTESIAN_POINT('Ctrl Pts',(4.50051285189156,0.636309800095188,7.84266468354586));
#54490=CARTESIAN_POINT('Ctrl Pts',(4.56342960718383,0.794772684000817,7.83690727777958));
#54491=CARTESIAN_POINT('Ctrl Pts',(4.66107975269782,1.06847604194511,7.81843533592283));
#54492=CARTESIAN_POINT('Ctrl Pts',(4.70528836283365,1.18514270861179,7.80929952045736));
#54493=CARTESIAN_POINT('Ctrl Pts',(4.75143645340681,1.30000000000004,7.79902370870333));
#54494=CARTESIAN_POINT('Ctrl Pts',(4.72917527752257,-1.30000000000241,8.02388370350364));
#54495=CARTESIAN_POINT('Ctrl Pts',(4.68746973293028,-1.18514270861341,8.0172359429138));
#54496=CARTESIAN_POINT('Ctrl Pts',(4.64742498238625,-1.06847604194593,8.00817660875066));
#54497=CARTESIAN_POINT('Ctrl Pts',(4.55875036419719,-0.794772684000832,
7.98167651713242));
#54498=CARTESIAN_POINT('Ctrl Pts',(4.50030656371858,-0.636309800095181,
7.95745763891306));
#54499=CARTESIAN_POINT('Ctrl Pts',(4.43433331923585,-0.31943490727715,7.92159031498128));
#54500=CARTESIAN_POINT('Ctrl Pts',(4.406226867755,-0.158333333333328,7.90202581739956));
#54501=CARTESIAN_POINT('Ctrl Pts',(4.41020012676641,0.15833333333333,7.87579960455339));
#54502=CARTESIAN_POINT('Ctrl Pts',(4.44224001576719,0.319434907277158,7.86926331378344));
#54503=CARTESIAN_POINT('Ctrl Pts',(4.51638761628297,0.636309800095189,7.85145424983308));
#54504=CARTESIAN_POINT('Ctrl Pts',(4.57950403080941,0.794772684000818,7.84655447181586));
#54505=CARTESIAN_POINT('Ctrl Pts',(4.67484086149381,1.06847604194511,7.82732413314217));
#54506=CARTESIAN_POINT('Ctrl Pts',(4.71752144744068,1.18514270861179,7.81747635695453));
#54507=CARTESIAN_POINT('Ctrl Pts',(4.76161483790889,1.30000000000004,7.80610490563682));
#54508=CARTESIAN_POINT('Ctrl Pts',(4.74172894757775,-1.30000000000241,8.03290675645279));
#54509=CARTESIAN_POINT('Ctrl Pts',(4.70251496843966,-1.18514270861341,8.0279335814323));
#54510=CARTESIAN_POINT('Ctrl Pts',(4.66432929110832,-1.06847604194593,8.01998788039034));
#54511=CARTESIAN_POINT('Ctrl Pts',(4.57848832033929,-0.794772684000832,
7.9947645916901));
#54512=CARTESIAN_POINT('Ctrl Pts',(4.51980586395291,-0.63630980009518,7.96957855615327));
#54513=CARTESIAN_POINT('Ctrl Pts',(4.45421672472527,-0.319434907277149,
7.93278122892627));
#54514=CARTESIAN_POINT('Ctrl Pts',(4.42551702402987,-0.158333333333328,
7.91186617049926));
#54515=CARTESIAN_POINT('Ctrl Pts',(4.42961312616382,0.15833333333333,7.88520561246107));
#54516=CARTESIAN_POINT('Ctrl Pts',(4.46235615477674,0.319434907277157,7.87959528850274));
#54517=CARTESIAN_POINT('Ctrl Pts',(4.53639625640105,0.636309800095188,7.86181163555795));
#54518=CARTESIAN_POINT('Ctrl Pts',(4.60003239837384,0.794772684000817,7.85702810288057));
#54519=CARTESIAN_POINT('Ctrl Pts',(4.69261022068255,1.0684760419451,7.83634193258301));
#54520=CARTESIAN_POINT('Ctrl Pts',(4.73339856048218,1.18514270861179,7.82551824541604));
#54521=CARTESIAN_POINT('Ctrl Pts',(4.77490173115041,1.30000000000004,7.81282514770576));
#54522=CARTESIAN_POINT('Ctrl Pts',(4.7564618490923,-1.3000000000024,8.04470262929104));
#54523=CARTESIAN_POINT('Ctrl Pts',(4.72034281583928,-1.1851427086134,8.04142414791164));
#54524=CARTESIAN_POINT('Ctrl Pts',(4.68447303677349,-1.06847604194592,8.03456109230727));
#54525=CARTESIAN_POINT('Ctrl Pts',(4.60218249844279,-0.794772684000827,
8.01042497736035));
#54526=CARTESIAN_POINT('Ctrl Pts',(4.54336090312408,-0.636309800095178,
7.98361406151805));
#54527=CARTESIAN_POINT('Ctrl Pts',(4.47807488179141,-0.31943490727715,7.94623932848582));
#54528=CARTESIAN_POINT('Ctrl Pts',(4.4482447018158,-0.158333333333327,7.92507344115463));
#54529=CARTESIAN_POINT('Ctrl Pts',(4.45228443140408,0.15833333333333,7.89856270081334));
#54530=CARTESIAN_POINT('Ctrl Pts',(4.48599321781917,0.319434907277156,7.89364309040658));
#54531=CARTESIAN_POINT('Ctrl Pts',(4.55983607370581,0.636309800095186,7.87615116563573));
#54532=CARTESIAN_POINT('Ctrl Pts',(4.62395355451121,0.794772684000817,7.87202113959796));
#54533=CARTESIAN_POINT('Ctrl Pts',(4.71318387302268,1.0684760419451,7.84979792163711));
#54534=CARTESIAN_POINT('Ctrl Pts',(4.75171193677337,1.18514270861179,7.83781462940899));
#54535=CARTESIAN_POINT('Ctrl Pts',(4.79014356570032,1.30000000000003,7.82346765255661));
#54536=CARTESIAN_POINT('Ctrl Pts',(4.7712546831859,-1.3000000000024,8.05621111744062));
#54537=CARTESIAN_POINT('Ctrl Pts',(4.73782127143929,-1.1851427086134,8.05576903410186));
#54538=CARTESIAN_POINT('Ctrl Pts',(4.70398052542868,-1.06847604194592,8.05080464184715));
#54539=CARTESIAN_POINT('Ctrl Pts',(4.62486060868961,-0.794772684000826,
8.02888846433499));
#54540=CARTESIAN_POINT('Ctrl Pts',(4.56590680565344,-0.636309800095177,
8.00062210173252));
#54541=CARTESIAN_POINT('Ctrl Pts',(4.50130284875518,-0.319434907277149,
7.96156634483499));
#54542=CARTESIAN_POINT('Ctrl Pts',(4.47101716764841,-0.158333333333327,
7.93805678516888));
#54543=CARTESIAN_POINT('Ctrl Pts',(4.47550015163245,0.158333333333329,7.91011414982581));
#54544=CARTESIAN_POINT('Ctrl Pts',(4.51032201344223,0.319434907277155,7.90534098618133));
#54545=CARTESIAN_POINT('Ctrl Pts',(4.5839491280442,0.636309800095185,7.88817234152425));
#54546=CARTESIAN_POINT('Ctrl Pts',(4.64809446566682,0.794772684000815,7.88619635929522));
#54547=CARTESIAN_POINT('Ctrl Pts',(4.73395633620671,1.0684760419451,7.86243688302862));
#54548=CARTESIAN_POINT('Ctrl Pts',(4.77030033016138,1.18514270861179,7.84900000871981));
#54549=CARTESIAN_POINT('Ctrl Pts',(4.80582189580988,1.30000000000003,7.83241085700264));
#54550=CARTESIAN_POINT('Ctrl Pts',(4.78614006404298,-1.3000000000024,8.06749734457243));
#54551=CARTESIAN_POINT('Ctrl Pts',(4.7558739845875,-1.18514270861339,8.06852826690951));
#54552=CARTESIAN_POINT('Ctrl Pts',(4.72435205105478,-1.06847604194592,8.06463278387327));
#54553=CARTESIAN_POINT('Ctrl Pts',(4.64862880450213,-0.794772684000822,
8.04425245683455));
#54554=CARTESIAN_POINT('Ctrl Pts',(4.58905049079883,-0.636309800095173,
8.01579961384292));
#54555=CARTESIAN_POINT('Ctrl Pts',(4.52465769933224,-0.319434907277147,
7.97644430868896));
#54556=CARTESIAN_POINT('Ctrl Pts',(4.49360222816118,-0.158333333333326,
7.95160804540723));
#54557=CARTESIAN_POINT('Ctrl Pts',(4.49801779013193,0.158333333333329,7.92388996056146));
#54558=CARTESIAN_POINT('Ctrl Pts',(4.53341734858637,0.319434907277155,7.92106635405216));
#54559=CARTESIAN_POINT('Ctrl Pts',(4.60694991064819,0.636309800095182,7.90384333626878));
#54560=CARTESIAN_POINT('Ctrl Pts',(4.67213697337497,0.79477268400081,7.90064758224056));
#54561=CARTESIAN_POINT('Ctrl Pts',(4.7547849514279,1.06847604194509,7.87493106055155));
#54562=CARTESIAN_POINT('Ctrl Pts',(4.7888369662119,1.18514270861178,7.86045823849655));
#54563=CARTESIAN_POINT('Ctrl Pts',(4.8211657484902,1.30000000000002,7.84264432373467));
#54564=CARTESIAN_POINT('Ctrl Pts',(4.80572350694021,-1.30000000000239,8.08315709719347));
#54565=CARTESIAN_POINT('Ctrl Pts',(4.77908700046572,-1.18514270861339,8.08778233032985));
#54566=CARTESIAN_POINT('Ctrl Pts',(4.75031148872691,-1.06847604194591,8.08626823027757));
#54567=CARTESIAN_POINT('Ctrl Pts',(4.678892770022,-0.794772684000819,8.06858726842701));
#54568=CARTESIAN_POINT('Ctrl Pts',(4.61928686686011,-0.636309800095172,
8.03774084106113));
#54569=CARTESIAN_POINT('Ctrl Pts',(4.55560515980317,-0.319434907277147,
7.9968316679897));
#54570=CARTESIAN_POINT('Ctrl Pts',(4.52350426881947,-0.158333333333326,
7.97033427815847));
#54571=CARTESIAN_POINT('Ctrl Pts',(4.52826408571188,0.158333333333328,7.94154897326003));
#54572=CARTESIAN_POINT('Ctrl Pts',(4.56517584864967,0.319434907277153,7.93885087863263));
#54573=CARTESIAN_POINT('Ctrl Pts',(4.63844896451369,0.63630980009518,7.92196196446686));
#54574=CARTESIAN_POINT('Ctrl Pts',(4.70380856892106,0.794772684000809,7.92110560016767));
#54575=CARTESIAN_POINT('Ctrl Pts',(4.78201031557717,1.06847604194509,7.89325959006359));
#54576=CARTESIAN_POINT('Ctrl Pts',(4.81315056856757,1.18514270861178,7.87690867767859));
#54577=CARTESIAN_POINT('Ctrl Pts',(4.84158043608123,1.30000000000002,7.85626035888629));
#54578=CARTESIAN_POINT('Ctrl Pts',(4.8212811930343,-1.30000000000238,8.09687619887558));
#54579=CARTESIAN_POINT('Ctrl Pts',(4.79789839802072,-1.18514270861338,8.10352243427901));
#54580=CARTESIAN_POINT('Ctrl Pts',(4.77153676353432,-1.06847604194591,8.10340154917221));
#54581=CARTESIAN_POINT('Ctrl Pts',(4.70375439914706,-0.794772684000816,
8.08748887825612));
#54582=CARTESIAN_POINT('Ctrl Pts',(4.6437836694552,-0.636309800095168,8.05567077476759));
#54583=CARTESIAN_POINT('Ctrl Pts',(4.58042492723703,-0.319434907277145,
8.01425946128189));
#54584=CARTESIAN_POINT('Ctrl Pts',(4.54732450489343,-0.158333333333325,
7.98688135529432));
#54585=CARTESIAN_POINT('Ctrl Pts',(4.55217177108714,0.158333333333327,7.957862440906));
#54586=CARTESIAN_POINT('Ctrl Pts',(4.59014492374784,0.319434907277152,7.95586253562142));
#54587=CARTESIAN_POINT('Ctrl Pts',(4.66332532960197,0.636309800095177,7.93889586442583));
#54588=CARTESIAN_POINT('Ctrl Pts',(4.72925564548018,0.794772684000805,7.93852029008944));
#54589=CARTESIAN_POINT('Ctrl Pts',(4.8040169197097,1.06847604194509,7.90843996467499));
#54590=CARTESIAN_POINT('Ctrl Pts',(4.83280848967938,1.18514270861177,7.89054411235512));
#54591=CARTESIAN_POINT('Ctrl Pts',(4.85803024418299,1.30000000000001,7.86777306600139));
#54592=CARTESIAN_POINT('Ctrl Pts',(4.83597411107337,-1.30000000000238,8.10851922151873));
#54593=CARTESIAN_POINT('Ctrl Pts',(4.81534154679997,-1.18514270861338,8.11774719602154));
#54594=CARTESIAN_POINT('Ctrl Pts',(4.79102914000993,-1.0684760419459,8.11941808524342));
#54595=CARTESIAN_POINT('Ctrl Pts',(4.72636144428147,-0.794772684000813,
8.10581979481759));
#54596=CARTESIAN_POINT('Ctrl Pts',(4.66610399033152,-0.636309800095166,
8.07295558482936));
#54597=CARTESIAN_POINT('Ctrl Pts',(4.60315685786802,-0.319434907277144,
8.03076446959183));
#54598=CARTESIAN_POINT('Ctrl Pts',(4.56938641996014,-0.158333333333324,
8.00187873773164));
#54599=CARTESIAN_POINT('Ctrl Pts',(4.57440911732778,0.158333333333327,7.97237130554391));
#54600=CARTESIAN_POINT('Ctrl Pts',(4.61325945310722,0.319434907277151,7.97127415946121));
#54601=CARTESIAN_POINT('Ctrl Pts',(4.68632094515445,0.636309800095175,7.95432920870802));
#54602=CARTESIAN_POINT('Ctrl Pts',(4.75276714075305,0.794772684000803,7.95446014804467));
#54603=CARTESIAN_POINT('Ctrl Pts',(4.82435463557553,1.06847604194508,7.92231770894031));
#54604=CARTESIAN_POINT('Ctrl Pts',(4.85098494139824,1.18514270861177,7.90297455592258));
#54605=CARTESIAN_POINT('Ctrl Pts',(4.87325797911311,1.30000000000001,7.87820152078065));
#54606=CARTESIAN_POINT('Ctrl Pts',(4.84561392829011,-1.30000000000238,8.11673827460531));
#54607=CARTESIAN_POINT('Ctrl Pts',(4.82702732226811,-1.18514270861338,8.12708722672374));
#54608=CARTESIAN_POINT('Ctrl Pts',(4.80420024520761,-1.0684760419459,8.12961304670658));
#54609=CARTESIAN_POINT('Ctrl Pts',(4.74166879425471,-0.794772684000813,
8.11737519591012));
#54610=CARTESIAN_POINT('Ctrl Pts',(4.68085372121343,-0.636309800095166,
8.08482027135769));
#54611=CARTESIAN_POINT('Ctrl Pts',(4.61809033912233,-0.319434907277144,
8.04236144674853));
#54612=CARTESIAN_POINT('Ctrl Pts',(4.58394762600498,-0.158333333333324,
8.01228869742108));
#54613=CARTESIAN_POINT('Ctrl Pts',(4.58920734463784,0.158333333333327,7.98211214185068));
#54614=CARTESIAN_POINT('Ctrl Pts',(4.62883416859871,0.31943490727715,7.98104157223286));
#54615=CARTESIAN_POINT('Ctrl Pts',(4.70185414805629,0.636309800095174,7.9640021533145));
#54616=CARTESIAN_POINT('Ctrl Pts',(4.76848548414612,0.794772684000801,7.96494516785146));
#54617=CARTESIAN_POINT('Ctrl Pts',(4.83789792807451,1.06847604194508,7.93160930152804));
#54618=CARTESIAN_POINT('Ctrl Pts',(4.86307582681345,1.18514270861177,7.91133835210395));
#54619=CARTESIAN_POINT('Ctrl Pts',(4.88338554929927,1.30000000000001,7.8852263145716));
#54620=CARTESIAN_POINT('Ctrl Pts',(4.85873584770498,-1.30000000000237,8.1283093707173));
#54621=CARTESIAN_POINT('Ctrl Pts',(4.84257246164534,-1.18514270861337,8.14123666706622));
#54622=CARTESIAN_POINT('Ctrl Pts',(4.82158036271301,-1.0684760419459,8.14548959140894));
#54623=CARTESIAN_POINT('Ctrl Pts',(4.76192912200796,-0.794772684000808,
8.13527516279878));
#54624=CARTESIAN_POINT('Ctrl Pts',(4.70109465465751,-0.636309800095162,
8.10115575541734));
#54625=CARTESIAN_POINT('Ctrl Pts',(4.6388360645949,-0.319434907277142,8.057667241152));
#54626=CARTESIAN_POINT('Ctrl Pts',(4.60413233863675,-0.158333333333323,
8.0260704578481));
#54627=CARTESIAN_POINT('Ctrl Pts',(4.60945901730333,0.158333333333325,7.9957454086737));
#54628=CARTESIAN_POINT('Ctrl Pts',(4.64966106351442,0.319434907277146,7.99617478942981));
#54629=CARTESIAN_POINT('Ctrl Pts',(4.72242009293445,0.636309800095168,7.97960917517307));
#54630=CARTESIAN_POINT('Ctrl Pts',(4.78943626148876,0.794772684000797,7.98127127696966));
#54631=CARTESIAN_POINT('Ctrl Pts',(4.85606191180836,1.06847604194508,7.94569709957012));
#54632=CARTESIAN_POINT('Ctrl Pts',(4.87937077991199,1.18514270861176,7.92377780620357));
#54633=CARTESIAN_POINT('Ctrl Pts',(4.89714874081958,1.3,7.89533796271355));
#54634=CARTESIAN_POINT('Ctrl Pts',(4.8706912457249,-1.30000000000236,8.13874397736797));
#54635=CARTESIAN_POINT('Ctrl Pts',(4.85688868177773,-1.18514270861336,8.15357144495233));
#54636=CARTESIAN_POINT('Ctrl Pts',(4.83764494620884,-1.06847604194588,8.1591651370575));
#54637=CARTESIAN_POINT('Ctrl Pts',(4.7806178724,-0.794772684000799,8.15075581626738));
#54638=CARTESIAN_POINT('Ctrl Pts',(4.71942401154056,-0.636309800095158,
8.11613756897579));
#54639=CARTESIAN_POINT('Ctrl Pts',(4.65752261305664,-0.31943490727714,8.07199190908468));
#54640=CARTESIAN_POINT('Ctrl Pts',(4.62236539069558,-0.158333333333322,
8.0388868963487));
#54641=CARTESIAN_POINT('Ctrl Pts',(4.62787715410413,0.158333333333325,8.00806696958337));
#54642=CARTESIAN_POINT('Ctrl Pts',(4.668801765522,0.319434907277146,8.00925309041465));
#54643=CARTESIAN_POINT('Ctrl Pts',(4.7414095381692,0.636309800095166,7.99285929145396));
#54644=CARTESIAN_POINT('Ctrl Pts',(4.80871779191284,0.794772684000793,7.99533965620724));
#54645=CARTESIAN_POINT('Ctrl Pts',(4.87272998284456,1.06847604194507,7.95798539139597));
#54646=CARTESIAN_POINT('Ctrl Pts',(4.89429019408294,1.18514270861175,7.93472762094081));
#54647=CARTESIAN_POINT('Ctrl Pts',(4.9097021109908,1.29999999999999,7.90438135715535));
#54648=CARTESIAN_POINT('Ctrl Pts',(4.87889684647338,-1.30000000000235,8.14643349039401));
#54649=CARTESIAN_POINT('Ctrl Pts',(4.86655780869544,-1.18514270861336,8.16306500747547));
#54650=CARTESIAN_POINT('Ctrl Pts',(4.84844221023227,-1.06847604194588,8.16983725152211));
#54651=CARTESIAN_POINT('Ctrl Pts',(4.79324654298962,-0.7947726840008,8.16270559700147));
#54652=CARTESIAN_POINT('Ctrl Pts',(4.73225201339823,-0.636309800095157,
8.12659044263502));
#54653=CARTESIAN_POINT('Ctrl Pts',(4.67064679511124,-0.31943490727714,8.08190437626722));
#54654=CARTESIAN_POINT('Ctrl Pts',(4.6348639598759,-0.158333333333322,8.04859156898635));
#54655=CARTESIAN_POINT('Ctrl Pts',(4.64046671223474,0.158333333333324,8.01753912185134));
#54656=CARTESIAN_POINT('Ctrl Pts',(4.68202664064609,0.319434907277145,8.01890020375431));
#54657=CARTESIAN_POINT('Ctrl Pts',(4.75468914238488,0.636309800095165,8.00216643618904));
#54658=CARTESIAN_POINT('Ctrl Pts',(4.82240570180082,0.794772684000792,8.0046151258808));
#54659=CARTESIAN_POINT('Ctrl Pts',(4.88460734747703,1.06847604194507,7.96596225571329));
#54660=CARTESIAN_POINT('Ctrl Pts',(4.90490036841996,1.18514270861175,7.94189610211271));
#54661=CARTESIAN_POINT('Ctrl Pts',(4.91856162269072,1.29999999999999,7.91049519017706));
#54662=CARTESIAN_POINT('Ctrl Pts',(4.88305998021748,-1.30000000000235,8.15012560460764));
#54663=CARTESIAN_POINT('Ctrl Pts',(4.87151822466341,-1.18514270861335,8.16749476044765));
#54664=CARTESIAN_POINT('Ctrl Pts',(4.85399470886098,-1.06847604194588,8.17478603452684));
#54665=CARTESIAN_POINT('Ctrl Pts',(4.79969281896955,-0.794772684000798,
8.16834841332337));
#54666=CARTESIAN_POINT('Ctrl Pts',(4.73859249823662,-0.636309800095156,
8.13200389578888));
#54667=CARTESIAN_POINT('Ctrl Pts',(4.67711069858125,-0.319434907277139,
8.08710327929875));
#54668=CARTESIAN_POINT('Ctrl Pts',(4.64116622640158,-0.158333333333322,
8.05328987531924));
#54669=CARTESIAN_POINT('Ctrl Pts',(4.64682226011323,0.158333333333324,8.02210546727675));
#54670=CARTESIAN_POINT('Ctrl Pts',(4.68861499160051,0.319434907277145,8.02378241015381));
#54671=CARTESIAN_POINT('Ctrl Pts',(4.76122617498029,0.636309800095164,8.00710189634627));
#54672=CARTESIAN_POINT('Ctrl Pts',(4.8290550323816,0.79477268400079,8.00980623275754));
#54673=CARTESIAN_POINT('Ctrl Pts',(4.8903791407941,1.06847604194507,7.970423587409));
#54674=CARTESIAN_POINT('Ctrl Pts',(4.91008229512971,1.18514270861175,7.94582590060862));
#54675=CARTESIAN_POINT('Ctrl Pts',(4.92294366955132,1.29999999999998,7.91367781490841));
#54676=CARTESIAN_POINT('Ctrl Pts',(4.88514455500464,-1.30000000000235,8.15196328232576));
#54677=CARTESIAN_POINT('Ctrl Pts',(4.87400495537845,-1.18514270861335,8.16969222727159));
#54678=CARTESIAN_POINT('Ctrl Pts',(4.85677856536373,-1.06847604194588,8.17724016881156));
#54679=CARTESIAN_POINT('Ctrl Pts',(4.80292045484665,-0.794772684000798,
8.17115726915921));
#54680=CARTESIAN_POINT('Ctrl Pts',(4.74175272104858,-0.636309800095156,
8.13473473304));
#54681=CARTESIAN_POINT('Ctrl Pts',(4.68032963434567,-0.319434907277139,
8.08973453534491));
#54682=CARTESIAN_POINT('Ctrl Pts',(4.64431371975998,-0.158333333333322,
8.05564697256633));
#54683=CARTESIAN_POINT('Ctrl Pts',(4.64999636724652,0.158333333333324,8.02439766002777));
#54684=CARTESIAN_POINT('Ctrl Pts',(4.69190028777524,0.319434907277145,8.02624679249682));
#54685=CARTESIAN_POINT('Ctrl Pts',(4.76448021785442,0.636309800095164,8.00960915225664));
#54686=CARTESIAN_POINT('Ctrl Pts',(4.83235724904279,0.794772684000791,8.01246456073939));
#54687=CARTESIAN_POINT('Ctrl Pts',(4.89324610269253,1.06847604194507,7.97270739073841));
#54688=CARTESIAN_POINT('Ctrl Pts',(4.91265872028842,1.18514270861175,7.94783152281172));
#54689=CARTESIAN_POINT('Ctrl Pts',(4.92512742688961,1.29999999999999,7.91528919270343));
#54690=CARTESIAN_POINT('Ctrl Pts',(4.88633804800046,-1.30000000000235,8.15300735731721));
#54691=CARTESIAN_POINT('Ctrl Pts',(4.87543043244414,-1.18514270861335,8.17093640497652));
#54692=CARTESIAN_POINT('Ctrl Pts',(4.85837471443863,-1.06847604194588,8.17862880124875));
#54693=CARTESIAN_POINT('Ctrl Pts',(4.80476924728013,-0.794772684000798,
8.17275106295702));
#54694=CARTESIAN_POINT('Ctrl Pts',(4.74355576934846,-0.636309800095156,
8.13630239380284));
#54695=CARTESIAN_POINT('Ctrl Pts',(4.6821652161533,-0.319434907277139,8.0912477084203));
#54696=CARTESIAN_POINT('Ctrl Pts',(4.64611367300213,-0.158333333333322,
8.05698977168253));
#54697=CARTESIAN_POINT('Ctrl Pts',(4.65181164585589,0.158333333333324,8.02570319836857));
#54698=CARTESIAN_POINT('Ctrl Pts',(4.69377602562051,0.319434907277145,8.02765895368757));
#54699=CARTESIAN_POINT('Ctrl Pts',(4.76633527724332,0.636309800095164,8.0110538625209));
#54700=CARTESIAN_POINT('Ctrl Pts',(4.83423660945324,0.79477268400079,8.01400531325613));
#54701=CARTESIAN_POINT('Ctrl Pts',(4.89487784889872,1.06847604194507,7.97403099752843));
#54702=CARTESIAN_POINT('Ctrl Pts',(4.91412607104847,1.18514270861175,7.9489914413801));
#54703=CARTESIAN_POINT('Ctrl Pts',(4.92637316977141,1.29999999999998,7.91621572916757));
#54704=CARTESIAN_POINT('Ctrl Pts',(4.89648125291073,-1.30000000000236,8.1618847443129));
#54705=CARTESIAN_POINT('Ctrl Pts',(4.88755289139152,-1.18514270861336,8.1814935536347));
#54706=CARTESIAN_POINT('Ctrl Pts',(4.8719501946499,-1.06847604194589,8.19040611650862));
#54707=CARTESIAN_POINT('Ctrl Pts',(4.82048579430827,-0.794772684000802,
8.18628545062815));
#54708=CARTESIAN_POINT('Ctrl Pts',(4.7588575532274,-0.636309800095158,8.14967904496894));
#54709=CARTESIAN_POINT('Ctrl Pts',(4.69772882947847,-0.31943490727714,8.10419982071705));
#54710=CARTESIAN_POINT('Ctrl Pts',(4.66137129118492,-0.158333333333322,
8.06850588104074));
#54711=CARTESIAN_POINT('Ctrl Pts',(4.66720410790064,0.158333333333325,8.03689346131535));
#54712=CARTESIAN_POINT('Ctrl Pts',(4.70970157980417,0.319434907277146,8.03970566614566));
#54713=CARTESIAN_POINT('Ctrl Pts',(4.78208575622587,0.636309800095167,8.02337817109365));
#54714=CARTESIAN_POINT('Ctrl Pts',(4.85017318446032,0.794772684000793,8.02719981142593));
#54715=CARTESIAN_POINT('Ctrl Pts',(4.90870759397174,1.06847604194507,7.98539139166514));
#54716=CARTESIAN_POINT('Ctrl Pts',(4.92656098233666,1.18514270861175,7.95895753979858));
#54717=CARTESIAN_POINT('Ctrl Pts',(4.93693038210267,1.29999999999999,7.92418715182528));
#54718=CARTESIAN_POINT('Ctrl Pts',(4.91551177580483,-1.30000000000243,8.1796774361804));
#54719=CARTESIAN_POINT('Ctrl Pts',(4.90997910059319,-1.18514270861342,8.2034115442133));
#54720=CARTESIAN_POINT('Ctrl Pts',(4.89695697654872,-1.06847604194594,8.21511380608156));
#54721=CARTESIAN_POINT('Ctrl Pts',(4.84957113987627,-0.794772684000837,
8.21435240042376));
#54722=CARTESIAN_POINT('Ctrl Pts',(4.7880382363761,-0.636309800095189,8.17525965214434));
#54723=CARTESIAN_POINT('Ctrl Pts',(4.72756392935862,-0.319434907277156,
8.12863812941445));
#54724=CARTESIAN_POINT('Ctrl Pts',(4.69012508813819,-0.158333333333331,
8.09152310390475));
#54725=CARTESIAN_POINT('Ctrl Pts',(4.69616504778515,0.158333333333333,8.05942743143656));
#54726=CARTESIAN_POINT('Ctrl Pts',(4.73980031308552,0.319434907277166,8.06355300046823));
#54727=CARTESIAN_POINT('Ctrl Pts',(4.81225887622818,0.636309800095201,8.046618523019));
#54728=CARTESIAN_POINT('Ctrl Pts',(4.8815204951006,0.794772684000832,8.04975140675556));
#54729=CARTESIAN_POINT('Ctrl Pts',(4.93590306301374,1.06847604194512,8.00490599430512));
#54730=CARTESIAN_POINT('Ctrl Pts',(4.9508094610885,1.18514270861181,7.97668237716761));
#54731=CARTESIAN_POINT('Ctrl Pts',(4.95708205866118,1.30000000000005,7.93964706025608));
#54732=CARTESIAN_POINT('Ctrl Pts',(4.9342581816127,-1.30000000000244,8.19708426160756));
#54733=CARTESIAN_POINT('Ctrl Pts',(4.93221572521055,-1.18514270861343,8.22447422101744));
#54734=CARTESIAN_POINT('Ctrl Pts',(4.92179501815014,-1.06847604194595,8.23874548314703));
#54735=CARTESIAN_POINT('Ctrl Pts',(4.87836566510154,-0.794772684000851,
8.24140813851867));
#54736=CARTESIAN_POINT('Ctrl Pts',(4.81647889550278,-0.636309800095196,
8.20100449682226));
#54737=CARTESIAN_POINT('Ctrl Pts',(4.75652394679049,-0.319434907277159,
8.15359245070489));
#54738=CARTESIAN_POINT('Ctrl Pts',(4.7181759471255,-0.158333333333332,8.11472494346454));
#54739=CARTESIAN_POINT('Ctrl Pts',(4.72452210841152,0.158333333333334,8.08191100418775));
#54740=CARTESIAN_POINT('Ctrl Pts',(4.76953814964653,0.319434907277167,8.08661121585654));
#54741=CARTESIAN_POINT('Ctrl Pts',(4.84176412499727,0.636309800095206,8.0699403196767));
#54742=CARTESIAN_POINT('Ctrl Pts',(4.91110009717076,0.79477268400084,8.07544025046478));
#54743=CARTESIAN_POINT('Ctrl Pts',(4.96159302088875,1.06847604194513,8.02697642301351));
#54744=CARTESIAN_POINT('Ctrl Pts',(4.97396758428922,1.18514270861182,7.99590387471389));
#54745=CARTESIAN_POINT('Ctrl Pts',(4.97686019535986,1.30000000000007,7.95473697325649));
#54746=CARTESIAN_POINT('Ctrl Pts',(4.94346631687566,-1.30000000000244,8.20619135799069));
#54747=CARTESIAN_POINT('Ctrl Pts',(4.94321747389921,-1.18514270861343,8.23526699291014));
#54748=CARTESIAN_POINT('Ctrl Pts',(4.93412052317187,-1.06847604194595,8.25074967063335));
#54749=CARTESIAN_POINT('Ctrl Pts',(4.89266384819064,-0.794772684000851,
8.25511530308793));
#54750=CARTESIAN_POINT('Ctrl Pts',(4.83045152777307,-0.636309800095196,
8.21442603970566));
#54751=CARTESIAN_POINT('Ctrl Pts',(4.77077828071587,-0.319434907277159,
8.16657178332084));
#54752=CARTESIAN_POINT('Ctrl Pts',(4.73214233677919,-0.158333333333332,
8.12643424340246));
#54753=CARTESIAN_POINT('Ctrl Pts',(4.73867559286303,0.158333333333334,8.09318929264053));
#54754=CARTESIAN_POINT('Ctrl Pts',(4.78422175451366,0.319434907277167,8.0985897035147));
#54755=CARTESIAN_POINT('Ctrl Pts',(4.85643493010519,0.636309800095206,8.08176584863399));
#54756=CARTESIAN_POINT('Ctrl Pts',(4.92620237914194,0.79477268400084,8.08735069514893));
#54757=CARTESIAN_POINT('Ctrl Pts',(4.9747053048224,1.06847604194513,8.03725889790454));
#54758=CARTESIAN_POINT('Ctrl Pts',(4.98569765033206,1.18514270861182,8.00512172787457));
#54759=CARTESIAN_POINT('Ctrl Pts',(4.98668722203483,1.30000000000007,7.9625302707577));
#54760=CARTESIAN_POINT('',(4.8959368873413,1.2,7.92959029267854));
#54761=CARTESIAN_POINT('Ctrl Pts',(4.8959368873413,1.2,7.92959029267854));
#54762=CARTESIAN_POINT('Ctrl Pts',(4.88797220813117,1.20916354636366,7.92086623504881));
#54763=CARTESIAN_POINT('Ctrl Pts',(4.88028989526128,1.21806687773866,7.91188259563126));
#54764=CARTESIAN_POINT('Ctrl Pts',(4.86522920737885,1.23542022164275,7.89477196315859));
#54765=CARTESIAN_POINT('Ctrl Pts',(4.86314220261871,1.23778099745235,7.89270625656617));
#54766=CARTESIAN_POINT('Ctrl Pts',(4.84481687043038,1.25867329971331,7.87296100721959));
#54767=CARTESIAN_POINT('Ctrl Pts',(4.83773131952392,1.26674820983433,7.86524036225158));
#54768=CARTESIAN_POINT('Ctrl Pts',(4.82529292629485,1.28086872210545,7.85193070389807));
#54769=CARTESIAN_POINT('Ctrl Pts',(4.81441133228405,1.29318854035898,7.84038199481636));
#54770=CARTESIAN_POINT('Ctrl Pts',(4.80835060740606,1.29999999999429,7.83424319965858));
#54771=CARTESIAN_POINT('',(4.87041241537771,0.653834841366681,8.0840717752332));
#54772=CARTESIAN_POINT('Ctrl Pts',(4.87041241541545,0.653834841365399,8.08407177523491));
#54773=CARTESIAN_POINT('Ctrl Pts',(4.87329721488191,0.717497006726158,8.06817921590771));
#54774=CARTESIAN_POINT('Ctrl Pts',(4.87561886639402,0.764618542304357,8.05505318984721));
#54775=CARTESIAN_POINT('Ctrl Pts',(4.88438527422149,0.949828857079461,8.0040620818735));
#54776=CARTESIAN_POINT('Ctrl Pts',(4.88934246800722,1.05665635942843,7.9738423354926));
#54777=CARTESIAN_POINT('Ctrl Pts',(4.8959368873413,1.2,7.92959029267854));
#54778=CARTESIAN_POINT('',(4.84356468978474,-0.653834841531101,8.22097066356995));
#54779=CARTESIAN_POINT('Ctrl Pts',(4.84356468978474,-0.653834841531103,
8.22097066356995));
#54780=CARTESIAN_POINT('Ctrl Pts',(4.81028563170247,-0.575993226556318,
8.19606516572056));
#54781=CARTESIAN_POINT('Ctrl Pts',(4.78259195720601,-0.493634718961504,
8.17437906484961));
#54782=CARTESIAN_POINT('Ctrl Pts',(4.74428736208887,-0.338122806465111,
8.14129310529133));
#54783=CARTESIAN_POINT('Ctrl Pts',(4.73158435908654,-0.265648779501229,
8.12870181591131));
#54784=CARTESIAN_POINT('Ctrl Pts',(4.71756129813914,-0.129709195779501,
8.10877449802887));
#54785=CARTESIAN_POINT('Ctrl Pts',(4.71484216847727,-0.0666211038089427,
8.10096227158569));
#54786=CARTESIAN_POINT('Ctrl Pts',(4.71704128756279,0.0595424094985919,
8.08781794729412));
#54787=CARTESIAN_POINT('Ctrl Pts',(4.72195866570481,0.122770513587566,8.08238767852916));
#54788=CARTESIAN_POINT('Ctrl Pts',(4.74093133359303,0.260121498042269,8.07400881902309));
#54789=CARTESIAN_POINT('Ctrl Pts',(4.75649446970959,0.333942046842514,8.07169269259132));
#54790=CARTESIAN_POINT('Ctrl Pts',(4.80133469428488,0.491203290822365,8.07254015000573));
#54791=CARTESIAN_POINT('Ctrl Pts',(4.83265376689795,0.574345776646004,8.07653115452104));
#54792=CARTESIAN_POINT('Ctrl Pts',(4.87041241535288,0.653834841383564,8.08407177517955));
#54793=CARTESIAN_POINT('',(4.8579715305892,-1.2,8.1500592655118));
#54794=CARTESIAN_POINT('Ctrl Pts',(4.8579715305892,-1.2,8.1500592655118));
#54795=CARTESIAN_POINT('Ctrl Pts',(4.85616916586142,-1.14986030831313,8.15927536060516));
#54796=CARTESIAN_POINT('Ctrl Pts',(4.85301485103969,-1.06105460662833,8.17530456062274));
#54797=CARTESIAN_POINT('Ctrl Pts',(4.84589300490481,-0.792168471237582,
8.2099540488437));
#54798=CARTESIAN_POINT('Ctrl Pts',(4.84486899479601,-0.738395515500054,
8.21478293857185));
#54799=CARTESIAN_POINT('Ctrl Pts',(4.84356468978474,-0.653834841531101,
8.22097066356995));
#54800=CARTESIAN_POINT('Ctrl Pts',(4.77352143851608,-1.29999999999999,8.05790038817305));
#54801=CARTESIAN_POINT('Ctrl Pts',(4.78821579301464,-1.28289249508473,8.0728526865888));
#54802=CARTESIAN_POINT('Ctrl Pts',(4.80235089926343,-1.26612407112286,8.08872140664403));
#54803=CARTESIAN_POINT('Ctrl Pts',(4.82249641224789,-1.2423446920112,8.11029336074994));
#54804=CARTESIAN_POINT('Ctrl Pts',(4.82684436345377,-1.23728814171469,8.11454897743682));
#54805=CARTESIAN_POINT('Ctrl Pts',(4.84402176769152,-1.21675291282038,8.13403542652456));
#54806=CARTESIAN_POINT('Ctrl Pts',(4.85107260119958,-1.20833011795947,8.14193421309319));
#54807=CARTESIAN_POINT('Ctrl Pts',(4.8579715305892,-1.2,8.1500592655118));
#54808=CARTESIAN_POINT('Origin',(0.,1.25,7.2));
#54809=CARTESIAN_POINT('Origin',(0.,1.2,7.2));
#54810=CARTESIAN_POINT('Origin',(0.,0.92691742076555,7.2));
#54811=CARTESIAN_POINT('Origin',(0.,0.653834841531101,7.2));
#54812=CARTESIAN_POINT('Origin',(0.,0.,7.2));
#54813=CARTESIAN_POINT('Origin',(0.,-0.653834841531101,7.2));
#54814=CARTESIAN_POINT('Origin',(0.,-0.926917420765551,7.2));
#54815=CARTESIAN_POINT('Origin',(0.,-1.2,7.2));
#54816=CARTESIAN_POINT('Origin',(0.,-1.25,7.2));
#54817=CARTESIAN_POINT('Ctrl Pts',(4.86571446294981,-1.30000000000085,8.53166235559583));
#54818=CARTESIAN_POINT('Ctrl Pts',(4.88213395050881,-1.18514270861236,8.49235062834033));
#54819=CARTESIAN_POINT('Ctrl Pts',(4.88516330785635,-1.06847604194541,8.45852087292604));
#54820=CARTESIAN_POINT('Ctrl Pts',(4.86122784987519,-0.794772684000851,
8.39303182191765));
#54821=CARTESIAN_POINT('Ctrl Pts',(4.79522055198899,-0.636309800095197,
8.36975685506468));
#54822=CARTESIAN_POINT('Ctrl Pts',(4.73609341170194,-0.319434907277159,
8.32501575423208));
#54823=CARTESIAN_POINT('Ctrl Pts',(4.69228837762394,-0.158333333333332,
8.31142398216115));
#54824=CARTESIAN_POINT('Ctrl Pts',(4.69984189087714,0.158333333333334,8.2783958937552));
#54825=CARTESIAN_POINT('Ctrl Pts',(4.75146299021043,0.319434907277167,8.25744308062087));
#54826=CARTESIAN_POINT('Ctrl Pts',(4.82544129359938,0.636309800095206,8.23799733826065));
#54827=CARTESIAN_POINT('Ctrl Pts',(4.89882489071899,0.79477268400084,8.22612987688632));
#54828=CARTESIAN_POINT('Ctrl Pts',(4.93492178514811,1.06847604194527,8.24698002939988));
#54829=CARTESIAN_POINT('Ctrl Pts',(4.93693489080205,1.1851427086121,8.26482422250729));
#54830=CARTESIAN_POINT('Ctrl Pts',(4.92533609403332,1.30000000000048,8.29148735027329));
#54831=CARTESIAN_POINT('Ctrl Pts',(4.85356720775251,-1.30000000000085,8.53478487530141));
#54832=CARTESIAN_POINT('Ctrl Pts',(4.86766876337789,-1.18514270861236,8.49600050856059));
#54833=CARTESIAN_POINT('Ctrl Pts',(4.86900238119364,-1.06847604194541,8.46258113483096));
#54834=CARTESIAN_POINT('Ctrl Pts',(4.84258681457994,-0.794772684000851,
8.39776990311183));
#54835=CARTESIAN_POINT('Ctrl Pts',(4.77700822871636,-0.636309800095197,
8.37459285932004));
#54836=CARTESIAN_POINT('Ctrl Pts',(4.71780718134389,-0.319434907277159,
8.32998628707835));
#54837=CARTESIAN_POINT('Ctrl Pts',(4.67477123304741,-0.158333333333332,
8.3159704706055));
#54838=CARTESIAN_POINT('Ctrl Pts',(4.68232035773856,0.158333333333334,8.28341222909386));
#54839=CARTESIAN_POINT('Ctrl Pts',(4.73316183806893,0.319434907277167,8.26350253105835));
#54840=CARTESIAN_POINT('Ctrl Pts',(4.80721762558706,0.636309800095206,8.2445753462594));
#54841=CARTESIAN_POINT('Ctrl Pts',(4.88018764438341,0.79477268400084,8.23283639981901));
#54842=CARTESIAN_POINT('Ctrl Pts',(4.91877933308295,1.06847604194527,8.25293316580915));
#54843=CARTESIAN_POINT('Ctrl Pts',(4.92249447744504,1.1851427086121,8.27020909591394));
#54844=CARTESIAN_POINT('Ctrl Pts',(4.91321985409419,1.30000000000048,8.29606181078497));
#54845=CARTESIAN_POINT('Ctrl Pts',(4.82936001910001,-1.30000000000095,8.54053438201199));
#54846=CARTESIAN_POINT('Ctrl Pts',(4.83869374469277,-1.18514270861245,8.50414804058056));
#54847=CARTESIAN_POINT('Ctrl Pts',(4.83655611686211,-1.06847604194549,8.47229936964699));
#54848=CARTESIAN_POINT('Ctrl Pts',(4.8051166476979,-0.79477268400091,8.40920549509364));
#54849=CARTESIAN_POINT('Ctrl Pts',(4.74057070959264,-0.636309800095242,
8.38388404752927));
#54850=CARTESIAN_POINT('Ctrl Pts',(4.68126380914895,-0.319434907277181,
8.33894697122637));
#54851=CARTESIAN_POINT('Ctrl Pts',(4.6397195201453,-0.158333333333344,8.32499215906552));
#54852=CARTESIAN_POINT('Ctrl Pts',(4.64725601130599,0.158333333333346,8.29321406701575));
#54853=CARTESIAN_POINT('Ctrl Pts',(4.69655683600114,0.319434907277193,8.27451647045124));
#54854=CARTESIAN_POINT('Ctrl Pts',(4.7707668114283,0.636309800095254,8.25650478146261));
#54855=CARTESIAN_POINT('Ctrl Pts',(4.84288041121132,0.794772684000897,8.24580151540382));
#54856=CARTESIAN_POINT('Ctrl Pts',(4.88647885739907,1.06847604194535,8.26438230695372));
#54857=CARTESIAN_POINT('Ctrl Pts',(4.89361505177938,1.18514270861218,8.28037652552305));
#54858=CARTESIAN_POINT('Ctrl Pts',(4.88901528866695,1.30000000000057,8.30432202648592));
#54859=CARTESIAN_POINT('Ctrl Pts',(4.804847149059,-1.30000000000139,8.54644403858434));
#54860=CARTESIAN_POINT('Ctrl Pts',(4.80955580396485,-1.18514270861285,8.51043725219642));
#54861=CARTESIAN_POINT('Ctrl Pts',(4.8040269923979,-1.06847604194585,8.47900494843386));
#54862=CARTESIAN_POINT('Ctrl Pts',(4.76760373609304,-0.794772684001179,
8.41695800871827));
#54863=CARTESIAN_POINT('Ctrl Pts',(4.70385131375091,-0.636309800095458,
8.39270228722005));
#54864=CARTESIAN_POINT('Ctrl Pts',(4.64436342255841,-0.319434907277289,
8.34837684794173));
#54865=CARTESIAN_POINT('Ctrl Pts',(4.6043649205092,-0.158333333333397,8.33379951860146));
#54866=CARTESIAN_POINT('Ctrl Pts',(4.61189316275056,0.158333333333399,8.30253910350606));
#54867=CARTESIAN_POINT('Ctrl Pts',(4.65965294569226,0.319434907277298,8.28459752774881));
#54868=CARTESIAN_POINT('Ctrl Pts',(4.73400064132595,0.636309800095468,8.26781120582232));
#54869=CARTESIAN_POINT('Ctrl Pts',(4.80519641332386,0.794772684001165,8.25934293293309));
#54870=CARTESIAN_POINT('Ctrl Pts',(4.85384625361791,1.06847604194571,8.27653965866762));
#54871=CARTESIAN_POINT('Ctrl Pts',(4.86444620305697,1.18514270861259,8.29107480451648));
#54872=CARTESIAN_POINT('Ctrl Pts',(4.86458738872603,1.30000000000101,8.31270127084519));
#54873=CARTESIAN_POINT('Ctrl Pts',(4.79233830189581,-1.30000000000142,8.54935194863464));
#54874=CARTESIAN_POINT('Ctrl Pts',(4.79459546837754,-1.18514270861288,8.51436530006081));
#54875=CARTESIAN_POINT('Ctrl Pts',(4.78728007149443,-1.06847604194588,8.48361409219813));
#54876=CARTESIAN_POINT('Ctrl Pts',(4.74826550489687,-0.794772684001197,
8.42235736561713));
#54877=CARTESIAN_POINT('Ctrl Pts',(4.68502149708521,-0.636309800095474,
8.39740911729828));
#54878=CARTESIAN_POINT('Ctrl Pts',(4.6254874340275,-0.319434907277297,8.35277492053589));
#54879=CARTESIAN_POINT('Ctrl Pts',(4.58629839263221,-0.158333333333401,
8.33765864174457));
#54880=CARTESIAN_POINT('Ctrl Pts',(4.59381754228615,0.158333333333403,8.30673962323839));
#54881=CARTESIAN_POINT('Ctrl Pts',(4.64074037977057,0.319434907277307,8.28993872672475));
#54882=CARTESIAN_POINT('Ctrl Pts',(4.71515318994323,0.636309800095484,8.27362628256271));
#54883=CARTESIAN_POINT('Ctrl Pts',(4.78591880090055,0.794772684001185,8.26513493816583));
#54884=CARTESIAN_POINT('Ctrl Pts',(4.83716058558056,1.06847604194574,8.28161897342502));
#54885=CARTESIAN_POINT('Ctrl Pts',(4.84953046676123,1.18514270861262,8.29564628708797));
#54886=CARTESIAN_POINT('Ctrl Pts',(4.85208955922982,1.30000000000105,8.31656558634388));
#54887=CARTESIAN_POINT('Ctrl Pts',(4.79158070392031,-1.30000000000142,8.5495235549734));
#54888=CARTESIAN_POINT('Ctrl Pts',(4.79368911312494,-1.18514270861288,8.51459945078696));
#54889=CARTESIAN_POINT('Ctrl Pts',(4.78626529793112,-1.06847604194588,8.48389016235608));
#54890=CARTESIAN_POINT('Ctrl Pts',(4.74709345442893,-0.794772684001196,
8.42268263027507));
#54891=CARTESIAN_POINT('Ctrl Pts',(4.68388019310939,-0.636309800095473,
8.39769404782994));
#54892=CARTESIAN_POINT('Ctrl Pts',(4.62434337779062,-0.319434907277297,
8.35304004667076));
#54893=CARTESIAN_POINT('Ctrl Pts',(4.58520366881382,-0.158333333333401,
8.3378870715479));
#54894=CARTESIAN_POINT('Ctrl Pts',(4.59272226060636,0.158333333333403,8.30698817777221));
#54895=CARTESIAN_POINT('Ctrl Pts',(4.63959412927933,0.319434907277307,8.29025879047028));
#54896=CARTESIAN_POINT('Ctrl Pts',(4.71401075228064,0.636309800095484,8.27397722462864));
#54897=CARTESIAN_POINT('Ctrl Pts',(4.78475025061342,0.794772684001185,8.26548651872526));
#54898=CARTESIAN_POINT('Ctrl Pts',(4.83614917978268,1.06847604194574,8.28192769191487));
#54899=CARTESIAN_POINT('Ctrl Pts',(4.84862638815205,1.18514270861262,8.29592383538026));
#54900=CARTESIAN_POINT('Ctrl Pts',(4.85133211297141,1.30000000000105,8.31679934764279));
#54901=CARTESIAN_POINT('Ctrl Pts',(4.79025491811528,-1.30000000000142,8.5498229553338));
#54902=CARTESIAN_POINT('Ctrl Pts',(4.79210326372372,-1.18514270861288,8.51500570025586));
#54903=CARTESIAN_POINT('Ctrl Pts',(4.78448988078939,-1.06847604194588,8.48436813993301));
#54904=CARTESIAN_POINT('Ctrl Pts',(4.74504295741298,-0.794772684001196,
8.42324517759365));
#54905=CARTESIAN_POINT('Ctrl Pts',(4.6818832785033,-0.636309800095473,8.39818804809511));
#54906=CARTESIAN_POINT('Ctrl Pts',(4.62234144669066,-0.319434907277297,
8.35350183815101));
#54907=CARTESIAN_POINT('Ctrl Pts',(4.58328782589623,-0.158333333333401,
8.33828810279069));
#54908=CARTESIAN_POINT('Ctrl Pts',(4.59080541024151,0.158333333333403,8.30742477131116));
#54909=CARTESIAN_POINT('Ctrl Pts',(4.63758835707064,0.319434907277307,8.29081652143042));
#54910=CARTESIAN_POINT('Ctrl Pts',(4.71201166433516,0.636309800095484,8.27458905607121));
#54911=CARTESIAN_POINT('Ctrl Pts',(4.78270525737022,0.794772684001185,8.26610317864001));
#54912=CARTESIAN_POINT('Ctrl Pts',(4.83437911060835,1.06847604194574,8.28247029593681));
#54913=CARTESIAN_POINT('Ctrl Pts',(4.84704412936208,1.18514270861262,8.29641178690816));
#54914=CARTESIAN_POINT('Ctrl Pts',(4.85000647050771,1.30000000000105,8.31721005023453));
#54915=CARTESIAN_POINT('Ctrl Pts',(4.78760459323741,-1.30000000000142,8.55040694471682));
#54916=CARTESIAN_POINT('Ctrl Pts',(4.78893359553989,-1.18514270861287,8.51579282764292));
#54917=CARTESIAN_POINT('Ctrl Pts',(4.78094149445432,-1.06847604194587,8.48529275713613));
#54918=CARTESIAN_POINT('Ctrl Pts',(4.74094452862561,-0.794772684001195,
8.42433576332957));
#54919=CARTESIAN_POINT('Ctrl Pts',(4.67789067928778,-0.636309800095472,
8.39915697652538));
#54920=CARTESIAN_POINT('Ctrl Pts',(4.61833799057227,-0.319434907277297,
8.35441543238267));
#54921=CARTESIAN_POINT('Ctrl Pts',(4.57945618696832,-0.158333333333401,
8.33908544628562));
#54922=CARTESIAN_POINT('Ctrl Pts',(4.58697165641103,0.158333333333403,8.30829237081323));
#54923=CARTESIAN_POINT('Ctrl Pts',(4.63357745927118,0.319434907277307,8.29191182788788));
#54924=CARTESIAN_POINT('Ctrl Pts',(4.70801385789431,0.636309800095483,8.27579888129089));
#54925=CARTESIAN_POINT('Ctrl Pts',(4.77861443131758,0.794772684001183,8.26734960385899));
#54926=CARTESIAN_POINT('Ctrl Pts',(4.83083801918334,1.06847604194574,8.28357264681678));
#54927=CARTESIAN_POINT('Ctrl Pts',(4.84387884673486,1.18514270861261,8.29740161341555));
#54928=CARTESIAN_POINT('Ctrl Pts',(4.84735484572544,1.30000000000104,8.31803719243965));
#54929=CARTESIAN_POINT('Ctrl Pts',(4.7823073456323,-1.30000000000142,8.55152432972443));
#54930=CARTESIAN_POINT('Ctrl Pts',(4.78260296703768,-1.18514270861287,8.51725343981543));
#54931=CARTESIAN_POINT('Ctrl Pts',(4.77385649639675,-1.06847604194587,8.4869912924405));
#54932=CARTESIAN_POINT('Ctrl Pts',(4.73276135799954,-0.794772684001193,
8.42634067528254));
#54933=CARTESIAN_POINT('Ctrl Pts',(4.66991234341115,-0.63630980009547,8.40099325973968));
#54934=CARTESIAN_POINT('Ctrl Pts',(4.61033295745482,-0.319434907277296,
8.35620033016389));
#54935=CARTESIAN_POINT('Ctrl Pts',(4.57179084334347,-0.1583333333334,8.3406966133674));
#54936=CARTESIAN_POINT('Ctrl Pts',(4.57930142550142,0.158333333333402,8.31004323747091));
#54937=CARTESIAN_POINT('Ctrl Pts',(4.62555820738196,0.319434907277305,8.29401937448729));
#54938=CARTESIAN_POINT('Ctrl Pts',(4.70002040071875,0.63630980009548,8.27815427484438));
#54939=CARTESIAN_POINT('Ctrl Pts',(4.77042932246061,0.794772684001181,8.26991151323194));
#54940=CARTESIAN_POINT('Ctrl Pts',(4.82375149465376,1.06847604194573,8.28586807724426));
#54941=CARTESIAN_POINT('Ctrl Pts',(4.83754449001921,1.18514270861261,8.29945840142342));
#54942=CARTESIAN_POINT('Ctrl Pts',(4.8420492881889,1.30000000000104,8.31973204446977));
#54943=CARTESIAN_POINT('Ctrl Pts',(4.7747469216486,-1.30000000000139,8.55297979474255));
#54944=CARTESIAN_POINT('Ctrl Pts',(4.77358950033188,-1.18514270861285,8.51894026910112));
#54945=CARTESIAN_POINT('Ctrl Pts',(4.76377912280778,-1.06847604194585,8.48886494552462));
#54946=CARTESIAN_POINT('Ctrl Pts',(4.72112512831088,-0.794772684001178,
8.42854303132101));
#54947=CARTESIAN_POINT('Ctrl Pts',(4.65854136944843,-0.636309800095459,
8.40325147775868));
#54948=CARTESIAN_POINT('Ctrl Pts',(4.59890417967612,-0.31943490727729,8.35863062757503));
#54949=CARTESIAN_POINT('Ctrl Pts',(4.56083048148958,-0.158333333333398,
8.34313951944532));
#54950=CARTESIAN_POINT('Ctrl Pts',(4.56833232593917,0.158333333333399,8.31267406642545));
#54951=CARTESIAN_POINT('Ctrl Pts',(4.61411391094263,0.319434907277299,8.29672355810624));
#54952=CARTESIAN_POINT('Ctrl Pts',(4.68861212424133,0.636309800095469,8.28127684869272));
#54953=CARTESIAN_POINT('Ctrl Pts',(4.75872285528296,0.794772684001166,8.27390069142831));
#54954=CARTESIAN_POINT('Ctrl Pts',(4.8136117200716,1.06847604194571,8.28954194395389));
#54955=CARTESIAN_POINT('Ctrl Pts',(4.82848228909124,1.18514270861259,8.30271669851244));
#54956=CARTESIAN_POINT('Ctrl Pts',(4.83446407139639,1.30000000000102,8.32229568897672));
#54957=CARTESIAN_POINT('Ctrl Pts',(4.76567097848328,-1.30000000000139,8.55472712245201));
#54958=CARTESIAN_POINT('Ctrl Pts',(4.76276845286623,-1.18514270861284,8.520959348338));
#54959=CARTESIAN_POINT('Ctrl Pts',(4.75168150209505,-1.06847604194585,8.4910915121608));
#54960=CARTESIAN_POINT('Ctrl Pts',(4.70716076848207,-0.794772684001175,
8.43110047236531));
#54961=CARTESIAN_POINT('Ctrl Pts',(4.6449053265792,-0.636309800095455,8.40577518511714));
#54962=CARTESIAN_POINT('Ctrl Pts',(4.58520363494991,-0.319434907277288,
8.36130772192686));
#54963=CARTESIAN_POINT('Ctrl Pts',(4.54769257845807,-0.158333333333397,
8.34583811065994));
#54964=CARTESIAN_POINT('Ctrl Pts',(4.55517888930291,0.158333333333399,8.31563506213017));
#54965=CARTESIAN_POINT('Ctrl Pts',(4.60037871346206,0.319434907277297,8.29986928442809));
#54966=CARTESIAN_POINT('Ctrl Pts',(4.67491709128006,0.636309800095465,8.28491811559864));
#54967=CARTESIAN_POINT('Ctrl Pts',(4.74467985764269,0.794772684001162,8.27841169407885));
#54968=CARTESIAN_POINT('Ctrl Pts',(4.80144680785053,1.06847604194571,8.29373247175476));
#54969=CARTESIAN_POINT('Ctrl Pts',(4.81760758149724,1.18514270861258,8.30648005005701));
#54970=CARTESIAN_POINT('Ctrl Pts',(4.8253568194685,1.30000000000101,8.32534340969635));
#54971=CARTESIAN_POINT('Ctrl Pts',(4.75354538128605,-1.30000000000136,8.55733659235512));
#54972=CARTESIAN_POINT('Ctrl Pts',(4.74827750446818,-1.18514270861282,8.52434007795708));
#54973=CARTESIAN_POINT('Ctrl Pts',(4.7354669278131,-1.06847604194583,8.49497482578842));
#54974=CARTESIAN_POINT('Ctrl Pts',(4.68844678745697,-0.794772684001161,
8.43552416096171));
#54975=CARTESIAN_POINT('Ctrl Pts',(4.62668088567543,-0.636309800095444,
8.40961132816583));
#54976=CARTESIAN_POINT('Ctrl Pts',(4.56694039954845,-0.319434907277282,
8.36478405455998));
#54977=CARTESIAN_POINT('Ctrl Pts',(4.53022662309791,-0.158333333333394,
8.34871583916773));
#54978=CARTESIAN_POINT('Ctrl Pts',(4.53769481795827,0.158333333333396,8.31884484338701));
#54979=CARTESIAN_POINT('Ctrl Pts',(4.58206034218961,0.319434907277293,8.30419551308267));
#54980=CARTESIAN_POINT('Ctrl Pts',(4.65663911943659,0.636309800095455,8.28990208029129));
#54981=CARTESIAN_POINT('Ctrl Pts',(4.72596785410255,0.794772684001148,8.28367740836966));
#54982=CARTESIAN_POINT('Ctrl Pts',(4.78524673561844,1.06847604194569,8.2984751364591));
#54983=CARTESIAN_POINT('Ctrl Pts',(4.80312837789116,1.18514270861256,8.31076137562564));
#54984=CARTESIAN_POINT('Ctrl Pts',(4.81323203112739,1.30000000000098,8.32892846577867));
#54985=CARTESIAN_POINT('Ctrl Pts',(4.73837355545878,-1.3000000000013,8.5606497694795));
#54986=CARTESIAN_POINT('Ctrl Pts',(4.73015115072486,-1.18514270861277,8.52857893756578));
#54987=CARTESIAN_POINT('Ctrl Pts',(4.71518579190561,-1.06847604194578,8.49983387381159));
#54988=CARTESIAN_POINT('Ctrl Pts',(4.66503524636295,-0.794772684001123,
8.44111021587534));
#54989=CARTESIAN_POINT('Ctrl Pts',(4.60386429694356,-0.636309800095414,
8.4146314440745));
#54990=CARTESIAN_POINT('Ctrl Pts',(4.54407057347046,-0.319434907277268,
8.36944529380717));
#54991=CARTESIAN_POINT('Ctrl Pts',(4.50835673161846,-0.158333333333386,
8.35269305007124));
#54992=CARTESIAN_POINT('Ctrl Pts',(4.51581536651864,0.158333333333388,8.32309148513968));
#54993=CARTESIAN_POINT('Ctrl Pts',(4.5591620075005,0.319434907277275,8.30942565772959));
#54994=CARTESIAN_POINT('Ctrl Pts',(4.63379367323015,0.636309800095423,8.29597871598314));
#54995=CARTESIAN_POINT('Ctrl Pts',(4.70255993381258,0.79477268400111,8.2905739348661));
#54996=CARTESIAN_POINT('Ctrl Pts',(4.76496472644855,1.06847604194564,8.30490136991313));
#54997=CARTESIAN_POINT('Ctrl Pts',(4.78499194360679,1.18514270861251,8.31663757162872));
#54998=CARTESIAN_POINT('Ctrl Pts',(4.7980336555166,1.30000000000093,8.33390815931181));
#54999=CARTESIAN_POINT('Ctrl Pts',(4.71416590268322,-1.30000000000123,8.56515386171744));
#55000=CARTESIAN_POINT('Ctrl Pts',(4.70126884943509,-1.1851427086127,8.53391407158018));
#55001=CARTESIAN_POINT('Ctrl Pts',(4.6828939690976,-1.06847604194572,8.50570019546546));
#55002=CARTESIAN_POINT('Ctrl Pts',(4.62778944322383,-0.79477268400108,8.44751096419801));
#55003=CARTESIAN_POINT('Ctrl Pts',(4.56758615172801,-0.636309800095381,
8.42009138315412));
#55004=CARTESIAN_POINT('Ctrl Pts',(4.50765180405554,-0.319434907277252,
8.37491070370344));
#55005=CARTESIAN_POINT('Ctrl Pts',(4.47342625780318,-0.158333333333378,
8.35817574772211));
#55006=CARTESIAN_POINT('Ctrl Pts',(4.48079197929825,0.15833333333338,8.32974691733967));
#55007=CARTESIAN_POINT('Ctrl Pts',(4.52249044329594,0.319434907277261,8.31789680836533));
#55008=CARTESIAN_POINT('Ctrl Pts',(4.59720988426097,0.636309800095392,8.30548824584704));
#55009=CARTESIAN_POINT('Ctrl Pts',(4.66512072251762,0.794772684001071,8.30029297084602));
#55010=CARTESIAN_POINT('Ctrl Pts',(4.73256761032737,1.06847604194558,8.31349399926102));
#55011=CARTESIAN_POINT('Ctrl Pts',(4.75604532845754,1.18514270861244,8.3243512014707));
#55012=CARTESIAN_POINT('Ctrl Pts',(4.77380550613851,1.30000000000085,8.34035136983552));
#55013=CARTESIAN_POINT('Ctrl Pts',(4.69297040123395,-1.30000000000116,8.5690572456906));
#55014=CARTESIAN_POINT('Ctrl Pts',(4.67599576681304,-1.18514270861264,8.53842933539974));
#55015=CARTESIAN_POINT('Ctrl Pts',(4.65463186400387,-1.06847604194566,8.51072878569245));
#55016=CARTESIAN_POINT('Ctrl Pts',(4.5951368866336,-0.794772684001033,8.4534977629572));
#55017=CARTESIAN_POINT('Ctrl Pts',(4.53562583044008,-0.636309800095344,
8.42662864582605));
#55018=CARTESIAN_POINT('Ctrl Pts',(4.47556129846,-0.319434907277232,8.38150467738444));
#55019=CARTESIAN_POINT('Ctrl Pts',(4.44274572059359,-0.158333333333369,
8.36393984045405));
#55020=CARTESIAN_POINT('Ctrl Pts',(4.45013328538506,0.158333333333371,8.33535479141151));
#55021=CARTESIAN_POINT('Ctrl Pts',(4.49048336803185,0.319434907277241,8.32363781472797));
#55022=CARTESIAN_POINT('Ctrl Pts',(4.56529653139247,0.636309800095353,8.31195535572491));
#55023=CARTESIAN_POINT('Ctrl Pts',(4.63236078486284,0.794772684001023,8.30841184376824));
#55024=CARTESIAN_POINT('Ctrl Pts',(4.70417877575155,1.06847604194552,8.32125124762597));
#55025=CARTESIAN_POINT('Ctrl Pts',(4.73066645536988,1.18514270861238,8.33147975320106));
#55026=CARTESIAN_POINT('Ctrl Pts',(4.75255446746963,1.30000000000078,8.34637906216803));
#55027=CARTESIAN_POINT('Ctrl Pts',(4.66873124297124,-1.30000000000112,8.57357009359638));
#55028=CARTESIAN_POINT('Ctrl Pts',(4.6470379636447,-1.1851427086126,8.54401642914705));
#55029=CARTESIAN_POINT('Ctrl Pts',(4.6222509633327,-1.06847604194563,8.51686786821153));
#55030=CARTESIAN_POINT('Ctrl Pts',(4.55784091961646,-0.794772684001013,
8.45970553165579));
#55031=CARTESIAN_POINT('Ctrl Pts',(4.49947416501879,-0.636309800095329,
8.43045783746727));
#55032=CARTESIAN_POINT('Ctrl Pts',(4.43931646189135,-0.319434907277226,
8.38487602674139));
#55033=CARTESIAN_POINT('Ctrl Pts',(4.40791159835173,-0.158333333333365,
8.36800874541527));
#55034=CARTESIAN_POINT('Ctrl Pts',(4.4151748412205,0.158333333333367,8.340614333267));
#55035=CARTESIAN_POINT('Ctrl Pts',(4.45390149438311,0.319434907277231,8.32995536807035));
#55036=CARTESIAN_POINT('Ctrl Pts',(4.52873464474054,0.636309800095336,8.32000527084179));
#55037=CARTESIAN_POINT('Ctrl Pts',(4.59480833328335,0.794772684001006,8.31860316319239));
#55038=CARTESIAN_POINT('Ctrl Pts',(4.67164168169231,1.0684760419455,8.3308669948441));
#55039=CARTESIAN_POINT('Ctrl Pts',(4.70159534229404,1.18514270861235,8.34013252429138));
#55040=CARTESIAN_POINT('Ctrl Pts',(4.72824435392736,1.30000000000075,8.35335502488365));
#55041=CARTESIAN_POINT('Ctrl Pts',(4.64455763696824,-1.30000000000109,8.57733417227618));
#55042=CARTESIAN_POINT('Ctrl Pts',(4.61828683665992,-1.18514270861258,8.5476972423875));
#55043=CARTESIAN_POINT('Ctrl Pts',(4.59013172517861,-1.0684760419456,8.52065311316078));
#55044=CARTESIAN_POINT('Ctrl Pts',(4.52073464948133,-0.794772684000996,
8.46416565270476));
#55045=CARTESIAN_POINT('Ctrl Pts',(4.46301202251514,-0.636309800095314,
8.43666670116118));
#55046=CARTESIAN_POINT('Ctrl Pts',(4.40271193562758,-0.319434907277218,
8.39105221918814));
#55047=CARTESIAN_POINT('Ctrl Pts',(4.37306118991602,-0.158333333333361,
8.37213853899525));
#55048=CARTESIAN_POINT('Ctrl Pts',(4.38032974813031,0.158333333333363,8.3447461412619));
#55049=CARTESIAN_POINT('Ctrl Pts',(4.41734870731225,0.319434907277224,8.33576102998205));
#55050=CARTESIAN_POINT('Ctrl Pts',(4.49225133334755,0.636309800095321,8.32661065767595));
#55051=CARTESIAN_POINT('Ctrl Pts',(4.55746683780738,0.794772684000987,8.32525270685827));
#55052=CARTESIAN_POINT('Ctrl Pts',(4.63929995689959,1.06847604194547,8.3371877182811));
#55053=CARTESIAN_POINT('Ctrl Pts',(4.67267882086693,1.18514270861232,8.34615086292065));
#55054=CARTESIAN_POINT('Ctrl Pts',(4.70401402376247,1.30000000000072,8.35891092799055));
#55055=CARTESIAN_POINT('Ctrl Pts',(4.62194387170432,-1.30000000000104,8.58059186454667));
#55056=CARTESIAN_POINT('Ctrl Pts',(4.59121967798365,-1.18514270861253,8.5520201756949));
#55057=CARTESIAN_POINT('Ctrl Pts',(4.55984620022608,-1.06847604194556,8.5254566912415));
#55058=CARTESIAN_POINT('Ctrl Pts',(4.48586721434936,-0.794772684000964,
8.46872908204751));
#55059=CARTESIAN_POINT('Ctrl Pts',(4.42933519750432,-0.636309800095286,
8.43828658202844));
#55060=CARTESIAN_POINT('Ctrl Pts',(4.36898105086931,-0.319434907277203,
8.39200530408134));
#55061=CARTESIAN_POINT('Ctrl Pts',(4.34063582129055,-0.158333333333354,
8.3738316313857));
#55062=CARTESIAN_POINT('Ctrl Pts',(4.347703736149,0.158333333333356,8.34811560974449));
#55063=CARTESIAN_POINT('Ctrl Pts',(4.38307446740542,0.319434907277211,8.34101388650739));
#55064=CARTESIAN_POINT('Ctrl Pts',(4.45791184029579,0.636309800095295,8.33401595714426));
#55065=CARTESIAN_POINT('Ctrl Pts',(4.52220357437114,0.794772684000952,8.33446497927006));
#55066=CARTESIAN_POINT('Ctrl Pts',(4.60874194005757,1.06847604194542,8.34592495844054));
#55067=CARTESIAN_POINT('Ctrl Pts',(4.64537970251158,1.18514270861227,8.35401420591919));
#55068=CARTESIAN_POINT('Ctrl Pts',(4.68119597547639,1.30000000000066,8.36523210052768));
#55069=CARTESIAN_POINT('Ctrl Pts',(4.60387932238281,-1.30000000000102,8.58288177294599));
#55070=CARTESIAN_POINT('Ctrl Pts',(4.56967256179496,-1.18514270861251,8.55453114462641));
#55071=CARTESIAN_POINT('Ctrl Pts',(4.53575217283572,-1.06847604194555,8.52813075555004));
#55072=CARTESIAN_POINT('Ctrl Pts',(4.45805086433994,-0.794772684000954,
8.47164601819983));
#55073=CARTESIAN_POINT('Ctrl Pts',(4.40215448199083,-0.636309800095278,
8.44131145778521));
#55074=CARTESIAN_POINT('Ctrl Pts',(4.3417232110165,-0.319434907277199,8.3947729050014));
#55075=CARTESIAN_POINT('Ctrl Pts',(4.31460517397489,-0.158333333333352,
8.37588671898424));
#55076=CARTESIAN_POINT('Ctrl Pts',(4.32166562292817,0.158333333333354,8.35014628586842));
#55077=CARTESIAN_POINT('Ctrl Pts',(4.35582539932203,0.319434907277208,8.34343069045799));
#55078=CARTESIAN_POINT('Ctrl Pts',(4.43067640655517,0.636309800095287,8.33725541085188));
#55079=CARTESIAN_POINT('Ctrl Pts',(4.49420718713358,0.794772684000941,8.33880717160197));
#55080=CARTESIAN_POINT('Ctrl Pts',(4.58444004850034,1.06847604194541,8.35062203874628));
#55081=CARTESIAN_POINT('Ctrl Pts',(4.6236371583146,1.18514270861225,8.35864762097586));
#55082=CARTESIAN_POINT('Ctrl Pts',(4.66297291571444,1.30000000000065,8.3695845672322));
#55083=CARTESIAN_POINT('Ctrl Pts',(4.59493977879337,-1.30000000000102,8.58342037655318));
#55084=CARTESIAN_POINT('Ctrl Pts',(4.55898890691848,-1.18514270861251,8.55517513605593));
#55085=CARTESIAN_POINT('Ctrl Pts',(4.52379498416204,-1.06847604194554,8.5288359222857));
#55086=CARTESIAN_POINT('Ctrl Pts',(4.44423868596545,-0.794772684000949,
8.47239037237364));
#55087=CARTESIAN_POINT('Ctrl Pts',(4.3886850447675,-0.636309800095275,8.44191394461041));
#55088=CARTESIAN_POINT('Ctrl Pts',(4.3282078191952,-0.319434907277198,8.39529412085592));
#55089=CARTESIAN_POINT('Ctrl Pts',(4.30168710817396,-0.158333333333352,
8.376177369922));
#55090=CARTESIAN_POINT('Ctrl Pts',(4.30869497686896,0.158333333333354,8.35080710552607));
#55091=CARTESIAN_POINT('Ctrl Pts',(4.34218746912544,0.319434907277206,8.34476661947023));
#55092=CARTESIAN_POINT('Ctrl Pts',(4.41701272620334,0.636309800095284,8.33927511988198));
#55093=CARTESIAN_POINT('Ctrl Pts',(4.48017134140349,0.794772684000937,8.34139007320928));
#55094=CARTESIAN_POINT('Ctrl Pts',(4.5722811881534,1.06847604194541,8.35308146316041));
#55095=CARTESIAN_POINT('Ctrl Pts',(4.61277899908719,1.18514270861225,8.36084944837583));
#55096=CARTESIAN_POINT('Ctrl Pts',(4.65390368130292,1.30000000000064,8.37132464930549));
#55097=CARTESIAN_POINT('Ctrl Pts',(4.58581707049687,-1.30000000000101,8.5850986834178));
#55098=CARTESIAN_POINT('Ctrl Pts',(4.54812928518205,-1.1851427086125,8.55694519581164));
#55099=CARTESIAN_POINT('Ctrl Pts',(4.51167300653039,-1.06847604194554,8.53061718102351));
#55100=CARTESIAN_POINT('Ctrl Pts',(4.43029673654555,-0.794772684000947,
8.47401140735594));
#55101=CARTESIAN_POINT('Ctrl Pts',(4.37512370956665,-0.636309800095272,
8.44312610006982));
#55102=CARTESIAN_POINT('Ctrl Pts',(4.31464442091295,-0.319434907277196,
8.3961375598802));
#55103=CARTESIAN_POINT('Ctrl Pts',(4.28874071971753,-0.158333333333351,
8.3766748156319));
#55104=CARTESIAN_POINT('Ctrl Pts',(4.29571856586336,0.158333333333353,8.3515037707682));
#55105=CARTESIAN_POINT('Ctrl Pts',(4.32854762139582,0.319434907277205,8.34606041006935));
#55106=CARTESIAN_POINT('Ctrl Pts',(4.40334720226197,0.636309800095282,8.34123768071327));
#55107=CARTESIAN_POINT('Ctrl Pts',(4.46612092809186,0.794772684000934,8.34401580888935));
#55108=CARTESIAN_POINT('Ctrl Pts',(4.56010178861599,1.0684760419454,8.35566243892948));
#55109=CARTESIAN_POINT('Ctrl Pts',(4.60189886394712,1.18514270861224,8.36320630783392));
#55110=CARTESIAN_POINT('Ctrl Pts',(4.64481218242255,1.30000000000064,8.37325265104859));
#55111=CARTESIAN_POINT('Ctrl Pts',(4.57976379072891,-1.30000000000101,8.58604105405601));
#55112=CARTESIAN_POINT('Ctrl Pts',(4.5409029819475,-1.18514270861251,8.55803781082764));
#55113=CARTESIAN_POINT('Ctrl Pts',(4.50359549349079,-1.06847604194554,8.53177312762207));
#55114=CARTESIAN_POINT('Ctrl Pts',(4.42099621250913,-0.794772684000947,
8.47511287663577));
#55115=CARTESIAN_POINT('Ctrl Pts',(4.36609611660324,-0.636309800095273,
8.44383161138913));
#55116=CARTESIAN_POINT('Ctrl Pts',(4.30561120695117,-0.319434907277196,
8.39662026242517));
#55117=CARTESIAN_POINT('Ctrl Pts',(4.28009950000537,-0.158333333333351,
8.37705031023949));
#55118=CARTESIAN_POINT('Ctrl Pts',(4.28705418197413,0.158333333333353,8.35202817045905));
#55119=CARTESIAN_POINT('Ctrl Pts',(4.31945284716805,0.319434907277205,8.34690681074705));
#55120=CARTESIAN_POINT('Ctrl Pts',(4.39424189157949,0.636309800095282,8.34247599005533));
#55121=CARTESIAN_POINT('Ctrl Pts',(4.45676575258676,0.794772684000934,8.34561202054393));
#55122=CARTESIAN_POINT('Ctrl Pts',(4.55198658002281,1.0684760419454,8.35730905319397));
#55123=CARTESIAN_POINT('Ctrl Pts',(4.59464305750395,1.18514270861224,8.36477760337297));
#55124=CARTESIAN_POINT('Ctrl Pts',(4.63873844454854,1.30000000000064,8.37465149171453));
#55125=CARTESIAN_POINT('Ctrl Pts',(4.55272395833052,-1.300000000001,8.58902013595507));
#55126=CARTESIAN_POINT('Ctrl Pts',(4.50863897250943,-1.18514270861249,8.56133756355169));
#55127=CARTESIAN_POINT('Ctrl Pts',(4.46752661973699,-1.06847604194553,8.53519270549119));
#55128=CARTESIAN_POINT('Ctrl Pts',(4.37941623735034,-0.794772684000935,
8.47834528086133));
#55129=CARTESIAN_POINT('Ctrl Pts',(4.32563627330862,-0.636309800095265,
8.44600322061239));
#55130=CARTESIAN_POINT('Ctrl Pts',(4.26502966611551,-0.319434907277193,
8.39842680825674));
#55131=CARTESIAN_POINT('Ctrl Pts',(4.24119970548086,-0.158333333333349,
8.37893073249655));
#55132=CARTESIAN_POINT('Ctrl Pts',(4.24805168854086,0.158333333333351,8.35452321283523));
#55133=CARTESIAN_POINT('Ctrl Pts',(4.27863088493474,0.319434907277202,8.35002401984986));
#55134=CARTESIAN_POINT('Ctrl Pts',(4.3534037771156,0.636309800095275,8.34704434662279));
#55135=CARTESIAN_POINT('Ctrl Pts',(4.41477543889416,0.794772684000924,8.35178927068111));
#55136=CARTESIAN_POINT('Ctrl Pts',(4.51551564193555,1.06847604194539,8.36419369067576));
#55137=CARTESIAN_POINT('Ctrl Pts',(4.56200224101305,1.18514270861223,8.37166838660108));
#55138=CARTESIAN_POINT('Ctrl Pts',(4.61136873806383,1.30000000000062,8.38124836466505));
#55139=CARTESIAN_POINT('Ctrl Pts',(4.5151925571782,-1.30000000000092,8.59274412866428));
#55140=CARTESIAN_POINT('Ctrl Pts',(4.46392074810623,-1.18514270861242,8.56502773770619));
#55141=CARTESIAN_POINT('Ctrl Pts',(4.41759507396831,-1.06847604194547,8.53861206670473));
#55142=CARTESIAN_POINT('Ctrl Pts',(4.32200006045904,-0.794772684000893,
8.48059150556247));
#55143=CARTESIAN_POINT('Ctrl Pts',(4.26994723219476,-0.63630980009523,8.44614168876008));
#55144=CARTESIAN_POINT('Ctrl Pts',(4.2092355775166,-0.319434907277175,8.39769428151512));
#55145=CARTESIAN_POINT('Ctrl Pts',(4.1876899933838,-0.158333333333341,8.37830484137755));
#55146=CARTESIAN_POINT('Ctrl Pts',(4.19425108882492,0.158333333333343,8.35548232070467));
#55147=CARTESIAN_POINT('Ctrl Pts',(4.22206620441759,0.319434907277185,8.35330808608328));
#55148=CARTESIAN_POINT('Ctrl Pts',(4.29673623293127,0.63630980009524,8.35270348350687));
#55149=CARTESIAN_POINT('Ctrl Pts',(4.35663864633831,0.794772684000882,8.35888172484033));
#55150=CARTESIAN_POINT('Ctrl Pts',(4.46510943585546,1.06847604194533,8.37153350165183));
#55151=CARTESIAN_POINT('Ctrl Pts',(4.51694046916774,1.18514270861216,8.37865665368745));
#55152=CARTESIAN_POINT('Ctrl Pts',(4.57364955024915,1.30000000000055,8.38742647237151));
#55153=CARTESIAN_POINT('Ctrl Pts',(4.47343222775881,-1.3000000000009,8.59504533441471));
#55154=CARTESIAN_POINT('Ctrl Pts',(4.41421631652258,-1.18514270861241,8.56655289837235));
#55155=CARTESIAN_POINT('Ctrl Pts',(4.36211950350135,-1.06847604194545,8.53934631629306));
#55156=CARTESIAN_POINT('Ctrl Pts',(4.2582119845381,-0.794772684000882,8.4794642489208));
#55157=CARTESIAN_POINT('Ctrl Pts',(4.20788743033015,-0.636309800095223,
8.44374706396478));
#55158=CARTESIAN_POINT('Ctrl Pts',(4.14724168103829,-0.319434907277172,
8.39349114738577));
#55159=CARTESIAN_POINT('Ctrl Pts',(4.12869895428878,-0.158333333333339,
8.3723767125966));
#55160=CARTESIAN_POINT('Ctrl Pts',(4.13506288582316,0.158333333333341,8.35034892732963));
#55161=CARTESIAN_POINT('Ctrl Pts',(4.15967453768392,0.31943490727718,8.35037750099606));
#55162=CARTESIAN_POINT('Ctrl Pts',(4.23388406413583,0.636309800095232,8.35384577337839));
#55163=CARTESIAN_POINT('Ctrl Pts',(4.29165071350381,0.794772684000874,8.36416771399849));
#55164=CARTESIAN_POINT('Ctrl Pts',(4.40846370800721,1.06847604194532,8.37947686697347));
#55165=CARTESIAN_POINT('Ctrl Pts',(4.46620340952472,1.18514270861215,8.38712836816309));
#55166=CARTESIAN_POINT('Ctrl Pts',(4.5311187955872,1.30000000000053,8.39580460547946));
#55167=CARTESIAN_POINT('Ctrl Pts',(4.45248023998025,-1.30000000000089,8.59655638746898));
#55168=CARTESIAN_POINT('Ctrl Pts',(4.38926946308294,-1.1851427086124,8.56782729269431));
#55169=CARTESIAN_POINT('Ctrl Pts',(4.33431432026877,-1.06847604194544,8.54013571994062));
#55170=CARTESIAN_POINT('Ctrl Pts',(4.22642911289548,-0.794772684000875,
8.47855953062353));
#55171=CARTESIAN_POINT('Ctrl Pts',(4.17742023988668,-0.636309800095217,
8.4401428888402));
#55172=CARTESIAN_POINT('Ctrl Pts',(4.11682467017945,-0.319434907277169,
8.38890277567568));
#55173=CARTESIAN_POINT('Ctrl Pts',(4.09936599852457,-0.158333333333337,
8.36882989779298));
#55174=CARTESIAN_POINT('Ctrl Pts',(4.10550426669319,0.158333333333339,8.34773080031627));
#55175=CARTESIAN_POINT('Ctrl Pts',(4.12864650391549,0.319434907277176,8.34824411924068));
#55176=CARTESIAN_POINT('Ctrl Pts',(4.2026714803712,0.636309800095225,8.353370960919));
#55177=CARTESIAN_POINT('Ctrl Pts',(4.25938213523715,0.794772684000867,8.36556525651938));
#55178=CARTESIAN_POINT('Ctrl Pts',(4.38038199558138,1.06847604194531,8.38183854958373));
#55179=CARTESIAN_POINT('Ctrl Pts',(4.44107950063504,1.18514270861214,8.38959222333433));
#55180=CARTESIAN_POINT('Ctrl Pts',(4.51009815468601,1.30000000000052,8.39805546525291));
#55181=CARTESIAN_POINT('Ctrl Pts',(4.44055346921691,-1.30000000000089,8.59708300700727));
#55182=CARTESIAN_POINT('Ctrl Pts',(4.37512897133373,-1.1851427086124,8.56774417847339));
#55183=CARTESIAN_POINT('Ctrl Pts',(4.31855986272212,-1.06847604194544,8.53957731078554));
#55184=CARTESIAN_POINT('Ctrl Pts',(4.20833162594993,-0.794772684000876,
8.4772136756684));
#55185=CARTESIAN_POINT('Ctrl Pts',(4.15973807352451,-0.636309800095216,
8.4388551336058));
#55186=CARTESIAN_POINT('Ctrl Pts',(4.0991733537175,-0.319434907277169,8.38710636932283));
#55187=CARTESIAN_POINT('Ctrl Pts',(4.08263878805536,-0.158333333333337,
8.36637619752324));
#55188=CARTESIAN_POINT('Ctrl Pts',(4.08874703354869,0.158333333333339,8.34535216591385));
#55189=CARTESIAN_POINT('Ctrl Pts',(4.1109595054656,0.319434907277176,8.34642176979204));
#55190=CARTESIAN_POINT('Ctrl Pts',(4.18484285157782,0.636309800095225,8.35256881810733));
#55191=CARTESIAN_POINT('Ctrl Pts',(4.24094387836209,0.794772684000865,8.36565943751016));
#55192=CARTESIAN_POINT('Ctrl Pts',(4.36429193579309,1.06847604194531,8.38295709174074));
#55193=CARTESIAN_POINT('Ctrl Pts',(4.4266554629292,1.18514270861214,8.39110489681365));
#55194=CARTESIAN_POINT('Ctrl Pts',(4.49798971363549,1.30000000000052,8.39991299338431));
#55195=CARTESIAN_POINT('Ctrl Pts',(4.42874610728218,-1.30000000000089,8.59716779009637));
#55196=CARTESIAN_POINT('Ctrl Pts',(4.36104944410423,-1.18514270861239,8.56782645212229));
#55197=CARTESIAN_POINT('Ctrl Pts',(4.30286558845658,-1.06847604194544,8.5394506370321));
#55198=CARTESIAN_POINT('Ctrl Pts',(4.19042573069578,-0.794772684000873,
8.47612737862547));
#55199=CARTESIAN_POINT('Ctrl Pts',(4.14268582717973,-0.636309800095214,
8.43593245973611));
#55200=CARTESIAN_POINT('Ctrl Pts',(4.08216704826761,-0.319434907277167,
8.38356446522101));
#55201=CARTESIAN_POINT('Ctrl Pts',(4.06617938619645,-0.158333333333336,
8.36352866686382));
#55202=CARTESIAN_POINT('Ctrl Pts',(4.07211627433835,0.158333333333338,8.34315532356739));
#55203=CARTESIAN_POINT('Ctrl Pts',(4.0935029512946,0.319434907277174,8.34450734638869));
#55204=CARTESIAN_POINT('Ctrl Pts',(4.16721035297765,0.636309800095221,8.35193477966307));
#55205=CARTESIAN_POINT('Ctrl Pts',(4.22263710270724,0.794772684000862,8.36643754302171));
#55206=CARTESIAN_POINT('Ctrl Pts',(4.34825873408589,1.0684760419453,8.38477500098801));
#55207=CARTESIAN_POINT('Ctrl Pts',(4.41225549120837,1.18514270861213,8.39320114282303));
#55208=CARTESIAN_POINT('Ctrl Pts',(4.48587205596967,1.30000000000051,8.40211582040922));
#55209=CARTESIAN_POINT('Ctrl Pts',(4.41383823973829,-1.30000000000088,8.59752605734597));
#55210=CARTESIAN_POINT('Ctrl Pts',(4.34323575450361,-1.18514270861238,8.5676056254189));
#55211=CARTESIAN_POINT('Ctrl Pts',(4.28296381514232,-1.06847604194543,8.53861966994724));
#55212=CARTESIAN_POINT('Ctrl Pts',(4.1675892054439,-0.794772684000868,8.47381514174061));
#55213=CARTESIAN_POINT('Ctrl Pts',(4.12081646532826,-0.636309800095211,
8.43166487740207));
#55214=CARTESIAN_POINT('Ctrl Pts',(4.0601312471902,-0.319434907277166,8.37952336556475));
#55215=CARTESIAN_POINT('Ctrl Pts',(4.04456692395272,-0.158333333333336,
8.36214229211));
#55216=CARTESIAN_POINT('Ctrl Pts',(4.05031201861363,0.158333333333338,8.34253290146348));
#55217=CARTESIAN_POINT('Ctrl Pts',(4.07096892152584,0.319434907277174,8.34241060896167));
#55218=CARTESIAN_POINT('Ctrl Pts',(4.1446856098719,0.63630980009522,8.35031938332042));
#55219=CARTESIAN_POINT('Ctrl Pts',(4.19927279717264,0.794772684000859,8.36638813371899));
#55220=CARTESIAN_POINT('Ctrl Pts',(4.3279741058351,1.0684760419453,8.38579543790554));
#55221=CARTESIAN_POINT('Ctrl Pts',(4.394144356726,1.18514270861212,8.39456864998641));
#55222=CARTESIAN_POINT('Ctrl Pts',(4.47077483084128,1.3000000000005,8.40371437127727));
#55223=CARTESIAN_POINT('Ctrl Pts',(4.39909825262287,-1.30000000000087,8.59776299484767));
#55224=CARTESIAN_POINT('Ctrl Pts',(4.32598568401036,-1.18514270861238,8.56674430457492));
#55225=CARTESIAN_POINT('Ctrl Pts',(4.26385091414587,-1.06847604194543,8.5371202391769));
#55226=CARTESIAN_POINT('Ctrl Pts',(4.14566807694991,-0.794772684000864,
8.47190458428794));
#55227=CARTESIAN_POINT('Ctrl Pts',(4.09914404087926,-0.636309800095205,
8.43126500260843));
#55228=CARTESIAN_POINT('Ctrl Pts',(4.03826094217273,-0.319434907277162,
8.37989489122064));
#55229=CARTESIAN_POINT('Ctrl Pts',(4.0235202967205,-0.158333333333334,8.36307402300566));
#55230=CARTESIAN_POINT('Ctrl Pts',(4.02935455541677,0.158333333333336,8.34294364536773));
#55231=CARTESIAN_POINT('Ctrl Pts',(4.04944030504608,0.319434907277171,8.34091036272037));
#55232=CARTESIAN_POINT('Ctrl Pts',(4.12320374117167,0.636309800095214,8.3486767622445));
#55233=CARTESIAN_POINT('Ctrl Pts',(4.17689422261378,0.794772684000851,8.36628209985493));
#55234=CARTESIAN_POINT('Ctrl Pts',(4.30834589610362,1.06847604194529,8.38657626165297));
#55235=CARTESIAN_POINT('Ctrl Pts',(4.37648195465194,1.18514270861211,8.39564439436043));
#55236=CARTESIAN_POINT('Ctrl Pts',(4.45585351305934,1.30000000000049,8.40499606910577));
#55237=CARTESIAN_POINT('Ctrl Pts',(4.38139541625333,-1.30000000000087,8.59735867632509));
#55238=CARTESIAN_POINT('Ctrl Pts',(4.30490212107633,-1.18514270861237,8.56477350564691));
#55239=CARTESIAN_POINT('Ctrl Pts',(4.24018872966067,-1.06847604194542,8.53441534828401));
#55240=CARTESIAN_POINT('Ctrl Pts',(4.11790178387139,-0.79477268400086,8.46942677791799));
#55241=CARTESIAN_POINT('Ctrl Pts',(4.07117551004531,-0.636309800095203,
8.4322641765055));
#55242=CARTESIAN_POINT('Ctrl Pts',(4.00965947048976,-0.319434907277162,
8.38299063618185));
#55243=CARTESIAN_POINT('Ctrl Pts',(3.99606948519409,-0.158333333333334,
8.36682478193899));
#55244=CARTESIAN_POINT('Ctrl Pts',(4.00186652210145,0.158333333333336,8.34676496522745));
#55245=CARTESIAN_POINT('Ctrl Pts',(4.02082206384393,0.31943490727717,8.343799130353));
#55246=CARTESIAN_POINT('Ctrl Pts',(4.09502514480978,0.636309800095212,8.35032173930797));
#55247=CARTESIAN_POINT('Ctrl Pts',(4.14852626078949,0.794772684000848,8.36633918891102));
#55248=CARTESIAN_POINT('Ctrl Pts',(4.28409749953885,1.06847604194528,8.38658611297483));
#55249=CARTESIAN_POINT('Ctrl Pts',(4.35491742327389,1.18514270861211,8.3960546780065));
#55250=CARTESIAN_POINT('Ctrl Pts',(4.43787350489881,1.3000000000005,8.40622766486509));
#55251=CARTESIAN_POINT('Ctrl Pts',(4.36932387841482,-1.30000000000085,8.59718401041862));
#55252=CARTESIAN_POINT('Ctrl Pts',(4.29080148664772,-1.18514270861236,8.56222163109241));
#55253=CARTESIAN_POINT('Ctrl Pts',(4.22452488361658,-1.06847604194541,8.53088546759122));
#55254=CARTESIAN_POINT('Ctrl Pts',(4.09970289376746,-0.794772684000851,
8.46686994510332));
#55255=CARTESIAN_POINT('Ctrl Pts',(4.05265002448005,-0.636309800095197,
8.43625327523035));
#55256=CARTESIAN_POINT('Ctrl Pts',(3.99084012998883,-0.319434907277159,
8.39044390410473));
#55257=CARTESIAN_POINT('Ctrl Pts',(3.97832338063956,-0.158333333333332,
8.37427477954486));
#55258=CARTESIAN_POINT('Ctrl Pts',(3.98412215794982,0.158333333333334,8.35438222413835));
#55259=CARTESIAN_POINT('Ctrl Pts',(4.00209599199945,0.319434907277167,8.35146503522703));
#55260=CARTESIAN_POINT('Ctrl Pts',(4.07641358158954,0.636309800095206,8.35511244653024));
#55261=CARTESIAN_POINT('Ctrl Pts',(4.12975510290133,0.79477268400084,8.36561273460513));
#55262=CARTESIAN_POINT('Ctrl Pts',(4.2678860136409,1.06847604194527,8.38482320588403));
#55263=CARTESIAN_POINT('Ctrl Pts',(4.34039737044288,1.1851427086121,8.39497038038826));
#55264=CARTESIAN_POINT('Ctrl Pts',(4.42562833104232,1.30000000000048,8.40694922819818));
#55265=CARTESIAN_POINT('Ctrl Pts',(4.36108289177536,-1.30000000000085,8.59965012915573));
#55266=CARTESIAN_POINT('Ctrl Pts',(4.28280795672178,-1.18514270861236,8.56464391562799));
#55267=CARTESIAN_POINT('Ctrl Pts',(4.21670728203312,-1.06847604194541,8.53360435815366));
#55268=CARTESIAN_POINT('Ctrl Pts',(4.09212647700321,-0.794772684000851,
8.47106053995604));
#55269=CARTESIAN_POINT('Ctrl Pts',(4.04497787349014,-0.636309800095197,
8.44300783150171));
#55270=CARTESIAN_POINT('Ctrl Pts',(3.98316982931346,-0.319434907277159,
8.39888504076963));
#55271=CARTESIAN_POINT('Ctrl Pts',(3.97060749458542,-0.158333333333332,
8.38269018459881));
#55272=CARTESIAN_POINT('Ctrl Pts',(3.97642822268415,0.158333333333334,8.36303343689645));
#55273=CARTESIAN_POINT('Ctrl Pts',(3.99446677770813,0.319434907277167,8.36065783751042));
#55274=CARTESIAN_POINT('Ctrl Pts',(4.06883296350448,0.636309800095206,8.36252854962085));
#55275=CARTESIAN_POINT('Ctrl Pts',(4.12234304385769,0.79477268400084,8.36938354588133));
#55276=CARTESIAN_POINT('Ctrl Pts',(4.26021093575307,1.06847604194527,8.38727435958102));
#55277=CARTESIAN_POINT('Ctrl Pts',(4.33251297633895,1.1851427086121,8.39744311267129));
#55278=CARTESIAN_POINT('Ctrl Pts',(4.41743915561804,1.30000000000048,8.41003634852119));
#55279=CARTESIAN_POINT('Ctrl Pts',(4.36108289177477,-1.3,8.59965012915547));
#55280=CARTESIAN_POINT('Ctrl Pts',(4.28280795672145,-1.18514270861178,8.56464391562783));
#55281=CARTESIAN_POINT('Ctrl Pts',(4.21670728203298,-1.06847604194512,8.53360435815359));
#55282=CARTESIAN_POINT('Ctrl Pts',(4.09212647700321,-0.794772684000851,
8.47106053995604));
#55283=CARTESIAN_POINT('Ctrl Pts',(4.04497787349014,-0.636309800095197,
8.44300783150172));
#55284=CARTESIAN_POINT('Ctrl Pts',(3.98316982931346,-0.319434907277159,
8.39888504076963));
#55285=CARTESIAN_POINT('Ctrl Pts',(3.97060749458543,-0.158333333333332,
8.38269018459881));
#55286=CARTESIAN_POINT('Ctrl Pts',(3.97642822268415,0.158333333333334,8.36303343689646));
#55287=CARTESIAN_POINT('Ctrl Pts',(3.99446677770813,0.319434907277167,8.36065783751042));
#55288=CARTESIAN_POINT('Ctrl Pts',(4.06883296350448,0.636309800095206,8.36252854962085));
#55289=CARTESIAN_POINT('Ctrl Pts',(4.12234304385769,0.79477268400084,8.36938354588133));
#55290=CARTESIAN_POINT('Ctrl Pts',(4.26021093575299,1.06847604194511,8.38727435958101));
#55291=CARTESIAN_POINT('Ctrl Pts',(4.33251297633875,1.18514270861178,8.39744311267126));
#55292=CARTESIAN_POINT('Ctrl Pts',(4.41743915561768,1.3,8.41003634852114));
#55293=CARTESIAN_POINT('',(4.76940206616454,-1.2,8.52487883644709));
#55294=CARTESIAN_POINT('Ctrl Pts',(4.76940206616454,-1.2,8.52487883644709));
#55295=CARTESIAN_POINT('Ctrl Pts',(4.74086940653868,-1.22420816645153,8.53714660115925));
#55296=CARTESIAN_POINT('Ctrl Pts',(4.71399385696744,-1.24658523341453,8.54972059636386));
#55297=CARTESIAN_POINT('Ctrl Pts',(4.69025100715547,-1.26662254821489,8.55981762870885));
#55298=CARTESIAN_POINT('Ctrl Pts',(4.67047629062826,-1.28318703090522,8.56846418154303));
#55299=CARTESIAN_POINT('Ctrl Pts',(4.65060554698671,-1.30000000000007,8.57636043474656));
#55300=CARTESIAN_POINT('',(4.80892752503401,-0.653834841367355,8.37333544163683));
#55301=CARTESIAN_POINT('Ctrl Pts',(4.80892752506904,-0.653834841366079,
8.37333544165056));
#55302=CARTESIAN_POINT('Ctrl Pts',(4.80510631376661,-0.717372755970661,
8.38899671596228));
#55303=CARTESIAN_POINT('Ctrl Pts',(4.80185727169085,-0.764980891039073,
8.40205461129384));
#55304=CARTESIAN_POINT('Ctrl Pts',(4.78917211258712,-0.949603287575588,
8.45202527125908));
#55305=CARTESIAN_POINT('Ctrl Pts',(4.78137785082631,-1.05619298999675,8.4817674737032));
#55306=CARTESIAN_POINT('Ctrl Pts',(4.76940206616454,-1.2,8.52487883644709));
#55307=CARTESIAN_POINT('',(4.84008270153004,0.653834841531101,8.23735213035386));
#55308=CARTESIAN_POINT('Ctrl Pts',(4.84008270153004,0.653834841531101,8.23735213035386));
#55309=CARTESIAN_POINT('Ctrl Pts',(4.79955227883107,0.5759960847206,8.24656828401657));
#55310=CARTESIAN_POINT('Ctrl Pts',(4.76543198768065,0.493633454934372,8.25510837225716));
#55311=CARTESIAN_POINT('Ctrl Pts',(4.71698053238237,0.338119094433763,8.26975736934253));
#55312=CARTESIAN_POINT('Ctrl Pts',(4.70025310872036,0.265645306504652,8.27610002608688));
#55313=CARTESIAN_POINT('Ctrl Pts',(4.67933681317188,0.129705370528769,8.28860475229142));
#55314=CARTESIAN_POINT('Ctrl Pts',(4.67367570084384,0.0666195825707109,
8.2946347965237));
#55315=CARTESIAN_POINT('Ctrl Pts',(4.67033844848027,-0.0595394781896691,
8.30753682247028));
#55316=CARTESIAN_POINT('Ctrl Pts',(4.67262159856367,-0.122765359287329,
8.31449795558557));
#55317=CARTESIAN_POINT('Ctrl Pts',(4.68654652654254,-0.260118360054571,
8.32986539262948));
#55318=CARTESIAN_POINT('Ctrl Pts',(4.69982349924885,-0.333937574098211,
8.33830433699626));
#55319=CARTESIAN_POINT('Ctrl Pts',(4.74113217604531,-0.491200648055129,
8.35576690161105));
#55320=CARTESIAN_POINT('Ctrl Pts',(4.77136431588038,-0.574341701776784,
8.36486586118048));
#55321=CARTESIAN_POINT('Ctrl Pts',(4.80892752498969,-0.653834841384169,
8.37333544167558));
#55322=CARTESIAN_POINT('',(4.82444304868815,1.2,8.30781283164827));
#55323=CARTESIAN_POINT('Ctrl Pts',(4.82444304868815,1.2,8.30781283164826));
#55324=CARTESIAN_POINT('Ctrl Pts',(4.82709025840723,1.13751278178995,8.29628442886868));
#55325=CARTESIAN_POINT('Ctrl Pts',(4.83082368709463,1.03911229509008,8.27981174430919));
#55326=CARTESIAN_POINT('Ctrl Pts',(4.83770053806196,0.793513023910657,8.24849002828812));
#55327=CARTESIAN_POINT('Ctrl Pts',(4.83876380524827,0.737991207933235,8.24350584314984));
#55328=CARTESIAN_POINT('Ctrl Pts',(4.84008270153004,0.653834841531101,8.23735213035386));
#55329=CARTESIAN_POINT('Ctrl Pts',(4.70979663593523,1.30000000000007,8.35772002147865));
#55330=CARTESIAN_POINT('Ctrl Pts',(4.72902725870907,1.28316203921417,8.35002540406659));
#55331=CARTESIAN_POINT('Ctrl Pts',(4.74814123467411,1.26659312888534,8.34147687556873));
#55332=CARTESIAN_POINT('Ctrl Pts',(4.78056818711222,1.23822793610611,8.32771710635259));
#55333=CARTESIAN_POINT('Ctrl Pts',(4.80199451884191,1.21941459056863,8.31882500817011));
#55334=CARTESIAN_POINT('Ctrl Pts',(4.82444304868815,1.2,8.30781283164826));
#55335=CARTESIAN_POINT('Ctrl Pts',(4.36108289177477,-1.3,8.59965012915547));
#55336=CARTESIAN_POINT('Ctrl Pts',(4.28280795672145,-1.18514270861178,8.56464391562783));
#55337=CARTESIAN_POINT('Ctrl Pts',(4.21670728203298,-1.06847604194512,8.53360435815359));
#55338=CARTESIAN_POINT('Ctrl Pts',(4.09212647700321,-0.794772684000851,
8.47106053995605));
#55339=CARTESIAN_POINT('Ctrl Pts',(4.04497787349015,-0.636309800095197,
8.44300783150172));
#55340=CARTESIAN_POINT('Ctrl Pts',(3.98316982931346,-0.319434907277159,
8.39888504076964));
#55341=CARTESIAN_POINT('Ctrl Pts',(3.97060749458543,-0.158333333333332,
8.38269018459882));
#55342=CARTESIAN_POINT('Ctrl Pts',(3.97642822268415,0.158333333333334,8.36303343689646));
#55343=CARTESIAN_POINT('Ctrl Pts',(3.99446677770813,0.319434907277167,8.36065783751042));
#55344=CARTESIAN_POINT('Ctrl Pts',(4.06883296350448,0.636309800095206,8.36252854962085));
#55345=CARTESIAN_POINT('Ctrl Pts',(4.12234304385769,0.794772684000841,8.36938354588133));
#55346=CARTESIAN_POINT('Ctrl Pts',(4.26021093575299,1.06847604194511,8.38727435958102));
#55347=CARTESIAN_POINT('Ctrl Pts',(4.33251297633875,1.18514270861178,8.39744311267126));
#55348=CARTESIAN_POINT('Ctrl Pts',(4.41743915561768,1.3,8.41003634852114));
#55349=CARTESIAN_POINT('Ctrl Pts',(4.33573021748671,-1.3,8.67228862570577));
#55350=CARTESIAN_POINT('Ctrl Pts',(4.25817731391276,-1.18514270861178,8.63570774538836));
#55351=CARTESIAN_POINT('Ctrl Pts',(4.19261998989961,-1.06847604194512,8.60359091403708));
#55352=CARTESIAN_POINT('Ctrl Pts',(4.06888164522439,-0.794772684000851,
8.53970745480723));
#55353=CARTESIAN_POINT('Ctrl Pts',(4.02167596618816,-0.636309800095197,
8.51237010663451));
#55354=CARTESIAN_POINT('Ctrl Pts',(3.96004957503508,-0.319434907277159,
8.46888894301598));
#55355=CARTESIAN_POINT('Ctrl Pts',(3.94727563345509,-0.158333333333332,
8.45391747327181));
#55356=CARTESIAN_POINT('Ctrl Pts',(3.95343774500623,0.158333333333334,8.4343716477771));
#55357=CARTESIAN_POINT('Ctrl Pts',(3.97202419499029,0.319434907277167,8.43088192859436));
#55358=CARTESIAN_POINT('Ctrl Pts',(4.04691448012462,0.636309800095206,8.43234032643418));
#55359=CARTESIAN_POINT('Ctrl Pts',(4.10079886363324,0.794772684000841,8.43858303591896));
#55360=CARTESIAN_POINT('Ctrl Pts',(4.2385608990303,1.06847604194511,8.45805282775219));
#55361=CARTESIAN_POINT('Ctrl Pts',(4.3106693138487,1.18514270861178,8.46941248723032));
#55362=CARTESIAN_POINT('Ctrl Pts',(4.39525406294861,1.3,8.48370405472888));
#55363=CARTESIAN_POINT('Ctrl Pts',(4.31037754319865,-1.3,8.74492712225608));
#55364=CARTESIAN_POINT('Ctrl Pts',(4.23354667110408,-1.18514270861178,8.70677157514888));
#55365=CARTESIAN_POINT('Ctrl Pts',(4.16853269776624,-1.06847604194512,8.67357746992056));
#55366=CARTESIAN_POINT('Ctrl Pts',(4.04563681344557,-0.794772684000851,
8.60835436965841));
#55367=CARTESIAN_POINT('Ctrl Pts',(3.99837405888618,-0.636309800095197,
8.58173238176729));
#55368=CARTESIAN_POINT('Ctrl Pts',(3.93692932075669,-0.319434907277159,
8.53889284526232));
#55369=CARTESIAN_POINT('Ctrl Pts',(3.92394377232475,-0.158333333333332,
8.5251447619448));
#55370=CARTESIAN_POINT('Ctrl Pts',(3.93044726732831,0.158333333333334,8.50570985865775));
#55371=CARTESIAN_POINT('Ctrl Pts',(3.94958161227244,0.319434907277167,8.50110601967831));
#55372=CARTESIAN_POINT('Ctrl Pts',(4.02499599674477,0.636309800095206,8.50215210324751));
#55373=CARTESIAN_POINT('Ctrl Pts',(4.07925468340879,0.794772684000841,8.50778252595658));
#55374=CARTESIAN_POINT('Ctrl Pts',(4.21691086230761,1.06847604194511,8.52883129592335));
#55375=CARTESIAN_POINT('Ctrl Pts',(4.28882565135864,1.18514270861178,8.54138186178938));
#55376=CARTESIAN_POINT('Ctrl Pts',(4.37306897027954,1.3,8.55737176093662));
#55377=CARTESIAN_POINT('Ctrl Pts',(4.28502486891058,-1.3,8.81756561880638));
#55378=CARTESIAN_POINT('Ctrl Pts',(4.20891602829539,-1.18514270861178,8.77783540490941));
#55379=CARTESIAN_POINT('Ctrl Pts',(4.14444540563287,-1.06847604194512,8.74356402580405));
#55380=CARTESIAN_POINT('Ctrl Pts',(4.02239198166675,-0.794772684000851,
8.67700128450959));
#55381=CARTESIAN_POINT('Ctrl Pts',(3.9750721515842,-0.636309800095197,8.65109465690008));
#55382=CARTESIAN_POINT('Ctrl Pts',(3.91380906647831,-0.319434907277159,
8.60889674750867));
#55383=CARTESIAN_POINT('Ctrl Pts',(3.90061191119441,-0.158333333333332,
8.59637205061779));
#55384=CARTESIAN_POINT('Ctrl Pts',(3.90745678965039,0.158333333333334,8.5770480695384));
#55385=CARTESIAN_POINT('Ctrl Pts',(3.9271390295546,0.319434907277167,8.57133011076225));
#55386=CARTESIAN_POINT('Ctrl Pts',(4.00307751336492,0.636309800095206,8.57196388006084));
#55387=CARTESIAN_POINT('Ctrl Pts',(4.05771050318434,0.794772684000841,8.57698201599421));
#55388=CARTESIAN_POINT('Ctrl Pts',(4.19526082558493,1.06847604194511,8.59960976409452));
#55389=CARTESIAN_POINT('Ctrl Pts',(4.26698198886859,1.18514270861178,8.61335123634844));
#55390=CARTESIAN_POINT('Ctrl Pts',(4.35088387761047,1.3,8.63103946714436));
#55391=CARTESIAN_POINT('Ctrl Pts',(4.28502486891058,-1.3,8.81756561880638));
#55392=CARTESIAN_POINT('Ctrl Pts',(4.20891602829539,-1.18514270861178,8.77783540490941));
#55393=CARTESIAN_POINT('Ctrl Pts',(4.14444540563287,-1.06847604194512,8.74356402580405));
#55394=CARTESIAN_POINT('Ctrl Pts',(4.02239198166675,-0.794772684000851,
8.67700128450959));
#55395=CARTESIAN_POINT('Ctrl Pts',(3.9750721515842,-0.636309800095197,8.65109465690008));
#55396=CARTESIAN_POINT('Ctrl Pts',(3.91380906647831,-0.319434907277159,
8.60889674750867));
#55397=CARTESIAN_POINT('Ctrl Pts',(3.90061191119441,-0.158333333333332,
8.59637205061778));
#55398=CARTESIAN_POINT('Ctrl Pts',(3.90745678965039,0.158333333333334,8.5770480695384));
#55399=CARTESIAN_POINT('Ctrl Pts',(3.9271390295546,0.319434907277167,8.57133011076225));
#55400=CARTESIAN_POINT('Ctrl Pts',(4.00307751336492,0.636309800095206,8.57196388006084));
#55401=CARTESIAN_POINT('Ctrl Pts',(4.05771050318434,0.79477268400084,8.5769820159942));
#55402=CARTESIAN_POINT('Ctrl Pts',(4.19526082558492,1.06847604194511,8.59960976409452));
#55403=CARTESIAN_POINT('Ctrl Pts',(4.26698198886859,1.18514270861178,8.61335123634844));
#55404=CARTESIAN_POINT('Ctrl Pts',(4.35088387761047,1.3,8.63103946714436));
#55405=CARTESIAN_POINT('Ctrl Pts',(4.28502486891387,-1.30000000000496,8.8175656188081));
#55406=CARTESIAN_POINT('Ctrl Pts',(4.20891602829725,-1.18514270861514,8.77783540491039));
#55407=CARTESIAN_POINT('Ctrl Pts',(4.14444540563363,-1.06847604194682,8.74356402580447));
#55408=CARTESIAN_POINT('Ctrl Pts',(4.02239198166675,-0.794772684000851,
8.67700128450959));
#55409=CARTESIAN_POINT('Ctrl Pts',(3.9750721515842,-0.636309800095197,8.65109465690009));
#55410=CARTESIAN_POINT('Ctrl Pts',(3.91380906647831,-0.319434907277159,
8.60889674750867));
#55411=CARTESIAN_POINT('Ctrl Pts',(3.90061191119441,-0.158333333333332,
8.59637205061778));
#55412=CARTESIAN_POINT('Ctrl Pts',(3.90745678965039,0.158333333333334,8.5770480695384));
#55413=CARTESIAN_POINT('Ctrl Pts',(3.9271390295546,0.319434907277167,8.57133011076225));
#55414=CARTESIAN_POINT('Ctrl Pts',(4.00307751336492,0.636309800095206,8.57196388006084));
#55415=CARTESIAN_POINT('Ctrl Pts',(4.05771050318434,0.79477268400084,8.57698201599421));
#55416=CARTESIAN_POINT('Ctrl Pts',(4.19526082558559,1.06847604194643,8.59960976409463));
#55417=CARTESIAN_POINT('Ctrl Pts',(4.26698198887019,1.18514270861437,8.61335123634875));
#55418=CARTESIAN_POINT('Ctrl Pts',(4.35088387761328,1.30000000000384,8.63103946714495));
#55419=CARTESIAN_POINT('Ctrl Pts',(4.28983548714786,-1.30000000000496,8.8248766281363));
#55420=CARTESIAN_POINT('Ctrl Pts',(4.21384120149965,-1.18514270861514,8.78447021791069));
#55421=CARTESIAN_POINT('Ctrl Pts',(4.14921392203966,-1.06847604194682,8.75005834837911));
#55422=CARTESIAN_POINT('Ctrl Pts',(4.02617203610171,-0.794772684000851,
8.68440863389773));
#55423=CARTESIAN_POINT('Ctrl Pts',(3.9768459243883,-0.636309800095197,8.66155018583716));
#55424=CARTESIAN_POINT('Ctrl Pts',(3.91457783683306,-0.319434907277159,
8.62081822041216));
#55425=CARTESIAN_POINT('Ctrl Pts',(3.90175138019541,-0.158333333333332,
8.60789341040585));
#55426=CARTESIAN_POINT('Ctrl Pts',(3.90875262150677,0.158333333333334,8.58839155923708));
#55427=CARTESIAN_POINT('Ctrl Pts',(3.92838285746568,0.319434907277167,8.58266762337897));
#55428=CARTESIAN_POINT('Ctrl Pts',(4.00531418532213,0.636309800095206,8.58193800807378));
#55429=CARTESIAN_POINT('Ctrl Pts',(4.06137678322636,0.79477268400084,8.58482558447746));
#55430=CARTESIAN_POINT('Ctrl Pts',(4.19998727431994,1.06847604194643,8.60640446367549));
#55431=CARTESIAN_POINT('Ctrl Pts',(4.2720251072689,1.18514270861437,8.62000938469766));
#55432=CARTESIAN_POINT('Ctrl Pts',(4.35610142759692,1.30000000000384,8.63787852951341));
#55433=CARTESIAN_POINT('Ctrl Pts',(4.29930376072963,-1.30000000000496,8.83268461488515));
#55434=CARTESIAN_POINT('Ctrl Pts',(4.2262195627153,-1.18514270861514,8.79214240758744));
#55435=CARTESIAN_POINT('Ctrl Pts',(4.16336519692289,-1.06847604194682,8.75816761714088));
#55436=CARTESIAN_POINT('Ctrl Pts',(4.04179199687415,-0.794772684000852,
8.69485110130973));
#55437=CARTESIAN_POINT('Ctrl Pts',(3.98908680587602,-0.636309800095197,
8.67637440288014));
#55438=CARTESIAN_POINT('Ctrl Pts',(3.92522495352783,-0.319434907277159,
8.63802912135571));
#55439=CARTESIAN_POINT('Ctrl Pts',(3.9116447724459,-0.158333333333332,8.6244628589329));
#55440=CARTESIAN_POINT('Ctrl Pts',(3.91874146174287,0.158333333333334,8.60483888933969));
#55441=CARTESIAN_POINT('Ctrl Pts',(3.93921600502161,0.319434907277167,8.5998008173125));
#55442=CARTESIAN_POINT('Ctrl Pts',(4.01794542822412,0.636309800095206,8.59609656237777));
#55443=CARTESIAN_POINT('Ctrl Pts',(4.07761409240379,0.794772684000841,8.59344330335423));
#55444=CARTESIAN_POINT('Ctrl Pts',(4.21475015139629,1.06847604194643,8.6127300716576));
#55445=CARTESIAN_POINT('Ctrl Pts',(4.28494704343638,1.18514270861437,8.62620793882529));
#55446=CARTESIAN_POINT('Ctrl Pts',(4.36597970897014,1.30000000000384,8.64481514580727));
#55447=CARTESIAN_POINT('Ctrl Pts',(4.31312792074545,-1.30000000000496,8.84424454249127));
#55448=CARTESIAN_POINT('Ctrl Pts',(4.243424146701,-1.18514270861514,8.80514758315398));
#55449=CARTESIAN_POINT('Ctrl Pts',(4.18297452507387,-1.06847604194682,8.77242899407481));
#55450=CARTESIAN_POINT('Ctrl Pts',(4.0647027495816,-0.794772684000851,8.71157781925591));
#55451=CARTESIAN_POINT('Ctrl Pts',(4.01090852828359,-0.636309800095196,
8.69427998926102));
#55452=CARTESIAN_POINT('Ctrl Pts',(3.94667172175643,-0.319434907277159,
8.65719965161783));
#55453=CARTESIAN_POINT('Ctrl Pts',(3.93163133024526,-0.158333333333332,
8.64372198961442));
#55454=CARTESIAN_POINT('Ctrl Pts',(3.93874497628404,0.158333333333334,8.62400686072403));
#55455=CARTESIAN_POINT('Ctrl Pts',(3.96054477515934,0.319434907277168,8.6190912105333));
#55456=CARTESIAN_POINT('Ctrl Pts',(4.03999312514226,0.636309800095207,8.61332080472688));
#55457=CARTESIAN_POINT('Ctrl Pts',(4.10152595983501,0.794772684000841,8.60777135386286));
#55458=CARTESIAN_POINT('Ctrl Pts',(4.23547535188849,1.06847604194643,8.6244638114006));
#55459=CARTESIAN_POINT('Ctrl Pts',(4.30315793171355,1.18514270861437,8.63701391339769));
#55460=CARTESIAN_POINT('Ctrl Pts',(4.38054136285748,1.30000000000383,8.65488857104023));
#55461=CARTESIAN_POINT('Ctrl Pts',(4.3244187971589,-1.30000000000496,8.85410663226077));
#55462=CARTESIAN_POINT('Ctrl Pts',(4.25707252974643,-1.18514270861514,8.81642818419089));
#55463=CARTESIAN_POINT('Ctrl Pts',(4.19840048318692,-1.06847604194682,8.78460695411973));
#55464=CARTESIAN_POINT('Ctrl Pts',(4.08289550377498,-0.794772684000848,
8.72462489215008));
#55465=CARTESIAN_POINT('Ctrl Pts',(4.02927403638533,-0.636309800095195,
8.70556215389797));
#55466=CARTESIAN_POINT('Ctrl Pts',(3.96499593377808,-0.319434907277158,
8.66861314096609));
#55467=CARTESIAN_POINT('Ctrl Pts',(3.94838335269583,-0.158333333333332,
8.65630976419325));
#55468=CARTESIAN_POINT('Ctrl Pts',(3.95524198209584,0.158333333333334,8.63711868842999));
#55469=CARTESIAN_POINT('Ctrl Pts',(3.97797880426114,0.319434907277165,8.63237791717527));
#55470=CARTESIAN_POINT('Ctrl Pts',(4.05772333724245,0.636309800095204,8.62586295336701));
#55471=CARTESIAN_POINT('Ctrl Pts',(4.12042170706468,0.794772684000838,8.61906302296074));
#55472=CARTESIAN_POINT('Ctrl Pts',(4.25186429647709,1.06847604194643,8.63440942857542));
#55473=CARTESIAN_POINT('Ctrl Pts',(4.31765404311617,1.18514270861437,8.64639681988873));
#55474=CARTESIAN_POINT('Ctrl Pts',(4.39233690986531,1.30000000000383,8.66372871216506));
#55475=CARTESIAN_POINT('Ctrl Pts',(4.33572321977573,-1.30000000000496,8.86421064164255));
#55476=CARTESIAN_POINT('Ctrl Pts',(4.27092732418113,-1.18514270861514,8.82814842879662));
#55477=CARTESIAN_POINT('Ctrl Pts',(4.21419946894931,-1.06847604194682,8.79734935690205));
#55478=CARTESIAN_POINT('Ctrl Pts',(4.10178556224008,-0.794772684000849,
8.73835624797819));
#55479=CARTESIAN_POINT('Ctrl Pts',(4.04840193500903,-0.636309800095196,
8.71754578928925));
#55480=CARTESIAN_POINT('Ctrl Pts',(3.98441167665988,-0.319434907277159,
8.68022362769928));
#55481=CARTESIAN_POINT('Ctrl Pts',(3.9663377392371,-0.158333333333332,8.66871093771688));
#55482=CARTESIAN_POINT('Ctrl Pts',(3.97352620747206,0.158333333333334,8.64870668848889));
#55483=CARTESIAN_POINT('Ctrl Pts',(3.99824681020785,0.319434907277166,8.64186510293906));
#55484=CARTESIAN_POINT('Ctrl Pts',(4.07798307430565,0.636309800095205,8.63507917158918));
#55485=CARTESIAN_POINT('Ctrl Pts',(4.14019739114876,0.79477268400084,8.63069489993545));
#55486=CARTESIAN_POINT('Ctrl Pts',(4.26838958459523,1.06847604194643,8.64554477741727));
#55487=CARTESIAN_POINT('Ctrl Pts',(4.33215125685333,1.18514270861437,8.65676559192588));
#55488=CARTESIAN_POINT('Ctrl Pts',(4.40418495081513,1.30000000000384,8.67277925922339));
#55489=CARTESIAN_POINT('Ctrl Pts',(4.34626852229784,-1.30000000000496,8.87552627072083));
#55490=CARTESIAN_POINT('Ctrl Pts',(4.28392604793638,-1.18514270861514,8.84094205580928));
#55491=CARTESIAN_POINT('Ctrl Pts',(4.2291044621075,-1.06847604194682,8.81099126755198));
#55492=CARTESIAN_POINT('Ctrl Pts',(4.11983038888185,-0.794772684000851,
8.75250309752858));
#55493=CARTESIAN_POINT('Ctrl Pts',(4.06679618167507,-0.636309800095197,
8.72976507628461));
#55494=CARTESIAN_POINT('Ctrl Pts',(4.00358038221854,-0.319434907277159,
8.69098406914389));
#55495=CARTESIAN_POINT('Ctrl Pts',(3.98490986621235,-0.158333333333332,
8.67847487346248));
#55496=CARTESIAN_POINT('Ctrl Pts',(3.99231677038997,0.158333333333334,8.65788882672129));
#55497=CARTESIAN_POINT('Ctrl Pts',(4.01788418085971,0.319434907277166,8.65128274813801));
#55498=CARTESIAN_POINT('Ctrl Pts',(4.0972261638769,0.636309800095205,8.64513560267597));
#55499=CARTESIAN_POINT('Ctrl Pts',(4.15925187332272,0.79477268400084,8.64255931406753));
#55500=CARTESIAN_POINT('Ctrl Pts',(4.28452235248451,1.06847604194643,8.65666215032348));
#55501=CARTESIAN_POINT('Ctrl Pts',(4.34645140535157,1.18514270861437,8.6669808430935));
#55502=CARTESIAN_POINT('Ctrl Pts',(4.41608456238495,1.30000000000383,8.68151363337989));
#55503=CARTESIAN_POINT('Ctrl Pts',(4.36422521226682,-1.30000000000495,8.89174180979307));
#55504=CARTESIAN_POINT('Ctrl Pts',(4.30586457287734,-1.18514270861514,8.85961335725795));
#55505=CARTESIAN_POINT('Ctrl Pts',(4.25405375016242,-1.06847604194682,8.83124862077492));
#55506=CARTESIAN_POINT('Ctrl Pts',(4.14949177177681,-0.794772684000853,
8.77441534216264));
#55507=CARTESIAN_POINT('Ctrl Pts',(4.09637737283048,-0.636309800095197,
8.74984090708147));
#55508=CARTESIAN_POINT('Ctrl Pts',(4.03399467514183,-0.319434907277159,
8.70955638867894));
#55509=CARTESIAN_POINT('Ctrl Pts',(4.01440519392537,-0.158333333333332,
8.69526969200356));
#55510=CARTESIAN_POINT('Ctrl Pts',(4.02204202455759,0.158333333333334,8.67410888232258));
#55511=CARTESIAN_POINT('Ctrl Pts',(4.04885947795462,0.319434907277165,8.66843761565224));
#55512=CARTESIAN_POINT('Ctrl Pts',(4.12763066499831,0.636309800095204,8.66316897698633));
#55513=CARTESIAN_POINT('Ctrl Pts',(4.18973120740827,0.794772684000841,8.66243987109688));
#55514=CARTESIAN_POINT('Ctrl Pts',(4.31019462438223,1.06847604194643,8.67527067605611));
#55515=CARTESIAN_POINT('Ctrl Pts',(4.36902600111067,1.18514270861437,8.68431305960336));
#55516=CARTESIAN_POINT('Ctrl Pts',(4.43454460496874,1.30000000000384,8.69684384665918));
#55517=CARTESIAN_POINT('Ctrl Pts',(4.38767994763338,-1.30000000000497,8.91609640196983));
#55518=CARTESIAN_POINT('Ctrl Pts',(4.33410494967261,-1.18514270861515,8.88837512378823));
#55519=CARTESIAN_POINT('Ctrl Pts',(4.28604603319652,-1.06847604194683,8.86275198152183));
#55520=CARTESIAN_POINT('Ctrl Pts',(4.1877635737022,-0.794772684000858,8.80840451068953));
#55521=CARTESIAN_POINT('Ctrl Pts',(4.13559346017687,-0.636309800095199,
8.7795612982255));
#55522=CARTESIAN_POINT('Ctrl Pts',(4.07488993204494,-0.319434907277158,
8.73635149198173));
#55523=CARTESIAN_POINT('Ctrl Pts',(4.054100148061,-0.158333333333332,8.71968410253834));
#55524=CARTESIAN_POINT('Ctrl Pts',(4.06223420124964,0.158333333333334,8.69731819149294));
#55525=CARTESIAN_POINT('Ctrl Pts',(4.09083196103889,0.319434907277167,8.69244165562464));
#55526=CARTESIAN_POINT('Ctrl Pts',(4.16876816599636,0.636309800095206,8.68841938571338));
#55527=CARTESIAN_POINT('Ctrl Pts',(4.2305305830476,0.794772684000839,8.69127158429364));
#55528=CARTESIAN_POINT('Ctrl Pts',(4.3446903395284,1.06847604194643,8.70198094260544));
#55529=CARTESIAN_POINT('Ctrl Pts',(4.39955289097199,1.18514270861438,8.70881915620342));
#55530=CARTESIAN_POINT('Ctrl Pts',(4.45986246531419,1.30000000000385,8.717859899007));
#55531=CARTESIAN_POINT('Ctrl Pts',(4.41533706763821,-1.30000000000497,8.94499626631974));
#55532=CARTESIAN_POINT('Ctrl Pts',(4.36794300895912,-1.18514270861515,8.92167148680998));
#55533=CARTESIAN_POINT('Ctrl Pts',(4.32451940762636,-1.06847604194683,8.89904773381702));
#55534=CARTESIAN_POINT('Ctrl Pts',(4.23337475244403,-0.79477268400086,8.84840185003111));
#55535=CARTESIAN_POINT('Ctrl Pts',(4.1806055452744,-0.636309800095201,8.81775565383643));
#55536=CARTESIAN_POINT('Ctrl Pts',(4.12134692798048,-0.31943490727716,8.77220167135861));
#55537=CARTESIAN_POINT('Ctrl Pts',(4.09987465453343,-0.158333333333333,
8.75128226254503));
#55538=CARTESIAN_POINT('Ctrl Pts',(4.10853203043528,0.158333333333335,8.72782643002757));
#55539=CARTESIAN_POINT('Ctrl Pts',(4.13856365854856,0.319434907277167,8.72560883261724));
#55540=CARTESIAN_POINT('Ctrl Pts',(4.21565638940201,0.636309800095208,8.72273554692928));
#55541=CARTESIAN_POINT('Ctrl Pts',(4.27778957553113,0.794772684000846,8.72786458211374));
#55542=CARTESIAN_POINT('Ctrl Pts',(4.3849967272625,1.06847604194643,8.73475299590499));
#55543=CARTESIAN_POINT('Ctrl Pts',(4.43532980429784,1.18514270861438,8.73853999810118));
#55544=CARTESIAN_POINT('Ctrl Pts',(4.48958995480018,1.30000000000384,8.7431322634042));
#55545=CARTESIAN_POINT('Ctrl Pts',(4.43404520828974,-1.30000000000497,8.96568188497049));
#55546=CARTESIAN_POINT('Ctrl Pts',(4.39031687507281,-1.18514270861515,8.94641560147379));
#55547=CARTESIAN_POINT('Ctrl Pts',(4.34974854817529,-1.06847604194683,8.92645120558581));
#55548=CARTESIAN_POINT('Ctrl Pts',(4.26332784413169,-0.794772684000854,
8.87871667794048));
#55549=CARTESIAN_POINT('Ctrl Pts',(4.21117558585354,-0.636309800095199,
8.84503073916913));
#55550=CARTESIAN_POINT('Ctrl Pts',(4.15303192935944,-0.31943490727716,8.79778076666981));
#55551=CARTESIAN_POINT('Ctrl Pts',(4.13046881562288,-0.158333333333333,
8.77524556471387));
#55552=CARTESIAN_POINT('Ctrl Pts',(4.1394779046875,0.158333333333335,8.75106187745542));
#55553=CARTESIAN_POINT('Ctrl Pts',(4.17089728038284,0.319434907277167,8.74974959162166));
#55554=CARTESIAN_POINT('Ctrl Pts',(4.24770310043635,0.636309800095207,8.74705432034812));
#55555=CARTESIAN_POINT('Ctrl Pts',(4.31030454314704,0.794772684000842,8.75340274182129));
#55556=CARTESIAN_POINT('Ctrl Pts',(4.4126725008907,1.06847604194643,8.7577656338405));
#55557=CARTESIAN_POINT('Ctrl Pts',(4.45978245913997,1.18514270861438,8.7596488012543));
#55558=CARTESIAN_POINT('Ctrl Pts',(4.50969107983768,1.30000000000385,8.76152660178787));
#55559=CARTESIAN_POINT('Ctrl Pts',(4.44619000963321,-1.30000000000497,8.98001366847455));
#55560=CARTESIAN_POINT('Ctrl Pts',(4.40525777118481,-1.18514270861515,8.9628531698774));
#55561=CARTESIAN_POINT('Ctrl Pts',(4.36679375885251,-1.06847604194683,8.94432506201643));
#55562=CARTESIAN_POINT('Ctrl Pts',(4.28363629176136,-0.794772684000856,
8.89836197533397));
#55563=CARTESIAN_POINT('Ctrl Pts',(4.23135175689816,-0.636309800095199,
8.86361341927445));
#55564=CARTESIAN_POINT('Ctrl Pts',(4.17374064951435,-0.319434907277159,
8.81562502062927));
#55565=CARTESIAN_POINT('Ctrl Pts',(4.15051793125772,-0.158333333333333,
8.79189493686576));
#55566=CARTESIAN_POINT('Ctrl Pts',(4.1597041449006,0.158333333333334,8.76736032302134));
#55567=CARTESIAN_POINT('Ctrl Pts',(4.19200174471018,0.319434907277166,8.76678545613091));
#55568=CARTESIAN_POINT('Ctrl Pts',(4.26855128330622,0.636309800095206,8.76433080554314));
#55569=CARTESIAN_POINT('Ctrl Pts',(4.33129030207517,0.794772684000839,8.77178079794625));
#55570=CARTESIAN_POINT('Ctrl Pts',(4.43064562884352,1.06847604194643,8.77401583737565));
#55571=CARTESIAN_POINT('Ctrl Pts',(4.47578660915789,1.18514270861438,8.77427158274088));
#55572=CARTESIAN_POINT('Ctrl Pts',(4.52306133030603,1.30000000000385,8.77381560771872));
#55573=CARTESIAN_POINT('Ctrl Pts',(4.45453765168186,-1.30000000000497,8.98912942527086));
#55574=CARTESIAN_POINT('Ctrl Pts',(4.41512586643895,-1.18514270861515,8.97395729129967));
#55575=CARTESIAN_POINT('Ctrl Pts',(4.37783983971279,-1.06847604194683,8.9567713308798));
#55576=CARTESIAN_POINT('Ctrl Pts',(4.2966125863621,-0.794772684000855,8.9124159823096));
#55577=CARTESIAN_POINT('Ctrl Pts',(4.24448056452864,-0.636309800095199,
8.87657622648389));
#55578=CARTESIAN_POINT('Ctrl Pts',(4.18740615513335,-0.31943490727716,8.82777629898448));
#55579=CARTESIAN_POINT('Ctrl Pts',(4.16398183654532,-0.158333333333333,
8.80279462257431));
#55580=CARTESIAN_POINT('Ctrl Pts',(4.17332167501868,0.158333333333335,8.77796636634553));
#55581=CARTESIAN_POINT('Ctrl Pts',(4.20602135108615,0.319434907277167,8.77823311288337));
#55582=CARTESIAN_POINT('Ctrl Pts',(4.28225168210284,0.636309800095207,8.77622883251019));
#55583=CARTESIAN_POINT('Ctrl Pts',(4.34500767159721,0.794772684000841,8.78455925488412));
#55584=CARTESIAN_POINT('Ctrl Pts',(4.44225791319782,1.06847604194643,8.78557151883606));
#55585=CARTESIAN_POINT('Ctrl Pts',(4.48605228741681,1.18514270861438,8.78481316963859));
#55586=CARTESIAN_POINT('Ctrl Pts',(4.53154500974223,1.30000000000385,8.78285829968693));
#55587=CARTESIAN_POINT('Ctrl Pts',(4.4649410339563,-1.30000000000497,9.00056527592849));
#55588=CARTESIAN_POINT('Ctrl Pts',(4.42761818610944,-1.18514270861515,8.9875491573474));
#55589=CARTESIAN_POINT('Ctrl Pts',(4.39191905643545,-1.06847604194683,8.97183901834883));
#55590=CARTESIAN_POINT('Ctrl Pts',(4.31319803910584,-0.794772684000856,
8.92932172835859));
#55591=CARTESIAN_POINT('Ctrl Pts',(4.26103365036649,-0.6363098000952,8.89248633726872));
#55592=CARTESIAN_POINT('Ctrl Pts',(4.20452828810145,-0.319434907277159,
8.84285662377426));
#55593=CARTESIAN_POINT('Ctrl Pts',(4.18080445888963,-0.158333333333333,
8.81643061427704));
#55594=CARTESIAN_POINT('Ctrl Pts',(4.19035476432787,0.158333333333335,8.79120304025113));
#55595=CARTESIAN_POINT('Ctrl Pts',(4.22354972932494,0.319434907277167,8.79252163388763));
#55596=CARTESIAN_POINT('Ctrl Pts',(4.29966963900563,0.636309800095207,8.79051984200613));
#55597=CARTESIAN_POINT('Ctrl Pts',(4.36290981102847,0.794772684000841,8.79907206384702));
#55598=CARTESIAN_POINT('Ctrl Pts',(4.4577640286338,1.06847604194643,8.7980867009406));
#55599=CARTESIAN_POINT('Ctrl Pts',(4.49991041851912,1.18514270861438,8.79598035517156));
#55600=CARTESIAN_POINT('Ctrl Pts',(4.54314432218328,1.30000000000385,8.79219419072437));
#55601=CARTESIAN_POINT('Ctrl Pts',(4.47689956690015,-1.30000000000497,9.01516635057687));
#55602=CARTESIAN_POINT('Ctrl Pts',(4.44225166083132,-1.18514270861515,9.00445134978857));
#55603=CARTESIAN_POINT('Ctrl Pts',(4.40859270265779,-1.06847604194683,8.99028169280819));
#55604=CARTESIAN_POINT('Ctrl Pts',(4.3331184433025,-0.794772684000854,8.94956600364834));
#55605=CARTESIAN_POINT('Ctrl Pts',(4.28115576151042,-0.636309800095201,
8.9111123353338));
#55606=CARTESIAN_POINT('Ctrl Pts',(4.22506688969079,-0.319434907277161,
8.86098093531374));
#55607=CARTESIAN_POINT('Ctrl Pts',(4.20028938187868,-0.158333333333333,
8.83407467074119));
#55608=CARTESIAN_POINT('Ctrl Pts',(4.20975340442327,0.158333333333335,8.80898190960155));
#55609=CARTESIAN_POINT('Ctrl Pts',(4.24374949284336,0.319434907277167,8.81117674665288));
#55610=CARTESIAN_POINT('Ctrl Pts',(4.31961584470656,0.636309800095208,8.80941924984648));
#55611=CARTESIAN_POINT('Ctrl Pts',(4.38319093328862,0.794772684000844,8.81871083360723));
#55612=CARTESIAN_POINT('Ctrl Pts',(4.47509038699624,1.06847604194644,8.81552607287147));
#55613=CARTESIAN_POINT('Ctrl Pts',(4.51526700412506,1.18514270861438,8.8118155481022));
#55614=CARTESIAN_POINT('Ctrl Pts',(4.55584037008276,1.30000000000385,8.80577306347917));
#55615=CARTESIAN_POINT('Ctrl Pts',(4.48897649417153,-1.30000000000497,9.02949874664839));
#55616=CARTESIAN_POINT('Ctrl Pts',(4.45636582527148,-1.18514270861515,9.02211642542208));
#55617=CARTESIAN_POINT('Ctrl Pts',(4.42429681123459,-1.06847604194683,9.01022573801647));
#55618=CARTESIAN_POINT('Ctrl Pts',(4.35146230451729,-0.794772684000857,
8.97234064361614));
#55619=CARTESIAN_POINT('Ctrl Pts',(4.29967282671666,-0.636309800095202,
8.9324359539744));
#55620=CARTESIAN_POINT('Ctrl Pts',(4.24460051930937,-0.319434907277161,
8.88080222914568));
#55621=CARTESIAN_POINT('Ctrl Pts',(4.21986464943619,-0.158333333333333,
8.85150900811807));
#55622=CARTESIAN_POINT('Ctrl Pts',(4.2300599323088,0.158333333333335,8.82510783226668));
#55623=CARTESIAN_POINT('Ctrl Pts',(4.26511440832616,0.319434907277168,8.82767716361691));
#55624=CARTESIAN_POINT('Ctrl Pts',(4.34070257223563,0.636309800095209,8.82619093901148));
#55625=CARTESIAN_POINT('Ctrl Pts',(4.40385706271878,0.794772684000845,8.83759526436711));
#55626=CARTESIAN_POINT('Ctrl Pts',(4.49278112351848,1.06847604194644,8.83220749269224));
#55627=CARTESIAN_POINT('Ctrl Pts',(4.53112363495319,1.18514270861438,8.82662108018919));
#55628=CARTESIAN_POINT('Ctrl Pts',(4.56931672686336,1.30000000000385,8.81778042190455));
#55629=CARTESIAN_POINT('Ctrl Pts',(4.50119014476422,-1.30000000000497,9.04363299068084));
#55630=CARTESIAN_POINT('Ctrl Pts',(4.47137138258233,-1.18514270861515,9.03834985209589));
#55631=CARTESIAN_POINT('Ctrl Pts',(4.44134828489834,-1.06847604194683,9.02798673076185));
#55632=CARTESIAN_POINT('Ctrl Pts',(4.37151686726173,-0.794772684000857,
8.99231007094768));
#55633=CARTESIAN_POINT('Ctrl Pts',(4.31915516652733,-0.636309800095201,
8.95209331628435));
#55634=CARTESIAN_POINT('Ctrl Pts',(4.26435157519034,-0.319434907277161,
8.90021066968859));
#55635=CARTESIAN_POINT('Ctrl Pts',(4.23913849393376,-0.158333333333333,
8.86945988638939));
#55636=CARTESIAN_POINT('Ctrl Pts',(4.24922113999326,0.158333333333335,8.84326434603573));
#55637=CARTESIAN_POINT('Ctrl Pts',(4.28443545905308,0.319434907277168,8.84786052209751));
#55638=CARTESIAN_POINT('Ctrl Pts',(4.3599424971951,0.636309800095209,8.84630136132387));
#55639=CARTESIAN_POINT('Ctrl Pts',(4.42436953276321,0.794772684000845,8.8567291738621));
#55640=CARTESIAN_POINT('Ctrl Pts',(4.51055686536067,1.06847604194644,8.84875895539504));
#55641=CARTESIAN_POINT('Ctrl Pts',(4.54687289339834,1.18514270861438,8.8416827346635));
#55642=CARTESIAN_POINT('Ctrl Pts',(4.58219764674743,1.30000000000385,8.83098030544912));
#55643=CARTESIAN_POINT('Ctrl Pts',(4.51708986244,-1.30000000000497,9.06302202413031));
#55644=CARTESIAN_POINT('Ctrl Pts',(4.49007411997201,-1.18514270861515,9.06200911533405));
#55645=CARTESIAN_POINT('Ctrl Pts',(4.46224233834228,-1.06847604194683,9.05454625268663));
#55646=CARTESIAN_POINT('Ctrl Pts',(4.3960601413376,-0.794772684000856,9.02240486332576));
#55647=CARTESIAN_POINT('Ctrl Pts',(4.34416897458864,-0.636309800095202,
8.97984128700459));
#55648=CARTESIAN_POINT('Ctrl Pts',(4.29038389170619,-0.319434907277162,
8.92658673382167));
#55649=CARTESIAN_POINT('Ctrl Pts',(4.26449353889939,-0.158333333333333,
8.89399392534927));
#55650=CARTESIAN_POINT('Ctrl Pts',(4.27513479329512,0.158333333333335,8.86682608840896));
#55651=CARTESIAN_POINT('Ctrl Pts',(4.31180224590399,0.319434907277168,8.87185929610473));
#55652=CARTESIAN_POINT('Ctrl Pts',(4.38698609048331,0.63630980009521,8.87057291631606));
#55653=CARTESIAN_POINT('Ctrl Pts',(4.45109551779406,0.794772684000846,8.88332483627587));
#55654=CARTESIAN_POINT('Ctrl Pts',(4.53337656398258,1.06847604194644,8.87234725348443));
#55655=CARTESIAN_POINT('Ctrl Pts',(4.56723495535358,1.18514270861439,8.86282861704834));
#55656=CARTESIAN_POINT('Ctrl Pts',(4.59933532201359,1.30000000000385,8.84854313300709));
#55657=CARTESIAN_POINT('Ctrl Pts',(4.52945512605073,-1.30000000000498,9.0796760470566));
#55658=CARTESIAN_POINT('Ctrl Pts',(4.50520200778997,-1.18514270861516,9.08131599846587));
#55659=CARTESIAN_POINT('Ctrl Pts',(4.47944179574346,-1.06847604194683,9.0757175030803));
#55660=CARTESIAN_POINT('Ctrl Pts',(4.41644886446555,-0.794772684000859,
9.04606159862226));
#55661=CARTESIAN_POINT('Ctrl Pts',(4.36440246445019,-0.636309800095204,
9.00247234903706));
#55662=CARTESIAN_POINT('Ctrl Pts',(4.31103754745527,-0.319434907277162,
8.94879399171032));
#55663=CARTESIAN_POINT('Ctrl Pts',(4.28435267089773,-0.158333333333334,
8.91513189120031));
#55664=CARTESIAN_POINT('Ctrl Pts',(4.29512809994144,0.158333333333336,8.88775363725623));
#55665=CARTESIAN_POINT('Ctrl Pts',(4.33268871755653,0.319434907277169,8.89369019344123));
#55666=CARTESIAN_POINT('Ctrl Pts',(4.40779807930735,0.636309800095212,8.89230842428382));
#55667=CARTESIAN_POINT('Ctrl Pts',(4.47236566437713,0.794772684000848,8.90564944314382));
#55668=CARTESIAN_POINT('Ctrl Pts',(4.55174598911817,1.06847604194644,8.89177115316105));
#55669=CARTESIAN_POINT('Ctrl Pts',(4.58362827123485,1.18514270861439,8.88025305729823));
#55670=CARTESIAN_POINT('Ctrl Pts',(4.61303203421851,1.30000000000385,8.86322426306484));
#55671=CARTESIAN_POINT('Ctrl Pts',(4.54140619220528,-1.30000000000498,9.09411954148937));
#55672=CARTESIAN_POINT('Ctrl Pts',(4.51930652660192,-1.18514270861516,9.09885640928562));
#55673=CARTESIAN_POINT('Ctrl Pts',(4.49517828166395,-1.06847604194683,9.0954364657231));
#55674=CARTESIAN_POINT('Ctrl Pts',(4.43475078494002,-0.794772684000859,
9.06869184593323));
#55675=CARTESIAN_POINT('Ctrl Pts',(4.38264124396578,-0.636309800095204,
9.02402001715036));
#55676=CARTESIAN_POINT('Ctrl Pts',(4.32984101530184,-0.319434907277163,
8.96966456229311));
#55677=CARTESIAN_POINT('Ctrl Pts',(4.30281425189962,-0.158333333333334,
8.93438845416319));
#55678=CARTESIAN_POINT('Ctrl Pts',(4.31386287852357,0.158333333333336,8.9065687867174));
#55679=CARTESIAN_POINT('Ctrl Pts',(4.352093867694,0.319434907277169,8.91357065040671));
#55680=CARTESIAN_POINT('Ctrl Pts',(4.42708240901013,0.636309800095211,8.91218538636726));
#55681=CARTESIAN_POINT('Ctrl Pts',(4.49204923449338,0.794772684000849,8.92612918110719));
#55682=CARTESIAN_POINT('Ctrl Pts',(4.56875388326351,1.06847604194644,8.90957401593609));
#55683=CARTESIAN_POINT('Ctrl Pts',(4.59882305789642,1.18514270861439,8.89619090930866));
#55684=CARTESIAN_POINT('Ctrl Pts',(4.62575880689679,1.30000000000385,8.87659081362708));
#55685=CARTESIAN_POINT('Ctrl Pts',(4.54912648699166,-1.30000000000498,9.10416325960802));
#55686=CARTESIAN_POINT('Ctrl Pts',(4.52879502626638,-1.18514270861516,9.11042192478117));
#55687=CARTESIAN_POINT('Ctrl Pts',(4.50594191402208,-1.06847604194684,9.10814700627611));
#55688=CARTESIAN_POINT('Ctrl Pts',(4.44732113352516,-0.794772684000862,
9.08317720399946));
#55689=CARTESIAN_POINT('Ctrl Pts',(4.39460181867289,-0.636309800095205,
9.03869202390378));
#55690=CARTESIAN_POINT('Ctrl Pts',(4.34203697549782,-0.319434907277163,
8.98411292642917));
#55691=CARTESIAN_POINT('Ctrl Pts',(4.31489287862101,-0.158333333333334,
8.94759833383886));
#55692=CARTESIAN_POINT('Ctrl Pts',(4.3263124676311,0.158333333333336,8.91917344459879));
#55693=CARTESIAN_POINT('Ctrl Pts',(4.36529744874918,0.319434907277169,8.92636274356103));
#55694=CARTESIAN_POINT('Ctrl Pts',(4.44026502444849,0.636309800095212,8.92487644722071));
#55695=CARTESIAN_POINT('Ctrl Pts',(4.505244095131,0.79477268400085,8.93965306842763));
#55696=CARTESIAN_POINT('Ctrl Pts',(4.58006936595371,1.06847604194644,8.92147834091787));
#55697=CARTESIAN_POINT('Ctrl Pts',(4.60891078384074,1.18514270861439,8.90688574169778));
#55698=CARTESIAN_POINT('Ctrl Pts',(4.63420453242497,1.30000000000386,8.88556770935661));
#55699=CARTESIAN_POINT('Ctrl Pts',(4.55955577529855,-1.30000000000498,9.11820985555783));
#55700=CARTESIAN_POINT('Ctrl Pts',(4.54105857280266,-1.18514270861516,9.1274941410361));
#55701=CARTESIAN_POINT('Ctrl Pts',(4.51964128858355,-1.06847604194684,9.12728996869032));
#55702=CARTESIAN_POINT('Ctrl Pts',(4.4634171045838,-0.794772684000861,9.10489805399411));
#55703=CARTESIAN_POINT('Ctrl Pts',(4.41100399482857,-0.636309800095205,
9.05887870635694));
#55704=CARTESIAN_POINT('Ctrl Pts',(4.35914697435268,-0.319434907277163,
9.00339740234672));
#55705=CARTESIAN_POINT('Ctrl Pts',(4.33177102369644,-0.158333333333334,
8.96527542330471));
#55706=CARTESIAN_POINT('Ctrl Pts',(4.34328698802605,0.158333333333336,8.9367192103428));
#55707=CARTESIAN_POINT('Ctrl Pts',(4.38252275214732,0.319434907277167,8.94549528055361));
#55708=CARTESIAN_POINT('Ctrl Pts',(4.4571365668548,0.636309800095211,8.94441818850174));
#55709=CARTESIAN_POINT('Ctrl Pts',(4.52234252698688,0.79477268400085,8.95997819955137));
#55710=CARTESIAN_POINT('Ctrl Pts',(4.59490732490742,1.06847604194644,8.93903467779169));
#55711=CARTESIAN_POINT('Ctrl Pts',(4.62226330419147,1.18514270861439,8.92244116718351));
#55712=CARTESIAN_POINT('Ctrl Pts',(4.64556465053033,1.30000000000386,8.898319820503));
#55713=CARTESIAN_POINT('Ctrl Pts',(4.56908022620465,-1.30000000000498,9.13090239008075));
#55714=CARTESIAN_POINT('Ctrl Pts',(4.55249723205479,-1.18514270861516,9.14253591637494));
#55715=CARTESIAN_POINT('Ctrl Pts',(4.53251137184418,-1.06847604194684,9.14400653961888));
#55716=CARTESIAN_POINT('Ctrl Pts',(4.47847873525912,-0.794772684000863,
9.12392563438181));
#55717=CARTESIAN_POINT('Ctrl Pts',(4.42581774727667,-0.636309800095209,
9.07734372287633));
#55718=CARTESIAN_POINT('Ctrl Pts',(4.37444674746134,-0.319434907277166,
9.02129387638326));
#55719=CARTESIAN_POINT('Ctrl Pts',(4.34694084754741,-0.158333333333335,
8.98160230860927));
#55720=CARTESIAN_POINT('Ctrl Pts',(4.35874071915001,0.158333333333337,8.95260057221036));
#55721=CARTESIAN_POINT('Ctrl Pts',(4.39852582926343,0.319434907277171,8.96226720782046));
#55722=CARTESIAN_POINT('Ctrl Pts',(4.47295593970602,0.636309800095217,8.96132678156408));
#55723=CARTESIAN_POINT('Ctrl Pts',(4.53827746161824,0.794772684000856,8.9777478532546));
#55724=CARTESIAN_POINT('Ctrl Pts',(4.60865612671007,1.06847604194645,8.95451974947366));
#55725=CARTESIAN_POINT('Ctrl Pts',(4.6345800275273,1.1851427086144,8.9362534324678));
#55726=CARTESIAN_POINT('Ctrl Pts',(4.65596351282986,1.30000000000386,8.90977538389685));
#55727=CARTESIAN_POINT('Ctrl Pts',(4.57550772428327,-1.30000000000498,9.1401299753939));
#55728=CARTESIAN_POINT('Ctrl Pts',(4.55998119412574,-1.18514270861516,9.1538323657346));
#55729=CARTESIAN_POINT('Ctrl Pts',(4.54085378640419,-1.06847604194684,9.15669030357686));
#55730=CARTESIAN_POINT('Ctrl Pts',(4.48834690061704,-0.794772684000866,
9.13823985702445));
#55731=CARTESIAN_POINT('Ctrl Pts',(4.43619211733095,-0.63630980009521,9.09023518980654));
#55732=CARTESIAN_POINT('Ctrl Pts',(4.38522319009914,-0.319434907277167,
9.03371831030787));
#55733=CARTESIAN_POINT('Ctrl Pts',(4.35714856386029,-0.158333333333335,
8.99369341011036));
#55734=CARTESIAN_POINT('Ctrl Pts',(4.36908576900311,0.158333333333337,8.96448317410072));
#55735=CARTESIAN_POINT('Ctrl Pts',(4.40945590413185,0.319434907277171,8.97445308559024));
#55736=CARTESIAN_POINT('Ctrl Pts',(4.48401021979826,0.636309800095217,8.97319151796637));
#55737=CARTESIAN_POINT('Ctrl Pts',(4.54973770956819,0.794772684000858,8.98966648233755));
#55738=CARTESIAN_POINT('Ctrl Pts',(4.61861542110489,1.06847604194645,8.96479170360382));
#55739=CARTESIAN_POINT('Ctrl Pts',(4.64346791710096,1.1851427086144,8.94547119712179));
#55740=CARTESIAN_POINT('Ctrl Pts',(4.66335829993943,1.30000000000386,8.91759755417022));
#55741=CARTESIAN_POINT('Ctrl Pts',(4.57881223363908,-1.30000000000498,9.14460699339319));
#55742=CARTESIAN_POINT('Ctrl Pts',(4.5639121987517,-1.18514270861516,9.15919665540848));
#55743=CARTESIAN_POINT('Ctrl Pts',(4.54525602294494,-1.06847604194684,9.16268537215633));
#55744=CARTESIAN_POINT('Ctrl Pts',(4.49347908773936,-0.794772684000865,
9.14509960145507));
#55745=CARTESIAN_POINT('Ctrl Pts',(4.44126851719988,-0.63630980009521,9.09684858201501));
#55746=CARTESIAN_POINT('Ctrl Pts',(4.39046492224128,-0.319434907277166,
9.04014749524157));
#55747=CARTESIAN_POINT('Ctrl Pts',(4.3623362735984,-0.158333333333335,8.99959933142438));
#55748=CARTESIAN_POINT('Ctrl Pts',(4.37435302808331,0.158333333333337,8.97027110368226));
#55749=CARTESIAN_POINT('Ctrl Pts',(4.41488519752389,0.319434907277171,8.98059839181612));
#55750=CARTESIAN_POINT('Ctrl Pts',(4.48937824100214,0.636309800095217,8.97937824996481));
#55751=CARTESIAN_POINT('Ctrl Pts',(4.5551624237004,0.794772684000857,8.99612661572198));
#55752=CARTESIAN_POINT('Ctrl Pts',(4.62333351307415,1.06847604194645,8.97035555419667));
#55753=CARTESIAN_POINT('Ctrl Pts',(4.64771955111663,1.1851427086144,8.95039248736616));
#55754=CARTESIAN_POINT('Ctrl Pts',(4.66698288859931,1.30000000000386,8.92162169132757));
#55755=CARTESIAN_POINT('Ctrl Pts',(4.5804691755298,-1.30000000000498,9.14683792771085));
#55756=CARTESIAN_POINT('Ctrl Pts',(4.56588770201385,-1.18514270861516,9.16186312841252));
#55757=CARTESIAN_POINT('Ctrl Pts',(4.5474687940014,-1.06847604194684,9.16566467794608));
#55758=CARTESIAN_POINT('Ctrl Pts',(4.49605219044009,-0.794772684000865,
9.1485181383841));
#55759=CARTESIAN_POINT('Ctrl Pts',(4.44379190666503,-0.63630980009521,9.10017678111588));
#55760=CARTESIAN_POINT('Ctrl Pts',(4.39306644821312,-0.319434907277166,
9.04339049217918));
#55761=CARTESIAN_POINT('Ctrl Pts',(4.36492491951435,-0.158333333333335,
9.00255930733304));
#55762=CARTESIAN_POINT('Ctrl Pts',(4.37698119812884,0.158333333333337,8.97317313112529));
#55763=CARTESIAN_POINT('Ctrl Pts',(4.41758632105313,0.319434907277172,8.98369197243874));
#55764=CARTESIAN_POINT('Ctrl Pts',(4.49203987838997,0.636309800095217,8.98250727246983));
#55765=CARTESIAN_POINT('Ctrl Pts',(4.55783977349975,0.794772684000857,8.99941342141394));
#55766=CARTESIAN_POINT('Ctrl Pts',(4.62566299182014,1.06847604194645,8.97318552162207));
#55767=CARTESIAN_POINT('Ctrl Pts',(4.64982268195567,1.1851427086144,8.95288994480363));
#55768=CARTESIAN_POINT('Ctrl Pts',(4.66878390411358,1.30000000000386,8.92365187714725));
#55769=CARTESIAN_POINT('Ctrl Pts',(4.58141951381765,-1.30000000000498,9.14810732654966));
#55770=CARTESIAN_POINT('Ctrl Pts',(4.56702335251096,-1.18514270861516,9.16337648868155));
#55771=CARTESIAN_POINT('Ctrl Pts',(4.54874135366842,-1.06847604194684,9.16735482092146));
#55772=CARTESIAN_POINT('Ctrl Pts',(4.49752921697429,-0.794772684000865,
9.15046148848517));
#55773=CARTESIAN_POINT('Ctrl Pts',(4.44522961904313,-0.63630980009521,9.10208506291557));
#55774=CARTESIAN_POINT('Ctrl Pts',(4.39454731060875,-0.319434907277166,
9.04525224300041));
#55775=CARTESIAN_POINT('Ctrl Pts',(4.36640635472226,-0.158333333333335,
9.00424699940882));
#55776=CARTESIAN_POINT('Ctrl Pts',(4.37848537183999,0.158333333333337,8.97482756115475));
#55777=CARTESIAN_POINT('Ctrl Pts',(4.41912746697037,0.319434907277171,8.98546326183054));
#55778=CARTESIAN_POINT('Ctrl Pts',(4.49355403117831,0.636309800095217,8.98430609907814));
#55779=CARTESIAN_POINT('Ctrl Pts',(4.55935772741226,0.794772684000857,9.00131124541432));
#55780=CARTESIAN_POINT('Ctrl Pts',(4.626983888122,1.06847604194645,8.97481946469352));
#55781=CARTESIAN_POINT('Ctrl Pts',(4.65101680698759,1.1851427086144,8.95432959774862));
#55782=CARTESIAN_POINT('Ctrl Pts',(4.66980978554356,1.30000000000386,8.92481717411571));
#55783=CARTESIAN_POINT('Ctrl Pts',(4.589495289761,-1.30000000000499,9.1588996934203));
#55784=CARTESIAN_POINT('Ctrl Pts',(4.57668584766636,-1.18514270861516,9.17622343193904));
#55785=CARTESIAN_POINT('Ctrl Pts',(4.55957141230676,-1.06847604194684,9.18169735807558));
#55786=CARTESIAN_POINT('Ctrl Pts',(4.51008824724248,-0.794772684000866,
9.16696778535652));
#55787=CARTESIAN_POINT('Ctrl Pts',(4.4574158485065,-0.63630980009521,9.11835068551886));
#55788=CARTESIAN_POINT('Ctrl Pts',(4.40707795604764,-0.319434907277166,
9.06115697298211));
#55789=CARTESIAN_POINT('Ctrl Pts',(4.37893625271658,-0.158333333333335,
9.01868349747425));
#55790=CARTESIAN_POINT('Ctrl Pts',(4.39121487505806,0.158333333333337,8.98897343669169));
#55791=CARTESIAN_POINT('Ctrl Pts',(4.43220026295886,0.319434907277172,9.0005578427106));
#55792=CARTESIAN_POINT('Ctrl Pts',(4.50639783396403,0.636309800095217,8.99963585647209));
#55793=CARTESIAN_POINT('Ctrl Pts',(4.57220265609131,0.794772684000856,9.01753081392735));
#55794=CARTESIAN_POINT('Ctrl Pts',(4.63814941728848,1.06847604194645,8.98880692016474));
#55795=CARTESIAN_POINT('Ctrl Pts',(4.66110791114137,1.1851427086144,8.96666319460686));
#55796=CARTESIAN_POINT('Ctrl Pts',(4.67847898949305,1.30000000000386,8.93480925277583));
#55797=CARTESIAN_POINT('Ctrl Pts',(4.60440976406856,-1.30000000000497,9.18026138249439));
#55798=CARTESIAN_POINT('Ctrl Pts',(4.59406355054399,-1.18514270861514,9.20232644769543));
#55799=CARTESIAN_POINT('Ctrl Pts',(4.57889302949929,-1.06847604194682,9.21106553327939));
#55800=CARTESIAN_POINT('Ctrl Pts',(4.53270097556317,-0.794772684000849,
9.20046889045802));
#55801=CARTESIAN_POINT('Ctrl Pts',(4.48064018084823,-0.636309800095198,
9.14943754449245));
#55802=CARTESIAN_POINT('Ctrl Pts',(4.43118040068378,-0.319434907277161,
9.09126173355088));
#55803=CARTESIAN_POINT('Ctrl Pts',(4.40227632851896,-0.158333333333333,
9.04717378278747));
#55804=CARTESIAN_POINT('Ctrl Pts',(4.41485754451359,0.158333333333335,9.01703496000808));
#55805=CARTESIAN_POINT('Ctrl Pts',(4.4566818611374,0.31943490727717,9.03014210602715));
#55806=CARTESIAN_POINT('Ctrl Pts',(4.53107809583426,0.63630980009521,9.02864236167228));
#55807=CARTESIAN_POINT('Ctrl Pts',(4.59817489800802,0.794772684000843,9.04610702271642));
#55808=CARTESIAN_POINT('Ctrl Pts',(4.66069269942063,1.06847604194643,9.01354866946066));
#55809=CARTESIAN_POINT('Ctrl Pts',(4.68114117144808,1.18514270861438,8.98904126395909));
#55810=CARTESIAN_POINT('Ctrl Pts',(4.69497647578415,1.30000000000384,8.95411975767454));
#55811=CARTESIAN_POINT('Ctrl Pts',(4.61912732702719,-1.30000000000496,9.20118553969072));
#55812=CARTESIAN_POINT('Ctrl Pts',(4.6114348104255,-1.18514270861514,9.22755231220806));
#55813=CARTESIAN_POINT('Ctrl Pts',(4.59827465857687,-1.06847604194682,9.23934512619528));
#55814=CARTESIAN_POINT('Ctrl Pts',(4.55524074391044,-0.794772684000851,
9.23292012593516));
#55815=CARTESIAN_POINT('Ctrl Pts',(4.50310673817058,-0.636309800095197,
9.18053241784251));
#55816=CARTESIAN_POINT('Ctrl Pts',(4.45431946760892,-0.319434907277159,
9.12169110392727));
#55817=CARTESIAN_POINT('Ctrl Pts',(4.42489047289185,-0.158333333333332,
9.07569994752371));
#55818=CARTESIAN_POINT('Ctrl Pts',(4.43792035692505,0.158333333333334,9.04492251267268));
#55819=CARTESIAN_POINT('Ctrl Pts',(4.48097546069836,0.319434907277167,9.05887937468661));
#55820=CARTESIAN_POINT('Ctrl Pts',(4.55508919941058,0.636309800095206,9.05758940224239));
#55821=CARTESIAN_POINT('Ctrl Pts',(4.62176651432713,0.79477268400084,9.07738490555604));
#55822=CARTESIAN_POINT('Ctrl Pts',(4.6812322428251,1.06847604194643,9.04047819815655));
#55823=CARTESIAN_POINT('Ctrl Pts',(4.69979673838051,1.18514270861437,9.01265747598786));
#55824=CARTESIAN_POINT('Ctrl Pts',(4.71118521904681,1.30000000000384,8.97299157775552));
#55825=CARTESIAN_POINT('Ctrl Pts',(4.62624077063439,-1.30000000000496,9.21200810313932));
#55826=CARTESIAN_POINT('Ctrl Pts',(4.61995220105635,-1.18514270861514,9.24039662831204));
#55827=CARTESIAN_POINT('Ctrl Pts',(4.60783501082454,-1.06847604194682,9.25364960997313));
#55828=CARTESIAN_POINT('Ctrl Pts',(4.566376597632,-0.794772684000851,9.24930051549322));
#55829=CARTESIAN_POINT('Ctrl Pts',(4.5139835392274,-0.636309800095197,9.19656574141252));
#55830=CARTESIAN_POINT('Ctrl Pts',(4.46556375514821,-0.319434907277159,
9.13735044965255));
#55831=CARTESIAN_POINT('Ctrl Pts',(4.43611716307415,-0.158333333333332,
9.09005714685182));
#55832=CARTESIAN_POINT('Ctrl Pts',(4.44941966576161,0.158333333333334,9.05889701834647));
#55833=CARTESIAN_POINT('Ctrl Pts',(4.49284772594685,0.319434907277167,9.07364899676505));
#55834=CARTESIAN_POINT('Ctrl Pts',(4.5669807465074,0.636309800095206,9.07220674691494));
#55835=CARTESIAN_POINT('Ctrl Pts',(4.63406245451013,0.79477268400084,9.09217501942727));
#55836=CARTESIAN_POINT('Ctrl Pts',(4.6919201451545,1.06847604194643,9.05326217342387));
#55837=CARTESIAN_POINT('Ctrl Pts',(4.70935397490034,1.18514270861437,9.02411271480519));
#55838=CARTESIAN_POINT('Ctrl Pts',(4.71917718395066,1.30000000000384,8.98265772673976));
#55839=CARTESIAN_POINT('',(4.63725822693025,1.2,8.93157042500954));
#55840=CARTESIAN_POINT('Ctrl Pts',(4.63725822693025,1.2,8.93157042500954));
#55841=CARTESIAN_POINT('Ctrl Pts',(4.63128124328469,1.20916376532628,8.92138093370866));
#55842=CARTESIAN_POINT('Ctrl Pts',(4.62563454624119,1.21806711335843,8.91099649596368));
#55843=CARTESIAN_POINT('Ctrl Pts',(4.61446044706189,1.23542033719071,8.89112890253183));
#55844=CARTESIAN_POINT('Ctrl Pts',(4.61284959590184,1.2377794891268,8.88867625506117));
#55845=CARTESIAN_POINT('Ctrl Pts',(4.59902849842327,1.25867388818129,8.86555040087628));
#55846=CARTESIAN_POINT('Ctrl Pts',(4.59370304156697,1.26674865903275,8.85652559222203));
#55847=CARTESIAN_POINT('Ctrl Pts',(4.58430375459195,1.28086893631048,8.84092122371427));
#55848=CARTESIAN_POINT('Ctrl Pts',(4.57606112972981,1.2931885321623,8.82736295603023));
#55849=CARTESIAN_POINT('Ctrl Pts',(4.57140911795195,1.30000000000385,8.82009835388732));
#55850=CARTESIAN_POINT('',(4.58017336109578,0.65383484136663,9.07736836607464));
#55851=CARTESIAN_POINT('Ctrl Pts',(4.58017336113235,0.653834841365347,9.07736836608417));
#55852=CARTESIAN_POINT('Ctrl Pts',(4.58629935664999,0.71749686228372,9.06242291265736));
#55853=CARTESIAN_POINT('Ctrl Pts',(4.59129975116674,0.764620654576998,9.05006536969652));
#55854=CARTESIAN_POINT('Ctrl Pts',(4.61047635077669,0.949828416998684,9.00201087745227));
#55855=CARTESIAN_POINT('Ctrl Pts',(4.6216073392214,1.05665100713802,8.9734845202946));
#55856=CARTESIAN_POINT('Ctrl Pts',(4.63725822693025,1.2,8.93157042500954));
#55857=CARTESIAN_POINT('',(4.52544944337377,-0.653834841531101,9.20569372922889));
#55858=CARTESIAN_POINT('Ctrl Pts',(4.52544944337376,-0.6538348415311,9.20569372922889));
#55859=CARTESIAN_POINT('Ctrl Pts',(4.49807563320008,-0.575992875294331,
9.17441322987441));
#55860=CARTESIAN_POINT('Ctrl Pts',(4.47549584426781,-0.493634267952995,
9.1474433434323));
#55861=CARTESIAN_POINT('Ctrl Pts',(4.44490715110221,-0.33812193113357,9.10711659987178));
#55862=CARTESIAN_POINT('Ctrl Pts',(4.43509965619256,-0.265647808821891,
9.09215933056172));
#55863=CARTESIAN_POINT('Ctrl Pts',(4.42552631194356,-0.129708474507909,
9.0697518790094));
#55864=CARTESIAN_POINT('Ctrl Pts',(4.42449090793631,-0.066620743275029,
9.06154502477452));
#55865=CARTESIAN_POINT('Ctrl Pts',(4.42937482211724,0.0595420623316575,
9.04914518506414));
#55866=CARTESIAN_POINT('Ctrl Pts',(4.43531371317915,0.122769838845346,9.04485596687489));
#55867=CARTESIAN_POINT('Ctrl Pts',(4.45561375097078,0.260120332718061,9.0406046621017));
#55868=CARTESIAN_POINT('Ctrl Pts',(4.47131835950836,0.333940862872961,9.0415746906149));
#55869=CARTESIAN_POINT('Ctrl Pts',(4.51500250949231,0.491202455585993,9.05172634132229));
#55870=CARTESIAN_POINT('Ctrl Pts',(4.54480743097227,0.57434536642225,9.06214198151124));
#55871=CARTESIAN_POINT('Ctrl Pts',(4.58017336108264,0.653834841383517,9.07736836601699));
#55872=CARTESIAN_POINT('',(4.55428580344216,-1.2,9.13932483626781));
#55873=CARTESIAN_POINT('Ctrl Pts',(4.55428580344216,-1.2,9.13932483626781));
#55874=CARTESIAN_POINT('Ctrl Pts',(4.55060440973257,-1.14982825705369,9.14797017447775));
#55875=CARTESIAN_POINT('Ctrl Pts',(4.54418965220607,-1.0610632869042,9.16298565727555));
#55876=CARTESIAN_POINT('Ctrl Pts',(4.53001580454928,-0.792138505468391,
9.195405511297));
#55877=CARTESIAN_POINT('Ctrl Pts',(4.52801179202698,-0.738397016064537,
9.19991229853613));
#55878=CARTESIAN_POINT('Ctrl Pts',(4.52544944337376,-0.653834841531101,
9.20569372922889));
#55879=CARTESIAN_POINT('Ctrl Pts',(4.4908419881269,-1.3,9.03162175071067));
#55880=CARTESIAN_POINT('Ctrl Pts',(4.50210674878835,-1.28289219427241,9.04930258333981));
#55881=CARTESIAN_POINT('Ctrl Pts',(4.51263386006301,-1.26612351152865,9.06776363958348));
#55882=CARTESIAN_POINT('Ctrl Pts',(4.52785419473793,-1.24234399593774,9.09305279140919));
#55883=CARTESIAN_POINT('Ctrl Pts',(4.53122248474684,-1.23728725185213,9.09811956679317));
#55884=CARTESIAN_POINT('Ctrl Pts',(4.54397312679041,-1.2167518469017,9.12075188380719));
#55885=CARTESIAN_POINT('Ctrl Pts',(4.54922724341664,-1.20832960273817,9.12994352731759));
#55886=CARTESIAN_POINT('Ctrl Pts',(4.55428580344217,-1.2,9.13932483626781));
#55887=CARTESIAN_POINT('Origin',(0.,1.25,7.2));
#55888=CARTESIAN_POINT('Origin',(0.,1.2,7.2));
#55889=CARTESIAN_POINT('Origin',(0.,0.92691742076555,7.2));
#55890=CARTESIAN_POINT('Origin',(0.,0.653834841531101,7.2));
#55891=CARTESIAN_POINT('Origin',(0.,0.,7.2));
#55892=CARTESIAN_POINT('Origin',(0.,-0.653834841531101,7.2));
#55893=CARTESIAN_POINT('Origin',(0.,-0.926917420765551,7.2));
#55894=CARTESIAN_POINT('Origin',(0.,-1.2,7.2));
#55895=CARTESIAN_POINT('Origin',(0.,-1.25,7.2));
#55896=CARTESIAN_POINT('Ctrl Pts',(4.48251875583964,-1.30000000000184,9.51420125914222));
#55897=CARTESIAN_POINT('Ctrl Pts',(4.50675280588356,-1.18514270861303,9.47916239086718));
#55898=CARTESIAN_POINT('Ctrl Pts',(4.51674956615302,-1.06847604194575,9.4467017355834));
#55899=CARTESIAN_POINT('Ctrl Pts',(4.50695309468149,-0.794772684000851,
9.37766731592577));
#55900=CARTESIAN_POINT('Ctrl Pts',(4.44722735233531,-0.636309800095197,
9.34117727403155));
#55901=CARTESIAN_POINT('Ctrl Pts',(4.39869447984843,-0.319434907277159,
9.28512064988765));
#55902=CARTESIAN_POINT('Ctrl Pts',(4.35867257917745,-0.158333333333332,
9.26271831194526));
#55903=CARTESIAN_POINT('Ctrl Pts',(4.37292795574814,0.158333333333334,9.23198243022624));
#55904=CARTESIAN_POINT('Ctrl Pts',(4.42777734501438,0.319434907277167,9.22222011637453));
#55905=CARTESIAN_POINT('Ctrl Pts',(4.50418204215397,0.636309800095206,9.21858026428182));
#55906=CARTESIAN_POINT('Ctrl Pts',(4.57842941556978,0.79477268400084,9.22222944316713));
#55907=CARTESIAN_POINT('Ctrl Pts',(4.6094025157868,1.06847604194648,9.25012893617736));
#55908=CARTESIAN_POINT('Ctrl Pts',(4.60766161389181,1.18514270861448,9.26800173905295));
#55909=CARTESIAN_POINT('Ctrl Pts',(4.59077270268428,1.30000000000399,9.29167068805804));
#55910=CARTESIAN_POINT('Ctrl Pts',(4.47625324740048,-1.30000000000184,9.51446562353792));
#55911=CARTESIAN_POINT('Ctrl Pts',(4.49929883545649,-1.18514270861303,9.4794437109002));
#55912=CARTESIAN_POINT('Ctrl Pts',(4.50842359237374,-1.06847604194575,9.44700748050992));
#55913=CARTESIAN_POINT('Ctrl Pts',(4.4973437014707,-0.794772684000851,9.37804674271844));
#55914=CARTESIAN_POINT('Ctrl Pts',(4.43781745126807,-0.636309800095197,
9.34164915954862));
#55915=CARTESIAN_POINT('Ctrl Pts',(4.38923444772865,-0.319434907277159,
9.28565064674039));
#55916=CARTESIAN_POINT('Ctrl Pts',(4.34963276865795,-0.158333333333332,
9.26312087075345));
#55917=CARTESIAN_POINT('Ctrl Pts',(4.36383715556681,0.158333333333334,9.23261432262395));
#55918=CARTESIAN_POINT('Ctrl Pts',(4.41819681569251,0.319434907277167,9.22328112308529));
#55919=CARTESIAN_POINT('Ctrl Pts',(4.49458550119995,0.636309800095206,9.21990293883793));
#55920=CARTESIAN_POINT('Ctrl Pts',(4.56861724441485,0.79477268400084,9.22357197712616));
#55921=CARTESIAN_POINT('Ctrl Pts',(4.60088880207979,1.06847604194648,9.25136235697374));
#55922=CARTESIAN_POINT('Ctrl Pts',(4.60003939698503,1.18514270861448,9.26913417417586));
#55923=CARTESIAN_POINT('Ctrl Pts',(4.58437142526133,1.30000000000399,9.29264838287906));
#55924=CARTESIAN_POINT('Ctrl Pts',(4.4636537898411,-1.30000000000163,9.5151766357535));
#55925=CARTESIAN_POINT('Ctrl Pts',(4.48437051028303,-1.18514270861284,9.48004204082684));
#55926=CARTESIAN_POINT('Ctrl Pts',(4.49178865623133,-1.06847604194558,9.44753738145579));
#55927=CARTESIAN_POINT('Ctrl Pts',(4.47820368991595,-0.794772684000723,
9.37852079302433));
#55928=CARTESIAN_POINT('Ctrl Pts',(4.4191182508642,-0.636309800095096,9.34213437097525));
#55929=CARTESIAN_POINT('Ctrl Pts',(4.37038259295847,-0.319434907277108,
9.28643717126287));
#55930=CARTESIAN_POINT('Ctrl Pts',(4.33146875773393,-0.158333333333307,
9.2642035768315));
#55931=CARTESIAN_POINT('Ctrl Pts',(4.34553130112576,0.158333333333309,9.23430515295839));
#55932=CARTESIAN_POINT('Ctrl Pts',(4.39899684163401,0.319434907277116,9.22553420796642));
#55933=CARTESIAN_POINT('Ctrl Pts',(4.47538050033928,0.636309800095105,9.22258354874013));
#55934=CARTESIAN_POINT('Ctrl Pts',(4.54896787756259,0.794772684000714,9.22632763177204));
#55935=CARTESIAN_POINT('Ctrl Pts',(4.58383417417162,1.06847604194631,9.25390659861801));
#55936=CARTESIAN_POINT('Ctrl Pts',(4.58476621776767,1.18514270861429,9.27148350566701));
#55937=CARTESIAN_POINT('Ctrl Pts',(4.57153797708125,1.30000000000378,9.29469940691876));
#55938=CARTESIAN_POINT('Ctrl Pts',(4.44507713121895,-1.3000000000013,9.51538739937688));
#55939=CARTESIAN_POINT('Ctrl Pts',(4.46185228716617,-1.18514270861254,9.48147746182544));
#55940=CARTESIAN_POINT('Ctrl Pts',(4.46643042464635,-1.06847604194531,9.44972969566701));
#55941=CARTESIAN_POINT('Ctrl Pts',(4.44882928541479,-0.794772684000524,
9.38138105318114));
#55942=CARTESIAN_POINT('Ctrl Pts',(4.390854245645,-0.636309800094935,9.34354911727094));
#55943=CARTESIAN_POINT('Ctrl Pts',(4.34213240301002,-0.319434907277027,
9.28744768961452));
#55944=CARTESIAN_POINT('Ctrl Pts',(4.30436347268256,-0.158333333333267,
9.26527844603672));
#55945=CARTESIAN_POINT('Ctrl Pts',(4.3183608160147,0.158333333333269,9.23567613861453));
#55946=CARTESIAN_POINT('Ctrl Pts',(4.37056632183711,0.319434907277035,9.22726662244557));
#55947=CARTESIAN_POINT('Ctrl Pts',(4.44690506070763,0.636309800094944,9.22505924439812));
#55948=CARTESIAN_POINT('Ctrl Pts',(4.51956844370301,0.794772684000513,9.22997966496454));
#55949=CARTESIAN_POINT('Ctrl Pts',(4.55835037802316,1.06847604194604,9.25723650525971));
#55950=CARTESIAN_POINT('Ctrl Pts',(4.56202364758899,1.18514270861399,9.27430113235338));
#55951=CARTESIAN_POINT('Ctrl Pts',(4.55258292436565,1.30000000000345,9.29663191034234));
#55952=CARTESIAN_POINT('Ctrl Pts',(4.42643317267789,-1.30000000000096,9.515578775066));
#55953=CARTESIAN_POINT('Ctrl Pts',(4.43974876127799,-1.18514270861223,9.48130961825889));
#55954=CARTESIAN_POINT('Ctrl Pts',(4.4417700587056,-1.06847604194503,9.44939627659556));
#55955=CARTESIAN_POINT('Ctrl Pts',(4.42034758809898,-0.794772684000313,
9.38111247737266));
#55956=CARTESIAN_POINT('Ctrl Pts',(4.36277825954423,-0.636309800094768,
9.34422411328257));
#55957=CARTESIAN_POINT('Ctrl Pts',(4.31387722949841,-0.319434907276944,
9.28837259268112));
#55958=CARTESIAN_POINT('Ctrl Pts',(4.2774674602139,-0.158333333333226,9.26549350140391));
#55959=CARTESIAN_POINT('Ctrl Pts',(4.29133181086155,0.158333333333228,9.23645138949429));
#55960=CARTESIAN_POINT('Ctrl Pts',(4.34207293703372,0.319434907276952,9.22919622035688));
#55961=CARTESIAN_POINT('Ctrl Pts',(4.41826339299713,0.636309800094779,9.22811567796723));
#55962=CARTESIAN_POINT('Ctrl Pts',(4.490057534896,0.794772684000307,9.2339656388837));
#55963=CARTESIAN_POINT('Ctrl Pts',(4.5327322702054,1.06847604194576,9.26098446136783));
#55964=CARTESIAN_POINT('Ctrl Pts',(4.53913143621231,1.18514270861368,9.2776017498823));
#55965=CARTESIAN_POINT('Ctrl Pts',(4.53345745656538,1.30000000000311,9.29914087980385));
#55966=CARTESIAN_POINT('Ctrl Pts',(4.41373519238219,-1.30000000000076,9.51624950733163));
#55967=CARTESIAN_POINT('Ctrl Pts',(4.42460441374993,-1.18514270861205,9.4821579466063));
#55968=CARTESIAN_POINT('Ctrl Pts',(4.42484694140117,-1.06847604194486,9.45034196039577));
#55969=CARTESIAN_POINT('Ctrl Pts',(4.40085744044516,-0.794772684000194,
9.38209769983969));
#55970=CARTESIAN_POINT('Ctrl Pts',(4.34386504757947,-0.63630980009467,9.34478404741106));
#55971=CARTESIAN_POINT('Ctrl Pts',(4.29486459997575,-0.319434907276894,
9.28904431421725));
#55972=CARTESIAN_POINT('Ctrl Pts',(4.25911395670897,-0.158333333333201,
9.26661498524898));
#55973=CARTESIAN_POINT('Ctrl Pts',(4.27291141754749,0.158333333333204,9.23785393627474));
#55974=CARTESIAN_POINT('Ctrl Pts',(4.32289562721979,0.319434907276904,9.2305201364458));
#55975=CARTESIAN_POINT('Ctrl Pts',(4.39911219346208,0.636309800094681,9.2297168481906));
#55976=CARTESIAN_POINT('Ctrl Pts',(4.47031997754529,0.794772684000183,9.2361776056407));
#55977=CARTESIAN_POINT('Ctrl Pts',(4.51562250607443,1.06847604194559,9.26301592798594));
#55978=CARTESIAN_POINT('Ctrl Pts',(4.52384920305348,1.18514270861349,9.27936931824648));
#55979=CARTESIAN_POINT('Ctrl Pts',(4.52069281103532,1.30000000000291,9.30045878348211));
#55980=CARTESIAN_POINT('Ctrl Pts',(4.40732364295139,-1.30000000000072,9.5163476170774));
#55981=CARTESIAN_POINT('Ctrl Pts',(4.41688212528442,-1.185142708612,9.4825166004766));
#55982=CARTESIAN_POINT('Ctrl Pts',(4.41617619561562,-1.06847604194482,9.45085919745731));
#55983=CARTESIAN_POINT('Ctrl Pts',(4.3908325117472,-0.794772684000164,9.38274574564437));
#55984=CARTESIAN_POINT('Ctrl Pts',(4.33416209500732,-0.636309800094647,
9.34514478063228));
#55985=CARTESIAN_POINT('Ctrl Pts',(4.28517680049427,-0.319434907276883,
9.28922943073272));
#55986=CARTESIAN_POINT('Ctrl Pts',(4.24989006589237,-0.158333333333196,
9.26657728374074));
#55987=CARTESIAN_POINT('Ctrl Pts',(4.26364781909912,0.158333333333198,9.23798085352293));
#55988=CARTESIAN_POINT('Ctrl Pts',(4.31309155506437,0.319434907276893,9.23116227835363));
#55989=CARTESIAN_POINT('Ctrl Pts',(4.38928716252029,0.636309800094658,9.2306096286486));
#55990=CARTESIAN_POINT('Ctrl Pts',(4.46029277662821,0.794772684000154,9.23699316303097));
#55991=CARTESIAN_POINT('Ctrl Pts',(4.50693744924969,1.06847604194556,9.26375131247191));
#55992=CARTESIAN_POINT('Ctrl Pts',(4.5160820507918,1.18514270861345,9.28004256007604));
#55993=CARTESIAN_POINT('Ctrl Pts',(4.51418050345352,1.30000000000286,9.30104244387841));
#55994=CARTESIAN_POINT('Ctrl Pts',(4.40693494709678,-1.30000000000072,9.51635378924249));
#55995=CARTESIAN_POINT('Ctrl Pts',(4.41641424333561,-1.185142708612,9.48253774192878));
#55996=CARTESIAN_POINT('Ctrl Pts',(4.41565098622941,-1.06847604194483,9.45088943875991));
#55997=CARTESIAN_POINT('Ctrl Pts',(4.39022536238229,-0.794772684000165,
9.38278344984892));
#55998=CARTESIAN_POINT('Ctrl Pts',(4.33357424794786,-0.636309800094647,
9.34516565367199));
#55999=CARTESIAN_POINT('Ctrl Pts',(4.28458959106321,-0.319434907276883,
9.28924061795055));
#56000=CARTESIAN_POINT('Ctrl Pts',(4.24933053908302,-0.158333333333196,
9.26657659299652));
#56001=CARTESIAN_POINT('Ctrl Pts',(4.26308592317885,0.158333333333198,9.23798998978505));
#56002=CARTESIAN_POINT('Ctrl Pts',(4.31249752241387,0.319434907276893,9.23120031554562));
#56003=CARTESIAN_POINT('Ctrl Pts',(4.38869191352301,0.636309800094659,9.23066271091136));
#56004=CARTESIAN_POINT('Ctrl Pts',(4.45968470525621,0.794772684000155,9.23704377278317));
#56005=CARTESIAN_POINT('Ctrl Pts',(4.50641071191899,1.06847604194556,9.26379718946541));
#56006=CARTESIAN_POINT('Ctrl Pts',(4.51561104408737,1.18514270861345,9.28008433893661));
#56007=CARTESIAN_POINT('Ctrl Pts',(4.51378575150887,1.30000000000286,9.30107807510901));
#56008=CARTESIAN_POINT('Ctrl Pts',(4.40625511335241,-1.30000000000072,9.51636345978948));
#56009=CARTESIAN_POINT('Ctrl Pts',(4.41559577277618,-1.185142708612,9.48257376197577));
#56010=CARTESIAN_POINT('Ctrl Pts',(4.41473214646469,-1.06847604194482,9.45094150564397));
#56011=CARTESIAN_POINT('Ctrl Pts',(4.38916305550854,-0.794772684000165,
9.38284878692444));
#56012=CARTESIAN_POINT('Ctrl Pts',(4.33254567044107,-0.636309800094647,
9.34520178464511));
#56013=CARTESIAN_POINT('Ctrl Pts',(4.28356221756368,-0.319434907276883,
9.28925946376379));
#56014=CARTESIAN_POINT('Ctrl Pts',(4.24835188088717,-0.158333333333196,
9.26657361786353));
#56015=CARTESIAN_POINT('Ctrl Pts',(4.26210308617438,0.158333333333198,9.23800430500409));
#56016=CARTESIAN_POINT('Ctrl Pts',(4.3114581334876,0.319434907276893,9.2312663631012));
#56017=CARTESIAN_POINT('Ctrl Pts',(4.3876502593518,0.636309800094659,9.23075555468273));
#56018=CARTESIAN_POINT('Ctrl Pts',(4.45862071633395,0.794772684000154,9.23713186553507));
#56019=CARTESIAN_POINT('Ctrl Pts',(4.50548899771879,1.06847604194556,9.26387717733866));
#56020=CARTESIAN_POINT('Ctrl Pts',(4.51478681262742,1.18514270861345,9.28015730713193));
#56021=CARTESIAN_POINT('Ctrl Pts',(4.51309490007407,1.30000000000286,9.3011405122501));
#56022=CARTESIAN_POINT('Ctrl Pts',(4.40489630813951,-1.30000000000072,9.51637992315095));
#56023=CARTESIAN_POINT('Ctrl Pts',(4.4139602797652,-1.185142708612,9.48264089498604));
#56024=CARTESIAN_POINT('Ctrl Pts',(4.41289624599819,-1.06847604194483,9.45103956130732));
#56025=CARTESIAN_POINT('Ctrl Pts',(4.38704039657951,-0.794772684000165,
9.38297266059196));
#56026=CARTESIAN_POINT('Ctrl Pts',(4.33048964010808,-0.636309800094648,
9.34526993358207));
#56027=CARTESIAN_POINT('Ctrl Pts',(4.28150803914452,-0.319434907276883,
9.28929483673244));
#56028=CARTESIAN_POINT('Ctrl Pts',(4.24639473941324,-0.158333333333196,
9.26656675541383));
#56029=CARTESIAN_POINT('Ctrl Pts',(4.26013758794051,0.158333333333198,9.2380318952314));
#56030=CARTESIAN_POINT('Ctrl Pts',(4.30938034274635,0.319434907276893,9.23139432594687));
#56031=CARTESIAN_POINT('Ctrl Pts',(4.38556764694175,0.63630980009466,9.23093822745109));
#56032=CARTESIAN_POINT('Ctrl Pts',(4.45649207513945,0.794772684000156,9.23731024709754));
#56033=CARTESIAN_POINT('Ctrl Pts',(4.50364469895256,1.06847604194556,9.26404023102797));
#56034=CARTESIAN_POINT('Ctrl Pts',(4.51313763686427,1.18514270861345,9.2803057751366));
#56035=CARTESIAN_POINT('Ctrl Pts',(4.51171288901579,1.30000000000287,9.30126644375381));
#56036=CARTESIAN_POINT('Ctrl Pts',(4.40295803520288,-1.30000000000072,9.51639394221811));
#56037=CARTESIAN_POINT('Ctrl Pts',(4.41162876886495,-1.18514270861201,9.48272037623868));
#56038=CARTESIAN_POINT('Ctrl Pts',(4.41027958777538,-1.06847604194483,9.45115925064401));
#56039=CARTESIAN_POINT('Ctrl Pts',(4.38401470200241,-0.794772684000167,
9.38312689662002));
#56040=CARTESIAN_POINT('Ctrl Pts',(4.32755626093074,-0.636309800094648,
9.34535399900702));
#56041=CARTESIAN_POINT('Ctrl Pts',(4.27857540304651,-0.319434907276883,
9.28933824055801));
#56042=CARTESIAN_POINT('Ctrl Pts',(4.24359943941272,-0.158333333333196,
9.26655422181915));
#56043=CARTESIAN_POINT('Ctrl Pts',(4.257330269631,0.158333333333198,9.2380684615706));
#56044=CARTESIAN_POINT('Ctrl Pts',(4.30641513030752,0.319434907276894,9.2315648170422));
#56045=CARTESIAN_POINT('Ctrl Pts',(4.38259460579412,0.63630980009466,9.23119055161795));
#56046=CARTESIAN_POINT('Ctrl Pts',(4.45344909871239,0.794772684000156,9.23757258812502));
#56047=CARTESIAN_POINT('Ctrl Pts',(4.50100714780742,1.06847604194556,9.26428370184697));
#56048=CARTESIAN_POINT('Ctrl Pts',(4.51077922924535,1.18514270861345,9.2805268872598));
#56049=CARTESIAN_POINT('Ctrl Pts',(4.50973727486727,1.30000000000287,9.30145100669949));
#56050=CARTESIAN_POINT('Ctrl Pts',(4.40063620137717,-1.30000000000072,9.51639636097817));
#56051=CARTESIAN_POINT('Ctrl Pts',(4.40884040560399,-1.18514270861201,9.48278358005253));
#56052=CARTESIAN_POINT('Ctrl Pts',(4.40715216314469,-1.06847604194483,9.45126031194313));
#56053=CARTESIAN_POINT('Ctrl Pts',(4.38039845450992,-0.794772684000169,
9.38326244901355));
#56054=CARTESIAN_POINT('Ctrl Pts',(4.32404406839143,-0.63630980009465,9.3454270707552));
#56055=CARTESIAN_POINT('Ctrl Pts',(4.27505914465387,-0.319434907276884,
9.28937895677977));
#56056=CARTESIAN_POINT('Ctrl Pts',(4.24024360938201,-0.158333333333197,
9.26654337849712));
#56057=CARTESIAN_POINT('Ctrl Pts',(4.25396001813677,0.158333333333199,9.23811575818366));
#56058=CARTESIAN_POINT('Ctrl Pts',(4.30286294992823,0.319434907276894,9.2317445901503));
#56059=CARTESIAN_POINT('Ctrl Pts',(4.37903153532005,0.636309800094662,9.23147471197206));
#56060=CARTESIAN_POINT('Ctrl Pts',(4.44979163239843,0.794772684000159,9.23790935230491));
#56061=CARTESIAN_POINT('Ctrl Pts',(4.49783488694176,1.06847604194556,9.2646031551418));
#56062=CARTESIAN_POINT('Ctrl Pts',(4.50794326995182,1.18514270861346,9.28081450128029));
#56063=CARTESIAN_POINT('Ctrl Pts',(4.50736389125802,1.30000000000287,9.30168243541202));
#56064=CARTESIAN_POINT('Ctrl Pts',(4.39600056929137,-1.30000000000072,9.51637194624509));
#56065=CARTESIAN_POINT('Ctrl Pts',(4.4032848721401,-1.18514270861201,9.48283732300393));
#56066=CARTESIAN_POINT('Ctrl Pts',(4.40092622520048,-1.06847604194483,9.45136419869777));
#56067=CARTESIAN_POINT('Ctrl Pts',(4.37320013584774,-0.79477268400017,9.3834174603151));
#56068=CARTESIAN_POINT('Ctrl Pts',(4.31703826235303,-0.636309800094651,
9.34550726188743));
#56069=CARTESIAN_POINT('Ctrl Pts',(4.2680325520994,-0.319434907276885,9.28943663898676));
#56070=CARTESIAN_POINT('Ctrl Pts',(4.23352528126376,-0.158333333333197,
9.26654268431001));
#56071=CARTESIAN_POINT('Ctrl Pts',(4.24721267322164,0.158333333333199,9.23823022692339));
#56072=CARTESIAN_POINT('Ctrl Pts',(4.29577139823858,0.319434907276895,9.23205090857317));
#56073=CARTESIAN_POINT('Ctrl Pts',(4.37191577184974,0.636309800094663,9.23200082102078));
#56074=CARTESIAN_POINT('Ctrl Pts',(4.4424629594934,0.79477268400016,9.23863489727255));
#56075=CARTESIAN_POINT('Ctrl Pts',(4.49147316778346,1.06847604194556,9.26530786724832));
#56076=CARTESIAN_POINT('Ctrl Pts',(4.50225681955632,1.18514270861346,9.28144515444429));
#56077=CARTESIAN_POINT('Ctrl Pts',(4.50260941994036,1.30000000000287,9.30217398846459));
#56078=CARTESIAN_POINT('Ctrl Pts',(4.39061441318341,-1.30000000000076,9.51626458451879));
#56079=CARTESIAN_POINT('Ctrl Pts',(4.3968636067614,-1.18514270861204,9.48269776371229));
#56080=CARTESIAN_POINT('Ctrl Pts',(4.39374548939964,-1.06847604194486,9.45121006362946));
#56081=CARTESIAN_POINT('Ctrl Pts',(4.36490165232186,-0.794772684000192,
9.38327036214381));
#56082=CARTESIAN_POINT('Ctrl Pts',(4.30892116882036,-0.636309800094669,
9.34541395146925));
#56083=CARTESIAN_POINT('Ctrl Pts',(4.25985708215244,-0.319434907276894,
9.28943161594754));
#56084=CARTESIAN_POINT('Ctrl Pts',(4.22567540968377,-0.158333333333201,
9.26658863881072));
#56085=CARTESIAN_POINT('Ctrl Pts',(4.23932815218653,0.158333333333203,9.23840732600793));
#56086=CARTESIAN_POINT('Ctrl Pts',(4.28753888340787,0.319434907276904,9.23225185888506));
#56087=CARTESIAN_POINT('Ctrl Pts',(4.36364609441846,0.636309800094681,9.23249532729164));
#56088=CARTESIAN_POINT('Ctrl Pts',(4.43387415143865,0.794772684000182,9.23963750981833));
#56089=CARTESIAN_POINT('Ctrl Pts',(4.48400376887349,1.06847604194559,9.26631847888963));
#56090=CARTESIAN_POINT('Ctrl Pts',(4.49558416661022,1.18514270861349,9.28233330857485));
#56091=CARTESIAN_POINT('Ctrl Pts',(4.4970457081814,1.30000000000291,9.3028137650616));
#56092=CARTESIAN_POINT('Ctrl Pts',(4.38138051521408,-1.30000000000076,9.51606529202356));
#56093=CARTESIAN_POINT('Ctrl Pts',(4.3858740921445,-1.18514270861204,9.48237596358173));
#56094=CARTESIAN_POINT('Ctrl Pts',(4.38146750644091,-1.06847604194486,9.45081488014051));
#56095=CARTESIAN_POINT('Ctrl Pts',(4.35072625577525,-0.794772684000191,
9.38281913532378));
#56096=CARTESIAN_POINT('Ctrl Pts',(4.29505520611644,-0.636309800094668,
9.3450577261607));
#56097=CARTESIAN_POINT('Ctrl Pts',(4.24588137556484,-0.319434907276893,
9.28926085579798));
#56098=CARTESIAN_POINT('Ctrl Pts',(4.21223423013499,-0.158333333333201,
9.26659537988078));
#56099=CARTESIAN_POINT('Ctrl Pts',(4.22582062844705,0.158333333333203,9.23865691599574));
#56100=CARTESIAN_POINT('Ctrl Pts',(4.27344941401814,0.319434907276903,9.23247303789332));
#56101=CARTESIAN_POINT('Ctrl Pts',(4.3494926805306,0.636309800094679,9.23321668657625));
#56102=CARTESIAN_POINT('Ctrl Pts',(4.41916887909758,0.79477268400018,9.24125576604867));
#56103=CARTESIAN_POINT('Ctrl Pts',(4.4712039151015,1.06847604194559,9.26800796128312));
#56104=CARTESIAN_POINT('Ctrl Pts',(4.48414225235254,1.18514270861349,9.2838457080482));
#56105=CARTESIAN_POINT('Ctrl Pts',(4.48749488785651,1.30000000000291,9.30394116752782));
#56106=CARTESIAN_POINT('Ctrl Pts',(4.36900022363105,-1.30000000000082,9.5160307765818));
#56107=CARTESIAN_POINT('Ctrl Pts',(4.37103552052153,-1.1851427086121,9.48255553524329));
#56108=CARTESIAN_POINT('Ctrl Pts',(4.36484769496369,-1.06847604194491,9.45109997584673));
#56109=CARTESIAN_POINT('Ctrl Pts',(4.3315555221693,-0.794772684000226,9.38309721029964));
#56110=CARTESIAN_POINT('Ctrl Pts',(4.27646882106592,-0.636309800094698,
9.3449197704111));
#56111=CARTESIAN_POINT('Ctrl Pts',(4.22731242869909,-0.319434907276909,
9.28882624102019));
#56112=CARTESIAN_POINT('Ctrl Pts',(4.19454828163421,-0.158333333333209,
9.26580707041848));
#56113=CARTESIAN_POINT('Ctrl Pts',(4.20804004063657,0.158333333333211,9.23821287817429));
#56114=CARTESIAN_POINT('Ctrl Pts',(4.25463605943907,0.319434907276918,9.23289355404711));
#56115=CARTESIAN_POINT('Ctrl Pts',(4.33058140830202,0.63630980009471,9.23429579125412));
#56116=CARTESIAN_POINT('Ctrl Pts',(4.39976178926623,0.794772684000219,9.24257867334419));
#56117=CARTESIAN_POINT('Ctrl Pts',(4.45436072170246,1.06847604194564,9.26934382114282));
#56118=CARTESIAN_POINT('Ctrl Pts',(4.46907953701949,1.18514270861355,9.28507758450468));
#56119=CARTESIAN_POINT('Ctrl Pts',(4.47488331289161,1.30000000000297,9.30495947049279));
#56120=CARTESIAN_POINT('Ctrl Pts',(4.35192791261779,-1.30000000000091,9.51610713954233));
#56121=CARTESIAN_POINT('Ctrl Pts',(4.35054611088779,-1.18514270861218,9.48303106026128));
#56122=CARTESIAN_POINT('Ctrl Pts',(4.3418827947019,-1.06847604194499,9.45179530857522));
#56123=CARTESIAN_POINT('Ctrl Pts',(4.30504704616706,-0.794772684000287,
9.38388599839058));
#56124=CARTESIAN_POINT('Ctrl Pts',(4.25076713902507,-0.636309800094743,
9.34512876400693));
#56125=CARTESIAN_POINT('Ctrl Pts',(4.20165589012478,-0.31943490727693,9.2885679982112));
#56126=CARTESIAN_POINT('Ctrl Pts',(4.17013613981169,-0.15833333333322,9.26498708049703));
#56127=CARTESIAN_POINT('Ctrl Pts',(4.18355074309137,0.158333333333222,9.23769387423214));
#56128=CARTESIAN_POINT('Ctrl Pts',(4.22879523333919,0.319434907276941,9.23330848676313));
#56129=CARTESIAN_POINT('Ctrl Pts',(4.30459933720093,0.636309800094755,9.23564601060515));
#56130=CARTESIAN_POINT('Ctrl Pts',(4.37300885395577,0.794772684000274,9.2445977591603));
#56131=CARTESIAN_POINT('Ctrl Pts',(4.43108597948329,1.06847604194572,9.27154766519164));
#56132=CARTESIAN_POINT('Ctrl Pts',(4.4482401057954,1.18514270861363,9.28717976384003));
#56133=CARTESIAN_POINT('Ctrl Pts',(4.45740892274821,1.30000000000306,9.30677834540822));
#56134=CARTESIAN_POINT('Ctrl Pts',(4.32733788924607,-1.30000000000102,9.51541096929758));
#56135=CARTESIAN_POINT('Ctrl Pts',(4.32121146294237,-1.18514270861228,9.48217278909515));
#56136=CARTESIAN_POINT('Ctrl Pts',(4.30910080586344,-1.06847604194508,9.45075308655846));
#56137=CARTESIAN_POINT('Ctrl Pts',(4.26729799505055,-0.794772684000351,
9.38236833540205));
#56138=CARTESIAN_POINT('Ctrl Pts',(4.21413587457917,-0.636309800094796,
9.34297025808628));
#56139=CARTESIAN_POINT('Ctrl Pts',(4.1648852499766,-0.319434907276958,9.28638795906878));
#56140=CARTESIAN_POINT('Ctrl Pts',(4.13484613211291,-0.158333333333233,
9.26304383309945));
#56141=CARTESIAN_POINT('Ctrl Pts',(4.14792251264182,0.158333333333235,9.23688755391369));
#56142=CARTESIAN_POINT('Ctrl Pts',(4.19114634054308,0.319434907276968,9.23402788190919));
#56143=CARTESIAN_POINT('Ctrl Pts',(4.26681195134328,0.636309800094809,9.23742851588972));
#56144=CARTESIAN_POINT('Ctrl Pts',(4.33436034864448,0.794772684000341,9.2463596608503));
#56145=CARTESIAN_POINT('Ctrl Pts',(4.39760093960311,1.06847604194581,9.27326308511272));
#56146=CARTESIAN_POINT('Ctrl Pts',(4.4183083085949,1.18514270861373,9.2887637381985));
#56147=CARTESIAN_POINT('Ctrl Pts',(4.43234853804718,1.30000000000317,9.30811954887692));
#56148=CARTESIAN_POINT('Ctrl Pts',(4.30273880285957,-1.30000000000114,9.51468456739312));
#56149=CARTESIAN_POINT('Ctrl Pts',(4.29187060135338,-1.18514270861239,9.48126859996238));
#56150=CARTESIAN_POINT('Ctrl Pts',(4.27627765814262,-1.06847604194517,9.44976536215955));
#56151=CARTESIAN_POINT('Ctrl Pts',(4.22933974144936,-0.794772684000421,
9.38140536871477));
#56152=CARTESIAN_POINT('Ctrl Pts',(4.17691683537209,-0.636309800094852,
9.34251697935878));
#56153=CARTESIAN_POINT('Ctrl Pts',(4.12751372739255,-0.319434907276985,
9.28594210505695));
#56154=CARTESIAN_POINT('Ctrl Pts',(4.09917775569068,-0.158333333333247,
9.26219277655249));
#56155=CARTESIAN_POINT('Ctrl Pts',(4.11230177225596,0.158333333333249,9.23590136321851));
#56156=CARTESIAN_POINT('Ctrl Pts',(4.1540238940554,0.319434907276995,9.23276786236089));
#56157=CARTESIAN_POINT('Ctrl Pts',(4.22962573168682,0.636309800094862,9.23699369261186));
#56158=CARTESIAN_POINT('Ctrl Pts',(4.29580778766756,0.794772684000408,9.24765378099704));
#56159=CARTESIAN_POINT('Ctrl Pts',(4.36402625703275,1.0684760419459,9.27517340626912));
#56160=CARTESIAN_POINT('Ctrl Pts',(4.388256376591,1.18514270861384,9.29065921387979));
#56161=CARTESIAN_POINT('Ctrl Pts',(4.40718736806254,1.30000000000329,9.30971860302339));
#56162=CARTESIAN_POINT('Ctrl Pts',(4.28117479265866,-1.30000000000118,9.51412312894823));
#56163=CARTESIAN_POINT('Ctrl Pts',(4.26607290792941,-1.18514270861243,9.48076524600039));
#56164=CARTESIAN_POINT('Ctrl Pts',(4.24745842260437,-1.0684760419452,9.44908372835292));
#56165=CARTESIAN_POINT('Ctrl Pts',(4.19634042761899,-0.794772684000445,
9.37976582392113));
#56166=CARTESIAN_POINT('Ctrl Pts',(4.14539567067865,-0.636309800094874,
9.33884536284604));
#56167=CARTESIAN_POINT('Ctrl Pts',(4.09603748520983,-0.319434907276998,
9.28173674872678));
#56168=CARTESIAN_POINT('Ctrl Pts',(4.06882109985603,-0.158333333333252,
9.25872525037652));
#56169=CARTESIAN_POINT('Ctrl Pts',(4.08153941272377,0.158333333333254,9.23368959813871));
#56170=CARTESIAN_POINT('Ctrl Pts',(4.12148988815201,0.319434907277006,9.23175370316326));
#56171=CARTESIAN_POINT('Ctrl Pts',(4.19672222414941,0.636309800094885,9.23768671925175));
#56172=CARTESIAN_POINT('Ctrl Pts',(4.26176605935896,0.794772684000438,9.24968928688449));
#56173=CARTESIAN_POINT('Ctrl Pts',(4.33438372448306,1.06847604194594,9.27762359043197));
#56174=CARTESIAN_POINT('Ctrl Pts',(4.36174457272238,1.18514270861388,9.29295079370866));
#56175=CARTESIAN_POINT('Ctrl Pts',(4.38503277271829,1.30000000000333,9.31151347532423));
#56176=CARTESIAN_POINT('Ctrl Pts',(4.27051303598667,-1.3000000000012,9.51346869990321));
#56177=CARTESIAN_POINT('Ctrl Pts',(4.25344088139478,-1.18514270861245,9.4797098983446));
#56178=CARTESIAN_POINT('Ctrl Pts',(4.23336359696833,-1.06847604194522,9.44780039991522));
#56179=CARTESIAN_POINT('Ctrl Pts',(4.18003860240438,-0.79477268400046,9.3783553352506));
#56180=CARTESIAN_POINT('Ctrl Pts',(4.12924913693472,-0.636309800094885,
9.33814873258178));
#56181=CARTESIAN_POINT('Ctrl Pts',(4.07980211357947,-0.319434907277003,
9.28110399012567));
#56182=CARTESIAN_POINT('Ctrl Pts',(4.05341076727602,-0.158333333333255,
9.25769362498906));
#56183=CARTESIAN_POINT('Ctrl Pts',(4.0661756651677,0.158333333333257,9.23250840130699));
#56184=CARTESIAN_POINT('Ctrl Pts',(4.10543111529468,0.319434907277012,9.23055773383978));
#56185=CARTESIAN_POINT('Ctrl Pts',(4.18067724121201,0.636309800094896,9.23666009916673));
#56186=CARTESIAN_POINT('Ctrl Pts',(4.24524187540873,0.794772684000452,9.24893194569463));
#56187=CARTESIAN_POINT('Ctrl Pts',(4.32002843361178,1.06847604194596,9.27718049743058));
#56188=CARTESIAN_POINT('Ctrl Pts',(4.34889750809698,1.1851427086139,9.29264391254179));
#56189=CARTESIAN_POINT('Ctrl Pts',(4.37426332713616,1.30000000000335,9.31134299142965));
#56190=CARTESIAN_POINT('Ctrl Pts',(4.26513816686888,-1.30000000000121,9.51325891814912));
#56191=CARTESIAN_POINT('Ctrl Pts',(4.24707151218177,-1.18514270861245,9.47932840796016));
#56192=CARTESIAN_POINT('Ctrl Pts',(4.22626625202657,-1.06847604194523,9.44729494305863));
#56193=CARTESIAN_POINT('Ctrl Pts',(4.17187521250272,-0.794772684000461,
9.37767378498013));
#56194=CARTESIAN_POINT('Ctrl Pts',(4.12125301165255,-0.636309800094886,
9.33755155961958));
#56195=CARTESIAN_POINT('Ctrl Pts',(4.07179835604984,-0.319434907277004,
9.28043168037745));
#56196=CARTESIAN_POINT('Ctrl Pts',(4.04582179527502,-0.158333333333255,
9.25681962487196));
#56197=CARTESIAN_POINT('Ctrl Pts',(4.05854114942379,0.158333333333257,9.2317767541839));
#56198=CARTESIAN_POINT('Ctrl Pts',(4.09731949157577,0.319434907277012,9.23021766431748));
#56199=CARTESIAN_POINT('Ctrl Pts',(4.17251465742636,0.636309800094897,9.23658830540946));
#56200=CARTESIAN_POINT('Ctrl Pts',(4.23690164518344,0.794772684000453,9.24881082069698));
#56201=CARTESIAN_POINT('Ctrl Pts',(4.31276279944828,1.06847604194596,9.27725003928142));
#56202=CARTESIAN_POINT('Ctrl Pts',(4.34237324230651,1.1851427086139,9.29282104199691));
#56203=CARTESIAN_POINT('Ctrl Pts',(4.3687566452743,1.30000000000336,9.31165276347954));
#56204=CARTESIAN_POINT('Ctrl Pts',(4.26245981977714,-1.30000000000121,9.51312991696811));
#56205=CARTESIAN_POINT('Ctrl Pts',(4.24389098837022,-1.18514270861245,9.47912613808092));
#56206=CARTESIAN_POINT('Ctrl Pts',(4.22271888801939,-1.06847604194523,9.4470378528054));
#56207=CARTESIAN_POINT('Ctrl Pts',(4.16779302870235,-0.794772684000462,
9.37733266801583));
#56208=CARTESIAN_POINT('Ctrl Pts',(4.11726184280991,-0.636309800094887,
9.33723297019308));
#56209=CARTESIAN_POINT('Ctrl Pts',(4.06780584876013,-0.319434907277004,
9.28006824332014));
#56210=CARTESIAN_POINT('Ctrl Pts',(4.04203758847583,-0.158333333333256,
9.25635174774498));
#56211=CARTESIAN_POINT('Ctrl Pts',(4.05473007673294,0.158333333333258,9.23139149387313));
#56212=CARTESIAN_POINT('Ctrl Pts',(4.09326328303475,0.319434907277013,9.23004610934002));
#56213=CARTESIAN_POINT('Ctrl Pts',(4.16842537053399,0.636309800094898,9.23657560160018));
#56214=CARTESIAN_POINT('Ctrl Pts',(4.23271443442531,0.794772684000455,9.24880740652821));
#56215=CARTESIAN_POINT('Ctrl Pts',(4.30911750776002,1.06847604194596,9.27732764435698));
#56216=CARTESIAN_POINT('Ctrl Pts',(4.3391041711311,1.1851427086139,9.29293405573285));
#56217=CARTESIAN_POINT('Ctrl Pts',(4.36600543843937,1.30000000000336,9.31180152430741));
#56218=CARTESIAN_POINT('Ctrl Pts',(4.26112167304248,-1.30000000000121,9.51306293852468));
#56219=CARTESIAN_POINT('Ctrl Pts',(4.24229982152744,-1.18514270861245,9.47902777087902));
#56220=CARTESIAN_POINT('Ctrl Pts',(4.22094355162894,-1.06847604194523,9.44691397418521));
#56221=CARTESIAN_POINT('Ctrl Pts',(4.16575128238195,-0.794772684000462,
9.37716343074742));
#56222=CARTESIAN_POINT('Ctrl Pts',(4.11527210765485,-0.636309800094887,
9.33705607537697));
#56223=CARTESIAN_POINT('Ctrl Pts',(4.06581685723877,-0.319434907277004,
9.27986478205432));
#56224=CARTESIAN_POINT('Ctrl Pts',(4.04015061657582,-0.158333333333255,
9.2561022147184));
#56225=CARTESIAN_POINT('Ctrl Pts',(4.05282623100244,0.158333333333258,9.23119371657798));
#56226=CARTESIAN_POINT('Ctrl Pts',(4.09123284757633,0.319434907277012,9.22996738025275));
#56227=CARTESIAN_POINT('Ctrl Pts',(4.16637549742435,0.636309800094898,9.23658563659111));
#56228=CARTESIAN_POINT('Ctrl Pts',(4.23061539482181,0.794772684000454,9.24882385034909));
#56229=CARTESIAN_POINT('Ctrl Pts',(4.30729007606217,1.06847604194596,9.27738261100104));
#56230=CARTESIAN_POINT('Ctrl Pts',(4.33746559938657,1.1851427086139,9.29300416345298));
#56231=CARTESIAN_POINT('Ctrl Pts',(4.36462701760318,1.30000000000336,9.31188523907697));
#56232=CARTESIAN_POINT('Ctrl Pts',(4.26035799968545,-1.30000000000121,9.51302203515777));
#56233=CARTESIAN_POINT('Ctrl Pts',(4.24139110836822,-1.18514270861245,9.4789700338413));
#56234=CARTESIAN_POINT('Ctrl Pts',(4.21992935678055,-1.06847604194523,9.44684220684509));
#56235=CARTESIAN_POINT('Ctrl Pts',(4.16458479088466,-0.794772684000462,
9.37706572694382));
#56236=CARTESIAN_POINT('Ctrl Pts',(4.11413635908148,-0.636309800094887,
9.33695116082272));
#56237=CARTESIAN_POINT('Ctrl Pts',(4.064681560807,-0.319434907277004,9.27974460162218));
#56238=CARTESIAN_POINT('Ctrl Pts',(4.0390729692768,-0.158333333333255,9.25595759594241));
#56239=CARTESIAN_POINT('Ctrl Pts',(4.05173850640223,0.158333333333258,9.23107985921052));
#56240=CARTESIAN_POINT('Ctrl Pts',(4.09007277335858,0.319434907277012,9.22992136116913));
#56241=CARTESIAN_POINT('Ctrl Pts',(4.16520386142014,0.636309800094898,9.23659179838107));
#56242=CARTESIAN_POINT('Ctrl Pts',(4.22941469577267,0.794772684000454,9.2488370629054));
#56243=CARTESIAN_POINT('Ctrl Pts',(4.30624506240245,1.06847604194596,9.27741642908466));
#56244=CARTESIAN_POINT('Ctrl Pts',(4.33652905264565,1.1851427086139,9.29304491214065));
#56245=CARTESIAN_POINT('Ctrl Pts',(4.36384001426349,1.30000000000336,9.31193092960344));
#56246=CARTESIAN_POINT('Ctrl Pts',(4.25386871221725,-1.30000000000122,9.5126707048174));
#56247=CARTESIAN_POINT('Ctrl Pts',(4.23366468109142,-1.18514270861246,9.47848859867081));
#56248=CARTESIAN_POINT('Ctrl Pts',(4.21130410672917,-1.06847604194523,9.44624842090527));
#56249=CARTESIAN_POINT('Ctrl Pts',(4.15466466044384,-0.794772684000465,
9.37625340368326));
#56250=CARTESIAN_POINT('Ctrl Pts',(4.10448617408231,-0.636309800094891,
9.33605325953235));
#56251=CARTESIAN_POINT('Ctrl Pts',(4.05503843749056,-0.319434907277006,
9.27870748019983));
#56252=CARTESIAN_POINT('Ctrl Pts',(4.02991987648068,-0.158333333333256,
9.25471095276929));
#56253=CARTESIAN_POINT('Ctrl Pts',(4.0424964711577,0.158333333333258,9.23010493361964));
#56254=CARTESIAN_POINT('Ctrl Pts',(4.08020951067749,0.319434907277014,9.22954365534675));
#56255=CARTESIAN_POINT('Ctrl Pts',(4.15523843700153,0.636309800094901,9.23667053804519));
#56256=CARTESIAN_POINT('Ctrl Pts',(4.21920311517671,0.794772684000459,9.24897446745093));
#56257=CARTESIAN_POINT('Ctrl Pts',(4.29735601881323,1.06847604194597,9.27772965857063));
#56258=CARTESIAN_POINT('Ctrl Pts',(4.32856167605119,1.18514270861391,9.2934164645392));
#56259=CARTESIAN_POINT('Ctrl Pts',(4.35714349439314,1.30000000000336,9.3123430197254));
#56260=CARTESIAN_POINT('Ctrl Pts',(4.24178124330891,-1.3000000000013,9.51117036285141));
#56261=CARTESIAN_POINT('Ctrl Pts',(4.21909655253804,-1.18514270861253,9.47704359218079));
#56262=CARTESIAN_POINT('Ctrl Pts',(4.19496119016866,-1.0684760419453,9.44473352233143));
#56263=CARTESIAN_POINT('Ctrl Pts',(4.13585233323443,-0.794772684000518,
9.37428773969915));
#56264=CARTESIAN_POINT('Ctrl Pts',(4.08651822363923,-0.63630980009493,9.33301961812018));
#56265=CARTESIAN_POINT('Ctrl Pts',(4.03705041811503,-0.319434907277025,
9.27550054041365));
#56266=CARTESIAN_POINT('Ctrl Pts',(4.012560323088,-0.158333333333266,9.25196927902043));
#56267=CARTESIAN_POINT('Ctrl Pts',(4.02483699477286,0.158333333333268,9.2282262725902));
#56268=CARTESIAN_POINT('Ctrl Pts',(4.06145877578896,0.319434907277035,9.22848581931836));
#56269=CARTESIAN_POINT('Ctrl Pts',(4.13622860300854,0.636309800094941,9.23668211508822));
#56270=CARTESIAN_POINT('Ctrl Pts',(4.19949354935448,0.794772684000507,9.24987010723203));
#56271=CARTESIAN_POINT('Ctrl Pts',(4.28028599443832,1.06847604194603,9.27860275469367));
#56272=CARTESIAN_POINT('Ctrl Pts',(4.31337706345077,1.18514270861398,9.29399745869907));
#56273=CARTESIAN_POINT('Ctrl Pts',(4.34458714565379,1.30000000000345,9.31234956827316));
#56274=CARTESIAN_POINT('Ctrl Pts',(4.22320612684256,-1.30000000000134,9.51079938881643));
#56275=CARTESIAN_POINT('Ctrl Pts',(4.19704373245862,-1.18514270861257,9.47626373784351));
#56276=CARTESIAN_POINT('Ctrl Pts',(4.17038815369448,-1.06847604194534,9.44359119137219));
#56277=CARTESIAN_POINT('Ctrl Pts',(4.10766907973974,-0.794772684000543,
9.37241521701459));
#56278=CARTESIAN_POINT('Ctrl Pts',(4.0591594781697,-0.636309800094952,9.33075549355686));
#56279=CARTESIAN_POINT('Ctrl Pts',(4.00971417153467,-0.319434907277036,
9.27284812988568));
#56280=CARTESIAN_POINT('Ctrl Pts',(3.98640076421902,-0.158333333333271,
9.24934159322923));
#56281=CARTESIAN_POINT('Ctrl Pts',(3.99868569747104,0.158333333333273,9.22555001433102));
#56282=CARTESIAN_POINT('Ctrl Pts',(4.03419060433982,0.319434907277044,9.22553226129214));
#56283=CARTESIAN_POINT('Ctrl Pts',(4.1088497531818,0.636309800094962,9.23443344293737));
#56284=CARTESIAN_POINT('Ctrl Pts',(4.1711027666005,0.794772684000536,9.24868382172846));
#56285=CARTESIAN_POINT('Ctrl Pts',(4.25538439556395,1.06847604194607,9.27869255642126));
#56286=CARTESIAN_POINT('Ctrl Pts',(4.29096174293842,1.18514270861402,9.29464472144887));
#56287=CARTESIAN_POINT('Ctrl Pts',(4.32563404345099,1.30000000000348,9.31355938218873));
#56288=CARTESIAN_POINT('Ctrl Pts',(4.2054458088272,-1.30000000000139,9.50826165136687));
#56289=CARTESIAN_POINT('Ctrl Pts',(4.17587338761788,-1.18514270861262,9.47309275299579));
#56290=CARTESIAN_POINT('Ctrl Pts',(4.14671963387226,-1.06847604194538,9.43996758529192));
#56291=CARTESIAN_POINT('Ctrl Pts',(4.08033583612687,-0.794772684000577,
9.36816324791727));
#56292=CARTESIAN_POINT('Ctrl Pts',(4.03239495345726,-0.636309800094979,
9.32680868495316));
#56293=CARTESIAN_POINT('Ctrl Pts',(3.98289150201526,-0.31943490727705,9.26872905500331));
#56294=CARTESIAN_POINT('Ctrl Pts',(3.96095814577377,-0.158333333333278,
9.24469994491065));
#56295=CARTESIAN_POINT('Ctrl Pts',(3.97306681687221,0.15833333333328,9.22138423758945));
#56296=CARTESIAN_POINT('Ctrl Pts',(4.00701746190735,0.319434907277058,9.22231997097444));
#56297=CARTESIAN_POINT('Ctrl Pts',(4.08137154369871,0.63630980009499,9.23245431244624));
#56298=CARTESIAN_POINT('Ctrl Pts',(4.1426660014168,0.794772684000571,9.24761943765885));
#56299=CARTESIAN_POINT('Ctrl Pts',(4.23063602231676,1.06847604194612,9.27826577639269));
#56300=CARTESIAN_POINT('Ctrl Pts',(4.26883860452601,1.18514270861407,9.29433484784612));
#56301=CARTESIAN_POINT('Ctrl Pts',(4.3071648065072,1.30000000000354,9.31320732627382));
#56302=CARTESIAN_POINT('Ctrl Pts',(4.18686936798153,-1.30000000000144,9.50784799049483));
#56303=CARTESIAN_POINT('Ctrl Pts',(4.1537455453232,-1.18514270861266,9.47244915742316));
#56304=CARTESIAN_POINT('Ctrl Pts',(4.12205853653029,-1.06847604194542,9.43898252789801));
#56305=CARTESIAN_POINT('Ctrl Pts',(4.0521745347172,-0.794772684000604,9.36613169544727));
#56306=CARTESIAN_POINT('Ctrl Pts',(4.00540931861376,-0.636309800095,9.32344327305321));
#56307=CARTESIAN_POINT('Ctrl Pts',(3.95609732960451,-0.319434907277061,
9.26452386114696));
#56308=CARTESIAN_POINT('Ctrl Pts',(3.9353800935742,-0.158333333333284,9.24041782432346));
#56309=CARTESIAN_POINT('Ctrl Pts',(3.94730070634834,0.158333333333286,9.21760153467538));
#56310=CARTESIAN_POINT('Ctrl Pts',(3.97972332532001,0.319434907277068,9.21939301129695));
#56311=CARTESIAN_POINT('Ctrl Pts',(4.05375515190992,0.63630980009501,9.23081529726131));
#56312=CARTESIAN_POINT('Ctrl Pts',(4.11404925717502,0.794772684000596,9.24703854429435));
#56313=CARTESIAN_POINT('Ctrl Pts',(4.2056799580573,1.06847604194615,9.27843300161521));
#56314=CARTESIAN_POINT('Ctrl Pts',(4.24649949110921,1.18514270861411,9.29465790225651));
#56315=CARTESIAN_POINT('Ctrl Pts',(4.28847502205294,1.30000000000358,9.31351820624413));
#56316=CARTESIAN_POINT('Ctrl Pts',(4.16917315736043,-1.30000000000149,9.5051037777749));
#56317=CARTESIAN_POINT('Ctrl Pts',(4.13281824485764,-1.1851427086127,9.46859744828135));
#56318=CARTESIAN_POINT('Ctrl Pts',(4.09875074033596,-1.06847604194545,9.43436481465258));
#56319=CARTESIAN_POINT('Ctrl Pts',(4.02533235974092,-0.794772684000632,
9.36053327505436));
#56320=CARTESIAN_POINT('Ctrl Pts',(3.97904689603395,-0.636309800095023,
9.31837014559696));
#56321=CARTESIAN_POINT('Ctrl Pts',(3.92952225134954,-0.319434907277072,
9.25968834249974));
#56322=CARTESIAN_POINT('Ctrl Pts',(3.90987087920662,-0.158333333333289,
9.23593319703193));
#56323=CARTESIAN_POINT('Ctrl Pts',(3.92167555233481,0.158333333333291,9.21338919330623));
#56324=CARTESIAN_POINT('Ctrl Pts',(3.95296650613317,0.319434907277081,9.21493431476278));
#56325=CARTESIAN_POINT('Ctrl Pts',(4.02687269945799,0.636309800095034,9.22701531286196));
#56326=CARTESIAN_POINT('Ctrl Pts',(4.0862629071067,0.794772684000624,9.24384636807182));
#56327=CARTESIAN_POINT('Ctrl Pts',(4.18128339050235,1.06847604194619,9.2767867802146));
#56328=CARTESIAN_POINT('Ctrl Pts',(4.22450478135387,1.18514270861415,9.29383823078633));
#56329=CARTESIAN_POINT('Ctrl Pts',(4.26981671665059,1.30000000000363,9.31368244807567));
#56330=CARTESIAN_POINT('Ctrl Pts',(4.15072826470058,-1.30000000000153,9.50428049865681));
#56331=CARTESIAN_POINT('Ctrl Pts',(4.11092006387152,-1.18514270861274,9.4672585114039));
#56332=CARTESIAN_POINT('Ctrl Pts',(4.07439573712881,-1.06847604194549,9.43247028158174));
#56333=CARTESIAN_POINT('Ctrl Pts',(3.99760364176302,-0.794772684000661,
9.35726293785791));
#56334=CARTESIAN_POINT('Ctrl Pts',(3.95249877951535,-0.636309800095045,
9.31381998566838));
#56335=CARTESIAN_POINT('Ctrl Pts',(3.90321841546551,-0.319434907277083,
9.25418271625328));
#56336=CARTESIAN_POINT('Ctrl Pts',(3.88484358864865,-0.158333333333294,
9.23019185009763));
#56337=CARTESIAN_POINT('Ctrl Pts',(3.89640048618951,0.158333333333296,9.20826547681166));
#56338=CARTESIAN_POINT('Ctrl Pts',(3.92606467876695,0.31943490727709,9.21084090843296));
#56339=CARTESIAN_POINT('Ctrl Pts',(3.99943055395677,0.636309800095054,9.22477498876752));
#56340=CARTESIAN_POINT('Ctrl Pts',(4.05750970766444,0.794772684000651,9.24358249041576));
#56341=CARTESIAN_POINT('Ctrl Pts',(4.15618511747296,1.06847604194623,9.2772753226398));
#56342=CARTESIAN_POINT('Ctrl Pts',(4.2021015888093,1.1851427086142,9.29425122806245));
#56343=CARTESIAN_POINT('Ctrl Pts',(4.2512216028599,1.30000000000368,9.31361866028035));
#56344=CARTESIAN_POINT('Ctrl Pts',(4.13311774283548,-1.30000000000156,9.50129808886456));
#56345=CARTESIAN_POINT('Ctrl Pts',(4.09001770799959,-1.18514270861277,9.463322669032));
#56346=CARTESIAN_POINT('Ctrl Pts',(4.05109040073584,-1.06847604194552,9.4278236837884));
#56347=CARTESIAN_POINT('Ctrl Pts',(3.97080036901856,-0.794772684000679,
9.35153498563776));
#56348=CARTESIAN_POINT('Ctrl Pts',(3.92636363324339,-0.636309800095061,
9.3081280151374));
#56349=CARTESIAN_POINT('Ctrl Pts',(3.87696881815577,-0.319434907277091,
9.24846564558703));
#56350=CARTESIAN_POINT('Ctrl Pts',(3.859680635308,-0.158333333333299,9.22476527997279));
#56351=CARTESIAN_POINT('Ctrl Pts',(3.87107002642811,0.158333333333301,9.20323489741686));
#56352=CARTESIAN_POINT('Ctrl Pts',(3.89943998848835,0.319434907277099,9.20600033683233));
#56353=CARTESIAN_POINT('Ctrl Pts',(3.97266075653131,0.63630980009507,9.22059396562998));
#56354=CARTESIAN_POINT('Ctrl Pts',(4.02997743362364,0.79477268400067,9.23954790476794));
#56355=CARTESIAN_POINT('Ctrl Pts',(4.13207914134066,1.06847604194625,9.27465870538211));
#56356=CARTESIAN_POINT('Ctrl Pts',(4.18039578318188,1.18514270861422,9.29246707686264));
#56357=CARTESIAN_POINT('Ctrl Pts',(4.23283302083448,1.30000000000371,9.31288565522111));
#56358=CARTESIAN_POINT('Ctrl Pts',(4.10903671786866,-1.30000000000159,9.49882516426784));
#56359=CARTESIAN_POINT('Ctrl Pts',(4.061351450167,-1.1851427086128,9.46007569419142));
#56360=CARTESIAN_POINT('Ctrl Pts',(4.01917031236304,-1.06847604194555,9.42376332368494));
#56361=CARTESIAN_POINT('Ctrl Pts',(3.93443908688951,-0.794772684000702,
9.34550467109699));
#56362=CARTESIAN_POINT('Ctrl Pts',(3.89161685908087,-0.636309800095078,
9.30038240926461));
#56363=CARTESIAN_POINT('Ctrl Pts',(3.84262378705535,-0.319434907277099,
9.23930224859468));
#56364=CARTESIAN_POINT('Ctrl Pts',(3.82713019619362,-0.158333333333302,
9.2150928225414));
#56365=CARTESIAN_POINT('Ctrl Pts',(3.83816214263699,0.158333333333304,9.19438010112749));
#56366=CARTESIAN_POINT('Ctrl Pts',(3.86415948701236,0.319434907277105,9.19892024455919));
#56367=CARTESIAN_POINT('Ctrl Pts',(3.93669973058322,0.636309800095086,9.21568467338448));
#56368=CARTESIAN_POINT('Ctrl Pts',(3.99271182765839,0.794772684000693,9.23585465060728));
#56369=CARTESIAN_POINT('Ctrl Pts',(4.09946236095896,1.06847604194628,9.27261956501576));
#56370=CARTESIAN_POINT('Ctrl Pts',(4.15113581682079,1.18514270861425,9.29105755113202));
#56371=CARTESIAN_POINT('Ctrl Pts',(4.20827437817544,1.30000000000374,9.31201935419136));
#56372=CARTESIAN_POINT('Ctrl Pts',(4.08562660246539,-1.3000000000017,9.49464937055466));
#56373=CARTESIAN_POINT('Ctrl Pts',(4.03371314955642,-1.1851427086129,9.4542482621586));
#56374=CARTESIAN_POINT('Ctrl Pts',(3.98845561452364,-1.06847604194563,9.41668722866343));
#56375=CARTESIAN_POINT('Ctrl Pts',(3.89927815666511,-0.794772684000763,
9.33647486840692));
#56376=CARTESIAN_POINT('Ctrl Pts',(3.8573058510564,-0.636309800095127,9.29149740985962));
#56377=CARTESIAN_POINT('Ctrl Pts',(3.80838819730487,-0.319434907277124,
9.22985627576571));
#56378=CARTESIAN_POINT('Ctrl Pts',(3.79467846287215,-0.158333333333315,
9.20528955941735));
#56379=CARTESIAN_POINT('Ctrl Pts',(3.80554313196228,0.158333333333317,9.18491910142369));
#56380=CARTESIAN_POINT('Ctrl Pts',(3.82971530510416,0.319434907277131,9.18977189492765));
#56381=CARTESIAN_POINT('Ctrl Pts',(3.90158282183463,0.636309800095136,9.20858255798319));
#56382=CARTESIAN_POINT('Ctrl Pts',(3.95581854544446,0.794772684000755,9.23100648829692));
#56383=CARTESIAN_POINT('Ctrl Pts',(4.06686014882141,1.06847604194636,9.27036243486625));
#56384=CARTESIAN_POINT('Ctrl Pts',(4.1217476047809,1.18514270861435,9.28985272324412));
#56385=CARTESIAN_POINT('Ctrl Pts',(4.18345672109462,1.30000000000384,9.31179756901142));
#56386=CARTESIAN_POINT('Ctrl Pts',(4.06476527097544,-1.30000000000171,9.49189931303782));
#56387=CARTESIAN_POINT('Ctrl Pts',(4.00893066569573,-1.18514270861291,9.45058725719531));
#56388=CARTESIAN_POINT('Ctrl Pts',(3.96094698949746,-1.06847604194565,9.41203188116684));
#56389=CARTESIAN_POINT('Ctrl Pts',(3.86823231512926,-0.794772684000776,
9.32932973140712));
#56390=CARTESIAN_POINT('Ctrl Pts',(3.82824956240086,-0.636309800095136,
9.28164581924606));
#56391=CARTESIAN_POINT('Ctrl Pts',(3.77963133894567,-0.319434907277128,
9.21892992138924));
#56392=CARTESIAN_POINT('Ctrl Pts',(3.76674394264146,-0.158333333333317,
9.19563699343125));
#56393=CARTESIAN_POINT('Ctrl Pts',(3.77714975638311,0.158333333333319,9.17623377571701));
#56394=CARTESIAN_POINT('Ctrl Pts',(3.79968841658033,0.319434907277137,9.18150531272934));
#56395=CARTESIAN_POINT('Ctrl Pts',(3.87103949709614,0.636309800095146,9.20188357154754));
#56396=CARTESIAN_POINT('Ctrl Pts',(3.92397236152757,0.794772684000764,9.22562109864878));
#56397=CARTESIAN_POINT('Ctrl Pts',(4.03895466182375,1.06847604194638,9.26668233308603));
#56398=CARTESIAN_POINT('Ctrl Pts',(4.09671988751846,1.18514270861436,9.28687634149948));
#56399=CARTESIAN_POINT('Ctrl Pts',(4.16247876162346,1.30000000000386,9.30949047140706));
#56400=CARTESIAN_POINT('Ctrl Pts',(4.05300830437315,-1.30000000000172,9.48988652188689));
#56401=CARTESIAN_POINT('Ctrl Pts',(3.9951467741753,-1.18514270861292,9.44748701561431));
#56402=CARTESIAN_POINT('Ctrl Pts',(3.94568816028232,-1.06847604194565,9.40811724880978));
#56403=CARTESIAN_POINT('Ctrl Pts',(3.85084128568987,-0.794772684000781,
9.32416451586521));
#56404=CARTESIAN_POINT('Ctrl Pts',(3.81121873941074,-0.63630980009514,9.27670424684079));
#56405=CARTESIAN_POINT('Ctrl Pts',(3.76272615397381,-0.31943490727713,9.21352490123455));
#56406=CARTESIAN_POINT('Ctrl Pts',(3.75088814885211,-0.158333333333318,
9.18976750887703));
#56407=CARTESIAN_POINT('Ctrl Pts',(3.76125912769879,0.15833333333332,9.17040872169655));
#56408=CARTESIAN_POINT('Ctrl Pts',(3.78279108341697,0.319434907277138,9.17598169012332));
#56409=CARTESIAN_POINT('Ctrl Pts',(3.85378766382737,0.636309800095149,9.19733648673911));
#56410=CARTESIAN_POINT('Ctrl Pts',(3.9059106641595,0.794772684000769,9.22188953620525));
#56411=CARTESIAN_POINT('Ctrl Pts',(4.02296625161793,1.06847604194638,9.26447013023481));
#56412=CARTESIAN_POINT('Ctrl Pts',(4.08227787528785,1.18514270861437,9.28540156791325));
#56413=CARTESIAN_POINT('Ctrl Pts',(4.15023209615361,1.30000000000387,9.30883288188111));
#56414=CARTESIAN_POINT('Ctrl Pts',(4.04144316270885,-1.30000000000174,9.48751020962183));
#56415=CARTESIAN_POINT('Ctrl Pts',(3.98134733969823,-1.18514270861294,9.44466768895473));
#56416=CARTESIAN_POINT('Ctrl Pts',(3.93034658136215,-1.06847604194567,9.40477431602907));
#56417=CARTESIAN_POINT('Ctrl Pts',(3.83353604579894,-0.794772684000792,
9.31942576518684));
#56418=CARTESIAN_POINT('Ctrl Pts',(3.79515903035351,-0.636309800095149,
9.27027912947151));
#56419=CARTESIAN_POINT('Ctrl Pts',(3.74684641269738,-0.319434907277135,
9.20648707084666));
#56420=CARTESIAN_POINT('Ctrl Pts',(3.7353888107615,-0.15833333333332,9.18354148532602));
#56421=CARTESIAN_POINT('Ctrl Pts',(3.74544793581991,0.158333333333322,9.16480478031421));
#56422=CARTESIAN_POINT('Ctrl Pts',(3.76610354892916,0.319434907277142,9.17051118864721));
#56423=CARTESIAN_POINT('Ctrl Pts',(3.8366599070298,0.636309800095158,9.19308757189826));
#56424=CARTESIAN_POINT('Ctrl Pts',(3.88783887820413,0.794772684000781,9.21885807701802));
#56425=CARTESIAN_POINT('Ctrl Pts',(4.00690630380797,1.0684760419464,9.26291631106989));
#56426=CARTESIAN_POINT('Ctrl Pts',(4.06775871787748,1.18514270861439,9.28445566000726));
#56427=CARTESIAN_POINT('Ctrl Pts',(4.13792366935522,1.30000000000389,9.30846318087929));
#56428=CARTESIAN_POINT('Ctrl Pts',(4.02679641465004,-1.30000000000176,9.48473812544725));
#56429=CARTESIAN_POINT('Ctrl Pts',(3.96397800532106,-1.18514270861296,9.44073038492449));
#56430=CARTESIAN_POINT('Ctrl Pts',(3.91106087662922,-1.06847604194569,9.39981049157656));
#56431=CARTESIAN_POINT('Ctrl Pts',(3.81168566233224,-0.794772684000809,
9.31241089664204));
#56432=CARTESIAN_POINT('Ctrl Pts',(3.77465916953601,-0.636309800095161,
9.26155524778288));
#56433=CARTESIAN_POINT('Ctrl Pts',(3.72613506221229,-0.31943490727714,9.19795344267425));
#56434=CARTESIAN_POINT('Ctrl Pts',(3.71453984184334,-0.158333333333323,
9.1776908962965));
#56435=CARTESIAN_POINT('Ctrl Pts',(3.72425182411421,0.158333333333325,9.15966462875999));
#56436=CARTESIAN_POINT('Ctrl Pts',(3.74449936440215,0.319434907277149,9.1637828297215));
#56437=CARTESIAN_POINT('Ctrl Pts',(3.8149645362383,0.63630980009517,9.1868330859365));
#56438=CARTESIAN_POINT('Ctrl Pts',(3.86499909873929,0.794772684000796,9.21395294551675));
#56439=CARTESIAN_POINT('Ctrl Pts',(3.98685367567479,1.06847604194642,9.2597023465543));
#56440=CARTESIAN_POINT('Ctrl Pts',(4.0497576568466,1.18514270861441,9.28203736398851));
#56441=CARTESIAN_POINT('Ctrl Pts',(4.12281928799156,1.30000000000391,9.30690417833001));
#56442=CARTESIAN_POINT('Ctrl Pts',(4.01233725084441,-1.30000000000178,9.48188657085733));
#56443=CARTESIAN_POINT('Ctrl Pts',(3.9472834804975,-1.18514270861298,9.43630715904329));
#56444=CARTESIAN_POINT('Ctrl Pts',(3.89267239169235,-1.0684760419457,9.39438957704579));
#56445=CARTESIAN_POINT('Ctrl Pts',(3.79063453505462,-0.794772684000821,
9.306011136471));
#56446=CARTESIAN_POINT('Ctrl Pts',(3.75355465833583,-0.636309800095172,
9.25664233164415));
#56447=CARTESIAN_POINT('Ctrl Pts',(3.70467963936613,-0.319434907277146,
9.1937453763877));
#56448=CARTESIAN_POINT('Ctrl Pts',(3.69376706484766,-0.158333333333326,
9.17421339617309));
#56449=CARTESIAN_POINT('Ctrl Pts',(3.70366827837763,0.158333333333328,9.15571193937935));
#56450=CARTESIAN_POINT('Ctrl Pts',(3.72374766534792,0.319434907277155,9.15786439977874));
#56451=CARTESIAN_POINT('Ctrl Pts',(3.79428666548469,0.636309800095182,9.18078991485239));
#56452=CARTESIAN_POINT('Ctrl Pts',(3.84313183150337,0.79477268400081,9.20920658112124));
#56453=CARTESIAN_POINT('Ctrl Pts',(3.96749298935426,1.06847604194644,9.25639049870806));
#56454=CARTESIAN_POINT('Ctrl Pts',(4.03225771668887,1.18514270861443,9.27942293886111));
#56455=CARTESIAN_POINT('Ctrl Pts',(4.10795583415916,1.30000000000393,9.3050636495802));
#56456=CARTESIAN_POINT('Ctrl Pts',(3.99511068658432,-1.3000000000018,9.47779791444803));
#56457=CARTESIAN_POINT('Ctrl Pts',(3.9270731722259,-1.18514270861299,9.42999191937879));
#56458=CARTESIAN_POINT('Ctrl Pts',(3.87009092852604,-1.06847604194572,9.38682542708467));
#56459=CARTESIAN_POINT('Ctrl Pts',(3.7639904331415,-0.794772684000831,9.29782037399825));
#56460=CARTESIAN_POINT('Ctrl Pts',(3.72599406279882,-0.63630980009518,9.25179941472985));
#56461=CARTESIAN_POINT('Ctrl Pts',(3.67606437133554,-0.31943490727715,9.19082028115558));
#56462=CARTESIAN_POINT('Ctrl Pts',(3.66613937014711,-0.158333333333328,
9.17217087182118));
#56463=CARTESIAN_POINT('Ctrl Pts',(3.67598751442257,0.15833333333333,9.15373611402291));
#56464=CARTESIAN_POINT('Ctrl Pts',(3.69515312446211,0.319434907277158,9.15474944508824));
#56465=CARTESIAN_POINT('Ctrl Pts',(3.76638028263996,0.636309800095189,9.17655145167988));
#56466=CARTESIAN_POINT('Ctrl Pts',(3.81537314735066,0.794772684000819,9.20336749787024));
#56467=CARTESIAN_POINT('Ctrl Pts',(3.94377298237415,1.06847604194645,9.25136176898206));
#56468=CARTESIAN_POINT('Ctrl Pts',(4.01107872912038,1.18514270861444,9.27534533028923));
#56469=CARTESIAN_POINT('Ctrl Pts',(4.09011069171359,1.30000000000395,9.30253751130213));
#56470=CARTESIAN_POINT('Ctrl Pts',(3.9833527785113,-1.30000000000184,9.47508570286668));
#56471=CARTESIAN_POINT('Ctrl Pts',(3.9138153768009,-1.18514270861303,9.42456161217328));
#56472=CARTESIAN_POINT('Ctrl Pts',(3.85550223129827,-1.06847604194575,9.38013053843038));
#56473=CARTESIAN_POINT('Ctrl Pts',(3.74671747692744,-0.794772684000851,
9.29156195773824));
#56474=CARTESIAN_POINT('Ctrl Pts',(3.70705838932682,-0.636309800095197,
9.25183149394815));
#56475=CARTESIAN_POINT('Ctrl Pts',(3.65612349313465,-0.319434907277159,
9.19417216781756));
#56476=CARTESIAN_POINT('Ctrl Pts',(3.64724201481595,-0.158333333333332,
9.17575399890262));
#56477=CARTESIAN_POINT('Ctrl Pts',(3.65704996975842,0.158333333333334,9.15750177715454));
#56478=CARTESIAN_POINT('Ctrl Pts',(3.67523755008904,0.319434907277167,9.15838530604779));
#56479=CARTESIAN_POINT('Ctrl Pts',(3.74717278258775,0.636309800095206,9.17740450837209));
#56480=CARTESIAN_POINT('Ctrl Pts',(3.79716553103066,0.79477268400084,9.19876566584626));
#56481=CARTESIAN_POINT('Ctrl Pts',(3.92828386839332,1.06847604194648,9.24627537344296));
#56482=CARTESIAN_POINT('Ctrl Pts',(3.99710096186775,1.18514270861448,9.27127676663499));
#56483=CARTESIAN_POINT('Ctrl Pts',(4.07797887898519,1.30000000000399,9.30071436100847));
#56484=CARTESIAN_POINT('Ctrl Pts',(3.97477914228584,-1.30000000000184,9.47578453352629));
#56485=CARTESIAN_POINT('Ctrl Pts',(3.90549290340901,-1.18514270861303,9.42526901565753));
#56486=CARTESIAN_POINT('Ctrl Pts',(3.84729017393194,-1.06847604194575,9.38116464394731));
#56487=CARTESIAN_POINT('Ctrl Pts',(3.73843534938598,-0.794772684000851,
9.29408575241927));
#56488=CARTESIAN_POINT('Ctrl Pts',(3.69814954202848,-0.636309800095197,
9.25684331707449));
#56489=CARTESIAN_POINT('Ctrl Pts',(3.64686579593571,-0.319434907277159,
9.20083410021132));
#56490=CARTESIAN_POINT('Ctrl Pts',(3.6379450782909,-0.158333333333332,9.18238128424967));
#56491=CARTESIAN_POINT('Ctrl Pts',(3.64772547716597,0.158333333333334,9.16436428106718));
#56492=CARTESIAN_POINT('Ctrl Pts',(3.66586376136843,0.319434907277167,9.16579102070237));
#56493=CARTESIAN_POINT('Ctrl Pts',(3.73821592466294,0.636309800095206,9.18308245269344));
#56494=CARTESIAN_POINT('Ctrl Pts',(3.78913144751243,0.79477268400084,9.20091302212069));
#56495=CARTESIAN_POINT('Ctrl Pts',(3.9202668858623,1.06847604194648,9.24707722512988));
#56496=CARTESIAN_POINT('Ctrl Pts',(3.98887475074185,1.18514270861448,9.27205620607566));
#56497=CARTESIAN_POINT('Ctrl Pts',(4.06932680828582,1.30000000000399,9.30203139503673));
#56498=CARTESIAN_POINT('Ctrl Pts',(3.97477914228473,-1.3,9.47578453352548));
#56499=CARTESIAN_POINT('Ctrl Pts',(3.90549290340839,-1.18514270861178,9.42526901565706));
#56500=CARTESIAN_POINT('Ctrl Pts',(3.84729017393168,-1.06847604194512,9.38116464394711));
#56501=CARTESIAN_POINT('Ctrl Pts',(3.73843534938597,-0.794772684000851,
9.29408575241928));
#56502=CARTESIAN_POINT('Ctrl Pts',(3.69814954202848,-0.636309800095197,
9.25684331707449));
#56503=CARTESIAN_POINT('Ctrl Pts',(3.64686579593571,-0.319434907277159,
9.20083410021132));
#56504=CARTESIAN_POINT('Ctrl Pts',(3.6379450782909,-0.158333333333332,9.18238128424967));
#56505=CARTESIAN_POINT('Ctrl Pts',(3.64772547716596,0.158333333333334,9.16436428106718));
#56506=CARTESIAN_POINT('Ctrl Pts',(3.66586376136843,0.319434907277167,9.16579102070237));
#56507=CARTESIAN_POINT('Ctrl Pts',(3.73821592466293,0.636309800095206,9.18308245269344));
#56508=CARTESIAN_POINT('Ctrl Pts',(3.78913144751243,0.79477268400084,9.20091302212069));
#56509=CARTESIAN_POINT('Ctrl Pts',(3.92026688586164,1.06847604194511,9.24707722512964));
#56510=CARTESIAN_POINT('Ctrl Pts',(3.98887475074027,1.18514270861178,9.27205620607508));
#56511=CARTESIAN_POINT('Ctrl Pts',(4.06932680828303,1.3,9.30203139503569));
#56512=CARTESIAN_POINT('',(4.38969958549801,-1.2,9.48758334254264));
#56513=CARTESIAN_POINT('Ctrl Pts',(4.38969958549801,-1.2,9.48758334254265));
#56514=CARTESIAN_POINT('Ctrl Pts',(4.37179496097857,-1.21424592766347,9.49111483394103));
#56515=CARTESIAN_POINT('Ctrl Pts',(4.37023623801035,-1.2152654494871,9.49188100659603));
#56516=CARTESIAN_POINT('Ctrl Pts',(4.34578951938456,-1.23433940646938,9.49736529100142));
#56517=CARTESIAN_POINT('Ctrl Pts',(4.34413559802252,-1.23568262283785,9.4976366021116));
#56518=CARTESIAN_POINT('Ctrl Pts',(4.30607628505062,-1.26582530512805,9.50500210141761));
#56519=CARTESIAN_POINT('Ctrl Pts',(4.28598494523318,-1.28169477849993,9.50887284971023));
#56520=CARTESIAN_POINT('Ctrl Pts',(4.26568396548156,-1.29775190384789,9.51262878777734));
#56521=CARTESIAN_POINT('Ctrl Pts',(4.26402397189108,-1.29906490328061,9.51293567589886));
#56522=CARTESIAN_POINT('Ctrl Pts',(4.26284481534483,-1.30000000000121,9.51314808870421));
#56523=CARTESIAN_POINT('',(4.45989077443978,-0.653834841416792,9.34752748057694));
#56524=CARTESIAN_POINT('Ctrl Pts',(4.45989077444373,-0.653834841406665,
9.34752748062317));
#56525=CARTESIAN_POINT('Ctrl Pts',(4.45335390424296,-0.71324393711409,9.36110296562405));
#56526=CARTESIAN_POINT('Ctrl Pts',(4.44674825867249,-0.767188910741388,
9.37466736400092));
#56527=CARTESIAN_POINT('Ctrl Pts',(4.42424889216865,-0.949633080775671,
9.42030531501031));
#56528=CARTESIAN_POINT('Ctrl Pts',(4.40765622707638,-1.07514642494888,9.4531259041501));
#56529=CARTESIAN_POINT('Ctrl Pts',(4.38969958549801,-1.2,9.48758334254265));
#56530=CARTESIAN_POINT('',(4.51863764645953,0.653834841531101,9.22099327559463));
#56531=CARTESIAN_POINT('Ctrl Pts',(4.51863764645953,0.653834841531103,9.22099327559463));
#56532=CARTESIAN_POINT('Ctrl Pts',(4.47693045016882,0.575722054508995,9.22158335555513));
#56533=CARTESIAN_POINT('Ctrl Pts',(4.44183847005026,0.493687365915951,9.22304499129017));
#56534=CARTESIAN_POINT('Ctrl Pts',(4.39135806826372,0.338003356428067,9.22732111455017));
#56535=CARTESIAN_POINT('Ctrl Pts',(4.37365341868297,0.265535567213328,9.23010606782248));
#56536=CARTESIAN_POINT('Ctrl Pts',(4.35059352006431,0.12961539563281,9.23802064758203));
#56537=CARTESIAN_POINT('Ctrl Pts',(4.34382820017673,0.0665936360836524,
9.24270343198728));
#56538=CARTESIAN_POINT('Ctrl Pts',(4.33790267606707,-0.059460756060269,
9.25457757758834));
#56539=CARTESIAN_POINT('Ctrl Pts',(4.3386898198503,-0.122628115771336,9.26183704158793));
#56540=CARTESIAN_POINT('Ctrl Pts',(4.34915453823114,-0.259985608121654,
9.27964603169459));
#56541=CARTESIAN_POINT('Ctrl Pts',(4.36043113662999,-0.33385866782113,9.29057829402112));
#56542=CARTESIAN_POINT('Ctrl Pts',(4.39738321548536,-0.491574905831985,
9.31616686070628));
#56543=CARTESIAN_POINT('Ctrl Pts',(4.42520378272057,-0.575006518919015,
9.33156382633747));
#56544=CARTESIAN_POINT('Ctrl Pts',(4.45989077438544,-0.653834841429743,
9.34752748063108));
#56545=CARTESIAN_POINT('',(4.48864234752075,1.2,9.28676540992117));
#56546=CARTESIAN_POINT('Ctrl Pts',(4.48864234752074,1.2,9.28676540992118));
#56547=CARTESIAN_POINT('Ctrl Pts',(4.49218132781357,1.15574893393819,9.27915304643561));
#56548=CARTESIAN_POINT('Ctrl Pts',(4.49913702961667,1.06765896451643,9.26416425729077));
#56549=CARTESIAN_POINT('Ctrl Pts',(4.51513968970315,0.771844892429185,9.22886092983354));
#56550=CARTESIAN_POINT('Ctrl Pts',(4.51659259837948,0.720814231765372,9.22556569617361));
#56551=CARTESIAN_POINT('Ctrl Pts',(4.51863764645953,0.6538348415311,9.22099327559463));
#56552=CARTESIAN_POINT('Ctrl Pts',(4.36609756959132,1.2999999999998,9.31179828885494));
#56553=CARTESIAN_POINT('Ctrl Pts',(4.37593955631733,1.29200222100087,9.30981805892408));
#56554=CARTESIAN_POINT('Ctrl Pts',(4.38571147514364,1.28374785188112,9.30854997600552));
#56555=CARTESIAN_POINT('Ctrl Pts',(4.41170127702802,1.26274495050229,9.302916177652));
#56556=CARTESIAN_POINT('Ctrl Pts',(4.41770216098965,1.25781029718418,9.30177599792278));
#56557=CARTESIAN_POINT('Ctrl Pts',(4.44118715552041,1.23854687998326,9.29721179869033));
#56558=CARTESIAN_POINT('Ctrl Pts',(4.46588814099277,1.21819525011631,9.29254900537115));
#56559=CARTESIAN_POINT('Ctrl Pts',(4.48864234752075,1.2,9.28676540992118));
#56560=CARTESIAN_POINT('Ctrl Pts',(3.97477914228473,-1.3,9.47578453352548));
#56561=CARTESIAN_POINT('Ctrl Pts',(3.90549290340839,-1.18514270861178,9.42526901565706));
#56562=CARTESIAN_POINT('Ctrl Pts',(3.84729017393169,-1.06847604194512,9.38116464394711));
#56563=CARTESIAN_POINT('Ctrl Pts',(3.73843534938598,-0.794772684000851,
9.29408575241928));
#56564=CARTESIAN_POINT('Ctrl Pts',(3.69814954202848,-0.636309800095196,
9.2568433170745));
#56565=CARTESIAN_POINT('Ctrl Pts',(3.64686579593571,-0.319434907277159,
9.20083410021132));
#56566=CARTESIAN_POINT('Ctrl Pts',(3.6379450782909,-0.158333333333332,9.18238128424968));
#56567=CARTESIAN_POINT('Ctrl Pts',(3.64772547716597,0.158333333333334,9.16436428106718));
#56568=CARTESIAN_POINT('Ctrl Pts',(3.66586376136843,0.319434907277167,9.16579102070238));
#56569=CARTESIAN_POINT('Ctrl Pts',(3.73821592466294,0.636309800095206,9.18308245269344));
#56570=CARTESIAN_POINT('Ctrl Pts',(3.78913144751243,0.79477268400084,9.20091302212069));
#56571=CARTESIAN_POINT('Ctrl Pts',(3.92026688586164,1.06847604194511,9.24707722512965));
#56572=CARTESIAN_POINT('Ctrl Pts',(3.98887475074027,1.18514270861178,9.27205620607508));
#56573=CARTESIAN_POINT('Ctrl Pts',(4.06932680828303,1.3,9.30203139503569));
#56574=CARTESIAN_POINT('Ctrl Pts',(3.93487809212144,-1.3,9.54156458726909));
#56575=CARTESIAN_POINT('Ctrl Pts',(3.86662549823905,-1.18514270861178,9.48965893164399));
#56576=CARTESIAN_POINT('Ctrl Pts',(3.80917822375501,-1.06847604194512,9.4446137960335));
#56577=CARTESIAN_POINT('Ctrl Pts',(3.70142597681593,-0.794772684000851,
9.35639969520083));
#56578=CARTESIAN_POINT('Ctrl Pts',(3.6609356094067,-0.636309800095196,9.31984512113064));
#56579=CARTESIAN_POINT('Ctrl Pts',(3.60969614500507,-0.319434907277159,
9.26450127807643));
#56580=CARTESIAN_POINT('Ctrl Pts',(3.60031408828524,-0.158333333333332,
9.2472011190744));
#56581=CARTESIAN_POINT('Ctrl Pts',(3.61040534854147,0.158333333333334,9.22936359179401));
#56582=CARTESIAN_POINT('Ctrl Pts',(3.6293111934153,0.319434907277167,9.22981447159066));
#56583=CARTESIAN_POINT('Ctrl Pts',(3.70226172817696,0.636309800095206,9.2468115657467));
#56584=CARTESIAN_POINT('Ctrl Pts',(3.75367067633866,0.79477268400084,9.26412105033525));
#56585=CARTESIAN_POINT('Ctrl Pts',(3.88437428339459,1.06847604194511,9.31180771821361));
#56586=CARTESIAN_POINT('Ctrl Pts',(3.95254515033271,1.18514270861178,9.33791132432438));
#56587=CARTESIAN_POINT('Ctrl Pts',(4.0323101357604,1.3,9.36947674498659));
#56588=CARTESIAN_POINT('Ctrl Pts',(3.89497704195815,-1.3,9.60734464101269));
#56589=CARTESIAN_POINT('Ctrl Pts',(3.8277580930697,-1.18514270861178,9.55404884763092));
#56590=CARTESIAN_POINT('Ctrl Pts',(3.77106627357833,-1.06847604194512,9.50806294811988));
#56591=CARTESIAN_POINT('Ctrl Pts',(3.66441660424588,-0.794772684000851,
9.41871363798238));
#56592=CARTESIAN_POINT('Ctrl Pts',(3.62372167678492,-0.636309800095196,
9.38284692518678));
#56593=CARTESIAN_POINT('Ctrl Pts',(3.57252649407444,-0.319434907277159,
9.32816845594153));
#56594=CARTESIAN_POINT('Ctrl Pts',(3.56268309827958,-0.158333333333332,
9.31202095389912));
#56595=CARTESIAN_POINT('Ctrl Pts',(3.57308521991698,0.158333333333334,9.29436290252083));
#56596=CARTESIAN_POINT('Ctrl Pts',(3.59275862546217,0.319434907277167,9.29383792247894));
#56597=CARTESIAN_POINT('Ctrl Pts',(3.66630753169098,0.636309800095206,9.31054067879995));
#56598=CARTESIAN_POINT('Ctrl Pts',(3.71820990516489,0.79477268400084,9.32732907854981));
#56599=CARTESIAN_POINT('Ctrl Pts',(3.84848168092753,1.06847604194511,9.37653821129757));
#56600=CARTESIAN_POINT('Ctrl Pts',(3.91621554992515,1.18514270861178,9.40376644257368));
#56601=CARTESIAN_POINT('Ctrl Pts',(3.99529346323778,1.3,9.43692209493747));
#56602=CARTESIAN_POINT('Ctrl Pts',(3.85507599179486,-1.3,9.6731246947563));
#56603=CARTESIAN_POINT('Ctrl Pts',(3.78889068790036,-1.18514270861178,9.61843876361785));
#56604=CARTESIAN_POINT('Ctrl Pts',(3.73295432340165,-1.06847604194512,9.57151210020627));
#56605=CARTESIAN_POINT('Ctrl Pts',(3.62740723167584,-0.794772684000851,
9.48102758076393));
#56606=CARTESIAN_POINT('Ctrl Pts',(3.58650774416314,-0.636309800095196,
9.44584872924292));
#56607=CARTESIAN_POINT('Ctrl Pts',(3.5353568431438,-0.319434907277159,9.39183563380664));
#56608=CARTESIAN_POINT('Ctrl Pts',(3.52505210827392,-0.158333333333332,
9.37684078872385));
#56609=CARTESIAN_POINT('Ctrl Pts',(3.53576509129249,0.158333333333334,9.35936221324765));
#56610=CARTESIAN_POINT('Ctrl Pts',(3.55620605750904,0.319434907277167,9.35786137336723));
#56611=CARTESIAN_POINT('Ctrl Pts',(3.630353335205,0.636309800095206,9.37426979185321));
#56612=CARTESIAN_POINT('Ctrl Pts',(3.68274913399112,0.79477268400084,9.39053710676437));
#56613=CARTESIAN_POINT('Ctrl Pts',(3.81258907846048,1.06847604194511,9.44126870438153));
#56614=CARTESIAN_POINT('Ctrl Pts',(3.8798859495176,1.18514270861178,9.46962156082298));
#56615=CARTESIAN_POINT('Ctrl Pts',(3.95827679071515,1.3,9.50436744488836));
#56616=CARTESIAN_POINT('Ctrl Pts',(3.85507599179486,-1.3,9.6731246947563));
#56617=CARTESIAN_POINT('Ctrl Pts',(3.78889068790036,-1.18514270861178,9.61843876361785));
#56618=CARTESIAN_POINT('Ctrl Pts',(3.73295432340165,-1.06847604194512,9.57151210020627));
#56619=CARTESIAN_POINT('Ctrl Pts',(3.62740723167584,-0.794772684000851,
9.48102758076393));
#56620=CARTESIAN_POINT('Ctrl Pts',(3.58650774416314,-0.636309800095197,
9.44584872924292));
#56621=CARTESIAN_POINT('Ctrl Pts',(3.5353568431438,-0.319434907277159,9.39183563380664));
#56622=CARTESIAN_POINT('Ctrl Pts',(3.52505210827391,-0.158333333333332,
9.37684078872385));
#56623=CARTESIAN_POINT('Ctrl Pts',(3.53576509129248,0.158333333333334,9.35936221324765));
#56624=CARTESIAN_POINT('Ctrl Pts',(3.55620605750904,0.319434907277167,9.35786137336722));
#56625=CARTESIAN_POINT('Ctrl Pts',(3.630353335205,0.636309800095206,9.3742697918532));
#56626=CARTESIAN_POINT('Ctrl Pts',(3.68274913399112,0.79477268400084,9.39053710676437));
#56627=CARTESIAN_POINT('Ctrl Pts',(3.81258907846048,1.06847604194511,9.44126870438153));
#56628=CARTESIAN_POINT('Ctrl Pts',(3.8798859495176,1.18514270861178,9.46962156082298));
#56629=CARTESIAN_POINT('Ctrl Pts',(3.95827679071515,1.3,9.50436744488836));
#56630=CARTESIAN_POINT('Ctrl Pts',(3.85507599179591,-1.30000000000182,9.67312469475717));
#56631=CARTESIAN_POINT('Ctrl Pts',(3.78889068790095,-1.18514270861302,9.61843876361835));
#56632=CARTESIAN_POINT('Ctrl Pts',(3.73295432340189,-1.06847604194574,9.57151210020649));
#56633=CARTESIAN_POINT('Ctrl Pts',(3.62740723167583,-0.794772684000851,
9.48102758076393));
#56634=CARTESIAN_POINT('Ctrl Pts',(3.58650774416313,-0.636309800095197,
9.44584872924292));
#56635=CARTESIAN_POINT('Ctrl Pts',(3.5353568431438,-0.319434907277159,9.39183563380664));
#56636=CARTESIAN_POINT('Ctrl Pts',(3.52505210827391,-0.158333333333332,
9.37684078872385));
#56637=CARTESIAN_POINT('Ctrl Pts',(3.53576509129248,0.158333333333334,9.35936221324765));
#56638=CARTESIAN_POINT('Ctrl Pts',(3.55620605750903,0.319434907277167,9.35786137336722));
#56639=CARTESIAN_POINT('Ctrl Pts',(3.630353335205,0.636309800095206,9.3742697918532));
#56640=CARTESIAN_POINT('Ctrl Pts',(3.68274913399112,0.79477268400084,9.39053710676436));
#56641=CARTESIAN_POINT('Ctrl Pts',(3.81258907846058,1.06847604194533,9.44126870438157));
#56642=CARTESIAN_POINT('Ctrl Pts',(3.87988594951784,1.18514270861221,9.46962156082308));
#56643=CARTESIAN_POINT('Ctrl Pts',(3.95827679071559,1.30000000000064,9.50436744488855));
#56644=CARTESIAN_POINT('Ctrl Pts',(3.85826144216853,-1.30000000000182,9.68127612476138));
#56645=CARTESIAN_POINT('Ctrl Pts',(3.79232877906293,-1.18514270861302,9.62595259112397));
#56646=CARTESIAN_POINT('Ctrl Pts',(3.73626839069632,-1.06847604194574,9.57885593655991));
#56647=CARTESIAN_POINT('Ctrl Pts',(3.62956460831631,-0.794772684000851,
9.48905897930467));
#56648=CARTESIAN_POINT('Ctrl Pts',(3.58606892907603,-0.636309800095197,
9.45644456788996));
#56649=CARTESIAN_POINT('Ctrl Pts',(3.53363020043342,-0.319434907277159,
9.40365643026874));
#56650=CARTESIAN_POINT('Ctrl Pts',(3.52377125174929,-0.158333333333332,
9.38834728808437));
#56651=CARTESIAN_POINT('Ctrl Pts',(3.53467416199073,0.158333333333334,9.37072723907264));
#56652=CARTESIAN_POINT('Ctrl Pts',(3.55506550337818,0.319434907277167,9.36920974049564));
#56653=CARTESIAN_POINT('Ctrl Pts',(3.63046739269399,0.636309800095206,9.3844909914869));
#56654=CARTESIAN_POINT('Ctrl Pts',(3.68470452743246,0.79477268400084,9.39897153694001));
#56655=CARTESIAN_POINT('Ctrl Pts',(3.81579954547164,1.06847604194533,9.44889760742223));
#56656=CARTESIAN_POINT('Ctrl Pts',(3.88343455679883,1.18514270861221,9.47718273592917));
#56657=CARTESIAN_POINT('Ctrl Pts',(3.96195840369317,1.30000000000064,9.51214184697453));
#56658=CARTESIAN_POINT('Ctrl Pts',(3.86592075441267,-1.3000000000016,9.69085660596058));
#56659=CARTESIAN_POINT('Ctrl Pts',(3.80285615568279,-1.18514270861281,9.6360113152689));
#56660=CARTESIAN_POINT('Ctrl Pts',(3.74843370181331,-1.06847604194556,9.58971588520396));
#56661=CARTESIAN_POINT('Ctrl Pts',(3.64267202968321,-0.794772684000714,
9.50251606882662));
#56662=CARTESIAN_POINT('Ctrl Pts',(3.59495986472817,-0.636309800095087,
9.4734863929025));
#56663=CARTESIAN_POINT('Ctrl Pts',(3.54045869646006,-0.319434907277103,
9.42271066769787));
#56664=CARTESIAN_POINT('Ctrl Pts',(3.52998469589636,-0.158333333333305,
9.40663233159606));
#56665=CARTESIAN_POINT('Ctrl Pts',(3.54101091709157,0.158333333333307,9.38890595207223));
#56666=CARTESIAN_POINT('Ctrl Pts',(3.56210793646514,0.319434907277111,9.38820387356399));
#56667=CARTESIAN_POINT('Ctrl Pts',(3.63989001762102,0.636309800095095,9.40094537760262));
#56668=CARTESIAN_POINT('Ctrl Pts',(3.69878792708314,0.794772684000703,9.41078085457383));
#56669=CARTESIAN_POINT('Ctrl Pts',(3.82891377614039,1.06847604194514,9.45816504858586));
#56670=CARTESIAN_POINT('Ctrl Pts',(3.89477549884898,1.185142708612,9.48594306864129));
#56671=CARTESIAN_POINT('Ctrl Pts',(3.97017228584713,1.30000000000041,9.52098824692175));
#56672=CARTESIAN_POINT('Ctrl Pts',(3.87702049239457,-1.30000000000152,9.70505728721452));
#56673=CARTESIAN_POINT('Ctrl Pts',(3.81695192563871,-1.18514270861274,9.65233487555218));
#56674=CARTESIAN_POINT('Ctrl Pts',(3.76461562236306,-1.06847604194549,9.60776978846544));
#56675=CARTESIAN_POINT('Ctrl Pts',(3.66157136742828,-0.794772684000663,
9.52366057371701));
#56676=CARTESIAN_POINT('Ctrl Pts',(3.61256958719336,-0.636309800095047,
9.49553345653393));
#56677=CARTESIAN_POINT('Ctrl Pts',(3.55745187272802,-0.319434907277084,
9.44590006181212));
#56678=CARTESIAN_POINT('Ctrl Pts',(3.54553271193669,-0.158333333333295,
9.42960489072957));
#56679=CARTESIAN_POINT('Ctrl Pts',(3.55660302454435,0.158333333333297,9.41177959321342));
#56680=CARTESIAN_POINT('Ctrl Pts',(3.57898330847349,0.319434907277092,9.41144980867689));
#56681=CARTESIAN_POINT('Ctrl Pts',(3.65789132771862,0.636309800095056,9.42232934580547));
#56682=CARTESIAN_POINT('Ctrl Pts',(3.71918153657403,0.794772684000653,9.42976789819879));
#56683=CARTESIAN_POINT('Ctrl Pts',(3.84673170978875,1.06847604194508,9.47395772293737));
#56684=CARTESIAN_POINT('Ctrl Pts',(3.91033538333747,1.18514270861193,9.50029893905725));
#56685=CARTESIAN_POINT('Ctrl Pts',(3.98233098664991,1.30000000000033,9.53385323356206));
#56686=CARTESIAN_POINT('Ctrl Pts',(3.88609751225472,-1.30000000000136,9.71696191407412));
#56687=CARTESIAN_POINT('Ctrl Pts',(3.8280562708361,-1.18514270861259,9.66611118291763));
#56688=CARTESIAN_POINT('Ctrl Pts',(3.77727688753419,-1.06847604194536,9.622797964979));
#56689=CARTESIAN_POINT('Ctrl Pts',(3.67674269870558,-0.794772684000565,
9.54014893016903));
#56690=CARTESIAN_POINT('Ctrl Pts',(3.62822311218295,-0.636309800094969,
9.51039538953031));
#56691=CARTESIAN_POINT('Ctrl Pts',(3.57299221293527,-0.319434907277045,
9.46094020063014));
#56692=CARTESIAN_POINT('Ctrl Pts',(3.55926865253983,-0.158333333333275,
9.44549008317312));
#56693=CARTESIAN_POINT('Ctrl Pts',(3.56996630046896,0.158333333333277,9.42814702429819));
#56694=CARTESIAN_POINT('Ctrl Pts',(3.59323177200466,0.31943490727705,9.42819201949836));
#56695=CARTESIAN_POINT('Ctrl Pts',(3.67260716245088,0.636309800094976,9.43837320885701));
#56696=CARTESIAN_POINT('Ctrl Pts',(3.73535384608084,0.794772684000557,9.44474638814701));
#56697=CARTESIAN_POINT('Ctrl Pts',(3.8607200019921,1.06847604194495,9.4870934019074));
#56698=CARTESIAN_POINT('Ctrl Pts',(3.92256824207985,1.18514270861178,9.51250695438991));
#56699=CARTESIAN_POINT('Ctrl Pts',(3.99199835863522,1.30000000000017,9.54500360620956));
#56700=CARTESIAN_POINT('Ctrl Pts',(3.89668925415032,-1.30000000000122,9.7318062296122));
#56701=CARTESIAN_POINT('Ctrl Pts',(3.84118533284187,-1.18514270861247,9.68351819215851));
#56702=CARTESIAN_POINT('Ctrl Pts',(3.7924107075366,-1.06847604194525,9.64189074955766));
#56703=CARTESIAN_POINT('Ctrl Pts',(3.69527758570974,-0.794772684000484,
9.56111033616606));
#56704=CARTESIAN_POINT('Ctrl Pts',(3.6476050737869,-0.636309800094904,9.52920935386177));
#56705=CARTESIAN_POINT('Ctrl Pts',(3.59290071013923,-0.319434907277012,
9.47926493980645));
#56706=CARTESIAN_POINT('Ctrl Pts',(3.57729331001879,-0.158333333333259,
9.4643543837362));
#56707=CARTESIAN_POINT('Ctrl Pts',(3.58862627895774,0.158333333333261,9.44606816444191));
#56708=CARTESIAN_POINT('Ctrl Pts',(3.61478304260594,0.319434907277019,9.44405152824428));
#56709=CARTESIAN_POINT('Ctrl Pts',(3.69416799578257,0.636309800094912,9.45397999004903));
#56710=CARTESIAN_POINT('Ctrl Pts',(3.75556658383759,0.794772684000476,9.46332859835313));
#56711=CARTESIAN_POINT('Ctrl Pts',(3.87726096117718,1.06847604194484,9.50430770534805));
#56712=CARTESIAN_POINT('Ctrl Pts',(3.93697193200774,1.18514270861166,9.52827507090723));
#56713=CARTESIAN_POINT('Ctrl Pts',(4.0037168869396,1.30000000000004,9.55847146503303));
#56714=CARTESIAN_POINT('Ctrl Pts',(3.90634129735519,-1.3000000000009,9.74759065323477));
#56715=CARTESIAN_POINT('Ctrl Pts',(3.85342469448244,-1.18514270861217,9.70153780835584));
#56716=CARTESIAN_POINT('Ctrl Pts',(3.80670493679023,-1.06847604194498,9.66133186724594));
#56717=CARTESIAN_POINT('Ctrl Pts',(3.71308890230765,-0.794772684000283,
9.58195561748694));
#56718=CARTESIAN_POINT('Ctrl Pts',(3.66601329086534,-0.636309800094744,
9.54824301996284));
#56719=CARTESIAN_POINT('Ctrl Pts',(3.61258653861628,-0.319434907276932,
9.49675443327196));
#56720=CARTESIAN_POINT('Ctrl Pts',(3.59690518833244,-0.15833333333322,9.48001577447521));
#56721=CARTESIAN_POINT('Ctrl Pts',(3.608493963035,0.158333333333222,9.461317513484));
#56722=CARTESIAN_POINT('Ctrl Pts',(3.63496333697317,0.31943490727694,9.46067316835298));
#56723=CARTESIAN_POINT('Ctrl Pts',(3.71362666110114,0.636309800094754,9.47139565978765));
#56724=CARTESIAN_POINT('Ctrl Pts',(3.77484661577608,0.794772684000275,9.48210622793863));
#56725=CARTESIAN_POINT('Ctrl Pts',(3.89338202163702,1.06847604194457,9.52137630637699));
#56726=CARTESIAN_POINT('Ctrl Pts',(3.95113583823423,1.18514270861136,9.5438845238286));
#56727=CARTESIAN_POINT('Ctrl Pts',(4.01533388640107,1.29999999999971,9.57190239687566));
#56728=CARTESIAN_POINT('Ctrl Pts',(3.92055275904314,-1.30000000000069,9.76714384265902));
#56729=CARTESIAN_POINT('Ctrl Pts',(3.87074553539678,-1.18514270861199,9.72462993178228));
#56730=CARTESIAN_POINT('Ctrl Pts',(3.82646932967549,-1.06847604194481,9.68679759168984));
#56731=CARTESIAN_POINT('Ctrl Pts',(3.73696019491823,-0.794772684000161,
9.61021268279958));
#56732=CARTESIAN_POINT('Ctrl Pts',(3.69053367825845,-0.636309800094645,
9.57431182373749));
#56733=CARTESIAN_POINT('Ctrl Pts',(3.63824691831124,-0.319434907276882,
9.5215524571651));
#56734=CARTESIAN_POINT('Ctrl Pts',(3.62175628555497,-0.158333333333195,
9.50327554072841));
#56735=CARTESIAN_POINT('Ctrl Pts',(3.63382136573945,0.158333333333197,9.48387740247822));
#56736=CARTESIAN_POINT('Ctrl Pts',(3.66183719787731,0.319434907276889,9.48366594610305));
#56737=CARTESIAN_POINT('Ctrl Pts',(3.73979935576851,0.636309800094653,9.49505957507951));
#56738=CARTESIAN_POINT('Ctrl Pts',(3.80018656415803,0.794772684000152,9.50830811335043));
#56739=CARTESIAN_POINT('Ctrl Pts',(3.91424294631096,1.0684760419444,9.5454000284948));
#56740=CARTESIAN_POINT('Ctrl Pts',(3.96930245432026,1.18514270861118,9.5659264892443));
#56741=CARTESIAN_POINT('Ctrl Pts',(4.03005068871032,1.29999999999951,9.59092369506821));
#56742=CARTESIAN_POINT('Ctrl Pts',(3.94293405228111,-1.30000000000015,9.80416499781465));
#56743=CARTESIAN_POINT('Ctrl Pts',(3.8983024693755,-1.18514270861149,9.76803405560948));
#56744=CARTESIAN_POINT('Ctrl Pts',(3.85820837626867,-1.06847604194437,9.73438444526762));
#56745=CARTESIAN_POINT('Ctrl Pts',(3.77606550955316,-0.794772683999828,
9.66237948678966));
#56746=CARTESIAN_POINT('Ctrl Pts',(3.73140337306608,-0.636309800094378,
9.62201111664065));
#56747=CARTESIAN_POINT('Ctrl Pts',(3.68201299142563,-0.319434907276748,
9.56597413151367));
#56748=CARTESIAN_POINT('Ctrl Pts',(3.66527160877993,-0.158333333333129,
9.54356452515937));
#56749=CARTESIAN_POINT('Ctrl Pts',(3.67795836472447,0.158333333333131,9.52326664911772));
#56750=CARTESIAN_POINT('Ctrl Pts',(3.70674579656327,0.319434907276756,9.52630170301223));
#56751=CARTESIAN_POINT('Ctrl Pts',(3.78328326010629,0.636309800094388,9.53911263248325));
#56752=CARTESIAN_POINT('Ctrl Pts',(3.84350301597519,0.794772683999818,9.55503418266844));
#56753=CARTESIAN_POINT('Ctrl Pts',(3.95059279887267,1.06847604194395,9.58729351177311));
#56754=CARTESIAN_POINT('Ctrl Pts',(4.00127565766729,1.18514270861068,9.60400458986381));
#56755=CARTESIAN_POINT('Ctrl Pts',(4.0562861763077,1.29999999999897,9.62346287780173));
#56756=CARTESIAN_POINT('Ctrl Pts',(3.96875291306454,-1.29999999999862,9.84603918270511));
#56757=CARTESIAN_POINT('Ctrl Pts',(3.93016088876956,-1.1851427086101,9.81706547124778));
#56758=CARTESIAN_POINT('Ctrl Pts',(3.89466683773055,-1.06847604194311,9.78844476197471));
#56759=CARTESIAN_POINT('Ctrl Pts',(3.81982541723873,-0.794772683998892,
9.72314070366436));
#56760=CARTESIAN_POINT('Ctrl Pts',(3.77508220407105,-0.636309800093627,
9.68031539928032));
#56761=CARTESIAN_POINT('Ctrl Pts',(3.72755718756055,-0.319434907276371,
9.62250450440374));
#56762=CARTESIAN_POINT('Ctrl Pts',(3.71010374373434,-0.158333333332942,
9.59611900134765));
#56763=CARTESIAN_POINT('Ctrl Pts',(3.723858703403,0.158333333332944,9.57443114782916));
#56764=CARTESIAN_POINT('Ctrl Pts',(3.75491767159857,0.319434907276382,9.57935654222014));
#56765=CARTESIAN_POINT('Ctrl Pts',(3.8307649395092,0.63630980009364,9.59252694118864));
#56766=CARTESIAN_POINT('Ctrl Pts',(3.89074061160296,0.79477268399888,9.61149586566595));
#56767=CARTESIAN_POINT('Ctrl Pts',(3.99041779475234,1.06847604194269,9.63743017681932));
#56768=CARTESIAN_POINT('Ctrl Pts',(4.03637498942812,1.18514270860928,9.64938301440751));
#56769=CARTESIAN_POINT('Ctrl Pts',(4.08514281959792,1.29999999999743,9.6620626872465));
#56770=CARTESIAN_POINT('Ctrl Pts',(3.98735158280415,-1.29999999999731,9.87931932511148));
#56771=CARTESIAN_POINT('Ctrl Pts',(3.95241863019103,-1.1851427086089,9.8568395664758));
#56772=CARTESIAN_POINT('Ctrl Pts',(3.91986501806147,-1.06847604194203,9.83267478419246));
#56773=CARTESIAN_POINT('Ctrl Pts',(3.85015641421704,-0.794772683998091,
9.77295656125614));
#56774=CARTESIAN_POINT('Ctrl Pts',(3.80654379785225,-0.636309800092987,
9.72693137572071));
#56775=CARTESIAN_POINT('Ctrl Pts',(3.76096461886723,-0.31943490727605,9.66723501569675));
#56776=CARTESIAN_POINT('Ctrl Pts',(3.74319802800101,-0.158333333332783,
9.63761237718672));
#56777=CARTESIAN_POINT('Ctrl Pts',(3.75756771109968,0.158333333332785,9.61518494541643));
#56778=CARTESIAN_POINT('Ctrl Pts',(3.78960399643097,0.319434907276058,9.62250093354075));
#56779=CARTESIAN_POINT('Ctrl Pts',(3.8646568548837,0.636309800092997,9.63626820689347));
#56780=CARTESIAN_POINT('Ctrl Pts',(3.924559082504,0.794772683998081,9.65734774837526));
#56781=CARTESIAN_POINT('Ctrl Pts',(4.01902525308205,1.06847604194162,9.6779119389689));
#56782=CARTESIAN_POINT('Ctrl Pts',(4.06167184187158,1.18514270860809,9.68588862628807));
#56783=CARTESIAN_POINT('Ctrl Pts',(4.10607411452398,1.29999999999612,9.69294052479679));
#56784=CARTESIAN_POINT('Ctrl Pts',(3.99403512297787,-1.29999999999721,9.89169252950751));
#56785=CARTESIAN_POINT('Ctrl Pts',(3.9606540177041,-1.18514270860881,9.87137520140306));
#56786=CARTESIAN_POINT('Ctrl Pts',(3.92930683107614,-1.06847604194195,9.84871399883852));
#56787=CARTESIAN_POINT('Ctrl Pts',(3.86158731793836,-0.794772683998027,
9.79094726866334));
#56788=CARTESIAN_POINT('Ctrl Pts',(3.81817773071631,-0.636309800092936,
9.74398831071881));
#56789=CARTESIAN_POINT('Ctrl Pts',(3.77313731734351,-0.319434907276024,
9.6838093055602));
#56790=CARTESIAN_POINT('Ctrl Pts',(3.75513147909687,-0.15833333333277,9.65314579603697));
#56791=CARTESIAN_POINT('Ctrl Pts',(3.76958198214413,0.158333333332772,9.63061650050148));
#56792=CARTESIAN_POINT('Ctrl Pts',(3.80185442000686,0.319434907276032,9.63895252512564));
#56793=CARTESIAN_POINT('Ctrl Pts',(3.87670406566407,0.636309800092946,9.65282990370601));
#56794=CARTESIAN_POINT('Ctrl Pts',(3.93688123514687,0.794772683998017,9.67432964771585));
#56795=CARTESIAN_POINT('Ctrl Pts',(4.0295951989573,1.06847604194153,9.69271824339368));
#56796=CARTESIAN_POINT('Ctrl Pts',(4.07106409330812,1.185142708608,9.69918153666264));
#56797=CARTESIAN_POINT('Ctrl Pts',(4.11386944246713,1.29999999999602,9.70414838149625));
#56798=CARTESIAN_POINT('Ctrl Pts',(3.99548245121749,-1.2999999999972,9.89448355290227));
#56799=CARTESIAN_POINT('Ctrl Pts',(3.96245342304708,-1.1851427086088,9.87463893210296));
#56800=CARTESIAN_POINT('Ctrl Pts',(3.93138095929411,-1.06847604194195,9.85230465165239));
#56801=CARTESIAN_POINT('Ctrl Pts',(3.8641174072135,-0.794772683998026,9.79495638400513));
#56802=CARTESIAN_POINT('Ctrl Pts',(3.82076935379783,-0.636309800092935,
9.7477713080824));
#56803=CARTESIAN_POINT('Ctrl Pts',(3.77584147348526,-0.319434907276024,
9.68749407186112));
#56804=CARTESIAN_POINT('Ctrl Pts',(3.75775134690968,-0.15833333333277,9.65663560839093));
#56805=CARTESIAN_POINT('Ctrl Pts',(3.77220906636897,0.158333333332772,9.63409644252598));
#56806=CARTESIAN_POINT('Ctrl Pts',(3.8045508416485,0.319434907276032,9.64263942631028));
#56807=CARTESIAN_POINT('Ctrl Pts',(3.87934780680038,0.636309800092945,9.65655037189766));
#56808=CARTESIAN_POINT('Ctrl Pts',(3.93956300403386,0.794772683998015,9.67817041277619));
#56809=CARTESIAN_POINT('Ctrl Pts',(4.03187898273703,1.06847604194153,9.69608662897828));
#56810=CARTESIAN_POINT('Ctrl Pts',(4.07308576997995,1.18514270860799,9.70221472645836));
#56811=CARTESIAN_POINT('Ctrl Pts',(4.11553917792927,1.29999999999602,9.70671565528587));
#56812=CARTESIAN_POINT('Ctrl Pts',(3.99797166780253,-1.29999999999717,9.89941379417368));
#56813=CARTESIAN_POINT('Ctrl Pts',(3.96557500474023,-1.18514270860878,9.88037837286466));
#56814=CARTESIAN_POINT('Ctrl Pts',(3.93499238939632,-1.06847604194192,9.85860615648363));
#56815=CARTESIAN_POINT('Ctrl Pts',(3.86853124304929,-0.794772683998007,
9.80198543701632));
#56816=CARTESIAN_POINT('Ctrl Pts',(3.82525865750305,-0.636309800092921,
9.75444054534181));
#56817=CARTESIAN_POINT('Ctrl Pts',(3.78052866433776,-0.319434907276017,
9.6939911087952));
#56818=CARTESIAN_POINT('Ctrl Pts',(3.7623170733993,-0.158333333332766,9.66276336039861));
#56819=CARTESIAN_POINT('Ctrl Pts',(3.77679422781962,0.158333333332768,9.64020027376793));
#56820=CARTESIAN_POINT('Ctrl Pts',(3.80924760100915,0.319434907276024,9.64911659737234));
#56821=CARTESIAN_POINT('Ctrl Pts',(3.88394595150036,0.63630980009293,9.66309403400363));
#56822=CARTESIAN_POINT('Ctrl Pts',(3.9442291986607,0.794772683997997,9.68492192453384));
#56823=CARTESIAN_POINT('Ctrl Pts',(4.03583458505829,1.06847604194151,9.7020296605304));
#56824=CARTESIAN_POINT('Ctrl Pts',(4.07657380738917,1.18514270860797,9.70758279402453));
#56825=CARTESIAN_POINT('Ctrl Pts',(4.11839967459347,1.29999999999599,9.71128375600398));
#56826=CARTESIAN_POINT('Ctrl Pts',(4.00320446632834,-1.2999999999971,9.90899225940445));
#56827=CARTESIAN_POINT('Ctrl Pts',(3.97182844926294,-1.18514270860871,9.89183616775541));
#56828=CARTESIAN_POINT('Ctrl Pts',(3.94207265564493,-1.06847604194186,9.87135239871074));
#56829=CARTESIAN_POINT('Ctrl Pts',(3.87707386004942,-0.794772683997962,
9.81634319397025));
#56830=CARTESIAN_POINT('Ctrl Pts',(3.83424674884023,-0.636309800092884,
9.76777093058625));
#56831=CARTESIAN_POINT('Ctrl Pts',(3.78993922064094,-0.319434907275998,
9.70695278349702));
#56832=CARTESIAN_POINT('Ctrl Pts',(3.77129151705819,-0.158333333332757,
9.67520013979713));
#56833=CARTESIAN_POINT('Ctrl Pts',(3.78589928806803,0.158333333332759,9.65247549954131));
#56834=CARTESIAN_POINT('Ctrl Pts',(3.81890980236496,0.319434907276005,9.6617440984977));
#56835=CARTESIAN_POINT('Ctrl Pts',(3.89347127480144,0.636309800092893,9.67578371387904));
#56836=CARTESIAN_POINT('Ctrl Pts',(3.95361913043491,0.794772683997952,9.69835270852644));
#56837=CARTESIAN_POINT('Ctrl Pts',(4.0437826366301,1.06847604194144,9.71386634146029));
#56838=CARTESIAN_POINT('Ctrl Pts',(4.08361996487777,1.1851427086079,9.71822828741913));
#56839=CARTESIAN_POINT('Ctrl Pts',(4.12426618042834,1.29999999999591,9.72023690247649));
#56840=CARTESIAN_POINT('Ctrl Pts',(4.01323645802655,-1.29999999999633,9.92858671349471));
#56841=CARTESIAN_POINT('Ctrl Pts',(3.98384646628841,-1.18514270860801,9.91523289095328));
#56842=CARTESIAN_POINT('Ctrl Pts',(3.95563047679174,-1.06847604194123,9.8974408084055));
#56843=CARTESIAN_POINT('Ctrl Pts',(3.89315807650135,-0.794772683997495,
9.84608426994085));
#56844=CARTESIAN_POINT('Ctrl Pts',(3.85023033533171,-0.63630980009251,9.79657078654875));
#56845=CARTESIAN_POINT('Ctrl Pts',(3.80723555286186,-0.319434907275811,
9.73450522600868));
#56846=CARTESIAN_POINT('Ctrl Pts',(3.78939487367443,-0.158333333332664,
9.69984558077839));
#56847=CARTESIAN_POINT('Ctrl Pts',(3.80497460358648,0.158333333332666,9.6760204528219));
#56848=CARTESIAN_POINT('Ctrl Pts',(3.83867077453724,0.319434907275819,9.686480371128));
#56849=CARTESIAN_POINT('Ctrl Pts',(3.91283863802461,0.636309800092521,9.70077889261199));
#56850=CARTESIAN_POINT('Ctrl Pts',(3.97250164099645,0.794772683997486,9.72506305942813));
#56851=CARTESIAN_POINT('Ctrl Pts',(4.0598594729798,1.06847604194082,9.73728377547029));
#56852=CARTESIAN_POINT('Ctrl Pts',(4.09799742777746,1.1851427086072,9.73913642114516));
#56853=CARTESIAN_POINT('Ctrl Pts',(4.13645936883385,1.29999999999515,9.7375518173424));
#56854=CARTESIAN_POINT('Ctrl Pts',(4.02401382537848,-1.29999999999515,9.9473557434411));
#56855=CARTESIAN_POINT('Ctrl Pts',(3.99658515229895,-1.18514270860693,9.93781974419851));
#56856=CARTESIAN_POINT('Ctrl Pts',(3.96992373723207,-1.06847604194025,9.92269524025967));
#56857=CARTESIAN_POINT('Ctrl Pts',(3.91010305432856,-0.794772683996766,
9.87484404668957));
#56858=CARTESIAN_POINT('Ctrl Pts',(3.86776283598717,-0.636309800091926,
9.82362940522103));
#56859=CARTESIAN_POINT('Ctrl Pts',(3.82540760025208,-0.319434907275517,
9.76107975393186));
#56860=CARTESIAN_POINT('Ctrl Pts',(3.80694211371491,-0.158333333332519,
9.72512312909289));
#56861=CARTESIAN_POINT('Ctrl Pts',(3.82234834042072,0.158333333332521,9.70149098605119));
#56862=CARTESIAN_POINT('Ctrl Pts',(3.85606966362876,0.319434907275526,9.71389736476582));
#56863=CARTESIAN_POINT('Ctrl Pts',(3.93011260755125,0.636309800091936,9.72814322412588));
#56864=CARTESIAN_POINT('Ctrl Pts',(3.99101408165235,0.794772683996756,9.75215086712417));
#56865=CARTESIAN_POINT('Ctrl Pts',(4.07584817888741,1.06847604193984,9.76079341287856));
#56866=CARTESIAN_POINT('Ctrl Pts',(4.11210970515826,1.18514270860611,9.76036799993197));
#56867=CARTESIAN_POINT('Ctrl Pts',(4.14791122041998,1.29999999999395,9.75577613621959));
#56868=CARTESIAN_POINT('Ctrl Pts',(4.03457043750772,-1.29999999999448,9.97065174313936));
#56869=CARTESIAN_POINT('Ctrl Pts',(4.00948073920188,-1.18514270860633,9.96535096285632));
#56870=CARTESIAN_POINT('Ctrl Pts',(3.98464701546341,-1.06847604193971,9.95320760337727));
#56871=CARTESIAN_POINT('Ctrl Pts',(3.92786749811646,-0.794772683996364,
9.90934628691403));
#56872=CARTESIAN_POINT('Ctrl Pts',(3.88575480123707,-0.636309800091603,
9.85670437769421));
#56873=CARTESIAN_POINT('Ctrl Pts',(3.84455648997016,-0.319434907275354,
9.79316184315602));
#56874=CARTESIAN_POINT('Ctrl Pts',(3.82602794471147,-0.158333333332438,
9.75503933008314));
#56875=CARTESIAN_POINT('Ctrl Pts',(3.842391775896,0.15833333333244,9.7303546939524));
#56876=CARTESIAN_POINT('Ctrl Pts',(3.87770341865184,0.319434907275365,9.74321118973647));
#56877=CARTESIAN_POINT('Ctrl Pts',(3.95137966051613,0.636309800091614,9.75765712938725));
#56878=CARTESIAN_POINT('Ctrl Pts',(4.01111397319714,0.794772683996351,9.78428068645223));
#56879=CARTESIAN_POINT('Ctrl Pts',(4.09274234391537,1.06847604193929,9.78918670955597));
#56880=CARTESIAN_POINT('Ctrl Pts',(4.12717304692835,1.18514270860551,9.78579317965512));
#56881=CARTESIAN_POINT('Ctrl Pts',(4.16070055589961,1.29999999999329,9.77688248423786));
#56882=CARTESIAN_POINT('Ctrl Pts',(4.04634921388171,-1.29999999999287,9.99261507851378));
#56883=CARTESIAN_POINT('Ctrl Pts',(4.02330211125708,-1.18514270860486,9.99186037780706));
#56884=CARTESIAN_POINT('Ctrl Pts',(4.00010340364208,-1.06847604193839,9.98289979062435));
#56885=CARTESIAN_POINT('Ctrl Pts',(3.94615951030976,-0.794772683995377,
9.94324180233157));
#56886=CARTESIAN_POINT('Ctrl Pts',(3.90486148846194,-0.636309800090813,
9.88853779748812));
#56887=CARTESIAN_POINT('Ctrl Pts',(3.86425783077975,-0.319434907274957,
9.8246199928221));
#56888=CARTESIAN_POINT('Ctrl Pts',(3.84472846232997,-0.158333333332242,
9.78535172278455));
#56889=CARTESIAN_POINT('Ctrl Pts',(3.86088111472339,0.158333333332244,9.76091246291785));
#56890=CARTESIAN_POINT('Ctrl Pts',(3.89644952316345,0.319434907274968,9.77572751296444));
#56891=CARTESIAN_POINT('Ctrl Pts',(3.97018639102631,0.636309800090824,9.78989274073506));
#56892=CARTESIAN_POINT('Ctrl Pts',(4.03129986387343,0.794772683995363,9.81625797980789));
#56893=CARTESIAN_POINT('Ctrl Pts',(4.11043152187304,1.06847604193797,9.81664722734172));
#56894=CARTESIAN_POINT('Ctrl Pts',(4.1429577847685,1.18514270860404,9.81038162838847));
#56895=CARTESIAN_POINT('Ctrl Pts',(4.17375714792826,1.29999999999168,9.79768193964762));
#56896=CARTESIAN_POINT('Ctrl Pts',(4.05635056619991,-1.29999999998975,10.0142690078584));
#56897=CARTESIAN_POINT('Ctrl Pts',(4.03544628027288,-1.18514270860201,10.0175057276255));
#56898=CARTESIAN_POINT('Ctrl Pts',(4.01384845430562,-1.06847604193582,10.0114363617991));
#56899=CARTESIAN_POINT('Ctrl Pts',(3.96235093945595,-0.79477268399347,9.97591599317089));
#56900=CARTESIAN_POINT('Ctrl Pts',(3.92055436487356,-0.636309800089288,
9.92062666986226));
#56901=CARTESIAN_POINT('Ctrl Pts',(3.8808985634387,-0.319434907274192,9.85594791688383));
#56902=CARTESIAN_POINT('Ctrl Pts',(3.86189554664143,-0.158333333331862,
9.81407600400371));
#56903=CARTESIAN_POINT('Ctrl Pts',(3.87899850634942,0.158333333331864,9.78863250623016));
#56904=CARTESIAN_POINT('Ctrl Pts',(3.91559292543677,0.3194349072742,9.80438067216241));
#56905=CARTESIAN_POINT('Ctrl Pts',(3.98909130197214,0.636309800089297,9.81861847075731));
#56906=CARTESIAN_POINT('Ctrl Pts',(4.04965588928553,0.794772683993459,9.84680488231586));
#56907=CARTESIAN_POINT('Ctrl Pts',(4.12603725524005,1.06847604193541,9.84343121678803));
#56908=CARTESIAN_POINT('Ctrl Pts',(4.15689741615992,1.1851427086012,9.83434719176427));
#56909=CARTESIAN_POINT('Ctrl Pts',(4.18555507488646,1.29999999998857,9.81763947651711));
#56910=CARTESIAN_POINT('Ctrl Pts',(4.06273679756711,-1.29999999998941,10.0279056870545));
#56911=CARTESIAN_POINT('Ctrl Pts',(4.04305412357837,-1.1851427086017,10.0338073315529));
#56912=CARTESIAN_POINT('Ctrl Pts',(4.02240682746204,-1.06847604193554,10.0296324218589));
#56913=CARTESIAN_POINT('Ctrl Pts',(3.97247897286925,-0.794772683993263,
9.9967086892858));
#56914=CARTESIAN_POINT('Ctrl Pts',(3.93074708407459,-0.636309800089121,
9.94065147793032));
#56915=CARTESIAN_POINT('Ctrl Pts',(3.89171929918422,-0.319434907274109,
9.875472533128));
#56916=CARTESIAN_POINT('Ctrl Pts',(3.87294279440502,-0.158333333331821,
9.83207404610695));
#56917=CARTESIAN_POINT('Ctrl Pts',(3.89023914234746,0.158333333331822,9.80644326801721));
#56918=CARTESIAN_POINT('Ctrl Pts',(3.9268624976559,0.319434907274116,9.82345867854917));
#56919=CARTESIAN_POINT('Ctrl Pts',(4.00000036379485,0.63630980008913,9.83796195153213));
#56920=CARTESIAN_POINT('Ctrl Pts',(4.06050936822068,0.794772683993251,9.86696403121066));
#56921=CARTESIAN_POINT('Ctrl Pts',(4.13543227900064,1.06847604193513,9.86089790353117));
#56922=CARTESIAN_POINT('Ctrl Pts',(4.16538632929968,1.18514270860089,9.84987076073));
#56923=CARTESIAN_POINT('Ctrl Pts',(4.19286307798853,1.29999999998823,9.83044227702793));
#56924=CARTESIAN_POINT('Ctrl Pts',(4.06407190888843,-1.29999999998939,10.030785444544));
#56925=CARTESIAN_POINT('Ctrl Pts',(4.0446499038056,-1.18514270860168,10.0372436682821));
#56926=CARTESIAN_POINT('Ctrl Pts',(4.02420436638832,-1.06847604193552,10.0334654494754));
#56927=CARTESIAN_POINT('Ctrl Pts',(3.97460652038925,-0.79477268399325,10.0010887781306));
#56928=CARTESIAN_POINT('Ctrl Pts',(3.93288084414568,-0.636309800089111,
9.94487936290763));
#56929=CARTESIAN_POINT('Ctrl Pts',(3.89398020931323,-0.319434907274104,
9.87960085633521));
#56930=CARTESIAN_POINT('Ctrl Pts',(3.87523649645876,-0.158333333331818,
9.83589642165554));
#56931=CARTESIAN_POINT('Ctrl Pts',(3.89259805848843,0.15833333333182,9.81019947911735));
#56932=CARTESIAN_POINT('Ctrl Pts',(3.92927976210183,0.319434907274111,9.8274250670269));
#56933=CARTESIAN_POINT('Ctrl Pts',(4.00237050489757,0.636309800089121,9.84195343451171));
#56934=CARTESIAN_POINT('Ctrl Pts',(4.06286845920188,0.794772683993239,9.8711272305367));
#56935=CARTESIAN_POINT('Ctrl Pts',(4.13746609783607,1.06847604193511,9.86451433880063));
#56936=CARTESIAN_POINT('Ctrl Pts',(4.16721451160574,1.18514270860087,9.85309427136058));
#56937=CARTESIAN_POINT('Ctrl Pts',(4.19442078549526,1.2999999999882,9.83311661228122));
#56938=CARTESIAN_POINT('Ctrl Pts',(4.06539413056257,-1.29999999998936,10.0336772368117));
#56939=CARTESIAN_POINT('Ctrl Pts',(4.04622008422138,-1.18514270860165,10.0407041704229));
#56940=CARTESIAN_POINT('Ctrl Pts',(4.02597047400536,-1.0684760419355,10.0373281368284));
#56941=CARTESIAN_POINT('Ctrl Pts',(3.97670505576914,-0.79477268399323,10.0054958885001));
#56942=CARTESIAN_POINT('Ctrl Pts',(3.93502274247802,-0.636309800089095,
9.94909767065479));
#56943=CARTESIAN_POINT('Ctrl Pts',(3.89625125716468,-0.319434907274095,
9.88371848291633));
#56944=CARTESIAN_POINT('Ctrl Pts',(3.8775116970533,-0.158333333331814,9.83973775688691));
#56945=CARTESIAN_POINT('Ctrl Pts',(3.89493180960951,0.158333333331816,9.81398187906456));
#56946=CARTESIAN_POINT('Ctrl Pts',(3.93167968973624,0.319434907274104,9.83140992297885));
#56947=CARTESIAN_POINT('Ctrl Pts',(4.00473655379493,0.636309800089104,9.84594927505052));
#56948=CARTESIAN_POINT('Ctrl Pts',(4.06524505505404,0.794772683993218,9.87527100401899));
#56949=CARTESIAN_POINT('Ctrl Pts',(4.13951924770019,1.06847604193508,9.86810947420546));
#56950=CARTESIAN_POINT('Ctrl Pts',(4.16905771469347,1.18514270860084,9.85630127118908));
#56951=CARTESIAN_POINT('Ctrl Pts',(4.19598410281357,1.29999999998817,9.83578482605177));
#56952=CARTESIAN_POINT('Ctrl Pts',(4.06702106849627,-1.29999999998931,10.0373163253182));
#56953=CARTESIAN_POINT('Ctrl Pts',(4.04813576014217,-1.18514270860161,10.0450740546847));
#56954=CARTESIAN_POINT('Ctrl Pts',(4.02812092299354,-1.06847604193546,10.0422101886781));
#56955=CARTESIAN_POINT('Ctrl Pts',(3.97927320774905,-0.7947726839932,10.0110560751343));
#56956=CARTESIAN_POINT('Ctrl Pts',(3.93770348720174,-0.636309800089071,
9.95436547522951));
#56957=CARTESIAN_POINT('Ctrl Pts',(3.89909560486339,-0.319434907274084,
9.88885990982302));
#56958=CARTESIAN_POINT('Ctrl Pts',(3.88030760619111,-0.158333333331808,
9.84458913724083));
#56959=CARTESIAN_POINT('Ctrl Pts',(3.89780562564834,0.15833333333181,9.81875431996012));
#56960=CARTESIAN_POINT('Ctrl Pts',(3.93467978356113,0.319434907274091,9.83638947813788));
#56961=CARTESIAN_POINT('Ctrl Pts',(4.00773187324364,0.63630980008908,9.85090254699385));
#56962=CARTESIAN_POINT('Ctrl Pts',(4.0682867679093,0.794772683993188,9.88037321740751));
#56963=CARTESIAN_POINT('Ctrl Pts',(4.14214844183579,1.06847604193504,9.87253512493884));
#56964=CARTESIAN_POINT('Ctrl Pts',(4.17140894963151,1.1851427086008,9.86025872487337));
#56965=CARTESIAN_POINT('Ctrl Pts',(4.1979579834249,1.29999999998812,9.83909874454217));
#56966=CARTESIAN_POINT('Ctrl Pts',(4.06893477246844,-1.29999999998919,10.0417192296828));
#56967=CARTESIAN_POINT('Ctrl Pts',(4.05035550228226,-1.1851427086015,10.0503926853874));
#56968=CARTESIAN_POINT('Ctrl Pts',(4.03060230955086,-1.06847604193536,10.0481625746812));
#56969=CARTESIAN_POINT('Ctrl Pts',(3.98225648680696,-0.794772683993127,
10.0178211531579));
#56970=CARTESIAN_POINT('Ctrl Pts',(3.94092454857736,-0.636309800089012,
9.96067906367977));
#56971=CARTESIAN_POINT('Ctrl Pts',(3.90251876080255,-0.319434907274054,
9.89501868530541));
#56972=CARTESIAN_POINT('Ctrl Pts',(3.88359133101194,-0.158333333331793,
9.85048421334946));
#56973=CARTESIAN_POINT('Ctrl Pts',(3.90117604894202,0.158333333331795,9.82456207766625));
#56974=CARTESIAN_POINT('Ctrl Pts',(3.93824360631013,0.319434907274062,9.8424022812568));
#56975=CARTESIAN_POINT('Ctrl Pts',(4.01133686890583,0.636309800089021,9.85683391437836));
#56976=CARTESIAN_POINT('Ctrl Pts',(4.07200338624086,0.794772683993115,9.88642225662819));
#56977=CARTESIAN_POINT('Ctrl Pts',(4.14536995439803,1.06847604193494,9.87777292559078));
#56978=CARTESIAN_POINT('Ctrl Pts',(4.1742813560123,1.18514270860069,9.86495189325206));
#56979=CARTESIAN_POINT('Ctrl Pts',(4.20034649038486,1.299999999988,9.84305380349143));
#56980=CARTESIAN_POINT('Ctrl Pts',(4.07083807594505,-1.29999999998909,10.0461309059185));
#56981=CARTESIAN_POINT('Ctrl Pts',(4.05255207824646,-1.18514270860141,10.055732233939));
#56982=CARTESIAN_POINT('Ctrl Pts',(4.03305249272199,-1.06847604193528,10.054143531469));
#56983=CARTESIAN_POINT('Ctrl Pts',(3.98520091862669,-0.794772683993069,
10.0246221019535));
#56984=CARTESIAN_POINT('Ctrl Pts',(3.94412315433243,-0.636309800088966,
9.9670123053312));
#56985=CARTESIAN_POINT('Ctrl Pts',(3.90591806478903,-0.319434907274031,
9.90119978391372));
#56986=CARTESIAN_POINT('Ctrl Pts',(3.88683852260301,-0.158333333331782,
9.8564163676154));
#56987=CARTESIAN_POINT('Ctrl Pts',(3.90450748901525,0.158333333331784,9.83041016796613));
#56988=CARTESIAN_POINT('Ctrl Pts',(3.94177224561851,0.319434907274039,9.84845092754632));
#56989=CARTESIAN_POINT('Ctrl Pts',(4.01491618752075,0.636309800088976,9.86279080280935));
#56990=CARTESIAN_POINT('Ctrl Pts',(4.0757057334192,0.794772683993058,9.89248424162781));
#56991=CARTESIAN_POINT('Ctrl Pts',(4.14858696511739,1.06847604193487,9.88301352662142));
#56992=CARTESIAN_POINT('Ctrl Pts',(4.17715248654312,1.1851427086006,9.86964469808969));
#56993=CARTESIAN_POINT('Ctrl Pts',(4.20273594470819,1.29999999998791,9.84700656262791));
#56994=CARTESIAN_POINT('Ctrl Pts',(4.07228048230189,-1.29999999998897,10.0494243716724));
#56995=CARTESIAN_POINT('Ctrl Pts',(4.05422942402522,-1.1851427086013,10.0597069074288));
#56996=CARTESIAN_POINT('Ctrl Pts',(4.03492509698501,-1.06847604193518,10.0585942639093));
#56997=CARTESIAN_POINT('Ctrl Pts',(3.98743293814549,-0.794772683992996,
10.0296986910705));
#56998=CARTESIAN_POINT('Ctrl Pts',(3.94648567623039,-0.636309800088908,
9.97179668357852));
#56999=CARTESIAN_POINT('Ctrl Pts',(3.90842363585003,-0.319434907274002,
9.90587732661702));
#57000=CARTESIAN_POINT('Ctrl Pts',(3.88927784857038,-0.158333333331767,
9.86086012943157));
#57001=CARTESIAN_POINT('Ctrl Pts',(3.90700922326024,0.158333333331769,9.83479267464078));
#57002=CARTESIAN_POINT('Ctrl Pts',(3.94438905042288,0.319434907274009,9.85301735823453));
#57003=CARTESIAN_POINT('Ctrl Pts',(4.01754473153985,0.636309800088917,9.86731607927766));
#57004=CARTESIAN_POINT('Ctrl Pts',(4.0783981912992,0.794772683992985,9.8971189187593));
#57005=CARTESIAN_POINT('Ctrl Pts',(4.15093233607749,1.06847604193477,9.88701418427292));
#57006=CARTESIAN_POINT('Ctrl Pts',(4.17925759836599,1.18514270860049,9.87321409232173));
#57007=CARTESIAN_POINT('Ctrl Pts',(4.2045107793234,1.29999999998779,9.84998787356118));
#57008=CARTESIAN_POINT('Ctrl Pts',(4.07325465779156,-1.29999999998895,10.0516075489123));
#57009=CARTESIAN_POINT('Ctrl Pts',(4.05537342858916,-1.18514270860128,10.0623313519078));
#57010=CARTESIAN_POINT('Ctrl Pts',(4.03620456978458,-1.06847604193516,10.0615309202005));
#57011=CARTESIAN_POINT('Ctrl Pts',(3.98894598925863,-0.794772683992982,
10.0330584752522));
#57012=CARTESIAN_POINT('Ctrl Pts',(3.94804077865574,-0.636309800088896,
9.97500564443789));
#57013=CARTESIAN_POINT('Ctrl Pts',(3.91006897550654,-0.319434907273996,
9.9090197877421));
#57014=CARTESIAN_POINT('Ctrl Pts',(3.89091373212821,-0.158333333331765,
9.86381201354059));
#57015=CARTESIAN_POINT('Ctrl Pts',(3.90868748732497,0.158333333331766,9.8377033636354));
#57016=CARTESIAN_POINT('Ctrl Pts',(3.94612284879179,0.319434907274004,9.85607234905735));
#57017=CARTESIAN_POINT('Ctrl Pts',(4.01926708677286,0.636309800088906,9.87036400609676));
#57018=CARTESIAN_POINT('Ctrl Pts',(4.08014064074479,0.794772683992971,9.9002641596514));
#57019=CARTESIAN_POINT('Ctrl Pts',(4.15245205032798,1.06847604193475,9.88972747831268));
#57020=CARTESIAN_POINT('Ctrl Pts',(4.18062907000966,1.18514270860047,9.87562707692026));
#57021=CARTESIAN_POINT('Ctrl Pts',(4.20568217956622,1.29999999998777,9.85198721306445));
#57022=CARTESIAN_POINT('Ctrl Pts',(4.07390722870856,-1.29999999998894,10.0530598988483));
#57023=CARTESIAN_POINT('Ctrl Pts',(4.05614258391025,-1.18514270860127,10.0640745886785));
#57024=CARTESIAN_POINT('Ctrl Pts',(4.03706538461292,-1.06847604193515,10.0634809773882));
#57025=CARTESIAN_POINT('Ctrl Pts',(3.98996097438718,-0.794772683992973,
10.0352921187352));
#57026=CARTESIAN_POINT('Ctrl Pts',(3.94907237020012,-0.636309800088889,
9.97714992134904));
#57027=CARTESIAN_POINT('Ctrl Pts',(3.91115931189588,-0.319434907273992,
9.91112104424304));
#57028=CARTESIAN_POINT('Ctrl Pts',(3.89200639945563,-0.158333333331763,
9.86577758659279));
#57029=CARTESIAN_POINT('Ctrl Pts',(3.9098085767008,0.158333333331765,9.8396414179453));
#57030=CARTESIAN_POINT('Ctrl Pts',(3.94727573788883,0.319434907274,9.85811195946995));
#57031=CARTESIAN_POINT('Ctrl Pts',(4.02040749666177,0.636309800088899,9.87240404447289));
#57032=CARTESIAN_POINT('Ctrl Pts',(4.08128868412945,0.794772683992962,9.90237530578483));
#57033=CARTESIAN_POINT('Ctrl Pts',(4.15345377064241,1.06847604193474,9.89154835775589));
#57034=CARTESIAN_POINT('Ctrl Pts',(4.18153497571546,1.18514270860046,9.87724452862485));
#57035=CARTESIAN_POINT('Ctrl Pts',(4.20645979389006,1.29999999998775,9.85332345498654));
#57036=CARTESIAN_POINT('Ctrl Pts',(4.07472883611629,-1.2999999999889,10.0548694806607));
#57037=CARTESIAN_POINT('Ctrl Pts',(4.05711645448729,-1.18514270860124,10.066241372499));
#57038=CARTESIAN_POINT('Ctrl Pts',(4.03815646541594,-1.06847604193512,10.0659036912195));
#57039=CARTESIAN_POINT('Ctrl Pts',(3.99124185494869,-0.794772683992953,
10.0380721235173));
#57040=CARTESIAN_POINT('Ctrl Pts',(3.95035207494585,-0.636309800088874,
9.9798396914538));
#57041=CARTESIAN_POINT('Ctrl Pts',(3.9125096217793,-0.319434907273985,9.91375966696656));
#57042=CARTESIAN_POINT('Ctrl Pts',(3.89337589264243,-0.158333333331759,
9.86823033469163));
#57043=CARTESIAN_POINT('Ctrl Pts',(3.91121402898208,0.158333333331761,9.84205954147312));
#57044=CARTESIAN_POINT('Ctrl Pts',(3.94871139904287,0.319434907273992,9.86066680643706));
#57045=CARTESIAN_POINT('Ctrl Pts',(4.02181843654429,0.636309800088883,9.87496910073066));
#57046=CARTESIAN_POINT('Ctrl Pts',(4.08269805463338,0.794772683992942,9.90504125970458));
#57047=CARTESIAN_POINT('Ctrl Pts',(4.15468415069764,1.06847604193471,9.89384734872794));
#57048=CARTESIAN_POINT('Ctrl Pts',(4.18265120271854,1.18514270860043,9.87928324884646));
#57049=CARTESIAN_POINT('Ctrl Pts',(4.20742519312184,1.29999999998772,9.85500047836999));
#57050=CARTESIAN_POINT('Ctrl Pts',(4.07547411574327,-1.29999999998887,10.0564922662393));
#57051=CARTESIAN_POINT('Ctrl Pts',(4.05800529143892,-1.18514270860121,10.0681792184617));
#57052=CARTESIAN_POINT('Ctrl Pts',(4.03915337222251,-1.0684760419351,10.0680693180286));
#57053=CARTESIAN_POINT('Ctrl Pts',(3.99240644158517,-0.794772683992932,
10.0405623364562));
#57054=CARTESIAN_POINT('Ctrl Pts',(3.95149348925175,-0.636309800088857,
9.98227038205354));
#57055=CARTESIAN_POINT('Ctrl Pts',(3.91371116847997,-0.319434907273976,
9.91614756042613));
#57056=CARTESIAN_POINT('Ctrl Pts',(3.89461012291728,-0.158333333331755,
9.87043553006687));
#57057=CARTESIAN_POINT('Ctrl Pts',(3.91248106890848,0.158333333331757,9.84423334416848));
#57058=CARTESIAN_POINT('Ctrl Pts',(3.94999712337104,0.319434907273984,9.86297239204567));
#57059=CARTESIAN_POINT('Ctrl Pts',(4.02307305740497,0.636309800088866,9.87729330475985));
#57060=CARTESIAN_POINT('Ctrl Pts',(4.08393969766434,0.794772683992921,9.90746875231371));
#57061=CARTESIAN_POINT('Ctrl Pts',(4.15576841570156,1.06847604193468,9.89594071535657));
#57062=CARTESIAN_POINT('Ctrl Pts',(4.18363827625216,1.1851427086004,9.88113649555721));
#57063=CARTESIAN_POINT('Ctrl Pts',(4.20828600683132,1.29999999998768,9.85651811600137));
#57064=CARTESIAN_POINT('Ctrl Pts',(4.07597260778046,-1.29999999998886,10.057572446527));
#57065=CARTESIAN_POINT('Ctrl Pts',(4.0586012438042,-1.1851427086012,10.0694676935615));
#57066=CARTESIAN_POINT('Ctrl Pts',(4.03982201553618,-1.06847604193509,10.0695089994242));
#57067=CARTESIAN_POINT('Ctrl Pts',(3.99318579330915,-0.794772683992927,
10.0422194487507));
#57068=CARTESIAN_POINT('Ctrl Pts',(3.95225110097318,-0.636309800088852,
9.98389400970228));
#57069=CARTESIAN_POINT('Ctrl Pts',(3.91450758576179,-0.319434907273974,
9.91774390726409));
#57070=CARTESIAN_POINT('Ctrl Pts',(3.89543222585983,-0.158333333331754,
9.87190619314399));
#57071=CARTESIAN_POINT('Ctrl Pts',(3.91332514424889,0.158333333331756,9.84568304911986));
#57072=CARTESIAN_POINT('Ctrl Pts',(3.95085174404416,0.319434907273981,9.86451192091105));
#57073=CARTESIAN_POINT('Ctrl Pts',(4.0239045849775,0.636309800088861,9.87884777797579));
#57074=CARTESIAN_POINT('Ctrl Pts',(4.08475912371384,0.794772683992915,9.90909579798807));
#57075=CARTESIAN_POINT('Ctrl Pts',(4.1564839138414,1.06847604193467,9.89734401763171));
#57076=CARTESIAN_POINT('Ctrl Pts',(4.18429053005257,1.18514270860039,9.8823780981469));
#57077=CARTESIAN_POINT('Ctrl Pts',(4.20885675849407,1.29999999998768,9.85753316944717));
#57078=CARTESIAN_POINT('Ctrl Pts',(4.07622210167524,-1.29999999998886,10.0581122784215));
#57079=CARTESIAN_POINT('Ctrl Pts',(4.05889975895958,-1.1851427086012,10.0701113802034));
#57080=CARTESIAN_POINT('Ctrl Pts',(4.04015697781387,-1.06847604193509,10.0702281847756));
#57081=CARTESIAN_POINT('Ctrl Pts',(3.99357590695571,-0.794772683992926,
10.0430475431045));
#57082=CARTESIAN_POINT('Ctrl Pts',(3.95262928543621,-0.636309800088851,
9.984706405372));
#57083=CARTESIAN_POINT('Ctrl Pts',(3.91490488517323,-0.319434907273973,
9.91854294778371));
#57084=CARTESIAN_POINT('Ctrl Pts',(3.89584289171174,-0.158333333331753,
9.87264187569554));
#57085=CARTESIAN_POINT('Ctrl Pts',(3.91374682290024,0.158333333331755,9.84640823972977));
#57086=CARTESIAN_POINT('Ctrl Pts',(3.95127853286302,0.319434907273981,9.86528219251662));
#57087=CARTESIAN_POINT('Ctrl Pts',(4.02431948788694,0.636309800088861,9.87962589094895));
#57088=CARTESIAN_POINT('Ctrl Pts',(4.08516735885034,0.794772683992914,9.90991085607916));
#57089=CARTESIAN_POINT('Ctrl Pts',(4.15684031488721,1.06847604193467,9.89804708400454));
#57090=CARTESIAN_POINT('Ctrl Pts',(4.18461554710164,1.18514270860039,9.88300007185356));
#57091=CARTESIAN_POINT('Ctrl Pts',(4.20914144460686,1.29999999998767,9.85804143488663));
#57092=CARTESIAN_POINT('Ctrl Pts',(4.07643021999955,-1.29999999998885,10.0585619219469));
#57093=CARTESIAN_POINT('Ctrl Pts',(4.05914893020202,-1.18514270860119,10.0706473663804));
#57094=CARTESIAN_POINT('Ctrl Pts',(4.04043658915353,-1.06847604193508,10.0708270173388));
#57095=CARTESIAN_POINT('Ctrl Pts',(3.99390132327006,-0.794772683992922,
10.0437372823191));
#57096=CARTESIAN_POINT('Ctrl Pts',(3.95294397013955,-0.636309800088849,
9.98538384510396));
#57097=CARTESIAN_POINT('Ctrl Pts',(3.91523534848828,-0.319434907273972,
9.91920940614504));
#57098=CARTESIAN_POINT('Ctrl Pts',(3.89618502062803,-0.158333333331753,
9.87325500922776));
#57099=CARTESIAN_POINT('Ctrl Pts',(3.91409812835474,0.158333333331755,9.84701264030445));
#57100=CARTESIAN_POINT('Ctrl Pts',(3.95163379350589,0.31943490727398,9.86592447240053));
#57101=CARTESIAN_POINT('Ctrl Pts',(4.02466453538962,0.636309800088858,9.8802750368039));
#57102=CARTESIAN_POINT('Ctrl Pts',(4.08550645564106,0.794772683992911,9.91059121737707));
#57103=CARTESIAN_POINT('Ctrl Pts',(4.15713636041993,1.06847604193467,9.8986339757222));
#57104=CARTESIAN_POINT('Ctrl Pts',(4.18488564025264,1.18514270860038,9.8835191770097));
#57105=CARTESIAN_POINT('Ctrl Pts',(4.20937826828882,1.29999999998767,9.85846542643763));
#57106=CARTESIAN_POINT('Ctrl Pts',(4.0765759208084,-1.29999999998886,10.0588766470101));
#57107=CARTESIAN_POINT('Ctrl Pts',(4.05932344329039,-1.1851427086012,10.0710224510075));
#57108=CARTESIAN_POINT('Ctrl Pts',(4.04063243052271,-1.06847604193509,10.071246070143));
#57109=CARTESIAN_POINT('Ctrl Pts',(3.99412914770043,-0.794772683992925,
10.0442200430249));
#57110=CARTESIAN_POINT('Ctrl Pts',(3.95316401095664,-0.63630980008885,9.98585826277267));
#57111=CARTESIAN_POINT('Ctrl Pts',(3.91546623180345,-0.319434907273973,
9.91967634285258));
#57112=CARTESIAN_POINT('Ctrl Pts',(3.89642395968892,-0.158333333331753,
9.87368474052135));
#57113=CARTESIAN_POINT('Ctrl Pts',(3.91434351989717,0.158333333331755,9.84743623607467));
#57114=CARTESIAN_POINT('Ctrl Pts',(3.95188221366601,0.319434907273981,9.86637431922968));
#57115=CARTESIAN_POINT('Ctrl Pts',(4.02490582148206,0.63630980008886,9.88072968258797));
#57116=CARTESIAN_POINT('Ctrl Pts',(4.08574333395374,0.794772683992913,9.91106796282547));
#57117=CARTESIAN_POINT('Ctrl Pts',(4.15734306508055,1.06847604193467,9.89904534991704));
#57118=CARTESIAN_POINT('Ctrl Pts',(4.18507419912739,1.18514270860039,9.88388309052645));
#57119=CARTESIAN_POINT('Ctrl Pts',(4.20954359664774,1.29999999998767,9.85876271539161));
#57120=CARTESIAN_POINT('Ctrl Pts',(4.07665927356971,-1.29999999998885,10.0590563943251));
#57121=CARTESIAN_POINT('Ctrl Pts',(4.0594232795469,-1.18514270860119,10.0712366737565));
#57122=CARTESIAN_POINT('Ctrl Pts',(4.04074446090144,-1.06847604193508,10.0714854138474));
#57123=CARTESIAN_POINT('Ctrl Pts',(3.99425943963133,-0.79477268399292,10.0444958104446));
#57124=CARTESIAN_POINT('Ctrl Pts',(3.95328971468093,-0.636309800088847,
9.98612940636483));
#57125=CARTESIAN_POINT('Ctrl Pts',(3.91559824531298,-0.319434907273971,
9.91994309394241));
#57126=CARTESIAN_POINT('Ctrl Pts',(3.89656095268153,-0.158333333331752,
9.87392984326917));
#57127=CARTESIAN_POINT('Ctrl Pts',(3.91448416414649,0.158333333331754,9.84767786770841));
#57128=CARTESIAN_POINT('Ctrl Pts',(3.95202417120306,0.319434907273979,9.86663137801879));
#57129=CARTESIAN_POINT('Ctrl Pts',(4.02504352600686,0.636309800088856,9.88098966516978));
#57130=CARTESIAN_POINT('Ctrl Pts',(4.08587855467762,0.794772683992909,9.91134055056134));
#57131=CARTESIAN_POINT('Ctrl Pts',(4.15746116232731,1.06847604193466,9.89928044564848));
#57132=CARTESIAN_POINT('Ctrl Pts',(4.18518201547413,1.18514270860038,9.88409096295741));
#57133=CARTESIAN_POINT('Ctrl Pts',(4.20963826331322,1.29999999998766,9.8589323701211));
#57134=CARTESIAN_POINT('Ctrl Pts',(4.08202434161241,-1.29999999998988,10.0706609615285));
#57135=CARTESIAN_POINT('Ctrl Pts',(4.06585221433066,-1.18514270860213,10.0850635262272));
#57136=CARTESIAN_POINT('Ctrl Pts',(4.04795985258241,-1.06847604193593,10.0869320838313));
#57137=CARTESIAN_POINT('Ctrl Pts',(4.00265083184004,-0.794772683993552,
10.0622927618923));
#57138=CARTESIAN_POINT('Ctrl Pts',(3.96139094918821,-0.636309800089352,
10.0036217614018));
#57139=CARTESIAN_POINT('Ctrl Pts',(3.92408339830617,-0.319434907274224,
9.93717581140978));
#57140=CARTESIAN_POINT('Ctrl Pts',(3.90531558877303,-0.158333333331878,
9.88981993991924));
#57141=CARTESIAN_POINT('Ctrl Pts',(3.92347994603432,0.15833333333188,9.86333885041616));
#57142=CARTESIAN_POINT('Ctrl Pts',(3.96116781285423,0.319434907274233,9.88322291920571));
#57143=CARTESIAN_POINT('Ctrl Pts',(4.03393554506074,0.636309800089361,9.89774680803204));
#57144=CARTESIAN_POINT('Ctrl Pts',(4.09459577648591,0.794772683993539,9.92892413859132));
#57145=CARTESIAN_POINT('Ctrl Pts',(4.1650575688749,1.06847604193551,9.91446533303684));
#57146=CARTESIAN_POINT('Ctrl Pts',(4.1921052148016,1.18514270860132,9.89753237258154));
#57147=CARTESIAN_POINT('Ctrl Pts',(4.2157002075965,1.2999999999887,9.86992513284393));
#57148=CARTESIAN_POINT('Ctrl Pts',(4.09192286002323,-1.29999999999578,10.0944502050367));
#57149=CARTESIAN_POINT('Ctrl Pts',(4.07727446967434,-1.18514270860751,10.1138220103929));
#57150=CARTESIAN_POINT('Ctrl Pts',(4.06064929695951,-1.06847604194078,10.1191840229114));
#57151=CARTESIAN_POINT('Ctrl Pts',(4.01767505941472,-0.79477268399716,10.0992059203913));
#57152=CARTESIAN_POINT('Ctrl Pts',(3.9771938286849,-0.636309800092241,10.0386265544923));
#57153=CARTESIAN_POINT('Ctrl Pts',(3.94096363261905,-0.319434907275675,
9.97138572994343));
#57154=CARTESIAN_POINT('Ctrl Pts',(3.92206607032949,-0.158333333332597,
9.92205052577164));
#57155=CARTESIAN_POINT('Ctrl Pts',(3.94073450593346,0.158333333332599,9.89509432820567));
#57156=CARTESIAN_POINT('Ctrl Pts',(3.97883278048616,0.319434907275683,9.91670040028087));
#57157=CARTESIAN_POINT('Ctrl Pts',(4.0520050264758,0.63630980009225,9.93060780328429));
#57158=CARTESIAN_POINT('Ctrl Pts',(4.11428870108699,0.794772683997148,9.96133867191485));
#57159=CARTESIAN_POINT('Ctrl Pts',(4.18211124466442,1.06847604194036,9.94259844987382));
#57160=CARTESIAN_POINT('Ctrl Pts',(4.2070799298394,1.1851427086067,9.92301686204623));
#57161=CARTESIAN_POINT('Ctrl Pts',(4.22765943414761,1.2999999999946,9.89196563411893));
#57162=CARTESIAN_POINT('Ctrl Pts',(4.1021184432181,-1.30000000000182,10.1178254069371));
#57163=CARTESIAN_POINT('Ctrl Pts',(4.08911206630516,-1.18514270861302,10.1420166380803));
#57164=CARTESIAN_POINT('Ctrl Pts',(4.07378763145368,-1.06847604194574,10.1508156013653));
#57165=CARTESIAN_POINT('Ctrl Pts',(4.03302994374026,-0.794772684000851,
10.1355837488154));
#57166=CARTESIAN_POINT('Ctrl Pts',(3.99292720807675,-0.636309800095197,
10.073501568554));
#57167=CARTESIAN_POINT('Ctrl Pts',(3.95743985349657,-0.319434907277159,
10.0058026346109));
#57168=CARTESIAN_POINT('Ctrl Pts',(3.93821605201261,-0.158333333333332,
9.95469786326921));
#57169=CARTESIAN_POINT('Ctrl Pts',(3.95736019033645,0.158333333333334,9.92730205443344));
#57170=CARTESIAN_POINT('Ctrl Pts',(3.99657264201183,0.319434907277167,9.94990558494987));
#57171=CARTESIAN_POINT('Ctrl Pts',(4.06933501806659,0.636309800095206,9.964052914227));
#57172=CARTESIAN_POINT('Ctrl Pts',(4.13043955711106,0.79477268400084,9.99727883158207));
#57173=CARTESIAN_POINT('Ctrl Pts',(4.1962791527049,1.06847604194533,9.97354224444612));
#57174=CARTESIAN_POINT('Ctrl Pts',(4.22022222287693,1.18514270861221,9.9501892474666));
#57175=CARTESIAN_POINT('Ctrl Pts',(4.23960884188585,1.30000000000064,9.91375794255148));
#57176=CARTESIAN_POINT('Ctrl Pts',(4.10682630354988,-1.30000000000182,10.1298904394961));
#57177=CARTESIAN_POINT('Ctrl Pts',(4.09477284803666,-1.18514270861302,10.1563511401478));
#57178=CARTESIAN_POINT('Ctrl Pts',(4.08016499765835,-1.06847604194574,10.1667952068529));
#57179=CARTESIAN_POINT('Ctrl Pts',(4.04051677785084,-0.794772684000851,
10.1539214617366));
#57180=CARTESIAN_POINT('Ctrl Pts',(4.00023280952129,-0.636309800095197,
10.0914459396343));
#57181=CARTESIAN_POINT('Ctrl Pts',(3.96518266532825,-0.319434907277159,
10.0234576048956));
#57182=CARTESIAN_POINT('Ctrl Pts',(3.94621238249089,-0.158333333333332,
9.97107548348332));
#57183=CARTESIAN_POINT('Ctrl Pts',(3.96570274858202,0.158333333333334,9.9433620243731));
#57184=CARTESIAN_POINT('Ctrl Pts',(4.00511469268082,0.319434907277167,9.96682083809137));
#57185=CARTESIAN_POINT('Ctrl Pts',(4.07792758948219,0.636309800095206,9.980823226511));
#57186=CARTESIAN_POINT('Ctrl Pts',(4.13939176391744,0.79477268400084,10.0143022156935));
#57187=CARTESIAN_POINT('Ctrl Pts',(4.20407556081207,1.06847604194533,9.98826899902637));
#57188=CARTESIAN_POINT('Ctrl Pts',(4.22718893277723,1.18514270861221,9.96338122303606));
#57189=CARTESIAN_POINT('Ctrl Pts',(4.24541645780274,1.30000000000064,9.92487448592493));
#57190=CARTESIAN_POINT('',(4.17590025661761,1.2,9.85788582275105));
#57191=CARTESIAN_POINT('Ctrl Pts',(4.1759002566176,1.2,9.85788582275105));
#57192=CARTESIAN_POINT('Ctrl Pts',(4.16896082769767,1.2168198732892,9.83746357236339));
#57193=CARTESIAN_POINT('Ctrl Pts',(4.16291248161029,1.23318519494961,9.81637367715788));
#57194=CARTESIAN_POINT('Ctrl Pts',(4.14915525508964,1.26588873502216,9.77666804147682));
#57195=CARTESIAN_POINT('Ctrl Pts',(4.14279328726094,1.28160640282059,9.75708360059621));
#57196=CARTESIAN_POINT('Ctrl Pts',(4.13532454217556,1.29842424618538,9.7371004320105));
#57197=CARTESIAN_POINT('Ctrl Pts',(4.1349729583003,1.29921220855233,9.73616663537405));
#57198=CARTESIAN_POINT('Ctrl Pts',(4.13461958894908,1.29999999999519,9.73523585780992));
#57199=CARTESIAN_POINT('',(4.08975875486489,0.653834841416977,9.98861494773806));
#57200=CARTESIAN_POINT('Ctrl Pts',(4.08975875488793,0.653834841416293,9.98861494775051));
#57201=CARTESIAN_POINT('Ctrl Pts',(4.09893898656859,0.71805776923962,9.97515129873787));
#57202=CARTESIAN_POINT('Ctrl Pts',(4.10629442287966,0.76350939074164,9.96425948435249));
#57203=CARTESIAN_POINT('Ctrl Pts',(4.13517026026942,0.949775842008898,9.92104750271804));
#57204=CARTESIAN_POINT('Ctrl Pts',(4.1507016403391,1.04906307388899,9.89747627742111));
#57205=CARTESIAN_POINT('Ctrl Pts',(4.1759002566176,1.2,9.85788582275105));
#57206=CARTESIAN_POINT('',(4.00955034077163,-0.653834841531101,10.1027583545342));
#57207=CARTESIAN_POINT('Ctrl Pts',(4.00955034077162,-0.653834841531098,
10.1027583545342));
#57208=CARTESIAN_POINT('Ctrl Pts',(3.9892268254758,-0.575795237079985,10.0663779392223));
#57209=CARTESIAN_POINT('Ctrl Pts',(3.97279425521263,-0.493919038588913,
10.0355515093655));
#57210=CARTESIAN_POINT('Ctrl Pts',(3.95122422996677,-0.338198219021382,
9.98967393256177));
#57211=CARTESIAN_POINT('Ctrl Pts',(3.94476187062674,-0.265711864048123,
9.97296500528629));
#57212=CARTESIAN_POINT('Ctrl Pts',(3.94008040260285,-0.129741091012596,
9.9490073533817));
#57213=CARTESIAN_POINT('Ctrl Pts',(3.94077929528986,-0.066641501326757,
9.94075353629532));
#57214=CARTESIAN_POINT('Ctrl Pts',(3.9481430854642,0.0595501401552381,9.92962711164072));
#57215=CARTESIAN_POINT('Ctrl Pts',(3.95484997220342,0.122796625322549,9.92666046019834));
#57216=CARTESIAN_POINT('Ctrl Pts',(3.97559498700695,0.260149217292054,9.92672328284864));
#57217=CARTESIAN_POINT('Ctrl Pts',(3.99074823399124,0.33394912587413,9.93094211655924));
#57218=CARTESIAN_POINT('Ctrl Pts',(4.03134493898561,0.491142174428259,9.94994913888734));
#57219=CARTESIAN_POINT('Ctrl Pts',(4.05829569965353,0.574254018778612,9.96634212921925));
#57220=CARTESIAN_POINT('Ctrl Pts',(4.08975875486384,0.653834841428668,9.98861494769777));
#57221=CARTESIAN_POINT('',(4.05146214282868,-1.2,10.0439680914571));
#57222=CARTESIAN_POINT('Ctrl Pts',(4.05146214282868,-1.2,10.0439680914571));
#57223=CARTESIAN_POINT('Ctrl Pts',(4.04427281420881,-1.1339556629759,10.0542098704782));
#57224=CARTESIAN_POINT('Ctrl Pts',(4.03488407820185,-1.03841658953484,10.067500381683));
#57225=CARTESIAN_POINT('Ctrl Pts',(4.0163549400073,-0.795343226740802,10.0933659085415));
#57226=CARTESIAN_POINT('Ctrl Pts',(4.01340110853449,-0.741643831139491,
10.0974393285217));
#57227=CARTESIAN_POINT('Ctrl Pts',(4.00955034077162,-0.653834841531102,
10.1027583545342));
#57228=CARTESIAN_POINT('Ctrl Pts',(4.01179369694817,-1.29999999999639,9.9254378241233));
#57229=CARTESIAN_POINT('Ctrl Pts',(4.01906436001224,-1.28293734428946,9.945099061467));
#57230=CARTESIAN_POINT('Ctrl Pts',(4.02556213161071,-1.26616775796805,9.96528846164041));
#57231=CARTESIAN_POINT('Ctrl Pts',(4.03670033314328,-1.23890235909598,9.99713900241556));
#57232=CARTESIAN_POINT('Ctrl Pts',(4.04542626944918,-1.21716802518332,10.0226852886214));
#57233=CARTESIAN_POINT('Ctrl Pts',(4.05146214282868,-1.2,10.0439680914571));
#57234=CARTESIAN_POINT('Origin',(0.,1.25,7.2));
#57235=CARTESIAN_POINT('Origin',(0.,1.2,7.2));
#57236=CARTESIAN_POINT('Origin',(0.,0.92691742076555,7.2));
#57237=CARTESIAN_POINT('Origin',(0.,0.653834841531101,7.2));
#57238=CARTESIAN_POINT('Origin',(0.,0.,7.2));
#57239=CARTESIAN_POINT('Origin',(0.,-0.653834841531101,7.2));
#57240=CARTESIAN_POINT('Origin',(0.,-0.926917420765551,7.2));
#57241=CARTESIAN_POINT('Origin',(0.,-1.2,7.2));
#57242=CARTESIAN_POINT('Origin',(0.,-1.25,7.2));
#57243=CARTESIAN_POINT('Ctrl Pts',(3.90341546958847,-1.30000000000005,10.3955984628936));
#57244=CARTESIAN_POINT('Ctrl Pts',(3.93440493784208,-1.18514270861181,10.3663638202781));
#57245=CARTESIAN_POINT('Ctrl Pts',(3.95093219463971,-1.06847604194513,10.3366909515245));
#57246=CARTESIAN_POINT('Ctrl Pts',(3.9557028624898,-0.794772684000851,10.2671282986208));
#57247=CARTESIAN_POINT('Ctrl Pts',(3.90486897722008,-0.636309800095197,
10.2190179716147));
#57248=CARTESIAN_POINT('Ctrl Pts',(3.86905149194761,-0.319434907277159,
10.1540957676241));
#57249=CARTESIAN_POINT('Ctrl Pts',(3.83456187378936,-0.158333333333332,
10.1238619534767));
#57250=CARTESIAN_POINT('Ctrl Pts',(3.85489608531651,0.158333333333334,10.0967615839629));
#57251=CARTESIAN_POINT('Ctrl Pts',(3.9105765830082,0.319434907277167,10.0986164293539));
#57252=CARTESIAN_POINT('Ctrl Pts',(3.986068422003,0.636309800095206,10.1109415465311));
#57253=CARTESIAN_POINT('Ctrl Pts',(4.05793460521832,0.79477268400084,10.1299478790481));
#57254=CARTESIAN_POINT('Ctrl Pts',(4.08243023811811,1.0684760419458,10.1636773708336));
#57255=CARTESIAN_POINT('Ctrl Pts',(4.07701141444102,1.18514270861313,10.1807976562281));
#57256=CARTESIAN_POINT('Ctrl Pts',(4.05557051525715,1.300000000002,10.200437979824));
#57257=CARTESIAN_POINT('Ctrl Pts',(3.8972319130928,-1.30000000000005,10.3945543778395));
#57258=CARTESIAN_POINT('Ctrl Pts',(3.92705536482917,-1.18514270861181,10.3650892251986));
#57259=CARTESIAN_POINT('Ctrl Pts',(3.9427245954191,-1.06847604194513,10.3352589479046));
#57260=CARTESIAN_POINT('Ctrl Pts',(3.94622457031017,-0.794772684000851,
10.2655015288375));
#57261=CARTESIAN_POINT('Ctrl Pts',(3.89556659455229,-0.636309800095197,
10.2175231168598));
#57262=CARTESIAN_POINT('Ctrl Pts',(3.85968799168501,-0.319434907277159,
10.1526473315009));
#57263=CARTESIAN_POINT('Ctrl Pts',(3.82563590813615,-0.158333333333332,
10.1223762331194));
#57264=CARTESIAN_POINT('Ctrl Pts',(3.84587256311358,0.158333333333334,10.0954895843591));
#57265=CARTESIAN_POINT('Ctrl Pts',(3.90098481553906,0.319434907277167,10.0976623464721));
#57266=CARTESIAN_POINT('Ctrl Pts',(3.97640658899012,0.636309800095206,10.1102400844189));
#57267=CARTESIAN_POINT('Ctrl Pts',(4.04805772503971,0.79477268400084,10.1292210103236));
#57268=CARTESIAN_POINT('Ctrl Pts',(4.07384612687898,1.0684760419458,10.1631137378143));
#57269=CARTESIAN_POINT('Ctrl Pts',(4.06932031476021,1.18514270861313,10.1803205969217));
#57270=CARTESIAN_POINT('Ctrl Pts',(4.0491058469209,1.300000000002,10.200063409255));
#57271=CARTESIAN_POINT('Ctrl Pts',(3.88471837690218,-1.29999999999985,10.3927059310096));
#57272=CARTESIAN_POINT('Ctrl Pts',(3.91227329929968,-1.18514270861163,10.3626773220286));
#57273=CARTESIAN_POINT('Ctrl Pts',(3.92628138935286,-1.06847604194497,10.332439936458));
#57274=CARTESIAN_POINT('Ctrl Pts',(3.92734698693467,-0.79477268400073,10.2621032111342));
#57275=CARTESIAN_POINT('Ctrl Pts',(3.8771691524999,-0.636309800095101,10.2141284835984));
#57276=CARTESIAN_POINT('Ctrl Pts',(3.84106775360212,-0.319434907277111,
10.1495363480085));
#57277=CARTESIAN_POINT('Ctrl Pts',(3.80755160262496,-0.158333333333308,
10.1198406743019));
#57278=CARTESIAN_POINT('Ctrl Pts',(3.82753192323713,0.15833333333331,10.0935016391188));
#57279=CARTESIAN_POINT('Ctrl Pts',(3.88173624342239,0.319434907277118,10.0958780309468));
#57280=CARTESIAN_POINT('Ctrl Pts',(3.95709428015321,0.63630980009511,10.1088161402808));
#57281=CARTESIAN_POINT('Ctrl Pts',(4.02825982105977,0.794772684000721,10.1278489843642));
#57282=CARTESIAN_POINT('Ctrl Pts',(4.05663569066553,1.06847604194564,10.1620627825047));
#57283=CARTESIAN_POINT('Ctrl Pts',(4.05390038764762,1.18514270861295,10.1794336337835));
#57284=CARTESIAN_POINT('Ctrl Pts',(4.03614691908903,1.30000000000181,10.1993654508722));
#57285=CARTESIAN_POINT('Ctrl Pts',(3.86050496345744,-1.29999999999983,10.3876974682567));
#57286=CARTESIAN_POINT('Ctrl Pts',(3.88261846239695,-1.18514270861162,10.3580947882787));
#57287=CARTESIAN_POINT('Ctrl Pts',(3.89273073077964,-1.06847604194496,10.3280188949586));
#57288=CARTESIAN_POINT('Ctrl Pts',(3.88836685027176,-0.79477268400072,10.257444347241));
#57289=CARTESIAN_POINT('Ctrl Pts',(3.83991593350838,-0.636309800095094,
10.2081207376447));
#57290=CARTESIAN_POINT('Ctrl Pts',(3.80396032762788,-0.319434907277108,
10.1429732908664));
#57291=CARTESIAN_POINT('Ctrl Pts',(3.77207195551128,-0.158333333333307,
10.113390850971));
#57292=CARTESIAN_POINT('Ctrl Pts',(3.79187459039628,0.158333333333309,10.0874431279985));
#57293=CARTESIAN_POINT('Ctrl Pts',(3.84418233538711,0.319434907277116,10.0902375668533));
#57294=CARTESIAN_POINT('Ctrl Pts',(3.91921823181388,0.636309800095104,10.1042429561577));
#57295=CARTESIAN_POINT('Ctrl Pts',(3.98890458788481,0.794772684000714,10.1244479769042));
#57296=CARTESIAN_POINT('Ctrl Pts',(4.02247474477858,1.06847604194563,10.1593341744568));
#57297=CARTESIAN_POINT('Ctrl Pts',(4.02345098386902,1.18514270861294,10.176811067091));
#57298=CARTESIAN_POINT('Ctrl Pts',(4.01087218502744,1.30000000000179,10.1966639101));
#57299=CARTESIAN_POINT('Ctrl Pts',(3.84178186561024,-1.29999999999939,10.3843671205557));
#57300=CARTESIAN_POINT('Ctrl Pts',(3.86080495295138,-1.18514270861122,10.3532467534984));
#57301=CARTESIAN_POINT('Ctrl Pts',(3.86858527719493,-1.06847604194459,10.3221965910117));
#57302=CARTESIAN_POINT('Ctrl Pts',(3.86058635078354,-0.794772684000451,
10.2506266907062));
#57303=CARTESIAN_POINT('Ctrl Pts',(3.81212911135781,-0.636309800094877,
10.2026892754764));
#57304=CARTESIAN_POINT('Ctrl Pts',(3.77575940271681,-0.319434907276998,
10.1380984101569));
#57305=CARTESIAN_POINT('Ctrl Pts',(3.74512432345125,-0.158333333333252,
10.1085544874522));
#57306=CARTESIAN_POINT('Ctrl Pts',(3.76466940587767,0.158333333333255,10.0831483511506));
#57307=CARTESIAN_POINT('Ctrl Pts',(3.81555764025485,0.319434907277006,10.0862626912517));
#57308=CARTESIAN_POINT('Ctrl Pts',(3.89029698142897,0.636309800094886,10.1011877726536));
#57309=CARTESIAN_POINT('Ctrl Pts',(3.95881995092127,0.79477268400044,10.1223398957364));
#57310=CARTESIAN_POINT('Ctrl Pts',(3.99629237825836,1.06847604194526,10.157799288423));
#57311=CARTESIAN_POINT('Ctrl Pts',(4.00007247219514,1.18514270861254,10.1753757244196));
#57312=CARTESIAN_POINT('Ctrl Pts',(3.99141223476473,1.30000000000135,10.1951795392188));
#57313=CARTESIAN_POINT('Ctrl Pts',(3.82918677459915,-1.29999999999936,10.3819124216719));
#57314=CARTESIAN_POINT('Ctrl Pts',(3.8455386514497,-1.18514270861119,10.350755495859));
#57315=CARTESIAN_POINT('Ctrl Pts',(3.85139900877872,-1.06847604194456,10.3196192408126));
#57316=CARTESIAN_POINT('Ctrl Pts',(3.84070009765322,-0.794772684000428,
10.2477360164746));
#57317=CARTESIAN_POINT('Ctrl Pts',(3.79300134625836,-0.636309800094859,
10.1993514351645));
#57318=CARTESIAN_POINT('Ctrl Pts',(3.75672553111135,-0.31943490727699,10.134439742147));
#57319=CARTESIAN_POINT('Ctrl Pts',(3.72706155916688,-0.158333333333248,
10.1047089972824));
#57320=CARTESIAN_POINT('Ctrl Pts',(3.74646404977274,0.15833333333325,10.0796011966045));
#57321=CARTESIAN_POINT('Ctrl Pts',(3.79611713161317,0.319434907276997,10.0834276162307));
#57322=CARTESIAN_POINT('Ctrl Pts',(3.87071952184266,0.636309800094868,10.0988189902669));
#57323=CARTESIAN_POINT('Ctrl Pts',(3.93885479502108,0.794772684000418,10.1197848490444));
#57324=CARTESIAN_POINT('Ctrl Pts',(3.97898689489694,1.06847604194523,10.155644952634));
#57325=CARTESIAN_POINT('Ctrl Pts',(3.98459288328237,1.18514270861251,10.173473174971));
#57326=CARTESIAN_POINT('Ctrl Pts',(3.97843316105777,1.30000000000132,10.1936071095487));
#57327=CARTESIAN_POINT('Ctrl Pts',(3.8286151440339,-1.29999999999936,10.3817992007246));
#57328=CARTESIAN_POINT('Ctrl Pts',(3.84484631571692,-1.18514270861119,10.3506392320354));
#57329=CARTESIAN_POINT('Ctrl Pts',(3.85061978962886,-1.06847604194456,10.3194982992646));
#57330=CARTESIAN_POINT('Ctrl Pts',(3.8397982954385,-0.794772684000429,10.2476004916214));
#57331=CARTESIAN_POINT('Ctrl Pts',(3.79213265237141,-0.63630980009486,10.1991981158477));
#57332=CARTESIAN_POINT('Ctrl Pts',(3.75586081820926,-0.31943490727699,10.1342723455195));
#57333=CARTESIAN_POINT('Ctrl Pts',(3.72624169362474,-0.158333333333248,
10.1045317909193));
#57334=CARTESIAN_POINT('Ctrl Pts',(3.74563757775941,0.15833333333325,10.0794377892856));
#57335=CARTESIAN_POINT('Ctrl Pts',(3.79523397063094,0.319434907276997,10.0832975993543));
#57336=CARTESIAN_POINT('Ctrl Pts',(3.86982958656818,0.636309800094869,10.0987112338179));
#57337=CARTESIAN_POINT('Ctrl Pts',(3.93794685561963,0.794772684000419,10.1196693783045));
#57338=CARTESIAN_POINT('Ctrl Pts',(3.97819966709136,1.06847604194523,10.1555480993504));
#57339=CARTESIAN_POINT('Ctrl Pts',(3.98388865979907,1.18514270861251,10.1733877785578));
#57340=CARTESIAN_POINT('Ctrl Pts',(3.97784269464199,1.30000000000132,10.1935365680694));
#57341=CARTESIAN_POINT('Ctrl Pts',(3.82804377053059,-1.29999999999936,10.381685549878));
#57342=CARTESIAN_POINT('Ctrl Pts',(3.844154236367,-1.18514270861119,10.3505225480926));
#57343=CARTESIAN_POINT('Ctrl Pts',(3.84984083038205,-1.06847604194456,10.3193769349447));
#57344=CARTESIAN_POINT('Ctrl Pts',(3.83889677096033,-0.794772684000428,
10.2474645091452));
#57345=CARTESIAN_POINT('Ctrl Pts',(3.79126435532817,-0.636309800094859,
10.1990440997006));
#57346=CARTESIAN_POINT('Ctrl Pts',(3.75499635039537,-0.31943490727699,10.1341045185275));
#57347=CARTESIAN_POINT('Ctrl Pts',(3.72542163358055,-0.158333333333248,
10.104354973886));
#57348=CARTESIAN_POINT('Ctrl Pts',(3.74481096465794,0.15833333333325,10.0792746415237));
#57349=CARTESIAN_POINT('Ctrl Pts',(3.79435128175347,0.319434907276997,10.0831666439978));
#57350=CARTESIAN_POINT('Ctrl Pts',(3.86894013913835,0.636309800094868,10.0986025144048));
#57351=CARTESIAN_POINT('Ctrl Pts',(3.93703879316676,0.794772684000419,10.1195541647746));
#57352=CARTESIAN_POINT('Ctrl Pts',(3.97741223777967,1.06847604194523,10.155451656625));
#57353=CARTESIAN_POINT('Ctrl Pts',(3.9831843006373,1.18514270861251,10.1733026583442));
#57354=CARTESIAN_POINT('Ctrl Pts',(3.97725225816315,1.30000000000132,10.1934659676937));
#57355=CARTESIAN_POINT('Ctrl Pts',(3.82690210090624,-1.29999999999936,10.3814562692382));
#57356=CARTESIAN_POINT('Ctrl Pts',(3.84277195760607,-1.18514270861119,10.3502856909788));
#57357=CARTESIAN_POINT('Ctrl Pts',(3.84828524002961,-1.06847604194457,10.3191298633125));
#57358=CARTESIAN_POINT('Ctrl Pts',(3.83709626695257,-0.794772684000429,
10.2471877455224));
#57359=CARTESIAN_POINT('Ctrl Pts',(3.78952903120354,-0.63630980009486,10.1987335903228));
#57360=CARTESIAN_POINT('Ctrl Pts',(3.75326808760653,-0.31943490727699,10.1337674532044));
#57361=CARTESIAN_POINT('Ctrl Pts',(3.72378212165099,-0.158333333333248,
10.1040000534961));
#57362=CARTESIAN_POINT('Ctrl Pts',(3.74315831541199,0.158333333333251,10.0789470831623));
#57363=CARTESIAN_POINT('Ctrl Pts',(3.79258701178728,0.319434907276997,10.0829024027525));
#57364=CARTESIAN_POINT('Ctrl Pts',(3.86716187256129,0.636309800094869,10.0983836951478));
#57365=CARTESIAN_POINT('Ctrl Pts',(3.93522189720306,0.79477268400042,10.1193251494811));
#57366=CARTESIAN_POINT('Ctrl Pts',(3.97583634524737,1.06847604194523,10.155260735818));
#57367=CARTESIAN_POINT('Ctrl Pts',(3.98177469585523,1.18514270861251,10.173134107549));
#57368=CARTESIAN_POINT('Ctrl Pts',(3.97607090742614,1.30000000000132,10.1933256672303));
#57369=CARTESIAN_POINT('Ctrl Pts',(3.82443325455095,-1.29999999999936,10.3809508004002));
#57370=CARTESIAN_POINT('Ctrl Pts',(3.83978528105836,-1.18514270861119,10.3497573367654));
#57371=CARTESIAN_POINT('Ctrl Pts',(3.84492505588982,-1.06847604194457,10.3185756333572));
#57372=CARTESIAN_POINT('Ctrl Pts',(3.83320661963357,-0.79477268400043,10.2465668290817));
#57373=CARTESIAN_POINT('Ctrl Pts',(3.78577595644831,-0.63630980009486,10.1980479216123));
#57374=CARTESIAN_POINT('Ctrl Pts',(3.74952702321827,-0.31943490727699,10.1330301437214));
#57375=CARTESIAN_POINT('Ctrl Pts',(3.72023070654343,-0.158333333333248,
10.1032290247907));
#57376=CARTESIAN_POINT('Ctrl Pts',(3.73957843869313,0.158333333333251,10.078235079962));
#57377=CARTESIAN_POINT('Ctrl Pts',(3.78877035130657,0.319434907276997,10.0823175948477));
#57378=CARTESIAN_POINT('Ctrl Pts',(3.86331326275209,0.636309800094869,10.0979005853927));
#57379=CARTESIAN_POINT('Ctrl Pts',(3.93128157816105,0.79477268400042,10.1188360067461));
#57380=CARTESIAN_POINT('Ctrl Pts',(3.97241679402589,1.06847604194523,10.1548570128613));
#57381=CARTESIAN_POINT('Ctrl Pts',(3.97871623257295,1.18514270861251,10.1727772922235));
#57382=CARTESIAN_POINT('Ctrl Pts',(3.97350919892911,1.30000000000132,10.1930256921104));
#57383=CARTESIAN_POINT('Ctrl Pts',(3.82065344079858,-1.29999999999937,10.3801385168388));
#57384=CARTESIAN_POINT('Ctrl Pts',(3.83523203439744,-1.18514270861119,10.3488676639844));
#57385=CARTESIAN_POINT('Ctrl Pts',(3.83981066839133,-1.06847604194457,10.3176215936814));
#57386=CARTESIAN_POINT('Ctrl Pts',(3.82728632169733,-0.794772684000434,
10.2454941731782));
#57387=CARTESIAN_POINT('Ctrl Pts',(3.78003649534408,-0.636309800094864,
10.1969280615303));
#57388=CARTESIAN_POINT('Ctrl Pts',(3.74378425590443,-0.319434907276992,
10.1318704540711));
#57389=CARTESIAN_POINT('Ctrl Pts',(3.71476004854344,-0.158333333333249,
10.1020547371762));
#57390=CARTESIAN_POINT('Ctrl Pts',(3.73406460988566,0.158333333333251,10.0771492785743));
#57391=CARTESIAN_POINT('Ctrl Pts',(3.78292725211545,0.319434907276999,10.0813588866284));
#57392=CARTESIAN_POINT('Ctrl Pts',(3.85741403110121,0.636309800094873,10.0971130422566));
#57393=CARTESIAN_POINT('Ctrl Pts',(3.92519231535607,0.794772684000425,10.1181374888045));
#57394=CARTESIAN_POINT('Ctrl Pts',(3.9671225199414,1.06847604194524,10.1543025913043));
#57395=CARTESIAN_POINT('Ctrl Pts',(3.97398362703879,1.18514270861251,10.1722827757587));
#57396=CARTESIAN_POINT('Ctrl Pts',(3.96955580933573,1.30000000000132,10.1925886118444));
#57397=CARTESIAN_POINT('Ctrl Pts',(3.81614245087933,-1.29999999999937,10.3791150120397));
#57398=CARTESIAN_POINT('Ctrl Pts',(3.82983834935375,-1.1851427086112,10.3476691706384));
#57399=CARTESIAN_POINT('Ctrl Pts',(3.83377063915946,-1.06847604194458,10.3162969473966));
#57400=CARTESIAN_POINT('Ctrl Pts',(3.82029912603461,-0.794772684000437,
10.2439909083921));
#57401=CARTESIAN_POINT('Ctrl Pts',(3.77321602696589,-0.636309800094866,
10.1954579000826));
#57402=CARTESIAN_POINT('Ctrl Pts',(3.7369168456406,-0.319434907276993,10.1304313131957));
#57403=CARTESIAN_POINT('Ctrl Pts',(3.7081728540808,-0.15833333333325,10.1006862676617));
#57404=CARTESIAN_POINT('Ctrl Pts',(3.72742496407903,0.158333333333252,10.0758859834643));
#57405=CARTESIAN_POINT('Ctrl Pts',(3.775962962915,0.319434907277,10.0801096387451));
#57406=CARTESIAN_POINT('Ctrl Pts',(3.85037350037145,0.636309800094875,10.0960886735164));
#57407=CARTESIAN_POINT('Ctrl Pts',(3.91783701116371,0.794772684000426,10.1173953048217));
#57408=CARTESIAN_POINT('Ctrl Pts',(3.96070864750431,1.06847604194524,10.1537588347598));
#57409=CARTESIAN_POINT('Ctrl Pts',(3.96825327759921,1.18514270861252,10.1717915915041));
#57410=CARTESIAN_POINT('Ctrl Pts',(3.96478499496778,1.30000000000133,10.192116680284));
#57411=CARTESIAN_POINT('Ctrl Pts',(3.81014719913854,-1.29999999999938,10.3777111866877));
#57412=CARTESIAN_POINT('Ctrl Pts',(3.82270608604597,-1.18514270861121,10.3459599070711));
#57413=CARTESIAN_POINT('Ctrl Pts',(3.82580088545279,-1.06847604194459,10.3143755614268));
#57414=CARTESIAN_POINT('Ctrl Pts',(3.81108655578441,-0.794772684000444,
10.2417950554328));
#57415=CARTESIAN_POINT('Ctrl Pts',(3.76418481193213,-0.636309800094871,
10.1933794802241));
#57416=CARTESIAN_POINT('Ctrl Pts',(3.72779025172961,-0.319434907276995,
10.1284546694874));
#57417=CARTESIAN_POINT('Ctrl Pts',(3.69938415143322,-0.158333333333251,
10.0988725580143));
#57418=CARTESIAN_POINT('Ctrl Pts',(3.71856629006732,0.158333333333253,10.0742101181523));
#57419=CARTESIAN_POINT('Ctrl Pts',(3.76672800780696,0.319434907277003,10.0783396132334));
#57420=CARTESIAN_POINT('Ctrl Pts',(3.84102706820497,0.63630980009488,10.0946383424229));
#57421=CARTESIAN_POINT('Ctrl Pts',(3.90799558118256,0.794772684000434,10.1164728658535));
#57422=CARTESIAN_POINT('Ctrl Pts',(3.95211208871403,1.06847604194525,10.1531224721248));
#57423=CARTESIAN_POINT('Ctrl Pts',(3.96057690181205,1.18514270861253,10.1712079622024));
#57424=CARTESIAN_POINT('Ctrl Pts',(3.95841012657538,1.30000000000134,10.1915146858042));
#57425=CARTESIAN_POINT('Ctrl Pts',(3.80264558611359,-1.29999999999939,10.3759652989145));
#57426=CARTESIAN_POINT('Ctrl Pts',(3.81378061794709,-1.18514270861122,10.3438347634036));
#57427=CARTESIAN_POINT('Ctrl Pts',(3.81583146444968,-1.06847604194459,10.3119786158427));
#57428=CARTESIAN_POINT('Ctrl Pts',(3.79958304474167,-0.794772684000448,
10.2390184332324));
#57429=CARTESIAN_POINT('Ctrl Pts',(3.75294760073062,-0.636309800094874,
10.1906800667924));
#57430=CARTESIAN_POINT('Ctrl Pts',(3.71645495728067,-0.319434907276997,
10.1258446517031));
#57431=CARTESIAN_POINT('Ctrl Pts',(3.68847208962925,-0.158333333333252,
10.0964653215993));
#57432=CARTESIAN_POINT('Ctrl Pts',(3.70755240882307,0.158333333333254,10.0719990818131));
#57433=CARTESIAN_POINT('Ctrl Pts',(3.75520362998421,0.319434907277005,10.0760810388163));
#57434=CARTESIAN_POINT('Ctrl Pts',(3.82936372624179,0.636309800094884,10.0927734438064));
#57435=CARTESIAN_POINT('Ctrl Pts',(3.89577441947964,0.794772684000437,10.115148633787));
#57436=CARTESIAN_POINT('Ctrl Pts',(3.94143070159432,1.06847604194526,10.1521886133447));
#57437=CARTESIAN_POINT('Ctrl Pts',(3.95102321959067,1.18514270861253,10.1703851611552));
#57438=CARTESIAN_POINT('Ctrl Pts',(3.95044534278784,1.30000000000135,10.1907450220921));
#57439=CARTESIAN_POINT('Ctrl Pts',(3.79051760574996,-1.29999999999941,10.3734001477454));
#57440=CARTESIAN_POINT('Ctrl Pts',(3.79917807880938,-1.18514270861123,10.3410116256646));
#57441=CARTESIAN_POINT('Ctrl Pts',(3.79944890201863,-1.06847604194461,10.3089148904893));
#57442=CARTESIAN_POINT('Ctrl Pts',(3.78069278831246,-0.794772684000462,
10.2354390974279));
#57443=CARTESIAN_POINT('Ctrl Pts',(3.73473563294115,-0.636309800094885,
10.1867768390611));
#57444=CARTESIAN_POINT('Ctrl Pts',(3.69834920030187,-0.319434907277002,
10.1216048277028));
#57445=CARTESIAN_POINT('Ctrl Pts',(3.6713374077935,-0.158333333333255,10.0920043628996));
#57446=CARTESIAN_POINT('Ctrl Pts',(3.69026903992965,0.158333333333257,10.0678283520062));
#57447=CARTESIAN_POINT('Ctrl Pts',(3.73671140064775,0.31943490727701,10.0725764750798));
#57448=CARTESIAN_POINT('Ctrl Pts',(3.81064390796835,0.636309800094894,10.089881330195));
#57449=CARTESIAN_POINT('Ctrl Pts',(3.87654066801923,0.79477268400045,10.1123448087573));
#57450=CARTESIAN_POINT('Ctrl Pts',(3.92470370339651,1.06847604194527,10.1499305823319));
#57451=CARTESIAN_POINT('Ctrl Pts',(3.93605571402822,1.18514270861255,10.1684059123361));
#57452=CARTESIAN_POINT('Ctrl Pts',(3.9379117418931,1.30000000000137,10.1890870836542));
#57453=CARTESIAN_POINT('Ctrl Pts',(3.77531269856596,-1.29999999999947,10.3702508598051));
#57454=CARTESIAN_POINT('Ctrl Pts',(3.7808830596038,-1.18514270861129,10.3375282984927));
#57455=CARTESIAN_POINT('Ctrl Pts',(3.77892690458547,-1.06847604194466,10.3051304292443));
#57456=CARTESIAN_POINT('Ctrl Pts',(3.75702003740151,-0.794772684000497,
10.2310349737318));
#57457=CARTESIAN_POINT('Ctrl Pts',(3.71188048972456,-0.636309800094912,
10.1820244175521));
#57458=CARTESIAN_POINT('Ctrl Pts',(3.67559935454688,-0.319434907277015,
10.1164887747854));
#57459=CARTESIAN_POINT('Ctrl Pts',(3.64976156025509,-0.158333333333261,
10.0866994517134));
#57460=CARTESIAN_POINT('Ctrl Pts',(3.66855436893452,0.158333333333263,10.0627999913768));
#57461=CARTESIAN_POINT('Ctrl Pts',(3.71364679734388,0.319434907277024,10.0680628729313));
#57462=CARTESIAN_POINT('Ctrl Pts',(3.78726682550946,0.636309800094921,10.0861941513323));
#57463=CARTESIAN_POINT('Ctrl Pts',(3.85231154121724,0.794772684000484,10.1091939955424));
#57464=CARTESIAN_POINT('Ctrl Pts',(3.90352518701274,1.06847604194532,10.1476179483369));
#57465=CARTESIAN_POINT('Ctrl Pts',(3.91706593765084,1.1851427086126,10.1664548632847));
#57466=CARTESIAN_POINT('Ctrl Pts',(3.9219789493147,1.30000000000142,10.1874963877634));
#57467=CARTESIAN_POINT('Ctrl Pts',(3.75144143449034,-1.29999999999955,10.3644010333803));
#57468=CARTESIAN_POINT('Ctrl Pts',(3.75240741099658,-1.18514270861136,10.3305289846406));
#57469=CARTESIAN_POINT('Ctrl Pts',(3.7471129191241,-1.06847604194473,10.2972421000756));
#57470=CARTESIAN_POINT('Ctrl Pts',(3.72041864938193,-0.79477268400055,10.2216945840175));
#57471=CARTESIAN_POINT('Ctrl Pts',(3.676449916003,-0.636309800094955,10.1723815037641));
#57472=CARTESIAN_POINT('Ctrl Pts',(3.64000955362952,-0.319434907277037,
10.1068397469521));
#57473=CARTESIAN_POINT('Ctrl Pts',(3.61556008210046,-0.158333333333272,
10.0776086571675));
#57474=CARTESIAN_POINT('Ctrl Pts',(3.63383454621419,0.158333333333274,10.0546636777887));
#57475=CARTESIAN_POINT('Ctrl Pts',(3.67672943965919,0.319434907277046,10.0608301121857));
#57476=CARTESIAN_POINT('Ctrl Pts',(3.75004534089352,0.636309800094965,10.0798783695091));
#57477=CARTESIAN_POINT('Ctrl Pts',(3.81422848444124,0.794772684000539,10.1027155580515));
#57478=CARTESIAN_POINT('Ctrl Pts',(3.87050679078574,1.06847604194539,10.1421616302036));
#57479=CARTESIAN_POINT('Ctrl Pts',(3.8875527138798,1.18514270861268,10.1616070485395));
#57480=CARTESIAN_POINT('Ctrl Pts',(3.89728376656809,1.30000000000151,10.1834231421977));
#57481=CARTESIAN_POINT('Ctrl Pts',(3.72739820580732,-1.29999999999965,10.3587858048955));
#57482=CARTESIAN_POINT('Ctrl Pts',(3.72376039659815,-1.18514270861146,10.3237624646455));
#57483=CARTESIAN_POINT('Ctrl Pts',(3.71509786759347,-1.06847604194481,10.2896362036518));
#57484=CARTESIAN_POINT('Ctrl Pts',(3.68347758474028,-0.794772684000613,
10.2128701463635));
#57485=CARTESIAN_POINT('Ctrl Pts',(3.64034334348832,-0.636309800095004,
10.1638240822689));
#57486=CARTESIAN_POINT('Ctrl Pts',(3.60378905924222,-0.319434907277061,
10.0981981455333));
#57487=CARTESIAN_POINT('Ctrl Pts',(3.58098080217359,-0.158333333333283,
10.0691232838899));
#57488=CARTESIAN_POINT('Ctrl Pts',(3.59917771711532,0.158333333333285,10.0463299146732));
#57489=CARTESIAN_POINT('Ctrl Pts',(3.64045609269603,0.319434907277065,10.052281540449));
#57490=CARTESIAN_POINT('Ctrl Pts',(3.71351968645555,0.636309800095008,10.0721509398841));
#57491=CARTESIAN_POINT('Ctrl Pts',(3.77629943079809,0.7947726840006,10.0958594558066));
#57492=CARTESIAN_POINT('Ctrl Pts',(3.83726787830799,1.06847604194547,10.1370353786994));
#57493=CARTESIAN_POINT('Ctrl Pts',(3.85767445872077,1.18514270861277,10.1573602260567));
#57494=CARTESIAN_POINT('Ctrl Pts',(3.87209663772287,1.3000000000016,10.1801863894691));
#57495=CARTESIAN_POINT('Ctrl Pts',(3.70360350260276,-1.29999999999968,10.3527512023952));
#57496=CARTESIAN_POINT('Ctrl Pts',(3.69524543931284,-1.18514270861149,10.3167362009834));
#57497=CARTESIAN_POINT('Ctrl Pts',(3.68324054739408,-1.06847604194484,10.2817005801307));
#57498=CARTESIAN_POINT('Ctrl Pts',(3.64708194181316,-0.794772684000633,
10.2030238521252));
#57499=CARTESIAN_POINT('Ctrl Pts',(3.60585793754741,-0.63630980009502,10.1524461653563));
#57500=CARTESIAN_POINT('Ctrl Pts',(3.5693783489072,-0.319434907277069,10.0864042491589));
#57501=CARTESIAN_POINT('Ctrl Pts',(3.54762896415299,-0.158333333333288,
10.0584464163139));
#57502=CARTESIAN_POINT('Ctrl Pts',(3.56523065483139,0.15833333333329,10.0366788876955));
#57503=CARTESIAN_POINT('Ctrl Pts',(3.60455752023384,0.319434907277076,10.0429968367841));
#57504=CARTESIAN_POINT('Ctrl Pts',(3.67693979951042,0.636309800095027,10.0644398611071));
#57505=CARTESIAN_POINT('Ctrl Pts',(3.73796629905055,0.794772684000619,10.0896540846223));
#57506=CARTESIAN_POINT('Ctrl Pts',(3.80379882167682,1.0684760419455,10.1322624369106));
#57507=CARTESIAN_POINT('Ctrl Pts',(3.82778999860573,1.1851427086128,10.1530748961532));
#57508=CARTESIAN_POINT('Ctrl Pts',(3.84727589275395,1.30000000000164,10.1762562377278));
#57509=CARTESIAN_POINT('Ctrl Pts',(3.68570115410586,-1.29999999999973,10.3482444573312));
#57510=CARTESIAN_POINT('Ctrl Pts',(3.67428383436732,-1.18514270861152,10.3106980921864));
#57511=CARTESIAN_POINT('Ctrl Pts',(3.65997227456622,-1.06847604194487,10.2746581733336));
#57512=CARTESIAN_POINT('Ctrl Pts',(3.62022343487266,-0.794772684000658,
10.1948789433209));
#57513=CARTESIAN_POINT('Ctrl Pts',(3.57884262070824,-0.636309800095039,
10.1458049927457));
#57514=CARTESIAN_POINT('Ctrl Pts',(3.54228491914268,-0.319434907277079,
10.079684590746));
#57515=CARTESIAN_POINT('Ctrl Pts',(3.52237947065255,-0.158333333333293,
10.050831400517));
#57516=CARTESIAN_POINT('Ctrl Pts',(3.54007106517567,0.158333333333295,10.0289178015944));
#57517=CARTESIAN_POINT('Ctrl Pts',(3.57782735161353,0.319434907277085,10.035674057266));
#57518=CARTESIAN_POINT('Ctrl Pts',(3.65009718999559,0.636309800095045,10.0575314775792));
#57519=CARTESIAN_POINT('Ctrl Pts',(3.71059118059011,0.794772684000643,10.082369063769));
#57520=CARTESIAN_POINT('Ctrl Pts',(3.77984387637945,1.06847604194553,10.1264643368999));
#57521=CARTESIAN_POINT('Ctrl Pts',(3.80618333956597,1.18514270861284,10.1482800998854));
#57522=CARTESIAN_POINT('Ctrl Pts',(3.82888533999698,1.30000000000168,10.1728244160087));
#57523=CARTESIAN_POINT('Ctrl Pts',(3.66853450170536,-1.29999999999975,10.3426239775828));
#57524=CARTESIAN_POINT('Ctrl Pts',(3.65350080759412,-1.18514270861155,10.3044212694721));
#57525=CARTESIAN_POINT('Ctrl Pts',(3.63664732387774,-1.06847604194489,10.2677322320564));
#57526=CARTESIAN_POINT('Ctrl Pts',(3.5935083269295,-0.794772684000673,10.1864700981242));
#57527=CARTESIAN_POINT('Ctrl Pts',(3.55376029588737,-0.636309800095053,
10.1359540029149));
#57528=CARTESIAN_POINT('Ctrl Pts',(3.5173108952179,-0.319434907277086,10.0694354783221));
#57529=CARTESIAN_POINT('Ctrl Pts',(3.49827260555614,-0.158333333333296,
10.0412853620192));
#57530=CARTESIAN_POINT('Ctrl Pts',(3.515186898278,0.158333333333298,10.0206766993231));
#57531=CARTESIAN_POINT('Ctrl Pts',(3.55086120578275,0.319434907277093,10.0287266459559));
#57532=CARTESIAN_POINT('Ctrl Pts',(3.62233062874898,0.636309800095061,10.0522310448285));
#57533=CARTESIAN_POINT('Ctrl Pts',(3.68168671424421,0.794772684000661,10.0778898702516));
#57534=CARTESIAN_POINT('Ctrl Pts',(3.7547029246493,1.06847604194556,10.1228699535018));
#57535=CARTESIAN_POINT('Ctrl Pts',(3.78380047762748,1.18514270861286,10.144941328333));
#57536=CARTESIAN_POINT('Ctrl Pts',(3.81038957161665,1.30000000000171,10.1696138666328));
#57537=CARTESIAN_POINT('Ctrl Pts',(3.65042204492736,-1.29999999999978,10.3384258601433));
#57538=CARTESIAN_POINT('Ctrl Pts',(3.63209486961421,-1.18514270861158,10.2990618837114));
#57539=CARTESIAN_POINT('Ctrl Pts',(3.61286153133498,-1.06847604194492,10.2614783916334));
#57540=CARTESIAN_POINT('Ctrl Pts',(3.56633525456491,-0.794772684000693,
10.1787662814238));
#57541=CARTESIAN_POINT('Ctrl Pts',(3.52740334221702,-0.636309800095068,
10.1281600041754));
#57542=CARTESIAN_POINT('Ctrl Pts',(3.49104594994429,-0.319434907277094,
10.0612870409283));
#57543=CARTESIAN_POINT('Ctrl Pts',(3.47317522219543,-0.1583333333333,10.0333749380405));
#57544=CARTESIAN_POINT('Ctrl Pts',(3.49016458763537,0.158333333333302,10.0126203440089));
#57545=CARTESIAN_POINT('Ctrl Pts',(3.52488674318907,0.3194349072771,10.0200149695696));
#57546=CARTESIAN_POINT('Ctrl Pts',(3.59613121861891,0.636309800095075,10.0441293295008));
#57547=CARTESIAN_POINT('Ctrl Pts',(3.65419761495957,0.794772684000681,10.0707537876965));
#57548=CARTESIAN_POINT('Ctrl Pts',(3.73039928648562,1.06847604194558,10.1176424164178));
#57549=CARTESIAN_POINT('Ctrl Pts',(3.76184998177745,1.18514270861289,10.1407124916779));
#57550=CARTESIAN_POINT('Ctrl Pts',(3.79176649230761,1.30000000000173,10.1665562922197));
#57551=CARTESIAN_POINT('Ctrl Pts',(3.63654746083435,-1.2999999999998,10.333034031973));
#57552=CARTESIAN_POINT('Ctrl Pts',(3.61550547136668,-1.18514270861159,10.2926301002341));
#57553=CARTESIAN_POINT('Ctrl Pts',(3.59428098834889,-1.06847604194493,10.2542942008572));
#57554=CARTESIAN_POINT('Ctrl Pts',(3.54482659002603,-0.794772684000701,
10.1705081726912));
#57555=CARTESIAN_POINT('Ctrl Pts',(3.50633075381572,-0.636309800095076,
10.1202089866768));
#57556=CARTESIAN_POINT('Ctrl Pts',(3.4699133232566,-0.319434907277098,10.0532488577123));
#57557=CARTESIAN_POINT('Ctrl Pts',(3.45318708873705,-0.158333333333302,
10.0252571936496));
#57558=CARTESIAN_POINT('Ctrl Pts',(3.46993367159814,0.158333333333304,10.0048871610833));
#57559=CARTESIAN_POINT('Ctrl Pts',(3.5032635327371,0.319434907277105,10.0127351329886));
#57560=CARTESIAN_POINT('Ctrl Pts',(3.5740837383614,0.636309800095084,10.0377419331908));
#57561=CARTESIAN_POINT('Ctrl Pts',(3.63128566085972,0.79477268400069,10.0648118403662));
#57562=CARTESIAN_POINT('Ctrl Pts',(3.71032993277458,1.06847604194559,10.1129544035429));
#57563=CARTESIAN_POINT('Ctrl Pts',(3.74384697749113,1.18514270861291,10.1366687284428));
#57564=CARTESIAN_POINT('Ctrl Pts',(3.77666573049112,1.30000000000175,10.163258246501));
#57565=CARTESIAN_POINT('Ctrl Pts',(3.62446370502867,-1.29999999999981,10.3302238019512));
#57566=CARTESIAN_POINT('Ctrl Pts',(3.60122766761322,-1.18514270861159,10.2890330237839));
#57567=CARTESIAN_POINT('Ctrl Pts',(3.57844949673732,-1.06847604194493,10.2500408126944));
#57568=CARTESIAN_POINT('Ctrl Pts',(3.52688512855879,-0.794772684000705,
10.1650401344845));
#57569=CARTESIAN_POINT('Ctrl Pts',(3.48917206155801,-0.636309800095079,
10.1142973381355));
#57570=CARTESIAN_POINT('Ctrl Pts',(3.45299373509218,-0.3194349072771,10.046822738906));
#57571=CARTESIAN_POINT('Ctrl Pts',(3.43720357052491,-0.158333333333303,
10.0187504466707));
#57572=CARTESIAN_POINT('Ctrl Pts',(3.4537702078461,0.158333333333305,9.99866359183929));
#57573=CARTESIAN_POINT('Ctrl Pts',(3.48590490068051,0.319434907277106,10.0069760041332));
#57574=CARTESIAN_POINT('Ctrl Pts',(3.55628069468287,0.636309800095087,10.0328691020645));
#57575=CARTESIAN_POINT('Ctrl Pts',(3.61260245590577,0.794772684000694,10.0606382417998));
#57576=CARTESIAN_POINT('Ctrl Pts',(3.69401004463299,1.0684760419456,10.109639868439));
#57577=CARTESIAN_POINT('Ctrl Pts',(3.72928544829501,1.18514270861291,10.1336918740997));
#57578=CARTESIAN_POINT('Ctrl Pts',(3.76459792690738,1.30000000000176,10.1605848969381));
#57579=CARTESIAN_POINT('Ctrl Pts',(3.60720160452376,-1.29999999999982,10.3246930658666));
#57580=CARTESIAN_POINT('Ctrl Pts',(3.58063922988522,-1.18514270861161,10.2823745958345));
#57581=CARTESIAN_POINT('Ctrl Pts',(3.55547182313521,-1.06847604194495,10.2424875527587));
#57582=CARTESIAN_POINT('Ctrl Pts',(3.50055273370511,-0.794772684000714,
10.155957586552));
#57583=CARTESIAN_POINT('Ctrl Pts',(3.46384163195749,-0.636309800095088,
10.104820967497));
#57584=CARTESIAN_POINT('Ctrl Pts',(3.42770026301507,-0.319434907277105,
10.0370681906501));
#57585=CARTESIAN_POINT('Ctrl Pts',(3.41292545540548,-0.158333333333305,
10.0094712140234));
#57586=CARTESIAN_POINT('Ctrl Pts',(3.42927917675529,0.158333333333307,9.98970646933673));
#57587=CARTESIAN_POINT('Ctrl Pts',(3.46011271931971,0.319434907277111,9.99795680932176));
#57588=CARTESIAN_POINT('Ctrl Pts',(3.53016630719154,0.636309800095096,10.024598568368));
#57589=CARTESIAN_POINT('Ctrl Pts',(3.58554467377616,0.794772684000705,10.0527059489922));
#57590=CARTESIAN_POINT('Ctrl Pts',(3.67010612733831,1.06847604194562,10.1036611532208));
#57591=CARTESIAN_POINT('Ctrl Pts',(3.70765640796908,1.18514270861293,10.1288493866877));
#57592=CARTESIAN_POINT('Ctrl Pts',(3.7461534492941,1.30000000000178,10.1571692337871));
#57593=CARTESIAN_POINT('Ctrl Pts',(3.58378319929592,-1.29999999999985,10.3178735693703));
#57594=CARTESIAN_POINT('Ctrl Pts',(3.55311880004611,-1.18514270861164,10.2735172558038));
#57595=CARTESIAN_POINT('Ctrl Pts',(3.52502338935574,-1.06847604194497,10.2320295366664));
#57596=CARTESIAN_POINT('Ctrl Pts',(3.46605224769,-0.794772684000734,10.142811632861));
#57597=CARTESIAN_POINT('Ctrl Pts',(3.43067766881984,-0.636309800095103,
10.0911930054387));
#57598=CARTESIAN_POINT('Ctrl Pts',(3.39475905345327,-0.319434907277112,
10.0228204783981));
#57599=CARTESIAN_POINT('Ctrl Pts',(3.38152701401965,-0.158333333333309,
9.99557018368774));
#57600=CARTESIAN_POINT('Ctrl Pts',(3.39744303920166,0.158333333333311,9.9764535028626));
#57601=CARTESIAN_POINT('Ctrl Pts',(3.42625716100374,0.31943490727712,9.98498852827799));
#57602=CARTESIAN_POINT('Ctrl Pts',(3.49527579114069,0.636309800095112,10.0136041065402));
#57603=CARTESIAN_POINT('Ctrl Pts',(3.54840272315516,0.794772684000723,10.0438906055675));
#57604=CARTESIAN_POINT('Ctrl Pts',(3.6373929333043,1.06847604194564,10.097067130942));
#57605=CARTESIAN_POINT('Ctrl Pts',(3.6783751929315,1.18514270861296,10.1230878921532));
#57606=CARTESIAN_POINT('Ctrl Pts',(3.72181914762449,1.30000000000182,10.1521112671253));
#57607=CARTESIAN_POINT('Ctrl Pts',(3.56138672197762,-1.29999999999988,10.3095005735531));
#57608=CARTESIAN_POINT('Ctrl Pts',(3.5264945322361,-1.18514270861167,10.2633053010594));
#57609=CARTESIAN_POINT('Ctrl Pts',(3.49537043823022,-1.068476041945,10.2203754927062));
#57610=CARTESIAN_POINT('Ctrl Pts',(3.43217260967728,-0.794772684000756,
10.1287429227498));
#57611=CARTESIAN_POINT('Ctrl Pts',(3.39811853902977,-0.63630980009512,10.0766656342623));
#57612=CARTESIAN_POINT('Ctrl Pts',(3.36231880711828,-0.31943490727712,10.007828718619));
#57613=CARTESIAN_POINT('Ctrl Pts',(3.35051604805238,-0.158333333333313,
9.98109823159642));
#57614=CARTESIAN_POINT('Ctrl Pts',(3.36603468341215,0.158333333333315,9.96255096961667));
#57615=CARTESIAN_POINT('Ctrl Pts',(3.3928274124033,0.319434907277128,9.97140476165473));
#57616=CARTESIAN_POINT('Ctrl Pts',(3.46131434058875,0.636309800095128,10.0010963434057));
#57617=CARTESIAN_POINT('Ctrl Pts',(3.51336861172402,0.794772684000745,10.0314617398297));
#57618=CARTESIAN_POINT('Ctrl Pts',(3.60651490650398,1.06847604194567,10.0872896694177));
#57619=CARTESIAN_POINT('Ctrl Pts',(3.65047241819542,1.18514270861299,10.1149204214575));
#57620=CARTESIAN_POINT('Ctrl Pts',(3.69806786197832,1.30000000000184,10.1460160834469));
#57621=CARTESIAN_POINT('Ctrl Pts',(3.53855149764873,-1.2999999999999,10.3017508966993));
#57622=CARTESIAN_POINT('Ctrl Pts',(3.49941489950663,-1.18514270861168,10.2537129280734));
#57623=CARTESIAN_POINT('Ctrl Pts',(3.46532473422636,-1.06847604194501,10.2092310982888));
#57624=CARTESIAN_POINT('Ctrl Pts',(3.39822790216101,-0.794772684000764,
10.1146845650534));
#57625=CARTESIAN_POINT('Ctrl Pts',(3.3660310219522,-0.636309800095125,10.0613869862023));
#57626=CARTESIAN_POINT('Ctrl Pts',(3.33082756807032,-0.319434907277123,
9.99139500095045));
#57627=CARTESIAN_POINT('Ctrl Pts',(3.32078738128955,-0.158333333333315,
9.96471106885896));
#57628=CARTESIAN_POINT('Ctrl Pts',(3.33573966037722,0.158333333333317,9.94695881112389));
#57629=CARTESIAN_POINT('Ctrl Pts',(3.35992214767888,0.319434907277132,9.95690953203665));
#57630=CARTESIAN_POINT('Ctrl Pts',(3.42723218548264,0.636309800095136,9.98866572202563));
#57631=CARTESIAN_POINT('Ctrl Pts',(3.4776049539938,0.794772684000752,10.020182490244));
#57632=CARTESIAN_POINT('Ctrl Pts',(3.57489815356795,1.06847604194568,10.078696696035));
#57633=CARTESIAN_POINT('Ctrl Pts',(3.62200692329494,1.185142708613,10.1076542382111));
#57634=CARTESIAN_POINT('Ctrl Pts',(3.67410984172149,1.30000000000186,10.1402406910412));
#57635=CARTESIAN_POINT('Ctrl Pts',(3.51929591785351,-1.29999999999997,10.2939294651204));
#57636=CARTESIAN_POINT('Ctrl Pts',(3.47679697345141,-1.18514270861175,10.2438286551357));
#57637=CARTESIAN_POINT('Ctrl Pts',(3.4402855928125,-1.06847604194507,10.1977848253857));
#57638=CARTESIAN_POINT('Ctrl Pts',(3.36976946956097,-0.794772684000805,
10.1007868035652));
#57639=CARTESIAN_POINT('Ctrl Pts',(3.338399999449,-0.636309800095159,10.0476074585909));
#57640=CARTESIAN_POINT('Ctrl Pts',(3.30347328960332,-0.31943490727714,9.97698760693245));
#57641=CARTESIAN_POINT('Ctrl Pts',(3.29508348591708,-0.158333333333323,
9.95018329512672));
#57642=CARTESIAN_POINT('Ctrl Pts',(3.30987058860113,0.158333333333325,9.93261597869159));
#57643=CARTESIAN_POINT('Ctrl Pts',(3.33244160595743,0.31943490727715,9.9425092179148));
#57644=CARTESIAN_POINT('Ctrl Pts',(3.39872273155985,0.63630980009517,9.97600898940697));
#57645=CARTESIAN_POINT('Ctrl Pts',(3.4470306553148,0.794772684000795,10.0093452012326));
#57646=CARTESIAN_POINT('Ctrl Pts',(3.54741396098122,1.06847604194573,10.0709607253317));
#57647=CARTESIAN_POINT('Ctrl Pts',(3.5970435863886,1.18514270861306,10.1014181357824));
#57648=CARTESIAN_POINT('Ctrl Pts',(3.65285062374829,1.30000000000192,10.1356618793814));
#57649=CARTESIAN_POINT('Ctrl Pts',(3.49657587699451,-1.29999999999997,10.2859305508819));
#57650=CARTESIAN_POINT('Ctrl Pts',(3.45002544710238,-1.18514270861174,10.2336461217128));
#57651=CARTESIAN_POINT('Ctrl Pts',(3.41074789121993,-1.06847604194507,10.1857246550423));
#57652=CARTESIAN_POINT('Ctrl Pts',(3.33681067357917,-0.794772684000805,
10.085095796556));
#57653=CARTESIAN_POINT('Ctrl Pts',(3.30793311972073,-0.63630980009516,10.0298699456148));
#57654=CARTESIAN_POINT('Ctrl Pts',(3.27349123802796,-0.319434907277141,
9.95827558428957));
#57655=CARTESIAN_POINT('Ctrl Pts',(3.2658527784058,-0.158333333333323,9.93297551112294));
#57656=CARTESIAN_POINT('Ctrl Pts',(3.27998125659245,0.158333333333325,9.91627742782468));
#57657=CARTESIAN_POINT('Ctrl Pts',(3.3006655020231,0.319434907277149,9.92615406278584));
#57658=CARTESIAN_POINT('Ctrl Pts',(3.36609144291574,0.63630980009517,9.96113927045787));
#57659=CARTESIAN_POINT('Ctrl Pts',(3.4127066905504,0.794772684000796,9.99550087406892));
#57660=CARTESIAN_POINT('Ctrl Pts',(3.51714884489834,1.06847604194574,10.0599476959581));
#57661=CARTESIAN_POINT('Ctrl Pts',(3.56984258657858,1.18514270861306,10.091908326306));
#57662=CARTESIAN_POINT('Ctrl Pts',(3.63002093128492,1.30000000000192,10.1279329457959));
#57663=CARTESIAN_POINT('Ctrl Pts',(3.4802295000654,-1.3,10.2789860295797));
#57664=CARTESIAN_POINT('Ctrl Pts',(3.43091440205945,-1.18514270861177,10.2247844835619));
#57665=CARTESIAN_POINT('Ctrl Pts',(3.38968103217071,-1.06847604194509,10.175373649079));
#57666=CARTESIAN_POINT('Ctrl Pts',(3.31309410771521,-0.794772684000823,
10.0722922388441));
#57667=CARTESIAN_POINT('Ctrl Pts',(3.28513733028894,-0.636309800095174,
10.0169134300136));
#57668=CARTESIAN_POINT('Ctrl Pts',(3.25116537962811,-0.319434907277147,
9.94448213163101));
#57669=CARTESIAN_POINT('Ctrl Pts',(3.24507410638107,-0.158333333333326,
9.91889631942219));
#57670=CARTESIAN_POINT('Ctrl Pts',(3.25900350812188,0.158333333333329,9.90241295720868));
#57671=CARTESIAN_POINT('Ctrl Pts',(3.27802168356298,0.319434907277155,9.91261429661292));
#57672=CARTESIAN_POINT('Ctrl Pts',(3.34240884201399,0.636309800095183,9.94923181440477));
#57673=CARTESIAN_POINT('Ctrl Pts',(3.38741908809698,0.794772684000813,9.98480266593302));
#57674=CARTESIAN_POINT('Ctrl Pts',(3.49424009078888,1.06847604194576,10.0522670360987));
#57675=CARTESIAN_POINT('Ctrl Pts',(3.548901837997,1.18514270861309,10.0858023098939));
#57676=CARTESIAN_POINT('Ctrl Pts',(3.61198647845601,1.30000000000195,10.1236700314407));
#57677=CARTESIAN_POINT('Ctrl Pts',(3.46380404043217,-1.30000000000001,10.2720051436094));
#57678=CARTESIAN_POINT('Ctrl Pts',(3.41143469758712,-1.18514270861178,10.2160283216677));
#57679=CARTESIAN_POINT('Ctrl Pts',(3.36815068395304,-1.0684760419451,10.1650646631163));
#57680=CARTESIAN_POINT('Ctrl Pts',(3.2891448815123,-0.79477268400083,10.0589098269297));
#57681=CARTESIAN_POINT('Ctrl Pts',(3.2637249951748,-0.63630980009518,10.0011599660398));
#57682=CARTESIAN_POINT('Ctrl Pts',(3.22953275013871,-0.319434907277151,
9.92878866647668));
#57683=CARTESIAN_POINT('Ctrl Pts',(3.22230664903844,-0.158333333333328,
9.90666524664121));
#57684=CARTESIAN_POINT('Ctrl Pts',(3.2354888075062,0.15833333333333,9.89114113457973));
#57685=CARTESIAN_POINT('Ctrl Pts',(3.25440572980874,0.319434907277158,9.89944511143236));
#57686=CARTESIAN_POINT('Ctrl Pts',(3.31848682912671,0.636309800095189,9.93672262432642));
#57687=CARTESIAN_POINT('Ctrl Pts',(3.36175770004629,0.79477268400082,9.97370681958844));
#57688=CARTESIAN_POINT('Ctrl Pts',(3.47142677497237,1.06847604194577,10.0437803832112));
#57689=CARTESIAN_POINT('Ctrl Pts',(3.5283166481924,1.1851427086131,10.078680079522));
#57690=CARTESIAN_POINT('Ctrl Pts',(3.59462471573652,1.30000000000196,10.1181472229327));
#57691=CARTESIAN_POINT('Ctrl Pts',(3.45022017105532,-1.30000000000002,10.2662412177575));
#57692=CARTESIAN_POINT('Ctrl Pts',(3.39606660535214,-1.18514270861179,10.2081259394358));
#57693=CARTESIAN_POINT('Ctrl Pts',(3.35136323908567,-1.06847604194511,10.1557680049425));
#57694=CARTESIAN_POINT('Ctrl Pts',(3.26992137133707,-0.794772684000838,
10.04811131809));
#57695=CARTESIAN_POINT('Ctrl Pts',(3.2438885726079,-0.636309800095184,9.99214438464443));
#57696=CARTESIAN_POINT('Ctrl Pts',(3.20916354990404,-0.319434907277152,
9.92045275636352));
#57697=CARTESIAN_POINT('Ctrl Pts',(3.20258479929904,-0.158333333333329,
9.89903738322094));
#57698=CARTESIAN_POINT('Ctrl Pts',(3.21612697191109,0.158333333333331,9.88298698307226));
#57699=CARTESIAN_POINT('Ctrl Pts',(3.23530727064128,0.319434907277161,9.88928439861708));
#57700=CARTESIAN_POINT('Ctrl Pts',(3.29953270823961,0.636309800095194,9.92638319912416));
#57701=CARTESIAN_POINT('Ctrl Pts',(3.34140180159176,0.794772684000824,9.96433113446368));
#57702=CARTESIAN_POINT('Ctrl Pts',(3.45322975452854,1.06847604194578,10.036354963907));
#57703=CARTESIAN_POINT('Ctrl Pts',(3.51178755380993,1.18514270861311,10.072358936718));
#57704=CARTESIAN_POINT('Ctrl Pts',(3.58049697518027,1.30000000000198,10.1131904353198));
#57705=CARTESIAN_POINT('Ctrl Pts',(3.43423105359299,-1.30000000000003,10.258649491102));
#57706=CARTESIAN_POINT('Ctrl Pts',(3.37760262054861,-1.1851427086118,10.1977714595931));
#57707=CARTESIAN_POINT('Ctrl Pts',(3.33083250059634,-1.06847604194512,10.1437157323749));
#57708=CARTESIAN_POINT('Ctrl Pts',(3.2455588425677,-0.794772684000841,10.0345970763986));
#57709=CARTESIAN_POINT('Ctrl Pts',(3.21800531622045,-0.636309800095188,
9.98161924932007));
#57710=CARTESIAN_POINT('Ctrl Pts',(3.18185839235816,-0.319434907277154,
9.91157187300279));
#57711=CARTESIAN_POINT('Ctrl Pts',(3.17601680631054,-0.15833333333333,9.89127734987168));
#57712=CARTESIAN_POINT('Ctrl Pts',(3.18947052405278,0.158333333333332,9.87531030441977));
#57713=CARTESIAN_POINT('Ctrl Pts',(3.20799409399132,0.319434907277162,9.88030865988734));
#57714=CARTESIAN_POINT('Ctrl Pts',(3.27311723848317,0.636309800095197,9.91646578453442));
#57715=CARTESIAN_POINT('Ctrl Pts',(3.315456288054,0.794772684000828,9.95289384391755));
#57716=CARTESIAN_POINT('Ctrl Pts',(3.43106717232058,1.06847604194578,10.0265379844801));
#57717=CARTESIAN_POINT('Ctrl Pts',(3.49191566964394,1.18514270861312,10.0639884215424));
#57718=CARTESIAN_POINT('Ctrl Pts',(3.56356899629696,1.30000000000199,10.1070114760016));
#57719=CARTESIAN_POINT('Ctrl Pts',(3.42329004793795,-1.30000000000005,10.2535552330257));
#57720=CARTESIAN_POINT('Ctrl Pts',(3.36577675441716,-1.18514270861181,10.1896775761705));
#57721=CARTESIAN_POINT('Ctrl Pts',(3.31797563071956,-1.06847604194513,10.1340934433128));
#57722=CARTESIAN_POINT('Ctrl Pts',(3.22998252760056,-0.794772684000851,
10.0248426763922));
#57723=CARTESIAN_POINT('Ctrl Pts',(3.19945051412027,-0.636309800095197,
9.97773483060053));
#57724=CARTESIAN_POINT('Ctrl Pts',(3.16161671560349,-0.319434907277159,
9.91074553869703));
#57725=CARTESIAN_POINT('Ctrl Pts',(3.15675867153595,-0.158333333333332,
9.89088328778878));
#57726=CARTESIAN_POINT('Ctrl Pts',(3.17014714941586,0.158333333333334,9.8750691093734));
#57727=CARTESIAN_POINT('Ctrl Pts',(3.18775359149335,0.319434907277167,9.87971474161891));
#57728=CARTESIAN_POINT('Ctrl Pts',(3.25416255205695,0.636309800095206,9.91327450455847));
#57729=CARTESIAN_POINT('Ctrl Pts',(3.29862160463217,0.79477268400084,9.94456294634815));
#57730=CARTESIAN_POINT('Ctrl Pts',(3.41699686809867,1.0684760419458,10.0182954880635));
#57731=CARTESIAN_POINT('Ctrl Pts',(3.47911206103839,1.18514270861313,10.0570584190905));
#57732=CARTESIAN_POINT('Ctrl Pts',(3.55210218159882,1.300000000002,10.1026681958956));
#57733=CARTESIAN_POINT('Ctrl Pts',(3.41475847117042,-1.30000000000005,10.2524562333547));
#57734=CARTESIAN_POINT('Ctrl Pts',(3.3574890695822,-1.18514270861181,10.1886391816766));
#57735=CARTESIAN_POINT('Ctrl Pts',(3.30972802388307,-1.06847604194513,10.133397568411));
#57736=CARTESIAN_POINT('Ctrl Pts',(3.22135665799747,-0.794772684000851,
10.0255893689635));
#57737=CARTESIAN_POINT('Ctrl Pts',(3.18969432988981,-0.636309800095197,
9.98078487986184));
#57738=CARTESIAN_POINT('Ctrl Pts',(3.15117622767193,-0.319434907277159,
9.91533710840653));
#57739=CARTESIAN_POINT('Ctrl Pts',(3.14628700527777,-0.158333333333332,
9.89543280925802));
#57740=CARTESIAN_POINT('Ctrl Pts',(3.15959962456677,0.158333333333334,9.87984298008964));
#57741=CARTESIAN_POINT('Ctrl Pts',(3.17704490789093,0.319434907277167,9.88500970337775));
#57742=CARTESIAN_POINT('Ctrl Pts',(3.24422091196343,0.636309800095206,9.91696613669794));
#57743=CARTESIAN_POINT('Ctrl Pts',(3.29031662464091,0.79477268400084,9.94499299784744));
#57744=CARTESIAN_POINT('Ctrl Pts',(3.40898836153082,1.0684760419458,10.0174129929739));
#57745=CARTESIAN_POINT('Ctrl Pts',(3.47090355779047,1.18514270861313,10.0561105004451));
#57746=CARTESIAN_POINT('Ctrl Pts',(3.54336535263118,1.300000000002,10.1021575829223));
#57747=CARTESIAN_POINT('Ctrl Pts',(3.4147584711704,-1.3,10.2524562333546));
#57748=CARTESIAN_POINT('Ctrl Pts',(3.35748906958219,-1.18514270861178,10.1886391816766));
#57749=CARTESIAN_POINT('Ctrl Pts',(3.30972802388306,-1.06847604194512,10.133397568411));
#57750=CARTESIAN_POINT('Ctrl Pts',(3.22135665799747,-0.794772684000851,
10.0255893689635));
#57751=CARTESIAN_POINT('Ctrl Pts',(3.18969432988981,-0.636309800095197,
9.98078487986184));
#57752=CARTESIAN_POINT('Ctrl Pts',(3.15117622767193,-0.319434907277159,
9.91533710840653));
#57753=CARTESIAN_POINT('Ctrl Pts',(3.14628700527777,-0.158333333333332,
9.89543280925802));
#57754=CARTESIAN_POINT('Ctrl Pts',(3.15959962456677,0.158333333333334,9.87984298008964));
#57755=CARTESIAN_POINT('Ctrl Pts',(3.17704490789093,0.319434907277167,9.88500970337774));
#57756=CARTESIAN_POINT('Ctrl Pts',(3.24422091196343,0.636309800095206,9.91696613669794));
#57757=CARTESIAN_POINT('Ctrl Pts',(3.29031662464091,0.79477268400084,9.94499299784744));
#57758=CARTESIAN_POINT('Ctrl Pts',(3.40898836153052,1.06847604194511,10.0174129929737));
#57759=CARTESIAN_POINT('Ctrl Pts',(3.47090355778975,1.18514270861178,10.0561105004446));
#57760=CARTESIAN_POINT('Ctrl Pts',(3.54336535262991,1.3,10.1021575829215));
#57761=CARTESIAN_POINT('',(3.81826036790159,-1.2,10.3501409115962));
#57762=CARTESIAN_POINT('Ctrl Pts',(3.81826036790159,-1.2,10.3501409115962));
#57763=CARTESIAN_POINT('Ctrl Pts',(3.79666911560247,-1.21682679214414,10.3498705750651));
#57764=CARTESIAN_POINT('Ctrl Pts',(3.77476187409666,-1.23325258729674,10.3505181001901));
#57765=CARTESIAN_POINT('Ctrl Pts',(3.74202710674506,-1.25864657309861,10.3500191474087));
#57766=CARTESIAN_POINT('Ctrl Pts',(3.7314954635025,-1.26676751286954,10.3499115167687));
#57767=CARTESIAN_POINT('Ctrl Pts',(3.71258831258587,-1.28141947219131,10.3495705776323));
#57768=CARTESIAN_POINT('Ctrl Pts',(3.69913033630965,-1.29187184462129,10.3492642451596));
#57769=CARTESIAN_POINT('Ctrl Pts',(3.69072511418734,-1.298457549969,10.348970093154));
#57770=CARTESIAN_POINT('Ctrl Pts',(3.68974253591884,-1.29922936208746,10.3489325435325));
#57771=CARTESIAN_POINT('Ctrl Pts',(3.68876499475237,-1.29999999999972,10.3488907274614));
#57772=CARTESIAN_POINT('',(3.91593538932197,-0.653834841327623,10.227862286537));
#57773=CARTESIAN_POINT('Ctrl Pts',(3.9159353893185,-0.653834841312177,10.2278622866113));
#57774=CARTESIAN_POINT('Ctrl Pts',(3.90700550388882,-0.711393414252494,
10.2394113106641));
#57775=CARTESIAN_POINT('Ctrl Pts',(3.89748289441163,-0.767209744945321,
10.2516191953437));
#57776=CARTESIAN_POINT('Ctrl Pts',(3.87754062849598,-0.881633194810645,
10.2769213651307));
#57777=CARTESIAN_POINT('Ctrl Pts',(3.86793349028196,-0.939021993186391,
10.2890044992134));
#57778=CARTESIAN_POINT('Ctrl Pts',(3.84975474046838,-1.03714157084077,10.3115895811745));
#57779=CARTESIAN_POINT('Ctrl Pts',(3.84918980540933,-1.03956975094,10.3123276742784));
#57780=CARTESIAN_POINT('Ctrl Pts',(3.83021697552951,-1.13871235067932,10.3356129960789));
#57781=CARTESIAN_POINT('Ctrl Pts',(3.82499289590527,-1.16608643702209,10.3419804687545));
#57782=CARTESIAN_POINT('Ctrl Pts',(3.81826036790159,-1.2,10.3501409115962));
#57783=CARTESIAN_POINT('',(3.99970644340964,0.653834841531101,10.1163073168902));
#57784=CARTESIAN_POINT('Ctrl Pts',(3.99970644340962,0.653834841531101,10.1163073168902));
#57785=CARTESIAN_POINT('Ctrl Pts',(3.95879318609505,0.575732021690897,10.1082141213102));
#57786=CARTESIAN_POINT('Ctrl Pts',(3.9241762431234,0.493687875304555,10.1023287044845));
#57787=CARTESIAN_POINT('Ctrl Pts',(3.8739058242527,0.33806901713317,10.0960431987292));
#57788=CARTESIAN_POINT('Ctrl Pts',(3.85599434530751,0.26561107497815,10.095104067982));
#57789=CARTESIAN_POINT('Ctrl Pts',(3.83175003836914,0.129684465390305,10.0980902516012));
#57790=CARTESIAN_POINT('Ctrl Pts',(3.82414429286697,0.0666362255820432,
10.1012767240369));
#57791=CARTESIAN_POINT('Ctrl Pts',(3.81587160814996,-0.0594727714086463,
10.111667545938));
#57792=CARTESIAN_POINT('Ctrl Pts',(3.81513703688267,-0.122669468213772,
10.118928970212));
#57793=CARTESIAN_POINT('Ctrl Pts',(3.82170332152409,-0.260037978472135,
10.1384960942812));
#57794=CARTESIAN_POINT('Ctrl Pts',(3.83047324685118,-0.333902761432303,
10.1515184133504));
#57795=CARTESIAN_POINT('Ctrl Pts',(3.86128895474085,-0.491493501304615,
10.1841880364153));
#57796=CARTESIAN_POINT('Ctrl Pts',(3.88528595310545,-0.574905758777795,
10.2050069107913));
#57797=CARTESIAN_POINT('Ctrl Pts',(3.91593538921434,-0.653834841350336,
10.2278622866029));
#57798=CARTESIAN_POINT('',(3.95671216659572,1.2,10.1743787302079));
#57799=CARTESIAN_POINT('Ctrl Pts',(3.95671216659571,1.2,10.1743787302079));
#57800=CARTESIAN_POINT('Ctrl Pts',(3.96397347835393,1.13608680445646,10.1647192607237));
#57801=CARTESIAN_POINT('Ctrl Pts',(3.97397889641972,1.03790262443427,10.1513283596737));
#57802=CARTESIAN_POINT('Ctrl Pts',(3.9927072208627,0.79689965730155,10.1259111994147));
#57803=CARTESIAN_POINT('Ctrl Pts',(3.99584992410113,0.741366419488911,10.1215965211651));
#57804=CARTESIAN_POINT('Ctrl Pts',(3.99970644340962,0.653834841531098,10.1163073168902));
#57805=CARTESIAN_POINT('Ctrl Pts',(3.83165700304165,1.29999999999992,10.1733658723815));
#57806=CARTESIAN_POINT('Ctrl Pts',(3.85238006927995,1.28313652450894,10.1741677159342));
#57807=CARTESIAN_POINT('Ctrl Pts',(3.87334649564944,1.26654461476687,10.1741346610164));
#57808=CARTESIAN_POINT('Ctrl Pts',(3.90825716504668,1.23847808482738,10.1746669753888));
#57809=CARTESIAN_POINT('Ctrl Pts',(3.93166057066595,1.21946611443686,10.1753082311882));
#57810=CARTESIAN_POINT('Ctrl Pts',(3.95671216659572,1.2,10.1743787302079));
#57811=CARTESIAN_POINT('Ctrl Pts',(3.4147584711704,-1.3,10.2524562333546));
#57812=CARTESIAN_POINT('Ctrl Pts',(3.35748906958219,-1.18514270861178,10.1886391816766));
#57813=CARTESIAN_POINT('Ctrl Pts',(3.30972802388306,-1.06847604194512,10.133397568411));
#57814=CARTESIAN_POINT('Ctrl Pts',(3.22135665799746,-0.794772684000851,
10.0255893689635));
#57815=CARTESIAN_POINT('Ctrl Pts',(3.18969432988981,-0.636309800095197,
9.98078487986184));
#57816=CARTESIAN_POINT('Ctrl Pts',(3.15117622767193,-0.319434907277159,
9.91533710840652));
#57817=CARTESIAN_POINT('Ctrl Pts',(3.14628700527777,-0.158333333333332,
9.89543280925802));
#57818=CARTESIAN_POINT('Ctrl Pts',(3.15959962456677,0.158333333333334,9.87984298008963));
#57819=CARTESIAN_POINT('Ctrl Pts',(3.17704490789093,0.319434907277167,9.88500970337774));
#57820=CARTESIAN_POINT('Ctrl Pts',(3.24422091196343,0.636309800095206,9.91696613669794));
#57821=CARTESIAN_POINT('Ctrl Pts',(3.29031662464091,0.79477268400084,9.94499299784744));
#57822=CARTESIAN_POINT('Ctrl Pts',(3.40898836153052,1.06847604194511,10.0174129929737));
#57823=CARTESIAN_POINT('Ctrl Pts',(3.47090355778975,1.18514270861178,10.0561105004446));
#57824=CARTESIAN_POINT('Ctrl Pts',(3.54336535262991,1.3,10.1021575829215));
#57825=CARTESIAN_POINT('Ctrl Pts',(3.3620529124905,-1.3,10.3085029402952));
#57826=CARTESIAN_POINT('Ctrl Pts',(3.30608359416459,-1.18514270861178,10.2435410355842));
#57827=CARTESIAN_POINT('Ctrl Pts',(3.25925709076723,-1.06847604194512,10.1875362842913));
#57828=CARTESIAN_POINT('Ctrl Pts',(3.17220023180818,-0.794772684000851,
10.0788469213604));
#57829=CARTESIAN_POINT('Ctrl Pts',(3.14019479937607,-0.636309800095197,
10.0346727316879));
#57830=CARTESIAN_POINT('Ctrl Pts',(3.10158167219449,-0.319434907277159,
9.96988500070868));
#57831=CARTESIAN_POINT('Ctrl Pts',(3.09600154123355,-0.158333333333332,
9.95101225241256));
#57832=CARTESIAN_POINT('Ctrl Pts',(3.10958091369844,0.158333333333334,9.93566260888257));
#57833=CARTESIAN_POINT('Ctrl Pts',(3.12797987732074,0.319434907277167,9.94003438204794));
#57834=CARTESIAN_POINT('Ctrl Pts',(3.19580237328514,0.636309800095206,9.97182731794448));
#57835=CARTESIAN_POINT('Ctrl Pts',(3.24248906837777,0.79477268400084,9.99944707010018));
#57836=CARTESIAN_POINT('Ctrl Pts',(3.36042187227873,1.06847604194511,10.0732664778114));
#57837=CARTESIAN_POINT('Ctrl Pts',(3.42167579733126,1.18514270861178,10.1129731777087));
#57838=CARTESIAN_POINT('Ctrl Pts',(3.49313490646867,1.3,10.1604328911839));
#57839=CARTESIAN_POINT('Ctrl Pts',(3.3093473538106,-1.3,10.3645496472358));
#57840=CARTESIAN_POINT('Ctrl Pts',(3.25467811874699,-1.18514270861178,10.2984428894918));
#57841=CARTESIAN_POINT('Ctrl Pts',(3.20878615765139,-1.06847604194512,10.2416750001716));
#57842=CARTESIAN_POINT('Ctrl Pts',(3.12304380561889,-0.794772684000851,
10.1321044737573));
#57843=CARTESIAN_POINT('Ctrl Pts',(3.09069526886232,-0.636309800095197,
10.0885605835139));
#57844=CARTESIAN_POINT('Ctrl Pts',(3.05198711671704,-0.319434907277159,
10.0244328930108));
#57845=CARTESIAN_POINT('Ctrl Pts',(3.04571607718934,-0.158333333333332,
10.0065916955671));
#57846=CARTESIAN_POINT('Ctrl Pts',(3.05956220283012,0.158333333333334,9.99148223767551));
#57847=CARTESIAN_POINT('Ctrl Pts',(3.07891484675056,0.319434907277167,9.99505906071815));
#57848=CARTESIAN_POINT('Ctrl Pts',(3.14738383460685,0.636309800095206,10.026688499191));
#57849=CARTESIAN_POINT('Ctrl Pts',(3.19466151211463,0.79477268400084,10.0539011423529));
#57850=CARTESIAN_POINT('Ctrl Pts',(3.31185538302693,1.06847604194511,10.129119962649));
#57851=CARTESIAN_POINT('Ctrl Pts',(3.37244803687278,1.18514270861178,10.1698358549729));
#57852=CARTESIAN_POINT('Ctrl Pts',(3.44290446030743,1.3,10.2187081994464));
#57853=CARTESIAN_POINT('Ctrl Pts',(3.25664179513071,-1.3,10.4205963541764));
#57854=CARTESIAN_POINT('Ctrl Pts',(3.20327264332939,-1.18514270861178,10.3533447433995));
#57855=CARTESIAN_POINT('Ctrl Pts',(3.15831522453555,-1.06847604194512,10.2958137160519));
#57856=CARTESIAN_POINT('Ctrl Pts',(3.0738873794296,-0.794772684000851,10.1853620261542));
#57857=CARTESIAN_POINT('Ctrl Pts',(3.04119573834857,-0.636309800095197,
10.14244843534));
#57858=CARTESIAN_POINT('Ctrl Pts',(3.0023925612396,-0.319434907277159,10.078980785313));
#57859=CARTESIAN_POINT('Ctrl Pts',(2.99543061314513,-0.158333333333332,
10.0621711387217));
#57860=CARTESIAN_POINT('Ctrl Pts',(3.00954349196179,0.158333333333334,10.0473018664684));
#57861=CARTESIAN_POINT('Ctrl Pts',(3.02984981618037,0.319434907277167,10.0500837393884));
#57862=CARTESIAN_POINT('Ctrl Pts',(3.09896529592856,0.636309800095206,10.0815496804376));
#57863=CARTESIAN_POINT('Ctrl Pts',(3.14683395585149,0.79477268400084,10.1083552146057));
#57864=CARTESIAN_POINT('Ctrl Pts',(3.26328889377514,1.06847604194511,10.1849734474866));
#57865=CARTESIAN_POINT('Ctrl Pts',(3.32322027641429,1.18514270861178,10.226698532237));
#57866=CARTESIAN_POINT('Ctrl Pts',(3.39267401414619,1.3,10.2769835077089));
#57867=CARTESIAN_POINT('Ctrl Pts',(3.2566417951307,-1.3,10.4205963541764));
#57868=CARTESIAN_POINT('Ctrl Pts',(3.20327264332939,-1.18514270861178,10.3533447433995));
#57869=CARTESIAN_POINT('Ctrl Pts',(3.15831522453555,-1.06847604194512,10.2958137160519));
#57870=CARTESIAN_POINT('Ctrl Pts',(3.0738873794296,-0.794772684000851,10.1853620261542));
#57871=CARTESIAN_POINT('Ctrl Pts',(3.04119573834857,-0.636309800095197,
10.14244843534));
#57872=CARTESIAN_POINT('Ctrl Pts',(3.0023925612396,-0.319434907277159,10.078980785313));
#57873=CARTESIAN_POINT('Ctrl Pts',(2.99543061314513,-0.158333333333332,
10.0621711387217));
#57874=CARTESIAN_POINT('Ctrl Pts',(3.00954349196179,0.158333333333334,10.0473018664685));
#57875=CARTESIAN_POINT('Ctrl Pts',(3.02984981618038,0.319434907277167,10.0500837393884));
#57876=CARTESIAN_POINT('Ctrl Pts',(3.09896529592856,0.636309800095206,10.0815496804376));
#57877=CARTESIAN_POINT('Ctrl Pts',(3.14683395585149,0.79477268400084,10.1083552146057));
#57878=CARTESIAN_POINT('Ctrl Pts',(3.26328889377514,1.06847604194511,10.1849734474866));
#57879=CARTESIAN_POINT('Ctrl Pts',(3.32322027641429,1.18514270861178,10.226698532237));
#57880=CARTESIAN_POINT('Ctrl Pts',(3.39267401414619,1.3,10.2769835077089));
#57881=CARTESIAN_POINT('Ctrl Pts',(3.25664179513082,-1.30000000000024,10.4205963541766));
#57882=CARTESIAN_POINT('Ctrl Pts',(3.20327264332946,-1.18514270861195,10.3533447433995));
#57883=CARTESIAN_POINT('Ctrl Pts',(3.15831522453558,-1.0684760419452,10.2958137160519));
#57884=CARTESIAN_POINT('Ctrl Pts',(3.0738873794296,-0.794772684000852,10.1853620261542));
#57885=CARTESIAN_POINT('Ctrl Pts',(3.04119573834858,-0.636309800095197,
10.14244843534));
#57886=CARTESIAN_POINT('Ctrl Pts',(3.0023925612396,-0.319434907277159,10.078980785313));
#57887=CARTESIAN_POINT('Ctrl Pts',(2.99543061314513,-0.158333333333333,
10.0621711387217));
#57888=CARTESIAN_POINT('Ctrl Pts',(3.00954349196179,0.158333333333334,10.0473018664685));
#57889=CARTESIAN_POINT('Ctrl Pts',(3.02984981618038,0.319434907277167,10.0500837393884));
#57890=CARTESIAN_POINT('Ctrl Pts',(3.09896529592856,0.636309800095206,10.0815496804376));
#57891=CARTESIAN_POINT('Ctrl Pts',(3.14683395585149,0.79477268400084,10.1083552146057));
#57892=CARTESIAN_POINT('Ctrl Pts',(3.26328889377515,1.06847604194515,10.1849734474866));
#57893=CARTESIAN_POINT('Ctrl Pts',(3.32322027641433,1.18514270861185,10.226698532237));
#57894=CARTESIAN_POINT('Ctrl Pts',(3.39267401414626,1.30000000000011,10.276983507709));
#57895=CARTESIAN_POINT('Ctrl Pts',(3.25806285817532,-1.30000000000024,10.4292319482507));
#57896=CARTESIAN_POINT('Ctrl Pts',(3.20507339136947,-1.18514270861195,10.3614091950932));
#57897=CARTESIAN_POINT('Ctrl Pts',(3.16003000207498,-1.0684760419452,10.3036861052959));
#57898=CARTESIAN_POINT('Ctrl Pts',(3.07432779056413,-0.794772684000852,
10.1936664631924));
#57899=CARTESIAN_POINT('Ctrl Pts',(3.03856351369519,-0.636309800095197,
10.1527214947036));
#57900=CARTESIAN_POINT('Ctrl Pts',(2.99824596803585,-0.319434907277159,
10.0901842798058));
#57901=CARTESIAN_POINT('Ctrl Pts',(2.99178541067131,-0.158333333333333,
10.0731598884183));
#57902=CARTESIAN_POINT('Ctrl Pts',(3.0061134803473,0.158333333333334,10.0581917222558));
#57903=CARTESIAN_POINT('Ctrl Pts',(3.02637472769607,0.319434907277167,10.0609469829295));
#57904=CARTESIAN_POINT('Ctrl Pts',(3.0969517540897,0.636309800095206,10.0915712362213));
#57905=CARTESIAN_POINT('Ctrl Pts',(3.14699300261571,0.79477268400084,10.1170118814022));
#57906=CARTESIAN_POINT('Ctrl Pts',(3.26484306624898,1.06847604194515,10.1931031343167));
#57907=CARTESIAN_POINT('Ctrl Pts',(3.3251192814113,1.18514270861185,10.2348322744656));
#57908=CARTESIAN_POINT('Ctrl Pts',(3.39465878596432,1.30000000000011,10.2853534708356));
#57909=CARTESIAN_POINT('Ctrl Pts',(3.26356969889503,-1.30000000000025,10.4401936173531));
#57910=CARTESIAN_POINT('Ctrl Pts',(3.21329092939248,-1.18514270861195,10.3734371595662));
#57911=CARTESIAN_POINT('Ctrl Pts',(3.16968495310836,-1.0684760419452,10.3168412032106));
#57912=CARTESIAN_POINT('Ctrl Pts',(3.08436191176865,-0.794772684000854,
10.2095660129541));
#57913=CARTESIAN_POINT('Ctrl Pts',(3.04371183747672,-0.636309800095199,
10.1712622580596));
#57914=CARTESIAN_POINT('Ctrl Pts',(3.00095575774754,-0.31943490727716,10.1102671958419));
#57915=CARTESIAN_POINT('Ctrl Pts',(2.99406129097652,-0.158333333333333,
10.09235461781));
#57916=CARTESIAN_POINT('Ctrl Pts',(3.00853841930703,0.158333333333334,10.0773036860582));
#57917=CARTESIAN_POINT('Ctrl Pts',(3.02932442025788,0.319434907277166,10.0810031003646));
#57918=CARTESIAN_POINT('Ctrl Pts',(3.10276218112927,0.636309800095207,10.1096340251586));
#57919=CARTESIAN_POINT('Ctrl Pts',(3.15833123374125,0.794772684000843,10.13149710373));
#57920=CARTESIAN_POINT('Ctrl Pts',(3.27575915332341,1.06847604194515,10.2048959093763));
#57921=CARTESIAN_POINT('Ctrl Pts',(3.33440348949289,1.18514270861185,10.2457583004224));
#57922=CARTESIAN_POINT('Ctrl Pts',(3.40086196657799,1.30000000000011,10.295711459244));
#57923=CARTESIAN_POINT('Ctrl Pts',(3.27142362945863,-1.30000000000024,10.4564287702393));
#57924=CARTESIAN_POINT('Ctrl Pts',(3.22363852910097,-1.18514270861195,10.3923648793724));
#57925=CARTESIAN_POINT('Ctrl Pts',(3.18171939699315,-1.0684760419452,10.3378877549538));
#57926=CARTESIAN_POINT('Ctrl Pts',(3.09842937607048,-0.794772684000849,
10.2341820477573));
#57927=CARTESIAN_POINT('Ctrl Pts',(3.05634439996193,-0.636309800095195,
10.1964809634167));
#57928=CARTESIAN_POINT('Ctrl Pts',(3.01277478602804,-0.319434907277158,
10.1364512789006));
#57929=CARTESIAN_POINT('Ctrl Pts',(3.00454466836801,-0.158333333333332,
10.1179985536727));
#57930=CARTESIAN_POINT('Ctrl Pts',(3.01907920995353,0.158333333333334,10.1028653588534));
#57931=CARTESIAN_POINT('Ctrl Pts',(3.0409919197028,0.319434907277166,10.1072385910851));
#57932=CARTESIAN_POINT('Ctrl Pts',(3.11590270810618,0.636309800095204,10.1342967326359));
#57933=CARTESIAN_POINT('Ctrl Pts',(3.17432978460092,0.794772684000836,10.1542963989277));
#57934=CARTESIAN_POINT('Ctrl Pts',(3.28991423038207,1.06847604194514,10.2240301459796));
#57935=CARTESIAN_POINT('Ctrl Pts',(3.34665398616072,1.18514270861184,10.2630161354823));
#57936=CARTESIAN_POINT('Ctrl Pts',(3.41010127396518,1.3000000000001,10.310802959279));
#57937=CARTESIAN_POINT('Ctrl Pts',(3.27796208619403,-1.30000000000025,10.4698652030683));
#57938=CARTESIAN_POINT('Ctrl Pts',(3.23176481591554,-1.18514270861195,10.4080730465707));
#57939=CARTESIAN_POINT('Ctrl Pts',(3.19109466270881,-1.0684760419452,10.3551662448441));
#57940=CARTESIAN_POINT('Ctrl Pts',(3.10990721889679,-0.794772684000851,
10.2534678959159));
#57941=CARTESIAN_POINT('Ctrl Pts',(3.06857338381887,-0.636309800095197,
10.2143229029676));
#57942=CARTESIAN_POINT('Ctrl Pts',(3.0247851677372,-0.319434907277159,10.1545065948969));
#57943=CARTESIAN_POINT('Ctrl Pts',(3.01454525909152,-0.158333333333332,
10.1365625803566));
#57944=CARTESIAN_POINT('Ctrl Pts',(3.02864087085784,0.158333333333334,10.121803258227));
#57945=CARTESIAN_POINT('Ctrl Pts',(3.05147554439313,0.319434907277166,10.1266183922667));
#57946=CARTESIAN_POINT('Ctrl Pts',(3.12703262374841,0.636309800095204,10.1530499316631));
#57947=CARTESIAN_POINT('Ctrl Pts',(3.18705715886167,0.794772684000839,10.1723497025203));
#57948=CARTESIAN_POINT('Ctrl Pts',(3.3008563485775,1.06847604194514,10.2398340350002));
#57949=CARTESIAN_POINT('Ctrl Pts',(3.35605604577011,1.18514270861185,10.27754874129));
#57950=CARTESIAN_POINT('Ctrl Pts',(3.4171959876029,1.3000000000001,10.3237666868799));
#57951=CARTESIAN_POINT('Ctrl Pts',(3.28607792754349,-1.30000000000025,10.489640941086));
#57952=CARTESIAN_POINT('Ctrl Pts',(3.24218111798405,-1.18514270861195,10.4313369990907));
#57953=CARTESIAN_POINT('Ctrl Pts',(3.20343144405725,-1.0684760419452,10.3807831278332));
#57954=CARTESIAN_POINT('Ctrl Pts',(3.12580285843302,-0.794772684000849,
10.2818977857617));
#57955=CARTESIAN_POINT('Ctrl Pts',(3.08608263838369,-0.636309800095196,
10.2404042408254));
#57956=CARTESIAN_POINT('Ctrl Pts',(3.04321031720232,-0.319434907277159,
10.1799842860208));
#57957=CARTESIAN_POINT('Ctrl Pts',(3.03091044242816,-0.158333333333332,
10.1620145105244));
#57958=CARTESIAN_POINT('Ctrl Pts',(3.04590331244293,0.158333333333334,10.1463791141261));
#57959=CARTESIAN_POINT('Ctrl Pts',(3.07216452409039,0.319434907277166,10.1498515511517));
#57960=CARTESIAN_POINT('Ctrl Pts',(3.14767740070571,0.636309800095205,10.1761051872238));
#57961=CARTESIAN_POINT('Ctrl Pts',(3.20558241578882,0.794772684000837,10.1983580205055));
#57962=CARTESIAN_POINT('Ctrl Pts',(3.31561037222147,1.06847604194514,10.2633608929864));
#57963=CARTESIAN_POINT('Ctrl Pts',(3.36876295429219,1.18514270861185,10.298899079907));
#57964=CARTESIAN_POINT('Ctrl Pts',(3.42744109303151,1.30000000000011,10.3418381188451));
#57965=CARTESIAN_POINT('Ctrl Pts',(3.29502533151816,-1.30000000000025,10.5123524713943));
#57966=CARTESIAN_POINT('Ctrl Pts',(3.25382565282047,-1.18514270861195,10.4577554197642));
#57967=CARTESIAN_POINT('Ctrl Pts',(3.21726195101644,-1.0684760419452,10.4097280550216));
#57968=CARTESIAN_POINT('Ctrl Pts',(3.143502519354,-0.794772684000853,10.3139525255965));
#57969=CARTESIAN_POINT('Ctrl Pts',(3.10460687574095,-0.636309800095195,
10.2706384477954));
#57970=CARTESIAN_POINT('Ctrl Pts',(3.06356477871524,-0.319434907277157,
10.2087826959084));
#57971=CARTESIAN_POINT('Ctrl Pts',(3.05174093240499,-0.158333333333332,
10.188339847756));
#57972=CARTESIAN_POINT('Ctrl Pts',(3.06722648156504,0.158333333333334,10.1722176724411));
#57973=CARTESIAN_POINT('Ctrl Pts',(3.0936447643894,0.319434907277168,10.1775056433325));
#57974=CARTESIAN_POINT('Ctrl Pts',(3.16804494235512,0.636309800095206,10.2045513684504));
#57975=CARTESIAN_POINT('Ctrl Pts',(3.22532456748403,0.794772684000835,10.2285080909687));
#57976=CARTESIAN_POINT('Ctrl Pts',(3.33162160566429,1.06847604194514,10.2904224485944));
#57977=CARTESIAN_POINT('Ctrl Pts',(3.3825688942346,1.18514270861184,10.3235343192389));
#57978=CARTESIAN_POINT('Ctrl Pts',(3.43845142224042,1.30000000000011,10.3629576292649));
#57979=CARTESIAN_POINT('Ctrl Pts',(3.30450367753543,-1.30000000000025,10.5347011036464));
#57980=CARTESIAN_POINT('Ctrl Pts',(3.2653523505081,-1.18514270861195,10.4844098414235));
#57981=CARTESIAN_POINT('Ctrl Pts',(3.23053973946106,-1.0684760419452,10.4393268926439));
#57982=CARTESIAN_POINT('Ctrl Pts',(3.1601389455751,-0.794772684000851,10.3472085081238));
#57983=CARTESIAN_POINT('Ctrl Pts',(3.12273813965249,-0.636309800095196,
10.3015948945104));
#57984=CARTESIAN_POINT('Ctrl Pts',(3.08323596962934,-0.319434907277158,
10.2386328801667));
#57985=CARTESIAN_POINT('Ctrl Pts',(3.07090138700804,-0.158333333333333,
10.2165712937593));
#57986=CARTESIAN_POINT('Ctrl Pts',(3.08702512194723,0.158333333333334,10.1998384592567));
#57987=CARTESIAN_POINT('Ctrl Pts',(3.11490498355869,0.319434907277169,10.205802664897));
#57988=CARTESIAN_POINT('Ctrl Pts',(3.18842831382349,0.636309800095208,10.233386726658));
#57989=CARTESIAN_POINT('Ctrl Pts',(3.24412642596474,0.794772684000837,10.2598651214132));
#57990=CARTESIAN_POINT('Ctrl Pts',(3.34662974959848,1.06847604194514,10.3185985123408));
#57991=CARTESIAN_POINT('Ctrl Pts',(3.39549307711668,1.18514270861185,10.3490899716152));
#57992=CARTESIAN_POINT('Ctrl Pts',(3.44884984147448,1.30000000000011,10.384649381518));
#57993=CARTESIAN_POINT('Ctrl Pts',(3.31134556628304,-1.30000000000025,10.555306793775));
#57994=CARTESIAN_POINT('Ctrl Pts',(3.27421412686849,-1.18514270861196,10.5085498757349));
#57995=CARTESIAN_POINT('Ctrl Pts',(3.241079812679,-1.06847604194521,10.4658911880933));
#57996=CARTESIAN_POINT('Ctrl Pts',(3.17376707729655,-0.794772684000857,
10.3768088178691));
#57997=CARTESIAN_POINT('Ctrl Pts',(3.1373310728862,-0.6363098000952,10.329485060397));
#57998=CARTESIAN_POINT('Ctrl Pts',(3.09935867807212,-0.319434907277159,
10.2654171552566));
#57999=CARTESIAN_POINT('Ctrl Pts',(3.0872424959219,-0.158333333333333,10.2413968868924));
#58000=CARTESIAN_POINT('Ctrl Pts',(3.10377833472793,0.158333333333334,10.2242936402102));
#58001=CARTESIAN_POINT('Ctrl Pts',(3.13175556627714,0.319434907277168,10.2318950276049));
#58002=CARTESIAN_POINT('Ctrl Pts',(3.20478477155487,0.636309800095208,10.2597308470479));
#58003=CARTESIAN_POINT('Ctrl Pts',(3.2606917912936,0.794772684000841,10.286994013888));
#58004=CARTESIAN_POINT('Ctrl Pts',(3.3604446389725,1.06847604194515,10.3425115054252));
#58005=CARTESIAN_POINT('Ctrl Pts',(3.40751986583463,1.18514270861185,10.3707253370665));
#58006=CARTESIAN_POINT('Ctrl Pts',(3.458491008006,1.30000000000011,10.4031215353883));
#58007=CARTESIAN_POINT('Ctrl Pts',(3.31769888764463,-1.30000000000025,10.5725971040921));
#58008=CARTESIAN_POINT('Ctrl Pts',(3.28202446624183,-1.18514270861195,10.5290890206369));
#58009=CARTESIAN_POINT('Ctrl Pts',(3.25011584783553,-1.06847604194521,10.4886833545695));
#58010=CARTESIAN_POINT('Ctrl Pts',(3.18510031428796,-0.794772684000854,
10.4025053876304));
#58011=CARTESIAN_POINT('Ctrl Pts',(3.14935000680282,-0.636309800095199,
10.3538691897764));
#58012=CARTESIAN_POINT('Ctrl Pts',(3.11280902090405,-0.31943490727716,10.288776895608));
#58013=CARTESIAN_POINT('Ctrl Pts',(3.10139537328697,-0.158333333333333,
10.2626576970449));
#58014=CARTESIAN_POINT('Ctrl Pts',(3.11834904634676,0.158333333333334,10.245178008912));
#58015=CARTESIAN_POINT('Ctrl Pts',(3.14625294407796,0.319434907277168,10.2542881797259));
#58016=CARTESIAN_POINT('Ctrl Pts',(3.21827130046734,0.636309800095208,10.2828169064337));
#58017=CARTESIAN_POINT('Ctrl Pts',(3.27332792887522,0.79477268400084,10.3116295963842));
#58018=CARTESIAN_POINT('Ctrl Pts',(3.37062679205695,1.06847604194515,10.3644450457924));
#58019=CARTESIAN_POINT('Ctrl Pts',(3.41636433385336,1.18514270861185,10.3905247514617));
#58020=CARTESIAN_POINT('Ctrl Pts',(3.46572234485302,1.30000000000012,10.4198223117566));
#58021=CARTESIAN_POINT('Ctrl Pts',(3.32402656077166,-1.30000000000025,10.5898959986511));
#58022=CARTESIAN_POINT('Ctrl Pts',(3.29037048057002,-1.18514270861195,10.5492220550332));
#58023=CARTESIAN_POINT('Ctrl Pts',(3.25998575361421,-1.06847604194521,10.5108491154506));
#58024=CARTESIAN_POINT('Ctrl Pts',(3.19734843633234,-0.794772684000856,
10.4275157281707));
#58025=CARTESIAN_POINT('Ctrl Pts',(3.16145626521804,-0.636309800095199,
10.3781493048116));
#58026=CARTESIAN_POINT('Ctrl Pts',(3.12549096178903,-0.31943490727716,10.3127222436558));
#58027=CARTESIAN_POINT('Ctrl Pts',(3.11386317686832,-0.158333333333333,
10.2853097158677));
#58028=CARTESIAN_POINT('Ctrl Pts',(3.13122089061224,0.158333333333334,10.267482774936));
#58029=CARTESIAN_POINT('Ctrl Pts',(3.15986025444291,0.319434907277167,10.2774327625591));
#58030=CARTESIAN_POINT('Ctrl Pts',(3.23188702270569,0.636309800095208,10.3058053704956));
#58031=CARTESIAN_POINT('Ctrl Pts',(3.28715017080431,0.794772684000841,10.3352736952322));
#58032=CARTESIAN_POINT('Ctrl Pts',(3.38233829455662,1.06847604194515,10.385099208329));
#58033=CARTESIAN_POINT('Ctrl Pts',(3.42665634566863,1.18514270861185,10.4091142608124));
#58034=CARTESIAN_POINT('Ctrl Pts',(3.47408903618788,1.30000000000011,10.4355767473769));
#58035=CARTESIAN_POINT('Ctrl Pts',(3.32983519550131,-1.30000000000025,10.6075611244657));
#58036=CARTESIAN_POINT('Ctrl Pts',(3.29686746725483,-1.18514270861196,10.5706822971744));
#58037=CARTESIAN_POINT('Ctrl Pts',(3.26722319807112,-1.06847604194521,10.5349111259825));
#58038=CARTESIAN_POINT('Ctrl Pts',(3.2064168612317,-0.794772684000859,10.4548314717062));
#58039=CARTESIAN_POINT('Ctrl Pts',(3.1720371497533,-0.6363098000952,10.4035791334109));
#58040=CARTESIAN_POINT('Ctrl Pts',(3.13770761580401,-0.31943490727716,10.3370342383692));
#58041=CARTESIAN_POINT('Ctrl Pts',(3.12659304393993,-0.158333333333333,
10.3077270416474));
#58042=CARTESIAN_POINT('Ctrl Pts',(3.14448954447489,0.158333333333335,10.2894528640902));
#58043=CARTESIAN_POINT('Ctrl Pts',(3.17330341630422,0.319434907277168,10.3006888317874));
#58044=CARTESIAN_POINT('Ctrl Pts',(3.24448851661404,0.636309800095208,10.3295971513818));
#58045=CARTESIAN_POINT('Ctrl Pts',(3.2988649868747,0.794772684000842,10.3606116427013));
#58046=CARTESIAN_POINT('Ctrl Pts',(3.39169722187798,1.06847604194515,10.4076557293263));
#58047=CARTESIAN_POINT('Ctrl Pts',(3.43473197837859,1.18514270861185,10.429500999216));
#58048=CARTESIAN_POINT('Ctrl Pts',(3.4806178566202,1.30000000000011,10.4528278970506));
#58049=CARTESIAN_POINT('Ctrl Pts',(3.33543431689412,-1.30000000000026,10.6253660208351));
#58050=CARTESIAN_POINT('Ctrl Pts',(3.30447387826058,-1.18514270861196,10.5913293433328));
#58051=CARTESIAN_POINT('Ctrl Pts',(3.27638596789649,-1.06847604194521,10.557568389007));
#58052=CARTESIAN_POINT('Ctrl Pts',(3.21813339093802,-0.794772684000854,
10.4802108063544));
#58053=CARTESIAN_POINT('Ctrl Pts',(3.18404962061072,-0.6363098000952,10.4279113109503));
#58054=CARTESIAN_POINT('Ctrl Pts',(3.15026714188066,-0.319434907277161,
10.361072512131));
#58055=CARTESIAN_POINT('Ctrl Pts',(3.13850778186067,-0.158333333333333,
10.3308077811648));
#58056=CARTESIAN_POINT('Ctrl Pts',(3.15655965464604,0.158333333333334,10.3123911489482));
#58057=CARTESIAN_POINT('Ctrl Pts',(3.18598322614092,0.319434907277166,10.3245779265405));
#58058=CARTESIAN_POINT('Ctrl Pts',(3.25732570813374,0.636309800095207,10.353213507159));
#58059=CARTESIAN_POINT('Ctrl Pts',(3.31244332438267,0.794772684000842,10.3844471357686));
#58060=CARTESIAN_POINT('Ctrl Pts',(3.40324104275787,1.06847604194515,10.4284399262086));
#58061=CARTESIAN_POINT('Ctrl Pts',(3.44478755173034,1.18514270861186,10.4482767546045));
#58062=CARTESIAN_POINT('Ctrl Pts',(3.48857760177768,1.30000000000012,10.4689075625085));
#58063=CARTESIAN_POINT('Ctrl Pts',(3.34094149524622,-1.30000000000025,10.6432126996063));
#58064=CARTESIAN_POINT('Ctrl Pts',(3.31096178439977,-1.18514270861195,10.6127392800863));
#58065=CARTESIAN_POINT('Ctrl Pts',(3.28373855848769,-1.0684760419452,10.5814796933298));
#58066=CARTESIAN_POINT('Ctrl Pts',(3.22721549227442,-0.794772684000855,
10.5074475908752));
#58067=CARTESIAN_POINT('Ctrl Pts',(3.19385314783236,-0.6363098000952,10.4538609714195));
#58068=CARTESIAN_POINT('Ctrl Pts',(3.16133319050392,-0.319434907277161,
10.3862178147945));
#58069=CARTESIAN_POINT('Ctrl Pts',(3.15012119231218,-0.158333333333333,
10.3540840714003));
#58070=CARTESIAN_POINT('Ctrl Pts',(3.16878216455365,0.158333333333334,10.3351886489903));
#58071=CARTESIAN_POINT('Ctrl Pts',(3.19860862575582,0.319434907277166,10.3484737780535));
#58072=CARTESIAN_POINT('Ctrl Pts',(3.26923437586041,0.636309800095207,10.3775329750586));
#58073=CARTESIAN_POINT('Ctrl Pts',(3.32327179259272,0.794772684000843,10.4104342210879));
#58074=CARTESIAN_POINT('Ctrl Pts',(3.4120120682439,1.06847604194515,10.4514071685875));
#58075=CARTESIAN_POINT('Ctrl Pts',(3.45249543045058,1.18514270861185,10.4689059981687));
#58076=CARTESIAN_POINT('Ctrl Pts',(3.49504977768584,1.30000000000011,10.4861679865556));
#58077=CARTESIAN_POINT('Ctrl Pts',(3.34862517899029,-1.30000000000025,10.666765726311));
#58078=CARTESIAN_POINT('Ctrl Pts',(3.32059598526539,-1.18514270861196,10.6405999286535));
#58079=CARTESIAN_POINT('Ctrl Pts',(3.29494534462785,-1.06847604194521,10.6123835725847));
#58080=CARTESIAN_POINT('Ctrl Pts',(3.24118216682178,-0.794772684000855,
10.5424609452606));
#58081=CARTESIAN_POINT('Ctrl Pts',(3.20848037172561,-0.6363098000952,10.4873290346525));
#58082=CARTESIAN_POINT('Ctrl Pts',(3.17698900635549,-0.31943490727716,10.4190869541489));
#58083=CARTESIAN_POINT('Ctrl Pts',(3.16568642237986,-0.158333333333333,
10.3850813153639));
#58084=CARTESIAN_POINT('Ctrl Pts',(3.18435626144325,0.158333333333334,10.3661584983787));
#58085=CARTESIAN_POINT('Ctrl Pts',(3.21391244753801,0.319434907277167,10.3815490559967));
#58086=CARTESIAN_POINT('Ctrl Pts',(3.28428077549263,0.636309800095208,10.410619885086));
#58087=CARTESIAN_POINT('Ctrl Pts',(3.33933815331492,0.794772684000841,10.4438131317773));
#58088=CARTESIAN_POINT('Ctrl Pts',(3.42584267425899,1.06847604194515,10.4803480902833));
#58089=CARTESIAN_POINT('Ctrl Pts',(3.46469322031126,1.18514270861186,10.4948905487474));
#58090=CARTESIAN_POINT('Ctrl Pts',(3.50494971060752,1.30000000000012,10.5081608358921));
#58091=CARTESIAN_POINT('Ctrl Pts',(3.35477242854431,-1.30000000000025,10.6913545086937));
#58092=CARTESIAN_POINT('Ctrl Pts',(3.32803258482394,-1.18514270861196,10.6699233907188));
#58093=CARTESIAN_POINT('Ctrl Pts',(3.30354326255944,-1.06847604194521,10.6450206000984));
#58094=CARTESIAN_POINT('Ctrl Pts',(3.2521671838347,-0.794772684000857,10.579469913662));
#58095=CARTESIAN_POINT('Ctrl Pts',(3.22070121255191,-0.6363098000952,10.5224626389412));
#58096=CARTESIAN_POINT('Ctrl Pts',(3.19080582191474,-0.31943490727716,10.4532693753533));
#58097=CARTESIAN_POINT('Ctrl Pts',(3.17971659705789,-0.158333333333333,
10.417212370891));
#58098=CARTESIAN_POINT('Ctrl Pts',(3.19929932435408,0.158333333333335,10.3975993255158));
#58099=CARTESIAN_POINT('Ctrl Pts',(3.22998407396361,0.319434907277168,10.4139884899421));
#58100=CARTESIAN_POINT('Ctrl Pts',(3.29974200260255,0.636309800095208,10.4433430050657));
#58101=CARTESIAN_POINT('Ctrl Pts',(3.3532409800158,0.794772684000841,10.4788196557371));
#58102=CARTESIAN_POINT('Ctrl Pts',(3.43725631206308,1.06847604194515,10.5111268387956));
#58103=CARTESIAN_POINT('Ctrl Pts',(3.47484407697495,1.18514270861185,10.5224366375833));
#58104=CARTESIAN_POINT('Ctrl Pts',(3.51365248263028,1.30000000000012,10.5310716527117));
#58105=CARTESIAN_POINT('Ctrl Pts',(3.36577222422768,-1.30000000000026,10.7269652643744));
#58106=CARTESIAN_POINT('Ctrl Pts',(3.34162487994577,-1.18514270861196,10.7121939560135));
#58107=CARTESIAN_POINT('Ctrl Pts',(3.31912207672054,-1.06847604194521,10.6921008331891));
#58108=CARTESIAN_POINT('Ctrl Pts',(3.27093531843018,-0.794772684000855,
10.6333872438135));
#58109=CARTESIAN_POINT('Ctrl Pts',(3.23925223091895,-0.636309800095199,
10.5749795322508));
#58110=CARTESIAN_POINT('Ctrl Pts',(3.21075933021502,-0.319434907277159,
10.5050547005001));
#58111=CARTESIAN_POINT('Ctrl Pts',(3.20062822260473,-0.158333333333333,
10.4654774372491));
#58112=CARTESIAN_POINT('Ctrl Pts',(3.22074425502184,0.158333333333334,10.4454751695304));
#58113=CARTESIAN_POINT('Ctrl Pts',(3.25098152631975,0.319434907277168,10.4650006098656));
#58114=CARTESIAN_POINT('Ctrl Pts',(3.32046943854635,0.636309800095208,10.4942832028526));
#58115=CARTESIAN_POINT('Ctrl Pts',(3.37540064930299,0.794772684000839,10.5302830665368));
#58116=CARTESIAN_POINT('Ctrl Pts',(3.45624605781512,1.06847604194515,10.5558276779446));
#58117=CARTESIAN_POINT('Ctrl Pts',(3.49151207624827,1.18514270861185,10.5626262465742));
#58118=CARTESIAN_POINT('Ctrl Pts',(3.52704913138729,1.30000000000012,10.5651660680762));
#58119=CARTESIAN_POINT('Ctrl Pts',(3.37465670933942,-1.30000000000025,10.7639426884239));
#58120=CARTESIAN_POINT('Ctrl Pts',(3.35156199955871,-1.18514270861196,10.7568205400723));
#58121=CARTESIAN_POINT('Ctrl Pts',(3.33024799136158,-1.06847604194521,10.7420448903889));
#58122=CARTESIAN_POINT('Ctrl Pts',(3.28512214545966,-0.794772684000864,
10.6902290646073));
#58123=CARTESIAN_POINT('Ctrl Pts',(3.25658204085502,-0.636309800095202,
10.6281861136521));
#58124=CARTESIAN_POINT('Ctrl Pts',(3.23011273411839,-0.31943490727716,10.5571834304215));
#58125=CARTESIAN_POINT('Ctrl Pts',(3.21894204378883,-0.158333333333334,
10.5155650325798));
#58126=CARTESIAN_POINT('Ctrl Pts',(3.23986811073716,0.158333333333336,10.494972413652));
#58127=CARTESIAN_POINT('Ctrl Pts',(3.27199560830785,0.319434907277173,10.5158512738659));
#58128=CARTESIAN_POINT('Ctrl Pts',(3.34102719092835,0.636309800095214,10.5452075378715));
#58129=CARTESIAN_POINT('Ctrl Pts',(3.39431511704226,0.794772684000845,10.5840586607155));
#58130=CARTESIAN_POINT('Ctrl Pts',(3.472037879555,1.06847604194515,10.6028389087067));
#58131=CARTESIAN_POINT('Ctrl Pts',(3.50562864900718,1.18514270861185,10.6046586260853));
#58132=CARTESIAN_POINT('Ctrl Pts',(3.53916688393195,1.30000000000011,10.6001687873637));
#58133=CARTESIAN_POINT('Ctrl Pts',(3.38277473801816,-1.30000000000025,10.7960140500224));
#58134=CARTESIAN_POINT('Ctrl Pts',(3.36171527708658,-1.18514270861195,10.7948103933562));
#58135=CARTESIAN_POINT('Ctrl Pts',(3.34188342069616,-1.06847604194521,10.7843745616666));
#58136=CARTESIAN_POINT('Ctrl Pts',(3.29890387715655,-0.794772684000861,
10.7389375315884));
#58137=CARTESIAN_POINT('Ctrl Pts',(3.26941563404066,-0.636309800095202,
10.6762284222361));
#58138=CARTESIAN_POINT('Ctrl Pts',(3.24399580987047,-0.319434907277161,
10.6047768627138));
#58139=CARTESIAN_POINT('Ctrl Pts',(3.23409109017862,-0.158333333333334,
10.559888104658));
#58140=CARTESIAN_POINT('Ctrl Pts',(3.2560330799295,0.158333333333335,10.5386146162028));
#58141=CARTESIAN_POINT('Ctrl Pts',(3.28844573931014,0.31943490727717,10.5617080178589));
#58142=CARTESIAN_POINT('Ctrl Pts',(3.3574070174534,0.636309800095212,10.5908900205671));
#58143=CARTESIAN_POINT('Ctrl Pts',(3.41100341783752,0.794772684000845,10.6308930828505));
#58144=CARTESIAN_POINT('Ctrl Pts',(3.48642152170975,1.06847604194515,10.6434518917354));
#58145=CARTESIAN_POINT('Ctrl Pts',(3.5184541323885,1.18514270861186,10.6410018315667));
#58146=CARTESIAN_POINT('Ctrl Pts',(3.54987365109589,1.30000000000012,10.6306654682128));
#58147=CARTESIAN_POINT('Ctrl Pts',(3.38626628437866,-1.30000000000025,10.8115186948131));
#58148=CARTESIAN_POINT('Ctrl Pts',(3.36582717777872,-1.18514270861195,10.8133605040441));
#58149=CARTESIAN_POINT('Ctrl Pts',(3.3465333662151,-1.06847604194521,10.8050994622387));
#58150=CARTESIAN_POINT('Ctrl Pts',(3.30460666243877,-0.79477268400086,10.7626751960902));
#58151=CARTESIAN_POINT('Ctrl Pts',(3.2754688410601,-0.636309800095203,10.699115115923));
#58152=CARTESIAN_POINT('Ctrl Pts',(3.25087387028672,-0.319434907277163,
10.6272400354614));
#58153=CARTESIAN_POINT('Ctrl Pts',(3.24153842421982,-0.158333333333334,
10.5808270561062));
#58154=CARTESIAN_POINT('Ctrl Pts',(3.26376129942525,0.158333333333336,10.5593729013938));
#58155=CARTESIAN_POINT('Ctrl Pts',(3.29598529121409,0.31943490727717,10.583731898213));
#58156=CARTESIAN_POINT('Ctrl Pts',(3.36449073576851,0.636309800095213,10.6131282163632));
#58157=CARTESIAN_POINT('Ctrl Pts',(3.417724398162,0.794772684000848,10.6540551173811));
#58158=CARTESIAN_POINT('Ctrl Pts',(3.49220667372963,1.06847604194516,10.6635405170809));
#58159=CARTESIAN_POINT('Ctrl Pts',(3.5237435755897,1.18514270861186,10.6588825891453));
#58160=CARTESIAN_POINT('Ctrl Pts',(3.55457676205692,1.30000000000012,10.6454608552128));
#58161=CARTESIAN_POINT('Ctrl Pts',(3.38769780288249,-1.30000000000025,10.8176960564688));
#58162=CARTESIAN_POINT('Ctrl Pts',(3.36755620151121,-1.18514270861195,10.8207223471244));
#58163=CARTESIAN_POINT('Ctrl Pts',(3.34850087888628,-1.06847604194521,10.813315256739));
#58164=CARTESIAN_POINT('Ctrl Pts',(3.30698879283185,-0.79477268400086,10.7721001987698));
#58165=CARTESIAN_POINT('Ctrl Pts',(3.27788009191905,-0.636309800095203,
10.7082749221034));
#58166=CARTESIAN_POINT('Ctrl Pts',(3.25355472013789,-0.319434907277162,
10.6362713366291));
#58167=CARTESIAN_POINT('Ctrl Pts',(3.24441619455047,-0.158333333333334,
10.5892701532528));
#58168=CARTESIAN_POINT('Ctrl Pts',(3.266793663605,0.158333333333335,10.5677143586198));
#58169=CARTESIAN_POINT('Ctrl Pts',(3.29904752840448,0.31943490727717,10.5925071897121));
#58170=CARTESIAN_POINT('Ctrl Pts',(3.36745120503604,0.636309800095212,10.6219323865371));
#58171=CARTESIAN_POINT('Ctrl Pts',(3.42058911211841,0.794772684000847,10.6631913608502));
#58172=CARTESIAN_POINT('Ctrl Pts',(3.49466491110876,1.06847604194515,10.6714706894569));
#58173=CARTESIAN_POINT('Ctrl Pts',(3.52596499017303,1.18514270861186,10.6659577209332));
#58174=CARTESIAN_POINT('Ctrl Pts',(3.55650047969752,1.30000000000012,10.6513479693114));
#58175=CARTESIAN_POINT('Ctrl Pts',(3.39109987683895,-1.30000000000025,10.8350139320941));
#58176=CARTESIAN_POINT('Ctrl Pts',(3.37125853817352,-1.18514270861195,10.8416206060688));
#58177=CARTESIAN_POINT('Ctrl Pts',(3.35262039187588,-1.06847604194521,10.8367100040207));
#58178=CARTESIAN_POINT('Ctrl Pts',(3.31234216044733,-0.794772684000859,
10.798758319291));
#58179=CARTESIAN_POINT('Ctrl Pts',(3.28474943875151,-0.636309800095202,
10.7332931428369));
#58180=CARTESIAN_POINT('Ctrl Pts',(3.26137805267955,-0.319434907277162,
10.6608171980619));
#58181=CARTESIAN_POINT('Ctrl Pts',(3.25183148610066,-0.158333333333334,
10.6128327837711));
#58182=CARTESIAN_POINT('Ctrl Pts',(3.27458361122692,0.158333333333335,10.5910290471671));
#58183=CARTESIAN_POINT('Ctrl Pts',(3.307374631408,0.319434907277171,10.6167036041784));
#58184=CARTESIAN_POINT('Ctrl Pts',(3.37608762049819,0.636309800095212,10.6457978387865));
#58185=CARTESIAN_POINT('Ctrl Pts',(3.42976486332244,0.794772684000846,10.6874068292731));
#58186=CARTESIAN_POINT('Ctrl Pts',(3.5026472205099,1.06847604194515,10.692422154672));
#58187=CARTESIAN_POINT('Ctrl Pts',(3.5330325403784,1.18514270861186,10.6847421636972));
#58188=CARTESIAN_POINT('Ctrl Pts',(3.56225510824644,1.30000000000012,10.6672112332187));
#58189=CARTESIAN_POINT('Ctrl Pts',(3.3961039320677,-1.30000000000025,10.8566094221741));
#58190=CARTESIAN_POINT('Ctrl Pts',(3.37730930726364,-1.18514270861196,10.8673460146537));
#58191=CARTESIAN_POINT('Ctrl Pts',(3.35942825207076,-1.06847604194521,10.8654649821272));
#58192=CARTESIAN_POINT('Ctrl Pts',(3.32022996604323,-0.794772684000863,
10.8319701827806));
#58193=CARTESIAN_POINT('Ctrl Pts',(3.29209724359651,-0.636309800095203,
10.7659785582791));
#58194=CARTESIAN_POINT('Ctrl Pts',(3.26926298889969,-0.319434907277162,
10.6933358778177));
#58195=CARTESIAN_POINT('Ctrl Pts',(3.26044497555805,-0.158333333333334,
10.6433146168721));
#58196=CARTESIAN_POINT('Ctrl Pts',(3.28367719243551,0.158333333333335,10.6212189492113));
#58197=CARTESIAN_POINT('Ctrl Pts',(3.31668048625251,0.319434907277168,10.6483297640823));
#58198=CARTESIAN_POINT('Ctrl Pts',(3.38489577202755,0.636309800095211,10.6776248054219));
#58199=CARTESIAN_POINT('Ctrl Pts',(3.43761984386032,0.794772684000848,10.7208148378221));
#58200=CARTESIAN_POINT('Ctrl Pts',(3.50950537524388,1.06847604194515,10.7213304653958));
#58201=CARTESIAN_POINT('Ctrl Pts',(3.53947393670639,1.18514270861186,10.7103847949187));
#58202=CARTESIAN_POINT('Ctrl Pts',(3.56829447671692,1.30000000000011,10.6882702578935));
#58203=CARTESIAN_POINT('Ctrl Pts',(3.40212020418971,-1.30000000000024,10.8881223521638));
#58204=CARTESIAN_POINT('Ctrl Pts',(3.38389046357394,-1.18514270861195,10.9053147692767));
#58205=CARTESIAN_POINT('Ctrl Pts',(3.36664207879231,-1.0684760419452,10.9080258719001));
#58206=CARTESIAN_POINT('Ctrl Pts',(3.32906198771562,-0.794772684000856,
10.8808343278664));
#58207=CARTESIAN_POINT('Ctrl Pts',(3.30230971800406,-0.6363098000952,10.8127663703491));
#58208=CARTESIAN_POINT('Ctrl Pts',(3.28105505508516,-0.319434907277161,
10.7393933092971));
#58209=CARTESIAN_POINT('Ctrl Pts',(3.27279618739657,-0.158333333333333,
10.686782398982));
#58210=CARTESIAN_POINT('Ctrl Pts',(3.29672863406106,0.158333333333335,10.6642612576124));
#58211=CARTESIAN_POINT('Ctrl Pts',(3.32964993153132,0.319434907277167,10.6936694033216));
#58212=CARTESIAN_POINT('Ctrl Pts',(3.39816634206327,0.636309800095208,10.7225569384338));
#58213=CARTESIAN_POINT('Ctrl Pts',(3.45226798793885,0.794772684000844,10.7661248346689));
#58214=CARTESIAN_POINT('Ctrl Pts',(3.52231733001041,1.06847604194515,10.7605319396099));
#58215=CARTESIAN_POINT('Ctrl Pts',(3.5507893843304,1.18514270861185,10.7455636050312));
#58216=CARTESIAN_POINT('Ctrl Pts',(3.57741172837152,1.30000000000011,10.7180478929078));
#58217=CARTESIAN_POINT('Ctrl Pts',(3.4058272992921,-1.30000000000024,10.9069423026201));
#58218=CARTESIAN_POINT('Ctrl Pts',(3.38807550315061,-1.18514270861195,10.9279007195059));
#58219=CARTESIAN_POINT('Ctrl Pts',(3.37125653663408,-1.0684760419452,10.9333212751712));
#58220=CARTESIAN_POINT('Ctrl Pts',(3.33455638240376,-0.794772684000852,
10.9099482753785));
#58221=CARTESIAN_POINT('Ctrl Pts',(3.30823759879944,-0.636309800095197,
10.8408849121294));
#58222=CARTESIAN_POINT('Ctrl Pts',(3.28760112788311,-0.319434907277159,
10.7672871264273));
#58223=CARTESIAN_POINT('Ctrl Pts',(3.2794226920031,-0.158333333333333,10.7133022638828));
#58224=CARTESIAN_POINT('Ctrl Pts',(3.30384439390905,0.158333333333334,10.6904854093681));
#58225=CARTESIAN_POINT('Ctrl Pts',(3.3375004211861,0.319434907277167,10.7207477256399));
#58226=CARTESIAN_POINT('Ctrl Pts',(3.40573136959717,0.636309800095206,10.7497140504626));
#58227=CARTESIAN_POINT('Ctrl Pts',(3.45859257120118,0.79477268400084,10.7949182498349));
#58228=CARTESIAN_POINT('Ctrl Pts',(3.52792852763022,1.06847604194515,10.785389185721));
#58229=CARTESIAN_POINT('Ctrl Pts',(3.55620374536084,1.18514270861185,10.7675245519584));
#58230=CARTESIAN_POINT('Ctrl Pts',(3.58274121443434,1.30000000000011,10.7359200632015));
#58231=CARTESIAN_POINT('Ctrl Pts',(3.40792382026114,-1.30000000000024,10.9197225044722));
#58232=CARTESIAN_POINT('Ctrl Pts',(3.3906322726577,-1.18514270861195,10.9430989210123));
#58233=CARTESIAN_POINT('Ctrl Pts',(3.37417219529069,-1.0684760419452,10.9502776169302));
#58234=CARTESIAN_POINT('Ctrl Pts',(3.33806698632697,-0.794772684000852,
10.9294418656142));
#58235=CARTESIAN_POINT('Ctrl Pts',(3.31165271079239,-0.636309800095197,
10.859956075597));
#58236=CARTESIAN_POINT('Ctrl Pts',(3.29150406597601,-0.319434907277159,
10.7861661143519));
#58237=CARTESIAN_POINT('Ctrl Pts',(3.28383918476484,-0.158333333333333,
10.7309845243911));
#58238=CARTESIAN_POINT('Ctrl Pts',(3.30866559173632,0.158333333333334,10.7079289458231));
#58239=CARTESIAN_POINT('Ctrl Pts',(3.34233892867207,0.319434907277167,10.7390693321137));
#58240=CARTESIAN_POINT('Ctrl Pts',(3.410649428729,0.636309800095206,10.7679043872382));
#58241=CARTESIAN_POINT('Ctrl Pts',(3.46380979023611,0.79477268400084,10.8134309006136));
#58242=CARTESIAN_POINT('Ctrl Pts',(3.53249270106959,1.06847604194515,10.8014150897722));
#58243=CARTESIAN_POINT('Ctrl Pts',(3.56027544998898,1.18514270861185,10.7818767116455));
#58244=CARTESIAN_POINT('Ctrl Pts',(3.58611066068062,1.30000000000011,10.7480011546757));
#58245=CARTESIAN_POINT('',(3.53212178875801,1.2,10.6679411283038));
#58246=CARTESIAN_POINT('Ctrl Pts',(3.53212178875801,1.2,10.6679411283038));
#58247=CARTESIAN_POINT('Ctrl Pts',(3.53076600547773,1.20867356067025,10.656941710424));
#58248=CARTESIAN_POINT('Ctrl Pts',(3.52995217304133,1.21711400407322,10.6457006410991));
#58249=CARTESIAN_POINT('Ctrl Pts',(3.52771878247509,1.23357261918912,10.6243979759498));
#58250=CARTESIAN_POINT('Ctrl Pts',(3.5273107258133,1.23602988985319,10.6213028016734));
#58251=CARTESIAN_POINT('Ctrl Pts',(3.52277567166249,1.26657829400011,10.5820179245844));
#58252=CARTESIAN_POINT('Ctrl Pts',(3.5201115627438,1.28322142352916,10.5607323865177));
#58253=CARTESIAN_POINT('Ctrl Pts',(3.51702417250711,1.30000000000012,10.5396168897045));
#58254=CARTESIAN_POINT('',(3.42060206384614,0.653834841420791,10.7779856792003));
#58255=CARTESIAN_POINT('Ctrl Pts',(3.42060206386547,0.653834841420113,10.7779856792166));
#58256=CARTESIAN_POINT('Ctrl Pts',(3.43245989940398,0.718489900125914,10.7666494301781));
#58257=CARTESIAN_POINT('Ctrl Pts',(3.44115395086233,0.760264441102575,10.7582679025733));
#58258=CARTESIAN_POINT('Ctrl Pts',(3.47874216109659,0.949909181003267,10.7216567942924));
#58259=CARTESIAN_POINT('Ctrl Pts',(3.50505627305355,1.07520346740433,10.6955075414022));
#58260=CARTESIAN_POINT('Ctrl Pts',(3.53212178875801,1.2,10.6679411283038));
#58261=CARTESIAN_POINT('',(3.3184146483206,-0.653834841531101,10.8729585107664));
#58262=CARTESIAN_POINT('Ctrl Pts',(3.3184146483206,-0.653834841531098,10.8729585107664));
#58263=CARTESIAN_POINT('Ctrl Pts',(3.30612340454657,-0.575948840682229,
10.8332259573124));
#58264=CARTESIAN_POINT('Ctrl Pts',(3.29646275965704,-0.493565906078733,
10.7994009548295));
#58265=CARTESIAN_POINT('Ctrl Pts',(3.28493831203399,-0.33802586804748,10.7501065984067));
#58266=CARTESIAN_POINT('Ctrl Pts',(3.28207503415345,-0.265543988072748,
10.7324464737946));
#58267=CARTESIAN_POINT('Ctrl Pts',(3.28246020273128,-0.129635186233274,
10.7080854451719));
#58268=CARTESIAN_POINT('Ctrl Pts',(3.28485202508577,-0.066588188713728,
10.700174008646));
#58269=CARTESIAN_POINT('Ctrl Pts',(3.29435165456499,0.0594976330476124,
10.6908373400304));
#58270=CARTESIAN_POINT('Ctrl Pts',(3.30151562510345,0.122685832955994,10.6893328369104));
#58271=CARTESIAN_POINT('Ctrl Pts',(3.32176598313159,0.260008478785349,10.6937083254578));
#58272=CARTESIAN_POINT('Ctrl Pts',(3.33570383496495,0.333833694405106,10.7009899323094));
#58273=CARTESIAN_POINT('Ctrl Pts',(3.37146808014451,0.491082797991572,10.7280228209757));
#58274=CARTESIAN_POINT('Ctrl Pts',(3.39445295550189,0.574241316481935,10.749653710407));
#58275=CARTESIAN_POINT('Ctrl Pts',(3.42060206385329,0.653834841432093,10.7779856791619));
#58276=CARTESIAN_POINT('',(3.37169896859721,-1.2,10.8241062436359));
#58277=CARTESIAN_POINT('Ctrl Pts',(3.3716989685972,-1.2,10.8241062436359));
#58278=CARTESIAN_POINT('Ctrl Pts',(3.35768718230927,-1.09933264222173,10.8371421543403));
#58279=CARTESIAN_POINT('Ctrl Pts',(3.34788171370128,-1.01093493025459,10.8461501750024));
#58280=CARTESIAN_POINT('Ctrl Pts',(3.32759670212101,-0.799392291359797,
10.8646633041815));
#58281=CARTESIAN_POINT('Ctrl Pts',(3.32365825158216,-0.748331475394995,
10.8682210627876));
#58282=CARTESIAN_POINT('Ctrl Pts',(3.3184146483206,-0.653834841531101,10.8729585107664));
#58283=CARTESIAN_POINT('Ctrl Pts',(3.35750201349686,-1.3,10.6999543181825));
#58284=CARTESIAN_POINT('Ctrl Pts',(3.36058314309854,-1.28290082666877,10.7206934722446));
#58285=CARTESIAN_POINT('Ctrl Pts',(3.36310814969023,-1.26597626730214,10.7416599332655));
#58286=CARTESIAN_POINT('Ctrl Pts',(3.36677349478208,-1.23881242621742,10.7755644053774));
#58287=CARTESIAN_POINT('Ctrl Pts',(3.36768665493843,-1.23284191421401,10.7828987153576));
#58288=CARTESIAN_POINT('Ctrl Pts',(3.37058282004082,-1.21177341596379,10.8090655493132));
#58289=CARTESIAN_POINT('Ctrl Pts',(3.3708960298996,-1.20975903898414,10.8115238378433));
#58290=CARTESIAN_POINT('Ctrl Pts',(3.3716989685972,-1.2,10.8241062436359));
#58291=CARTESIAN_POINT('Origin',(0.,1.25,7.2));
#58292=CARTESIAN_POINT('Origin',(0.,1.2,7.2));
#58293=CARTESIAN_POINT('Origin',(0.,0.92691742076555,7.2));
#58294=CARTESIAN_POINT('Origin',(0.,0.653834841531101,7.2));
#58295=CARTESIAN_POINT('Origin',(0.,0.,7.2));
#58296=CARTESIAN_POINT('Origin',(0.,-0.653834841531101,7.2));
#58297=CARTESIAN_POINT('Origin',(0.,-0.926917420765551,7.2));
#58298=CARTESIAN_POINT('Origin',(0.,-1.2,7.2));
#58299=CARTESIAN_POINT('Origin',(0.,-1.25,7.2));
#58300=CARTESIAN_POINT('Ctrl Pts',(3.1537141966502,-1.30000000000047,11.1373326796344));
#58301=CARTESIAN_POINT('Ctrl Pts',(3.19010469464722,-1.1851427086121,11.1151799568439));
#58302=CARTESIAN_POINT('Ctrl Pts',(3.21244012754455,-1.06847604194528,11.089591721371));
#58303=CARTESIAN_POINT('Ctrl Pts',(3.231569433639,-0.794772684000851,11.0225410569516));
#58304=CARTESIAN_POINT('Ctrl Pts',(3.19184909016007,-0.636309800095197,
10.9649130969828));
#58305=CARTESIAN_POINT('Ctrl Pts',(3.17031238807978,-0.319434907277159,
10.8939627249912));
#58306=CARTESIAN_POINT('Ctrl Pts',(3.14286241424732,-0.158333333333332,
10.857218797395));
#58307=CARTESIAN_POINT('Ctrl Pts',(3.16838675811282,0.158333333333334,10.8349383562761));
#58308=CARTESIAN_POINT('Ctrl Pts',(3.22246485929617,0.319434907277167,10.8483292952657));
#58309=CARTESIAN_POINT('Ctrl Pts',(3.29374448453208,0.636309800095206,10.8760807149496));
#58310=CARTESIAN_POINT('Ctrl Pts',(3.36008858048819,0.79477268400084,10.9096135331648));
#58311=CARTESIAN_POINT('Ctrl Pts',(3.37703616937003,1.06847604194602,10.9476988830827));
#58312=CARTESIAN_POINT('Ctrl Pts',(3.36817625250779,1.18514270861357,10.9633184123723));
#58313=CARTESIAN_POINT('Ctrl Pts',(3.34312043552638,1.30000000000265,10.9780717341732));
#58314=CARTESIAN_POINT('Ctrl Pts',(3.14788284318891,-1.30000000000047,11.1350257766576));
#58315=CARTESIAN_POINT('Ctrl Pts',(3.18318073065629,-1.1851427086121,11.1124051525731));
#58316=CARTESIAN_POINT('Ctrl Pts',(3.20470961435297,-1.06847604194528,11.0864845546345));
#58317=CARTESIAN_POINT('Ctrl Pts',(3.22263648934064,-0.794772684000851,
11.018979188238));
#58318=CARTESIAN_POINT('Ctrl Pts',(3.18306078465209,-0.636309800095197,
10.9615168342817));
#58319=CARTESIAN_POINT('Ctrl Pts',(3.16145464956688,-0.319434907277159,
10.8905991595008));
#58320=CARTESIAN_POINT('Ctrl Pts',(3.13444040099099,-0.158333333333332,
10.8539097309809));
#58321=CARTESIAN_POINT('Ctrl Pts',(3.15982488510821,0.158333333333334,10.8318180571571));
#58322=CARTESIAN_POINT('Ctrl Pts',(3.21328105994455,0.319434907277167,10.8454018207915));
#58323=CARTESIAN_POINT('Ctrl Pts',(3.28443962792562,0.636309800095206,10.8733857734295));
#58324=CARTESIAN_POINT('Ctrl Pts',(3.35057865834427,0.794772684000841,10.9068490294079));
#58325=CARTESIAN_POINT('Ctrl Pts',(3.3687568274511,1.06847604194602,10.9453628297153));
#58326=CARTESIAN_POINT('Ctrl Pts',(3.36075240801503,1.18514270861357,10.9612527084174));
#58327=CARTESIAN_POINT('Ctrl Pts',(3.33687491330406,1.30000000000265,10.9763612687455));
#58328=CARTESIAN_POINT('Ctrl Pts',(3.13602666513719,-1.30000000000068,11.130616336331));
#58329=CARTESIAN_POINT('Ctrl Pts',(3.16922239039855,-1.18514270861229,11.1069731541362));
#58330=CARTESIAN_POINT('Ctrl Pts',(3.18921085134169,-1.06847604194545,11.0803090987668));
#58331=CARTESIAN_POINT('Ctrl Pts',(3.20487677211899,-0.794772684000972,
11.0117309753808));
#58332=CARTESIAN_POINT('Ctrl Pts',(3.1657701772128,-0.636309800095298,10.9543717086895));
#58333=CARTESIAN_POINT('Ctrl Pts',(3.14388752510033,-0.319434907277211,
10.883684741697));
#58334=CARTESIAN_POINT('Ctrl Pts',(3.11727844371661,-0.158333333333358,
10.847669131426));
#58335=CARTESIAN_POINT('Ctrl Pts',(3.1422984644438,0.15833333333336,10.8260597126675));
#58336=CARTESIAN_POINT('Ctrl Pts',(3.19482368720396,0.319434907277218,10.8396543810191));
#58337=CARTESIAN_POINT('Ctrl Pts',(3.26584498679678,0.636309800095308,10.8679775321775));
#58338=CARTESIAN_POINT('Ctrl Pts',(3.33149867825249,0.794772684000967,10.9013899895613));
#58339=CARTESIAN_POINT('Ctrl Pts',(3.35214112151248,1.06847604194619,10.9407558898041));
#58340=CARTESIAN_POINT('Ctrl Pts',(3.34585397033878,1.18514270861376,10.9571786227287));
#58341=CARTESIAN_POINT('Ctrl Pts',(3.32434431918199,1.30000000000286,10.9729840490132));
#58342=CARTESIAN_POINT('Ctrl Pts',(3.11338370685469,-1.30000000000069,11.120683044156));
#58343=CARTESIAN_POINT('Ctrl Pts',(3.14116836728438,-1.1851427086123,11.0963251324237));
#58344=CARTESIAN_POINT('Ctrl Pts',(3.15731256495897,-1.06847604194546,11.0690090454575));
#58345=CARTESIAN_POINT('Ctrl Pts',(3.16771709359208,-0.794772684000982,
10.99906944343));
#58346=CARTESIAN_POINT('Ctrl Pts',(3.1305800846218,-0.636309800095302,10.9407498665654));
#58347=CARTESIAN_POINT('Ctrl Pts',(3.10895551659859,-0.319434907277212,
10.8695500110699));
#58348=CARTESIAN_POINT('Ctrl Pts',(3.08391518852437,-0.158333333333359,
10.8339834973426));
#58349=CARTESIAN_POINT('Ctrl Pts',(3.10868004152326,0.15833333333336,10.8127199071209));
#58350=CARTESIAN_POINT('Ctrl Pts',(3.15926311797835,0.31943490727722,10.8263292826878));
#58351=CARTESIAN_POINT('Ctrl Pts',(3.22974739154896,0.636309800095311,10.855629443145));
#58352=CARTESIAN_POINT('Ctrl Pts',(3.29371057080877,0.794772684000972,10.889880846898));
#58353=CARTESIAN_POINT('Ctrl Pts',(3.31929399286086,1.0684760419462,10.9309844151448));
#58354=CARTESIAN_POINT('Ctrl Pts',(3.31661522091182,1.18514270861377,10.9482825629363));
#58355=CARTESIAN_POINT('Ctrl Pts',(3.30018356156654,1.30000000000287,10.9650866468623));
#58356=CARTESIAN_POINT('Ctrl Pts',(3.09576113927307,-1.30000000000115,11.1135336035834));
#58357=CARTESIAN_POINT('Ctrl Pts',(3.12083758156332,-1.18514270861272,11.0870492973935));
#58358=CARTESIAN_POINT('Ctrl Pts',(3.13490280767704,-1.06847604194583,11.0582957397077));
#58359=CARTESIAN_POINT('Ctrl Pts',(3.14195818158455,-0.794772684001263,
10.9866268444063));
#58360=CARTESIAN_POINT('Ctrl Pts',(3.10452754684833,-0.636309800095527,
10.9296607803433));
#58361=CARTESIAN_POINT('Ctrl Pts',(3.08238301721418,-0.319434907277325,
10.8589183599512));
#58362=CARTESIAN_POINT('Ctrl Pts',(3.05856153306589,-0.158333333333415,
10.8236494878642));
#58363=CARTESIAN_POINT('Ctrl Pts',(3.08296219079103,0.158333333333416,10.8028618150431));
#58364=CARTESIAN_POINT('Ctrl Pts',(3.1320895193213,0.319434907277332,10.8164895636833));
#58365=CARTESIAN_POINT('Ctrl Pts',(3.20209263179147,0.636309800095535,10.8466274087751));
#58366=CARTESIAN_POINT('Ctrl Pts',(3.26472168061616,0.794772684001252,10.8815622465489));
#58367=CARTESIAN_POINT('Ctrl Pts',(3.29400317768701,1.06847604194657,10.9240379528181));
#58368=CARTESIAN_POINT('Ctrl Pts',(3.29404630057274,1.18514270861419,10.9420167516264));
#58369=CARTESIAN_POINT('Ctrl Pts',(3.28145767124855,1.30000000000333,10.959588189879));
#58370=CARTESIAN_POINT('Ctrl Pts',(3.08395155918141,-1.30000000000119,11.1085139514224));
#58371=CARTESIAN_POINT('Ctrl Pts',(3.10642269462814,-1.18514270861275,11.0814385633059));
#58372=CARTESIAN_POINT('Ctrl Pts',(3.11862776653224,-1.06847604194586,11.0522016390918));
#58373=CARTESIAN_POINT('Ctrl Pts',(3.12310726374452,-0.794772684001286,
10.9796649145319));
#58374=CARTESIAN_POINT('Ctrl Pts',(3.08651157953333,-0.636309800095545,
10.9224190632179));
#58375=CARTESIAN_POINT('Ctrl Pts',(3.06452565510273,-0.319434907277333,
10.8513822824859));
#58376=CARTESIAN_POINT('Ctrl Pts',(3.04169295933292,-0.158333333333419,
10.8161325434434));
#58377=CARTESIAN_POINT('Ctrl Pts',(3.06589214051835,0.158333333333421,10.7956070164919));
#58378=CARTESIAN_POINT('Ctrl Pts',(3.11366321570065,0.319434907277342,10.8096745092449));
#58379=CARTESIAN_POINT('Ctrl Pts',(3.18343543624268,0.636309800095554,10.8402399594697));
#58380=CARTESIAN_POINT('Ctrl Pts',(3.24572403615328,0.794772684001273,10.8749119240156));
#58381=CARTESIAN_POINT('Ctrl Pts',(3.27752379286743,1.06847604194661,10.9183325711489));
#58382=CARTESIAN_POINT('Ctrl Pts',(3.27930056278751,1.18514270861422,10.9369373016276));
#58383=CARTESIAN_POINT('Ctrl Pts',(3.26908916624317,1.30000000000337,10.9553515733346));
#58384=CARTESIAN_POINT('Ctrl Pts',(3.08341596161804,-1.30000000000119,11.1082843545824));
#58385=CARTESIAN_POINT('Ctrl Pts',(3.10576966356819,-1.18514270861275,11.0811808930218));
#58386=CARTESIAN_POINT('Ctrl Pts',(3.11789072402595,-1.06847604194586,11.051921328677));
#58387=CARTESIAN_POINT('Ctrl Pts',(3.12225334961287,-0.794772684001286,
10.9793448529261));
#58388=CARTESIAN_POINT('Ctrl Pts',(3.08569374856489,-0.636309800095544,
10.9220884814296));
#58389=CARTESIAN_POINT('Ctrl Pts',(3.06371464384983,-0.319434907277333,
10.8510387599166));
#58390=CARTESIAN_POINT('Ctrl Pts',(3.04092785396088,-0.158333333333419,
10.8157887502987));
#58391=CARTESIAN_POINT('Ctrl Pts',(3.06511770359802,0.158333333333421,10.7952753476931));
#58392=CARTESIAN_POINT('Ctrl Pts',(3.1128263871204,0.319434907277341,10.8093637144019));
#58393=CARTESIAN_POINT('Ctrl Pts',(3.18258735290783,0.636309800095553,10.8399495306449));
#58394=CARTESIAN_POINT('Ctrl Pts',(3.2448599450106,0.794772684001273,10.8746102076726));
#58395=CARTESIAN_POINT('Ctrl Pts',(3.27677390434896,1.0684760419466,10.9180741625951));
#58396=CARTESIAN_POINT('Ctrl Pts',(3.27862948272818,1.18514270861422,10.9367073567007));
#58397=CARTESIAN_POINT('Ctrl Pts',(3.26852626901772,1.30000000000336,10.9551598093241));
#58398=CARTESIAN_POINT('Ctrl Pts',(3.08288070241116,-1.30000000000119,11.1080543928536));
#58399=CARTESIAN_POINT('Ctrl Pts',(3.10511696606915,-1.18514270861275,11.0809228689106));
#58400=CARTESIAN_POINT('Ctrl Pts',(3.11715401779151,-1.06847604194586,11.0516406634302));
#58401=CARTESIAN_POINT('Ctrl Pts',(3.12139979535742,-0.794772684001286,
10.9790244062912));
#58402=CARTESIAN_POINT('Ctrl Pts',(3.08487644576444,-0.636309800095544,
10.9217573025874));
#58403=CARTESIAN_POINT('Ctrl Pts',(3.06290395870727,-0.319434907277333,
10.8506948674407));
#58404=CARTESIAN_POINT('Ctrl Pts',(3.04016247600659,-0.158333333333419,
10.8154452967412));
#58405=CARTESIAN_POINT('Ctrl Pts',(3.06434307409562,0.158333333333421,10.794943901965));
#58406=CARTESIAN_POINT('Ctrl Pts',(3.11199021357481,0.319434907277341,10.8090520991058));
#58407=CARTESIAN_POINT('Ctrl Pts',(3.18173994553404,0.636309800095553,10.8396582599428));
#58408=CARTESIAN_POINT('Ctrl Pts',(3.24399568012213,0.794772684001273,10.8743087136978));
#58409=CARTESIAN_POINT('Ctrl Pts',(3.27602373403694,1.0684760419466,10.9178161103825));
#58410=CARTESIAN_POINT('Ctrl Pts',(3.27795821323474,1.18514270861422,10.9364776510779));
#58411=CARTESIAN_POINT('Ctrl Pts',(3.26796341384691,1.30000000000337,10.9549679925518));
#58412=CARTESIAN_POINT('Ctrl Pts',(3.08181165107633,-1.30000000000119,11.1075927560609));
#58413=CARTESIAN_POINT('Ctrl Pts',(3.10381413880235,-1.18514270861275,11.0804037955591));
#58414=CARTESIAN_POINT('Ctrl Pts',(3.1156837899324,-1.06847604194586,11.0510755651735));
#58415=CARTESIAN_POINT('Ctrl Pts',(3.11969617895471,-0.794772684001285,
10.9783793444991));
#58416=CARTESIAN_POINT('Ctrl Pts',(3.08324360047865,-0.636309800095544,
10.9210927847102));
#58417=CARTESIAN_POINT('Ctrl Pts',(3.06128354178067,-0.319434907277333,
10.8500058420244));
#58418=CARTESIAN_POINT('Ctrl Pts',(3.03863258335772,-0.158333333333419,
10.8147572582684));
#58419=CARTESIAN_POINT('Ctrl Pts',(3.06279464256912,0.158333333333421,10.7942798959418));
#58420=CARTESIAN_POINT('Ctrl Pts',(3.11031943612699,0.319434907277341,10.8084268192463));
#58421=CARTESIAN_POINT('Ctrl Pts',(3.18004603340595,0.636309800095553,10.8390744996214));
#58422=CARTESIAN_POINT('Ctrl Pts',(3.24226610208176,0.794772684001273,10.8737069492674));
#58423=CARTESIAN_POINT('Ctrl Pts',(3.27452197278349,1.0684760419466,10.9173017153762));
#58424=CARTESIAN_POINT('Ctrl Pts',(3.27661445517721,1.18514270861422,10.9360197102487));
#58425=CARTESIAN_POINT('Ctrl Pts',(3.26683704873562,1.30000000000336,10.9545851410903));
#58426=CARTESIAN_POINT('Ctrl Pts',(3.07950184481962,-1.30000000000118,11.1065850333065));
#58427=CARTESIAN_POINT('Ctrl Pts',(3.1010025742002,-1.18514270861275,11.0792660257947));
#58428=CARTESIAN_POINT('Ctrl Pts',(3.11251225821232,-1.06847604194586,11.0498348291874));
#58429=CARTESIAN_POINT('Ctrl Pts',(3.11602061728179,-0.794772684001284,
10.9769632979818));
#58430=CARTESIAN_POINT('Ctrl Pts',(3.07971509019369,-0.636309800095543,
10.9196417946398));
#58431=CARTESIAN_POINT('Ctrl Pts',(3.0577775182899,-0.319434907277332,10.8485068344066));
#58432=CARTESIAN_POINT('Ctrl Pts',(3.03531907925591,-0.158333333333419,
10.8132646959073));
#58433=CARTESIAN_POINT('Ctrl Pts',(3.05944102836239,0.15833333333342,10.7928391501656));
#58434=CARTESIAN_POINT('Ctrl Pts',(3.10670776553142,0.319434907277341,10.8070612599296));
#58435=CARTESIAN_POINT('Ctrl Pts',(3.17638196737474,0.636309800095552,10.8378017732288));
#58436=CARTESIAN_POINT('Ctrl Pts',(3.23851358524906,0.794772684001271,10.872409253674));
#58437=CARTESIAN_POINT('Ctrl Pts',(3.27126108509779,1.0684760419466,10.9161958468731));
#58438=CARTESIAN_POINT('Ctrl Pts',(3.27369701287854,1.18514270861422,10.9350347990276));
#58439=CARTESIAN_POINT('Ctrl Pts',(3.26439368916993,1.30000000000336,10.9537591095938));
#58440=CARTESIAN_POINT('Ctrl Pts',(3.07597350333202,-1.30000000000118,11.1050046386546));
#58441=CARTESIAN_POINT('Ctrl Pts',(3.09673378701756,-1.18514270861275,11.0774491271937));
#58442=CARTESIAN_POINT('Ctrl Pts',(3.10770797139586,-1.06847604194586,11.0478383027321));
#58443=CARTESIAN_POINT('Ctrl Pts',(3.11045268558565,-0.794772684001281,
10.9746831904049));
#58444=CARTESIAN_POINT('Ctrl Pts',(3.07433384945607,-0.636309800095541,
10.9173531191264));
#58445=CARTESIAN_POINT('Ctrl Pts',(3.0524013309648,-0.319434907277331,10.8461785054774));
#58446=CARTESIAN_POINT('Ctrl Pts',(3.03021210964003,-0.158333333333418,
10.8109786470852));
#58447=CARTESIAN_POINT('Ctrl Pts',(3.05427344270787,0.15833333333342,10.7906306695322));
#58448=CARTESIAN_POINT('Ctrl Pts',(3.10119167687428,0.319434907277339,10.8049086363646));
#58449=CARTESIAN_POINT('Ctrl Pts',(3.17077538272656,0.636309800095549,10.8358049063499));
#58450=CARTESIAN_POINT('Ctrl Pts',(3.23270260284628,0.794772684001268,10.8704599665709));
#58451=CARTESIAN_POINT('Ctrl Pts',(3.26619776529465,1.0684760419466,10.9145527946046));
#58452=CARTESIAN_POINT('Ctrl Pts',(3.26917063872204,1.18514270861421,10.9335671180071));
#58453=CARTESIAN_POINT('Ctrl Pts',(3.26061757087094,1.30000000000336,10.9525096133565));
#58454=CARTESIAN_POINT('Ctrl Pts',(3.07177387932149,-1.30000000000117,11.1030656186361));
#58455=CARTESIAN_POINT('Ctrl Pts',(3.09170713418827,-1.18514270861274,11.0751554212305));
#58456=CARTESIAN_POINT('Ctrl Pts',(3.10207532349415,-1.06847604194585,11.0452868189214));
#58457=CARTESIAN_POINT('Ctrl Pts',(3.10393070000947,-0.794772684001278,
10.9717600652894));
#58458=CARTESIAN_POINT('Ctrl Pts',(3.06796806118652,-0.636309800095538,
10.9144970405492));
#58459=CARTESIAN_POINT('Ctrl Pts',(3.0459831831553,-0.31943490727733,10.8433430032635));
#58460=CARTESIAN_POINT('Ctrl Pts',(3.02405337612695,-0.158333333333417,
10.8082705202785));
#58461=CARTESIAN_POINT('Ctrl Pts',(3.04804154375731,0.158333333333419,10.7880145069793));
#58462=CARTESIAN_POINT('Ctrl Pts',(3.09463930414011,0.319434907277338,10.8022387181697));
#58463=CARTESIAN_POINT('Ctrl Pts',(3.16410167785525,0.636309800095547,10.8333391027576));
#58464=CARTESIAN_POINT('Ctrl Pts',(3.22566232834457,0.794772684001265,10.8682047406006));
#58465=CARTESIAN_POINT('Ctrl Pts',(3.26003709903331,1.06847604194659,10.9126873948767));
#58466=CARTESIAN_POINT('Ctrl Pts',(3.26366763250543,1.18514270861421,10.931895253368));
#58467=CARTESIAN_POINT('Ctrl Pts',(3.25604913492926,1.30000000000335,10.9510560775591));
#58468=CARTESIAN_POINT('Ctrl Pts',(3.06620149427961,-1.30000000000116,11.1004459958638));
#58469=CARTESIAN_POINT('Ctrl Pts',(3.08508608417813,-1.18514270861273,11.0720006302833));
#58470=CARTESIAN_POINT('Ctrl Pts',(3.09467918146128,-1.06847604194585,11.041750414312));
#58471=CARTESIAN_POINT('Ctrl Pts',(3.09537594857965,-0.794772684001272,
10.9676967984221));
#58472=CARTESIAN_POINT('Ctrl Pts',(3.0595662544114,-0.636309800095533,10.9105863760201));
#58473=CARTESIAN_POINT('Ctrl Pts',(3.03746693216275,-0.319434907277327,
10.8395120488657));
#58474=CARTESIAN_POINT('Ctrl Pts',(3.01583380496636,-0.158333333333416,
10.8046691506071));
#58475=CARTESIAN_POINT('Ctrl Pts',(3.03972489261492,0.158333333333418,10.7845333994117));
#58476=CARTESIAN_POINT('Ctrl Pts',(3.08597416646741,0.319434907277335,10.7985872716408));
#58477=CARTESIAN_POINT('Ctrl Pts',(3.15526102104843,0.636309800095542,10.8299771972321));
#58478=CARTESIAN_POINT('Ctrl Pts',(3.21622770109064,0.794772684001259,10.8652563127961));
#58479=CARTESIAN_POINT('Ctrl Pts',(3.25176067465168,1.06847604194659,10.9102776134802));
#58480=CARTESIAN_POINT('Ctrl Pts',(3.25628033569737,1.1851427086142,10.9297283604134));
#58481=CARTESIAN_POINT('Ctrl Pts',(3.24993875016055,1.30000000000334,10.9491418014171));
#58482=CARTESIAN_POINT('Ctrl Pts',(3.05922678790802,-1.30000000000116,11.0971785950227));
#58483=CARTESIAN_POINT('Ctrl Pts',(3.07679748390835,-1.18514270861272,11.0680662244352));
#58484=CARTESIAN_POINT('Ctrl Pts',(3.08542594740892,-1.06847604194584,11.0373330959707));
#58485=CARTESIAN_POINT('Ctrl Pts',(3.08470107825154,-0.794772684001268,
10.9625891461495));
#58486=CARTESIAN_POINT('Ctrl Pts',(3.04913580107163,-0.63630980009553,10.9056096207377));
#58487=CARTESIAN_POINT('Ctrl Pts',(3.02692196067527,-0.319434907277326,
10.8346023343472));
#58488=CARTESIAN_POINT('Ctrl Pts',(3.00566068203787,-0.158333333333415,
10.8000457612598));
#58489=CARTESIAN_POINT('Ctrl Pts',(3.02941139388343,0.158333333333417,10.7800807424224));
#58490=CARTESIAN_POINT('Ctrl Pts',(3.07517120501442,0.319434907277334,10.7939819781425));
#58491=CARTESIAN_POINT('Ctrl Pts',(3.14424027851699,0.636309800095539,10.8257280878312));
#58492=CARTESIAN_POINT('Ctrl Pts',(3.20454890558993,0.794772684001255,10.8614200894816));
#58493=CARTESIAN_POINT('Ctrl Pts',(3.24150684993767,1.06847604194658,10.9071433700823));
#58494=CARTESIAN_POINT('Ctrl Pts',(3.24710649000357,1.18514270861419,10.9269372083692));
#58495=CARTESIAN_POINT('Ctrl Pts',(3.24230804545396,1.30000000000333,10.9467329709854));
#58496=CARTESIAN_POINT('Ctrl Pts',(3.04789713145505,-1.30000000000113,11.0921479553257));
#58497=CARTESIAN_POINT('Ctrl Pts',(3.06310098927792,-1.1851427086127,11.0622687081769));
#58498=CARTESIAN_POINT('Ctrl Pts',(3.0700383418749,-1.06847604194582,11.0309301451772));
#58499=CARTESIAN_POINT('Ctrl Pts',(3.06696773340605,-0.794772684001254,
10.9551604838395));
#58500=CARTESIAN_POINT('Ctrl Pts',(3.03213313253594,-0.636309800095519,
10.8980052996912));
#58501=CARTESIAN_POINT('Ctrl Pts',(3.01009318290283,-0.31943490727732,10.8266908353565));
#58502=CARTESIAN_POINT('Ctrl Pts',(2.9898278833591,-0.158333333333412,10.7921197278034));
#58503=CARTESIAN_POINT('Ctrl Pts',(3.01337288367669,0.158333333333414,10.7724076110835));
#58504=CARTESIAN_POINT('Ctrl Pts',(3.05781174577527,0.319434907277328,10.7867090965629));
#58505=CARTESIAN_POINT('Ctrl Pts',(3.12653082973974,0.636309800095527,10.8190069967226));
#58506=CARTESIAN_POINT('Ctrl Pts',(3.18631825942563,0.794772684001241,10.8546786608675));
#58507=CARTESIAN_POINT('Ctrl Pts',(3.22561474329067,1.06847604194656,10.9014569816872));
#58508=CARTESIAN_POINT('Ctrl Pts',(3.23287752278965,1.18514270861417,10.9218892880775));
#58509=CARTESIAN_POINT('Ctrl Pts',(3.23039309000059,1.30000000000331,10.942505299083));
#58510=CARTESIAN_POINT('Ctrl Pts',(3.0336791792996,-1.30000000000107,11.0859062407189));
#58511=CARTESIAN_POINT('Ctrl Pts',(3.04592990848317,-1.18514270861265,11.0550577019385));
#58512=CARTESIAN_POINT('Ctrl Pts',(3.05075153694945,-1.06847604194577,11.0229615337635));
#58513=CARTESIAN_POINT('Ctrl Pts',(3.04472775442659,-0.794772684001217,
10.9459306909737));
#58514=CARTESIAN_POINT('Ctrl Pts',(3.01076502342817,-0.636309800095489,
10.8886050922641));
#58515=CARTESIAN_POINT('Ctrl Pts',(2.9889037303266,-0.319434907277305,10.8169567751465));
#58516=CARTESIAN_POINT('Ctrl Pts',(2.96982639463246,-0.158333333333405,
10.7824447163113));
#58517=CARTESIAN_POINT('Ctrl Pts',(2.99317826302666,0.158333333333407,10.7629740839303));
#58518=CARTESIAN_POINT('Ctrl Pts',(3.03618964023698,0.319434907277314,10.7774983840959));
#58519=CARTESIAN_POINT('Ctrl Pts',(3.10443116313559,0.636309800095498,10.8105397740011));
#58520=CARTESIAN_POINT('Ctrl Pts',(3.16327335920585,0.794772684001204,10.8465592557145));
#58521=CARTESIAN_POINT('Ctrl Pts',(3.20537962279033,1.06847604194651,10.8947916765656));
#58522=CARTESIAN_POINT('Ctrl Pts',(3.21470826575225,1.18514270861411,10.9160326456722));
#58523=CARTESIAN_POINT('Ctrl Pts',(3.21513931036113,1.30000000000325,10.9376365560862));
#58524=CARTESIAN_POINT('Ctrl Pts',(3.01154573504434,-1.30000000000098,11.0752210934067));
#58525=CARTESIAN_POINT('Ctrl Pts',(3.01953178645156,-1.18514270861257,11.0422906197895));
#58526=CARTESIAN_POINT('Ctrl Pts',(3.0212728629428,-1.0684760419457,11.0086306666878));
#58527=CARTESIAN_POINT('Ctrl Pts',(3.01086795657992,-0.794772684001161,
10.9291841978312));
#58528=CARTESIAN_POINT('Ctrl Pts',(2.97811254408224,-0.636309800095444,
10.871806941579));
#58529=CARTESIAN_POINT('Ctrl Pts',(2.95609681690904,-0.319434907277283,
10.8001194966574));
#58530=CARTESIAN_POINT('Ctrl Pts',(2.9382621750574,-0.158333333333394,10.7664414319515));
#58531=CARTESIAN_POINT('Ctrl Pts',(2.96090895269562,0.158333333333396,10.7477962611558));
#58532=CARTESIAN_POINT('Ctrl Pts',(3.00158302123252,0.319434907277291,10.7627472791991));
#58533=CARTESIAN_POINT('Ctrl Pts',(3.06933619159502,0.636309800095453,10.7966226289519));
#58534=CARTESIAN_POINT('Ctrl Pts',(3.1273686119044,0.794772684001148,10.8323048514524));
#58535=CARTESIAN_POINT('Ctrl Pts',(3.17421656341115,1.06847604194644,10.8825900038451));
#58536=CARTESIAN_POINT('Ctrl Pts',(3.18684759319335,1.18514270861404,10.9051546963106));
#58537=CARTESIAN_POINT('Ctrl Pts',(3.19183091043806,1.30000000000316,10.9285175020193));
#58538=CARTESIAN_POINT('Ctrl Pts',(2.98919530248008,-1.30000000000088,11.0647296599117));
#58539=CARTESIAN_POINT('Ctrl Pts',(2.99291765020551,-1.18514270861247,11.0297155831156));
#58540=CARTESIAN_POINT('Ctrl Pts',(2.99153880663323,-1.06847604194561,10.9945342094214));
#58541=CARTESIAN_POINT('Ctrl Pts',(2.97656862975705,-0.794772684001099,
10.9128717088757));
#58542=CARTESIAN_POINT('Ctrl Pts',(2.94457308631418,-0.636309800095394,
10.8559300267459));
#58543=CARTESIAN_POINT('Ctrl Pts',(2.92246346658274,-0.319434907277257,
10.7841365189799));
#58544=CARTESIAN_POINT('Ctrl Pts',(2.90620251148595,-0.158333333333381,
10.7509517716306));
#58545=CARTESIAN_POINT('Ctrl Pts',(2.92874230896034,0.158333333333383,10.7324383617579));
#58546=CARTESIAN_POINT('Ctrl Pts',(2.96787991341664,0.319434907277266,10.7468429609936));
#58547=CARTESIAN_POINT('Ctrl Pts',(3.03521533464832,0.636309800095403,10.7814693124496));
#58548=CARTESIAN_POINT('Ctrl Pts',(3.09169297791346,0.794772684001086,10.8177130535361));
#58549=CARTESIAN_POINT('Ctrl Pts',(3.14276914107174,1.06847604194635,10.8706653479746));
#58550=CARTESIAN_POINT('Ctrl Pts',(3.15850488309139,1.18514270861394,10.8947887211331));
#58551=CARTESIAN_POINT('Ctrl Pts',(3.16786738865772,1.30000000000305,10.9201143812634));
#58552=CARTESIAN_POINT('Ctrl Pts',(2.96717524641191,-1.30000000000084,11.0538796667386));
#58553=CARTESIAN_POINT('Ctrl Pts',(2.96648675545647,-1.18514270861244,11.0169140357705));
#58554=CARTESIAN_POINT('Ctrl Pts',(2.96202768339402,-1.06847604194558,10.9801481702247));
#58555=CARTESIAN_POINT('Ctrl Pts',(2.94301553823612,-0.794772684001075,
10.8956731639161));
#58556=CARTESIAN_POINT('Ctrl Pts',(2.91320656941111,-0.636309800095375,
10.8376308550638));
#58557=CARTESIAN_POINT('Ctrl Pts',(2.89125645448967,-0.319434907277247,
10.7654460382644));
#58558=CARTESIAN_POINT('Ctrl Pts',(2.87579921818227,-0.158333333333377,
10.7335738837162));
#58559=CARTESIAN_POINT('Ctrl Pts',(2.89754362678226,0.158333333333378,10.7159400313523));
#58560=CARTESIAN_POINT('Ctrl Pts',(2.93469623921681,0.319434907277257,10.7302971169921));
#58561=CARTESIAN_POINT('Ctrl Pts',(3.0010380244238,0.636309800095384,10.7663210928599));
#58562=CARTESIAN_POINT('Ctrl Pts',(3.05548748670998,0.794772684001061,10.8036733359117));
#58563=CARTESIAN_POINT('Ctrl Pts',(3.11102365523955,1.06847604194632,10.8590380958667));
#58564=CARTESIAN_POINT('Ctrl Pts',(3.13016434939635,1.1851427086139,10.8843836848376));
#58565=CARTESIAN_POINT('Ctrl Pts',(3.14440618817126,1.30000000000302,10.9111095096614));
#58566=CARTESIAN_POINT('Ctrl Pts',(2.95060113807384,-1.3000000000008,11.0457492105973));
#58567=CARTESIAN_POINT('Ctrl Pts',(2.94723873270801,-1.1851427086124,11.0066494327933));
#58568=CARTESIAN_POINT('Ctrl Pts',(2.94073223438963,-1.06847604194555,10.968421535658));
#58569=CARTESIAN_POINT('Ctrl Pts',(2.91843743795963,-0.794772684001051,
10.8821216645747));
#58570=CARTESIAN_POINT('Ctrl Pts',(2.8881619930355,-0.636309800095356,10.825518085516));
#58571=CARTESIAN_POINT('Ctrl Pts',(2.86615173620415,-0.319434907277238,
10.7532403162218));
#58572=CARTESIAN_POINT('Ctrl Pts',(2.85268458474327,-0.158333333333372,
10.7208755131832));
#58573=CARTESIAN_POINT('Ctrl Pts',(2.8745474532907,0.158333333333374,10.7031173213864));
#58574=CARTESIAN_POINT('Ctrl Pts',(2.91007273900423,0.319434907277246,10.7175764682789));
#58575=CARTESIAN_POINT('Ctrl Pts',(2.97621834270599,0.636309800095365,10.7539824537767));
#58576=CARTESIAN_POINT('Ctrl Pts',(3.03022498028522,0.794772684001038,10.7908558682582));
#58577=CARTESIAN_POINT('Ctrl Pts',(3.08879748892997,1.06847604194629,10.8483861882998));
#58578=CARTESIAN_POINT('Ctrl Pts',(3.11002664482549,1.18514270861387,10.8752013558668));
#58579=CARTESIAN_POINT('Ctrl Pts',(3.12713108794945,1.30000000000298,10.903928947163));
#58580=CARTESIAN_POINT('Ctrl Pts',(2.93497824004345,-1.30000000000077,11.0366822995914));
#58581=CARTESIAN_POINT('Ctrl Pts',(2.92821505089552,-1.18514270861238,10.996188463152));
#58582=CARTESIAN_POINT('Ctrl Pts',(2.91935717498159,-1.06847604194552,10.9567970456551));
#58583=CARTESIAN_POINT('Ctrl Pts',(2.89405456413831,-0.794772684001033,
10.868341799307));
#58584=CARTESIAN_POINT('Ctrl Pts',(2.8656757178425,-0.636309800095341,10.8106674111858));
#58585=CARTESIAN_POINT('Ctrl Pts',(2.84385408820492,-0.31943490727723,10.7380228229021));
#58586=CARTESIAN_POINT('Ctrl Pts',(2.83108911726183,-0.158333333333368,
10.7065259198157));
#58587=CARTESIAN_POINT('Ctrl Pts',(2.85192044163665,0.15833333333337,10.6898824572087));
#58588=CARTESIAN_POINT('Ctrl Pts',(2.88514032487475,0.31943490727724,10.7051740588285));
#58589=CARTESIAN_POINT('Ctrl Pts',(2.95016058666272,0.636309800095351,10.7430246094566));
#58590=CARTESIAN_POINT('Ctrl Pts',(3.00288334881758,0.794772684001019,10.7804648325827));
#58591=CARTESIAN_POINT('Ctrl Pts',(3.06495317918483,1.06847604194626,10.8396431675606));
#58592=CARTESIAN_POINT('Ctrl Pts',(3.08882703350963,1.18514270861384,10.8672818218745));
#58593=CARTESIAN_POINT('Ctrl Pts',(3.10970701250702,1.30000000000295,10.8969430220637));
#58594=CARTESIAN_POINT('Ctrl Pts',(2.91813452753457,-1.30000000000074,11.0288099698746));
#58595=CARTESIAN_POINT('Ctrl Pts',(2.90839140218389,-1.18514270861235,10.9864952742596));
#58596=CARTESIAN_POINT('Ctrl Pts',(2.89739169724188,-1.0684760419455,10.9457340364746));
#58597=CARTESIAN_POINT('Ctrl Pts',(2.86907722810858,-0.794772684001015,
10.8551562212887));
#58598=CARTESIAN_POINT('Ctrl Pts',(2.84151498740897,-0.636309800095327,
10.7975637367191));
#58599=CARTESIAN_POINT('Ctrl Pts',(2.81985692566231,-0.319434907277224,
10.7245917132736));
#58600=CARTESIAN_POINT('Ctrl Pts',(2.80818466611494,-0.158333333333365,
10.6935702763831));
#58601=CARTESIAN_POINT('Ctrl Pts',(2.82911986192055,0.158333333333366,10.6767995837835));
#58602=CARTESIAN_POINT('Ctrl Pts',(2.86154473816526,0.319434907277231,10.6912520800743));
#58603=CARTESIAN_POINT('Ctrl Pts',(2.92621818688126,0.636309800095335,10.7296524559277));
#58604=CARTESIAN_POINT('Ctrl Pts',(2.97747860298749,0.794772684001002,10.7677691469733));
#58605=CARTESIAN_POINT('Ctrl Pts',(3.04226747723685,1.06847604194624,10.829476699648));
#58606=CARTESIAN_POINT('Ctrl Pts',(3.06823542225031,1.18514270861381,10.8585815195564));
#58607=CARTESIAN_POINT('Ctrl Pts',(3.09212660927895,1.30000000000292,10.8900802463102));
#58608=CARTESIAN_POINT('Ctrl Pts',(2.90568427085915,-1.30000000000073,11.0206511408274));
#58609=CARTESIAN_POINT('Ctrl Pts',(2.89350197144723,-1.18514270861233,10.976754637072));
#58610=CARTESIAN_POINT('Ctrl Pts',(2.88071110959298,-1.06847604194549,10.9348433793974));
#58611=CARTESIAN_POINT('Ctrl Pts',(2.84975575892226,-0.794772684001005,
10.8426063054447));
#58612=CARTESIAN_POINT('Ctrl Pts',(2.82255596465368,-0.63630980009532,10.7854051223092));
#58613=CARTESIAN_POINT('Ctrl Pts',(2.80085719239994,-0.319434907277221,
10.7123354663725));
#58614=CARTESIAN_POINT('Ctrl Pts',(2.79032098272189,-0.158333333333363,
10.6814741628591));
#58615=CARTESIAN_POINT('Ctrl Pts',(2.81093878189025,0.158333333333365,10.6650291179649));
#58616=CARTESIAN_POINT('Ctrl Pts',(2.84190760268583,0.319434907277228,10.6796354868406));
#58617=CARTESIAN_POINT('Ctrl Pts',(2.90598056204028,0.636309800095328,10.7188205295066));
#58618=CARTESIAN_POINT('Ctrl Pts',(2.95630282008806,0.794772684000994,10.7571931539108));
#58619=CARTESIAN_POINT('Ctrl Pts',(3.02361144613931,1.06847604194623,10.8207183172819));
#58620=CARTESIAN_POINT('Ctrl Pts',(3.05146661032784,1.1851427086138,10.8508829861494));
#58621=CARTESIAN_POINT('Ctrl Pts',(3.0780415285176,1.3000000000029,10.8837146345004));
#58622=CARTESIAN_POINT('Ctrl Pts',(2.89444889450715,-1.30000000000072,11.0153899166469));
#58623=CARTESIAN_POINT('Ctrl Pts',(2.88028412010224,-1.18514270861233,10.970267544928));
#58624=CARTESIAN_POINT('Ctrl Pts',(2.8661099915129,-1.06847604194548,10.9273912624621));
#58625=CARTESIAN_POINT('Ctrl Pts',(2.83334330890949,-0.794772684001001,
10.8335273880978));
#58626=CARTESIAN_POINT('Ctrl Pts',(2.80700132183935,-0.636309800095317,
10.7760551249637));
#58627=CARTESIAN_POINT('Ctrl Pts',(2.78564335508256,-0.319434907277219,
10.7025319931978));
#58628=CARTESIAN_POINT('Ctrl Pts',(2.77603953129172,-0.158333333333362,
10.6717864454594));
#58629=CARTESIAN_POINT('Ctrl Pts',(2.79642245405076,0.158333333333364,10.6555809652624));
#58630=CARTESIAN_POINT('Ctrl Pts',(2.82612568804013,0.319434907277227,10.6703931004593));
#58631=CARTESIAN_POINT('Ctrl Pts',(2.88957969551012,0.636309800095326,10.710352653672));
#58632=CARTESIAN_POINT('Ctrl Pts',(2.93889565643564,0.794772684000989,10.7492262233861));
#58633=CARTESIAN_POINT('Ctrl Pts',(3.0083373396324,1.06847604194622,10.8140830608064));
#58634=CARTESIAN_POINT('Ctrl Pts',(3.03784222283995,1.1851427086138,10.8449436333644));
#58635=CARTESIAN_POINT('Ctrl Pts',(3.06679325766699,1.3000000000029,10.8785906567437));
#58636=CARTESIAN_POINT('Ctrl Pts',(2.87871424024058,-1.3000000000007,11.0063906910496));
#58637=CARTESIAN_POINT('Ctrl Pts',(2.86153048821051,-1.18514270861231,10.9594734224498));
#58638=CARTESIAN_POINT('Ctrl Pts',(2.8452054816931,-1.06847604194547,10.9152249725586));
#58639=CARTESIAN_POINT('Ctrl Pts',(2.80947532475721,-0.794772684000991,
10.8191677065502));
#58640=CARTESIAN_POINT('Ctrl Pts',(2.78419484317971,-0.636309800095306,
10.7615189991352));
#58641=CARTESIAN_POINT('Ctrl Pts',(2.76293058764447,-0.319434907277213,
10.6877317353546));
#58642=CARTESIAN_POINT('Ctrl Pts',(2.75422099359627,-0.15833333333336,10.6576623718402));
#58643=CARTESIAN_POINT('Ctrl Pts',(2.77432869962127,0.158333333333361,10.6417276821006));
#58644=CARTESIAN_POINT('Ctrl Pts',(2.80277231653527,0.319434907277222,10.6562083569586));
#58645=CARTESIAN_POINT('Ctrl Pts',(2.86575568712979,0.636309800095315,10.6968330257819));
#58646=CARTESIAN_POINT('Ctrl Pts',(2.91407875105576,0.794772684000976,10.7358410645145));
#58647=CARTESIAN_POINT('Ctrl Pts',(2.98619913099117,1.0684760419462,10.8032646501883));
#58648=CARTESIAN_POINT('Ctrl Pts',(3.01769283609529,1.18514270861378,10.835709748802));
#58649=CARTESIAN_POINT('Ctrl Pts',(3.04946200615281,1.30000000000288,10.8714147740814));
#58650=CARTESIAN_POINT('Ctrl Pts',(2.85722596337426,-1.30000000000067,10.9948506738711));
#58651=CARTESIAN_POINT('Ctrl Pts',(2.8364538696826,-1.18514270861228,10.9450867954173));
#58652=CARTESIAN_POINT('Ctrl Pts',(2.81759781234889,-1.06847604194544,10.8986636485962));
#58653=CARTESIAN_POINT('Ctrl Pts',(2.77846297505534,-0.794772684000968,
10.7991346509037));
#58654=CARTESIAN_POINT('Ctrl Pts',(2.75458928518589,-0.636309800095292,
10.741293097816));
#58655=CARTESIAN_POINT('Ctrl Pts',(2.73367131294162,-0.319434907277208,
10.666946408431));
#58656=CARTESIAN_POINT('Ctrl Pts',(2.72639850410211,-0.158333333333356,
10.637537160389));
#58657=CARTESIAN_POINT('Ctrl Pts',(2.74594336818632,0.158333333333358,10.6221453477439));
#58658=CARTESIAN_POINT('Ctrl Pts',(2.77235282520389,0.319434907277214,10.636484262179));
#58659=CARTESIAN_POINT('Ctrl Pts',(2.83391378471908,0.636309800095301,10.6788241077998));
#58660=CARTESIAN_POINT('Ctrl Pts',(2.87958190266052,0.79477268400096,10.7194951393387));
#58661=CARTESIAN_POINT('Ctrl Pts',(2.95557229660141,1.06847604194618,10.7900125175906));
#58662=CARTESIAN_POINT('Ctrl Pts',(2.99024971050842,1.18514270861375,10.823985756658));
#58663=CARTESIAN_POINT('Ctrl Pts',(3.02671111250687,1.30000000000285,10.8614078746738));
#58664=CARTESIAN_POINT('Ctrl Pts',(2.83706008972707,-1.30000000000064,10.9820037922095));
#58665=CARTESIAN_POINT('Ctrl Pts',(2.81253518548399,-1.18514270861225,10.9295618442951));
#58666=CARTESIAN_POINT('Ctrl Pts',(2.79101659633156,-1.06847604194541,10.8810982570713));
#58667=CARTESIAN_POINT('Ctrl Pts',(2.74824953988114,-0.794772684000949,
10.7783284845407));
#58668=CARTESIAN_POINT('Ctrl Pts',(2.725762568292,-0.636309800095276,10.7203131607811));
#58669=CARTESIAN_POINT('Ctrl Pts',(2.70505703675324,-0.319434907277199,
10.6455373550391));
#58670=CARTESIAN_POINT('Ctrl Pts',(2.69907374711529,-0.158333333333352,
10.6169341839772));
#58671=CARTESIAN_POINT('Ctrl Pts',(2.71811137123917,0.158333333333354,10.6020168768041));
#58672=CARTESIAN_POINT('Ctrl Pts',(2.74247756448409,0.319434907277207,10.6162470884632));
#58673=CARTESIAN_POINT('Ctrl Pts',(2.80329498416027,0.636309800095286,10.6595286163612));
#58674=CARTESIAN_POINT('Ctrl Pts',(2.84789785676197,0.794772684000939,10.7000533919715));
#58675=CARTESIAN_POINT('Ctrl Pts',(2.92740222562294,1.06847604194615,10.7740283999209));
#58676=CARTESIAN_POINT('Ctrl Pts',(2.96465501981579,1.18514270861372,10.8101951862368));
#58677=CARTESIAN_POINT('Ctrl Pts',(3.00474611284864,1.30000000000282,10.8505077189715));
#58678=CARTESIAN_POINT('Ctrl Pts',(2.81633525801835,-1.30000000000062,10.9696756101456));
#58679=CARTESIAN_POINT('Ctrl Pts',(2.78804194764148,-1.18514270861224,10.9145486304021));
#58680=CARTESIAN_POINT('Ctrl Pts',(2.76394486494591,-1.0684760419454,10.8639501740209));
#58681=CARTESIAN_POINT('Ctrl Pts',(2.71796990871058,-0.794772684000942,
10.7575194124892));
#58682=CARTESIAN_POINT('Ctrl Pts',(2.69755314336305,-0.636309800095269,
10.6986967248109));
#58683=CARTESIAN_POINT('Ctrl Pts',(2.67767079655553,-0.319434907277195,
10.6229152835093));
#58684=CARTESIAN_POINT('Ctrl Pts',(2.67340159212905,-0.15833333333335,10.5947243926643));
#58685=CARTESIAN_POINT('Ctrl Pts',(2.69171984891177,0.158333333333352,10.5804670646744));
#58686=CARTESIAN_POINT('Ctrl Pts',(2.71330489916008,0.319434907277201,10.595227423328));
#58687=CARTESIAN_POINT('Ctrl Pts',(2.77254205502706,0.636309800095276,10.6402835905659));
#58688=CARTESIAN_POINT('Ctrl Pts',(2.81526104756883,0.794772684000931,10.6815847005431));
#58689=CARTESIAN_POINT('Ctrl Pts',(2.89826319371668,1.06847604194614,10.7590494756952));
#58690=CARTESIAN_POINT('Ctrl Pts',(2.93832246151959,1.1851427086137,10.7971693128279));
#58691=CARTESIAN_POINT('Ctrl Pts',(2.98251244359048,1.30000000000279,10.8398773562828));
#58692=CARTESIAN_POINT('Ctrl Pts',(2.79912697785942,-1.30000000000055,10.9580213491864));
#58693=CARTESIAN_POINT('Ctrl Pts',(2.76797398191822,-1.18514270861218,10.9001773311542));
#58694=CARTESIAN_POINT('Ctrl Pts',(2.74183357444361,-1.06847604194534,10.8475474650426));
#58695=CARTESIAN_POINT('Ctrl Pts',(2.69302408592936,-0.794772684000901,
10.7380076797805));
#58696=CARTESIAN_POINT('Ctrl Pts',(2.67339238690378,-0.636309800095235,
10.679472442146));
#58697=CARTESIAN_POINT('Ctrl Pts',(2.65391067895453,-0.319434907277177,
10.6031350095598));
#58698=CARTESIAN_POINT('Ctrl Pts',(2.65127946748484,-0.158333333333342,
10.5751707266414));
#58699=CARTESIAN_POINT('Ctrl Pts',(2.66939714574104,0.158333333333343,10.561060519015));
#58700=CARTESIAN_POINT('Ctrl Pts',(2.68941821557786,0.319434907277186,10.5754293992273));
#58701=CARTESIAN_POINT('Ctrl Pts',(2.74728684632815,0.636309800095243,10.6219767342921));
#58702=CARTESIAN_POINT('Ctrl Pts',(2.78760864054499,0.794772684000887,10.6646274176482));
#58703=CARTESIAN_POINT('Ctrl Pts',(2.87298857137924,1.06847604194608,10.7457680695785));
#58704=CARTESIAN_POINT('Ctrl Pts',(2.9152015734891,1.18514270861364,10.7858792184749));
#58705=CARTESIAN_POINT('Ctrl Pts',(2.96266976928875,1.30000000000273,10.8309787346044));
#58706=CARTESIAN_POINT('Ctrl Pts',(2.77856646432018,-1.30000000000055,10.945473506968));
#58707=CARTESIAN_POINT('Ctrl Pts',(2.74390448340325,-1.18514270861217,10.8846512852128));
#58708=CARTESIAN_POINT('Ctrl Pts',(2.71544871744191,-1.06847604194534,10.8296097182275));
#58709=CARTESIAN_POINT('Ctrl Pts',(2.66404780361125,-0.794772684000899,
10.7158071563984));
#58710=CARTESIAN_POINT('Ctrl Pts',(2.64727915488273,-0.636309800095235,
10.6557881406909));
#58711=CARTESIAN_POINT('Ctrl Pts',(2.6284743497969,-0.319434907277178,10.5785982396017));
#58712=CARTESIAN_POINT('Ctrl Pts',(2.62626533131418,-0.158333333333342,
10.5522615108711));
#58713=CARTESIAN_POINT('Ctrl Pts',(2.64355804675884,0.158333333333343,10.5388646112871));
#58714=CARTESIAN_POINT('Ctrl Pts',(2.66173699543718,0.319434907277185,10.5528250058107));
#58715=CARTESIAN_POINT('Ctrl Pts',(2.71846023507552,0.636309800095243,10.600647568866));
#58716=CARTESIAN_POINT('Ctrl Pts',(2.75691308777398,0.794772684000889,10.643949379081));
#58717=CARTESIAN_POINT('Ctrl Pts',(2.84567449106146,1.06847604194608,10.7287033424145));
#58718=CARTESIAN_POINT('Ctrl Pts',(2.89057211835406,1.18514270861364,10.7709219103223));
#58719=CARTESIAN_POINT('Ctrl Pts',(2.94194585039009,1.30000000000272,10.8186721958546));
#58720=CARTESIAN_POINT('Ctrl Pts',(2.76402116993866,-1.30000000000053,10.9352822600269));
#58721=CARTESIAN_POINT('Ctrl Pts',(2.72705341699935,-1.18514270861216,10.8720103361742));
#58722=CARTESIAN_POINT('Ctrl Pts',(2.69699423975246,-1.06847604194533,10.815105475105));
#58723=CARTESIAN_POINT('Ctrl Pts',(2.64351171889973,-0.794772684000889,
10.6983530510131));
#58724=CARTESIAN_POINT('Ctrl Pts',(2.62767640765532,-0.636309800095225,
10.6383750495022));
#58725=CARTESIAN_POINT('Ctrl Pts',(2.60950534885464,-0.319434907277172,
10.5604641396208));
#58726=CARTESIAN_POINT('Ctrl Pts',(2.60886846140746,-0.158333333333339,
10.5341700616904));
#58727=CARTESIAN_POINT('Ctrl Pts',(2.62592147012438,0.158333333333341,10.5209421222037));
#58728=CARTESIAN_POINT('Ctrl Pts',(2.64240323947071,0.319434907277179,10.5348738755294));
#58729=CARTESIAN_POINT('Ctrl Pts',(2.69777091651019,0.636309800095232,10.5840772299315));
#58730=CARTESIAN_POINT('Ctrl Pts',(2.73440246840488,0.794772684000875,10.6282281775035));
#58731=CARTESIAN_POINT('Ctrl Pts',(2.82486322897247,1.06847604194607,10.7164281967985));
#58732=CARTESIAN_POINT('Ctrl Pts',(2.87135839004095,1.18514270861362,10.7605960620217));
#58733=CARTESIAN_POINT('Ctrl Pts',(2.92519160082957,1.3000000000027,10.8107532722481));
#58734=CARTESIAN_POINT('Ctrl Pts',(2.74940605748626,-1.30000000000051,10.9250389677115));
#58735=CARTESIAN_POINT('Ctrl Pts',(2.70981978889349,-1.18514270861214,10.8593957950081));
#58736=CARTESIAN_POINT('Ctrl Pts',(2.67807761042904,-1.06847604194531,10.8005458133735));
#58737=CARTESIAN_POINT('Ctrl Pts',(2.62286824557641,-0.794772684000878,
10.6802842132411));
#58738=CARTESIAN_POINT('Ctrl Pts',(2.61000799397286,-0.636309800095218,
10.6185138370675));
#58739=CARTESIAN_POINT('Ctrl Pts',(2.59160907804646,-0.31943490727717,10.5406157221883));
#58740=CARTESIAN_POINT('Ctrl Pts',(2.58914190271259,-0.158333333333338,
10.5174726977482));
#58741=CARTESIAN_POINT('Ctrl Pts',(2.60526434112811,0.158333333333339,10.5050278888623));
#58742=CARTESIAN_POINT('Ctrl Pts',(2.6220415134188,0.319434907277178,10.5170828129627));
#58743=CARTESIAN_POINT('Ctrl Pts',(2.67697248829484,0.636309800095228,10.5668682305745));
#58744=CARTESIAN_POINT('Ctrl Pts',(2.71160879902238,0.794772684000868,10.6120400639937));
#58745=CARTESIAN_POINT('Ctrl Pts',(2.80431283473728,1.06847604194606,10.70338432225));
#58746=CARTESIAN_POINT('Ctrl Pts',(2.85270371729135,1.18514270861361,10.7493499675256));
#58747=CARTESIAN_POINT('Ctrl Pts',(2.9093573403614,1.30000000000269,10.8017417133158));
#58748=CARTESIAN_POINT('Ctrl Pts',(2.73731735276389,-1.3000000000005,10.9165770042155));
#58749=CARTESIAN_POINT('Ctrl Pts',(2.6964303190073,-1.18514270861213,10.8484715701028));
#58750=CARTESIAN_POINT('Ctrl Pts',(2.66358967733224,-1.0684760419453,10.7879629098742));
#58751=CARTESIAN_POINT('Ctrl Pts',(2.60631000069861,-0.794772684000871,
10.6657258674321));
#58752=CARTESIAN_POINT('Ctrl Pts',(2.59248039945063,-0.63630980009521,10.6055712036968));
#58753=CARTESIAN_POINT('Ctrl Pts',(2.57341924514479,-0.319434907277165,
10.5282269350905));
#58754=CARTESIAN_POINT('Ctrl Pts',(2.57143763839085,-0.158333333333336,
10.5059113031678));
#58755=CARTESIAN_POINT('Ctrl Pts',(2.58802141554789,0.158333333333337,10.4930267753833));
#58756=CARTESIAN_POINT('Ctrl Pts',(2.60547335406668,0.319434907277174,10.5031739460727));
#58757=CARTESIAN_POINT('Ctrl Pts',(2.66058247646301,0.636309800095219,10.5528147832921));
#58758=CARTESIAN_POINT('Ctrl Pts',(2.69364714043103,0.794772684000856,10.5986380530358));
#58759=CARTESIAN_POINT('Ctrl Pts',(2.78805721331708,1.06847604194604,10.6923386658196));
#58760=CARTESIAN_POINT('Ctrl Pts',(2.83784990751017,1.1851427086136,10.7397310796062));
#58761=CARTESIAN_POINT('Ctrl Pts',(2.89656867358178,1.30000000000268,10.7939563838551));
#58762=CARTESIAN_POINT('Ctrl Pts',(2.72325603000434,-1.30000000000049,10.9058269403029));
#58763=CARTESIAN_POINT('Ctrl Pts',(2.68052254051567,-1.18514270861212,10.8345047589383));
#58764=CARTESIAN_POINT('Ctrl Pts',(2.64601328600309,-1.0684760419453,10.7719058016326));
#58765=CARTESIAN_POINT('Ctrl Pts',(2.58528963257371,-0.794772684000865,
10.6474420800289));
#58766=CARTESIAN_POINT('Ctrl Pts',(2.56935149160544,-0.636309800095207,
10.5898946254132));
#58767=CARTESIAN_POINT('Ctrl Pts',(2.54855773656525,-0.319434907277164,
10.5138629625327));
#58768=CARTESIAN_POINT('Ctrl Pts',(2.54706392153435,-0.158333333333335,
10.4927970916832));
#58769=CARTESIAN_POINT('Ctrl Pts',(2.56354371788599,0.158333333333336,10.4799758266955));
#58770=CARTESIAN_POINT('Ctrl Pts',(2.58062333772424,0.319434907277171,10.4887158780038));
#58771=CARTESIAN_POINT('Ctrl Pts',(2.6368062477542,0.636309800095216,10.5376223605652));
#58772=CARTESIAN_POINT('Ctrl Pts',(2.67064655634535,0.794772684000852,10.5820567515548));
#58773=CARTESIAN_POINT('Ctrl Pts',(2.76841994636897,1.06847604194604,10.6781287217965));
#58774=CARTESIAN_POINT('Ctrl Pts',(2.82015251793265,1.18514270861359,10.7274121893936));
#58775=CARTESIAN_POINT('Ctrl Pts',(2.88129518337976,1.30000000000268,10.7843931284875));
#58776=CARTESIAN_POINT('Ctrl Pts',(2.71361311550279,-1.30000000000047,10.898569746919));
#58777=CARTESIAN_POINT('Ctrl Pts',(2.67063753707731,-1.1851427086121,10.824130284025));
#58778=CARTESIAN_POINT('Ctrl Pts',(2.63543757366513,-1.06847604194528,10.7598223853803));
#58779=CARTESIAN_POINT('Ctrl Pts',(2.57208184264171,-0.794772684000851,
10.6346642149887));
#58780=CARTESIAN_POINT('Ctrl Pts',(2.55201129877974,-0.636309800095197,
10.5822378261051));
#58781=CARTESIAN_POINT('Ctrl Pts',(2.52893211648025,-0.319434907277159,
10.5088463219352));
#58782=CARTESIAN_POINT('Ctrl Pts',(2.52830982650113,-0.158333333333333,
10.4884080647079));
#58783=CARTESIAN_POINT('Ctrl Pts',(2.54469368659007,0.158333333333334,10.4757230851068));
#58784=CARTESIAN_POINT('Ctrl Pts',(2.56094950441052,0.319434907277167,10.4839277842833));
#58785=CARTESIAN_POINT('Ctrl Pts',(2.61892980279681,0.636309800095206,10.53056138516));
#58786=CARTESIAN_POINT('Ctrl Pts',(2.65591208556864,0.79477268400084,10.5704096562204));
#58787=CARTESIAN_POINT('Ctrl Pts',(2.75637070809838,1.06847604194602,10.6671425661737));
#58788=CARTESIAN_POINT('Ctrl Pts',(2.80906926851073,1.18514270861357,10.7179729089448));
#58789=CARTESIAN_POINT('Ctrl Pts',(2.87098157400095,1.30000000000265,10.7777615020756));
#58790=CARTESIAN_POINT('Ctrl Pts',(2.70549646903697,-1.30000000000047,10.8957209484764));
#58791=CARTESIAN_POINT('Ctrl Pts',(2.6627468523953,-1.1851427086121,10.8213914743752));
#58792=CARTESIAN_POINT('Ctrl Pts',(2.62751487735367,-1.06847604194528,10.7574269431321));
#58793=CARTESIAN_POINT('Ctrl Pts',(2.56348922287021,-0.794772684000851,
10.6336011714019));
#58794=CARTESIAN_POINT('Ctrl Pts',(2.54183416968341,-0.636309800095197,
10.5831927997129));
#58795=CARTESIAN_POINT('Ctrl Pts',(2.51776513723769,-0.319434907277159,
10.5111668553313));
#58796=CARTESIAN_POINT('Ctrl Pts',(2.5171210925739,-0.158333333333333,10.4906809863802));
#58797=CARTESIAN_POINT('Ctrl Pts',(2.53338410693288,0.158333333333334,10.4781996815688));
#58798=CARTESIAN_POINT('Ctrl Pts',(2.54937394678571,0.319434907277167,10.4868805779095));
#58799=CARTESIAN_POINT('Ctrl Pts',(2.60843787791201,0.636309800095206,10.5321053630787));
#58800=CARTESIAN_POINT('Ctrl Pts',(2.64769917658169,0.79477268400084,10.5691036076304));
#58801=CARTESIAN_POINT('Ctrl Pts',(2.74872068765979,1.06847604194602,10.6646142935777));
#58802=CARTESIAN_POINT('Ctrl Pts',(2.80123722412148,1.18514270861357,10.7153390608067));
#58803=CARTESIAN_POINT('Ctrl Pts',(2.86254182811488,1.30000000000265,10.7754455583378));
#58804=CARTESIAN_POINT('Ctrl Pts',(2.70549646903679,-1.3,10.8957209484761));
#58805=CARTESIAN_POINT('Ctrl Pts',(2.6627468523952,-1.18514270861178,10.821391474375));
#58806=CARTESIAN_POINT('Ctrl Pts',(2.62751487735363,-1.06847604194512,10.757426943132));
#58807=CARTESIAN_POINT('Ctrl Pts',(2.56348922287021,-0.794772684000851,
10.6336011714019));
#58808=CARTESIAN_POINT('Ctrl Pts',(2.54183416968341,-0.636309800095197,
10.5831927997129));
#58809=CARTESIAN_POINT('Ctrl Pts',(2.5177651372377,-0.319434907277159,10.5111668553313));
#58810=CARTESIAN_POINT('Ctrl Pts',(2.5171210925739,-0.158333333333332,10.4906809863802));
#58811=CARTESIAN_POINT('Ctrl Pts',(2.53338410693288,0.158333333333334,10.4781996815689));
#58812=CARTESIAN_POINT('Ctrl Pts',(2.54937394678571,0.319434907277167,10.4868805779095));
#58813=CARTESIAN_POINT('Ctrl Pts',(2.60843787791201,0.636309800095206,10.5321053630787));
#58814=CARTESIAN_POINT('Ctrl Pts',(2.64769917658169,0.79477268400084,10.5691036076304));
#58815=CARTESIAN_POINT('Ctrl Pts',(2.74872068765945,1.06847604194511,10.6646142935774));
#58816=CARTESIAN_POINT('Ctrl Pts',(2.80123722412067,1.18514270861178,10.715339060806));
#58817=CARTESIAN_POINT('Ctrl Pts',(2.86254182811346,1.3,10.7754455583364));
#58818=CARTESIAN_POINT('',(3.07986858154633,-1.2,11.0751657410237));
#58819=CARTESIAN_POINT('Ctrl Pts',(3.07986858154632,-1.2,11.0751657410237));
#58820=CARTESIAN_POINT('Ctrl Pts',(3.0588058189093,-1.21682649969802,11.0704122326966));
#58821=CARTESIAN_POINT('Ctrl Pts',(3.03724316373786,-1.23325202986004,11.0664907783325));
#58822=CARTESIAN_POINT('Ctrl Pts',(3.00532794741497,-1.25864588707498,11.0591965660954));
#58823=CARTESIAN_POINT('Ctrl Pts',(2.99504873255066,-1.26676696435895,11.0569015286308));
#58824=CARTESIAN_POINT('Ctrl Pts',(2.97662419564679,-1.28142016386729,11.0526365617568));
#58825=CARTESIAN_POINT('Ctrl Pts',(2.96352566190721,-1.29187129415509,11.0495391320497));
#58826=CARTESIAN_POINT('Ctrl Pts',(2.95536519311266,-1.29845709646629,11.0475038001274));
#58827=CARTESIAN_POINT('Ctrl Pts',(2.9544116176196,-1.29922913626852,11.0472627061011));
#58828=CARTESIAN_POINT('Ctrl Pts',(2.95346386092393,-1.30000000000081,11.047018484776));
#58829=CARTESIAN_POINT('',(3.20083483810839,-0.653834841326313,10.9758649788792));
#58830=CARTESIAN_POINT('Ctrl Pts',(3.20083483808943,-0.653834841310767,
10.9758649789516));
#58831=CARTESIAN_POINT('Ctrl Pts',(3.18968063418913,-0.71148786346381,10.9853204983185));
#58832=CARTESIAN_POINT('Ctrl Pts',(3.17784572765889,-0.767209565144657,
10.9952666810981));
#58833=CARTESIAN_POINT('Ctrl Pts',(3.15307493364191,-0.881644238580126,
11.0158727714609));
#58834=CARTESIAN_POINT('Ctrl Pts',(3.14116546938795,-0.939027188339406,
11.0256944086798));
#58835=CARTESIAN_POINT('Ctrl Pts',(3.1186899032036,-1.03713813150292,11.0440050160884));
#58836=CARTESIAN_POINT('Ctrl Pts',(3.11797981192923,-1.0395835969434,11.0446127766246));
#58837=CARTESIAN_POINT('Ctrl Pts',(3.0945837734477,-1.13871331705522,11.0634417597094));
#58838=CARTESIAN_POINT('Ctrl Pts',(3.08815072335477,-1.16608504285682,11.0685833365413));
#58839=CARTESIAN_POINT('Ctrl Pts',(3.07986858154633,-1.2,11.0751657410237));
#58840=CARTESIAN_POINT('',(3.30596887606183,0.653834841531101,10.8841647344426));
#58841=CARTESIAN_POINT('Ctrl Pts',(3.30596887606185,0.653834841531093,10.8841647344426));
#58842=CARTESIAN_POINT('Ctrl Pts',(3.26763302528942,0.57573341465223,10.8677423429967));
#58843=CARTESIAN_POINT('Ctrl Pts',(3.23499600897867,0.493689278811273,10.8547882313081));
#58844=CARTESIAN_POINT('Ctrl Pts',(3.18713105414667,0.338071090157941,10.8381881285872));
#58845=CARTESIAN_POINT('Ctrl Pts',(3.1698063196683,0.265613244956949,10.833545327178));
#58846=CARTESIAN_POINT('Ctrl Pts',(3.14547080626902,0.129685982985353,10.8314253163346));
#58847=CARTESIAN_POINT('Ctrl Pts',(3.1373686249214,0.0666369657923969,10.8329608190411));
#58848=CARTESIAN_POINT('Ctrl Pts',(3.12711618576932,-0.0594736424808039,
10.8414047274726));
#58849=CARTESIAN_POINT('Ctrl Pts',(3.12488792546582,-0.122671100085152,
10.848354887244));
#58850=CARTESIAN_POINT('Ctrl Pts',(3.12724247067773,-0.26004029845045,10.8688600472412));
#58851=CARTESIAN_POINT('Ctrl Pts',(3.13311315541594,-0.333905072283287,
10.8834214141036));
#58852=CARTESIAN_POINT('Ctrl Pts',(3.15646284017181,-0.491494288206911,
10.9217840503474));
#58853=CARTESIAN_POINT('Ctrl Pts',(3.17560692255383,-0.574905330097381,
10.9471365207566));
#58854=CARTESIAN_POINT('Ctrl Pts',(3.20083483798866,-0.653834841349173,
10.9758649789215));
#58855=CARTESIAN_POINT('',(3.25184183711249,1.2,10.9320268844697));
#58856=CARTESIAN_POINT('Ctrl Pts',(3.25184183711248,1.2,10.9320268844697));
#58857=CARTESIAN_POINT('Ctrl Pts',(3.26095346810344,1.13608448126568,10.924087610778));
#58858=CARTESIAN_POINT('Ctrl Pts',(3.27352444019252,1.03790800343057,10.9130694922008));
#58859=CARTESIAN_POINT('Ctrl Pts',(3.29712370513444,0.796926080875369,10.8921054224812));
#58860=CARTESIAN_POINT('Ctrl Pts',(3.30109675685001,0.741369773818892,10.8885367089974));
#58861=CARTESIAN_POINT('Ctrl Pts',(3.30596887606185,0.653834841531104,10.8841647344426));
#58862=CARTESIAN_POINT('Ctrl Pts',(3.12973060102437,1.3000000000001,10.9050352717634));
#58863=CARTESIAN_POINT('Ctrl Pts',(3.14983364557944,1.28313670183624,10.9101283089392));
#58864=CARTESIAN_POINT('Ctrl Pts',(3.17034835597043,1.26654498650491,10.9144552385832));
#58865=CARTESIAN_POINT('Ctrl Pts',(3.20438384465397,1.23847958744894,10.9222341523255));
#58866=CARTESIAN_POINT('Ctrl Pts',(3.2271445203699,1.21946594797124,10.9277276993067));
#58867=CARTESIAN_POINT('Ctrl Pts',(3.25184183711249,1.2,10.9320268844697));
#58868=CARTESIAN_POINT('Ctrl Pts',(2.70549646903679,-1.3,10.8957209484761));
#58869=CARTESIAN_POINT('Ctrl Pts',(2.6627468523952,-1.18514270861178,10.821391474375));
#58870=CARTESIAN_POINT('Ctrl Pts',(2.62751487735363,-1.06847604194512,10.757426943132));
#58871=CARTESIAN_POINT('Ctrl Pts',(2.56348922287021,-0.794772684000851,
10.6336011714019));
#58872=CARTESIAN_POINT('Ctrl Pts',(2.54183416968341,-0.636309800095197,
10.5831927997129));
#58873=CARTESIAN_POINT('Ctrl Pts',(2.5177651372377,-0.319434907277159,10.5111668553313));
#58874=CARTESIAN_POINT('Ctrl Pts',(2.5171210925739,-0.158333333333332,10.4906809863802));
#58875=CARTESIAN_POINT('Ctrl Pts',(2.53338410693288,0.158333333333334,10.4781996815688));
#58876=CARTESIAN_POINT('Ctrl Pts',(2.54937394678571,0.319434907277167,10.4868805779095));
#58877=CARTESIAN_POINT('Ctrl Pts',(2.60843787791201,0.636309800095206,10.5321053630787));
#58878=CARTESIAN_POINT('Ctrl Pts',(2.64769917658169,0.79477268400084,10.5691036076304));
#58879=CARTESIAN_POINT('Ctrl Pts',(2.74872068765945,1.06847604194511,10.6646142935774));
#58880=CARTESIAN_POINT('Ctrl Pts',(2.80123722412067,1.18514270861178,10.715339060806));
#58881=CARTESIAN_POINT('Ctrl Pts',(2.86254182811346,1.3,10.7754455583364));
#58882=CARTESIAN_POINT('Ctrl Pts',(2.64228988766393,-1.3,10.9395847985784));
#58883=CARTESIAN_POINT('Ctrl Pts',(2.60104997267594,-1.18514270861178,10.8644057917392));
#58884=CARTESIAN_POINT('Ctrl Pts',(2.5668907832622,-1.06847604194512,10.7998891011359));
#58885=CARTESIAN_POINT('Ctrl Pts',(2.50433411476486,-0.794772684000851,
10.6754747228163));
#58886=CARTESIAN_POINT('Ctrl Pts',(2.48221240828625,-0.636309800095197,
10.6256115416015));
#58887=CARTESIAN_POINT('Ctrl Pts',(2.45791319726889,-0.319434907277159,
10.5542114574271));
#58888=CARTESIAN_POINT('Ctrl Pts',(2.4563788705663,-0.158333333333332,10.5345909494989));
#58889=CARTESIAN_POINT('Ctrl Pts',(2.47285287150207,0.158333333333334,10.5224000427974));
#58890=CARTESIAN_POINT('Ctrl Pts',(2.48994083087453,0.319434907277167,10.530501641866));
#58891=CARTESIAN_POINT('Ctrl Pts',(2.54967111951957,0.636309800095206,10.5757009156449));
#58892=CARTESIAN_POINT('Ctrl Pts',(2.58959512893996,0.79477268400084,10.6124238196643));
#58893=CARTESIAN_POINT('Ctrl Pts',(2.68960290025109,1.06847604194511,10.7091497048665));
#58894=CARTESIAN_POINT('Ctrl Pts',(2.7412627929643,1.18514270861178,10.7607241252311));
#58895=CARTESIAN_POINT('Ctrl Pts',(2.80129291984328,1.3,10.8220039143035));
#58896=CARTESIAN_POINT('Ctrl Pts',(2.57908330629106,-1.3,10.9834486486808));
#58897=CARTESIAN_POINT('Ctrl Pts',(2.53935309295667,-1.18514270861178,10.9074201091034));
#58898=CARTESIAN_POINT('Ctrl Pts',(2.50626668917077,-1.06847604194512,10.8423512591397));
#58899=CARTESIAN_POINT('Ctrl Pts',(2.4451790066595,-0.794772684000851,10.7173482742307));
#58900=CARTESIAN_POINT('Ctrl Pts',(2.42259064688909,-0.636309800095197,
10.66803028349));
#58901=CARTESIAN_POINT('Ctrl Pts',(2.39806125730008,-0.319434907277159,
10.5972560595229));
#58902=CARTESIAN_POINT('Ctrl Pts',(2.39563664855869,-0.158333333333332,
10.5785009126177));
#58903=CARTESIAN_POINT('Ctrl Pts',(2.41232163607126,0.158333333333334,10.5666004040259));
#58904=CARTESIAN_POINT('Ctrl Pts',(2.43050771496334,0.319434907277167,10.5741227058226));
#58905=CARTESIAN_POINT('Ctrl Pts',(2.49090436112714,0.636309800095206,10.6192964682111));
#58906=CARTESIAN_POINT('Ctrl Pts',(2.53149108129823,0.79477268400084,10.6557440316982));
#58907=CARTESIAN_POINT('Ctrl Pts',(2.63048511284273,1.06847604194511,10.7536851161556));
#58908=CARTESIAN_POINT('Ctrl Pts',(2.68128836180793,1.18514270861178,10.8061091896562));
#58909=CARTESIAN_POINT('Ctrl Pts',(2.74004401157309,1.3,10.8685622702705));
#58910=CARTESIAN_POINT('Ctrl Pts',(2.5158767249182,-1.3,11.0273124987831));
#58911=CARTESIAN_POINT('Ctrl Pts',(2.47765621323741,-1.18514270861178,10.9504344264676));
#58912=CARTESIAN_POINT('Ctrl Pts',(2.44564259507935,-1.06847604194512,10.8848134171436));
#58913=CARTESIAN_POINT('Ctrl Pts',(2.38602389855415,-0.794772684000851,
10.7592218256451));
#58914=CARTESIAN_POINT('Ctrl Pts',(2.36296888549193,-0.636309800095197,
10.7104490253786));
#58915=CARTESIAN_POINT('Ctrl Pts',(2.33820931733127,-0.319434907277159,
10.6403006616186));
#58916=CARTESIAN_POINT('Ctrl Pts',(2.33489442655109,-0.158333333333332,
10.6224108757364));
#58917=CARTESIAN_POINT('Ctrl Pts',(2.35179040064045,0.158333333333334,10.6108007652544));
#58918=CARTESIAN_POINT('Ctrl Pts',(2.37107459905216,0.319434907277167,10.6177437697791));
#58919=CARTESIAN_POINT('Ctrl Pts',(2.4321376027347,0.636309800095206,10.6628920207773));
#58920=CARTESIAN_POINT('Ctrl Pts',(2.4733870336565,0.79477268400084,10.699064243732));
#58921=CARTESIAN_POINT('Ctrl Pts',(2.57136732543437,1.06847604194511,10.7982205274447));
#58922=CARTESIAN_POINT('Ctrl Pts',(2.62131393065155,1.18514270861178,10.8514942540813));
#58923=CARTESIAN_POINT('Ctrl Pts',(2.67879510330291,1.3,10.9151206262376));
#58924=CARTESIAN_POINT('Ctrl Pts',(2.5158767249182,-1.3,11.0273124987831));
#58925=CARTESIAN_POINT('Ctrl Pts',(2.47765621323741,-1.18514270861178,10.9504344264676));
#58926=CARTESIAN_POINT('Ctrl Pts',(2.44564259507935,-1.06847604194512,10.8848134171436));
#58927=CARTESIAN_POINT('Ctrl Pts',(2.38602389855415,-0.794772684000851,
10.7592218256451));
#58928=CARTESIAN_POINT('Ctrl Pts',(2.36296888549193,-0.636309800095197,
10.7104490253786));
#58929=CARTESIAN_POINT('Ctrl Pts',(2.33820931733128,-0.319434907277159,
10.6403006616186));
#58930=CARTESIAN_POINT('Ctrl Pts',(2.33489442655109,-0.158333333333332,
10.6224108757364));
#58931=CARTESIAN_POINT('Ctrl Pts',(2.35179040064045,0.158333333333334,10.6108007652544));
#58932=CARTESIAN_POINT('Ctrl Pts',(2.37107459905216,0.319434907277167,10.6177437697791));
#58933=CARTESIAN_POINT('Ctrl Pts',(2.4321376027347,0.636309800095206,10.6628920207773));
#58934=CARTESIAN_POINT('Ctrl Pts',(2.4733870336565,0.79477268400084,10.699064243732));
#58935=CARTESIAN_POINT('Ctrl Pts',(2.57136732543437,1.06847604194511,10.7982205274447));
#58936=CARTESIAN_POINT('Ctrl Pts',(2.62131393065155,1.18514270861178,10.8514942540813));
#58937=CARTESIAN_POINT('Ctrl Pts',(2.67879510330291,1.3,10.9151206262376));
#58938=CARTESIAN_POINT('Ctrl Pts',(2.51587672491823,-1.3000000000001,11.0273124987832));
#58939=CARTESIAN_POINT('Ctrl Pts',(2.47765621323743,-1.18514270861185,10.9504344264677));
#58940=CARTESIAN_POINT('Ctrl Pts',(2.44564259507935,-1.06847604194515,10.8848134171436));
#58941=CARTESIAN_POINT('Ctrl Pts',(2.38602389855415,-0.794772684000851,
10.7592218256451));
#58942=CARTESIAN_POINT('Ctrl Pts',(2.36296888549193,-0.636309800095197,
10.7104490253785));
#58943=CARTESIAN_POINT('Ctrl Pts',(2.33820931733127,-0.319434907277159,
10.6403006616186));
#58944=CARTESIAN_POINT('Ctrl Pts',(2.33489442655109,-0.158333333333332,
10.6224108757364));
#58945=CARTESIAN_POINT('Ctrl Pts',(2.35179040064045,0.158333333333334,10.6108007652544));
#58946=CARTESIAN_POINT('Ctrl Pts',(2.37107459905216,0.319434907277167,10.6177437697791));
#58947=CARTESIAN_POINT('Ctrl Pts',(2.4321376027347,0.636309800095206,10.6628920207773));
#58948=CARTESIAN_POINT('Ctrl Pts',(2.4733870336565,0.79477268400084,10.699064243732));
#58949=CARTESIAN_POINT('Ctrl Pts',(2.57136732543439,1.06847604194518,10.7982205274448));
#58950=CARTESIAN_POINT('Ctrl Pts',(2.62131393065161,1.18514270861191,10.8514942540814));
#58951=CARTESIAN_POINT('Ctrl Pts',(2.67879510330301,1.3000000000002,10.9151206262377));
#58952=CARTESIAN_POINT('Ctrl Pts',(2.51547129336052,-1.3000000000001,11.0360548400281));
#58953=CARTESIAN_POINT('Ctrl Pts',(2.47774091682513,-1.18514270861185,10.9586970471128));
#58954=CARTESIAN_POINT('Ctrl Pts',(2.4456831388568,-1.06847604194515,10.8928702980922));
#58955=CARTESIAN_POINT('Ctrl Pts',(2.38472809610279,-0.794772684000851,
10.7674363574331));
#58956=CARTESIAN_POINT('Ctrl Pts',(2.35825829212047,-0.636309800095197,
10.719950323469));
#58957=CARTESIAN_POINT('Ctrl Pts',(2.33182399965475,-0.319434907277159,
10.6503972076724));
#58958=CARTESIAN_POINT('Ctrl Pts',(2.3290441909677,-0.158333333333332,10.6324016146775));
#58959=CARTESIAN_POINT('Ctrl Pts',(2.34617121467972,0.158333333333334,10.6207395120507));
#58960=CARTESIAN_POINT('Ctrl Pts',(2.36541685425652,0.319434907277167,10.6276471138625));
#58961=CARTESIAN_POINT('Ctrl Pts',(2.42808446300845,0.636309800095206,10.6722759426345));
#58962=CARTESIAN_POINT('Ctrl Pts',(2.47174278263681,0.79477268400084,10.707564809271));
#58963=CARTESIAN_POINT('Ctrl Pts',(2.57119727857613,1.06847604194518,10.8064956917392));
#58964=CARTESIAN_POINT('Ctrl Pts',(2.62148033773375,1.18514270861191,10.8598450798671));
#58965=CARTESIAN_POINT('Ctrl Pts',(2.6789962899091,1.3000000000002,10.9237203428529));
#58966=CARTESIAN_POINT('Ctrl Pts',(2.51857146778973,-1.30000000000032,11.0479195112411));
#58967=CARTESIAN_POINT('Ctrl Pts',(2.48325342336936,-1.18514270861205,10.9721660225919));
#58968=CARTESIAN_POINT('Ctrl Pts',(2.45235801114653,-1.06847604194533,10.9077374417252));
#58969=CARTESIAN_POINT('Ctrl Pts',(2.39120059342659,-0.794772684000985,
10.785057333547));
#58970=CARTESIAN_POINT('Ctrl Pts',(2.35943542004083,-0.636309800095307,
10.7391265107922));
#58971=CARTESIAN_POINT('Ctrl Pts',(2.33030727174369,-0.319434907277215,
10.670568975796));
#58972=CARTESIAN_POINT('Ctrl Pts',(2.32728124734563,-0.158333333333359,
10.6516210457096));
#58973=CARTESIAN_POINT('Ctrl Pts',(2.34457235037549,0.158333333333361,10.6399062117895));
#58974=CARTESIAN_POINT('Ctrl Pts',(2.36415032204647,0.31943490727722,10.6478306450851));
#58975=CARTESIAN_POINT('Ctrl Pts',(2.43000480927062,0.636309800095314,10.6911177029276));
#58976=CARTESIAN_POINT('Ctrl Pts',(2.47974272185716,0.794772684000979,10.7240958626731));
#58977=CARTESIAN_POINT('Ctrl Pts',(2.57934531851815,1.06847604194536,10.8203168161419));
#58978=CARTESIAN_POINT('Ctrl Pts',(2.62822954911322,1.18514270861212,10.872477632872));
#58979=CARTESIAN_POINT('Ctrl Pts',(2.68288373684876,1.30000000000043,10.9351487809134));
#58980=CARTESIAN_POINT('Ctrl Pts',(2.5229571659635,-1.30000000000041,11.0653989115702));
#58981=CARTESIAN_POINT('Ctrl Pts',(2.48952415770217,-1.18514270861213,10.9928011317144));
#58982=CARTESIAN_POINT('Ctrl Pts',(2.45983648036719,-1.0684760419454,10.9308015699233));
#58983=CARTESIAN_POINT('Ctrl Pts',(2.39990447041465,-0.794772684001037,
10.8120541831117));
#58984=CARTESIAN_POINT('Ctrl Pts',(2.36657301912039,-0.636309800095346,
10.7664337210332));
#58985=CARTESIAN_POINT('Ctrl Pts',(2.33640023139148,-0.319434907277234,
10.6986777815866));
#58986=CARTESIAN_POINT('Ctrl Pts',(2.3321412631122,-0.15833333333337,10.6789419290149));
#58987=CARTESIAN_POINT('Ctrl Pts',(2.3494892057368,0.158333333333372,10.6671691177473));
#58988=CARTESIAN_POINT('Ctrl Pts',(2.37004660615991,0.319434907277242,10.6759842208015));
#58989=CARTESIAN_POINT('Ctrl Pts',(2.43769368120383,0.636309800095356,10.7180242029322));
#58990=CARTESIAN_POINT('Ctrl Pts',(2.49066133130325,0.794772684001027,10.7497428934053));
#58991=CARTESIAN_POINT('Ctrl Pts',(2.58921334045794,1.06847604194543,10.8419907638107));
#58992=CARTESIAN_POINT('Ctrl Pts',(2.63660706951893,1.18514270861219,10.891924533788));
#58993=CARTESIAN_POINT('Ctrl Pts',(2.68873501458967,1.30000000000051,10.9518613887646));
#58994=CARTESIAN_POINT('Ctrl Pts',(2.52635301603752,-1.30000000000056,11.0799823544973));
#58995=CARTESIAN_POINT('Ctrl Pts',(2.49396067914516,-1.18514270861227,11.0099259838581));
#58996=CARTESIAN_POINT('Ctrl Pts',(2.46515876836807,-1.06847604194553,10.9497039097242));
#58997=CARTESIAN_POINT('Ctrl Pts',(2.40691519525901,-0.794772684001131,
10.833298063362));
#58998=CARTESIAN_POINT('Ctrl Pts',(2.37476208248342,-0.636309800095422,
10.7863545007645));
#58999=CARTESIAN_POINT('Ctrl Pts',(2.34446960788244,-0.319434907277272,
10.7186868616691));
#59000=CARTESIAN_POINT('Ctrl Pts',(2.33822531911909,-0.158333333333389,
10.6989950561829));
#59001=CARTESIAN_POINT('Ctrl Pts',(2.35510922389385,0.158333333333391,10.6874657078855));
#59002=CARTESIAN_POINT('Ctrl Pts',(2.3764579682565,0.31943490727728,10.6968871203843));
#59003=CARTESIAN_POINT('Ctrl Pts',(2.44476635104801,0.636309800095432,10.7385059058195));
#59004=CARTESIAN_POINT('Ctrl Pts',(2.49921534396651,0.794772684001122,10.7700106903359));
#59005=CARTESIAN_POINT('Ctrl Pts',(2.5965131888299,1.06847604194556,10.8597152614524));
#59006=CARTESIAN_POINT('Ctrl Pts',(2.64273478663872,1.18514270861233,10.9080711339211));
#59007=CARTESIAN_POINT('Ctrl Pts',(2.69306135045547,1.30000000000067,10.9659530939042));
#59008=CARTESIAN_POINT('Ctrl Pts',(2.52949729038841,-1.30000000000068,11.0948340954079));
#59009=CARTESIAN_POINT('Ctrl Pts',(2.498246111899,-1.18514270861238,11.027575622754));
#59010=CARTESIAN_POINT('Ctrl Pts',(2.47044007281215,-1.06847604194563,10.9693149858493));
#59011=CARTESIAN_POINT('Ctrl Pts',(2.41416152116015,-0.794772684001209,
10.8555080601903));
#59012=CARTESIAN_POINT('Ctrl Pts',(2.38325128408465,-0.636309800095483,
10.8072772945341));
#59013=CARTESIAN_POINT('Ctrl Pts',(2.35342591954673,-0.319434907277302,
10.739467090569));
#59014=CARTESIAN_POINT('Ctrl Pts',(2.34555635753045,-0.158333333333403,
10.7195360315603));
#59015=CARTESIAN_POINT('Ctrl Pts',(2.36310790745465,0.158333333333405,10.7075878849588));
#59016=CARTESIAN_POINT('Ctrl Pts',(2.38711149284824,0.31943490727731,10.716591055916));
#59017=CARTESIAN_POINT('Ctrl Pts',(2.45557550033893,0.636309800095491,10.7579855523441));
#59018=CARTESIAN_POINT('Ctrl Pts',(2.50844634115406,0.794772684001198,10.7910229501937));
#59019=CARTESIAN_POINT('Ctrl Pts',(2.60342979908886,1.06847604194566,10.878394919682));
#59020=CARTESIAN_POINT('Ctrl Pts',(2.64843089562557,1.18514270861245,10.9249519019435));
#59021=CARTESIAN_POINT('Ctrl Pts',(2.69731826924301,1.30000000000079,10.9802457783254));
#59022=CARTESIAN_POINT('Ctrl Pts',(2.53115568101871,-1.3000000000008,11.1070342157947));
#59023=CARTESIAN_POINT('Ctrl Pts',(2.50071937953504,-1.18514270861249,11.0419082216444));
#59024=CARTESIAN_POINT('Ctrl Pts',(2.47368625233276,-1.06847604194572,10.9851123539511));
#59025=CARTESIAN_POINT('Ctrl Pts',(2.41909633392961,-0.79477268400128,10.8731467961566));
#59026=CARTESIAN_POINT('Ctrl Pts',(2.38929623923248,-0.636309800095539,
10.8238510490312));
#59027=CARTESIAN_POINT('Ctrl Pts',(2.36062812572704,-0.31943490727733,10.7554809547292));
#59028=CARTESIAN_POINT('Ctrl Pts',(2.35278188327807,-0.158333333333417,
10.7346727850495));
#59029=CARTESIAN_POINT('Ctrl Pts',(2.37090460852261,0.158333333333419,10.7223575101951));
#59030=CARTESIAN_POINT('Ctrl Pts',(2.39574478287964,0.319434907277338,10.7316613178487));
#59031=CARTESIAN_POINT('Ctrl Pts',(2.46362685357932,0.636309800095547,10.7732943129577));
#59032=CARTESIAN_POINT('Ctrl Pts',(2.51498647070657,0.794772684001268,10.807725905247));
#59033=CARTESIAN_POINT('Ctrl Pts',(2.60837910365363,1.06847604194575,10.8932897381592));
#59034=CARTESIAN_POINT('Ctrl Pts',(2.65269218043737,1.18514270861255,10.9383714982061));
#59035=CARTESIAN_POINT('Ctrl Pts',(2.70089212374016,1.3000000000009,10.9914976054846));
#59036=CARTESIAN_POINT('Ctrl Pts',(2.53311426036294,-1.30000000000088,11.1191314014661));
#59037=CARTESIAN_POINT('Ctrl Pts',(2.50368560768768,-1.18514270861256,11.0561160669588));
#59038=CARTESIAN_POINT('Ctrl Pts',(2.47752324765872,-1.06847604194579,11.0007904609959));
#59039=CARTESIAN_POINT('Ctrl Pts',(2.42462875166215,-0.794772684001331,
10.8907420546341));
#59040=CARTESIAN_POINT('Ctrl Pts',(2.39556266522996,-0.636309800095579,
10.8405576140811));
#59041=CARTESIAN_POINT('Ctrl Pts',(2.36784559501801,-0.31943490727735,10.7717264801919));
#59042=CARTESIAN_POINT('Ctrl Pts',(2.36022979153471,-0.158333333333428,
10.7498679872182));
#59043=CARTESIAN_POINT('Ctrl Pts',(2.37840647634529,0.15833333333343,10.7375054743309));
#59044=CARTESIAN_POINT('Ctrl Pts',(2.40289325713683,0.319434907277359,10.7478983619531));
#59045=CARTESIAN_POINT('Ctrl Pts',(2.47029455771141,0.636309800095589,10.7897210111506));
#59046=CARTESIAN_POINT('Ctrl Pts',(2.5218467791608,0.794772684001319,10.8245237971547));
#59047=CARTESIAN_POINT('Ctrl Pts',(2.61376060587789,1.06847604194582,10.9081066573638));
#59048=CARTESIAN_POINT('Ctrl Pts',(2.65711797522866,1.18514270861262,10.9518037873114));
#59049=CARTESIAN_POINT('Ctrl Pts',(2.70404662408732,1.30000000000098,11.0030181240723));
#59050=CARTESIAN_POINT('Ctrl Pts',(2.53754735173857,-1.30000000000107,11.1397803649751));
#59051=CARTESIAN_POINT('Ctrl Pts',(2.50931079439629,-1.18514270861273,11.0806753829874));
#59052=CARTESIAN_POINT('Ctrl Pts',(2.48422342692299,-1.06847604194595,11.0281025821637));
#59053=CARTESIAN_POINT('Ctrl Pts',(2.43354184793964,-0.794772684001446,
10.9217395403549));
#59054=CARTESIAN_POINT('Ctrl Pts',(2.40565406829729,-0.636309800095671,
10.8701032747467));
#59055=CARTESIAN_POINT('Ctrl Pts',(2.37936841418338,-0.319434907277396,
10.8006254984324));
#59056=CARTESIAN_POINT('Ctrl Pts',(2.3718237015065,-0.15833333333345,10.7771882625865));
#59057=CARTESIAN_POINT('Ctrl Pts',(2.39085375351299,0.158333333333452,10.7643015226548));
#59058=CARTESIAN_POINT('Ctrl Pts',(2.41672864221899,0.319434907277404,10.7753678578031));
#59059=CARTESIAN_POINT('Ctrl Pts',(2.48320273903407,0.63630980009568,10.8175455453742));
#59060=CARTESIAN_POINT('Ctrl Pts',(2.5324724155591,0.794772684001431,10.8545003349912));
#59061=CARTESIAN_POINT('Ctrl Pts',(2.62157979244895,1.06847604194598,10.9348071271772));
#59062=CARTESIAN_POINT('Ctrl Pts',(2.66363910270278,1.1851427086128,10.9759116346936));
#59063=CARTESIAN_POINT('Ctrl Pts',(2.70918644150855,1.30000000000118,11.023358815049));
#59064=CARTESIAN_POINT('Ctrl Pts',(2.54105191070825,-1.30000000000159,11.1706110977417));
#59065=CARTESIAN_POINT('Ctrl Pts',(2.51417660802196,-1.18514270861321,11.1172681824025));
#59066=CARTESIAN_POINT('Ctrl Pts',(2.49055089600778,-1.06847604194638,11.0686769423299));
#59067=CARTESIAN_POINT('Ctrl Pts',(2.44347797947852,-0.79477268400177,10.9673987775533));
#59068=CARTESIAN_POINT('Ctrl Pts',(2.41870862467442,-0.636309800095931,
10.9130391729152));
#59069=CARTESIAN_POINT('Ctrl Pts',(2.39535351963636,-0.319434907277527,
10.8422287662361));
#59070=CARTESIAN_POINT('Ctrl Pts',(2.38845762174984,-0.158333333333515,
10.8161996107113));
#59071=CARTESIAN_POINT('Ctrl Pts',(2.40788738242878,0.158333333333517,10.8030575116266));
#59072=CARTESIAN_POINT('Ctrl Pts',(2.43309353593705,0.319434907277534,10.8166301418116));
#59073=CARTESIAN_POINT('Ctrl Pts',(2.49830601568335,0.636309800095939,10.8592745745622));
#59074=CARTESIAN_POINT('Ctrl Pts',(2.54726271990942,0.79477268400176,10.8975846532159));
#59075=CARTESIAN_POINT('Ctrl Pts',(2.63319751287982,1.06847604194641,10.9726989423475));
#59076=CARTESIAN_POINT('Ctrl Pts',(2.67337024206067,1.18514270861328,11.0101028369147));
#59077=CARTESIAN_POINT('Ctrl Pts',(2.71651771274338,1.30000000000169,11.0523964335426));
#59078=CARTESIAN_POINT('Ctrl Pts',(2.54573452006115,-1.30000000000214,11.2008309367231));
#59079=CARTESIAN_POINT('Ctrl Pts',(2.52086608529417,-1.18514270861371,11.1529297276386));
#59080=CARTESIAN_POINT('Ctrl Pts',(2.49882047056423,-1.06847604194683,11.1082635887547));
#59081=CARTESIAN_POINT('Ctrl Pts',(2.45441196931678,-0.794772684002102,
11.012549531839));
#59082=CARTESIAN_POINT('Ctrl Pts',(2.42963382118069,-0.636309800096196,
10.9570191287474));
#59083=CARTESIAN_POINT('Ctrl Pts',(2.40791535751862,-0.31943490727766,10.8855638121978));
#59084=CARTESIAN_POINT('Ctrl Pts',(2.40224133814692,-0.158333333333581,
10.8567451642823));
#59085=CARTESIAN_POINT('Ctrl Pts',(2.4227463682387,0.158333333333583,10.8430023574533));
#59086=CARTESIAN_POINT('Ctrl Pts',(2.44848527367546,0.319434907277667,10.8583709235438));
#59087=CARTESIAN_POINT('Ctrl Pts',(2.5128675489143,0.636309800096204,10.9012368723411));
#59088=CARTESIAN_POINT('Ctrl Pts',(2.56049934069731,0.794772684002089,10.9414699237767));
#59089=CARTESIAN_POINT('Ctrl Pts',(2.64370514089814,1.06847604194686,11.0111681329601));
#59090=CARTESIAN_POINT('Ctrl Pts',(2.68243485838104,1.18514270861377,11.0446394012812));
#59091=CARTESIAN_POINT('Ctrl Pts',(2.72387758551865,1.30000000000224,11.0814121657409));
#59092=CARTESIAN_POINT('Ctrl Pts',(2.54836608072529,-1.30000000000248,11.2255071987808));
#59093=CARTESIAN_POINT('Ctrl Pts',(2.52393507525495,-1.18514270861402,11.1824878552591));
#59094=CARTESIAN_POINT('Ctrl Pts',(2.5024945085245,-1.06847604194711,11.1412612342161));
#59095=CARTESIAN_POINT('Ctrl Pts',(2.45987102193083,-0.794772684002315,
11.0501610398079));
#59096=CARTESIAN_POINT('Ctrl Pts',(2.43704879532756,-0.636309800096365,
10.9927988361827));
#59097=CARTESIAN_POINT('Ctrl Pts',(2.41716111947609,-0.319434907277745,
10.9206309940565));
#59098=CARTESIAN_POINT('Ctrl Pts',(2.41189670128007,-0.158333333333623,
10.8898972969641));
#59099=CARTESIAN_POINT('Ctrl Pts',(2.43312364813147,0.158333333333625,10.875776020971));
#59100=CARTESIAN_POINT('Ctrl Pts',(2.45928344885959,0.319434907277752,10.8925936823699));
#59101=CARTESIAN_POINT('Ctrl Pts',(2.52308425970147,0.636309800096373,10.9355794423511));
#59102=CARTESIAN_POINT('Ctrl Pts',(2.56984233349844,0.794772684002302,10.9772056763508));
#59103=CARTESIAN_POINT('Ctrl Pts',(2.65098016815178,1.06847604194714,11.0424969464296));
#59104=CARTESIAN_POINT('Ctrl Pts',(2.68858640056851,1.18514270861408,11.0728076022862));
#59105=CARTESIAN_POINT('Ctrl Pts',(2.72867730323362,1.30000000000258,11.1051667424625));
#59106=CARTESIAN_POINT('Ctrl Pts',(2.54980989363998,-1.30000000000297,11.2393849186444));
#59107=CARTESIAN_POINT('Ctrl Pts',(2.52612452584294,-1.18514270861447,11.198879185939));
#59108=CARTESIAN_POINT('Ctrl Pts',(2.50533570791932,-1.06847604194751,11.1594418349136));
#59109=CARTESIAN_POINT('Ctrl Pts',(2.46400098938739,-0.794772684002612,
11.0708018400401));
#59110=CARTESIAN_POINT('Ctrl Pts',(2.44180654845669,-0.636309800096603,
11.0126237558631));
#59111=CARTESIAN_POINT('Ctrl Pts',(2.42260741951521,-0.319434907277864,
10.9402126409294));
#59112=CARTESIAN_POINT('Ctrl Pts',(2.41731072158857,-0.158333333333682,
10.9085257012698));
#59113=CARTESIAN_POINT('Ctrl Pts',(2.43873104500735,0.158333333333684,10.8942947595499));
#59114=CARTESIAN_POINT('Ctrl Pts',(2.46501515299822,0.319434907277872,10.9119896164857));
#59115=CARTESIAN_POINT('Ctrl Pts',(2.5287277517617,0.636309800096611,10.9549267892209));
#59116=CARTESIAN_POINT('Ctrl Pts',(2.57570949841196,0.794772684002596,10.9969773639694));
#59117=CARTESIAN_POINT('Ctrl Pts',(2.65571139818719,1.06847604194754,11.0597836540679));
#59118=CARTESIAN_POINT('Ctrl Pts',(2.69254102065129,1.18514270861453,11.0883937347858));
#59119=CARTESIAN_POINT('Ctrl Pts',(2.73157040752932,1.30000000000308,11.1184273804406));
#59120=CARTESIAN_POINT('Ctrl Pts',(2.55054244654307,-1.30000000000299,11.2487391367418));
#59121=CARTESIAN_POINT('Ctrl Pts',(2.52732873238259,-1.18514270861449,11.2099260883804));
#59122=CARTESIAN_POINT('Ctrl Pts',(2.50694403362782,-1.06847604194753,11.1717000363166));
#59123=CARTESIAN_POINT('Ctrl Pts',(2.46638689308905,-0.794772684002624,
11.0847462878297));
#59124=CARTESIAN_POINT('Ctrl Pts',(2.44450444954104,-0.636309800096613,
11.0260748419584));
#59125=CARTESIAN_POINT('Ctrl Pts',(2.42574179818932,-0.319434907277869,
10.9535202363304));
#59126=CARTESIAN_POINT('Ctrl Pts',(2.42047967216221,-0.158333333333685,
10.9211814492335));
#59127=CARTESIAN_POINT('Ctrl Pts',(2.44211395856567,0.158333333333686,10.9068395144513));
#59128=CARTESIAN_POINT('Ctrl Pts',(2.46864358766412,0.319434907277877,10.9250337490112));
#59129=CARTESIAN_POINT('Ctrl Pts',(2.53222083393765,0.636309800096621,10.9679728127198));
#59130=CARTESIAN_POINT('Ctrl Pts',(2.57888464825532,0.794772684002608,11.0105378218198));
#59131=CARTESIAN_POINT('Ctrl Pts',(2.65828389481309,1.06847604194756,11.0716024122322));
#59132=CARTESIAN_POINT('Ctrl Pts',(2.69479503048837,1.18514270861455,11.0989748818083));
#59133=CARTESIAN_POINT('Ctrl Pts',(2.73344831003611,1.30000000000309,11.1272872224371));
#59134=CARTESIAN_POINT('Ctrl Pts',(2.55109152476668,-1.30000000000301,11.2549467364805));
#59135=CARTESIAN_POINT('Ctrl Pts',(2.52807171161312,-1.1851427086145,11.2173141635663));
#59136=CARTESIAN_POINT('Ctrl Pts',(2.50787758280969,-1.06847604194754,11.1799299336598));
#59137=CARTESIAN_POINT('Ctrl Pts',(2.46775300157717,-0.794772684002634,
11.0941386059151));
#59138=CARTESIAN_POINT('Ctrl Pts',(2.44615279179159,-0.636309800096621,
11.035109988901));
#59139=CARTESIAN_POINT('Ctrl Pts',(2.42776583447895,-0.319434907277873,
10.9624211245349));
#59140=CARTESIAN_POINT('Ctrl Pts',(2.42267338937598,-0.158333333333687,
10.9295749559879));
#59141=CARTESIAN_POINT('Ctrl Pts',(2.44443627628138,0.158333333333688,10.9151679786746));
#59142=CARTESIAN_POINT('Ctrl Pts',(2.47097314162531,0.319434907277881,10.9337745236639));
#59143=CARTESIAN_POINT('Ctrl Pts',(2.5343382262495,0.636309800096629,10.9767765250291));
#59144=CARTESIAN_POINT('Ctrl Pts',(2.58073260912702,0.794772684002619,11.019711698812));
#59145=CARTESIAN_POINT('Ctrl Pts',(2.65969549076213,1.06847604194757,11.0796337120957));
#59146=CARTESIAN_POINT('Ctrl Pts',(2.69599491986027,1.18514270861457,11.1061818466973));
#59147=CARTESIAN_POINT('Ctrl Pts',(2.73441367245983,1.30000000000311,11.1333400966794));
#59148=CARTESIAN_POINT('Ctrl Pts',(2.55189116477321,-1.30000000000311,11.262654253516));
#59149=CARTESIAN_POINT('Ctrl Pts',(2.52899683365425,-1.1851427086146,11.2265472851811));
#59150=CARTESIAN_POINT('Ctrl Pts',(2.50896306374532,-1.06847604194763,11.1902488904775));
#59151=CARTESIAN_POINT('Ctrl Pts',(2.46928951616223,-0.794772684002696,
11.1059501040369));
#59152=CARTESIAN_POINT('Ctrl Pts',(2.4481159970497,-0.63630980009667,11.04644652644));
#59153=CARTESIAN_POINT('Ctrl Pts',(2.43024865253925,-0.319434907277897,
10.9735674216262));
#59154=CARTESIAN_POINT('Ctrl Pts',(2.4254499088154,-0.158333333333699,10.9400458510263));
#59155=CARTESIAN_POINT('Ctrl Pts',(2.44736033776891,0.158333333333701,10.9255647667845));
#59156=CARTESIAN_POINT('Ctrl Pts',(2.47379113461325,0.319434907277905,10.9447442922543));
#59157=CARTESIAN_POINT('Ctrl Pts',(2.53685547682693,0.636309800096678,10.9878432584808));
#59158=CARTESIAN_POINT('Ctrl Pts',(2.58299396834651,0.794772684002679,11.0312002969059));
#59159=CARTESIAN_POINT('Ctrl Pts',(2.66136955241411,1.06847604194765,11.0897169836481));
#59160=CARTESIAN_POINT('Ctrl Pts',(2.69736482543664,1.18514270861466,11.1152557748196));
#59161=CARTESIAN_POINT('Ctrl Pts',(2.73542948524044,1.30000000000321,11.1410036517289));
#59162=CARTESIAN_POINT('Ctrl Pts',(2.55305163254526,-1.30000000000315,11.2718129170802));
#59163=CARTESIAN_POINT('Ctrl Pts',(2.53025793961708,-1.18514270861464,11.2375568285257));
#59164=CARTESIAN_POINT('Ctrl Pts',(2.51037156929255,-1.06847604194766,11.2025800147505));
#59165=CARTESIAN_POINT('Ctrl Pts',(2.47114657241043,-0.794772684002722,
11.1201115584019));
#59166=CARTESIAN_POINT('Ctrl Pts',(2.45039055789746,-0.636309800096692,
11.0600811018468));
#59167=CARTESIAN_POINT('Ctrl Pts',(2.43317556682532,-0.319434907277908,
10.9869606787218));
#59168=CARTESIAN_POINT('Ctrl Pts',(2.42884313323382,-0.158333333333704,
10.9525799635657));
#59169=CARTESIAN_POINT('Ctrl Pts',(2.45108764636289,0.158333333333706,10.9379354534527));
#59170=CARTESIAN_POINT('Ctrl Pts',(2.47746497352781,0.319434907277916,10.9577646524049));
#59171=CARTESIAN_POINT('Ctrl Pts',(2.54039704684755,0.636309800096699,11.0008658409722));
#59172=CARTESIAN_POINT('Ctrl Pts',(2.58646885103811,0.794772684002707,11.0446111075323));
#59173=CARTESIAN_POINT('Ctrl Pts',(2.66426303314084,1.06847604194769,11.1013745995807));
#59174=CARTESIAN_POINT('Ctrl Pts',(2.69990460744472,1.1851427086147,11.1256927459517));
#59175=CARTESIAN_POINT('Ctrl Pts',(2.73751353717874,1.30000000000325,11.1497582262806));
#59176=CARTESIAN_POINT('Ctrl Pts',(2.55465518880791,-1.30000000000359,11.2904402301687));
#59177=CARTESIAN_POINT('Ctrl Pts',(2.53259793086932,-1.18514270861504,11.2596522944168));
#59178=CARTESIAN_POINT('Ctrl Pts',(2.51339426131821,-1.06847604194802,11.2271485250168));
#59179=CARTESIAN_POINT('Ctrl Pts',(2.47562230300768,-0.794772684002991,
11.1480943963678));
#59180=CARTESIAN_POINT('Ctrl Pts',(2.45581184919151,-0.636309800096907,
11.0869461896583));
#59181=CARTESIAN_POINT('Ctrl Pts',(2.43943340999145,-0.319434907278017,
11.013562248177));
#59182=CARTESIAN_POINT('Ctrl Pts',(2.43507099426907,-0.158333333333758,
10.9779177197142));
#59183=CARTESIAN_POINT('Ctrl Pts',(2.45731084375769,0.15833333333376,10.9632615584176));
#59184=CARTESIAN_POINT('Ctrl Pts',(2.48342526756427,0.319434907278024,10.9844604526388));
#59185=CARTESIAN_POINT('Ctrl Pts',(2.54609837666543,0.636309800096915,11.0275620203848));
#59186=CARTESIAN_POINT('Ctrl Pts',(2.5924380157363,0.794772684002976,11.0718931738382));
#59187=CARTESIAN_POINT('Ctrl Pts',(2.66931583504373,1.06847604194805,11.1250392686005));
#59188=CARTESIAN_POINT('Ctrl Pts',(2.70433250886816,1.1851427086151,11.1468810309115));
#59189=CARTESIAN_POINT('Ctrl Pts',(2.74108829714278,1.3000000000037,11.1675595803679));
#59190=CARTESIAN_POINT('Ctrl Pts',(2.55613434706331,-1.30000000000444,11.3187390268946));
#59191=CARTESIAN_POINT('Ctrl Pts',(2.5344480287897,-1.18514270861581,11.2934483376249));
#59192=CARTESIAN_POINT('Ctrl Pts',(2.51572174253609,-1.06847604194872,11.2648804522911));
#59193=CARTESIAN_POINT('Ctrl Pts',(2.47929854122811,-0.794772684003508,
11.1913119436756));
#59194=CARTESIAN_POINT('Ctrl Pts',(2.46054545403437,-0.636309800097323,
11.1286997802178));
#59195=CARTESIAN_POINT('Ctrl Pts',(2.44617199533978,-0.319434907278226,
11.0546191416089));
#59196=CARTESIAN_POINT('Ctrl Pts',(2.44323962778225,-0.158333333333861,
11.016443183048));
#59197=CARTESIAN_POINT('Ctrl Pts',(2.46696406362689,0.158333333333863,11.0010985155435));
#59198=CARTESIAN_POINT('Ctrl Pts',(2.49395365349794,0.319434907278231,11.0237309533097));
#59199=CARTESIAN_POINT('Ctrl Pts',(2.55597421771634,0.636309800097329,11.0669606588986));
#59200=CARTESIAN_POINT('Ctrl Pts',(2.60024222388047,0.794772684003496,11.1133466204794));
#59201=CARTESIAN_POINT('Ctrl Pts',(2.67532016924119,1.06847604194875,11.1612729977404));
#59202=CARTESIAN_POINT('Ctrl Pts',(2.70962808975909,1.18514270861587,11.1792940119223));
#59203=CARTESIAN_POINT('Ctrl Pts',(2.74574547016027,1.30000000000455,11.194590487417));
#59204=CARTESIAN_POINT('Ctrl Pts',(2.55860850442848,-1.30000000000579,11.3497860913864));
#59205=CARTESIAN_POINT('Ctrl Pts',(2.53751545758815,-1.18514270861704,11.3305075424009));
#59206=CARTESIAN_POINT('Ctrl Pts',(2.51937753972003,-1.06847604194983,11.3062765270361));
#59207=CARTESIAN_POINT('Ctrl Pts',(2.48430226006394,-0.794772684004337,
11.2388568460718));
#59208=CARTESIAN_POINT('Ctrl Pts',(2.46629217650461,-0.636309800097985,
11.174810769052));
#59209=CARTESIAN_POINT('Ctrl Pts',(2.45341294639711,-0.319434907278558,
11.1002998138001));
#59210=CARTESIAN_POINT('Ctrl Pts',(2.4518247445549,-0.158333333334026,11.0594421998351));
#59211=CARTESIAN_POINT('Ctrl Pts',(2.47582090449258,0.158333333334028,11.0439815364231));
#59212=CARTESIAN_POINT('Ctrl Pts',(2.50142593506735,0.319434907278566,11.0693057595259));
#59213=CARTESIAN_POINT('Ctrl Pts',(2.56314151434006,0.636309800097994,11.112472597192));
#59214=CARTESIAN_POINT('Ctrl Pts',(2.60884216623242,0.794772684004321,11.1593650834696));
#59215=CARTESIAN_POINT('Ctrl Pts',(2.68264613957165,1.06847604194986,11.2011751195402));
#59216=CARTESIAN_POINT('Ctrl Pts',(2.71587396605832,1.18514270861711,11.2151093124084));
#59217=CARTESIAN_POINT('Ctrl Pts',(2.75038261367983,1.3000000000059,11.2248796827443));
#59218=CARTESIAN_POINT('Ctrl Pts',(2.55905629130214,-1.30000000000684,11.3752444867707));
#59219=CARTESIAN_POINT('Ctrl Pts',(2.53856232140629,-1.18514270861799,11.360711619204));
#59220=CARTESIAN_POINT('Ctrl Pts',(2.52098885206739,-1.06847604195069,11.3399027700454));
#59221=CARTESIAN_POINT('Ctrl Pts',(2.48713756286471,-0.794772684004976,
11.2773313927096));
#59222=CARTESIAN_POINT('Ctrl Pts',(2.46980256661799,-0.636309800098496,
11.2121016469838));
#59223=CARTESIAN_POINT('Ctrl Pts',(2.45797412929981,-0.319434907278815,
11.137329505581));
#59224=CARTESIAN_POINT('Ctrl Pts',(2.45660151427198,-0.158333333334153,
11.0947466834272));
#59225=CARTESIAN_POINT('Ctrl Pts',(2.48167304904669,0.158333333334155,11.0788160349185));
#59226=CARTESIAN_POINT('Ctrl Pts',(2.50882228821183,0.319434907278822,11.1050728297802));
#59227=CARTESIAN_POINT('Ctrl Pts',(2.57028342039218,0.636309800098504,11.148200745329));
#59228=CARTESIAN_POINT('Ctrl Pts',(2.61397394650306,0.794772684004962,11.1969542390301));
#59229=CARTESIAN_POINT('Ctrl Pts',(2.68644480929014,1.06847604195072,11.2340180199183));
#59230=CARTESIAN_POINT('Ctrl Pts',(2.71921743764465,1.18514270861806,11.2444948363823));
#59231=CARTESIAN_POINT('Ctrl Pts',(2.75339274316326,1.30000000000694,11.2494049319124));
#59232=CARTESIAN_POINT('Ctrl Pts',(2.55994262970328,-1.30000000000743,11.3892732428768));
#59233=CARTESIAN_POINT('Ctrl Pts',(2.53918094648869,-1.18514270861853,11.3776508559804));
#59234=CARTESIAN_POINT('Ctrl Pts',(2.52156741134895,-1.06847604195118,11.3589108084953));
#59235=CARTESIAN_POINT('Ctrl Pts',(2.48814947343831,-0.794772684005335,
11.2991743300279));
#59236=CARTESIAN_POINT('Ctrl Pts',(2.47217241768286,-0.636309800098786,
11.2328962879459));
#59237=CARTESIAN_POINT('Ctrl Pts',(2.46094499315259,-0.319434907278961,
11.1579852824741));
#59238=CARTESIAN_POINT('Ctrl Pts',(2.45936890050809,-0.158333333334225,
11.1145552122263));
#59239=CARTESIAN_POINT('Ctrl Pts',(2.48418278940801,0.158333333334227,11.0987427049723));
#59240=CARTESIAN_POINT('Ctrl Pts',(2.5107119643918,0.319434907278967,11.1262000669487));
#59241=CARTESIAN_POINT('Ctrl Pts',(2.57219996693816,0.636309800098794,11.1692284516201));
#59242=CARTESIAN_POINT('Ctrl Pts',(2.61683048394594,0.794772684005325,11.218088941301));
#59243=CARTESIAN_POINT('Ctrl Pts',(2.68916196690512,1.06847604195121,11.252211993919));
#59244=CARTESIAN_POINT('Ctrl Pts',(2.72165838093492,1.1851427086186,11.2607572364805));
#59245=CARTESIAN_POINT('Ctrl Pts',(2.75534159016708,1.30000000000753,11.2630771165088));
#59246=CARTESIAN_POINT('Ctrl Pts',(2.56043963205252,-1.30000000000761,11.3986684693826));
#59247=CARTESIAN_POINT('Ctrl Pts',(2.53971559392325,-1.18514270861869,11.3889000088412));
#59248=CARTESIAN_POINT('Ctrl Pts',(2.52216612868449,-1.06847604195132,11.3715024840624));
#59249=CARTESIAN_POINT('Ctrl Pts',(2.48895725167271,-0.794772684005442,
11.3136860568827));
#59250=CARTESIAN_POINT('Ctrl Pts',(2.47314153776399,-0.636309800098872,
11.2470051381599));
#59251=CARTESIAN_POINT('Ctrl Pts',(2.46233031765432,-0.319434907279004,
11.171990172431));
#59252=CARTESIAN_POINT('Ctrl Pts',(2.46113595337433,-0.158333333334247,
11.1277883569861));
#59253=CARTESIAN_POINT('Ctrl Pts',(2.48627126153669,0.158333333334249,11.1118421866752));
#59254=CARTESIAN_POINT('Ctrl Pts',(2.51288193508593,0.319434907279011,11.1398722695075));
#59255=CARTESIAN_POINT('Ctrl Pts',(2.57431958909811,0.63630980009888,11.1828654886432));
#59256=CARTESIAN_POINT('Ctrl Pts',(2.61878266938189,0.794772684005431,11.2321557830996));
#59257=CARTESIAN_POINT('Ctrl Pts',(2.6907660779171,1.06847604195135,11.2644332938282));
#59258=CARTESIAN_POINT('Ctrl Pts',(2.72307264878172,1.18514270861876,11.2716932006324));
#59259=CARTESIAN_POINT('Ctrl Pts',(2.75652684020421,1.30000000000771,11.2722412758461));
#59260=CARTESIAN_POINT('Ctrl Pts',(2.56074962849714,-1.30000000000768,11.4049426372132));
#59261=CARTESIAN_POINT('Ctrl Pts',(2.54019409865066,-1.18514270861876,11.396352129411));
#59262=CARTESIAN_POINT('Ctrl Pts',(2.52276515408483,-1.06847604195138,11.3798179070198));
#59263=CARTESIAN_POINT('Ctrl Pts',(2.48972384295886,-0.794772684005487,
11.3232689758011));
#59264=CARTESIAN_POINT('Ctrl Pts',(2.47375221387631,-0.636309800098908,
11.256423467468));
#59265=CARTESIAN_POINT('Ctrl Pts',(2.46313517489945,-0.319434907279023,
11.1813728839924));
#59266=CARTESIAN_POINT('Ctrl Pts',(2.462244652973,-0.158333333334256,11.1366394146029));
#59267=CARTESIAN_POINT('Ctrl Pts',(2.48763458590687,0.158333333334258,11.1205881948526));
#59268=CARTESIAN_POINT('Ctrl Pts',(2.5143615223482,0.319434907279029,11.1489735521833));
#59269=CARTESIAN_POINT('Ctrl Pts',(2.57578657574276,0.636309800098917,11.1919337050089));
#59270=CARTESIAN_POINT('Ctrl Pts',(2.6201004340866,0.794772684005478,11.241524759152));
#59271=CARTESIAN_POINT('Ctrl Pts',(2.69183909251073,1.06847604195141,11.2725770687319));
#59272=CARTESIAN_POINT('Ctrl Pts',(2.72401603463284,1.18514270861883,11.2789816445278));
#59273=CARTESIAN_POINT('Ctrl Pts',(2.75731691182452,1.30000000000778,11.2783494019041));
#59274=CARTESIAN_POINT('Ctrl Pts',(2.56103579688896,-1.30000000000785,11.4160227709829));
#59275=CARTESIAN_POINT('Ctrl Pts',(2.54076331719582,-1.18514270861891,11.4094926909521));
#59276=CARTESIAN_POINT('Ctrl Pts',(2.52354853451578,-1.06847604195152,11.3944645225392));
#59277=CARTESIAN_POINT('Ctrl Pts',(2.4908428345099,-0.79477268400559,11.3401141629314));
#59278=CARTESIAN_POINT('Ctrl Pts',(2.47470146542819,-0.63630980009899,11.2729465823724));
#59279=CARTESIAN_POINT('Ctrl Pts',(2.46446875723411,-0.319434907279063,
11.197819192777));
#59280=CARTESIAN_POINT('Ctrl Pts',(2.46406873556494,-0.158333333334276,
11.1521726753847));
#59281=CARTESIAN_POINT('Ctrl Pts',(2.48992192949735,0.158333333334278,11.135931025976));
#59282=CARTESIAN_POINT('Ctrl Pts',(2.51690809226955,0.31943490727907,11.1649136564021));
#59283=CARTESIAN_POINT('Ctrl Pts',(2.57830893439958,0.636309800098998,11.2078180430919));
#59284=CARTESIAN_POINT('Ctrl Pts',(2.62228210208185,0.794772684005578,11.2579713983951));
#59285=CARTESIAN_POINT('Ctrl Pts',(2.6936023450048,1.06847604195155,11.2868764756407));
#59286=CARTESIAN_POINT('Ctrl Pts',(2.72557456179929,1.18514270861898,11.2917749851617));
#59287=CARTESIAN_POINT('Ctrl Pts',(2.75864710490237,1.30000000000795,11.2890600673027));
#59288=CARTESIAN_POINT('Ctrl Pts',(2.56112206126383,-1.30000000000865,11.4263687093571));
#59289=CARTESIAN_POINT('Ctrl Pts',(2.540699396725,-1.18514270861965,11.4219114957384));
#59290=CARTESIAN_POINT('Ctrl Pts',(2.5234670531941,-1.06847604195218,11.4083652099156));
#59291=CARTESIAN_POINT('Ctrl Pts',(2.49102717206907,-0.794772684006079,
11.3560730046852));
#59292=CARTESIAN_POINT('Ctrl Pts',(2.47555119068125,-0.636309800099382,
11.2882854431247));
#59293=CARTESIAN_POINT('Ctrl Pts',(2.46594535857682,-0.31943490727926,11.21298322481));
#59294=CARTESIAN_POINT('Ctrl Pts',(2.46593945638988,-0.158333333334374,
11.1665098238689));
#59295=CARTESIAN_POINT('Ctrl Pts',(2.4919045200863,0.158333333334376,11.150229554003));
#59296=CARTESIAN_POINT('Ctrl Pts',(2.51854886381738,0.319434907279267,11.1800188124387));
#59297=CARTESIAN_POINT('Ctrl Pts',(2.57967203893382,0.636309800099391,11.2229819527419));
#59298=CARTESIAN_POINT('Ctrl Pts',(2.62345772028888,0.794772684006069,11.2736002846783));
#59299=CARTESIAN_POINT('Ctrl Pts',(2.69463519912823,1.06847604195221,11.3004076861347));
#59300=CARTESIAN_POINT('Ctrl Pts',(2.72657802782751,1.18514270861971,11.3038400737063));
#59301=CARTESIAN_POINT('Ctrl Pts',(2.75965359202203,1.30000000000876,11.299100918071));
#59302=CARTESIAN_POINT('Ctrl Pts',(2.56129546843634,-1.30000000000876,11.4342848832129));
#59303=CARTESIAN_POINT('Ctrl Pts',(2.54091671291285,-1.18514270861975,11.4313604430906));
#59304=CARTESIAN_POINT('Ctrl Pts',(2.52374737348591,-1.06847604195227,11.4189243389879));
#59305=CARTESIAN_POINT('Ctrl Pts',(2.49149715791968,-0.794772684006148,
11.3682206040802));
#59306=CARTESIAN_POINT('Ctrl Pts',(2.4761305193737,-0.636309800099438,11.3001113323577));
#59307=CARTESIAN_POINT('Ctrl Pts',(2.46692567203707,-0.319434907279288,
11.2247053495164));
#59308=CARTESIAN_POINT('Ctrl Pts',(2.46740121156712,-0.158333333334387,
11.1775278104391));
#59309=CARTESIAN_POINT('Ctrl Pts',(2.49354674043552,0.158333333334389,11.161178234315));
#59310=CARTESIAN_POINT('Ctrl Pts',(2.5199846193292,0.319434907279294,11.1915600622205));
#59311=CARTESIAN_POINT('Ctrl Pts',(2.5808818906959,0.636309800099446,11.2345718806749));
#59312=CARTESIAN_POINT('Ctrl Pts',(2.62441089832543,0.794772684006138,11.2855955914427));
#59313=CARTESIAN_POINT('Ctrl Pts',(2.69543525206671,1.0684760419523,11.3108084753575));
#59314=CARTESIAN_POINT('Ctrl Pts',(2.72735024371145,1.18514270861981,11.3131159302143));
#59315=CARTESIAN_POINT('Ctrl Pts',(2.76043641597799,1.30000000000887,11.3068171167106));
#59316=CARTESIAN_POINT('Ctrl Pts',(2.56135170972681,-1.30000000000878,11.4374560436823));
#59317=CARTESIAN_POINT('Ctrl Pts',(2.54098523470469,-1.18514270861976,11.4351463180369));
#59318=CARTESIAN_POINT('Ctrl Pts',(2.52383902071098,-1.06847604195228,11.4231548492346));
#59319=CARTESIAN_POINT('Ctrl Pts',(2.49166728348375,-0.794772684006158,
11.3730853938981));
#59320=CARTESIAN_POINT('Ctrl Pts',(2.47636415999359,-0.636309800099446,
11.304840460273));
#59321=CARTESIAN_POINT('Ctrl Pts',(2.46731911733327,-0.319434907279292,
11.2293936628138));
#59322=CARTESIAN_POINT('Ctrl Pts',(2.46796493347666,-0.158333333334389,
11.1819434771854));
#59323=CARTESIAN_POINT('Ctrl Pts',(2.49418543138234,0.158333333334391,11.1655649762754));
#59324=CARTESIAN_POINT('Ctrl Pts',(2.52056038064123,0.319434907279298,11.1961756769492));
#59325=CARTESIAN_POINT('Ctrl Pts',(2.58138460232752,0.636309800099453,11.239199638653));
#59326=CARTESIAN_POINT('Ctrl Pts',(2.62482644752311,0.794772684006148,11.2903787340127));
#59327=CARTESIAN_POINT('Ctrl Pts',(2.69578560891973,1.06847604195231,11.3149555468183));
#59328=CARTESIAN_POINT('Ctrl Pts',(2.72768216853481,1.18514270861983,11.3168162007128));
#59329=CARTESIAN_POINT('Ctrl Pts',(2.76075969609242,1.30000000000888,11.3098991168989));
#59330=CARTESIAN_POINT('Ctrl Pts',(2.56140557135158,-1.30000000000887,11.4414254376085));
#59331=CARTESIAN_POINT('Ctrl Pts',(2.54104555333389,-1.18514270861985,11.4398867089293));
#59332=CARTESIAN_POINT('Ctrl Pts',(2.52392434518461,-1.06847604195236,11.4284520593091));
#59333=CARTESIAN_POINT('Ctrl Pts',(2.49185322799154,-0.794772684006215,
11.3791741741465));
#59334=CARTESIAN_POINT('Ctrl Pts',(2.47665973194801,-0.636309800099492,
11.3107490308637));
#59335=CARTESIAN_POINT('Ctrl Pts',(2.46781118185094,-0.319434907279315,
11.2352532787707));
#59336=CARTESIAN_POINT('Ctrl Pts',(2.46863056405601,-0.158333333334401,
11.187478369364));
#59337=CARTESIAN_POINT('Ctrl Pts',(2.49495184665048,0.158333333334403,11.1710606307331));
#59338=CARTESIAN_POINT('Ctrl Pts',(2.52128802686867,0.319434907279321,11.2019405645075));
#59339=CARTESIAN_POINT('Ctrl Pts',(2.58205176647432,0.6363098000995,11.2449666625359));
#59340=CARTESIAN_POINT('Ctrl Pts',(2.62540694357562,0.794772684006205,11.2963303662771));
#59341=CARTESIAN_POINT('Ctrl Pts',(2.69627572005436,1.06847604195239,11.3201162448801));
#59342=CARTESIAN_POINT('Ctrl Pts',(2.72813605567496,1.18514270861991,11.3214242688008));
#59343=CARTESIAN_POINT('Ctrl Pts',(2.76118025952548,1.30000000000898,11.3137442911486));
#59344=CARTESIAN_POINT('Ctrl Pts',(2.56141229749596,-1.3000000000089,11.446209086765));
#59345=CARTESIAN_POINT('Ctrl Pts',(2.54101000436551,-1.18514270861988,11.445613246977));
#59346=CARTESIAN_POINT('Ctrl Pts',(2.52389520829441,-1.06847604195239,11.4348550346065));
#59347=CARTESIAN_POINT('Ctrl Pts',(2.49195138143556,-0.794772684006233,
11.3865242982164));
#59348=CARTESIAN_POINT('Ctrl Pts',(2.47702990295093,-0.636309800099506,
11.317831298212));
#59349=CARTESIAN_POINT('Ctrl Pts',(2.46842316379507,-0.319434907279323,
11.242276596958));
#59350=CARTESIAN_POINT('Ctrl Pts',(2.46932820638159,-0.158333333334405,
11.1941611977995));
#59351=CARTESIAN_POINT('Ctrl Pts',(2.49577070833345,0.158333333334406,11.1776961065491));
#59352=CARTESIAN_POINT('Ctrl Pts',(2.52214156267838,0.319434907279329,11.2088659098694));
#59353=CARTESIAN_POINT('Ctrl Pts',(2.58291220881987,0.636309800099515,11.2518611590204));
#59354=CARTESIAN_POINT('Ctrl Pts',(2.62624751185239,0.794772684006224,11.3034099160023));
#59355=CARTESIAN_POINT('Ctrl Pts',(2.6969959403622,1.06847604195242,11.3262520270084));
#59356=CARTESIAN_POINT('Ctrl Pts',(2.72878085125029,1.18514270861994,11.3269107772538));
#59357=CARTESIAN_POINT('Ctrl Pts',(2.76172629981222,1.30000000000901,11.3183407742738));
#59358=CARTESIAN_POINT('Ctrl Pts',(2.56137136298278,-1.30000000000901,11.4510090609822));
#59359=CARTESIAN_POINT('Ctrl Pts',(2.54087625856207,-1.18514270861997,11.4513742353937));
#59360=CARTESIAN_POINT('Ctrl Pts',(2.52374266560532,-1.06847604195247,11.4413014326463));
#59361=CARTESIAN_POINT('Ctrl Pts',(2.49192640226148,-0.794772684006295,
11.393917427895));
#59362=CARTESIAN_POINT('Ctrl Pts',(2.47740478277498,-0.636309800099556,
11.3249090921007));
#59363=CARTESIAN_POINT('Ctrl Pts',(2.46904555195898,-0.319434907279348,
11.2492951852861));
#59364=CARTESIAN_POINT('Ctrl Pts',(2.46993104457879,-0.158333333334417,
11.2008819504006));
#59365=CARTESIAN_POINT('Ctrl Pts',(2.49648908044561,0.158333333334419,11.1843719645541));
#59366=CARTESIAN_POINT('Ctrl Pts',(2.52295468317368,0.319434907279354,11.2158070281581));
#59367=CARTESIAN_POINT('Ctrl Pts',(2.58379531574759,0.636309800099564,11.2587449425823));
#59368=CARTESIAN_POINT('Ctrl Pts',(2.62718132427679,0.794772684006285,11.3104481557108));
#59369=CARTESIAN_POINT('Ctrl Pts',(2.69780711715852,1.0684760419525,11.3323479241051));
#59370=CARTESIAN_POINT('Ctrl Pts',(2.72949516865402,1.18514270862003,11.3323668908108));
#59371=CARTESIAN_POINT('Ctrl Pts',(2.76229998285004,1.30000000000911,11.3229252259507));
#59372=CARTESIAN_POINT('Ctrl Pts',(2.56131666944869,-1.30000000000913,11.4558130511715));
#59373=CARTESIAN_POINT('Ctrl Pts',(2.54071115869131,-1.18514270862008,11.4571454949206));
#59374=CARTESIAN_POINT('Ctrl Pts',(2.52354787125624,-1.06847604195257,11.4477619682194));
#59375=CARTESIAN_POINT('Ctrl Pts',(2.49184946826631,-0.794772684006371,
11.4013281089084));
#59376=CARTESIAN_POINT('Ctrl Pts',(2.4777522540972,-0.636309800099617,11.3319951009902));
#59377=CARTESIAN_POINT('Ctrl Pts',(2.46963844675668,-0.319434907279378,
11.2563237702013));
#59378=CARTESIAN_POINT('Ctrl Pts',(2.47048528287712,-0.158333333334432,
11.2076216623077));
#59379=CARTESIAN_POINT('Ctrl Pts',(2.49715360110744,0.158333333334434,11.1910694940594));
#59380=CARTESIAN_POINT('Ctrl Pts',(2.5237174938095,0.319434907279384,11.222768031268));
#59381=CARTESIAN_POINT('Ctrl Pts',(2.58464050828157,0.636309800099625,11.2656432613921));
#59382=CARTESIAN_POINT('Ctrl Pts',(2.62809396689711,0.794772684006361,11.3174935285109));
#59383=CARTESIAN_POINT('Ctrl Pts',(2.69861118974356,1.0684760419526,11.3384452605758));
#59384=CARTESIAN_POINT('Ctrl Pts',(2.73020709155904,1.18514270862015,11.3378226912375));
#59385=CARTESIAN_POINT('Ctrl Pts',(2.76287460234039,1.30000000000923,11.327508324088));
#59386=CARTESIAN_POINT('Ctrl Pts',(2.56128874706338,-1.30000000000925,11.460606417697));
#59387=CARTESIAN_POINT('Ctrl Pts',(2.54059919774736,-1.18514270862019,11.4628963272545));
#59388=CARTESIAN_POINT('Ctrl Pts',(2.52341514362887,-1.06847604195267,11.4541987306546));
#59389=CARTESIAN_POINT('Ctrl Pts',(2.49181493613513,-0.794772684006444,
11.4087222052943));
#59390=CARTESIAN_POINT('Ctrl Pts',(2.47803662716417,-0.636309800099675,
11.3391034991509));
#59391=CARTESIAN_POINT('Ctrl Pts',(2.47015524119871,-0.319434907279407,
11.2633795288095));
#59392=CARTESIAN_POINT('Ctrl Pts',(2.47104744026839,-0.158333333334447,
11.2143570172613));
#59393=CARTESIAN_POINT('Ctrl Pts',(2.49782482983666,0.158333333334448,11.1977641059529));
#59394=CARTESIAN_POINT('Ctrl Pts',(2.52442978411062,0.319434907279414,11.2297487364126));
#59395=CARTESIAN_POINT('Ctrl Pts',(2.58538867760488,0.636309800099683,11.2725805125511));
#59396=CARTESIAN_POINT('Ctrl Pts',(2.62885836607784,0.794772684006434,11.3245997575365));
#59397=CARTESIAN_POINT('Ctrl Pts',(2.69929693074833,1.0684760419527,11.344590867485));
#59398=CARTESIAN_POINT('Ctrl Pts',(2.7308347615203,1.18514270862026,11.3433123840418));
#59399=CARTESIAN_POINT('Ctrl Pts',(2.76342017842444,1.30000000000935,11.3321020064024));
#59400=CARTESIAN_POINT('Ctrl Pts',(2.56130713243344,-1.30000000000936,11.4641865202654));
#59401=CARTESIAN_POINT('Ctrl Pts',(2.54059650491898,-1.18514270862029,11.467178976126));
#59402=CARTESIAN_POINT('Ctrl Pts',(2.52341374472244,-1.06847604195276,11.4589895513125));
#59403=CARTESIAN_POINT('Ctrl Pts',(2.49186821052087,-0.79477268400651,11.4142379604201));
#59404=CARTESIAN_POINT('Ctrl Pts',(2.4781866708489,-0.636309800099728,11.3444578235712));
#59405=CARTESIAN_POINT('Ctrl Pts',(2.47046333705133,-0.319434907279434,
11.2686998715368));
#59406=CARTESIAN_POINT('Ctrl Pts',(2.47149975376307,-0.15833333333446,11.21939479967));
#59407=CARTESIAN_POINT('Ctrl Pts',(2.49836072670033,0.158333333334462,11.2027714476665));
#59408=CARTESIAN_POINT('Ctrl Pts',(2.52492852326674,0.319434907279441,11.2349976571573));
#59409=CARTESIAN_POINT('Ctrl Pts',(2.58585179782396,0.636309800099737,11.2778228799129));
#59410=CARTESIAN_POINT('Ctrl Pts',(2.6292601226087,0.794772684006501,11.3300004655705));
#59411=CARTESIAN_POINT('Ctrl Pts',(2.69966785275523,1.06847604195279,11.3492592714812));
#59412=CARTESIAN_POINT('Ctrl Pts',(2.73120098151679,1.18514270862035,11.3474724099805));
#59413=CARTESIAN_POINT('Ctrl Pts',(2.76379034152299,1.30000000000946,11.3355622635095));
#59414=CARTESIAN_POINT('Ctrl Pts',(2.56133053553565,-1.30000000000937,11.4663697219108));
#59415=CARTESIAN_POINT('Ctrl Pts',(2.54062092754015,-1.1851427086203,11.4697863261517));
#59416=CARTESIAN_POINT('Ctrl Pts',(2.52344453798962,-1.06847604195277,11.461905362338));
#59417=CARTESIAN_POINT('Ctrl Pts',(2.49192608342873,-0.794772684006519,
11.4175991170701));
#59418=CARTESIAN_POINT('Ctrl Pts',(2.47825706367865,-0.636309800099735,
11.3477377234317));
#59419=CARTESIAN_POINT('Ctrl Pts',(2.47062360734013,-0.319434907279438,
11.2719613563287));
#59420=CARTESIAN_POINT('Ctrl Pts',(2.47178145129884,-0.158333333334462,
11.2224707868178));
#59421=CARTESIAN_POINT('Ctrl Pts',(2.49869442133726,0.158333333334463,11.2058287322166));
#59422=CARTESIAN_POINT('Ctrl Pts',(2.52522064186388,0.319434907279444,11.238210140243));
#59423=CARTESIAN_POINT('Ctrl Pts',(2.58610321650479,0.636309800099743,11.2810393034797));
#59424=CARTESIAN_POINT('Ctrl Pts',(2.62945008104189,0.794772684006509,11.333323903885));
#59425=CARTESIAN_POINT('Ctrl Pts',(2.69984688561952,1.0684760419528,11.352131918274));
#59426=CARTESIAN_POINT('Ctrl Pts',(2.73138883622815,1.18514270862037,11.3500294681154));
#59427=CARTESIAN_POINT('Ctrl Pts',(2.76400056920245,1.30000000000948,11.3376832752746));
#59428=CARTESIAN_POINT('Ctrl Pts',(2.56134006102012,-1.30000000000938,11.467163217126));
#59429=CARTESIAN_POINT('Ctrl Pts',(2.54063196431958,-1.18514270862031,11.4707336261399));
#59430=CARTESIAN_POINT('Ctrl Pts',(2.52345832930351,-1.06847604195277,11.4629646624051));
#59431=CARTESIAN_POINT('Ctrl Pts',(2.49194911040026,-0.794772684006521,
11.418820582519));
#59432=CARTESIAN_POINT('Ctrl Pts',(2.47828069101631,-0.636309800099737,
11.348931118347));
#59433=CARTESIAN_POINT('Ctrl Pts',(2.47067921082616,-0.319434907279439,
11.2731483113593));
#59434=CARTESIAN_POINT('Ctrl Pts',(2.47188381244264,-0.158333333334462,
11.2235892926567));
#59435=CARTESIAN_POINT('Ctrl Pts',(2.49881575706648,0.158333333334464,11.2069404358377));
#59436=CARTESIAN_POINT('Ctrl Pts',(2.52532549432616,0.319434907279445,11.2393788263393));
#59437=CARTESIAN_POINT('Ctrl Pts',(2.586191725793,0.636309800099745,11.2822100750807));
#59438=CARTESIAN_POINT('Ctrl Pts',(2.62951411036498,0.794772684006511,11.3345344993265));
#59439=CARTESIAN_POINT('Ctrl Pts',(2.69990758027193,1.0684760419528,11.3531783372742));
#59440=CARTESIAN_POINT('Ctrl Pts',(2.73145372198533,1.18514270862037,11.3509607217599));
#59441=CARTESIAN_POINT('Ctrl Pts',(2.76407528062454,1.30000000000948,11.3384552641061));
#59442=CARTESIAN_POINT('Ctrl Pts',(2.56135024134104,-1.30000000000938,11.4679564555889));
#59443=CARTESIAN_POINT('Ctrl Pts',(2.54064438626549,-1.18514270862031,11.4716803923896));
#59444=CARTESIAN_POINT('Ctrl Pts',(2.52347378436581,-1.06847604195277,11.4640233214816));
#59445=CARTESIAN_POINT('Ctrl Pts',(2.49197340107165,-0.794772684006522,
11.4200415513229));
#59446=CARTESIAN_POINT('Ctrl Pts',(2.47830304739703,-0.636309800099738,
11.3501249648034));
#59447=CARTESIAN_POINT('Ctrl Pts',(2.47073306099399,-0.319434907279439,
11.2743358940396));
#59448=CARTESIAN_POINT('Ctrl Pts',(2.47198603717078,-0.158333333334462,
11.2247078081228));
#59449=CARTESIAN_POINT('Ctrl Pts',(2.49893699854064,0.158333333334464,11.2080521484978));
#59450=CARTESIAN_POINT('Ctrl Pts',(2.5254294386272,0.319434907279445,11.2405478475419));
#59451=CARTESIAN_POINT('Ctrl Pts',(2.58627834539166,0.636309800099746,11.2833815979748));
#59452=CARTESIAN_POINT('Ctrl Pts',(2.62957484156349,0.794772684006513,11.3357464466506));
#59453=CARTESIAN_POINT('Ctrl Pts',(2.69996537414403,1.0684760419528,11.3542259534225));
#59454=CARTESIAN_POINT('Ctrl Pts',(2.73151633698734,1.18514270862037,11.3518929137309));
#59455=CARTESIAN_POINT('Ctrl Pts',(2.76414880934613,1.30000000000948,11.3392277405993));
#59456=CARTESIAN_POINT('Ctrl Pts',(2.56136125091565,-1.30000000000939,11.46874936247));
#59457=CARTESIAN_POINT('Ctrl Pts',(2.54065855362631,-1.18514270862031,11.4726264753955));
#59458=CARTESIAN_POINT('Ctrl Pts',(2.523491321396,-1.06847604195278,11.4650811647543));
#59459=CARTESIAN_POINT('Ctrl Pts',(2.49199921220471,-0.794772684006527,
11.4212619042518));
#59460=CARTESIAN_POINT('Ctrl Pts',(2.47832365766506,-0.636309800099742,
11.3513194187444));
#59461=CARTESIAN_POINT('Ctrl Pts',(2.47078446722792,-0.319434907279441,
11.275524343034));
#59462=CARTESIAN_POINT('Ctrl Pts',(2.47208778158329,-0.158333333334463,
11.2258264444291));
#59463=CARTESIAN_POINT('Ctrl Pts',(2.49905780903537,0.158333333334465,11.2091639849313));
#59464=CARTESIAN_POINT('Ctrl Pts',(2.52553203339442,0.319434907279447,11.2417173591179));
#59465=CARTESIAN_POINT('Ctrl Pts',(2.58636238554639,0.63630980009975,11.2845541361013));
#59466=CARTESIAN_POINT('Ctrl Pts',(2.62963112657045,0.794772684006517,11.3369602049926));
#59467=CARTESIAN_POINT('Ctrl Pts',(2.70001921062227,1.06847604195281,11.3552751988756));
#59468=CARTESIAN_POINT('Ctrl Pts',(2.73157579789778,1.18514270862038,11.3528264099193));
#59469=CARTESIAN_POINT('Ctrl Pts',(2.76422057899831,1.30000000000949,11.3400009497923));
#59470=CARTESIAN_POINT('Ctrl Pts',(2.56137065250099,-1.30000000000939,11.4693934098164));
#59471=CARTESIAN_POINT('Ctrl Pts',(2.54067104000972,-1.18514270862032,11.4733947758321));
#59472=CARTESIAN_POINT('Ctrl Pts',(2.52350671901196,-1.06847604195278,11.4659402001361));
#59473=CARTESIAN_POINT('Ctrl Pts',(2.49202093437909,-0.794772684006528,
11.4222531218883));
#59474=CARTESIAN_POINT('Ctrl Pts',(2.47833920790945,-0.636309800099742,
11.3522903276923));
#59475=CARTESIAN_POINT('Ctrl Pts',(2.4708244777701,-0.319434907279441,11.2764905873951));
#59476=CARTESIAN_POINT('Ctrl Pts',(2.47216961473139,-0.158333333334463,
11.2267356190202));
#59477=CARTESIAN_POINT('Ctrl Pts',(2.49915516214719,0.158333333334465,11.2100676389615));
#59478=CARTESIAN_POINT('Ctrl Pts',(2.52561430177766,0.319434907279448,11.2426679916367));
#59479=CARTESIAN_POINT('Ctrl Pts',(2.58642895659811,0.636309800099751,11.2855074984505));
#59480=CARTESIAN_POINT('Ctrl Pts',(2.62967401306659,0.794772684006518,11.3379475363054));
#59481=CARTESIAN_POINT('Ctrl Pts',(2.70006034491809,1.06847604195281,11.3561287847828));
#59482=CARTESIAN_POINT('Ctrl Pts',(2.73162193854099,1.18514270862038,11.3535857786671));
#59483=CARTESIAN_POINT('Ctrl Pts',(2.76427749079888,1.30000000000949,11.3406297776516));
#59484=CARTESIAN_POINT('Ctrl Pts',(2.56137504094225,-1.30000000000939,11.4696906405867));
#59485=CARTESIAN_POINT('Ctrl Pts',(2.54067693502122,-1.18514270862032,11.473749321531));
#59486=CARTESIAN_POINT('Ctrl Pts',(2.52351398448711,-1.06847604195278,11.4663366124304));
#59487=CARTESIAN_POINT('Ctrl Pts',(2.49203105146606,-0.794772684006529,
11.4227105656534));
#59488=CARTESIAN_POINT('Ctrl Pts',(2.47834615136286,-0.636309800099743,
11.3527385214951));
#59489=CARTESIAN_POINT('Ctrl Pts',(2.47084263239626,-0.319434907279442,
11.2769366585471));
#59490=CARTESIAN_POINT('Ctrl Pts',(2.47220725302156,-0.158333333334464,
11.2271552820576));
#59491=CARTESIAN_POINT('Ctrl Pts',(2.49919997574841,0.158333333334465,11.2104847522061));
#59492=CARTESIAN_POINT('Ctrl Pts',(2.52565207601259,0.319434907279448,11.2431068189532));
#59493=CARTESIAN_POINT('Ctrl Pts',(2.58645940270579,0.636309800099751,11.2859476223562));
#59494=CARTESIAN_POINT('Ctrl Pts',(2.62969341506726,0.794772684006519,11.3384033860378));
#59495=CARTESIAN_POINT('Ctrl Pts',(2.70007896751934,1.06847604195281,11.3565228972491));
#59496=CARTESIAN_POINT('Ctrl Pts',(2.73164292102903,1.18514270862038,11.3539363877475));
#59497=CARTESIAN_POINT('Ctrl Pts',(2.76430353043367,1.30000000000949,11.3409201037351));
#59498=CARTESIAN_POINT('Ctrl Pts',(2.56137726536325,-1.30000000000939,11.4698392430645));
#59499=CARTESIAN_POINT('Ctrl Pts',(2.54067991505903,-1.18514270862032,11.47392657979));
#59500=CARTESIAN_POINT('Ctrl Pts',(2.52351764709741,-1.06847604195278,11.4665348044257));
#59501=CARTESIAN_POINT('Ctrl Pts',(2.49203612220835,-0.794772684006528,
11.4229392792989));
#59502=CARTESIAN_POINT('Ctrl Pts',(2.47834961582534,-0.636309800099743,
11.3529626174887));
#59503=CARTESIAN_POINT('Ctrl Pts',(2.47085165080681,-0.319434907279441,
11.2771597134595));
#59504=CARTESIAN_POINT('Ctrl Pts',(2.47222594584845,-0.158333333334463,
11.2273651600113));
#59505=CARTESIAN_POINT('Ctrl Pts',(2.49922224671243,0.158333333334465,11.210693359286));
#59506=CARTESIAN_POINT('Ctrl Pts',(2.52567090780485,0.319434907279448,11.2433262507377));
#59507=CARTESIAN_POINT('Ctrl Pts',(2.58647455662111,0.636309800099751,11.2861677092373));
#59508=CARTESIAN_POINT('Ctrl Pts',(2.62970293393306,0.794772684006518,11.3386313825405));
#59509=CARTESIAN_POINT('Ctrl Pts',(2.70008810179692,1.06847604195281,11.3567200251167));
#59510=CARTESIAN_POINT('Ctrl Pts',(2.73165326189538,1.18514270862038,11.3541117541788));
#59511=CARTESIAN_POINT('Ctrl Pts',(2.76431645095154,1.30000000000949,11.341065309182));
#59512=CARTESIAN_POINT('Ctrl Pts',(2.56137945448883,-1.30000000000939,11.4699878598848));
#59513=CARTESIAN_POINT('Ctrl Pts',(2.54068290101624,-1.18514270862032,11.4741038375641));
#59514=CARTESIAN_POINT('Ctrl Pts',(2.52352133537992,-1.06847604195278,11.4667329890265));
#59515=CARTESIAN_POINT('Ctrl Pts',(2.49204121467428,-0.79477268400653,11.423167987879));
#59516=CARTESIAN_POINT('Ctrl Pts',(2.47835295767272,-0.636309800099744,
11.3531867634054));
#59517=CARTESIAN_POINT('Ctrl Pts',(2.47086060422438,-0.319434907279442,
11.2773827955655));
#59518=CARTESIAN_POINT('Ctrl Pts',(2.47224480791073,-0.158333333334464,
11.2275749735584));
#59519=CARTESIAN_POINT('Ctrl Pts',(2.49924471338305,0.158333333334466,11.2109018927394));
#59520=CARTESIAN_POINT('Ctrl Pts',(2.52568973349682,0.319434907279448,11.2435456904092));
#59521=CARTESIAN_POINT('Ctrl Pts',(2.58648968861374,0.636309800099752,11.2863878097201));
#59522=CARTESIAN_POINT('Ctrl Pts',(2.62971259824551,0.79477268400652,11.3388593240486));
#59523=CARTESIAN_POINT('Ctrl Pts',(2.70009738605776,1.06847604195281,11.3569170940394));
#59524=CARTESIAN_POINT('Ctrl Pts',(2.73166372477225,1.18514270862038,11.3542870718402));
#59525=CARTESIAN_POINT('Ctrl Pts',(2.76432943557074,1.30000000000949,11.3412104879192));
#59526=CARTESIAN_POINT('Ctrl Pts',(2.56157722268406,-1.30000000000894,11.4827649103601));
#59527=CARTESIAN_POINT('Ctrl Pts',(2.54094502819204,-1.1851427086199,11.4893453425908));
#59528=CARTESIAN_POINT('Ctrl Pts',(2.52384113867237,-1.06847604195241,11.4837750560872));
#59529=CARTESIAN_POINT('Ctrl Pts',(2.49247882258168,-0.79477268400625,11.4428359889128));
#59530=CARTESIAN_POINT('Ctrl Pts',(2.47865230654726,-0.63630980009952,11.3724576776822));
#59531=CARTESIAN_POINT('Ctrl Pts',(2.47162642797473,-0.31943490727933,11.2965685612173));
#59532=CARTESIAN_POINT('Ctrl Pts',(2.47382416304614,-0.158333333334408,
11.2456348906483));
#59533=CARTESIAN_POINT('Ctrl Pts',(2.50112935392846,0.15833333333441,11.2288534986333));
#59534=CARTESIAN_POINT('Ctrl Pts',(2.52729875131117,0.319434907279336,11.2624201131549));
#59535=CARTESIAN_POINT('Ctrl Pts',(2.58778023915259,0.636309800099529,11.3053196978508));
#59536=CARTESIAN_POINT('Ctrl Pts',(2.63049321521687,0.794772684006241,11.3584818961727));
#59537=CARTESIAN_POINT('Ctrl Pts',(2.70084575128737,1.06847604195244,11.3738850860774));
#59538=CARTESIAN_POINT('Ctrl Pts',(2.73252152503143,1.18514270861997,11.3693815185187));
#59539=CARTESIAN_POINT('Ctrl Pts',(2.76542006647301,1.30000000000904,11.353706913236));
#59540=CARTESIAN_POINT('Ctrl Pts',(2.56100445263162,-1.30000000000382,11.5021321526777));
#59541=CARTESIAN_POINT('Ctrl Pts',(2.53988697929534,-1.18514270861524,11.5125879114081));
#59542=CARTESIAN_POINT('Ctrl Pts',(2.52257778342055,-1.06847604194821,11.5098011038562));
#59543=CARTESIAN_POINT('Ctrl Pts',(2.49138796103636,-0.794772684003123,
11.4727700436339));
#59544=CARTESIAN_POINT('Ctrl Pts',(2.47874734569991,-0.636309800097017,
11.401291801289));
#59545=CARTESIAN_POINT('Ctrl Pts',(2.47260853930848,-0.319434907278073,
11.3252255099555));
#59546=CARTESIAN_POINT('Ctrl Pts',(2.4750472889405,-0.158333333333785,11.2730089588781));
#59547=CARTESIAN_POINT('Ctrl Pts',(2.50290453090846,0.158333333333787,11.2560331856762));
#59548=CARTESIAN_POINT('Ctrl Pts',(2.52919053511972,0.31943490727808,11.2907603607314));
#59549=CARTESIAN_POINT('Ctrl Pts',(2.59030547838485,0.636309800097026,11.3332943963133));
#59550=CARTESIAN_POINT('Ctrl Pts',(2.63427592232645,0.794772684003113,11.386638886161));
#59551=CARTESIAN_POINT('Ctrl Pts',(2.70398322000805,1.06847604194824,11.3983679306146));
#59552=CARTESIAN_POINT('Ctrl Pts',(2.73493078676626,1.18514270861531,11.3914654578382));
#59553=CARTESIAN_POINT('Ctrl Pts',(2.76665221402625,1.30000000000392,11.3725834435454));
#59554=CARTESIAN_POINT('Ctrl Pts',(2.56105038800803,-1.30000000000269,11.5275512529855));
#59555=CARTESIAN_POINT('Ctrl Pts',(2.53937103043282,-1.18514270861421,11.543123480386));
#59556=CARTESIAN_POINT('Ctrl Pts',(2.52180787412611,-1.06847604194728,11.5440280334857));
#59557=CARTESIAN_POINT('Ctrl Pts',(2.49074271793371,-0.794772684002436,
11.5122324702082));
#59558=CARTESIAN_POINT('Ctrl Pts',(2.47924052020287,-0.636309800096463,
11.4394727690071));
#59559=CARTESIAN_POINT('Ctrl Pts',(2.47425825925016,-0.319434907277794,
11.363172367664));
#59560=CARTESIAN_POINT('Ctrl Pts',(2.47759035916085,-0.158333333333648,
11.3090055592548));
#59561=CARTESIAN_POINT('Ctrl Pts',(2.50587326386845,0.158333333333649,11.2918877855756));
#59562=CARTESIAN_POINT('Ctrl Pts',(2.53186766187087,0.319434907277803,11.3283374655647));
#59563=CARTESIAN_POINT('Ctrl Pts',(2.59233443905784,0.636309800096473,11.370991036896));
#59564=CARTESIAN_POINT('Ctrl Pts',(2.63483846985725,0.794772684002421,11.4258929157626));
#59565=CARTESIAN_POINT('Ctrl Pts',(2.70491060050181,1.0684760419473,11.4321819710538));
#59566=CARTESIAN_POINT('Ctrl Pts',(2.73644526408019,1.18514270861427,11.4214123261886));
#59567=CARTESIAN_POINT('Ctrl Pts',(2.76918296230924,1.30000000000279,11.3971507374553));
#59568=CARTESIAN_POINT('Ctrl Pts',(2.56038193620446,-1.3000000000001,11.5405164392947));
#59569=CARTESIAN_POINT('Ctrl Pts',(2.53863428981172,-1.18514270861185,11.5585564843419));
#59570=CARTESIAN_POINT('Ctrl Pts',(2.52104861549718,-1.06847604194515,11.5612588970542));
#59571=CARTESIAN_POINT('Ctrl Pts',(2.49003717792876,-0.794772684000851,
11.5320690120589));
#59572=CARTESIAN_POINT('Ctrl Pts',(2.47864981464921,-0.636309800095197,
11.4588263413895));
#59573=CARTESIAN_POINT('Ctrl Pts',(2.47402470093622,-0.319434907277159,
11.3825030046764));
#59574=CARTESIAN_POINT('Ctrl Pts',(2.47762464049648,-0.158333333333332,
11.3274655474548));
#59575=CARTESIAN_POINT('Ctrl Pts',(2.50647930782813,0.158333333333334,11.3101501710681));
#59576=CARTESIAN_POINT('Ctrl Pts',(2.53302516600472,0.319434907277167,11.3471799051407));
#59577=CARTESIAN_POINT('Ctrl Pts',(2.59379521979637,0.636309800095206,11.3896433274067));
#59578=CARTESIAN_POINT('Ctrl Pts',(2.63621560063971,0.79477268400084,11.4450389031251));
#59579=CARTESIAN_POINT('Ctrl Pts',(2.70595672826436,1.06847604194518,11.4488497372808));
#59580=CARTESIAN_POINT('Ctrl Pts',(2.73726147277651,1.18514270861191,11.436384457426));
#59581=CARTESIAN_POINT('Ctrl Pts',(2.76968261181557,1.3000000000002,11.4098043288156));
#59582=CARTESIAN_POINT('Ctrl Pts',(2.56007871299431,-1.3000000000001,11.5469848467937));
#59583=CARTESIAN_POINT('Ctrl Pts',(2.53830479690493,-1.18514270861185,11.566255317647));
#59584=CARTESIAN_POINT('Ctrl Pts',(2.52071187691434,-1.06847604194515,11.5698548993192));
#59585=CARTESIAN_POINT('Ctrl Pts',(2.48972764967806,-0.794772684000851,
11.5419677641169));
#59586=CARTESIAN_POINT('Ctrl Pts',(2.47833749752908,-0.636309800095197,
11.4685085686384));
#59587=CARTESIAN_POINT('Ctrl Pts',(2.47397094455174,-0.319434907277159,
11.3921419562768));
#59588=CARTESIAN_POINT('Ctrl Pts',(2.47794645705588,-0.158333333333332,
11.3365725980395));
#59589=CARTESIAN_POINT('Ctrl Pts',(2.50702387179274,0.158333333333334,11.31918253943));
#59590=CARTESIAN_POINT('Ctrl Pts',(2.53348691515875,0.319434907277167,11.3566435139838));
#59591=CARTESIAN_POINT('Ctrl Pts',(2.5943095218286,0.636309800095206,11.3990510055383));
#59592=CARTESIAN_POINT('Ctrl Pts',(2.636842707518,0.79477268400084,11.4546353160117));
#59593=CARTESIAN_POINT('Ctrl Pts',(2.70652295950979,1.06847604194518,11.4571620595879));
#59594=CARTESIAN_POINT('Ctrl Pts',(2.73776084593925,1.18514270861191,11.4438270002045));
#59595=CARTESIAN_POINT('Ctrl Pts',(2.77007461961871,1.3000000000002,11.4160631477685));
#59596=CARTESIAN_POINT('',(2.73386551409056,1.2,11.3265578089815));
#59597=CARTESIAN_POINT('Ctrl Pts',(2.73386551409056,1.2,11.3265578089815));
#59598=CARTESIAN_POINT('Ctrl Pts',(2.73584462812093,1.21680977180052,11.3050825247105));
#59599=CARTESIAN_POINT('Ctrl Pts',(2.738942467519,1.23315185137663,11.2833531581086));
#59600=CARTESIAN_POINT('Ctrl Pts',(2.74170316331882,1.2586271482025,11.2507580722637));
#59601=CARTESIAN_POINT('Ctrl Pts',(2.74277442651819,1.2672419954071,11.2396242820028));
#59602=CARTESIAN_POINT('Ctrl Pts',(2.7446650447868,1.28369101331277,11.2184347711517));
#59603=CARTESIAN_POINT('Ctrl Pts',(2.7455088379524,1.29283848095844,11.2067731878531));
#59604=CARTESIAN_POINT('Ctrl Pts',(2.74612652659282,1.3,11.1976604533081));
#59605=CARTESIAN_POINT('',(2.60194863185246,0.653834841400135,11.4109812771984));
#59606=CARTESIAN_POINT('Ctrl Pts',(2.60194863188356,0.653834841395383,11.4109812772131));
#59607=CARTESIAN_POINT('Ctrl Pts',(2.61465202379657,0.712710396428781,11.4031319017273));
#59608=CARTESIAN_POINT('Ctrl Pts',(2.6275775914059,0.767437746451103,11.3950673517918));
#59609=CARTESIAN_POINT('Ctrl Pts',(2.65479253142727,0.881623511218933,11.3778990266176));
#59610=CARTESIAN_POINT('Ctrl Pts',(2.66791954153367,0.939267186110352,11.3695399452405));
#59611=CARTESIAN_POINT('Ctrl Pts',(2.69220097159631,1.03693057340345,11.3538721025205));
#59612=CARTESIAN_POINT('Ctrl Pts',(2.69334780775769,1.04076945910191,11.3531565955888));
#59613=CARTESIAN_POINT('Ctrl Pts',(2.71798212515219,1.13794123504627,11.337051941875));
#59614=CARTESIAN_POINT('Ctrl Pts',(2.72508909283384,1.16622167032162,11.3323722326541));
#59615=CARTESIAN_POINT('Ctrl Pts',(2.73386551409056,1.2,11.3265578089815));
#59616=CARTESIAN_POINT('',(2.48224831221779,-0.653834841531101,11.4826327552677));
#59617=CARTESIAN_POINT('Ctrl Pts',(2.48224831221779,-0.653834841531095,
11.4826327552677));
#59618=CARTESIAN_POINT('Ctrl Pts',(2.47847738061633,-0.575759531786473,
11.4411122856413));
#59619=CARTESIAN_POINT('Ctrl Pts',(2.47624817611948,-0.493700405580143,
11.4060576739905));
#59620=CARTESIAN_POINT('Ctrl Pts',(2.47524680930892,-0.338117536422364,
11.3554159398901));
#59621=CARTESIAN_POINT('Ctrl Pts',(2.47616672898253,-0.265668500424853,
11.3375148853909));
#59622=CARTESIAN_POINT('Ctrl Pts',(2.48166898014515,-0.129739059380434,
11.3137074236253));
#59623=CARTESIAN_POINT('Ctrl Pts',(2.48564176829179,-0.0666644104608011,
11.306467035274));
#59624=CARTESIAN_POINT('Ctrl Pts',(2.49684517723276,0.0595020246954211,
11.2993228621924));
#59625=CARTESIAN_POINT('Ctrl Pts',(2.50413753009899,0.122723937005544,11.2993588371747));
#59626=CARTESIAN_POINT('Ctrl Pts',(2.52290455712779,0.260104219793123,11.3079494537664));
#59627=CARTESIAN_POINT('Ctrl Pts',(2.5349515325394,0.333974009178121,11.3180297306754));
#59628=CARTESIAN_POINT('Ctrl Pts',(2.56422889724993,0.491511647282905,11.3520776397861));
#59629=CARTESIAN_POINT('Ctrl Pts',(2.58242354484658,0.574911057590937,11.3781128894232));
#59630=CARTESIAN_POINT('Ctrl Pts',(2.60194863188389,0.653834841414069,11.4109812771463));
#59631=CARTESIAN_POINT('',(2.54449880327374,-1.2,11.4459422794167));
#59632=CARTESIAN_POINT('Ctrl Pts',(2.54449880327374,-1.2,11.4459422794167));
#59633=CARTESIAN_POINT('Ctrl Pts',(2.53869459902857,-1.16426922222959,11.4494206099695));
#59634=CARTESIAN_POINT('Ctrl Pts',(2.52319531495474,-1.06850390950927,11.4586966913891));
#59635=CARTESIAN_POINT('Ctrl Pts',(2.49047921518896,-0.779246466377113,
11.4778788224293));
#59636=CARTESIAN_POINT('Ctrl Pts',(2.48693835700297,-0.726323271199487,
11.4799143676736));
#59637=CARTESIAN_POINT('Ctrl Pts',(2.48224831221779,-0.653834841531102,
11.4826327552677));
#59638=CARTESIAN_POINT('Ctrl Pts',(2.55649102449442,-1.30000000000134,11.3215110871701));
#59639=CARTESIAN_POINT('Ctrl Pts',(2.55495837329733,-1.28299097848429,11.3424771749858));
#59640=CARTESIAN_POINT('Ctrl Pts',(2.55369848352248,-1.2750263530914,11.3526315204527));
#59641=CARTESIAN_POINT('Ctrl Pts',(2.54995094158512,-1.23879982679597,11.3973438043548));
#59642=CARTESIAN_POINT('Ctrl Pts',(2.54791533845649,-1.21869813962824,11.4220961802047));
#59643=CARTESIAN_POINT('Ctrl Pts',(2.54449880327374,-1.2,11.4459422794167));
#59644=CARTESIAN_POINT('Origin',(0.,1.25,7.2));
#59645=CARTESIAN_POINT('Origin',(0.,1.2,7.2));
#59646=CARTESIAN_POINT('Origin',(0.,0.92691742076555,7.2));
#59647=CARTESIAN_POINT('Origin',(0.,0.653834841531101,7.2));
#59648=CARTESIAN_POINT('Origin',(0.,0.,7.2));
#59649=CARTESIAN_POINT('Origin',(0.,-0.653834841531101,7.2));
#59650=CARTESIAN_POINT('Origin',(0.,-0.926917420765551,7.2));
#59651=CARTESIAN_POINT('Origin',(0.,-1.2,7.2));
#59652=CARTESIAN_POINT('Origin',(0.,-1.25,7.2));
#59653=CARTESIAN_POINT('Ctrl Pts',(2.2661804801183,-1.3000000000017,11.7069865648569));
#59654=CARTESIAN_POINT('Ctrl Pts',(2.30638156847542,-1.18514270861294,11.6928839421778));
#59655=CARTESIAN_POINT('Ctrl Pts',(2.33354901187765,-1.0684760419457,11.6724986686618));
#59656=CARTESIAN_POINT('Ctrl Pts',(2.36620091374758,-0.794772684000851,
11.6108904285065));
#59657=CARTESIAN_POINT('Ctrl Pts',(2.33933008166883,-0.636309800095197,
11.5462634539553));
#59658=CARTESIAN_POINT('Ctrl Pts',(2.33301542000619,-0.319434907277159,
11.4723857856765));
#59659=CARTESIAN_POINT('Ctrl Pts',(2.31380478607559,-0.158333333333332,
11.4307376305842));
#59660=CARTESIAN_POINT('Ctrl Pts',(2.34340372597314,0.158333333333334,11.4142508800506));
#59661=CARTESIAN_POINT('Ctrl Pts',(2.3935159581309,0.319434907277167,11.438592664348));
#59662=CARTESIAN_POINT('Ctrl Pts',(2.45746810794752,0.636309800095206,11.4805575163326));
#59663=CARTESIAN_POINT('Ctrl Pts',(2.51539056129685,0.79477268400084,11.5271512751816));
#59664=CARTESIAN_POINT('Ctrl Pts',(2.524049415203,1.06847604194524,11.5679279706864));
#59665=CARTESIAN_POINT('Ctrl Pts',(2.51213562603731,1.18514270861203,11.5813640954902));
#59666=CARTESIAN_POINT('Ctrl Pts',(2.48455995069209,1.30000000000038,11.5905856245393));
#59667=CARTESIAN_POINT('Ctrl Pts',(2.25573189552087,-1.3000000000017,11.7000487685172));
#59668=CARTESIAN_POINT('Ctrl Pts',(2.29399007944011,-1.18514270861294,11.6845764597768));
#59669=CARTESIAN_POINT('Ctrl Pts',(2.31971787859578,-1.0684760419457,11.6632056051479));
#59670=CARTESIAN_POINT('Ctrl Pts',(2.35020654597517,-0.794772684000851,
11.6002078347277));
#59671=CARTESIAN_POINT('Ctrl Pts',(2.32354980721585,-0.636309800095197,
11.535964978615));
#59672=CARTESIAN_POINT('Ctrl Pts',(2.31708571783412,-0.319434907277159,
11.4621224038657));
#59673=CARTESIAN_POINT('Ctrl Pts',(2.2987048291419,-0.158333333333332,11.4207620498046));
#59674=CARTESIAN_POINT('Ctrl Pts',(2.32795166823,0.158333333333334,11.404586426871));
#59675=CARTESIAN_POINT('Ctrl Pts',(2.37676704786356,0.319434907277167,11.4290468215792));
#59676=CARTESIAN_POINT('Ctrl Pts',(2.44038568131415,0.636309800095206,11.4714162382288));
#59677=CARTESIAN_POINT('Ctrl Pts',(2.49793589154107,0.79477268400084,11.5177886417626));
#59678=CARTESIAN_POINT('Ctrl Pts',(2.50882396394658,1.06847604194524,11.5599152167389));
#59679=CARTESIAN_POINT('Ctrl Pts',(2.49847136268361,1.18514270861203,11.5742359606339));
#59680=CARTESIAN_POINT('Ctrl Pts',(2.47305311705618,1.30000000000038,11.5846424150601));
#59681=CARTESIAN_POINT('Ctrl Pts',(2.23530773828075,-1.30000000000279,11.6858870354544));
#59682=CARTESIAN_POINT('Ctrl Pts',(2.26834048320191,-1.18514270861393,11.6686655879137));
#59683=CARTESIAN_POINT('Ctrl Pts',(2.290425030513,-1.06847604194659,11.6458802525827));
#59684=CARTESIAN_POINT('Ctrl Pts',(2.31615222614137,-0.794772684001515,
11.58038787593));
#59685=CARTESIAN_POINT('Ctrl Pts',(2.29209956838144,-0.636309800095726,
11.5152335524785));
#59686=CARTESIAN_POINT('Ctrl Pts',(2.28591671441847,-0.319434907277423,
11.4410086031402));
#59687=CARTESIAN_POINT('Ctrl Pts',(2.26841145191158,-0.158333333333464,
11.400860557849));
#59688=CARTESIAN_POINT('Ctrl Pts',(2.29717109254721,0.158333333333466,11.3851123134352));
#59689=CARTESIAN_POINT('Ctrl Pts',(2.34426015135361,0.319434907277433,11.4090637091879));
#59690=CARTESIAN_POINT('Ctrl Pts',(2.40734557678233,0.636309800095736,11.4521239875194));
#59691=CARTESIAN_POINT('Ctrl Pts',(2.46336241513653,0.794772684001498,11.4987150878894));
#59692=CARTESIAN_POINT('Ctrl Pts',(2.47873912392656,1.06847604194613,11.543542198105));
#59693=CARTESIAN_POINT('Ctrl Pts',(2.47166857906692,1.18514270861302,11.5595159461311));
#59694=CARTESIAN_POINT('Ctrl Pts',(2.45087148187566,1.30000000000147,11.5720594471789));
#59695=CARTESIAN_POINT('Ctrl Pts',(2.21458925500902,-1.3000000000039,11.6716678043255));
#59696=CARTESIAN_POINT('Ctrl Pts',(2.24450821073624,-1.18514270861494,11.6510794388257));
#59697=CARTESIAN_POINT('Ctrl Pts',(2.26417301394859,-1.06847604194751,11.6259439271504));
#59698=CARTESIAN_POINT('Ctrl Pts',(2.28591349965399,-0.794772684002193,
11.5573710495198));
#59699=CARTESIAN_POINT('Ctrl Pts',(2.26124918157428,-0.636309800096272,
11.4937848894172));
#59700=CARTESIAN_POINT('Ctrl Pts',(2.25440606220613,-0.319434907277698,
11.4199013384659));
#59701=CARTESIAN_POINT('Ctrl Pts',(2.23856260174892,-0.1583333333336,11.380351465671));
#59702=CARTESIAN_POINT('Ctrl Pts',(2.26679504521323,0.158333333333602,11.3650566116884));
#59703=CARTESIAN_POINT('Ctrl Pts',(2.3119341972642,0.319434907277706,11.3886645054107));
#59704=CARTESIAN_POINT('Ctrl Pts',(2.37411901128249,0.636309800096281,11.4327116872793));
#59705=CARTESIAN_POINT('Ctrl Pts',(2.42815247031914,0.794772684002181,11.4798788903475));
#59706=CARTESIAN_POINT('Ctrl Pts',(2.44792960651189,1.06847604194704,11.5275204633));
#59707=CARTESIAN_POINT('Ctrl Pts',(2.44420720743149,1.18514270861403,11.545122958669));
#59708=CARTESIAN_POINT('Ctrl Pts',(2.42820161982799,1.30000000000257,11.5597056777701));
#59709=CARTESIAN_POINT('Ctrl Pts',(2.20422090175705,-1.30000000000403,11.6644270944969));
#59710=CARTESIAN_POINT('Ctrl Pts',(2.23177075940266,-1.18514270861506,11.6427215001599));
#59711=CARTESIAN_POINT('Ctrl Pts',(2.24975521241107,-1.06847604194762,11.6167302669627));
#59712=CARTESIAN_POINT('Ctrl Pts',(2.26920489837338,-0.794772684002276,
11.5467846356428));
#59713=CARTESIAN_POINT('Ctrl Pts',(2.2453879086411,-0.636309800096337,11.4831102051312));
#59714=CARTESIAN_POINT('Ctrl Pts',(2.23874366496151,-0.319434907277732,
11.4089868433271));
#59715=CARTESIAN_POINT('Ctrl Pts',(2.22383100673436,-0.158333333333616,
11.3696723109777));
#59716=CARTESIAN_POINT('Ctrl Pts',(2.25180953322925,0.158333333333618,11.3545940342089));
#59717=CARTESIAN_POINT('Ctrl Pts',(2.29556217988666,0.31943490727774,11.3783403252151));
#59718=CARTESIAN_POINT('Ctrl Pts',(2.3574419315806,0.636309800096347,11.422748345473));
#59719=CARTESIAN_POINT('Ctrl Pts',(2.4112044664916,0.794772684002265,11.4695896170442));
#59720=CARTESIAN_POINT('Ctrl Pts',(2.43321311783985,1.06847604194715,11.5186576826337));
#59721=CARTESIAN_POINT('Ctrl Pts',(2.43103091988541,1.18514270861416,11.5372194632602));
#59722=CARTESIAN_POINT('Ctrl Pts',(2.41713979430878,1.30000000000271,11.5531032770706));
#59723=CARTESIAN_POINT('Ctrl Pts',(2.20398271305387,-1.30000000000403,11.6642592255014));
#59724=CARTESIAN_POINT('Ctrl Pts',(2.23147772863584,-1.18514270861506,11.6425279411832));
#59725=CARTESIAN_POINT('Ctrl Pts',(2.24942324895868,-1.06847604194762,11.6165170527948));
#59726=CARTESIAN_POINT('Ctrl Pts',(2.26881974647487,-0.794772684002275,
11.5465399556231));
#59727=CARTESIAN_POINT('Ctrl Pts',(2.24502184968262,-0.636309800096337,
11.4828638696009));
#59728=CARTESIAN_POINT('Ctrl Pts',(2.23838253278702,-0.319434907277731,
11.4087346991213));
#59729=CARTESIAN_POINT('Ctrl Pts',(2.22349255559444,-0.158333333333616,
11.3694246448445));
#59730=CARTESIAN_POINT('Ctrl Pts',(2.25146532055883,0.158333333333618,11.3543512781286));
#59731=CARTESIAN_POINT('Ctrl Pts',(2.29518505465604,0.319434907277739,11.3781014732845));
#59732=CARTESIAN_POINT('Ctrl Pts',(2.3570572488014,0.636309800096346,11.422518231083));
#59733=CARTESIAN_POINT('Ctrl Pts',(2.41081342436635,0.794772684002264,11.469352080062));
#59734=CARTESIAN_POINT('Ctrl Pts',(2.43287351260473,1.06847604194715,11.5184531279471));
#59735=CARTESIAN_POINT('Ctrl Pts',(2.43072689081419,1.18514270861416,11.5370370274423));
#59736=CARTESIAN_POINT('Ctrl Pts',(2.41688465244154,1.30000000000271,11.5529508021763));
#59737=CARTESIAN_POINT('Ctrl Pts',(2.20374429237847,-1.30000000000403,11.6640915148277));
#59738=CARTESIAN_POINT('Ctrl Pts',(2.23118465586839,-1.18514270861506,11.6423344085549));
#59739=CARTESIAN_POINT('Ctrl Pts',(2.24909137662577,-1.06847604194762,11.6163037719359));
#59740=CARTESIAN_POINT('Ctrl Pts',(2.26843486189156,-0.794772684002275,
11.5462950839186));
#59741=CARTESIAN_POINT('Ctrl Pts',(2.24465608947658,-0.636309800096337,
11.4826173038171));
#59742=CARTESIAN_POINT('Ctrl Pts',(2.23802145507188,-0.319434907277731,
11.4084825157905));
#59743=CARTESIAN_POINT('Ctrl Pts',(2.22315358796243,-0.158333333333616,
11.3691773918339));
#59744=CARTESIAN_POINT('Ctrl Pts',(2.25112054657791,0.158333333333618,11.3541089715631));
#59745=CARTESIAN_POINT('Ctrl Pts',(2.29480790079592,0.31943490727774,11.3778626514247));
#59746=CARTESIAN_POINT('Ctrl Pts',(2.35667267705616,0.636309800096346,11.4222880370731));
#59747=CARTESIAN_POINT('Ctrl Pts',(2.41042225638184,0.794772684002264,11.469114651762));
#59748=CARTESIAN_POINT('Ctrl Pts',(2.43253374250881,1.06847604194715,11.5182487095283));
#59749=CARTESIAN_POINT('Ctrl Pts',(2.43042270360374,1.18514270861416,11.5368547201871));
#59750=CARTESIAN_POINT('Ctrl Pts',(2.41662938276054,1.30000000000271,11.5527984284941));
#59751=CARTESIAN_POINT('Ctrl Pts',(2.20326815095482,-1.30000000000403,11.6637555811632));
#59752=CARTESIAN_POINT('Ctrl Pts',(2.23059929868076,-1.18514270861506,11.6419467453765));
#59753=CARTESIAN_POINT('Ctrl Pts',(2.24842844762722,-1.06847604194762,11.6158765783256));
#59754=CARTESIAN_POINT('Ctrl Pts',(2.26766583035358,-0.794772684002275,
11.5458047494221));
#59755=CARTESIAN_POINT('Ctrl Pts',(2.24392490420093,-0.636309800096337,
11.4821238977744));
#59756=CARTESIAN_POINT('Ctrl Pts',(2.23729963343724,-0.319434907277731,
11.4079778659707));
#59757=CARTESIAN_POINT('Ctrl Pts',(2.22247638038832,-0.158333333333616,
11.3686822890953));
#59758=CARTESIAN_POINT('Ctrl Pts',(2.25043176433982,0.158333333333618,11.3536237233659));
#59759=CARTESIAN_POINT('Ctrl Pts',(2.2940541909032,0.319434907277739,11.3773844944774));
#59760=CARTESIAN_POINT('Ctrl Pts',(2.35590382733677,0.636309800096346,11.4218273788027));
#59761=CARTESIAN_POINT('Ctrl Pts',(2.40963980116502,0.794772684002264,11.4686398671136));
#59762=CARTESIAN_POINT('Ctrl Pts',(2.4318539817315,1.06847604194715,11.5178400351151));
#59763=CARTESIAN_POINT('Ctrl Pts',(2.42981415266791,1.18514270861415,11.5364902367237));
#59764=CARTESIAN_POINT('Ctrl Pts',(2.41611879889003,1.30000000000271,11.5524937102589));
#59765=CARTESIAN_POINT('Ctrl Pts',(2.2022382209217,-1.30000000000403,11.6630264246427));
#59766=CARTESIAN_POINT('Ctrl Pts',(2.22933390480984,-1.18514270861506,11.6411045997646));
#59767=CARTESIAN_POINT('Ctrl Pts',(2.24699565887793,-1.06847604194761,11.6149482520847));
#59768=CARTESIAN_POINT('Ctrl Pts',(2.26600357886143,-0.794772684002273,
11.544739261599));
#59769=CARTESIAN_POINT('Ctrl Pts',(2.24234313065998,-0.636309800096335,
11.4810528947618));
#59770=CARTESIAN_POINT('Ctrl Pts',(2.23573710080049,-0.319434907277731,
11.4068832834797));
#59771=CARTESIAN_POINT('Ctrl Pts',(2.22100969320709,-0.158333333333616,
11.3676090343005));
#59772=CARTESIAN_POINT('Ctrl Pts',(2.24893997869284,0.158333333333618,11.3525718078456));
#59773=CARTESIAN_POINT('Ctrl Pts',(2.29242331970258,0.319434907277739,11.3763466484417));
#59774=CARTESIAN_POINT('Ctrl Pts',(2.35423954466323,0.636309800096345,11.4208279438684));
#59775=CARTESIAN_POINT('Ctrl Pts',(2.40794337957116,0.794772684002263,11.4676120015508));
#59776=CARTESIAN_POINT('Ctrl Pts',(2.43037953301274,1.06847604194715,11.5169558556867));
#59777=CARTESIAN_POINT('Ctrl Pts',(2.4284942213846,1.18514270861415,11.5357016246912));
#59778=CARTESIAN_POINT('Ctrl Pts',(2.41501181864488,1.30000000000271,11.5518340366149));
#59779=CARTESIAN_POINT('Ctrl Pts',(2.20097659874509,-1.30000000000402,11.6621244262188));
#59780=CARTESIAN_POINT('Ctrl Pts',(2.22778734368446,-1.18514270861505,11.640059792093));
#59781=CARTESIAN_POINT('Ctrl Pts',(2.24524586504824,-1.06847604194761,11.6137952097305));
#59782=CARTESIAN_POINT('Ctrl Pts',(2.26397303459823,-0.794772684002269,
11.5434160496375));
#59783=CARTESIAN_POINT('Ctrl Pts',(2.2404050642365,-0.636309800096332,11.4797278359943));
#59784=CARTESIAN_POINT('Ctrl Pts',(2.23381838546602,-0.319434907277729,
11.405532456724));
#59785=CARTESIAN_POINT('Ctrl Pts',(2.21920578066758,-0.158333333333615,
11.3662869368743));
#59786=CARTESIAN_POINT('Ctrl Pts',(2.24710526181061,0.158333333333617,11.3512758015688));
#59787=CARTESIAN_POINT('Ctrl Pts',(2.29042401540504,0.319434907277737,11.3750625946385));
#59788=CARTESIAN_POINT('Ctrl Pts',(2.35219680450747,0.636309800096341,11.4195930837349));
#59789=CARTESIAN_POINT('Ctrl Pts',(2.40585019176021,0.794772684002258,11.4663511106323));
#59790=CARTESIAN_POINT('Ctrl Pts',(2.42855770162894,1.06847604194714,11.5158733572356));
#59791=CARTESIAN_POINT('Ctrl Pts',(2.4268637067064,1.18514270861415,11.5347358290338));
#59792=CARTESIAN_POINT('Ctrl Pts',(2.41364647723532,1.3000000000027,11.5510244270556));
#59793=CARTESIAN_POINT('Ctrl Pts',(2.19972111476395,-1.30000000000402,11.6612176268975));
#59794=CARTESIAN_POINT('Ctrl Pts',(2.22625418374014,-1.18514270861505,11.6390046508609));
#59795=CARTESIAN_POINT('Ctrl Pts',(2.24351370352598,-1.0684760419476,11.6126285984401));
#59796=CARTESIAN_POINT('Ctrl Pts',(2.26196289318945,-0.794772684002267,
11.542077101569));
#59797=CARTESIAN_POINT('Ctrl Pts',(2.23847840133977,-0.63630980009633,11.4783937795508));
#59798=CARTESIAN_POINT('Ctrl Pts',(2.23190425369703,-0.319434907277728,
11.4041778067659));
#59799=CARTESIAN_POINT('Ctrl Pts',(2.2174001040939,-0.158333333333614,11.3649660215187));
#59800=CARTESIAN_POINT('Ctrl Pts',(2.24526898456281,0.158333333333616,11.3499806797437));
#59801=CARTESIAN_POINT('Ctrl Pts',(2.28843442810971,0.319434907277736,11.3737702808472));
#59802=CARTESIAN_POINT('Ctrl Pts',(2.35016138944899,0.63630980009634,11.4183520078683));
#59803=CARTESIAN_POINT('Ctrl Pts',(2.40374838610745,0.794772684002256,11.4650971761613));
#59804=CARTESIAN_POINT('Ctrl Pts',(2.4267250436441,1.06847604194714,11.5147996835543));
#59805=CARTESIAN_POINT('Ctrl Pts',(2.42522425508426,1.18514270861414,11.533777318534));
#59806=CARTESIAN_POINT('Ctrl Pts',(2.41227693428602,1.3000000000027,11.5502182147024));
#59807=CARTESIAN_POINT('Ctrl Pts',(2.19846958455996,-1.30000000000402,11.6603077003021));
#59808=CARTESIAN_POINT('Ctrl Pts',(2.22473048776691,-1.18514270861504,11.6379422093842));
#59809=CARTESIAN_POINT('Ctrl Pts',(2.24179423622381,-1.0684760419476,11.6114522353677));
#59810=CARTESIAN_POINT('Ctrl Pts',(2.2599676413933,-0.794772684002265,11.5407267150302));
#59811=CARTESIAN_POINT('Ctrl Pts',(2.23656002147746,-0.636309800096329,
11.4770532238972));
#59812=CARTESIAN_POINT('Ctrl Pts',(2.22999320980567,-0.319434907277727,
11.402820611383));
#59813=CARTESIAN_POINT('Ctrl Pts',(2.21559242099688,-0.158333333333614,
11.3636465782712));
#59814=CARTESIAN_POINT('Ctrl Pts',(2.24343082185128,0.158333333333616,11.3486868387618));
#59815=CARTESIAN_POINT('Ctrl Pts',(2.28645160784339,0.319434907277736,11.372472245126));
#59816=CARTESIAN_POINT('Ctrl Pts',(2.34813118217902,0.636309800096338,11.41710655782));
#59817=CARTESIAN_POINT('Ctrl Pts',(2.40164008353647,0.794772684002254,11.463848543502));
#59818=CARTESIAN_POINT('Ctrl Pts',(2.42488430650129,1.06847604194714,11.5137326365625));
#59819=CARTESIAN_POINT('Ctrl Pts',(2.42357811786405,1.18514270861414,11.5328242879174));
#59820=CARTESIAN_POINT('Ctrl Pts',(2.41090417775146,1.30000000000269,11.5494146151291));
#59821=CARTESIAN_POINT('Ctrl Pts',(2.196289457676,-1.30000000000401,11.6587073086812));
#59822=CARTESIAN_POINT('Ctrl Pts',(2.22208944260743,-1.18514270861504,11.6360632937767));
#59823=CARTESIAN_POINT('Ctrl Pts',(2.23881963717771,-1.0684760419476,11.6093671057776));
#59824=CARTESIAN_POINT('Ctrl Pts',(2.25651670335936,-0.794772684002261,
11.5383322404626));
#59825=CARTESIAN_POINT('Ctrl Pts',(2.23322556856686,-0.636309800096326,
11.474689429772));
#59826=CARTESIAN_POINT('Ctrl Pts',(2.226657040534,-0.319434907277726,11.400438793734));
#59827=CARTESIAN_POINT('Ctrl Pts',(2.21242235554669,-0.158333333333613,
11.3613424939));
#59828=CARTESIAN_POINT('Ctrl Pts',(2.24020775659807,0.158333333333615,11.3464270281605));
#59829=CARTESIAN_POINT('Ctrl Pts',(2.28299994815951,0.319434907277734,11.3701852165769));
#59830=CARTESIAN_POINT('Ctrl Pts',(2.34459261416236,0.636309800096335,11.4149150216674));
#59831=CARTESIAN_POINT('Ctrl Pts',(2.39793244491085,0.79477268400225,11.4616782436047));
#59832=CARTESIAN_POINT('Ctrl Pts',(2.42164060809001,1.06847604194713,11.5118837130961));
#59833=CARTESIAN_POINT('Ctrl Pts',(2.42067884707763,1.18514270861413,11.53117169741));
#59834=CARTESIAN_POINT('Ctrl Pts',(2.40849293968664,1.30000000000269,11.548015578591));
#59835=CARTESIAN_POINT('Ctrl Pts',(2.19381875820583,-1.30000000000399,11.656861363637));
#59836=CARTESIAN_POINT('Ctrl Pts',(2.21912960775502,-1.18514270861502,11.6338706984122));
#59837=CARTESIAN_POINT('Ctrl Pts',(2.23550094426406,-1.06847604194758,11.60692200114));
#59838=CARTESIAN_POINT('Ctrl Pts',(2.25266994320834,-0.794772684002247,
11.5355212735421));
#59839=CARTESIAN_POINT('Ctrl Pts',(2.22946984941338,-0.636309800096315,
11.4719449319254));
#59840=CARTESIAN_POINT('Ctrl Pts',(2.22286379687592,-0.31943490727772,11.3977008907338));
#59841=CARTESIAN_POINT('Ctrl Pts',(2.20878069664508,-0.158333333333611,
11.3587236376341));
#59842=CARTESIAN_POINT('Ctrl Pts',(2.23650590193875,0.158333333333613,11.3438578368234));
#59843=CARTESIAN_POINT('Ctrl Pts',(2.27909738250193,0.319434907277728,11.3675359022546));
#59844=CARTESIAN_POINT('Ctrl Pts',(2.34058241077827,0.636309800096324,11.4123821553926));
#59845=CARTESIAN_POINT('Ctrl Pts',(2.39365232488814,0.794772684002237,11.459233165597));
#59846=CARTESIAN_POINT('Ctrl Pts',(2.41788040073657,1.06847604194712,11.5098144836929));
#59847=CARTESIAN_POINT('Ctrl Pts',(2.41732125518124,1.18514270861411,11.5293193830973));
#59848=CARTESIAN_POINT('Ctrl Pts',(2.40571552777447,1.30000000000266,11.546434403525));
#59849=CARTESIAN_POINT('Ctrl Pts',(2.19136056145869,-1.30000000000398,11.6550049970701));
#59850=CARTESIAN_POINT('Ctrl Pts',(2.21620612079724,-1.18514270861501,11.6316495906278));
#59851=CARTESIAN_POINT('Ctrl Pts',(2.23223326356462,-1.06847604194757,11.6044372461332));
#59852=CARTESIAN_POINT('Ctrl Pts',(2.24888686317861,-0.794772684002242,
11.5326609880614));
#59853=CARTESIAN_POINT('Ctrl Pts',(2.22575506717335,-0.636309800096311,
11.4691681493286));
#59854=CARTESIAN_POINT('Ctrl Pts',(2.21909151598682,-0.319434907277718,
11.3949460381804));
#59855=CARTESIAN_POINT('Ctrl Pts',(2.20513628823617,-0.15833333333361,11.3561066828364));
#59856=CARTESIAN_POINT('Ctrl Pts',(2.23280061172639,0.158333333333612,11.3412905160417));
#59857=CARTESIAN_POINT('Ctrl Pts',(2.27522625937924,0.319434907277726,11.3648597398984));
#59858=CARTESIAN_POINT('Ctrl Pts',(2.33659808526763,0.63630980009632,11.4098270794775));
#59859=CARTESIAN_POINT('Ctrl Pts',(2.38935396916815,0.794772684002232,11.4568025472316));
#59860=CARTESIAN_POINT('Ctrl Pts',(2.41409391815274,1.06847604194711,11.5077664944603));
#59861=CARTESIAN_POINT('Ctrl Pts',(2.41394125332881,1.18514270861411,11.527485158495));
#59862=CARTESIAN_POINT('Ctrl Pts',(2.40292691647096,1.30000000000265,11.5448620822094));
#59863=CARTESIAN_POINT('Ctrl Pts',(2.18890613509595,-1.30000000000397,11.6531452736484));
#59864=CARTESIAN_POINT('Ctrl Pts',(2.21329486975642,-1.185142708615,11.629418650736));
#59865=CARTESIAN_POINT('Ctrl Pts',(2.22898346622039,-1.06847604194757,11.6019383403953));
#59866=CARTESIAN_POINT('Ctrl Pts',(2.24512820285448,-0.794772684002238,
11.529781557209));
#59867=CARTESIAN_POINT('Ctrl Pts',(2.22206011856169,-0.636309800096307,
11.4663757108842));
#59868=CARTESIAN_POINT('Ctrl Pts',(2.21533413273925,-0.319434907277716,
11.3921793633731));
#59869=CARTESIAN_POINT('Ctrl Pts',(2.20149883179455,-0.158333333333609,
11.3534842563929));
#59870=CARTESIAN_POINT('Ctrl Pts',(2.22910075916764,0.158333333333611,11.3387185888212));
#59871=CARTESIAN_POINT('Ctrl Pts',(2.27136895221501,0.319434907277724,11.3621717074321));
#59872=CARTESIAN_POINT('Ctrl Pts',(2.33262546136905,0.636309800096317,11.4072616844316));
#59873=CARTESIAN_POINT('Ctrl Pts',(2.38505696532997,0.794772684002227,11.4543702890334));
#59874=CARTESIAN_POINT('Ctrl Pts',(2.41030485625289,1.0684760419471,11.5057201840077));
#59875=CARTESIAN_POINT('Ctrl Pts',(2.41055832334208,1.1851427086141,11.5256529414547));
#59876=CARTESIAN_POINT('Ctrl Pts',(2.4001363810665,1.30000000000265,11.5432909895155));
#59877=CARTESIAN_POINT('Ctrl Pts',(2.1858362201203,-1.30000000000395,11.6508213457672));
#59878=CARTESIAN_POINT('Ctrl Pts',(2.20965543231636,-1.18514270861498,11.6266293618945));
#59879=CARTESIAN_POINT('Ctrl Pts',(2.22492307718425,-1.06847604194755,11.5988122794044));
#59880=CARTESIAN_POINT('Ctrl Pts',(2.24043855984763,-0.794772684002225,
11.5261745510593));
#59881=CARTESIAN_POINT('Ctrl Pts',(2.21745805066438,-0.636309800096297,
11.462871622945));
#59882=CARTESIAN_POINT('Ctrl Pts',(2.21066095291805,-0.319434907277711,
11.3887023331593));
#59883=CARTESIAN_POINT('Ctrl Pts',(2.19697882939341,-0.158333333333606,
11.3501853121502));
#59884=CARTESIAN_POINT('Ctrl Pts',(2.22450100165638,0.158333333333608,11.3354837726768));
#59885=CARTESIAN_POINT('Ctrl Pts',(2.26656305125532,0.319434907277719,11.3587981689194));
#59886=CARTESIAN_POINT('Ctrl Pts',(2.3276736494858,0.636309800096306,11.4040421560062));
#59887=CARTESIAN_POINT('Ctrl Pts',(2.3797099125093,0.794772684002214,11.4513087737755));
#59888=CARTESIAN_POINT('Ctrl Pts',(2.40558757945241,1.06847604194709,11.5031454341553));
#59889=CARTESIAN_POINT('Ctrl Pts',(2.40634353421008,1.18514270861408,11.5233501989616));
#59890=CARTESIAN_POINT('Ctrl Pts',(2.39665396056781,1.30000000000263,11.5413215590332));
#59891=CARTESIAN_POINT('Ctrl Pts',(2.18274681931169,-1.30000000000394,11.6485118513956));
#59892=CARTESIAN_POINT('Ctrl Pts',(2.20596545257011,-1.18514270861498,11.6238773181772));
#59893=CARTESIAN_POINT('Ctrl Pts',(2.2207965192823,-1.06847604194754,11.5957348565602));
#59894=CARTESIAN_POINT('Ctrl Pts',(2.2356822936834,-0.79477268400222,11.5226161239857));
#59895=CARTESIAN_POINT('Ctrl Pts',(2.21284515572733,-0.636309800096293,
11.4593748350266));
#59896=CARTESIAN_POINT('Ctrl Pts',(2.20602242295296,-0.319434907277709,
11.3851980449969));
#59897=CARTESIAN_POINT('Ctrl Pts',(2.1925330202892,-0.158333333333605,11.3468283024874));
#59898=CARTESIAN_POINT('Ctrl Pts',(2.21996847361036,0.158333333333607,11.3321960418809));
#59899=CARTESIAN_POINT('Ctrl Pts',(2.2617470425695,0.319434907277717,11.355432011693));
#59900=CARTESIAN_POINT('Ctrl Pts',(2.32271486648178,0.636309800096302,11.4008254844439));
#59901=CARTESIAN_POINT('Ctrl Pts',(2.37444872503291,0.794772684002209,11.4481734012841));
#59902=CARTESIAN_POINT('Ctrl Pts',(2.40095716721983,1.06847604194708,11.5004963520746));
#59903=CARTESIAN_POINT('Ctrl Pts',(2.40219792525709,1.18514270861407,11.5209881575624));
#59904=CARTESIAN_POINT('Ctrl Pts',(2.39320491894349,1.30000000000262,11.5393231018971));
#59905=CARTESIAN_POINT('Ctrl Pts',(2.18025660829921,-1.30000000000394,11.646678211753));
#59906=CARTESIAN_POINT('Ctrl Pts',(2.20296867079828,-1.18514270861497,11.6217090029632));
#59907=CARTESIAN_POINT('Ctrl Pts',(2.21743567570788,-1.06847604194754,11.5933171726611));
#59908=CARTESIAN_POINT('Ctrl Pts',(2.23180961871364,-0.794772684002217,
11.5198194245105));
#59909=CARTESIAN_POINT('Ctrl Pts',(2.20911846574213,-0.63630980009629,11.4566041124908));
#59910=CARTESIAN_POINT('Ctrl Pts',(2.20231019257562,-0.319434907277708,
11.3823947825735));
#59911=CARTESIAN_POINT('Ctrl Pts',(2.18901523160592,-0.158333333333604,
11.3441120092495));
#59912=CARTESIAN_POINT('Ctrl Pts',(2.2163859784749,0.158333333333606,11.3295317990621));
#59913=CARTESIAN_POINT('Ctrl Pts',(2.2578893782394,0.319434907277716,11.3527429855684));
#59914=CARTESIAN_POINT('Ctrl Pts',(2.31874357388177,0.636309800096299,11.3982543759599));
#59915=CARTESIAN_POINT('Ctrl Pts',(2.37028507707526,0.794772684002206,11.4456257258716));
#59916=CARTESIAN_POINT('Ctrl Pts',(2.39730020603818,1.06847604194707,11.4983361946587));
#59917=CARTESIAN_POINT('Ctrl Pts',(2.3989204728418,1.18514270861407,11.5190648878959));
#59918=CARTESIAN_POINT('Ctrl Pts',(2.39046715813017,1.30000000000261,11.5377058655478));
#59919=CARTESIAN_POINT('Ctrl Pts',(2.17775975093903,-1.30000000000393,11.6448494909324));
#59920=CARTESIAN_POINT('Ctrl Pts',(2.1999539175159,-1.18514270861497,11.6195538847476));
#59921=CARTESIAN_POINT('Ctrl Pts',(2.21405164558089,-1.06847604194753,11.5909164716912));
#59922=CARTESIAN_POINT('Ctrl Pts',(2.22791582500244,-0.794772684002214,
11.5170380762368));
#59923=CARTESIAN_POINT('Ctrl Pts',(2.20539661759653,-0.636309800096288,
11.4538297129487));
#59924=CARTESIAN_POINT('Ctrl Pts',(2.19861822688681,-0.319434907277707,
11.3795761410745));
#59925=CARTESIAN_POINT('Ctrl Pts',(2.18552618106875,-0.158333333333604,
11.3413733749366));
#59926=CARTESIAN_POINT('Ctrl Pts',(2.21282429868796,0.158333333333606,11.3268511133002));
#59927=CARTESIAN_POINT('Ctrl Pts',(2.25401998840293,0.319434907277715,11.3500629397051));
#59928=CARTESIAN_POINT('Ctrl Pts',(2.31476188014544,0.636309800096297,11.3956903738005));
#59929=CARTESIAN_POINT('Ctrl Pts',(2.3661513861697,0.794772684002203,11.4430519749583));
#59930=CARTESIAN_POINT('Ctrl Pts',(2.39367608711183,1.06847604194707,11.4961478266809));
#59931=CARTESIAN_POINT('Ctrl Pts',(2.39566977940424,1.18514270861406,11.5171186416964));
#59932=CARTESIAN_POINT('Ctrl Pts',(2.38774274084191,1.30000000000261,11.5360770449118));
#59933=CARTESIAN_POINT('Ctrl Pts',(2.16579089614802,-1.30000000000387,11.6362433191586));
#59934=CARTESIAN_POINT('Ctrl Pts',(2.18540265690836,-1.18514270861491,11.6094888559996));
#59935=CARTESIAN_POINT('Ctrl Pts',(2.19766263552379,-1.06847604194748,11.5797471743966));
#59936=CARTESIAN_POINT('Ctrl Pts',(2.209001551252,-0.794772684002177,11.5041368678941));
#59937=CARTESIAN_POINT('Ctrl Pts',(2.18729931429024,-0.636309800096258,
11.440958509013));
#59938=CARTESIAN_POINT('Ctrl Pts',(2.1808226017509,-0.319434907277691,11.3663741715338));
#59939=CARTESIAN_POINT('Ctrl Pts',(2.16898780467268,-0.158333333333596,
11.3283326797682));
#59940=CARTESIAN_POINT('Ctrl Pts',(2.19607948758469,0.158333333333598,11.3139831473216));
#59941=CARTESIAN_POINT('Ctrl Pts',(2.23573338242787,0.3194349072777,11.3372605965225));
#59942=CARTESIAN_POINT('Ctrl Pts',(2.29591221071323,0.636309800096267,11.3834602968739));
#59943=CARTESIAN_POINT('Ctrl Pts',(2.3465312248773,0.794772684002165,11.4308060021429));
#59944=CARTESIAN_POINT('Ctrl Pts',(2.37647426338148,1.06847604194702,11.4857343454214));
#59945=CARTESIAN_POINT('Ctrl Pts',(2.38025268270869,1.18514270861401,11.5078485077896));
#59946=CARTESIAN_POINT('Ctrl Pts',(2.37484828949358,1.30000000000255,11.5283003880162));
#59947=CARTESIAN_POINT('Ctrl Pts',(2.14717526900777,-1.30000000000332,11.6224242908445));
#59948=CARTESIAN_POINT('Ctrl Pts',(2.16302496616783,-1.18514270861441,11.5931207467066));
#59949=CARTESIAN_POINT('Ctrl Pts',(2.17265618912359,-1.06847604194703,11.5614273824515));
#59950=CARTESIAN_POINT('Ctrl Pts',(2.18054032145746,-0.794772684001842,
11.4826884082334));
#59951=CARTESIAN_POINT('Ctrl Pts',(2.16070647808883,-0.63630980009599,11.4191546062562));
#59952=CARTESIAN_POINT('Ctrl Pts',(2.15432666181657,-0.319434907277558,
11.3443408313766));
#59953=CARTESIAN_POINT('Ctrl Pts',(2.14331228751259,-0.15833333333353,11.3074176251932));
#59954=CARTESIAN_POINT('Ctrl Pts',(2.16930606692612,0.158333333333532,11.2939081140232));
#59955=CARTESIAN_POINT('Ctrl Pts',(2.20631618296266,0.319434907277567,11.3174363365325));
#59956=CARTESIAN_POINT('Ctrl Pts',(2.26563945918351,0.636309800096001,11.364498925613));
#59957=CARTESIAN_POINT('Ctrl Pts',(2.31572832178763,0.794772684001833,11.4112877513487));
#59958=CARTESIAN_POINT('Ctrl Pts',(2.34953065051007,1.06847604194657,11.4690816213842));
#59959=CARTESIAN_POINT('Ctrl Pts',(2.35601714912541,1.18514270861351,11.493090142667));
#59960=CARTESIAN_POINT('Ctrl Pts',(2.35435837075185,1.300000000002,11.5160903603682));
#59961=CARTESIAN_POINT('Ctrl Pts',(2.12785423414619,-1.30000000000305,11.6072652710164));
#59962=CARTESIAN_POINT('Ctrl Pts',(2.14022095354043,-1.18514270861416,11.5748523654447));
#59963=CARTESIAN_POINT('Ctrl Pts',(2.1471949550396,-1.06847604194681,11.5409647164221));
#59964=CARTESIAN_POINT('Ctrl Pts',(2.15084803649971,-0.794772684001673,
11.4592705155861));
#59965=CARTESIAN_POINT('Ctrl Pts',(2.130612959672,-0.636309800095855,11.3970814063584));
#59966=CARTESIAN_POINT('Ctrl Pts',(2.12394752489425,-0.319434907277489,
11.322298665619));
#59967=CARTESIAN_POINT('Ctrl Pts',(2.11485403559682,-0.158333333333496,
11.2858356831044));
#59968=CARTESIAN_POINT('Ctrl Pts',(2.14111401956761,0.158333333333498,11.272141734391));
#59969=CARTESIAN_POINT('Ctrl Pts',(2.177089544414,0.319434907277498,11.2945546004707));
#59970=CARTESIAN_POINT('Ctrl Pts',(2.23597760148315,0.636309800095864,11.3421692416818));
#59971=CARTESIAN_POINT('Ctrl Pts',(2.28393046254491,0.794772684001663,11.3895527718085));
#59972=CARTESIAN_POINT('Ctrl Pts',(2.3216167171952,1.06847604194634,11.4506061376397));
#59973=CARTESIAN_POINT('Ctrl Pts',(2.33109765843318,1.18514270861326,11.4765734373573));
#59974=CARTESIAN_POINT('Ctrl Pts',(2.33374655768437,1.30000000000172,11.5020802969744));
#59975=CARTESIAN_POINT('Ctrl Pts',(2.10820023776197,-1.30000000000293,11.5923398545344));
#59976=CARTESIAN_POINT('Ctrl Pts',(2.11650951602755,-1.18514270861406,11.5572139196954));
#59977=CARTESIAN_POINT('Ctrl Pts',(2.1207230502368,-1.06847604194671,11.5211951992743));
#59978=CARTESIAN_POINT('Ctrl Pts',(2.12099516905386,-0.794772684001603,
11.4359222362857));
#59979=CARTESIAN_POINT('Ctrl Pts',(2.10348361829659,-0.6363098000958,11.3728458265936));
#59980=CARTESIAN_POINT('Ctrl Pts',(2.0970554529222,-0.319434907277462,11.2977193417764));
#59981=CARTESIAN_POINT('Ctrl Pts',(2.08824332842965,-0.158333333333482,
11.2628850822701));
#59982=CARTESIAN_POINT('Ctrl Pts',(2.11335652669121,0.158333333333484,11.2500334513889));
#59983=CARTESIAN_POINT('Ctrl Pts',(2.14718474037035,0.319434907277469,11.2721570984063));
#59984=CARTESIAN_POINT('Ctrl Pts',(2.20496448658686,0.636309800095809,11.3208184921549));
#59985=CARTESIAN_POINT('Ctrl Pts',(2.25147409348881,0.794772684001595,11.3682791264201));
#59986=CARTESIAN_POINT('Ctrl Pts',(2.2928104914806,1.06847604194625,11.432774068759));
#59987=CARTESIAN_POINT('Ctrl Pts',(2.30506520593544,1.18514270861315,11.4608706729831));
#59988=CARTESIAN_POINT('Ctrl Pts',(2.31168163981896,1.30000000000161,11.4891464106659));
#59989=CARTESIAN_POINT('Ctrl Pts',(2.09127259383845,-1.30000000000273,11.5790458884984));
#59990=CARTESIAN_POINT('Ctrl Pts',(2.09686929881197,-1.18514270861387,11.5409596357206));
#59991=CARTESIAN_POINT('Ctrl Pts',(2.09901345333544,-1.06847604194655,11.5028365731315));
#59992=CARTESIAN_POINT('Ctrl Pts',(2.09599079700133,-0.794772684001478,
11.4146796340307));
#59993=CARTESIAN_POINT('Ctrl Pts',(2.07807450668747,-0.636309800095701,
11.3528061731806));
#59994=CARTESIAN_POINT('Ctrl Pts',(2.07160690915555,-0.319434907277413,
11.2775500345261));
#59995=CARTESIAN_POINT('Ctrl Pts',(2.06472793802358,-0.158333333333458,
11.2429443190537));
#59996=CARTESIAN_POINT('Ctrl Pts',(2.09005130262075,0.15833333333346,11.2299402401507));
#59997=CARTESIAN_POINT('Ctrl Pts',(2.12265513190828,0.319434907277418,11.2513067596518));
#59998=CARTESIAN_POINT('Ctrl Pts',(2.17988678631191,0.636309800095708,11.3005534424449));
#59999=CARTESIAN_POINT('Ctrl Pts',(2.22464331497208,0.794772684001471,11.3484204259832));
#60000=CARTESIAN_POINT('Ctrl Pts',(2.26918865414128,1.06847604194609,11.4159190371282));
#60001=CARTESIAN_POINT('Ctrl Pts',(2.28393376959161,1.18514270861297,11.445840624386));
#60002=CARTESIAN_POINT('Ctrl Pts',(2.2941419737334,1.30000000000141,11.4764661512069));
#60003=CARTESIAN_POINT('Ctrl Pts',(2.07532697621282,-1.3000000000026,11.5651096373288));
#60004=CARTESIAN_POINT('Ctrl Pts',(2.07757854621287,-1.18514270861376,11.5244753995875));
#60005=CARTESIAN_POINT('Ctrl Pts',(2.07740481777085,-1.06847604194644,11.4843999320093));
#60006=CARTESIAN_POINT('Ctrl Pts',(2.07140054573513,-0.7947726840014,11.3931084556919));
#60007=CARTESIAN_POINT('Ctrl Pts',(2.05524052391013,-0.636309800095639,
11.3309321974488));
#60008=CARTESIAN_POINT('Ctrl Pts',(2.04907147176573,-0.319434907277382,
11.2553117316264));
#60009=CARTESIAN_POINT('Ctrl Pts',(2.04330560685149,-0.158333333333442,
11.2215124938134));
#60010=CARTESIAN_POINT('Ctrl Pts',(2.06743297899763,0.158333333333444,11.2093599746065));
#60011=CARTESIAN_POINT('Ctrl Pts',(2.09706149851041,0.319434907277387,11.2312251157515));
#60012=CARTESIAN_POINT('Ctrl Pts',(2.15291548107219,0.636309800095646,11.281646863975));
#60013=CARTESIAN_POINT('Ctrl Pts',(2.19674656650228,0.794772684001394,11.3293153036376));
#60014=CARTESIAN_POINT('Ctrl Pts',(2.24466047260869,1.06847604194598,11.3997083221982));
#60015=CARTESIAN_POINT('Ctrl Pts',(2.26192153729684,1.18514270861285,11.4314426906725));
#60016=CARTESIAN_POINT('Ctrl Pts',(2.27570351210487,1.30000000000128,11.4644408982047));
#60017=CARTESIAN_POINT('Ctrl Pts',(2.06703609102509,-1.30000000000259,11.558339409599));
#60018=CARTESIAN_POINT('Ctrl Pts',(2.06772789851115,-1.18514270861374,11.5163550766524));
#60019=CARTESIAN_POINT('Ctrl Pts',(2.06646378438015,-1.06847604194643,11.4752581383681));
#60020=CARTESIAN_POINT('Ctrl Pts',(2.0590248576362,-0.794772684001393,11.3823660487101));
#60021=CARTESIAN_POINT('Ctrl Pts',(2.0436160167612,-0.636309800095632,11.3201326163491));
#60022=CARTESIAN_POINT('Ctrl Pts',(2.03752310066315,-0.319434907277378,
11.244382528723));
#60023=CARTESIAN_POINT('Ctrl Pts',(2.0320493381238,-0.15833333333344,11.2111742109098));
#60024=CARTESIAN_POINT('Ctrl Pts',(2.05600239402219,0.158333333333442,11.199134702077));
#60025=CARTESIAN_POINT('Ctrl Pts',(2.08515449655414,0.319434907277383,11.2205112381063));
#60026=CARTESIAN_POINT('Ctrl Pts',(2.14059763935983,0.636309800095639,11.2713145880716));
#60027=CARTESIAN_POINT('Ctrl Pts',(2.18336041648741,0.794772684001385,11.3193186717382));
#60028=CARTESIAN_POINT('Ctrl Pts',(2.2327241535391,1.06847604194597,11.391334482169));
#60029=CARTESIAN_POINT('Ctrl Pts',(2.2511801808519,1.18514270861284,11.4240258251324));
#60030=CARTESIAN_POINT('Ctrl Pts',(2.26672450281456,1.30000000000127,11.4582355351724));
#60031=CARTESIAN_POINT('Ctrl Pts',(2.06279202116117,-1.30000000000259,11.5550170835906));
#60032=CARTESIAN_POINT('Ctrl Pts',(2.06275384366667,-1.18514270861374,11.5123250243607));
#60033=CARTESIAN_POINT('Ctrl Pts',(2.0609667907251,-1.06847604194643,11.4707029801893));
#60034=CARTESIAN_POINT('Ctrl Pts',(2.05279808878728,-0.79477268400139,11.3770196805328));
#60035=CARTESIAN_POINT('Ctrl Pts',(2.0375888362941,-0.63630980009563,11.3148756573714));
#60036=CARTESIAN_POINT('Ctrl Pts',(2.0315723503544,-0.319434907277377,11.2390344487862));
#60037=CARTESIAN_POINT('Ctrl Pts',(2.02645821684465,-0.15833333333344,11.2059761441961));
#60038=CARTESIAN_POINT('Ctrl Pts',(2.0503854531006,0.158333333333442,11.1939534624214));
#60039=CARTESIAN_POINT('Ctrl Pts',(2.07918299434904,0.319434907277382,11.215170594379));
#60040=CARTESIAN_POINT('Ctrl Pts',(2.13443419885736,0.636309800095637,11.2661527447975));
#60041=CARTESIAN_POINT('Ctrl Pts',(2.17683124436735,0.794772684001383,11.314194270533));
#60042=CARTESIAN_POINT('Ctrl Pts',(2.22683467051598,1.06847604194597,11.3870841418656));
#60043=CARTESIAN_POINT('Ctrl Pts',(2.24579847958093,1.18514270861284,11.4203214029125));
#60044=CARTESIAN_POINT('Ctrl Pts',(2.26208146734064,1.30000000000126,11.4552446005424));
#60045=CARTESIAN_POINT('Ctrl Pts',(2.06041334439403,-1.30000000000258,11.5530881430361));
#60046=CARTESIAN_POINT('Ctrl Pts',(2.05994859131143,-1.18514270861374,11.5099973689643));
#60047=CARTESIAN_POINT('Ctrl Pts',(2.05785557660839,-1.06847604194643,11.4680796159551));
#60048=CARTESIAN_POINT('Ctrl Pts',(2.04925868386235,-0.79477268400139,11.3739511342031));
#60049=CARTESIAN_POINT('Ctrl Pts',(2.03416509416363,-0.63630980009563,11.3118575049429));
#60050=CARTESIAN_POINT('Ctrl Pts',(2.02818749776246,-0.319434907277377,
11.2359674132999));
#60051=CARTESIAN_POINT('Ctrl Pts',(2.02327194124969,-0.15833333333344,11.2029996999416));
#60052=CARTESIAN_POINT('Ctrl Pts',(2.04718860755012,0.158333333333442,11.1909831628903));
#60053=CARTESIAN_POINT('Ctrl Pts',(2.07580107504722,0.319434907277382,11.2120960888184));
#60054=CARTESIAN_POINT('Ctrl Pts',(2.13094282440124,0.636309800095637,11.2631798873757));
#60055=CARTESIAN_POINT('Ctrl Pts',(2.17310855833032,0.794772684001382,11.3112589742065));
#60056=CARTESIAN_POINT('Ctrl Pts',(2.22348049294071,1.06847604194597,11.3846460506045));
#60057=CARTESIAN_POINT('Ctrl Pts',(2.2427407163222,1.18514270861284,11.4181907026243));
#60058=CARTESIAN_POINT('Ctrl Pts',(2.25945701905647,1.30000000000126,11.4535134605503));
#60059=CARTESIAN_POINT('Ctrl Pts',(2.05008175662492,-1.30000000000257,11.5441639496957));
#60060=CARTESIAN_POINT('Ctrl Pts',(2.04771030887034,-1.18514270861372,11.4992670371596));
#60061=CARTESIAN_POINT('Ctrl Pts',(2.04423529821295,-1.06847604194641,11.4560198397657));
#60062=CARTESIAN_POINT('Ctrl Pts',(2.03365787734839,-0.794772684001376,
11.3599213342163));
#60063=CARTESIAN_POINT('Ctrl Pts',(2.01895341088084,-0.63630980009562,11.2981450873994));
#60064=CARTESIAN_POINT('Ctrl Pts',(2.01310653757849,-0.319434907277372,
11.222064419379));
#60065=CARTESIAN_POINT('Ctrl Pts',(2.00918074438003,-0.158333333333437,
11.1894381952052));
#60066=CARTESIAN_POINT('Ctrl Pts',(2.03298765738055,0.158333333333439,11.1774913875267));
#60067=CARTESIAN_POINT('Ctrl Pts',(2.06058997240673,0.319434907277377,11.1982575640768));
#60068=CARTESIAN_POINT('Ctrl Pts',(2.11519541076701,0.636309800095627,11.2498267210703));
#60069=CARTESIAN_POINT('Ctrl Pts',(2.15641126259881,0.79477268400137,11.2980101206211));
#60070=CARTESIAN_POINT('Ctrl Pts',(2.20851609507492,1.06847604194595,11.3735793773766));
#60071=CARTESIAN_POINT('Ctrl Pts',(2.22914556343519,1.18514270861282,11.408481012808));
#60072=CARTESIAN_POINT('Ctrl Pts',(2.24785024885114,1.30000000000124,11.4455731525382));
#60073=CARTESIAN_POINT('Ctrl Pts',(2.02156140521162,-1.30000000000232,11.5201193794798));
#60074=CARTESIAN_POINT('Ctrl Pts',(2.01404955018037,-1.1851427086135,11.4702923408371));
#60075=CARTESIAN_POINT('Ctrl Pts',(2.0069663174992,-1.06847604194621,11.4233369281064));
#60076=CARTESIAN_POINT('Ctrl Pts',(1.99159283638421,-0.794772684001226,
11.3214945616243));
#60077=CARTESIAN_POINT('Ctrl Pts',(1.97899458630368,-0.636309800095498,
11.2598662087087));
#60078=CARTESIAN_POINT('Ctrl Pts',(1.97382404237879,-0.319434907277311,
11.1830580850164));
#60079=CARTESIAN_POINT('Ctrl Pts',(1.9721734549569,-0.158333333333407,11.1516538828691));
#60080=CARTESIAN_POINT('Ctrl Pts',(1.99518066312744,0.158333333333409,11.140241072183));
#60081=CARTESIAN_POINT('Ctrl Pts',(2.01959671087466,0.319434907277317,11.1603570980484));
#60082=CARTESIAN_POINT('Ctrl Pts',(2.07212370422326,0.636309800095506,11.2136642768154));
#60083=CARTESIAN_POINT('Ctrl Pts',(2.11003874386777,0.794772684001218,11.2626377884138));
#60084=CARTESIAN_POINT('Ctrl Pts',(2.16716226267848,1.06847604194575,11.3438957364248));
#60085=CARTESIAN_POINT('Ctrl Pts',(2.19191591882493,1.18514270861259,11.3821875190118));
#60086=CARTESIAN_POINT('Ctrl Pts',(2.21669657645966,1.30000000000099,11.4235975293956));
#60087=CARTESIAN_POINT('Ctrl Pts',(1.98618970204284,-1.30000000000202,11.4873857546929));
#60088=CARTESIAN_POINT('Ctrl Pts',(1.97258910993661,-1.18514270861323,11.43064141872));
#60089=CARTESIAN_POINT('Ctrl Pts',(1.96126776052509,-1.06847604194597,11.3784887101778));
#60090=CARTESIAN_POINT('Ctrl Pts',(1.94037868514204,-0.794772684001049,
11.2686130982488));
#60091=CARTESIAN_POINT('Ctrl Pts',(1.93083613120932,-0.636309800095354,
11.2070608321537));
#60092=CARTESIAN_POINT('Ctrl Pts',(1.92609493733045,-0.319434907277237,
11.1296040666681));
#60093=CARTESIAN_POINT('Ctrl Pts',(1.92608674948616,-0.158333333333371,
11.1006567592145));
#60094=CARTESIAN_POINT('Ctrl Pts',(1.94760007049155,0.158333333333373,11.0901609205059));
#60095=CARTESIAN_POINT('Ctrl Pts',(1.9681369910674,0.319434907277246,11.1091527146429));
#60096=CARTESIAN_POINT('Ctrl Pts',(2.01870480624482,0.636309800095363,11.1641296084854));
#60097=CARTESIAN_POINT('Ctrl Pts',(2.0541842077594,0.794772684001037,11.2127661066329));
#60098=CARTESIAN_POINT('Ctrl Pts',(2.11720864062985,1.0684760419455,11.3019861247598));
#60099=CARTESIAN_POINT('Ctrl Pts',(2.14648289278499,1.18514270861232,11.3453784510037));
#60100=CARTESIAN_POINT('Ctrl Pts',(2.17775045539106,1.3000000000007,11.3935430635718));
#60101=CARTESIAN_POINT('Ctrl Pts',(1.95657107896372,-1.30000000000192,11.4578927873015));
#60102=CARTESIAN_POINT('Ctrl Pts',(1.93806150394524,-1.18514270861314,11.394863359753));
#60103=CARTESIAN_POINT('Ctrl Pts',(1.92340308449501,-1.06847604194589,11.337959254602));
#60104=CARTESIAN_POINT('Ctrl Pts',(1.89843614294196,-0.79477268400099,11.220650108181));
#60105=CARTESIAN_POINT('Ctrl Pts',(1.89156991148624,-0.636309800095305,
11.1592104192819));
#60106=CARTESIAN_POINT('Ctrl Pts',(1.8883872827842,-0.319434907277212,11.0804848377892));
#60107=CARTESIAN_POINT('Ctrl Pts',(1.89152698230331,-0.158333333333359,
11.0526443347744));
#60108=CARTESIAN_POINT('Ctrl Pts',(1.91208041730841,0.158333333333361,11.0426727723083));
#60109=CARTESIAN_POINT('Ctrl Pts',(1.92853344745413,0.31943490727722,11.0609832641629));
#60110=CARTESIAN_POINT('Ctrl Pts',(1.97553883097018,0.636309800095313,11.1184980826711));
#60111=CARTESIAN_POINT('Ctrl Pts',(2.00639081156863,0.794772684000975,11.1684223167876));
#60112=CARTESIAN_POINT('Ctrl Pts',(2.07320017460509,1.06847604194542,11.2654468820485));
#60113=CARTESIAN_POINT('Ctrl Pts',(2.10619712120972,1.18514270861223,11.3134355555938));
#60114=CARTESIAN_POINT('Ctrl Pts',(2.14327171669138,1.3000000000006,11.3674145634973));
#60115=CARTESIAN_POINT('Ctrl Pts',(1.93919233834441,-1.30000000000188,11.4412683292781));
#60116=CARTESIAN_POINT('Ctrl Pts',(1.9180392072829,-1.1851427086131,11.3744922842501));
#60117=CARTESIAN_POINT('Ctrl Pts',(1.9016915027463,-1.06847604194585,11.3147015044614));
#60118=CARTESIAN_POINT('Ctrl Pts',(1.87502653151455,-0.794772684000963,
11.1927102021457));
#60119=CARTESIAN_POINT('Ctrl Pts',(1.87077154762912,-0.636309800095285,
11.1307075350712));
#60120=CARTESIAN_POINT('Ctrl Pts',(1.86832967967525,-0.319434907277203,
11.0513547758013));
#60121=CARTESIAN_POINT('Ctrl Pts',(1.87173814123926,-0.158333333333354,
11.0250975637534));
#60122=CARTESIAN_POINT('Ctrl Pts',(1.89154572095382,0.158333333333356,11.0155265525274));
#60123=CARTESIAN_POINT('Ctrl Pts',(1.9065535778102,0.319434907277211,11.032871367099));
#60124=CARTESIAN_POINT('Ctrl Pts',(1.95217595853164,0.636309800095294,11.0913871168503));
#60125=CARTESIAN_POINT('Ctrl Pts',(1.98078372227384,0.794772684000952,11.1417282263698));
#60126=CARTESIAN_POINT('Ctrl Pts',(2.04993983042539,1.06847604194539,11.2431289591996));
#60127=CARTESIAN_POINT('Ctrl Pts',(2.08504196414533,1.18514270861219,11.2937958862347));
#60128=CARTESIAN_POINT('Ctrl Pts',(2.12531111485276,1.30000000000056,11.3512371203305));
#60129=CARTESIAN_POINT('Ctrl Pts',(1.92704926329494,-1.30000000000182,11.4283111506925));
#60130=CARTESIAN_POINT('Ctrl Pts',(1.90399556245151,-1.18514270861305,11.3587746878215));
#60131=CARTESIAN_POINT('Ctrl Pts',(1.8864011954364,-1.0684760419458,11.296885098931));
#60132=CARTESIAN_POINT('Ctrl Pts',(1.85836684116995,-0.794772684000927,
11.1715735762711));
#60133=CARTESIAN_POINT('Ctrl Pts',(1.85548565900223,-0.636309800095255,
11.1095352181817));
#60134=CARTESIAN_POINT('Ctrl Pts',(1.85390906783529,-0.319434907277188,
11.0295476705844));
#60135=CARTESIAN_POINT('Ctrl Pts',(1.85864937632493,-0.158333333333347,
11.0037448778369));
#60136=CARTESIAN_POINT('Ctrl Pts',(1.87802031518014,0.158333333333349,10.9943852668516));
#60137=CARTESIAN_POINT('Ctrl Pts',(1.89121780193844,0.319434907277195,11.011465514906));
#60138=CARTESIAN_POINT('Ctrl Pts',(1.93517081113783,0.636309800095263,11.0710905506731));
#60139=CARTESIAN_POINT('Ctrl Pts',(1.9619143550451,0.794772684000913,11.1218360551467));
#60140=CARTESIAN_POINT('Ctrl Pts',(2.03209926506429,1.06847604194534,11.2268812699618));
#60141=CARTESIAN_POINT('Ctrl Pts',(2.06840033622108,1.18514270861214,11.2797402876574));
#60142=CARTESIAN_POINT('Ctrl Pts',(2.11062203159456,1.3000000000005,11.3399881418638));
#60143=CARTESIAN_POINT('Ctrl Pts',(1.914880110088,-1.30000000000179,11.4152490614093));
#60144=CARTESIAN_POINT('Ctrl Pts',(1.88981935390603,-1.18514270861302,11.3428017862381));
#60145=CARTESIAN_POINT('Ctrl Pts',(1.87101009618621,-1.06847604194578,11.278635514902));
#60146=CARTESIAN_POINT('Ctrl Pts',(1.84199916012994,-0.794772684000909,
11.1495293671655));
#60147=CARTESIAN_POINT('Ctrl Pts',(1.84221824671498,-0.636309800095243,
11.0864611756966));
#60148=CARTESIAN_POINT('Ctrl Pts',(1.84038936278642,-0.319434907277182,
11.0064566878396));
#60149=CARTESIAN_POINT('Ctrl Pts',(1.84277700745507,-0.158333333333344,
10.983313889559));
#60150=CARTESIAN_POINT('Ctrl Pts',(1.86114349767242,0.158333333333346,10.9744875571855));
#60151=CARTESIAN_POINT('Ctrl Pts',(1.87507451244635,0.31943490727719,10.9897506965998));
#60152=CARTESIAN_POINT('Ctrl Pts',(1.91848589835599,0.636309800095253,11.0498482751571));
#60153=CARTESIAN_POINT('Ctrl Pts',(1.9430051609863,0.794772684000899,11.1012117979008));
#60154=CARTESIAN_POINT('Ctrl Pts',(2.01469293575375,1.06847604194532,11.2098347414939));
#60155=CARTESIAN_POINT('Ctrl Pts',(2.05246100102385,1.18514270861212,11.2648637130279));
#60156=CARTESIAN_POINT('Ctrl Pts',(2.09696615016107,1.30000000000047,11.3279028086911));
#60157=CARTESIAN_POINT('Ctrl Pts',(1.90480129625303,-1.30000000000176,11.4044692218274));
#60158=CARTESIAN_POINT('Ctrl Pts',(1.87895670415632,-1.18514270861299,11.3293601806111));
#60159=CARTESIAN_POINT('Ctrl Pts',(1.85940829677877,-1.06847604194575,11.263351254962));
#60160=CARTESIAN_POINT('Ctrl Pts',(1.8287930113399,-0.794772684000891,11.1318805191049));
#60161=CARTESIAN_POINT('Ctrl Pts',(1.82780080485016,-0.636309800095226,
11.0701491495695));
#60162=CARTESIAN_POINT('Ctrl Pts',(1.82522869434448,-0.319434907277173,
10.9905363761722));
#60163=CARTESIAN_POINT('Ctrl Pts',(1.82789637381727,-0.15833333333334,10.9683131199583));
#60164=CARTESIAN_POINT('Ctrl Pts',(1.84678133526567,0.158333333333342,10.9591666172288));
#60165=CARTESIAN_POINT('Ctrl Pts',(1.86174136838708,0.319434907277182,10.9727236463819));
#60166=CARTESIAN_POINT('Ctrl Pts',(1.9053417109919,0.636309800095236,11.0327273653333));
#60167=CARTESIAN_POINT('Ctrl Pts',(1.92819293348889,0.794772684000877,11.0844005483245));
#60168=CARTESIAN_POINT('Ctrl Pts',(2.00107046142142,1.06847604194529,11.1956723375267));
#60169=CARTESIAN_POINT('Ctrl Pts',(2.03992079422669,1.18514270861209,11.2523804603006));
#60170=CARTESIAN_POINT('Ctrl Pts',(2.08607547837377,1.30000000000044,11.3176312713287));
#60171=CARTESIAN_POINT('Ctrl Pts',(1.89327770970022,-1.30000000000175,11.3910324012902));
#60172=CARTESIAN_POINT('Ctrl Pts',(1.86630585421885,-1.18514270861298,11.3123850522012));
#60173=CARTESIAN_POINT('Ctrl Pts',(1.8455645163665,-1.06847604194574,11.2439803084536));
#60174=CARTESIAN_POINT('Ctrl Pts',(1.81204161877102,-0.79477268400088,11.10961413344));
#60175=CARTESIAN_POINT('Ctrl Pts',(1.80841575954142,-0.636309800095219,
11.050011281481));
#60176=CARTESIAN_POINT('Ctrl Pts',(1.8038742456901,-0.31943490727717,10.9713236115184));
#60177=CARTESIAN_POINT('Ctrl Pts',(1.80677796494244,-0.158333333333338,
10.9504155263368));
#60178=CARTESIAN_POINT('Ctrl Pts',(1.82555990331626,0.15833333333334,10.9413025549763));
#60179=CARTESIAN_POINT('Ctrl Pts',(1.84045534302504,0.319434907277178,10.9533997001063));
#60180=CARTESIAN_POINT('Ctrl Pts',(1.88525616390058,0.636309800095228,11.012909687534));
#60181=CARTESIAN_POINT('Ctrl Pts',(1.90913975376704,0.794772684000867,11.0633947089013));
#60182=CARTESIAN_POINT('Ctrl Pts',(1.98480688961782,1.06847604194528,11.1776920503212));
#60183=CARTESIAN_POINT('Ctrl Pts',(2.02516002756491,1.18514270861207,11.2366557310892));
#60184=CARTESIAN_POINT('Ctrl Pts',(2.073112804093,1.30000000000043,11.3051080086584));
#60185=CARTESIAN_POINT('Ctrl Pts',(1.88533826855979,-1.3000000000017,11.3819390151657));
#60186=CARTESIAN_POINT('Ctrl Pts',(1.85877864422648,-1.18514270861294,11.3001911079613));
#60187=CARTESIAN_POINT('Ctrl Pts',(1.837718248409,-1.0684760419457,11.2299700072838));
#60188=CARTESIAN_POINT('Ctrl Pts',(1.80176883894143,-0.794772684000851,
11.0943744460428));
#60189=CARTESIAN_POINT('Ctrl Pts',(1.79303694377367,-0.636309800095197,
11.0389207988312));
#60190=CARTESIAN_POINT('Ctrl Pts',(1.78572104870416,-0.319434907277159,
10.9623346432985));
#60191=CARTESIAN_POINT('Ctrl Pts',(1.78936170987159,-0.158333333333332,
10.9422136296668));
#60192=CARTESIAN_POINT('Ctrl Pts',(1.8080248988652,0.158333333333334,10.9332122433578));
#60193=CARTESIAN_POINT('Ctrl Pts',(1.82221963518582,0.319434907277167,10.9446174247407));
#60194=CARTESIAN_POINT('Ctrl Pts',(1.869237254135,0.636309800095206,11.0022867514235));
#60195=CARTESIAN_POINT('Ctrl Pts',(1.89712646388558,0.79477268400084,11.0489532910959));
#60196=CARTESIAN_POINT('Ctrl Pts',(1.97527792161974,1.06847604194524,11.1644588769458));
#60197=CARTESIAN_POINT('Ctrl Pts',(2.0162566695385,1.18514270861203,11.2251351015703));
#60198=CARTESIAN_POINT('Ctrl Pts',(2.06438529511981,1.30000000000038,11.2964894626088));
#60199=CARTESIAN_POINT('Ctrl Pts',(1.87799128879424,-1.3000000000017,11.3774649241137));
#60200=CARTESIAN_POINT('Ctrl Pts',(1.85162982048174,-1.18514270861294,11.2958715822796));
#60201=CARTESIAN_POINT('Ctrl Pts',(1.83046672246868,-1.0684760419457,11.2259796900101));
#60202=CARTESIAN_POINT('Ctrl Pts',(1.79358500771746,-0.794772684000851,
11.0915481264036));
#60203=CARTESIAN_POINT('Ctrl Pts',(1.78288365918825,-0.636309800095197,
11.0377389598563));
#60204=CARTESIAN_POINT('Ctrl Pts',(1.77431562872862,-0.319434907277159,
10.9622827219367));
#60205=CARTESIAN_POINT('Ctrl Pts',(1.77794490963746,-0.158333333333332,
10.9421106139582));
#60206=CARTESIAN_POINT('Ctrl Pts',(1.79644754730033,0.158333333333334,10.9332833264162));
#60207=CARTESIAN_POINT('Ctrl Pts',(1.8102831109525,0.319434907277167,10.9450989989837));
#60208=CARTESIAN_POINT('Ctrl Pts',(1.85865359192218,0.636309800095206,11.0016155958775));
#60209=CARTESIAN_POINT('Ctrl Pts',(1.8893645694356,0.79477268400084,11.0459682230072));
#60210=CARTESIAN_POINT('Ctrl Pts',(1.96832072991246,1.06847604194524,11.1603953244879));
#60211=CARTESIAN_POINT('Ctrl Pts',(2.00914338193007,1.18514270861203,11.2209304357419));
#60212=CARTESIAN_POINT('Ctrl Pts',(2.05661148970894,1.30000000000038,11.292469405961));
#60213=CARTESIAN_POINT('Ctrl Pts',(1.87799128879385,-1.3,11.3774649241125));
#60214=CARTESIAN_POINT('Ctrl Pts',(1.85162982048153,-1.18514270861178,11.2958715822789));
#60215=CARTESIAN_POINT('Ctrl Pts',(1.8304667224686,-1.06847604194512,11.2259796900098));
#60216=CARTESIAN_POINT('Ctrl Pts',(1.79358500771746,-0.794772684000851,
11.0915481264036));
#60217=CARTESIAN_POINT('Ctrl Pts',(1.78288365918825,-0.636309800095197,
11.0377389598563));
#60218=CARTESIAN_POINT('Ctrl Pts',(1.77431562872862,-0.319434907277159,
10.9622827219367));
#60219=CARTESIAN_POINT('Ctrl Pts',(1.77794490963746,-0.158333333333332,
10.9421106139582));
#60220=CARTESIAN_POINT('Ctrl Pts',(1.79644754730033,0.158333333333334,10.9332833264162));
#60221=CARTESIAN_POINT('Ctrl Pts',(1.8102831109525,0.319434907277167,10.9450989989837));
#60222=CARTESIAN_POINT('Ctrl Pts',(1.85865359192218,0.636309800095206,11.0016155958775));
#60223=CARTESIAN_POINT('Ctrl Pts',(1.8893645694356,0.79477268400084,11.0459682230072));
#60224=CARTESIAN_POINT('Ctrl Pts',(1.96832072991242,1.06847604194511,11.1603953244878));
#60225=CARTESIAN_POINT('Ctrl Pts',(2.00914338192998,1.18514270861177,11.2209304357418));
#60226=CARTESIAN_POINT('Ctrl Pts',(2.05661148970878,1.3,11.2924694059607));
#60227=CARTESIAN_POINT('',(2.2068264837238,-1.2,11.6308483240498));
#60228=CARTESIAN_POINT('Ctrl Pts',(2.2068264837238,-1.2,11.6308483240498));
#60229=CARTESIAN_POINT('Ctrl Pts',(2.18724117329495,-1.21681996775978,11.6218122533617));
#60230=CARTESIAN_POINT('Ctrl Pts',(2.16689868522774,-1.23318534441601,11.6135926611327));
#60231=CARTESIAN_POINT('Ctrl Pts',(2.12884789480307,-1.2658888355048,11.5957608209235));
#60232=CARTESIAN_POINT('Ctrl Pts',(2.11003562568207,-1.28160650336713,11.5873866307135));
#60233=CARTESIAN_POINT('Ctrl Pts',(2.09094241353359,-1.2984242831365,11.5778701597891));
#60234=CARTESIAN_POINT('Ctrl Pts',(2.09005049051658,-1.29921222705947,11.5774229103209));
#60235=CARTESIAN_POINT('Ctrl Pts',(2.08916175672605,-1.30000000000272,11.5769742007701));
#60236=CARTESIAN_POINT('',(2.34584242549889,-0.653834841417007,11.5588442636176));
#60237=CARTESIAN_POINT('Ctrl Pts',(2.34584242550886,-0.653834841416324,
11.5588442636418));
#60238=CARTESIAN_POINT('Ctrl Pts',(2.33152214904514,-0.717927032198887,
11.5665511487796));
#60239=CARTESIAN_POINT('Ctrl Pts',(2.31982760984721,-0.763778390313212,
11.5727769806235));
#60240=CARTESIAN_POINT('Ctrl Pts',(2.2739524493678,-0.949540773186723,11.5969165862991));
#60241=CARTESIAN_POINT('Ctrl Pts',(2.24889659026364,-1.04883931167899,11.6098949041864));
#60242=CARTESIAN_POINT('Ctrl Pts',(2.2068264837238,-1.2,11.6308483240498));
#60243=CARTESIAN_POINT('',(2.46774460503139,0.653834841531101,11.491006474516));
#60244=CARTESIAN_POINT('Ctrl Pts',(2.46774460503136,0.6538348415311,11.491006474516));
#60245=CARTESIAN_POINT('Ctrl Pts',(2.43368778115467,0.575795030619156,11.4669914411289));
#60246=CARTESIAN_POINT('Ctrl Pts',(2.40474750894542,0.493918313629019,11.447426688817));
#60247=CARTESIAN_POINT('Ctrl Pts',(2.3613754176558,0.338197324327257,11.4211796538803));
#60248=CARTESIAN_POINT('Ctrl Pts',(2.34543349869105,0.265711097259163,11.4130062283616));
#60249=CARTESIAN_POINT('Ctrl Pts',(2.3220968049692,0.129740576115995,11.4058460663461));
#60250=CARTESIAN_POINT('Ctrl Pts',(2.3138153758775,0.0666412396508463,11.4056782828097));
#60251=CARTESIAN_POINT('Ctrl Pts',(2.30198027918302,-0.0595498475940219,
11.4118386452963));
#60252=CARTESIAN_POINT('Ctrl Pts',(2.29832871714705,-0.122796020472284,
11.4181987058642));
#60253=CARTESIAN_POINT('Ctrl Pts',(2.29622270118133,-0.260148735050006,
11.4388365912281));
#60254=CARTESIAN_POINT('Ctrl Pts',(2.29883477760314,-0.333948670529117,
11.4543476372232));
#60255=CARTESIAN_POINT('Ctrl Pts',(2.31349450820435,-0.491142050749671,
11.4967086246876));
#60256=CARTESIAN_POINT('Ctrl Pts',(2.32698040039238,-0.574253995386567,
11.5252254122324));
#60257=CARTESIAN_POINT('Ctrl Pts',(2.34584242545894,-0.653834841428697,
11.5588442636123));
#60258=CARTESIAN_POINT('',(2.40489628334222,1.2,11.5265429463218));
#60259=CARTESIAN_POINT('Ctrl Pts',(2.40489628334222,1.2,11.5265429463218));
#60260=CARTESIAN_POINT('Ctrl Pts',(2.41582048848703,1.1340365096965,11.5204707587399));
#60261=CARTESIAN_POINT('Ctrl Pts',(2.43005844632245,1.038218713922,11.5125009027098));
#60262=CARTESIAN_POINT('Ctrl Pts',(2.45771077440481,0.795149709173985,11.496781434669));
#60263=CARTESIAN_POINT('Ctrl Pts',(2.46206175224414,0.741496517834653,11.4942746656479));
#60264=CARTESIAN_POINT('Ctrl Pts',(2.46774460503137,0.653834841531098,11.491006474516));
#60265=CARTESIAN_POINT('Ctrl Pts',(2.29116136298904,1.3000000000003,11.4747022830536));
#60266=CARTESIAN_POINT('Ctrl Pts',(2.30969599627212,1.28317246189965,11.4838602831997));
#60267=CARTESIAN_POINT('Ctrl Pts',(2.32883998949747,1.26664026084675,11.492301893308));
#60268=CARTESIAN_POINT('Ctrl Pts',(2.36390070845054,1.23528691103208,11.5088851378804));
#60269=CARTESIAN_POINT('Ctrl Pts',(2.38633959798998,1.21551346690462,11.5191086603475));
#60270=CARTESIAN_POINT('Ctrl Pts',(2.40489628334222,1.2,11.5265429463218));
#60271=CARTESIAN_POINT('Ctrl Pts',(1.87799128879384,-1.3,11.3774649241125));
#60272=CARTESIAN_POINT('Ctrl Pts',(1.85162982048153,-1.18514270861178,11.2958715822789));
#60273=CARTESIAN_POINT('Ctrl Pts',(1.8304667224686,-1.06847604194512,11.2259796900098));
#60274=CARTESIAN_POINT('Ctrl Pts',(1.79358500771746,-0.794772684000851,
11.0915481264036));
#60275=CARTESIAN_POINT('Ctrl Pts',(1.78288365918825,-0.636309800095197,
11.0377389598563));
#60276=CARTESIAN_POINT('Ctrl Pts',(1.77431562872862,-0.319434907277159,
10.9622827219367));
#60277=CARTESIAN_POINT('Ctrl Pts',(1.77794490963746,-0.158333333333332,
10.9421106139582));
#60278=CARTESIAN_POINT('Ctrl Pts',(1.79644754730034,0.158333333333334,10.9332833264162));
#60279=CARTESIAN_POINT('Ctrl Pts',(1.8102831109525,0.319434907277167,10.9450989989837));
#60280=CARTESIAN_POINT('Ctrl Pts',(1.85865359192218,0.636309800095206,11.0016155958775));
#60281=CARTESIAN_POINT('Ctrl Pts',(1.8893645694356,0.79477268400084,11.0459682230072));
#60282=CARTESIAN_POINT('Ctrl Pts',(1.96832072991242,1.06847604194511,11.1603953244878));
#60283=CARTESIAN_POINT('Ctrl Pts',(2.00914338192998,1.18514270861178,11.2209304357418));
#60284=CARTESIAN_POINT('Ctrl Pts',(2.05661148970878,1.3,11.2924694059607));
#60285=CARTESIAN_POINT('Ctrl Pts',(1.80704611563284,-1.3,11.407228856645));
#60286=CARTESIAN_POINT('Ctrl Pts',(1.78233798615881,-1.18514270861178,11.3251184310253));
#60287=CARTESIAN_POINT('Ctrl Pts',(1.76233903122006,-1.06847604194512,11.2549094900764));
#60288=CARTESIAN_POINT('Ctrl Pts',(1.72701657977795,-0.794772684000851,
11.1202076017071));
#60289=CARTESIAN_POINT('Ctrl Pts',(1.71574542397769,-0.636309800095197,
11.0668346892391));
#60290=CARTESIAN_POINT('Ctrl Pts',(1.70682212124656,-0.319434907277159,
10.9919427781636));
#60291=CARTESIAN_POINT('Ctrl Pts',(1.70940065624172,-0.158333333333332,
10.9724320209495));
#60292=CARTESIAN_POINT('Ctrl Pts',(1.72804929275646,0.158333333333334,10.9639326521977));
#60293=CARTESIAN_POINT('Ctrl Pts',(1.74307942205737,0.319434907277167,10.9754099984146));
#60294=CARTESIAN_POINT('Ctrl Pts',(1.79210700315155,0.636309800095206,11.0320401849215));
#60295=CARTESIAN_POINT('Ctrl Pts',(1.82352345611137,0.79477268400084,11.0762612736829));
#60296=CARTESIAN_POINT('Ctrl Pts',(1.90123537533585,1.06847604194511,11.1916662510505));
#60297=CARTESIAN_POINT('Ctrl Pts',(1.9410434505065,1.18514270861178,11.2528543422308));
#60298=CARTESIAN_POINT('Ctrl Pts',(1.98702099052593,1.3,11.3252759860648));
#60299=CARTESIAN_POINT('Ctrl Pts',(1.73610094247183,-1.3,11.4369927891775));
#60300=CARTESIAN_POINT('Ctrl Pts',(1.71304615183608,-1.18514270861178,11.3543652797717));
#60301=CARTESIAN_POINT('Ctrl Pts',(1.69421133997152,-1.06847604194512,11.283839290143));
#60302=CARTESIAN_POINT('Ctrl Pts',(1.66044815183843,-0.794772684000851,
11.1488670770106));
#60303=CARTESIAN_POINT('Ctrl Pts',(1.64860718876712,-0.636309800095197,
11.0959304186219));
#60304=CARTESIAN_POINT('Ctrl Pts',(1.63932861376449,-0.319434907277159,
11.0216028343905));
#60305=CARTESIAN_POINT('Ctrl Pts',(1.64085640284598,-0.158333333333332,
11.0027534279408));
#60306=CARTESIAN_POINT('Ctrl Pts',(1.65965103821258,0.158333333333334,10.9945819779792));
#60307=CARTESIAN_POINT('Ctrl Pts',(1.67587573316224,0.319434907277167,11.0057209978454));
#60308=CARTESIAN_POINT('Ctrl Pts',(1.72556041438091,0.636309800095206,11.0624647739656));
#60309=CARTESIAN_POINT('Ctrl Pts',(1.75768234278715,0.79477268400084,11.1065543243585));
#60310=CARTESIAN_POINT('Ctrl Pts',(1.83415002075929,1.06847604194511,11.2229371776131));
#60311=CARTESIAN_POINT('Ctrl Pts',(1.87294351908302,1.18514270861178,11.2847782487198));
#60312=CARTESIAN_POINT('Ctrl Pts',(1.91743049134307,1.3,11.3580825661689));
#60313=CARTESIAN_POINT('Ctrl Pts',(1.66515576931082,-1.3,11.46675672171));
#60314=CARTESIAN_POINT('Ctrl Pts',(1.64375431751336,-1.18514270861178,11.3836121285181));
#60315=CARTESIAN_POINT('Ctrl Pts',(1.62608364872297,-1.06847604194512,11.3127690902096));
#60316=CARTESIAN_POINT('Ctrl Pts',(1.59387972389892,-0.794772684000851,
11.1775265523141));
#60317=CARTESIAN_POINT('Ctrl Pts',(1.58146895355656,-0.636309800095197,
11.1250261480047));
#60318=CARTESIAN_POINT('Ctrl Pts',(1.57183510628243,-0.319434907277159,
11.0512628906174));
#60319=CARTESIAN_POINT('Ctrl Pts',(1.57231214945024,-0.158333333333332,
11.0330748349321));
#60320=CARTESIAN_POINT('Ctrl Pts',(1.59125278366871,0.158333333333334,11.0252313037607));
#60321=CARTESIAN_POINT('Ctrl Pts',(1.60867204426711,0.319434907277167,11.0360319972763));
#60322=CARTESIAN_POINT('Ctrl Pts',(1.65901382561028,0.636309800095206,11.0928893630096));
#60323=CARTESIAN_POINT('Ctrl Pts',(1.69184122946292,0.79477268400084,11.1368473750342));
#60324=CARTESIAN_POINT('Ctrl Pts',(1.76706466618273,1.06847604194511,11.2542081041758));
#60325=CARTESIAN_POINT('Ctrl Pts',(1.80484358765954,1.18514270861178,11.3167021552088));
#60326=CARTESIAN_POINT('Ctrl Pts',(1.84783999216022,1.3,11.390889146273));
#60327=CARTESIAN_POINT('Ctrl Pts',(1.66515576931082,-1.3,11.46675672171));
#60328=CARTESIAN_POINT('Ctrl Pts',(1.64375431751336,-1.18514270861178,11.3836121285181));
#60329=CARTESIAN_POINT('Ctrl Pts',(1.62608364872297,-1.06847604194512,11.3127690902096));
#60330=CARTESIAN_POINT('Ctrl Pts',(1.59387972389892,-0.794772684000851,
11.1775265523141));
#60331=CARTESIAN_POINT('Ctrl Pts',(1.58146895355656,-0.636309800095197,
11.1250261480047));
#60332=CARTESIAN_POINT('Ctrl Pts',(1.57183510628243,-0.319434907277159,
11.0512628906174));
#60333=CARTESIAN_POINT('Ctrl Pts',(1.57231214945024,-0.158333333333332,
11.0330748349321));
#60334=CARTESIAN_POINT('Ctrl Pts',(1.59125278366871,0.158333333333334,11.0252313037607));
#60335=CARTESIAN_POINT('Ctrl Pts',(1.6086720442671,0.319434907277167,11.0360319972763));
#60336=CARTESIAN_POINT('Ctrl Pts',(1.65901382561028,0.636309800095206,11.0928893630096));
#60337=CARTESIAN_POINT('Ctrl Pts',(1.69184122946292,0.79477268400084,11.1368473750342));
#60338=CARTESIAN_POINT('Ctrl Pts',(1.76706466618273,1.06847604194511,11.2542081041758));
#60339=CARTESIAN_POINT('Ctrl Pts',(1.80484358765954,1.18514270861178,11.3167021552088));
#60340=CARTESIAN_POINT('Ctrl Pts',(1.84783999216022,1.3,11.390889146273));
#60341=CARTESIAN_POINT('Ctrl Pts',(1.66515576931083,-1.30000000000005,11.46675672171));
#60342=CARTESIAN_POINT('Ctrl Pts',(1.64375431751336,-1.18514270861182,11.3836121285181));
#60343=CARTESIAN_POINT('Ctrl Pts',(1.62608364872297,-1.06847604194513,11.3127690902096));
#60344=CARTESIAN_POINT('Ctrl Pts',(1.59387972389892,-0.794772684000851,
11.1775265523141));
#60345=CARTESIAN_POINT('Ctrl Pts',(1.58146895355655,-0.636309800095197,
11.1250261480047));
#60346=CARTESIAN_POINT('Ctrl Pts',(1.57183510628243,-0.319434907277159,
11.0512628906174));
#60347=CARTESIAN_POINT('Ctrl Pts',(1.57231214945024,-0.158333333333332,
11.0330748349321));
#60348=CARTESIAN_POINT('Ctrl Pts',(1.5912527836687,0.158333333333334,11.0252313037607));
#60349=CARTESIAN_POINT('Ctrl Pts',(1.6086720442671,0.319434907277167,11.0360319972763));
#60350=CARTESIAN_POINT('Ctrl Pts',(1.65901382561028,0.636309800095206,11.0928893630096));
#60351=CARTESIAN_POINT('Ctrl Pts',(1.69184122946292,0.79477268400084,11.1368473750342));
#60352=CARTESIAN_POINT('Ctrl Pts',(1.76706466618285,1.06847604194556,11.254208104176));
#60353=CARTESIAN_POINT('Ctrl Pts',(1.80484358765983,1.18514270861267,11.3167021552093));
#60354=CARTESIAN_POINT('Ctrl Pts',(1.84783999216071,1.30000000000132,11.3908891462739));
#60355=CARTESIAN_POINT('Ctrl Pts',(1.66294156245547,-1.30000000000005,11.4752237278628));
#60356=CARTESIAN_POINT('Ctrl Pts',(1.64211927469555,-1.18514270861182,11.391711801944));
#60357=CARTESIAN_POINT('Ctrl Pts',(1.62444818678087,-1.06847604194513,11.3206583385042));
#60358=CARTESIAN_POINT('Ctrl Pts',(1.59090434064678,-0.794772684000851,
11.1852921643951));
#60359=CARTESIAN_POINT('Ctrl Pts',(1.57488586700129,-0.636309800095197,
11.1333404325032));
#60360=CARTESIAN_POINT('Ctrl Pts',(1.56349013315575,-0.319434907277159,
11.0598112207211));
#60361=CARTESIAN_POINT('Ctrl Pts',(1.56451256412487,-0.158333333333332,
11.041630919885));
#60362=CARTESIAN_POINT('Ctrl Pts',(1.5836900087521,0.158333333333334,11.0337845706398));
#60363=CARTESIAN_POINT('Ctrl Pts',(1.60107891375656,0.319434907277167,11.044542618244));
#60364=CARTESIAN_POINT('Ctrl Pts',(1.65309822965178,0.636309800095206,11.1012255285261));
#60365=CARTESIAN_POINT('Ctrl Pts',(1.68846554231891,0.79477268400084,11.1448203238114));
#60366=CARTESIAN_POINT('Ctrl Pts',(1.7651778318562,1.06847604194556,11.2622670815464));
#60367=CARTESIAN_POINT('Ctrl Pts',(1.80327012403914,1.18514270861267,11.3249050933935));
#60368=CARTESIAN_POINT('Ctrl Pts',(1.84624880073474,1.30000000000132,11.3993427674954));
#60369=CARTESIAN_POINT('Ctrl Pts',(1.66352992364858,-1.30000000000005,11.487474413773));
#60370=CARTESIAN_POINT('Ctrl Pts',(1.64473762368632,-1.18514270861181,11.4060420060404));
#60371=CARTESIAN_POINT('Ctrl Pts',(1.62791338132392,-1.06847604194513,11.3366047299185));
#60372=CARTESIAN_POINT('Ctrl Pts',(1.59359262255284,-0.794772684000851,
11.2039018848358));
#60373=CARTESIAN_POINT('Ctrl Pts',(1.57205079459115,-0.636309800095196,
11.1523732203483));
#60374=CARTESIAN_POINT('Ctrl Pts',(1.55780491322402,-0.319434907277158,
11.0792600320647));
#60375=CARTESIAN_POINT('Ctrl Pts',(1.55879634907134,-0.158333333333332,
11.0600902727381));
#60376=CARTESIAN_POINT('Ctrl Pts',(1.57813469347016,0.158333333333334,11.0522311225344));
#60377=CARTESIAN_POINT('Ctrl Pts',(1.59559909903037,0.319434907277167,11.0640703860129));
#60378=CARTESIAN_POINT('Ctrl Pts',(1.65103339058184,0.636309800095205,11.1200982203511));
#60379=CARTESIAN_POINT('Ctrl Pts',(1.69291229251351,0.794772684000838,11.1626715245407));
#60380=CARTESIAN_POINT('Ctrl Pts',(1.77033498791918,1.06847604194556,11.2774862822592));
#60381=CARTESIAN_POINT('Ctrl Pts',(1.80728926966501,1.18514270861267,11.3386684002332));
#60382=CARTESIAN_POINT('Ctrl Pts',(1.8476844171091,1.30000000000132,11.4113335818709));
#60383=CARTESIAN_POINT('Ctrl Pts',(1.66410716288398,-1.30000000000005,11.5054993221241));
#60384=CARTESIAN_POINT('Ctrl Pts',(1.64649300104017,-1.18514270861181,11.4275420236061));
#60385=CARTESIAN_POINT('Ctrl Pts',(1.63034498930106,-1.06847604194513,11.3607271826284));
#60386=CARTESIAN_POINT('Ctrl Pts',(1.59642695182921,-0.794772684000851,
11.2321128396658));
#60387=CARTESIAN_POINT('Ctrl Pts',(1.57333448035651,-0.636309800095196,
11.1805501678138));
#60388=CARTESIAN_POINT('Ctrl Pts',(1.55795451949656,-0.319434907277159,
11.1079876496958));
#60389=CARTESIAN_POINT('Ctrl Pts',(1.55794686674891,-0.158333333333332,
11.0877806504958));
#60390=CARTESIAN_POINT('Ctrl Pts',(1.57736811047979,0.158333333333334,11.0798704180037));
#60391=CARTESIAN_POINT('Ctrl Pts',(1.59558105644426,0.319434907277167,11.0927852508965));
#60392=CARTESIAN_POINT('Ctrl Pts',(1.65299749605388,0.636309800095206,11.1479762386669));
#60393=CARTESIAN_POINT('Ctrl Pts',(1.69824705110065,0.79477268400084,11.1900093036634));
#60394=CARTESIAN_POINT('Ctrl Pts',(1.77547688951519,1.06847604194556,11.3007258083824));
#60395=CARTESIAN_POINT('Ctrl Pts',(1.81145476612715,1.18514270861267,11.3594189182278));
#60396=CARTESIAN_POINT('Ctrl Pts',(1.8499805839489,1.30000000000132,11.4288800654763));
#60397=CARTESIAN_POINT('Ctrl Pts',(1.66462615833063,-1.30000000000005,11.5204313880076));
#60398=CARTESIAN_POINT('Ctrl Pts',(1.64753050462642,-1.18514270861181,11.4451970340025));
#60399=CARTESIAN_POINT('Ctrl Pts',(1.63187981906843,-1.06847604194513,11.3803258984653));
#60400=CARTESIAN_POINT('Ctrl Pts',(1.59906177000319,-0.794772684000852,
11.2544017057635));
#60401=CARTESIAN_POINT('Ctrl Pts',(1.57725211952697,-0.636309800095197,
11.2018237808047));
#60402=CARTESIAN_POINT('Ctrl Pts',(1.56158886062262,-0.319434907277159,
11.1293666304791));
#60403=CARTESIAN_POINT('Ctrl Pts',(1.55954130633869,-0.158333333333332,
11.1088058076973));
#60404=CARTESIAN_POINT('Ctrl Pts',(1.57840295787679,0.158333333333334,11.1010602390785));
#60405=CARTESIAN_POINT('Ctrl Pts',(1.5972639021225,0.319434907277166,11.114757650731));
#60406=CARTESIAN_POINT('Ctrl Pts',(1.65551914847726,0.636309800095205,11.169640744191));
#60407=CARTESIAN_POINT('Ctrl Pts',(1.7025183349984,0.794772684000841,11.2116827099241));
#60408=CARTESIAN_POINT('Ctrl Pts',(1.77903235823731,1.06847604194556,11.3196178795441));
#60409=CARTESIAN_POINT('Ctrl Pts',(1.81412006596867,1.18514270861267,11.3765231624912));
#60410=CARTESIAN_POINT('Ctrl Pts',(1.85117539589519,1.30000000000132,11.443612592849));
#60411=CARTESIAN_POINT('Ctrl Pts',(1.66400832169345,-1.30000000000005,11.5417962198323));
#60412=CARTESIAN_POINT('Ctrl Pts',(1.64758473327318,-1.18514270861181,11.4706865804745));
#60413=CARTESIAN_POINT('Ctrl Pts',(1.63272474774337,-1.06847604194513,11.4087476415573));
#60414=CARTESIAN_POINT('Ctrl Pts',(1.6020074439142,-0.79477268400085,11.2868424544265));
#60415=CARTESIAN_POINT('Ctrl Pts',(1.58263872436519,-0.636309800095197,
11.2327733254491));
#60416=CARTESIAN_POINT('Ctrl Pts',(1.56806146471367,-0.31943490727716,11.1601365165436));
#60417=CARTESIAN_POINT('Ctrl Pts',(1.5641448387696,-0.158333333333333,11.1387133277057));
#60418=CARTESIAN_POINT('Ctrl Pts',(1.58417746458293,0.158333333333335,11.1305334738137));
#60419=CARTESIAN_POINT('Ctrl Pts',(1.60670357041116,0.319434907277167,11.1444007366524));
#60420=CARTESIAN_POINT('Ctrl Pts',(1.66498469223539,0.636309800095207,11.199104875956));
#60421=CARTESIAN_POINT('Ctrl Pts',(1.7088475093535,0.794772684000842,11.2429825724483));
#60422=CARTESIAN_POINT('Ctrl Pts',(1.7829276416763,1.06847604194556,11.3471161791167));
#60423=CARTESIAN_POINT('Ctrl Pts',(1.81703219785438,1.18514270861267,11.4011998294516));
#60424=CARTESIAN_POINT('Ctrl Pts',(1.85317476586736,1.30000000000132,11.4642915503249));
#60425=CARTESIAN_POINT('Ctrl Pts',(1.66297539345541,-1.30000000000005,11.5661771710961));
#60426=CARTESIAN_POINT('Ctrl Pts',(1.64748790809536,-1.18514270861181,11.4995551871625));
#60427=CARTESIAN_POINT('Ctrl Pts',(1.63358502843746,-1.06847604194513,11.4408160710686));
#60428=CARTESIAN_POINT('Ctrl Pts',(1.60512735133741,-0.794772684000852,
11.323327963844));
#60429=CARTESIAN_POINT('Ctrl Pts',(1.58727693515927,-0.636309800095197,
11.2679265316481));
#60430=CARTESIAN_POINT('Ctrl Pts',(1.57496440665297,-0.319434907277159,
11.1947206572407));
#60431=CARTESIAN_POINT('Ctrl Pts',(1.57249846469125,-0.158333333333333,
11.1712285313312));
#60432=CARTESIAN_POINT('Ctrl Pts',(1.59315812681989,0.158333333333335,11.1628098713027));
#60433=CARTESIAN_POINT('Ctrl Pts',(1.61504264595899,0.319434907277168,11.1784122730249));
#60434=CARTESIAN_POINT('Ctrl Pts',(1.67196541936092,0.636309800095208,11.2333925388939));
#60435=CARTESIAN_POINT('Ctrl Pts',(1.71458559513429,0.794772684000841,11.278566366693));
#60436=CARTESIAN_POINT('Ctrl Pts',(1.78651169444565,1.06847604194556,11.3783610653472));
#60437=CARTESIAN_POINT('Ctrl Pts',(1.81958498585978,1.18514270861267,11.4293319290012));
#60438=CARTESIAN_POINT('Ctrl Pts',(1.85459742542072,1.30000000000132,11.4880762290198));
#60439=CARTESIAN_POINT('Ctrl Pts',(1.66253954923371,-1.30000000000004,11.5904501135859));
#60440=CARTESIAN_POINT('Ctrl Pts',(1.64716745471438,-1.18514270861181,11.5285960424193));
#60441=CARTESIAN_POINT('Ctrl Pts',(1.63366347314043,-1.06847604194513,11.4732599425887));
#60442=CARTESIAN_POINT('Ctrl Pts',(1.60678228886089,-0.794772684000851,
11.360480299733));
#60443=CARTESIAN_POINT('Ctrl Pts',(1.59123488997867,-0.636309800095198,
11.303586068394));
#60444=CARTESIAN_POINT('Ctrl Pts',(1.58077906844529,-0.31943490727716,11.2299960490128));
#60445=CARTESIAN_POINT('Ctrl Pts',(1.57850031280611,-0.158333333333333,
11.2048184941379));
#60446=CARTESIAN_POINT('Ctrl Pts',(1.60000105270369,0.158333333333335,11.1960984995114));
#60447=CARTESIAN_POINT('Ctrl Pts',(1.62296696905983,0.319434907277167,11.2129066633604));
#60448=CARTESIAN_POINT('Ctrl Pts',(1.67887545187121,0.636309800095208,11.2680205272578));
#60449=CARTESIAN_POINT('Ctrl Pts',(1.71900525567967,0.794772684000844,11.3148611545452));
#60450=CARTESIAN_POINT('Ctrl Pts',(1.78876603729209,1.06847604194556,11.4102050857618));
#60451=CARTESIAN_POINT('Ctrl Pts',(1.82100896742402,1.18514270861267,11.4579322183308));
#60452=CARTESIAN_POINT('Ctrl Pts',(1.85529797021952,1.30000000000131,11.512115628486));
#60453=CARTESIAN_POINT('Ctrl Pts',(1.66047989040796,-1.30000000000004,11.6120422433131));
#60454=CARTESIAN_POINT('Ctrl Pts',(1.6454766653493,-1.18514270861181,11.554246150656));
#60455=CARTESIAN_POINT('Ctrl Pts',(1.63249668632829,-1.06847604194513,11.5018119048232));
#60456=CARTESIAN_POINT('Ctrl Pts',(1.60718444124979,-0.794772684000848,
11.3930652463123));
#60457=CARTESIAN_POINT('Ctrl Pts',(1.59326532192798,-0.636309800095197,
11.3349913012082));
#60458=CARTESIAN_POINT('Ctrl Pts',(1.58467614588915,-0.31943490727716,11.2610090519529));
#60459=CARTESIAN_POINT('Ctrl Pts',(1.58342008565865,-0.158333333333332,
11.2341227576192));
#60460=CARTESIAN_POINT('Ctrl Pts',(1.60539226152046,0.158333333333335,11.2252470755727));
#60461=CARTESIAN_POINT('Ctrl Pts',(1.62765787597471,0.319434907277167,11.2436246555957));
#60462=CARTESIAN_POINT('Ctrl Pts',(1.6829635831606,0.636309800095207,11.2987802927372));
#60463=CARTESIAN_POINT('Ctrl Pts',(1.72303227090909,0.794772684000842,11.3464031280536));
#60464=CARTESIAN_POINT('Ctrl Pts',(1.79157743098819,1.06847604194556,11.4376927581495));
#60465=CARTESIAN_POINT('Ctrl Pts',(1.82309787132108,1.18514270861267,11.4826159445079));
#60466=CARTESIAN_POINT('Ctrl Pts',(1.85646809203706,1.30000000000131,11.5329464189705));
#60467=CARTESIAN_POINT('Ctrl Pts',(1.65917440129577,-1.30000000000004,11.6304388748568));
#60468=CARTESIAN_POINT('Ctrl Pts',(1.64420105650356,-1.18514270861181,11.5762004678021));
#60469=CARTESIAN_POINT('Ctrl Pts',(1.63143500502946,-1.06847604194513,11.5263218385257));
#60470=CARTESIAN_POINT('Ctrl Pts',(1.60704216141674,-0.794772684000848,
11.4211641855496));
#60471=CARTESIAN_POINT('Ctrl Pts',(1.59424465224217,-0.636309800095196,
11.362178575418));
#60472=CARTESIAN_POINT('Ctrl Pts',(1.58736265267558,-0.319434907277159,
11.2878467698504));
#60473=CARTESIAN_POINT('Ctrl Pts',(1.58756458885484,-0.158333333333332,
11.259339331069));
#60474=CARTESIAN_POINT('Ctrl Pts',(1.61015009976414,0.158333333333334,11.2502671569896));
#60475=CARTESIAN_POINT('Ctrl Pts',(1.63190827410841,0.319434907277167,11.2699434288937));
#60476=CARTESIAN_POINT('Ctrl Pts',(1.68606922874198,0.636309800095207,11.3253049547619));
#60477=CARTESIAN_POINT('Ctrl Pts',(1.72461091140695,0.794772684000842,11.374034284718));
#60478=CARTESIAN_POINT('Ctrl Pts',(1.7920431619667,1.06847604194556,11.4618498796299));
#60479=CARTESIAN_POINT('Ctrl Pts',(1.82324641542261,1.18514270861266,11.5042689079887));
#60480=CARTESIAN_POINT('Ctrl Pts',(1.8564639996782,1.30000000000131,11.5510948475572));
#60481=CARTESIAN_POINT('Ctrl Pts',(1.65825661873328,-1.30000000000005,11.6457250585537));
#60482=CARTESIAN_POINT('Ctrl Pts',(1.64381244552155,-1.18514270861181,11.5943362651268));
#60483=CARTESIAN_POINT('Ctrl Pts',(1.63149135558789,-1.06847604194513,11.5465257061246));
#60484=CARTESIAN_POINT('Ctrl Pts',(1.60793192010925,-0.794772684000851,
11.4443401877041));
#60485=CARTESIAN_POINT('Ctrl Pts',(1.59534912366149,-0.636309800095197,
11.3847350317333));
#60486=CARTESIAN_POINT('Ctrl Pts',(1.58905040871725,-0.319434907277159,
11.3103362650791));
#60487=CARTESIAN_POINT('Ctrl Pts',(1.58958601175429,-0.158333333333333,
11.2807547785508));
#60488=CARTESIAN_POINT('Ctrl Pts',(1.61247567219755,0.158333333333335,11.2715894287578));
#60489=CARTESIAN_POINT('Ctrl Pts',(1.63424089574764,0.319434907277168,11.2922306293025));
#60490=CARTESIAN_POINT('Ctrl Pts',(1.68836361307204,0.636309800095207,11.3475017995811));
#60491=CARTESIAN_POINT('Ctrl Pts',(1.72701439575528,0.794772684000843,11.3967473603989));
#60492=CARTESIAN_POINT('Ctrl Pts',(1.79381277498766,1.06847604194556,11.4815812537823));
#60493=CARTESIAN_POINT('Ctrl Pts',(1.82458463182755,1.18514270861266,11.5219615759282));
#60494=CARTESIAN_POINT('Ctrl Pts',(1.85721380226146,1.30000000000131,11.5660007711799));
#60495=CARTESIAN_POINT('Ctrl Pts',(1.65692536543948,-1.30000000000004,11.6580787419226));
#60496=CARTESIAN_POINT('Ctrl Pts',(1.64220899771378,-1.18514270861181,11.6091207818142));
#60497=CARTESIAN_POINT('Ctrl Pts',(1.62982954970193,-1.06847604194513,11.5630568054575));
#60498=CARTESIAN_POINT('Ctrl Pts',(1.6066293003326,-0.794772684000852,11.463325486413));
#60499=CARTESIAN_POINT('Ctrl Pts',(1.59503084689484,-0.636309800095197,
11.4030703960431));
#60500=CARTESIAN_POINT('Ctrl Pts',(1.58976206576291,-0.319434907277159,
11.3284945702936));
#60501=CARTESIAN_POINT('Ctrl Pts',(1.59087843016237,-0.158333333333333,
11.2979672191158));
#60502=CARTESIAN_POINT('Ctrl Pts',(1.61436971205319,0.158333333333335,11.2886305261183));
#60503=CARTESIAN_POINT('Ctrl Pts',(1.63641500674446,0.319434907277168,11.3099564531826));
#60504=CARTESIAN_POINT('Ctrl Pts',(1.6902052555697,0.636309800095208,11.3652385745838));
#60505=CARTESIAN_POINT('Ctrl Pts',(1.72785782392614,0.794772684000843,11.415205044039));
#60506=CARTESIAN_POINT('Ctrl Pts',(1.79409927768552,1.06847604194556,11.4976721140785));
#60507=CARTESIAN_POINT('Ctrl Pts',(1.82473409501747,1.18514270861266,11.5363655582635));
#60508=CARTESIAN_POINT('Ctrl Pts',(1.85733025883666,1.30000000000131,11.5780555077196));
#60509=CARTESIAN_POINT('Ctrl Pts',(1.65574912520358,-1.30000000000004,11.6703942470278));
#60510=CARTESIAN_POINT('Ctrl Pts',(1.6407031272259,-1.18514270861181,11.6238751238318));
#60511=CARTESIAN_POINT('Ctrl Pts',(1.62825119945876,-1.06847604194513,11.5795576353598));
#60512=CARTESIAN_POINT('Ctrl Pts',(1.60547757644532,-0.794772684000851,
11.4822615879543));
#60513=CARTESIAN_POINT('Ctrl Pts',(1.59514663822623,-0.636309800095197,
11.421295595551));
#60514=CARTESIAN_POINT('Ctrl Pts',(1.59093997819171,-0.319434907277159,
11.3465383751006));
#60515=CARTESIAN_POINT('Ctrl Pts',(1.5926049519623,-0.158333333333333,11.3150659952534));
#60516=CARTESIAN_POINT('Ctrl Pts',(1.61628845463705,0.158333333333335,11.3056729345733));
#60517=CARTESIAN_POINT('Ctrl Pts',(1.63790215909678,0.319434907277169,11.327890922621));
#60518=CARTESIAN_POINT('Ctrl Pts',(1.69117500705595,0.636309800095208,11.3832326962634));
#60519=CARTESIAN_POINT('Ctrl Pts',(1.72848079306108,0.794772684000844,11.4337256827248));
#60520=CARTESIAN_POINT('Ctrl Pts',(1.79407775002516,1.06847604194556,11.5138447056087));
#60521=CARTESIAN_POINT('Ctrl Pts',(1.82441011941276,1.18514270861266,11.5508964676374));
#60522=CARTESIAN_POINT('Ctrl Pts',(1.85668036612498,1.30000000000131,11.5903194353906));
#60523=CARTESIAN_POINT('Ctrl Pts',(1.65199738732143,-1.30000000000004,11.704362262037));
#60524=CARTESIAN_POINT('Ctrl Pts',(1.6378062771533,-1.18514270861181,11.6641808214006));
#60525=CARTESIAN_POINT('Ctrl Pts',(1.62616635359825,-1.06847604194513,11.6244530030084));
#60526=CARTESIAN_POINT('Ctrl Pts',(1.60516955306668,-0.79477268400085,11.5337217531304));
#60527=CARTESIAN_POINT('Ctrl Pts',(1.59592366447477,-0.636309800095196,
11.471274853242));
#60528=CARTESIAN_POINT('Ctrl Pts',(1.59311075487144,-0.319434907277158,
11.3963705904157));
#60529=CARTESIAN_POINT('Ctrl Pts',(1.59515399903155,-0.158333333333332,
11.3626387070737));
#60530=CARTESIAN_POINT('Ctrl Pts',(1.61956472506171,0.158333333333334,11.3530266873265));
#60531=CARTESIAN_POINT('Ctrl Pts',(1.64148739776061,0.319434907277168,11.377265724066));
#60532=CARTESIAN_POINT('Ctrl Pts',(1.69492924291113,0.636309800095207,11.4323482476407));
#60533=CARTESIAN_POINT('Ctrl Pts',(1.73248328685883,0.794772684000842,11.4840051515948));
#60534=CARTESIAN_POINT('Ctrl Pts',(1.79698535281222,1.06847604194556,11.5574998117437));
#60535=CARTESIAN_POINT('Ctrl Pts',(1.82653771960054,1.18514270861266,11.5900247156801));
#60536=CARTESIAN_POINT('Ctrl Pts',(1.85772189886299,1.3000000000013,11.62326140842));
#60537=CARTESIAN_POINT('Ctrl Pts',(1.64649643543192,-1.30000000000004,11.7416097712608));
#60538=CARTESIAN_POINT('Ctrl Pts',(1.63060661304912,-1.1851427086118,11.7088267957282));
#60539=CARTESIAN_POINT('Ctrl Pts',(1.61824802687329,-1.06847604194512,11.6744099857127));
#60540=CARTESIAN_POINT('Ctrl Pts',(1.59785508253992,-0.794772684000845,
11.5911257850145));
#60541=CARTESIAN_POINT('Ctrl Pts',(1.5926968241364,-0.636309800095194,11.5266070008333));
#60542=CARTESIAN_POINT('Ctrl Pts',(1.59311422876906,-0.319434907277159,
11.4512484604098));
#60543=CARTESIAN_POINT('Ctrl Pts',(1.59670845495764,-0.158333333333332,
11.4147734770359));
#60544=CARTESIAN_POINT('Ctrl Pts',(1.62223794910294,0.158333333333334,11.4048930759665));
#60545=CARTESIAN_POINT('Ctrl Pts',(1.64405960030171,0.319434907277165,11.4314759978575));
#60546=CARTESIAN_POINT('Ctrl Pts',(1.69587536621376,0.636309800095204,11.4867326241377));
#60547=CARTESIAN_POINT('Ctrl Pts',(1.73004745102725,0.79477268400084,11.5405226830685));
#60548=CARTESIAN_POINT('Ctrl Pts',(1.79369763209872,1.06847604194556,11.606703417957));
#60549=CARTESIAN_POINT('Ctrl Pts',(1.82351106461192,1.18514270861266,11.6340200566103));
#60550=CARTESIAN_POINT('Ctrl Pts',(1.85558612472409,1.3000000000013,11.6600061460216));
#60551=CARTESIAN_POINT('Ctrl Pts',(1.64172822170271,-1.30000000000004,11.7786863448143));
#60552=CARTESIAN_POINT('Ctrl Pts',(1.62575513936202,-1.1851427086118,11.7529906415876));
#60553=CARTESIAN_POINT('Ctrl Pts',(1.6134054477271,-1.06847604194512,11.7237453000575));
#60554=CARTESIAN_POINT('Ctrl Pts',(1.59324594689023,-0.794772684000844,
11.6479823360285));
#60555=CARTESIAN_POINT('Ctrl Pts',(1.58810131644293,-0.636309800095194,
11.5821626800989));
#60556=CARTESIAN_POINT('Ctrl Pts',(1.58994436496101,-0.319434907277158,
11.5067370957953));
#60557=CARTESIAN_POINT('Ctrl Pts',(1.59579155076718,-0.158333333333332,
11.4674554470401));
#60558=CARTESIAN_POINT('Ctrl Pts',(1.62204300194924,0.158333333333334,11.4574151571969));
#60559=CARTESIAN_POINT('Ctrl Pts',(1.64236886504219,0.319434907277165,11.4866258555787));
#60560=CARTESIAN_POINT('Ctrl Pts',(1.69415783221999,0.636309800095203,11.5416625456892));
#60561=CARTESIAN_POINT('Ctrl Pts',(1.72953400768076,0.794772684000838,11.5964997079218));
#60562=CARTESIAN_POINT('Ctrl Pts',(1.79311454461587,1.06847604194556,11.6551995377656));
#60563=CARTESIAN_POINT('Ctrl Pts',(1.82265133069952,1.18514270861266,11.6774486937642));
#60564=CARTESIAN_POINT('Ctrl Pts',(1.85420324431865,1.30000000000131,11.6965380244651));
#60565=CARTESIAN_POINT('Ctrl Pts',(1.63779021696461,-1.30000000000003,11.8035075973253));
#60566=CARTESIAN_POINT('Ctrl Pts',(1.62058710253557,-1.1851427086118,11.7827369798234));
#60567=CARTESIAN_POINT('Ctrl Pts',(1.60761419841532,-1.06847604194512,11.7570469303984));
#60568=CARTESIAN_POINT('Ctrl Pts',(1.58741682674095,-0.794772684000843,
11.6863329050787));
#60569=CARTESIAN_POINT('Ctrl Pts',(1.58451908111622,-0.636309800095193,
11.6192608085749));
#60570=CARTESIAN_POINT('Ctrl Pts',(1.58800279136641,-0.319434907277159,
11.5436880101914));
#60571=CARTESIAN_POINT('Ctrl Pts',(1.5945687098384,-0.158333333333331,11.502703946869));
#60572=CARTESIAN_POINT('Ctrl Pts',(1.62157218186044,0.158333333333334,11.4925040044064));
#60573=CARTESIAN_POINT('Ctrl Pts',(1.64210579695489,0.319434907277164,11.5231920863286));
#60574=CARTESIAN_POINT('Ctrl Pts',(1.69343054444979,0.636309800095202,11.5781839607371));
#60575=CARTESIAN_POINT('Ctrl Pts',(1.72737668125019,0.794772684000839,11.6342229988072));
#60576=CARTESIAN_POINT('Ctrl Pts',(1.7906744665107,1.06847604194556,11.6879901617425));
#60577=CARTESIAN_POINT('Ctrl Pts',(1.8203501553843,1.18514270861266,11.7067887653584));
#60578=CARTESIAN_POINT('Ctrl Pts',(1.85230226730626,1.30000000000131,11.7211121600253));
#60579=CARTESIAN_POINT('Ctrl Pts',(1.63206766705696,-1.30000000000004,11.8346752939481));
#60580=CARTESIAN_POINT('Ctrl Pts',(1.61435973387503,-1.18514270861181,11.8198546331378));
#60581=CARTESIAN_POINT('Ctrl Pts',(1.60115205248425,-1.06847604194513,11.7984963698485));
#60582=CARTESIAN_POINT('Ctrl Pts',(1.58103614819377,-0.794772684000846,
11.7340513393747));
#60583=CARTESIAN_POINT('Ctrl Pts',(1.57905152455074,-0.636309800095194,
11.6657577606432));
#60584=CARTESIAN_POINT('Ctrl Pts',(1.58365486389055,-0.319434907277158,
11.5901827399508));
#60585=CARTESIAN_POINT('Ctrl Pts',(1.59110326196349,-0.158333333333332,
11.5470991950029));
#60586=CARTESIAN_POINT('Ctrl Pts',(1.61887637191083,0.158333333333334,11.536748396219));
#60587=CARTESIAN_POINT('Ctrl Pts',(1.63951288335966,0.319434907277167,11.5693233003321));
#60588=CARTESIAN_POINT('Ctrl Pts',(1.69084625596948,0.636309800095205,11.6241360020771));
#60589=CARTESIAN_POINT('Ctrl Pts',(1.72416805543662,0.794772684000839,11.6814128995574));
#60590=CARTESIAN_POINT('Ctrl Pts',(1.78767359202545,1.06847604194556,11.7289080614217));
#60591=CARTESIAN_POINT('Ctrl Pts',(1.81760534753292,1.18514270861266,11.7433876662583));
#60592=CARTESIAN_POINT('Ctrl Pts',(1.84997966487054,1.30000000000131,11.7517879802295));
#60593=CARTESIAN_POINT('Ctrl Pts',(1.62757496106193,-1.30000000000004,11.8610434436437));
#60594=CARTESIAN_POINT('Ctrl Pts',(1.60890493030257,-1.18514270861181,11.8513624255336));
#60595=CARTESIAN_POINT('Ctrl Pts',(1.59508081426732,-1.06847604194513,11.8337526333206));
#60596=CARTESIAN_POINT('Ctrl Pts',(1.57433937315554,-0.794772684000849,
11.7747534361581));
#60597=CARTESIAN_POINT('Ctrl Pts',(1.57280459694369,-0.636309800095195,
11.7054903069103));
#60598=CARTESIAN_POINT('Ctrl Pts',(1.57862731462552,-0.319434907277158,
11.6298804413981));
#60599=CARTESIAN_POINT('Ctrl Pts',(1.58783877253507,-0.158333333333332,
11.5848469494164));
#60600=CARTESIAN_POINT('Ctrl Pts',(1.616612712653,0.158333333333334,11.5743201399577));
#60601=CARTESIAN_POINT('Ctrl Pts',(1.63696911563611,0.319434907277164,11.6085667153463));
#60602=CARTESIAN_POINT('Ctrl Pts',(1.68813968272809,0.636309800095203,11.6632640474509));
#60603=CARTESIAN_POINT('Ctrl Pts',(1.72074210362639,0.794772684000839,11.721627553831));
#60604=CARTESIAN_POINT('Ctrl Pts',(1.7845030729319,1.06847604194556,11.7637824585709));
#60605=CARTESIAN_POINT('Ctrl Pts',(1.81475743751615,1.18514270861266,11.7745746641525));
#60606=CARTESIAN_POINT('Ctrl Pts',(1.84766640564899,1.30000000000131,11.7779117790467));
#60607=CARTESIAN_POINT('Ctrl Pts',(1.62446161102719,-1.30000000000004,11.8766283155242));
#60608=CARTESIAN_POINT('Ctrl Pts',(1.60517405537136,-1.18514270861181,11.8699722209449));
#60609=CARTESIAN_POINT('Ctrl Pts',(1.5909861623095,-1.06847604194513,11.8545628836417));
#60610=CARTESIAN_POINT('Ctrl Pts',(1.56999053183438,-0.794772684000848,
11.7987424900714));
#60611=CARTESIAN_POINT('Ctrl Pts',(1.56902003450696,-0.636309800095197,
11.7288624901258));
#60612=CARTESIAN_POINT('Ctrl Pts',(1.5757349176515,-0.31943490727716,11.6532066521009));
#60613=CARTESIAN_POINT('Ctrl Pts',(1.5861166141376,-0.158333333333332,11.6070056598578));
#60614=CARTESIAN_POINT('Ctrl Pts',(1.61521019215178,0.158333333333334,11.5964305482167));
#60615=CARTESIAN_POINT('Ctrl Pts',(1.63483676436541,0.319434907277165,11.6317671668772));
#60616=CARTESIAN_POINT('Ctrl Pts',(1.68552024576209,0.636309800095204,11.6864714696696));
#60617=CARTESIAN_POINT('Ctrl Pts',(1.7174936154201,0.794772684000843,11.7455132932636));
#60618=CARTESIAN_POINT('Ctrl Pts',(1.7816632929437,1.06847604194556,11.7844768543231));
#60619=CARTESIAN_POINT('Ctrl Pts',(1.81235488861359,1.18514270861267,11.7930523385357));
#60620=CARTESIAN_POINT('Ctrl Pts',(1.84596140427423,1.30000000000131,11.7933374251206));
#60621=CARTESIAN_POINT('Ctrl Pts',(1.62325910326905,-1.30000000000004,11.8828532156717));
#60622=CARTESIAN_POINT('Ctrl Pts',(1.60375087733459,-1.18514270861181,11.8774021306647));
#60623=CARTESIAN_POINT('Ctrl Pts',(1.5894276312557,-1.06847604194513,11.8628709907803));
#60624=CARTESIAN_POINT('Ctrl Pts',(1.56831640817595,-0.794772684000848,
11.8083244074774));
#60625=CARTESIAN_POINT('Ctrl Pts',(1.5674992324408,-0.636309800095196,11.7382106430618));
#60626=CARTESIAN_POINT('Ctrl Pts',(1.57451847326436,-0.31943490727716,11.662546109776));
#60627=CARTESIAN_POINT('Ctrl Pts',(1.58531440897992,-0.158333333333332,
11.6158888448209));
#60628=CARTESIAN_POINT('Ctrl Pts',(1.6145903331477,0.158333333333334,11.6052837860805));
#60629=CARTESIAN_POINT('Ctrl Pts',(1.63407113660023,0.319434907277164,11.6410280219121));
#60630=CARTESIAN_POINT('Ctrl Pts',(1.6846462572754,0.636309800095204,11.6957181276293));
#60631=CARTESIAN_POINT('Ctrl Pts',(1.71638682467756,0.794772684000842,11.7550267856039));
#60632=CARTESIAN_POINT('Ctrl Pts',(1.78067425165386,1.06847604194556,11.7927235360901));
#60633=CARTESIAN_POINT('Ctrl Pts',(1.81149866824387,1.18514270861266,11.8004212359001));
#60634=CARTESIAN_POINT('Ctrl Pts',(1.84531985636975,1.30000000000131,11.799499109037));
#60635=CARTESIAN_POINT('Ctrl Pts',(1.61932560970724,-1.30000000000004,11.9000572296304));
#60636=CARTESIAN_POINT('Ctrl Pts',(1.59863734714343,-1.18514270861181,11.8979988143724));
#60637=CARTESIAN_POINT('Ctrl Pts',(1.58368072051496,-1.06847604194513,11.8859178751391));
#60638=CARTESIAN_POINT('Ctrl Pts',(1.56236914656071,-0.794772684000847,
11.8348544533447));
#60639=CARTESIAN_POINT('Ctrl Pts',(1.56359939056409,-0.636309800095195,
11.7638599559));
#60640=CARTESIAN_POINT('Ctrl Pts',(1.57168045445783,-0.319434907277159,
11.6881522006818));
#60641=CARTESIAN_POINT('Ctrl Pts',(1.58250539610576,-0.158333333333332,
11.6404302732981));
#60642=CARTESIAN_POINT('Ctrl Pts',(1.61222232235546,0.158333333333334,11.629751579368));
#60643=CARTESIAN_POINT('Ctrl Pts',(1.63182988702215,0.319434907277165,11.6665211023994));
#60644=CARTESIAN_POINT('Ctrl Pts',(1.68282247714058,0.636309800095204,11.7210346553957));
#60645=CARTESIAN_POINT('Ctrl Pts',(1.71492005119327,0.79477268400084,11.7808809201514));
#60646=CARTESIAN_POINT('Ctrl Pts',(1.77944618880968,1.06847604194556,11.8151101249152));
#60647=CARTESIAN_POINT('Ctrl Pts',(1.81031592086132,1.18514270861266,11.8204561758092));
#60648=CARTESIAN_POINT('Ctrl Pts',(1.84412441091943,1.30000000000131,11.816331723172));
#60649=CARTESIAN_POINT('Ctrl Pts',(1.61514176393842,-1.30000000000004,11.9218149414855));
#60650=CARTESIAN_POINT('Ctrl Pts',(1.59369237945656,-1.18514270861181,11.9239622185499));
#60651=CARTESIAN_POINT('Ctrl Pts',(1.57817340785515,-1.06847604194512,11.9149610364403));
#60652=CARTESIAN_POINT('Ctrl Pts',(1.55602191902508,-0.794772684000845,
11.8684113341534));
#60653=CARTESIAN_POINT('Ctrl Pts',(1.5570312496809,-0.636309800095196,11.7967058631063));
#60654=CARTESIAN_POINT('Ctrl Pts',(1.56568570948374,-0.31943490727716,11.7210616480371));
#60655=CARTESIAN_POINT('Ctrl Pts',(1.57799472897679,-0.158333333333332,
11.6717765646414));
#60656=CARTESIAN_POINT('Ctrl Pts',(1.60825236528344,0.158333333333334,11.6610301361501));
#60657=CARTESIAN_POINT('Ctrl Pts',(1.62744678734947,0.319434907277165,11.6992035717281));
#60658=CARTESIAN_POINT('Ctrl Pts',(1.6778873384829,0.636309800095204,11.7537020112002));
#60659=CARTESIAN_POINT('Ctrl Pts',(1.70847024371082,0.794772684000842,11.814605530805));
#60660=CARTESIAN_POINT('Ctrl Pts',(1.77391916968909,1.06847604194556,11.8443178419405));
#60661=CARTESIAN_POINT('Ctrl Pts',(1.80574027615595,1.18514270861267,11.8465100349315));
#60662=CARTESIAN_POINT('Ctrl Pts',(1.84105207415533,1.30000000000131,11.8380330623724));
#60663=CARTESIAN_POINT('Ctrl Pts',(1.60783404495285,-1.30000000000004,11.9530476574059));
#60664=CARTESIAN_POINT('Ctrl Pts',(1.58426159374155,-1.18514270861181,11.9613249468198));
#60665=CARTESIAN_POINT('Ctrl Pts',(1.56744492513183,-1.06847604194513,11.9567777659226));
#60666=CARTESIAN_POINT('Ctrl Pts',(1.54420226577969,-0.794772684000849,
11.9166457764448));
#60667=CARTESIAN_POINT('Ctrl Pts',(1.54733643364015,-0.636309800095195,
11.8436015159348));
#60668=CARTESIAN_POINT('Ctrl Pts',(1.55773531862725,-0.319434907277158,
11.7679317466498));
#60669=CARTESIAN_POINT('Ctrl Pts',(1.57160625154768,-0.158333333333332,
11.7165083827316));
#60670=CARTESIAN_POINT('Ctrl Pts',(1.60266798886658,0.158333333333334,11.7056600071616));
#60671=CARTESIAN_POINT('Ctrl Pts',(1.62083885672664,0.319434907277168,11.7459022467507));
#60672=CARTESIAN_POINT('Ctrl Pts',(1.67171417543449,0.636309800095206,11.8001524413723));
#60673=CARTESIAN_POINT('Ctrl Pts',(1.7034077465642,0.794772684000839,11.8619602905416));
#60674=CARTESIAN_POINT('Ctrl Pts',(1.76966641057741,1.06847604194556,11.8853447403049));
#60675=CARTESIAN_POINT('Ctrl Pts',(1.8017577243743,1.18514270861266,11.8832530437335));
#60676=CARTESIAN_POINT('Ctrl Pts',(1.83725943144218,1.30000000000131,11.8689473887673));
#60677=CARTESIAN_POINT('Ctrl Pts',(1.60362879054004,-1.30000000000005,11.9717350649118));
#60678=CARTESIAN_POINT('Ctrl Pts',(1.57888716168168,-1.18514270861182,11.9836612254861));
#60679=CARTESIAN_POINT('Ctrl Pts',(1.56131753260336,-1.06847604194513,11.981772259511));
#60680=CARTESIAN_POINT('Ctrl Pts',(1.53729692888577,-0.794772684000851,
11.9454926641869));
#60681=CARTESIAN_POINT('Ctrl Pts',(1.54134412420084,-0.636309800095197,
11.8716953287081));
#60682=CARTESIAN_POINT('Ctrl Pts',(1.55242668622773,-0.319434907277159,
11.796066796982));
#60683=CARTESIAN_POINT('Ctrl Pts',(1.56691293504717,-0.158333333333332,
11.7434227014676));
#60684=CARTESIAN_POINT('Ctrl Pts',(1.59850372070212,0.158333333333334,11.7325116687194));
#60685=CARTESIAN_POINT('Ctrl Pts',(1.6169412386113,0.319434907277167,11.7738468098411));
#60686=CARTESIAN_POINT('Ctrl Pts',(1.66749164588227,0.636309800095206,11.8280608912181));
#60687=CARTESIAN_POINT('Ctrl Pts',(1.69739655218748,0.79477268400084,11.8908575699105));
#60688=CARTESIAN_POINT('Ctrl Pts',(1.76461391978401,1.06847604194556,11.9103538108361));
#60689=CARTESIAN_POINT('Ctrl Pts',(1.79771081767218,1.18514270861267,11.9055342229517));
#60690=CARTESIAN_POINT('Ctrl Pts',(1.83480870566485,1.30000000000132,11.8874558468933));
#60691=CARTESIAN_POINT('Ctrl Pts',(1.600345881349,-1.30000000000005,11.9842630921627));
#60692=CARTESIAN_POINT('Ctrl Pts',(1.57504122138965,-1.18514270861182,11.9985854052829));
#60693=CARTESIAN_POINT('Ctrl Pts',(1.55708435379925,-1.06847604194513,11.9984485537176));
#60694=CARTESIAN_POINT('Ctrl Pts',(1.53257526769946,-0.794772684000851,
11.9647288362548));
#60695=CARTESIAN_POINT('Ctrl Pts',(1.53670704324099,-0.636309800095197,
11.8905067546537));
#60696=CARTESIAN_POINT('Ctrl Pts',(1.54831342142086,-0.319434907277159,
11.8149010785834));
#60697=CARTESIAN_POINT('Ctrl Pts',(1.56375557866725,-0.158333333333332,
11.7613725996759));
#60698=CARTESIAN_POINT('Ctrl Pts',(1.59581317861656,0.158333333333334,11.7504080900329));
#60699=CARTESIAN_POINT('Ctrl Pts',(1.61390936643398,0.319434907277167,11.7925524285043));
#60700=CARTESIAN_POINT('Ctrl Pts',(1.66458583994602,0.636309800095206,11.8466789456142));
#60701=CARTESIAN_POINT('Ctrl Pts',(1.69463294550622,0.79477268400084,11.9098917520947));
#60702=CARTESIAN_POINT('Ctrl Pts',(1.76226517728142,1.06847604194556,11.9268506192697));
#60703=CARTESIAN_POINT('Ctrl Pts',(1.79559295568807,1.18514270861267,11.9203016847132));
#60704=CARTESIAN_POINT('Ctrl Pts',(1.83297302538702,1.30000000000132,11.899862950388));
#60705=CARTESIAN_POINT('',(1.81631379076882,1.2,11.8047262908302));
#60706=CARTESIAN_POINT('Ctrl Pts',(1.81631379076882,1.2,11.8047262908302));
#60707=CARTESIAN_POINT('Ctrl Pts',(1.81954172329026,1.20865297781299,11.7941512478302));
#60708=CARTESIAN_POINT('Ctrl Pts',(1.82334800037714,1.21707870846838,11.783575657389));
#60709=CARTESIAN_POINT('Ctrl Pts',(1.83010849452505,1.23366298102073,11.7630163352366));
#60710=CARTESIAN_POINT('Ctrl Pts',(1.83359564288739,1.24271606614613,11.7518564645226));
#60711=CARTESIAN_POINT('Ctrl Pts',(1.84611908787067,1.27553627908762,11.7113941521115));
#60712=CARTESIAN_POINT('Ctrl Pts',(1.84915634495443,1.28315372901467,11.701886753377));
#60713=CARTESIAN_POINT('Ctrl Pts',(1.85479302522287,1.30000000000131,11.6813215498971));
#60714=CARTESIAN_POINT('',(1.66957759488823,0.653834841417358,11.8599367650635));
#60715=CARTESIAN_POINT('Ctrl Pts',(1.66957759489952,0.653834841416676,11.859936765087));
#60716=CARTESIAN_POINT('Ctrl Pts',(1.68494198314014,0.71815705809227,11.8544319611253));
#60717=CARTESIAN_POINT('Ctrl Pts',(1.69640604766083,0.760168978913057,11.850270842599));
#60718=CARTESIAN_POINT('Ctrl Pts',(1.74570835223144,0.949887649636558,11.8320857710676));
#60719=CARTESIAN_POINT('Ctrl Pts',(1.78038525555478,1.07519041108246,11.8188981416352));
#60720=CARTESIAN_POINT('Ctrl Pts',(1.81631379076882,1.2,11.8047262908302));
#60721=CARTESIAN_POINT('',(1.53759581372214,-0.653834841531101,11.9051353980119));
#60722=CARTESIAN_POINT('Ctrl Pts',(1.53759581372214,-0.653834841531122,
11.9051353980119));
#60723=CARTESIAN_POINT('Ctrl Pts',(1.54252926752756,-0.57592707476385,11.8638270643046));
#60724=CARTESIAN_POINT('Ctrl Pts',(1.54744292193318,-0.493582421500596,
11.8290212458167));
#60725=CARTESIAN_POINT('Ctrl Pts',(1.55695050923341,-0.338052012707416,
11.7793054455627));
#60726=CARTESIAN_POINT('Ctrl Pts',(1.5615223834955,-0.265565628467728,11.7620037496986));
#60727=CARTESIAN_POINT('Ctrl Pts',(1.571794384339,-0.129646434571565,11.7398984122046));
#60728=CARTESIAN_POINT('Ctrl Pts',(1.57720257787791,-0.0665942542479303,
11.7336412316907));
#60729=CARTESIAN_POINT('Ctrl Pts',(1.58968469190397,0.0595028577922644,
11.7289735009213));
#60730=CARTESIAN_POINT('Ctrl Pts',(1.59684561072502,0.122699779224089,11.7305123643919));
#60731=CARTESIAN_POINT('Ctrl Pts',(1.61358182914933,0.260014810575644,11.7427412035281));
#60732=CARTESIAN_POINT('Ctrl Pts',(1.62336779242219,0.333833648164222,11.755055690296));
#60733=CARTESIAN_POINT('Ctrl Pts',(1.64505548717876,0.49116691886655,11.7943182041769));
#60734=CARTESIAN_POINT('Ctrl Pts',(1.65719828911254,0.574146030768171,11.823374616898));
#60735=CARTESIAN_POINT('Ctrl Pts',(1.66957759491099,0.653834841429009,11.8599367650304));
#60736=CARTESIAN_POINT('',(1.60613120890469,-1.2,11.8821835226508));
#60737=CARTESIAN_POINT('Ctrl Pts',(1.60613120890469,-1.2,11.8821835226508));
#60738=CARTESIAN_POINT('Ctrl Pts',(1.58809120755403,-1.09919977191309,11.8883717912306));
#60739=CARTESIAN_POINT('Ctrl Pts',(1.57551018723902,-1.0108368422167,11.8925996120367));
#60740=CARTESIAN_POINT('Ctrl Pts',(1.54791748959699,-0.787234072051788,
11.9017710545491));
#60741=CARTESIAN_POINT('Ctrl Pts',(1.5438100803565,-0.741256752224837,11.9031046317205));
#60742=CARTESIAN_POINT('Ctrl Pts',(1.53759581372215,-0.6538348415311,11.9051353980119));
#60743=CARTESIAN_POINT('Ctrl Pts',(1.64376583932815,-1.3,11.7629523189989));
#60744=CARTESIAN_POINT('Ctrl Pts',(1.63817081442155,-1.28288489407424,11.7831596690008));
#60745=CARTESIAN_POINT('Ctrl Pts',(1.63165744768168,-1.26605460703988,11.8033441571198));
#60746=CARTESIAN_POINT('Ctrl Pts',(1.62182860196257,-1.23991764288754,11.834504145476));
#60747=CARTESIAN_POINT('Ctrl Pts',(1.61939946340474,-1.23326875145929,11.8423946820282));
#60748=CARTESIAN_POINT('Ctrl Pts',(1.61100387997911,-1.21129319797848,11.8685758706849));
#60749=CARTESIAN_POINT('Ctrl Pts',(1.60993145974154,-1.20847825033892,11.8719167228947));
#60750=CARTESIAN_POINT('Ctrl Pts',(1.60613120890469,-1.2,11.8821835226508));
#60751=CARTESIAN_POINT('Origin',(0.,1.25,7.2));
#60752=CARTESIAN_POINT('Origin',(0.,1.2,7.2));
#60753=CARTESIAN_POINT('Origin',(0.,1.25,7.2));
#60754=CARTESIAN_POINT('',(1.45281637513429,1.20000000016485,11.9320000612277));
#60755=CARTESIAN_POINT('Ctrl Pts',(1.35226619967441,1.30000000000266,11.8576685289093));
#60756=CARTESIAN_POINT('Ctrl Pts',(1.35823284506601,1.2940797865347,11.862100905817));
#60757=CARTESIAN_POINT('Ctrl Pts',(1.3636491659162,1.28792143437105,11.8669357058832));
#60758=CARTESIAN_POINT('Ctrl Pts',(1.37478082571786,1.27683526110006,11.8752248429408));
#60759=CARTESIAN_POINT('Ctrl Pts',(1.38017594642871,1.27167604393436,11.8790171853508));
#60760=CARTESIAN_POINT('Ctrl Pts',(1.39340497014156,1.25863370373997,11.8886989987441));
#60761=CARTESIAN_POINT('Ctrl Pts',(1.39774281353032,1.25431389636448,11.8919151916413));
#60762=CARTESIAN_POINT('Ctrl Pts',(1.4116468894559,1.24027168164373,11.9024179757432));
#60763=CARTESIAN_POINT('Ctrl Pts',(1.43151180765357,1.21992450679007,11.9176985644207));
#60764=CARTESIAN_POINT('Ctrl Pts',(1.45281637515628,1.20000000013438,11.9320000611525));
#60765=CARTESIAN_POINT('Origin',(0.,1.2,7.2));
#60766=CARTESIAN_POINT('Origin',(0.,0.92691742076555,7.2));
#60767=CARTESIAN_POINT('Origin',(0.,0.653834841531101,7.2));
#60768=CARTESIAN_POINT('Origin',(0.,0.,7.2));
#60769=CARTESIAN_POINT('Origin',(0.,-0.653834841531101,7.2));
#60770=CARTESIAN_POINT('Origin',(0.,-0.926917420765551,7.2));
#60771=CARTESIAN_POINT('Origin',(0.,-1.2,7.2));
#60772=CARTESIAN_POINT('Origin',(0.,-1.25,7.2));
#60773=CARTESIAN_POINT('Ctrl Pts',(1.27960380226576,-1.30000000000011,12.0796635102738));
#60774=CARTESIAN_POINT('Ctrl Pts',(1.32185850051503,-1.18514270861186,12.0742273399892));
#60775=CARTESIAN_POINT('Ctrl Pts',(1.35267060678129,-1.06847604194516,12.0599359627022));
#60776=CARTESIAN_POINT('Ctrl Pts',(1.39741805963368,-0.794772684000851,
12.0064627225352));
#60777=CARTESIAN_POINT('Ctrl Pts',(1.38457112325749,-0.636309800095197,
11.9376612423041));
#60778=CARTESIAN_POINT('Ctrl Pts',(1.39375448302828,-0.319434907277159,
11.864085086346));
#60779=CARTESIAN_POINT('Ctrl Pts',(1.38362278588515,-0.158333333333333,
11.8193529279854));
#60780=CARTESIAN_POINT('Ctrl Pts',(1.41600270610974,0.158333333333334,11.8093804181475));
#60781=CARTESIAN_POINT('Ctrl Pts',(1.45995892423146,0.319434907277167,11.8436091949742));
#60782=CARTESIAN_POINT('Ctrl Pts',(1.51378858280534,0.636309800095206,11.8979534138578));
#60783=CARTESIAN_POINT('Ctrl Pts',(1.56075790439375,0.79477268400084,11.9555717424973));
#60784=CARTESIAN_POINT('Ctrl Pts',(1.56074958985878,1.06847604194602,11.9972576463276));
#60785=CARTESIAN_POINT('Ctrl Pts',(1.54630261814452,1.18514270861357,12.0079231435181));
#60786=CARTESIAN_POINT('Ctrl Pts',(1.51741227377009,1.30000000000265,12.011209854746));
#60787=CARTESIAN_POINT('Ctrl Pts',(1.27082599327824,-1.30000000000011,12.0707049385394));
#60788=CARTESIAN_POINT('Ctrl Pts',(1.31146501795804,-1.18514270861186,12.0635250605734));
#60789=CARTESIAN_POINT('Ctrl Pts',(1.34107385349426,-1.06847604194515,12.047970320616));
#60790=CARTESIAN_POINT('Ctrl Pts',(1.3839942433067,-0.794772684000847,11.9926881530137));
#60791=CARTESIAN_POINT('Ctrl Pts',(1.37127685908325,-0.636309800095196,
11.9243069098157));
#60792=CARTESIAN_POINT('Ctrl Pts',(1.38030676013406,-0.31943490727716,11.8507340127396));
#60793=CARTESIAN_POINT('Ctrl Pts',(1.37092683910606,-0.158333333333332,
11.8064558800024));
#60794=CARTESIAN_POINT('Ctrl Pts',(1.40289766570327,0.158333333333334,11.7967144930055));
#60795=CARTESIAN_POINT('Ctrl Pts',(1.44556071014891,0.319434907277165,11.8307896575199));
#60796=CARTESIAN_POINT('Ctrl Pts',(1.49898002676598,0.636309800095204,11.8854602584084));
#60797=CARTESIAN_POINT('Ctrl Pts',(1.54563126199516,0.79477268400084,11.9427846751805));
#60798=CARTESIAN_POINT('Ctrl Pts',(1.54752279646355,1.06847604194602,11.9862544409645));
#60799=CARTESIAN_POINT('Ctrl Pts',(1.53441897429966,1.18514270861357,11.9981098154132));
#60800=CARTESIAN_POINT('Ctrl Pts',(1.50739255478879,1.30000000000265,12.0030041134162));
#60801=CARTESIAN_POINT('Ctrl Pts',(1.25383737212069,-1.30000000000012,12.052589623136));
#60802=CARTESIAN_POINT('Ctrl Pts',(1.28972360254438,-1.18514270861186,12.0426154229797));
#60803=CARTESIAN_POINT('Ctrl Pts',(1.31605876757647,-1.06847604194516,12.0249219047458));
#60804=CARTESIAN_POINT('Ctrl Pts',(1.35483339539366,-0.79477268400085,11.9662131690461));
#60805=CARTESIAN_POINT('Ctrl Pts',(1.34485222586452,-0.636309800095198,
11.897481087427));
#60806=CARTESIAN_POINT('Ctrl Pts',(1.35423307167692,-0.31943490727716,11.8235941605412));
#60807=CARTESIAN_POINT('Ctrl Pts',(1.34545823241125,-0.158333333333333,
11.7806840788868));
#60808=CARTESIAN_POINT('Ctrl Pts',(1.37685655019847,0.158333333333334,11.771262559764));
#60809=CARTESIAN_POINT('Ctrl Pts',(1.41792802988074,0.319434907277167,11.8044845269271));
#60810=CARTESIAN_POINT('Ctrl Pts',(1.47067347813237,0.636309800095207,11.8597235333016));
#60811=CARTESIAN_POINT('Ctrl Pts',(1.51577191090823,0.794772684000843,11.9169468970452));
#60812=CARTESIAN_POINT('Ctrl Pts',(1.52149737687582,1.06847604194602,11.9639876772803));
#60813=CARTESIAN_POINT('Ctrl Pts',(1.51126569030078,1.18514270861357,11.9781387732636));
#60814=CARTESIAN_POINT('Ctrl Pts',(1.48832397508273,1.30000000000265,11.9860787544988));
#60815=CARTESIAN_POINT('Ctrl Pts',(1.2365731147009,-1.30000000000012,12.034356720118));
#60816=CARTESIAN_POINT('Ctrl Pts',(1.27010978630414,-1.18514270861187,12.0204441753879));
#60817=CARTESIAN_POINT('Ctrl Pts',(1.29456342074366,-1.06847604194516,11.9999506330389));
#60818=CARTESIAN_POINT('Ctrl Pts',(1.33007257532821,-0.794772684000856,
11.9374030294705));
#60819=CARTESIAN_POINT('Ctrl Pts',(1.31916493506146,-0.6363098000952,11.8700777360443));
#60820=CARTESIAN_POINT('Ctrl Pts',(1.32782448681212,-0.31943490727716,11.7963893863368));
#60821=CARTESIAN_POINT('Ctrl Pts',(1.32055135829017,-0.158333333333333,
11.754410128018));
#60822=CARTESIAN_POINT('Ctrl Pts',(1.35133196538818,0.158333333333335,11.7453259482025));
#60823=CARTESIAN_POINT('Ctrl Pts',(1.39055802938108,0.319434907277168,11.7778105062921));
#60824=CARTESIAN_POINT('Ctrl Pts',(1.44220840952662,0.636309800095208,11.8338312363221));
#60825=CARTESIAN_POINT('Ctrl Pts',(1.48524012839578,0.794772684000845,11.8912092691164));
#60826=CARTESIAN_POINT('Ctrl Pts',(1.49468958829248,1.06847604194603,11.9419141249711));
#60827=CARTESIAN_POINT('Ctrl Pts',(1.48739966201705,1.18514270861358,11.9583509797162));
#60828=CARTESIAN_POINT('Ctrl Pts',(1.46872948841386,1.30000000000266,11.9692764359068));
#60829=CARTESIAN_POINT('Ctrl Pts',(1.2279422538807,-1.30000000000012,12.0251164943471));
#60830=CARTESIAN_POINT('Ctrl Pts',(1.25939336556772,-1.18514270861187,12.0096188855853));
#60831=CARTESIAN_POINT('Ctrl Pts',(1.28238085235411,-1.06847604194516,11.9879392005477));
#60832=CARTESIAN_POINT('Ctrl Pts',(1.3159338787988,-0.794772684000856,11.9235729581872));
#60833=CARTESIAN_POINT('Ctrl Pts',(1.30587319655974,-0.636309800095201,
11.85633747634));
#60834=CARTESIAN_POINT('Ctrl Pts',(1.31477662826182,-0.319434907277161,
11.782456120855));
#60835=CARTESIAN_POINT('Ctrl Pts',(1.30836512397911,-0.158333333333333,
11.7409006005277));
#60836=CARTESIAN_POINT('Ctrl Pts',(1.33885141222359,0.158333333333335,11.7319758825528));
#60837=CARTESIAN_POINT('Ctrl Pts',(1.37669134199997,0.319434907277169,11.7643080243584));
#60838=CARTESIAN_POINT('Ctrl Pts',(1.42796721862588,0.636309800095209,11.8206187219591));
#60839=CARTESIAN_POINT('Ctrl Pts',(1.47080084715812,0.794772684000844,11.8776220530351));
#60840=CARTESIAN_POINT('Ctrl Pts',(1.48213706696437,1.06847604194603,11.9301857284284));
#60841=CARTESIAN_POINT('Ctrl Pts',(1.47615489814238,1.18514270861358,11.9478807037177));
#60842=CARTESIAN_POINT('Ctrl Pts',(1.45928353099258,1.30000000000266,11.9605177868944));
#60843=CARTESIAN_POINT('Ctrl Pts',(1.2277441157689,-1.30000000000012,12.0249027924082));
#60844=CARTESIAN_POINT('Ctrl Pts',(1.25914693044367,-1.18514270861187,12.0093686494923));
#60845=CARTESIAN_POINT('Ctrl Pts',(1.28210042632704,-1.06847604194516,11.9876616416957));
#60846=CARTESIAN_POINT('Ctrl Pts',(1.31560797696017,-0.794772684000856,
11.9232535584614));
#60847=CARTESIAN_POINT('Ctrl Pts',(1.30556631666563,-0.636309800095201,
11.8560204271351));
#60848=CARTESIAN_POINT('Ctrl Pts',(1.3144757803299,-0.319434907277161,11.7821344120641));
#60849=CARTESIAN_POINT('Ctrl Pts',(1.30808552937375,-0.158333333333333,
11.7405879874874));
#60850=CARTESIAN_POINT('Ctrl Pts',(1.33856517060333,0.158333333333335,11.7316668701696));
#60851=CARTESIAN_POINT('Ctrl Pts',(1.37637210730414,0.319434907277169,11.7639959828845));
#60852=CARTESIAN_POINT('Ctrl Pts',(1.42763878600979,0.636309800095209,11.8203136512801));
#60853=CARTESIAN_POINT('Ctrl Pts',(1.47046774593146,0.794772684000844,11.8773083954233));
#60854=CARTESIAN_POINT('Ctrl Pts',(1.48184741511707,1.06847604194603,11.9299150314142));
#60855=CARTESIAN_POINT('Ctrl Pts',(1.47589543953387,1.18514270861358,11.9476390432925));
#60856=CARTESIAN_POINT('Ctrl Pts',(1.4590656512353,1.30000000000266,11.9603156035967));
#60857=CARTESIAN_POINT('Ctrl Pts',(1.22754580284173,-1.30000000000012,12.0246891655378));
#60858=CARTESIAN_POINT('Ctrl Pts',(1.25890052554179,-1.18514270861187,12.00911840385));
#60859=CARTESIAN_POINT('Ctrl Pts',(1.28182017328752,-1.06847604194516,11.9873840137994));
#60860=CARTESIAN_POINT('Ctrl Pts',(1.3152824340645,-0.794772684000856,11.9229340102849));
#60861=CARTESIAN_POINT('Ctrl Pts',(1.30525983172521,-0.636309800095201,
11.8557031978233));
#60862=CARTESIAN_POINT('Ctrl Pts',(1.31417504098312,-0.319434907277161,
11.7818126625729));
#60863=CARTESIAN_POINT('Ctrl Pts',(1.307805392372,-0.158333333333333,11.7402756575975));
#60864=CARTESIAN_POINT('Ctrl Pts',(1.33827832071744,0.158333333333335,11.7313581736543));
#60865=CARTESIAN_POINT('Ctrl Pts',(1.37605285408983,0.319434907277169,11.7636839655362));
#60866=CARTESIAN_POINT('Ctrl Pts',(1.42731047763198,0.636309800095209,11.8200085332043));
#60867=CARTESIAN_POINT('Ctrl Pts',(1.47013448595545,0.794772684000844,11.8769948315385));
#60868=CARTESIAN_POINT('Ctrl Pts',(1.4815575698706,1.06847604194603,11.929644439847));
#60869=CARTESIAN_POINT('Ctrl Pts',(1.47563580573477,1.18514270861358,11.9473974756357));
#60870=CARTESIAN_POINT('Ctrl Pts',(1.45884764770319,1.30000000000266,11.9601134826365));
#60871=CARTESIAN_POINT('Ctrl Pts',(1.22714990870516,-1.30000000000012,12.0242615781458));
#60872=CARTESIAN_POINT('Ctrl Pts',(1.25840855833041,-1.18514270861187,12.0086175096358));
#60873=CARTESIAN_POINT('Ctrl Pts',(1.28126054876466,-1.06847604194516,11.9868283246064));
#60874=CARTESIAN_POINT('Ctrl Pts',(1.31463215371521,-0.794772684000856,
11.9222944997908));
#60875=CARTESIAN_POINT('Ctrl Pts',(1.30464720806962,-0.636309800095201,
11.8550685521741));
#60876=CARTESIAN_POINT('Ctrl Pts',(1.31357391352614,-0.319434907277161,
11.7811689659258));
#60877=CARTESIAN_POINT('Ctrl Pts',(1.30724591853039,-0.158333333333334,
11.7396505754641));
#60878=CARTESIAN_POINT('Ctrl Pts',(1.33770547706531,0.158333333333335,11.7307403238344));
#60879=CARTESIAN_POINT('Ctrl Pts',(1.37541502963884,0.319434907277169,11.7630595516123));
#60880=CARTESIAN_POINT('Ctrl Pts',(1.42665420609279,0.63630980009521,11.8193980878653));
#60881=CARTESIAN_POINT('Ctrl Pts',(1.46946784062387,0.794772684000844,11.876367741162));
#60882=CARTESIAN_POINT('Ctrl Pts',(1.4809776294413,1.06847604194603,11.9291033667068));
#60883=CARTESIAN_POINT('Ctrl Pts',(1.47511633151914,1.18514270861358,11.9469144330437));
#60884=CARTESIAN_POINT('Ctrl Pts',(1.45841157457544,1.30000000000266,11.9597092674665));
#60885=CARTESIAN_POINT('Ctrl Pts',(1.22629415633927,-1.30000000000012,12.0233341953758));
#60886=CARTESIAN_POINT('Ctrl Pts',(1.25734596825504,-1.18514270861187,12.0075306576544));
#60887=CARTESIAN_POINT('Ctrl Pts',(1.28005213212735,-1.06847604194516,11.9856223762587));
#60888=CARTESIAN_POINT('Ctrl Pts',(1.31322779650329,-0.794772684000856,
11.9209066843603));
#60889=CARTESIAN_POINT('Ctrl Pts',(1.30332272510325,-0.636309800095201,
11.8536920688135));
#60890=CARTESIAN_POINT('Ctrl Pts',(1.3122731506626,-0.319434907277161,11.7797734197834));
#60891=CARTESIAN_POINT('Ctrl Pts',(1.30603447327239,-0.158333333333333,
11.7382958186757));
#60892=CARTESIAN_POINT('Ctrl Pts',(1.33646502740032,0.158333333333335,11.7294012299134));
#60893=CARTESIAN_POINT('Ctrl Pts',(1.37403557863277,0.319434907277169,11.7617053160632));
#60894=CARTESIAN_POINT('Ctrl Pts',(1.42523407739856,0.636309800095209,11.8180744807929));
#60895=CARTESIAN_POINT('Ctrl Pts',(1.46802220160723,0.794772684000844,11.875009634575));
#60896=CARTESIAN_POINT('Ctrl Pts',(1.47971924795819,1.06847604194603,11.9279319497901));
#60897=CARTESIAN_POINT('Ctrl Pts',(1.4739892254602,1.18514270861358,11.9458686175773));
#60898=CARTESIAN_POINT('Ctrl Pts',(1.45746596251714,1.30000000000266,11.9588338438603));
#60899=CARTESIAN_POINT('Ctrl Pts',(1.22524790954672,-1.30000000000012,12.0221894989965));
#60900=CARTESIAN_POINT('Ctrl Pts',(1.25605069328636,-1.18514270861187,12.0061870364817));
#60901=CARTESIAN_POINT('Ctrl Pts',(1.2785805568903,-1.06847604194516,11.9841306379267));
#60902=CARTESIAN_POINT('Ctrl Pts',(1.31151694839366,-0.794772684000856,
11.9191901415583));
#60903=CARTESIAN_POINT('Ctrl Pts',(1.30170267453756,-0.636309800095201,
11.8519929619082));
#60904=CARTESIAN_POINT('Ctrl Pts',(1.31067734237213,-0.319434907277161,
11.7780531506376));
#60905=CARTESIAN_POINT('Ctrl Pts',(1.30454497855561,-0.158333333333333,
11.7366275268995));
#60906=CARTESIAN_POINT('Ctrl Pts',(1.33493994462557,0.158333333333335,11.727752068216));
#60907=CARTESIAN_POINT('Ctrl Pts',(1.37234701512126,0.319434907277168,11.7600336232914));
#60908=CARTESIAN_POINT('Ctrl Pts',(1.42349273638346,0.636309800095209,11.8164419034647));
#60909=CARTESIAN_POINT('Ctrl Pts',(1.46623680485781,0.794772684000844,11.8733411702764));
#60910=CARTESIAN_POINT('Ctrl Pts',(1.47816221397479,1.06847604194603,11.9264943787167));
#60911=CARTESIAN_POINT('Ctrl Pts',(1.47259511058383,1.18514270861358,11.9445849484738));
#60912=CARTESIAN_POINT('Ctrl Pts',(1.4562988360751,1.30000000000266,11.9577580335746));
#60913=CARTESIAN_POINT('Ctrl Pts',(1.22368876170903,-1.30000000000012,12.0204674403452));
#60914=CARTESIAN_POINT('Ctrl Pts',(1.25413034507549,-1.18514270861187,12.0041607583451));
#60915=CARTESIAN_POINT('Ctrl Pts',(1.27640296468573,-1.06847604194516,11.981878763065));
#60916=CARTESIAN_POINT('Ctrl Pts',(1.30898523113519,-0.794772684000856,
11.9165987274361));
#60917=CARTESIAN_POINT('Ctrl Pts',(1.29929200326749,-0.636309800095201,
11.8494347124025));
#60918=CARTESIAN_POINT('Ctrl Pts',(1.3082915033771,-0.319434907277161,11.7754685822411));
#60919=CARTESIAN_POINT('Ctrl Pts',(1.3023077506762,-0.158333333333333,11.7341262772798));
#60920=CARTESIAN_POINT('Ctrl Pts',(1.33264970510214,0.158333333333335,11.7252791534609));
#60921=CARTESIAN_POINT('Ctrl Pts',(1.36983080131772,0.319434907277169,11.7575170945062));
#60922=CARTESIAN_POINT('Ctrl Pts',(1.42089331169685,0.636309800095209,11.8139862500183));
#60923=CARTESIAN_POINT('Ctrl Pts',(1.46354419012881,0.794772684000844,11.8708458353556));
#60924=CARTESIAN_POINT('Ctrl Pts',(1.47580830789673,1.06847604194603,11.9243474423368));
#60925=CARTESIAN_POINT('Ctrl Pts',(1.47048874147005,1.18514270861358,11.9426672444924));
#60926=CARTESIAN_POINT('Ctrl Pts',(1.45454092646529,1.30000000000266,11.9561479855713));
#60927=CARTESIAN_POINT('Ctrl Pts',(1.22162818486884,-1.30000000000012,12.0181623433247));
#60928=CARTESIAN_POINT('Ctrl Pts',(1.251613764737,-1.18514270861187,12.0014380578494));
#60929=CARTESIAN_POINT('Ctrl Pts',(1.27355839427798,-1.06847604194516,11.9788482316104));
#60930=CARTESIAN_POINT('Ctrl Pts',(1.30567867468334,-0.794772684000856,
11.9131106413578));
#60931=CARTESIAN_POINT('Ctrl Pts',(1.29611619437512,-0.6363098000952,11.8460049698049));
#60932=CARTESIAN_POINT('Ctrl Pts',(1.3051245076517,-0.319434907277161,11.7720152250008));
#60933=CARTESIAN_POINT('Ctrl Pts',(1.29931487976112,-0.158333333333333,
11.7307958743874));
#60934=CARTESIAN_POINT('Ctrl Pts',(1.32958673997488,0.158333333333335,11.7219859083677));
#60935=CARTESIAN_POINT('Ctrl Pts',(1.3665072480433,0.319434907277169,11.7541449844838));
#60936=CARTESIAN_POINT('Ctrl Pts',(1.4174515111205,0.636309800095209,11.81069932319));
#60937=CARTESIAN_POINT('Ctrl Pts',(1.45992304453503,0.794772684000844,11.8675347589428));
#60938=CARTESIAN_POINT('Ctrl Pts',(1.47263148167845,1.06847604194603,11.9215047324072));
#60939=CARTESIAN_POINT('Ctrl Pts',(1.46764862113243,1.18514270861358,11.940126701114));
#60940=CARTESIAN_POINT('Ctrl Pts',(1.45218188849499,1.30000000000266,11.9540090367993));
#60941=CARTESIAN_POINT('Ctrl Pts',(1.21883413279385,-1.30000000000012,12.0149728629311));
#60942=CARTESIAN_POINT('Ctrl Pts',(1.24826042730895,-1.18514270861187,11.9976427476694));
#60943=CARTESIAN_POINT('Ctrl Pts',(1.26979427796863,-1.06847604194516,11.9746108564949));
#60944=CARTESIAN_POINT('Ctrl Pts',(1.30130865664055,-0.794772684000856,
11.9082303373725));
#60945=CARTESIAN_POINT('Ctrl Pts',(1.29185020172849,-0.636309800095201,
11.8412398015522));
#60946=CARTESIAN_POINT('Ctrl Pts',(1.30080646926028,-0.319434907277161,
11.767248042859));
#60947=CARTESIAN_POINT('Ctrl Pts',(1.29516702066596,-0.158333333333333,
11.7262319896314));
#60948=CARTESIAN_POINT('Ctrl Pts',(1.32534343698007,0.158333333333335,11.7174717384533));
#60949=CARTESIAN_POINT('Ctrl Pts',(1.36201587657113,0.319434907277169,11.7494661513915));
#60950=CARTESIAN_POINT('Ctrl Pts',(1.41278201534404,0.636309800095209,11.8061463399929));
#60951=CARTESIAN_POINT('Ctrl Pts',(1.45486644089265,0.794772684000844,11.8630221677633));
#60952=CARTESIAN_POINT('Ctrl Pts',(1.46816687496799,1.06847604194603,11.9176461708665));
#60953=CARTESIAN_POINT('Ctrl Pts',(1.46366343298579,1.18514270861358,11.9366750131029));
#60954=CARTESIAN_POINT('Ctrl Pts',(1.4488992839398,1.30000000000266,11.951087990651));
#60955=CARTESIAN_POINT('Ctrl Pts',(1.21581476102868,-1.30000000000012,12.0114782862877));
#60956=CARTESIAN_POINT('Ctrl Pts',(1.24468676622456,-1.18514270861187,11.9934610959788));
#60957=CARTESIAN_POINT('Ctrl Pts',(1.26580677376303,-1.06847604194516,11.9699308744671));
#60958=CARTESIAN_POINT('Ctrl Pts',(1.29668955084951,-0.794772684000855,
11.902835150614));
#60959=CARTESIAN_POINT('Ctrl Pts',(1.28729091458771,-0.6363098000952,11.8359950228554));
#60960=CARTESIAN_POINT('Ctrl Pts',(1.29614317182758,-0.31943490727716,11.7620236248868));
#60961=CARTESIAN_POINT('Ctrl Pts',(1.29063333737263,-0.158333333333333,
11.7212572543137));
#60962=CARTESIAN_POINT('Ctrl Pts',(1.32070432401616,0.158333333333335,11.7125508945433));
#60963=CARTESIAN_POINT('Ctrl Pts',(1.35718925414493,0.319434907277168,11.7443225736727));
#60964=CARTESIAN_POINT('Ctrl Pts',(1.40774782651833,0.636309800095208,11.8011470545255));
#60965=CARTESIAN_POINT('Ctrl Pts',(1.44930440815035,0.794772684000843,11.8581223765224));
#60966=CARTESIAN_POINT('Ctrl Pts',(1.46323198337746,1.06847604194603,11.9134697715173));
#60967=CARTESIAN_POINT('Ctrl Pts',(1.45926115161887,1.18514270861358,11.9329374893995));
#60968=CARTESIAN_POINT('Ctrl Pts',(1.44529075685338,1.30000000000266,11.9479150886937));
#60969=CARTESIAN_POINT('Ctrl Pts',(1.2127914376561,-1.30000000000012,12.0079846421543));
#60970=CARTESIAN_POINT('Ctrl Pts',(1.24110915570597,-1.18514270861187,11.9892800327384));
#60971=CARTESIAN_POINT('Ctrl Pts',(1.26181830932371,-1.06847604194516,11.9652498645401));
#60972=CARTESIAN_POINT('Ctrl Pts',(1.29208329110632,-0.794772684000854,
11.8974322626217));
#60973=CARTESIAN_POINT('Ctrl Pts',(1.28276751986128,-0.6363098000952,11.830732122404));
#60974=CARTESIAN_POINT('Ctrl Pts',(1.29153147513043,-0.31943490727716,11.7567738149627));
#60975=CARTESIAN_POINT('Ctrl Pts',(1.28615636910397,-0.158333333333333,
11.7162549003776));
#60976=CARTESIAN_POINT('Ctrl Pts',(1.31611486034211,0.158333333333335,11.7076052631193));
#60977=CARTESIAN_POINT('Ctrl Pts',(1.35238550590869,0.319434907277168,11.7391661228376));
#60978=CARTESIAN_POINT('Ctrl Pts',(1.40273614028725,0.636309800095208,11.7961339664401));
#60979=CARTESIAN_POINT('Ctrl Pts',(1.44380164635047,0.794772684000843,11.8531898499142));
#60980=CARTESIAN_POINT('Ctrl Pts',(1.45834763245817,1.06847604194603,11.9092653490168));
#60981=CARTESIAN_POINT('Ctrl Pts',(1.45489660611559,1.18514270861358,11.9291787884017));
#60982=CARTESIAN_POINT('Ctrl Pts',(1.44169813502628,1.30000000000266,11.9447326614119));
#60983=CARTESIAN_POINT('Ctrl Pts',(1.20872858075993,-1.30000000000012,12.0033407550191));
#60984=CARTESIAN_POINT('Ctrl Pts',(1.23625742321363,-1.18514270861187,11.9837420038142));
#60985=CARTESIAN_POINT('Ctrl Pts',(1.25639293334808,-1.06847604194516,11.9590567469262));
#60986=CARTESIAN_POINT('Ctrl Pts',(1.28582991316517,-0.794772684000855,
11.8902780195665));
#60987=CARTESIAN_POINT('Ctrl Pts',(1.27670502214909,-0.6363098000952,11.8237279150921));
#60988=CARTESIAN_POINT('Ctrl Pts',(1.28542646124839,-0.31943490727716,11.7497516876065));
#60989=CARTESIAN_POINT('Ctrl Pts',(1.28030515900938,-0.158333333333333,
11.709527140093));
#60990=CARTESIAN_POINT('Ctrl Pts',(1.31011045946272,0.158333333333335,11.7009544754783));
#60991=CARTESIAN_POINT('Ctrl Pts',(1.34597814359557,0.319434907277168,11.7322909617147));
#60992=CARTESIAN_POINT('Ctrl Pts',(1.39605104033275,0.636309800095208,11.7894477289245));
#60993=CARTESIAN_POINT('Ctrl Pts',(1.43658852574654,0.794772684000842,11.846544440666));
#60994=CARTESIAN_POINT('Ctrl Pts',(1.45195911272829,1.06847604194603,11.9035912069717));
#60995=CARTESIAN_POINT('Ctrl Pts',(1.44917663141501,1.18514270861358,11.9241123932074));
#60996=CARTESIAN_POINT('Ctrl Pts',(1.43695831122038,1.30000000000266,11.940461334336));
#60997=CARTESIAN_POINT('Ctrl Pts',(1.20145510658949,-1.30000000000012,11.9952901443843));
#60998=CARTESIAN_POINT('Ctrl Pts',(1.22737142220384,-1.18514270861187,11.9742330751038));
#60999=CARTESIAN_POINT('Ctrl Pts',(1.24637839959851,-1.06847604194516,11.9484584103413));
#61000=CARTESIAN_POINT('Ctrl Pts',(1.27432636621717,-0.794772684000854,
11.8780151892209));
#61001=CARTESIAN_POINT('Ctrl Pts',(1.26588617433029,-0.6363098000952,11.8115668131939));
#61002=CARTESIAN_POINT('Ctrl Pts',(1.27484109981736,-0.31943490727716,11.737414026359));
#61003=CARTESIAN_POINT('Ctrl Pts',(1.27046109361697,-0.158333333333333,
11.6975606099016));
#61004=CARTESIAN_POINT('Ctrl Pts',(1.29998168292981,0.158333333333335,11.6891312863438));
#61005=CARTESIAN_POINT('Ctrl Pts',(1.33464292223727,0.319434907277168,11.7203220298716));
#61006=CARTESIAN_POINT('Ctrl Pts',(1.38426993498686,0.636309800095208,11.7777802074196));
#61007=CARTESIAN_POINT('Ctrl Pts',(1.42450022186561,0.794772684000843,11.8346246185139));
#61008=CARTESIAN_POINT('Ctrl Pts',(1.44133915951881,1.06847604194603,11.8933588537356));
#61009=CARTESIAN_POINT('Ctrl Pts',(1.43961940851332,1.18514270861358,11.9150013498131));
#61010=CARTESIAN_POINT('Ctrl Pts',(1.42889095433638,1.30000000000266,11.9328624678583));
#61011=CARTESIAN_POINT('Ctrl Pts',(1.19312358840273,-1.30000000000012,11.986092224098));
#61012=CARTESIAN_POINT('Ctrl Pts',(1.21718649562038,-1.18514270861187,11.9633706907938));
#61013=CARTESIAN_POINT('Ctrl Pts',(1.23487329811423,-1.06847604194516,11.936363193005));
#61014=CARTESIAN_POINT('Ctrl Pts',(1.26100327266032,-0.794772684000852,
11.8640690349175));
#61015=CARTESIAN_POINT('Ctrl Pts',(1.25309742420552,-0.636309800095199,
11.7978514797918));
#61016=CARTESIAN_POINT('Ctrl Pts',(1.26234630009569,-0.31943490727716,11.723487627083));
#61017=CARTESIAN_POINT('Ctrl Pts',(1.25905343060208,-0.158333333333333,
11.6839559230984));
#61018=CARTESIAN_POINT('Ctrl Pts',(1.28845759211167,0.158333333333335,11.6755922274868));
#61019=CARTESIAN_POINT('Ctrl Pts',(1.32200304010692,0.319434907277168,11.7064777237483));
#61020=CARTESIAN_POINT('Ctrl Pts',(1.37092015971712,0.636309800095208,11.7643807875321));
#61021=CARTESIAN_POINT('Ctrl Pts',(1.40998322857041,0.794772684000842,11.8213481979597));
#61022=CARTESIAN_POINT('Ctrl Pts',(1.42851014512994,1.06847604194602,11.8820088745646));
#61023=CARTESIAN_POINT('Ctrl Pts',(1.42818966260314,1.18514270861358,11.9048416990058));
#61024=CARTESIAN_POINT('Ctrl Pts',(1.41952908186081,1.30000000000266,11.9242495886853));
#61025=CARTESIAN_POINT('Ctrl Pts',(1.18504714964652,-1.30000000000012,11.976770901141));
#61026=CARTESIAN_POINT('Ctrl Pts',(1.20752489221823,-1.18514270861186,11.9522592293794));
#61027=CARTESIAN_POINT('Ctrl Pts',(1.22409981608184,-1.06847604194516,11.9239215647813));
#61028=CARTESIAN_POINT('Ctrl Pts',(1.24875451393843,-0.79477268400085,11.84961708179));
#61029=CARTESIAN_POINT('Ctrl Pts',(1.24163979516002,-0.636309800095198,
11.7835146474624));
#61030=CARTESIAN_POINT('Ctrl Pts',(1.25083536704097,-0.31943490727716,11.7090985716443));
#61031=CARTESIAN_POINT('Ctrl Pts',(1.24776341731568,-0.158333333333333,
11.6702844395716));
#61032=CARTESIAN_POINT('Ctrl Pts',(1.27660485154415,0.158333333333334,11.662190750739));
#61033=CARTESIAN_POINT('Ctrl Pts',(1.30897301991081,0.319434907277167,11.6928095556046));
#61034=CARTESIAN_POINT('Ctrl Pts',(1.35759900979757,0.636309800095207,11.7509464000865));
#61035=CARTESIAN_POINT('Ctrl Pts',(1.39673351914396,0.794772684000841,11.8074159111043));
#61036=CARTESIAN_POINT('Ctrl Pts',(1.41683529369696,1.06847604194602,11.8700590369959));
#61037=CARTESIAN_POINT('Ctrl Pts',(1.4175582816801,1.18514270861358,11.8942602030662));
#61038=CARTESIAN_POINT('Ctrl Pts',(1.4103029442865,1.30000000000266,11.9155466471649));
#61039=CARTESIAN_POINT('Ctrl Pts',(1.173082577549,-1.30000000000012,11.9627193030931));
#61040=CARTESIAN_POINT('Ctrl Pts',(1.19325401770505,-1.18514270861186,11.9354877943743));
#61041=CARTESIAN_POINT('Ctrl Pts',(1.20817392342902,-1.06847604194516,11.9051476176419));
#61042=CARTESIAN_POINT('Ctrl Pts',(1.23050979526431,-0.794772684000851,
11.8278740948604));
#61043=CARTESIAN_POINT('Ctrl Pts',(1.22411878218085,-0.636309800095198,
11.7621572297401));
#61044=CARTESIAN_POINT('Ctrl Pts',(1.23331463099599,-0.31943490727716,11.687624974606));
#61045=CARTESIAN_POINT('Ctrl Pts',(1.23109745274161,-0.158333333333333,
11.6496486423212));
#61046=CARTESIAN_POINT('Ctrl Pts',(1.25933044141261,0.158333333333335,11.6418461038297));
#61047=CARTESIAN_POINT('Ctrl Pts',(1.28996838723369,0.319434907277169,11.672035062822));
#61048=CARTESIAN_POINT('Ctrl Pts',(1.33789861140877,0.636309800095208,11.7306432184318));
#61049=CARTESIAN_POINT('Ctrl Pts',(1.37628250493933,0.79477268400084,11.7867795523974));
#61050=CARTESIAN_POINT('Ctrl Pts',(1.39902063264288,1.06847604194602,11.8522725395376));
#61051=CARTESIAN_POINT('Ctrl Pts',(1.4016799951753,1.18514270861358,11.878353102107));
#61052=CARTESIAN_POINT('Ctrl Pts',(1.39715622728792,1.30000000000266,11.9021647398668));
#61053=CARTESIAN_POINT('Ctrl Pts',(1.15913005914174,-1.30000000000013,11.9463091067294));
#61054=CARTESIAN_POINT('Ctrl Pts',(1.17670119651856,-1.18514270861187,11.9158671500722));
#61055=CARTESIAN_POINT('Ctrl Pts',(1.18968778798641,-1.06847604194516,11.8831932196852));
#61056=CARTESIAN_POINT('Ctrl Pts',(1.20909819405085,-0.794772684000851,
11.8025535982731));
#61057=CARTESIAN_POINT('Ctrl Pts',(1.20291285503855,-0.636309800095199,
11.7375618676765));
#61058=CARTESIAN_POINT('Ctrl Pts',(1.21193377854271,-0.31943490727716,11.6629739236331));
#61059=CARTESIAN_POINT('Ctrl Pts',(1.21073094722639,-0.158333333333333,
11.6259876804447));
#61060=CARTESIAN_POINT('Ctrl Pts',(1.23896402942151,0.158333333333335,11.6181923045527));
#61061=CARTESIAN_POINT('Ctrl Pts',(1.26892852413936,0.319434907277168,11.6472300289417));
#61062=CARTESIAN_POINT('Ctrl Pts',(1.3163396743589,0.636309800095208,11.7062512946545));
#61063=CARTESIAN_POINT('Ctrl Pts',(1.3530093507216,0.794772684000842,11.7624106275473));
#61064=CARTESIAN_POINT('Ctrl Pts',(1.37814864427987,1.06847604194603,11.8315494906404));
#61065=CARTESIAN_POINT('Ctrl Pts',(1.38276042254293,1.18514270861358,11.8599659305594));
#61066=CARTESIAN_POINT('Ctrl Pts',(1.38110211039027,1.30000000000266,11.8868711584118));
#61067=CARTESIAN_POINT('Ctrl Pts',(1.14519361629814,-1.30000000000012,11.9298776634644));
#61068=CARTESIAN_POINT('Ctrl Pts',(1.15988682778115,-1.18514270861187,11.8963267159581));
#61069=CARTESIAN_POINT('Ctrl Pts',(1.17096728411276,-1.06847604194516,11.8612936567873));
#61070=CARTESIAN_POINT('Ctrl Pts',(1.18821916774755,-0.794772684000851,
11.7769363073234));
#61071=CARTESIAN_POINT('Ctrl Pts',(1.18437105667397,-0.636309800095198,
11.7117553462717));
#61072=CARTESIAN_POINT('Ctrl Pts',(1.19382220937109,-0.319434907277159,
11.6368413175492));
#61073=CARTESIAN_POINT('Ctrl Pts',(1.19296893064302,-0.158333333333333,
11.6011157302902));
#61074=CARTESIAN_POINT('Ctrl Pts',(1.22009217020531,0.158333333333334,11.5938150571528));
#61075=CARTESIAN_POINT('Ctrl Pts',(1.24804529143141,0.319434907277168,11.6223032872997));
#61076=CARTESIAN_POINT('Ctrl Pts',(1.29388988291989,0.636309800095208,11.6822174003226));
#61077=CARTESIAN_POINT('Ctrl Pts',(1.3285254716536,0.794772684000839,11.7385634639138));
#61078=CARTESIAN_POINT('Ctrl Pts',(1.35638827104748,1.06847604194602,11.8112107840679));
#61079=CARTESIAN_POINT('Ctrl Pts',(1.36332864649763,1.18514270861358,11.8417941355254));
#61080=CARTESIAN_POINT('Ctrl Pts',(1.36514862395873,1.30000000000266,11.8715145053942));
#61081=CARTESIAN_POINT('Ctrl Pts',(1.13751282886348,-1.30000000000012,11.9203535763013));
#61082=CARTESIAN_POINT('Ctrl Pts',(1.15107565576836,-1.18514270861187,11.8848081665791));
#61083=CARTESIAN_POINT('Ctrl Pts',(1.16125632286343,-1.06847604194516,11.8483479199077));
#61084=CARTESIAN_POINT('Ctrl Pts',(1.17696223472908,-0.794772684000853,
11.7620039998844));
#61085=CARTESIAN_POINT('Ctrl Pts',(1.17261396792746,-0.636309800095199,
11.697502731694));
#61086=CARTESIAN_POINT('Ctrl Pts',(1.18193573939001,-0.31943490727716,11.6225658847503));
#61087=CARTESIAN_POINT('Ctrl Pts',(1.18202816633933,-0.158333333333333,
11.5872503591164));
#61088=CARTESIAN_POINT('Ctrl Pts',(1.20932211372468,0.158333333333335,11.579872933071));
#61089=CARTESIAN_POINT('Ctrl Pts',(1.23678302590977,0.319434907277168,11.6077476966413));
#61090=CARTESIAN_POINT('Ctrl Pts',(1.28252869772572,0.636309800095208,11.6677862688316));
#61091=CARTESIAN_POINT('Ctrl Pts',(1.31664043959854,0.794772684000841,11.7238947651359));
#61092=CARTESIAN_POINT('Ctrl Pts',(1.34583653283923,1.06847604194602,11.7986518965237));
#61093=CARTESIAN_POINT('Ctrl Pts',(1.35375920212431,1.18514270861358,11.8306470269596));
#61094=CARTESIAN_POINT('Ctrl Pts',(1.35696663375241,1.30000000000266,11.8622776956782));
#61095=CARTESIAN_POINT('Ctrl Pts',(1.1259503820225,-1.30000000000012,11.9060906586386));
#61096=CARTESIAN_POINT('Ctrl Pts',(1.13752129822288,-1.18514270861187,11.8676764365745));
#61097=CARTESIAN_POINT('Ctrl Pts',(1.14627996941706,-1.06847604194516,11.8291030294281));
#61098=CARTESIAN_POINT('Ctrl Pts',(1.16001740348972,-0.794772684000853,
11.7396229929514));
#61099=CARTESIAN_POINT('Ctrl Pts',(1.15622634367563,-0.636309800095199,
11.6755780491627));
#61100=CARTESIAN_POINT('Ctrl Pts',(1.16583292808979,-0.31943490727716,11.6004014894004));
#61101=CARTESIAN_POINT('Ctrl Pts',(1.16739699622653,-0.158333333333333,
11.5656741781615));
#61102=CARTESIAN_POINT('Ctrl Pts',(1.19388648139649,0.158333333333335,11.5586551791307));
#61103=CARTESIAN_POINT('Ctrl Pts',(1.21868580967463,0.319434907277168,11.5864612973334));
#61104=CARTESIAN_POINT('Ctrl Pts',(1.26329323296083,0.636309800095208,11.6471414376856));
#61105=CARTESIAN_POINT('Ctrl Pts',(1.29710575820313,0.794772684000841,11.7027114515257));
#61106=CARTESIAN_POINT('Ctrl Pts',(1.32847580086383,1.06847604194602,11.7805544638185));
#61107=CARTESIAN_POINT('Ctrl Pts',(1.33798892842302,1.18514270861358,11.8146061751362));
#61108=CARTESIAN_POINT('Ctrl Pts',(1.34343625444816,1.30000000000266,11.8490142421176));
#61109=CARTESIAN_POINT('Ctrl Pts',(1.10885180968865,-1.30000000000012,11.8845870085044));
#61110=CARTESIAN_POINT('Ctrl Pts',(1.11709245468514,-1.18514270861186,11.8420002941912));
#61111=CARTESIAN_POINT('Ctrl Pts',(1.12356110285849,-1.06847604194516,11.8003158606242));
#61112=CARTESIAN_POINT('Ctrl Pts',(1.13441130703938,-0.794772684000849,
11.7061009291664));
#61113=CARTESIAN_POINT('Ctrl Pts',(1.13255043658639,-0.636309800095197,
11.6423045232017));
#61114=CARTESIAN_POINT('Ctrl Pts',(1.14245569830209,-0.319434907277159,
11.5668278190085));
#61115=CARTESIAN_POINT('Ctrl Pts',(1.1445785018066,-0.158333333333333,11.5336865077498));
#61116=CARTESIAN_POINT('Ctrl Pts',(1.17055816770753,0.158333333333334,11.5268703358465));
#61117=CARTESIAN_POINT('Ctrl Pts',(1.19430857035661,0.319434907277168,11.5532479824523));
#61118=CARTESIAN_POINT('Ctrl Pts',(1.23753886832307,0.636309800095207,11.6147336817711));
#61119=CARTESIAN_POINT('Ctrl Pts',(1.26836862766871,0.794772684000839,11.6706300949674));
#61120=CARTESIAN_POINT('Ctrl Pts',(1.30243416626119,1.06847604194602,11.7533592151628));
#61121=CARTESIAN_POINT('Ctrl Pts',(1.31442308574661,1.18514270861358,11.7904591111974));
#61122=CARTESIAN_POINT('Ctrl Pts',(1.3236552153133,1.30000000000266,11.8288485325497));
#61123=CARTESIAN_POINT('Ctrl Pts',(1.08716165682342,-1.30000000000012,11.8554460453488));
#61124=CARTESIAN_POINT('Ctrl Pts',(1.09163461330749,-1.18514270861186,11.8070094617491));
#61125=CARTESIAN_POINT('Ctrl Pts',(1.09539864499635,-1.06847604194516,11.7610253698515));
#61126=CARTESIAN_POINT('Ctrl Pts',(1.10245655309274,-0.794772684000854,
11.6604586649336));
#61127=CARTESIAN_POINT('Ctrl Pts',(1.10147273423353,-0.6363098000952,11.5976855395406));
#61128=CARTESIAN_POINT('Ctrl Pts',(1.11195971100687,-0.319434907277161,
11.521728456344));
#61129=CARTESIAN_POINT('Ctrl Pts',(1.11670449593826,-0.158333333333333,
11.4899360422753));
#61130=CARTESIAN_POINT('Ctrl Pts',(1.14205338335703,0.158333333333334,11.4833662346199));
#61131=CARTESIAN_POINT('Ctrl Pts',(1.16250208920525,0.319434907277166,11.5086383759976));
#61132=CARTESIAN_POINT('Ctrl Pts',(1.20396550268856,0.636309800095206,11.5711123348862));
#61133=CARTESIAN_POINT('Ctrl Pts',(1.23302071493999,0.794772684000843,11.6264001209399));
#61134=CARTESIAN_POINT('Ctrl Pts',(1.27061175970696,1.06847604194603,11.7156785368982));
#61135=CARTESIAN_POINT('Ctrl Pts',(1.28542248019329,1.18514270861358,11.7570763750097));
#61136=CARTESIAN_POINT('Ctrl Pts',(1.29877215077176,1.30000000000266,11.8012267330557));
#61137=CARTESIAN_POINT('Ctrl Pts',(1.06841695418305,-1.30000000000012,11.8313959298598));
#61138=CARTESIAN_POINT('Ctrl Pts',(1.06988891972052,-1.18514270861186,11.7780452189972));
#61139=CARTESIAN_POINT('Ctrl Pts',(1.07167056824593,-1.06847604194516,11.7283836920636));
#61140=CARTESIAN_POINT('Ctrl Pts',(1.07650196241119,-0.79477268400085,11.6221783829878));
#61141=CARTESIAN_POINT('Ctrl Pts',(1.07780198175782,-0.636309800095199,
11.5596463462105));
#61142=CARTESIAN_POINT('Ctrl Pts',(1.08914618742764,-0.319434907277161,
11.4831627993829));
#61143=CARTESIAN_POINT('Ctrl Pts',(1.0950312567616,-0.158333333333333,11.4529425339032));
#61144=CARTESIAN_POINT('Ctrl Pts',(1.11950704521747,0.158333333333335,11.4466974187544));
#61145=CARTESIAN_POINT('Ctrl Pts',(1.13785291367085,0.319434907277167,11.4707104453756));
#61146=CARTESIAN_POINT('Ctrl Pts',(1.17686286995234,0.636309800095208,11.5343959910323));
#61147=CARTESIAN_POINT('Ctrl Pts',(1.20210874432592,0.794772684000843,11.5902004428271));
#61148=CARTESIAN_POINT('Ctrl Pts',(1.24225934619864,1.06847604194603,11.685077607433));
#61149=CARTESIAN_POINT('Ctrl Pts',(1.2597239735542,1.18514270861358,11.7299119855198));
#61150=CARTESIAN_POINT('Ctrl Pts',(1.27727352044097,1.30000000000266,11.7785119326807));
#61151=CARTESIAN_POINT('Ctrl Pts',(1.05531692441144,-1.30000000000012,11.8114079524742));
#61152=CARTESIAN_POINT('Ctrl Pts',(1.0546407111963,-1.18514270861186,11.7539943304867));
#61153=CARTESIAN_POINT('Ctrl Pts',(1.05493059994745,-1.06847604194516,11.7013319032987));
#61154=CARTESIAN_POINT('Ctrl Pts',(1.05783218976483,-0.794772684000854,
11.5906473718717));
#61155=CARTESIAN_POINT('Ctrl Pts',(1.06027950848901,-0.636309800095201,
11.5286058085701));
#61156=CARTESIAN_POINT('Ctrl Pts',(1.07171063351252,-0.319434907277162,
11.4519220537149));
#61157=CARTESIAN_POINT('Ctrl Pts',(1.07811630542711,-0.158333333333333,
11.423080293972));
#61158=CARTESIAN_POINT('Ctrl Pts',(1.10178790521326,0.158333333333335,11.4171187681031));
#61159=CARTESIAN_POINT('Ctrl Pts',(1.11847728742668,0.319434907277166,11.4401420173214));
#61160=CARTESIAN_POINT('Ctrl Pts',(1.15643788874875,0.636309800095207,11.5043912612665));
#61161=CARTESIAN_POINT('Ctrl Pts',(1.18059788257868,0.794772684000845,11.5597062750224));
#61162=CARTESIAN_POINT('Ctrl Pts',(1.2227287743895,1.06847604194603,11.6591153862637));
#61163=CARTESIAN_POINT('Ctrl Pts',(1.24180134488315,1.18514270861358,11.7069489676139));
#61164=CARTESIAN_POINT('Ctrl Pts',(1.26170958390887,1.30000000000266,11.7595856095285));
#61165=CARTESIAN_POINT('Ctrl Pts',(1.0397243972048,-1.30000000000012,11.7892518976244));
#61166=CARTESIAN_POINT('Ctrl Pts',(1.03645879285365,-1.18514270861186,11.7273595872148));
#61167=CARTESIAN_POINT('Ctrl Pts',(1.03505188828116,-1.06847604194516,11.6713483817551));
#61168=CARTESIAN_POINT('Ctrl Pts',(1.0360956255887,-0.794772684000855,11.5555378210857));
#61169=CARTESIAN_POINT('Ctrl Pts',(1.04032196354068,-0.636309800095198,
11.4938500836594));
#61170=CARTESIAN_POINT('Ctrl Pts',(1.0531486514601,-0.319434907277158,11.416480256983));
#61171=CARTESIAN_POINT('Ctrl Pts',(1.06190772064469,-0.158333333333333,
11.38857937633));
#61172=CARTESIAN_POINT('Ctrl Pts',(1.0849067419774,0.158333333333334,11.3828389576133));
#61173=CARTESIAN_POINT('Ctrl Pts',(1.09837768607963,0.319434907277168,11.4051781230188));
#61174=CARTESIAN_POINT('Ctrl Pts',(1.13396476264952,0.636309800095207,11.4704911239939));
#61175=CARTESIAN_POINT('Ctrl Pts',(1.15604748076304,0.79477268400084,11.5256381923072));
#61176=CARTESIAN_POINT('Ctrl Pts',(1.19990113065527,1.06847604194602,11.6303206238347));
#61177=CARTESIAN_POINT('Ctrl Pts',(1.22073684896087,1.18514270861357,11.6815257532195));
#61178=CARTESIAN_POINT('Ctrl Pts',(1.24342566547151,1.30000000000265,11.738622866247));
#61179=CARTESIAN_POINT('Ctrl Pts',(1.02334846451551,-1.30000000000012,11.7642300009282));
#61180=CARTESIAN_POINT('Ctrl Pts',(1.01762825135153,-1.18514270861186,11.6971517312257));
#61181=CARTESIAN_POINT('Ctrl Pts',(1.01469621959795,-1.06847604194516,11.6372540829325));
#61182=CARTESIAN_POINT('Ctrl Pts',(1.01436389652807,-0.794772684000856,
11.5154672048252));
#61183=CARTESIAN_POINT('Ctrl Pts',(1.0215444001965,-0.636309800095199,11.4538984689758));
#61184=CARTESIAN_POINT('Ctrl Pts',(1.03490484456462,-0.319434907277159,
11.3761250793631));
#61185=CARTESIAN_POINT('Ctrl Pts',(1.04325944749601,-0.158333333333333,
11.3503042370641));
#61186=CARTESIAN_POINT('Ctrl Pts',(1.0650830312482,0.158333333333334,11.3449301805328));
#61187=CARTESIAN_POINT('Ctrl Pts',(1.07733643050619,0.319434907277167,11.365653493038));
#61188=CARTESIAN_POINT('Ctrl Pts',(1.11090510700976,0.636309800095207,11.4319170513878));
#61189=CARTESIAN_POINT('Ctrl Pts',(1.12960436174885,0.794772684000841,11.4872553750911));
#61190=CARTESIAN_POINT('Ctrl Pts',(1.17546572258528,1.06847604194602,11.5977926535385));
#61191=CARTESIAN_POINT('Ctrl Pts',(1.19846922681292,1.18514270861357,11.6526905755081));
#61192=CARTESIAN_POINT('Ctrl Pts',(1.22462455149293,1.30000000000266,11.714638927417));
#61193=CARTESIAN_POINT('Ctrl Pts',(1.00703467199694,-1.30000000000012,11.739219370099));
#61194=CARTESIAN_POINT('Ctrl Pts',(0.999134719940811,-1.18514270861186,
11.6669388808963));
#61195=CARTESIAN_POINT('Ctrl Pts',(0.994917017441277,-1.06847604194516,
11.603134999775));
#61196=CARTESIAN_POINT('Ctrl Pts',(0.993680014026088,-0.794772684000856,
11.4753179308695));
#61197=CARTESIAN_POINT('Ctrl Pts',(1.00356933560391,-0.636309800095199,
11.4139753193718));
#61198=CARTESIAN_POINT('Ctrl Pts',(1.0186375465584,-0.31943490727716,11.3354321895726));
#61199=CARTESIAN_POINT('Ctrl Pts',(1.02865194271522,-0.158333333333333,
11.3109890627905));
#61200=CARTESIAN_POINT('Ctrl Pts',(1.04965946900603,0.158333333333334,11.3058310424178));
#61201=CARTESIAN_POINT('Ctrl Pts',(1.05908788074018,0.319434907277167,11.3254614994301));
#61202=CARTESIAN_POINT('Ctrl Pts',(1.08999770696503,0.636309800095207,11.3927946588076));
#61203=CARTESIAN_POINT('Ctrl Pts',(1.10608353727842,0.794772684000843,11.4479350054623));
#61204=CARTESIAN_POINT('Ctrl Pts',(1.15295974013333,1.06847604194602,11.5645997130572));
#61205=CARTESIAN_POINT('Ctrl Pts',(1.17739635454459,1.18514270861357,11.6234322688973));
#61206=CARTESIAN_POINT('Ctrl Pts',(1.20597861208563,1.30000000000265,11.6905975515131));
#61207=CARTESIAN_POINT('Ctrl Pts',(0.996639789377811,-1.30000000000012,
11.7212674543398));
#61208=CARTESIAN_POINT('Ctrl Pts',(0.987178980341047,-1.18514270861186,
11.6452064782541));
#61209=CARTESIAN_POINT('Ctrl Pts',(0.982115189660983,-1.06847604194516,
11.5785418109598));
#61210=CARTESIAN_POINT('Ctrl Pts',(0.980574812206666,-0.794772684000854,
11.4462404463224));
#61211=CARTESIAN_POINT('Ctrl Pts',(0.993894584228217,-0.636309800095199,
11.38460189545));
#61212=CARTESIAN_POINT('Ctrl Pts',(1.00877894511221,-0.31943490727716,11.3059524142012));
#61213=CARTESIAN_POINT('Ctrl Pts',(1.01600681948604,-0.158333333333333,
11.2837759476425));
#61214=CARTESIAN_POINT('Ctrl Pts',(1.03581728561432,0.158333333333335,11.2789554106594));
#61215=CARTESIAN_POINT('Ctrl Pts',(1.04621763664454,0.319434907277168,11.2968028614693));
#61216=CARTESIAN_POINT('Ctrl Pts',(1.07613083609169,0.636309800095208,11.3646320626102));
#61217=CARTESIAN_POINT('Ctrl Pts',(1.08939609589899,0.794772684000843,11.4199880656248));
#61218=CARTESIAN_POINT('Ctrl Pts',(1.13689333586009,1.06847604194602,11.5411468399775));
#61219=CARTESIAN_POINT('Ctrl Pts',(1.16238177307412,1.18514270861357,11.6028236320556));
#61220=CARTESIAN_POINT('Ctrl Pts',(1.19279885226912,1.30000000000265,11.6737320721692));
#61221=CARTESIAN_POINT('Ctrl Pts',(0.988936150867084,-1.30000000000012,
11.7086498444924));
#61222=CARTESIAN_POINT('Ctrl Pts',(0.979260374531466,-1.18514270861186,
11.6298092175276));
#61223=CARTESIAN_POINT('Ctrl Pts',(0.97386258527909,-1.06847604194516,11.5611758706455));
#61224=CARTESIAN_POINT('Ctrl Pts',(0.971275618252736,-0.794772684000855,
11.4261999682441));
#61225=CARTESIAN_POINT('Ctrl Pts',(0.98322860322658,-0.636309800095198,
11.365581526662));
#61226=CARTESIAN_POINT('Ctrl Pts',(0.997261739605961,-0.319434907277158,
11.2871729392513));
#61227=CARTESIAN_POINT('Ctrl Pts',(1.00439654953326,-0.158333333333333,
11.2660209705762));
#61228=CARTESIAN_POINT('Ctrl Pts',(1.02475591643617,0.158333333333334,11.2610046392375));
#61229=CARTESIAN_POINT('Ctrl Pts',(1.03661944501925,0.319434907277167,11.2773588457922));
#61230=CARTESIAN_POINT('Ctrl Pts',(1.06682918993637,0.636309800095207,11.3451043176933));
#61231=CARTESIAN_POINT('Ctrl Pts',(1.07845024126375,0.79477268400084,11.4003959078489));
#61232=CARTESIAN_POINT('Ctrl Pts',(1.12663667854303,1.06847604194602,11.5243786857344));
#61233=CARTESIAN_POINT('Ctrl Pts',(1.15286519959577,1.18514270861357,11.5879206634263));
#61234=CARTESIAN_POINT('Ctrl Pts',(1.18446411848644,1.30000000000265,11.6613370682779));
#61235=CARTESIAN_POINT('Ctrl Pts',(0.980511229803926,-1.30000000000012,
11.6930945208311));
#61236=CARTESIAN_POINT('Ctrl Pts',(0.970473519190732,-1.18514270861186,
11.6105616290021));
#61237=CARTESIAN_POINT('Ctrl Pts',(0.96440575931758,-1.06847604194516,11.5393409241277));
#61238=CARTESIAN_POINT('Ctrl Pts',(0.959559400554817,-0.794772684000853,
11.4009402630753));
#61239=CARTESIAN_POINT('Ctrl Pts',(0.968435802254349,-0.636309800095197,
11.3418765139652));
#61240=CARTESIAN_POINT('Ctrl Pts',(0.980362066338188,-0.319434907277159,
11.2639606380389));
#61241=CARTESIAN_POINT('Ctrl Pts',(0.987534292221185,-0.158333333333333,
11.2441157359081));
#61242=CARTESIAN_POINT('Ctrl Pts',(1.00779765629327,0.158333333333334,11.2391069268715));
#61243=CARTESIAN_POINT('Ctrl Pts',(1.01985751736349,0.319434907277167,11.2540357236247));
#61244=CARTESIAN_POINT('Ctrl Pts',(1.05130690412056,0.636309800095206,11.321560185511));
#61245=CARTESIAN_POINT('Ctrl Pts',(1.06416712157485,0.794772684000839,11.3759106179189));
#61246=CARTESIAN_POINT('Ctrl Pts',(1.11442040326315,1.06847604194602,11.5034399801553));
#61247=CARTESIAN_POINT('Ctrl Pts',(1.14163565378195,1.18514270861357,11.5695028885468));
#61248=CARTESIAN_POINT('Ctrl Pts',(1.17431337124421,1.30000000000266,11.6464259698462));
#61249=CARTESIAN_POINT('Ctrl Pts',(0.974665092423404,-1.30000000000011,
11.682537481278));
#61250=CARTESIAN_POINT('Ctrl Pts',(0.96568220521313,-1.18514270861186,11.5970539055789));
#61251=CARTESIAN_POINT('Ctrl Pts',(0.959681817346747,-1.06847604194516,
11.523988601927));
#61252=CARTESIAN_POINT('Ctrl Pts',(0.952709891133254,-0.794772684000851,
11.3838818265229));
#61253=CARTESIAN_POINT('Ctrl Pts',(0.955698270378833,-0.636309800095197,
11.3278245114625));
#61254=CARTESIAN_POINT('Ctrl Pts',(0.964465402259398,-0.319434907277159,
11.2513908870651));
#61255=CARTESIAN_POINT('Ctrl Pts',(0.972209900210545,-0.158333333333333,
11.2324665018759));
#61256=CARTESIAN_POINT('Ctrl Pts',(0.992336747193892,0.158333333333334,
11.2275421126342));
#61257=CARTESIAN_POINT('Ctrl Pts',(1.00385002392356,0.319434907277167,11.2416493150689));
#61258=CARTESIAN_POINT('Ctrl Pts',(1.03785006787198,0.636309800095206,11.3078339412536));
#61259=CARTESIAN_POINT('Ctrl Pts',(1.05542731230797,0.79477268400084,11.3592791978235));
#61260=CARTESIAN_POINT('Ctrl Pts',(1.10785601153169,1.06847604194602,11.4885093112117));
#61261=CARTESIAN_POINT('Ctrl Pts',(1.13532397903559,1.18514270861357,11.5563795755177));
#61262=CARTESIAN_POINT('Ctrl Pts',(1.16756547282411,1.30000000000265,11.6361811764914));
#61263=CARTESIAN_POINT('Ctrl Pts',(0.96840887762859,-1.30000000000011,11.6766336368645));
#61264=CARTESIAN_POINT('Ctrl Pts',(0.959587680307159,-1.18514270861186,
11.5913424478649));
#61265=CARTESIAN_POINT('Ctrl Pts',(0.953418388257846,-1.06847604194516,
11.5185778056402));
#61266=CARTESIAN_POINT('Ctrl Pts',(0.945292521151707,-0.794772684000851,
11.3794157545617));
#61267=CARTESIAN_POINT('Ctrl Pts',(0.946012577561581,-0.636309800095197,
11.3245575119393));
#61268=CARTESIAN_POINT('Ctrl Pts',(0.953320013133084,-0.319434907277159,
11.248968780158));
#61269=CARTESIAN_POINT('Ctrl Pts',(0.961064002623636,-0.158333333333333,
11.2299920510673));
#61270=CARTESIAN_POINT('Ctrl Pts',(0.980997609539021,0.158333333333334,
11.2252045756181));
#61271=CARTESIAN_POINT('Ctrl Pts',(0.992074216468527,0.319434907277167,
11.2396386228234));
#61272=CARTESIAN_POINT('Ctrl Pts',(1.0276372251559,0.636309800095206,11.3049769849608));
#61273=CARTESIAN_POINT('Ctrl Pts',(1.04845566442809,0.79477268400084,11.3547455720355));
#61274=CARTESIAN_POINT('Ctrl Pts',(1.10189571121762,1.06847604194602,11.4830880756333));
#61275=CARTESIAN_POINT('Ctrl Pts',(1.12924033300978,1.18514270861357,11.5507878560718));
#61276=CARTESIAN_POINT('Ctrl Pts',(1.16079736048771,1.30000000000265,11.6306327026994));
#61277=CARTESIAN_POINT('Ctrl Pts',(0.968408877628581,-1.3,11.6766336368644));
#61278=CARTESIAN_POINT('Ctrl Pts',(0.959587680307155,-1.18514270861178,
11.5913424478648));
#61279=CARTESIAN_POINT('Ctrl Pts',(0.953418388257844,-1.06847604194512,
11.5185778056402));
#61280=CARTESIAN_POINT('Ctrl Pts',(0.945292521151707,-0.794772684000851,
11.3794157545617));
#61281=CARTESIAN_POINT('Ctrl Pts',(0.946012577561581,-0.636309800095197,
11.3245575119393));
#61282=CARTESIAN_POINT('Ctrl Pts',(0.953320013133084,-0.319434907277159,
11.248968780158));
#61283=CARTESIAN_POINT('Ctrl Pts',(0.961064002623637,-0.158333333333332,
11.2299920510673));
#61284=CARTESIAN_POINT('Ctrl Pts',(0.980997609539021,0.158333333333334,
11.2252045756181));
#61285=CARTESIAN_POINT('Ctrl Pts',(0.992074216468527,0.319434907277167,
11.2396386228234));
#61286=CARTESIAN_POINT('Ctrl Pts',(1.0276372251559,0.636309800095206,11.3049769849608));
#61287=CARTESIAN_POINT('Ctrl Pts',(1.04845566442809,0.79477268400084,11.3547455720355));
#61288=CARTESIAN_POINT('Ctrl Pts',(1.10189571121744,1.06847604194511,11.4830880756329));
#61289=CARTESIAN_POINT('Ctrl Pts',(1.12924033300936,1.18514270861178,11.5507878560707));
#61290=CARTESIAN_POINT('Ctrl Pts',(1.16079736048698,1.3,11.6306327026976));
#61291=CARTESIAN_POINT('',(1.23747338465645,-1.2,11.992823762905));
#61292=CARTESIAN_POINT('Ctrl Pts',(1.23747338465645,-1.2,11.992823762905));
#61293=CARTESIAN_POINT('Ctrl Pts',(1.22202142463578,-1.21504261691669,11.9812774246274));
#61294=CARTESIAN_POINT('Ctrl Pts',(1.22101763652485,-1.21547066370301,11.9810846963363));
#61295=CARTESIAN_POINT('Ctrl Pts',(1.20114420805669,-1.23406682102662,11.9669384589505));
#61296=CARTESIAN_POINT('Ctrl Pts',(1.19879977037005,-1.23640407488411,11.9651259639072));
#61297=CARTESIAN_POINT('Ctrl Pts',(1.16489618114301,-1.2694151087703,11.939553996061));
#61298=CARTESIAN_POINT('Ctrl Pts',(1.15239439192118,-1.28140639977682,11.9302651952717));
#61299=CARTESIAN_POINT('Ctrl Pts',(1.13369207118163,-1.30000000000012,11.91563805733));
#61300=CARTESIAN_POINT('',(1.38832545964766,-0.653834841418303,11.9513211234181));
#61301=CARTESIAN_POINT('Ctrl Pts',(1.38832545965232,-0.653834841417626,
11.9513211234436));
#61302=CARTESIAN_POINT('Ctrl Pts',(1.3726639062272,-0.718140327968288,11.9558973945044));
#61303=CARTESIAN_POINT('Ctrl Pts',(1.36006904497293,-0.763507044235833,
11.9595163718063));
#61304=CARTESIAN_POINT('Ctrl Pts',(1.310095733821,-0.949792418009667,11.9736128203625));
#61305=CARTESIAN_POINT('Ctrl Pts',(1.28314643916662,-1.04824234463106,11.9810313014776));
#61306=CARTESIAN_POINT('Ctrl Pts',(1.23747338465645,-1.2,11.992823762905));
#61307=CARTESIAN_POINT('',(1.52166805320867,0.653834841531101,11.9103106411196));
#61308=CARTESIAN_POINT('Ctrl Pts',(1.5216680532087,0.653834841531103,11.9103106411196));
#61309=CARTESIAN_POINT('Ctrl Pts',(1.49334701587912,0.575791054272758,11.8797380243135));
#61310=CARTESIAN_POINT('Ctrl Pts',(1.46910678427171,0.493913072109036,11.8545837028923));
#61311=CARTESIAN_POINT('Ctrl Pts',(1.43214296547969,0.338189409403288,11.8198918513023));
#61312=CARTESIAN_POINT('Ctrl Pts',(1.41825074992248,0.26570323421117,11.8085823585735));
#61313=CARTESIAN_POINT('Ctrl Pts',(1.39691398424971,0.129735728132282,11.7967274120108));
#61314=CARTESIAN_POINT('Ctrl Pts',(1.38884807661025,0.066638383369331,11.7948419035998));
#61315=CARTESIAN_POINT('Ctrl Pts',(1.37599207798182,-0.0595481201416573,
11.7984066861682));
#61316=CARTESIAN_POINT('Ctrl Pts',(1.3710999037416,-0.1227920732973,11.8038677116978));
#61317=CARTESIAN_POINT('Ctrl Pts',(1.3647527081023,-0.260144682905592,11.823615105641));
#61318=CARTESIAN_POINT('Ctrl Pts',(1.36408444680164,-0.333946167126978,
11.8393299926389));
#61319=CARTESIAN_POINT('Ctrl Pts',(1.36961150358366,-0.491143170270118,
11.8838155733034));
#61320=CARTESIAN_POINT('Ctrl Pts',(1.37686564932431,-0.574255514599531,
11.9145159732068));
#61321=CARTESIAN_POINT('Ctrl Pts',(1.3883254596101,-0.653834841429858,11.9513211234048));
#61322=CARTESIAN_POINT('Ctrl Pts',(1.45281637526615,1.20000000018694,11.9320000612594));
#61323=CARTESIAN_POINT('Ctrl Pts',(1.46460429832537,1.13482355934137,11.9283809388103));
#61324=CARTESIAN_POINT('Ctrl Pts',(1.48025049117954,1.03875021853169,11.9235272221373));
#61325=CARTESIAN_POINT('Ctrl Pts',(1.51065417803845,0.795063418652971,11.9138728568002));
#61326=CARTESIAN_POINT('Ctrl Pts',(1.51542476738704,0.741568492646493,11.912327537521));
#61327=CARTESIAN_POINT('Ctrl Pts',(1.5216680532087,0.653834841531106,11.9103106411195));
#61328=CARTESIAN_POINT('Ctrl Pts',(0.968408877628581,-1.3,11.6766336368644));
#61329=CARTESIAN_POINT('Ctrl Pts',(0.959587680307155,-1.18514270861178,
11.5913424478648));
#61330=CARTESIAN_POINT('Ctrl Pts',(0.953418388257845,-1.06847604194512,
11.5185778056402));
#61331=CARTESIAN_POINT('Ctrl Pts',(0.945292521151707,-0.794772684000851,
11.3794157545617));
#61332=CARTESIAN_POINT('Ctrl Pts',(0.946012577561581,-0.636309800095197,
11.3245575119393));
#61333=CARTESIAN_POINT('Ctrl Pts',(0.953320013133084,-0.319434907277159,
11.248968780158));
#61334=CARTESIAN_POINT('Ctrl Pts',(0.961064002623636,-0.158333333333332,
11.2299920510673));
#61335=CARTESIAN_POINT('Ctrl Pts',(0.980997609539021,0.158333333333334,
11.2252045756181));
#61336=CARTESIAN_POINT('Ctrl Pts',(0.992074216468527,0.319434907277167,
11.2396386228234));
#61337=CARTESIAN_POINT('Ctrl Pts',(1.0276372251559,0.636309800095206,11.3049769849608));
#61338=CARTESIAN_POINT('Ctrl Pts',(1.04845566442809,0.79477268400084,11.3547455720355));
#61339=CARTESIAN_POINT('Ctrl Pts',(1.10189571121744,1.06847604194511,11.4830880756329));
#61340=CARTESIAN_POINT('Ctrl Pts',(1.12924033300936,1.18514270861178,11.5507878560707));
#61341=CARTESIAN_POINT('Ctrl Pts',(1.16079736048698,1.3,11.6306327026976));
#61342=CARTESIAN_POINT('Ctrl Pts',(0.892825757179277,-1.3,11.6909968251522));
#61343=CARTESIAN_POINT('Ctrl Pts',(0.885729277039985,-1.18514270861178,
11.6055436003612));
#61344=CARTESIAN_POINT('Ctrl Pts',(0.880764606872679,-1.06847604194512,
11.5327108766861));
#61345=CARTESIAN_POINT('Ctrl Pts',(0.874220133109747,-0.794772684000851,
11.3936085971602));
#61346=CARTESIAN_POINT('Ctrl Pts',(0.874292131581309,-0.636309800095197,
11.3390586058255));
#61347=CARTESIAN_POINT('Ctrl Pts',(0.881134728284516,-0.319434907277159,
11.2639480037341));
#61348=CARTESIAN_POINT('Ctrl Pts',(0.88771343062497,-0.158333333333332,
11.2453997109473));
#61349=CARTESIAN_POINT('Ctrl Pts',(0.907721667816888,0.158333333333334,
11.2409633433442));
#61350=CARTESIAN_POINT('Ctrl Pts',(0.920037078273241,0.319434907277167,
11.2553148216052));
#61351=CARTESIAN_POINT('Ctrl Pts',(0.956219211262304,0.636309800095206,
11.3209009099481));
#61352=CARTESIAN_POINT('Ctrl Pts',(0.977755058014351,0.79477268400084,11.3706875096762));
#61353=CARTESIAN_POINT('Ctrl Pts',(1.02977474137891,1.06847604194511,11.4997278279237));
#61354=CARTESIAN_POINT('Ctrl Pts',(1.0559911951017,1.18514270861178,11.5678553767222));
#61355=CARTESIAN_POINT('Ctrl Pts',(1.08590670913801,1.3,11.6482537019647));
#61356=CARTESIAN_POINT('Ctrl Pts',(0.817242636729973,-1.3,11.70536001344));
#61357=CARTESIAN_POINT('Ctrl Pts',(0.811870873772815,-1.18514270861178,
11.6197447528576));
#61358=CARTESIAN_POINT('Ctrl Pts',(0.808110825487514,-1.06847604194512,
11.5468439477319));
#61359=CARTESIAN_POINT('Ctrl Pts',(0.803147745067786,-0.794772684000851,
11.4078014397586));
#61360=CARTESIAN_POINT('Ctrl Pts',(0.802571685601037,-0.636309800095197,
11.3535596997118));
#61361=CARTESIAN_POINT('Ctrl Pts',(0.808949443435948,-0.319434907277159,
11.2789272273103));
#61362=CARTESIAN_POINT('Ctrl Pts',(0.814362858626305,-0.158333333333332,
11.2608073708274));
#61363=CARTESIAN_POINT('Ctrl Pts',(0.834445726094754,0.158333333333334,
11.2567221110703));
#61364=CARTESIAN_POINT('Ctrl Pts',(0.847999940077955,0.319434907277167,
11.270991020387));
#61365=CARTESIAN_POINT('Ctrl Pts',(0.884801197368705,0.636309800095206,
11.3368248349354));
#61366=CARTESIAN_POINT('Ctrl Pts',(0.907054451600615,0.79477268400084,11.3866294473169));
#61367=CARTESIAN_POINT('Ctrl Pts',(0.957653771540387,1.06847604194511,11.5163675802146));
#61368=CARTESIAN_POINT('Ctrl Pts',(0.982742057194051,1.18514270861178,11.5849228973736));
#61369=CARTESIAN_POINT('Ctrl Pts',(1.01101605778904,1.3,11.6658747012318));
#61370=CARTESIAN_POINT('Ctrl Pts',(0.741659516280668,-1.3,11.7197232017278));
#61371=CARTESIAN_POINT('Ctrl Pts',(0.738012470505645,-1.18514270861178,
11.633945905354));
#61372=CARTESIAN_POINT('Ctrl Pts',(0.735457044102349,-1.06847604194512,
11.5609770187778));
#61373=CARTESIAN_POINT('Ctrl Pts',(0.732075357025825,-0.794772684000851,
11.421994282357));
#61374=CARTESIAN_POINT('Ctrl Pts',(0.730851239620764,-0.636309800095197,
11.368060793598));
#61375=CARTESIAN_POINT('Ctrl Pts',(0.73676415858738,-0.319434907277159,
11.2939064508864));
#61376=CARTESIAN_POINT('Ctrl Pts',(0.741012286627639,-0.158333333333332,
11.2762150307074));
#61377=CARTESIAN_POINT('Ctrl Pts',(0.76116978437262,0.158333333333334,11.2724808787964));
#61378=CARTESIAN_POINT('Ctrl Pts',(0.775962801882669,0.319434907277167,
11.2866672191688));
#61379=CARTESIAN_POINT('Ctrl Pts',(0.813383183475107,0.636309800095206,
11.3527487599227));
#61380=CARTESIAN_POINT('Ctrl Pts',(0.836353845186878,0.79477268400084,11.4025713849577));
#61381=CARTESIAN_POINT('Ctrl Pts',(0.885532801701863,1.06847604194511,11.5330073325055));
#61382=CARTESIAN_POINT('Ctrl Pts',(0.909492919286399,1.18514270861178,11.6019904180251));
#61383=CARTESIAN_POINT('Ctrl Pts',(0.936125406440074,1.3,11.683495700499));
#61384=CARTESIAN_POINT('Ctrl Pts',(0.741659516280668,-1.3,11.7197232017278));
#61385=CARTESIAN_POINT('Ctrl Pts',(0.738012470505645,-1.18514270861178,
11.633945905354));
#61386=CARTESIAN_POINT('Ctrl Pts',(0.735457044102348,-1.06847604194512,
11.5609770187778));
#61387=CARTESIAN_POINT('Ctrl Pts',(0.732075357025825,-0.794772684000851,
11.421994282357));
#61388=CARTESIAN_POINT('Ctrl Pts',(0.730851239620765,-0.636309800095197,
11.368060793598));
#61389=CARTESIAN_POINT('Ctrl Pts',(0.736764158587381,-0.319434907277159,
11.2939064508864));
#61390=CARTESIAN_POINT('Ctrl Pts',(0.741012286627639,-0.158333333333332,
11.2762150307074));
#61391=CARTESIAN_POINT('Ctrl Pts',(0.76116978437262,0.158333333333334,11.2724808787964));
#61392=CARTESIAN_POINT('Ctrl Pts',(0.775962801882669,0.319434907277167,
11.2866672191688));
#61393=CARTESIAN_POINT('Ctrl Pts',(0.813383183475106,0.636309800095206,
11.3527487599227));
#61394=CARTESIAN_POINT('Ctrl Pts',(0.836353845186878,0.79477268400084,11.4025713849577));
#61395=CARTESIAN_POINT('Ctrl Pts',(0.885532801701862,1.06847604194511,11.5330073325055));
#61396=CARTESIAN_POINT('Ctrl Pts',(0.909492919286399,1.18514270861178,11.6019904180251));
#61397=CARTESIAN_POINT('Ctrl Pts',(0.936125406440073,1.3,11.683495700499));
#61398=CARTESIAN_POINT('Ctrl Pts',(0.741659516280677,-1.30000000000028,
11.719723201728));
#61399=CARTESIAN_POINT('Ctrl Pts',(0.738012470505649,-1.18514270861197,
11.6339459053541));
#61400=CARTESIAN_POINT('Ctrl Pts',(0.735457044102349,-1.06847604194521,
11.5609770187778));
#61401=CARTESIAN_POINT('Ctrl Pts',(0.732075357025825,-0.794772684000851,
11.421994282357));
#61402=CARTESIAN_POINT('Ctrl Pts',(0.730851239620765,-0.636309800095197,
11.368060793598));
#61403=CARTESIAN_POINT('Ctrl Pts',(0.736764158587381,-0.319434907277159,
11.2939064508864));
#61404=CARTESIAN_POINT('Ctrl Pts',(0.741012286627639,-0.158333333333332,
11.2762150307074));
#61405=CARTESIAN_POINT('Ctrl Pts',(0.76116978437262,0.158333333333334,11.2724808787964));
#61406=CARTESIAN_POINT('Ctrl Pts',(0.77596280188267,0.319434907277167,11.2866672191688));
#61407=CARTESIAN_POINT('Ctrl Pts',(0.813383183475107,0.636309800095206,
11.3527487599227));
#61408=CARTESIAN_POINT('Ctrl Pts',(0.836353845186879,0.79477268400084,11.4025713849577));
#61409=CARTESIAN_POINT('Ctrl Pts',(0.885532801702161,1.06847604194677,11.5330073325063));
#61410=CARTESIAN_POINT('Ctrl Pts',(0.90949291928707,1.18514270861505,11.601990418027));
#61411=CARTESIAN_POINT('Ctrl Pts',(0.936125406441193,1.30000000000483,11.6834957005024));
#61412=CARTESIAN_POINT('Ctrl Pts',(0.739042042488344,-1.30000000000028,
11.7249376165698));
#61413=CARTESIAN_POINT('Ctrl Pts',(0.735823583834715,-1.18514270861197,
11.6390010597618));
#61414=CARTESIAN_POINT('Ctrl Pts',(0.733297050684359,-1.06847604194521,
11.5658948972));
#61415=CARTESIAN_POINT('Ctrl Pts',(0.729058740007599,-0.794772684000851,
11.4266458142653));
#61416=CARTESIAN_POINT('Ctrl Pts',(0.725405994775785,-0.636309800095197,
11.3725700581163));
#61417=CARTESIAN_POINT('Ctrl Pts',(0.73013754978232,-0.319434907277159,
11.2983241249589));
#61418=CARTESIAN_POINT('Ctrl Pts',(0.734740249452905,-0.158333333333332,
11.2807133567046));
#61419=CARTESIAN_POINT('Ctrl Pts',(0.755052561493668,0.158333333333334,
11.2770101909005));
#61420=CARTESIAN_POINT('Ctrl Pts',(0.769831695225161,0.319434907277167,
11.2911645144203));
#61421=CARTESIAN_POINT('Ctrl Pts',(0.808370175300976,0.636309800095206,
11.3573648124169));
#61422=CARTESIAN_POINT('Ctrl Pts',(0.833047452158995,0.79477268400084,11.4073026355546));
#61423=CARTESIAN_POINT('Ctrl Pts',(0.883185362981537,1.06847604194677,11.5380010488157));
#61424=CARTESIAN_POINT('Ctrl Pts',(0.907329875011758,1.18514270861505,11.607121446575));
#61425=CARTESIAN_POINT('Ctrl Pts',(0.933916055269645,1.30000000000483,11.6887877418462));
#61426=CARTESIAN_POINT('Ctrl Pts',(0.736513353027043,-1.30000000000024,
11.7335029101657));
#61427=CARTESIAN_POINT('Ctrl Pts',(0.734197104083671,-1.18514270861194,
11.6485493198283));
#61428=CARTESIAN_POINT('Ctrl Pts',(0.731891266475708,-1.06847604194518,
11.5761286952239));
#61429=CARTESIAN_POINT('Ctrl Pts',(0.726588372587658,-0.79477268400083,
11.4377762227459));
#61430=CARTESIAN_POINT('Ctrl Pts',(0.719179900276991,-0.636309800095178,
11.3832624369924));
#61431=CARTESIAN_POINT('Ctrl Pts',(0.722022671202612,-0.319434907277149,
11.3088658603034));
#61432=CARTESIAN_POINT('Ctrl Pts',(0.726936954002692,-0.158333333333327,
11.2908872748991));
#61433=CARTESIAN_POINT('Ctrl Pts',(0.747449048780318,0.15833333333333,11.2872075458618));
#61434=CARTESIAN_POINT('Ctrl Pts',(0.762206183434706,0.319434907277157,
11.3017933991775));
#61435=CARTESIAN_POINT('Ctrl Pts',(0.802857471827774,0.636309800095187,
11.3681100406464));
#61436=CARTESIAN_POINT('Ctrl Pts',(0.831207002399099,0.794772684000817,
11.4183174781789));
#61437=CARTESIAN_POINT('Ctrl Pts',(0.882448094814532,1.06847604194674,11.5481255882124));
#61438=CARTESIAN_POINT('Ctrl Pts',(0.906391184552781,1.18514270861501,11.6166006607166));
#61439=CARTESIAN_POINT('Ctrl Pts',(0.932096993792065,1.30000000000479,11.6973616847556));
#61440=CARTESIAN_POINT('Ctrl Pts',(0.734690372091587,-1.30000000000024,
11.7455625251118));
#61441=CARTESIAN_POINT('Ctrl Pts',(0.733386866582579,-1.18514270861193,
11.6632066715271));
#61442=CARTESIAN_POINT('Ctrl Pts',(0.731407157793679,-1.06847604194518,
11.5926822187035));
#61443=CARTESIAN_POINT('Ctrl Pts',(0.725271469601385,-0.794772684000829,
11.4570895269343));
#61444=CARTESIAN_POINT('Ctrl Pts',(0.714394232863423,-0.636309800095177,
11.4020845254731));
#61445=CARTESIAN_POINT('Ctrl Pts',(0.7152493773471,-0.319434907277149,11.3277048294426));
#61446=CARTESIAN_POINT('Ctrl Pts',(0.71994876732749,-0.158333333333327,
11.3087599499422));
#61447=CARTESIAN_POINT('Ctrl Pts',(0.740554013134365,0.158333333333329,
11.3050802735153));
#61448=CARTESIAN_POINT('Ctrl Pts',(0.755401586135559,0.319434907277157,
11.3206828608572));
#61449=CARTESIAN_POINT('Ctrl Pts',(0.798673489649781,0.636309800095186,
11.3868800934896));
#61450=CARTESIAN_POINT('Ctrl Pts',(0.831837381161029,0.794772684000816,
11.437299798421));
#61451=CARTESIAN_POINT('Ctrl Pts',(0.883912658960803,1.06847604194674,11.5643693378906));
#61452=CARTESIAN_POINT('Ctrl Pts',(0.907206670173654,1.18514270861501,11.6310263922609));
#61453=CARTESIAN_POINT('Ctrl Pts',(0.931253234418874,1.30000000000479,11.7093368057551));
#61454=CARTESIAN_POINT('Ctrl Pts',(0.732507359893536,-1.3000000000002,11.7573468723062));
#61455=CARTESIAN_POINT('Ctrl Pts',(0.731446973883555,-1.18514270861191,
11.6773389107016));
#61456=CARTESIAN_POINT('Ctrl Pts',(0.729521126215045,-1.06847604194515,
11.6085578501234));
#61457=CARTESIAN_POINT('Ctrl Pts',(0.723072643270074,-0.794772684000809,
11.4755962278889));
#61458=CARTESIAN_POINT('Ctrl Pts',(0.711265049464907,-0.636309800095161,
11.4203598204888));
#61459=CARTESIAN_POINT('Ctrl Pts',(0.711336217967816,-0.31943490727714,
11.3461817951623));
#61460=CARTESIAN_POINT('Ctrl Pts',(0.715519917280257,-0.158333333333323,
11.3264634689159));
#61461=CARTESIAN_POINT('Ctrl Pts',(0.736192836746224,0.158333333333325,
11.3227634990918));
#61462=CARTESIAN_POINT('Ctrl Pts',(0.751417880673255,0.319434907277149,
11.3391299261724));
#61463=CARTESIAN_POINT('Ctrl Pts',(0.796030996572588,0.63630980009517,11.405062384505));
#61464=CARTESIAN_POINT('Ctrl Pts',(0.831284152871013,0.794772684000795,
11.4556021487431));
#61465=CARTESIAN_POINT('Ctrl Pts',(0.88380018897958,1.06847604194671,11.5800628855438));
#61466=CARTESIAN_POINT('Ctrl Pts',(0.90684379510631,1.18514270861498,11.6450189495381));
#61467=CARTESIAN_POINT('Ctrl Pts',(0.930198761239113,1.30000000000475,11.72105663629));
#61468=CARTESIAN_POINT('Ctrl Pts',(0.729739714965373,-1.30000000000017,
11.772078421086));
#61469=CARTESIAN_POINT('Ctrl Pts',(0.728627363429549,-1.18514270861187,
11.6948641909879));
#61470=CARTESIAN_POINT('Ctrl Pts',(0.72679940596954,-1.06847604194513,11.6281040130364));
#61471=CARTESIAN_POINT('Ctrl Pts',(0.720923265713938,-0.794772684000789,
11.4980255984249));
#61472=CARTESIAN_POINT('Ctrl Pts',(0.710628506046623,-0.636309800095146,
11.4420613460075));
#61473=CARTESIAN_POINT('Ctrl Pts',(0.710519142033698,-0.319434907277133,
11.3679189145324));
#61474=CARTESIAN_POINT('Ctrl Pts',(0.712895820440734,-0.15833333333332,
11.3474097803368));
#61475=CARTESIAN_POINT('Ctrl Pts',(0.733068591135251,0.158333333333322,
11.3437410226042));
#61476=CARTESIAN_POINT('Ctrl Pts',(0.748783293766575,0.319434907277142,
11.3610032250158));
#61477=CARTESIAN_POINT('Ctrl Pts',(0.794222780061106,0.636309800095155,
11.4268134320641));
#61478=CARTESIAN_POINT('Ctrl Pts',(0.830997222534945,0.794772684000776,
11.4777581767203));
#61479=CARTESIAN_POINT('Ctrl Pts',(0.883398438514725,1.06847604194668,11.5993299343026));
#61480=CARTESIAN_POINT('Ctrl Pts',(0.905989964443896,1.18514270861495,11.6623326059402));
#61481=CARTESIAN_POINT('Ctrl Pts',(0.92849047156083,1.30000000000472,11.7357140400351));
#61482=CARTESIAN_POINT('Ctrl Pts',(0.726871111169889,-1.30000000000014,
11.7854327933036));
#61483=CARTESIAN_POINT('Ctrl Pts',(0.725662375630626,-1.18514270861184,
11.7109232510307));
#61484=CARTESIAN_POINT('Ctrl Pts',(0.723931742859821,-1.0684760419451,11.6461298391096));
#61485=CARTESIAN_POINT('Ctrl Pts',(0.718727947937321,-0.79477268400077,
11.5188903005118));
#61486=CARTESIAN_POINT('Ctrl Pts',(0.70996917089403,-0.636309800095129,
11.4623191156996));
#61487=CARTESIAN_POINT('Ctrl Pts',(0.710300254588474,-0.319434907277125,
11.3882293156305));
#61488=CARTESIAN_POINT('Ctrl Pts',(0.711401496061413,-0.158333333333315,
11.3669370146061));
#61489=CARTESIAN_POINT('Ctrl Pts',(0.732257858090713,0.158333333333317,
11.3631717685982));
#61490=CARTESIAN_POINT('Ctrl Pts',(0.750292771558832,0.319434907277133,
11.3810603770313));
#61491=CARTESIAN_POINT('Ctrl Pts',(0.795948533589905,0.636309800095138,
11.4467441838119));
#61492=CARTESIAN_POINT('Ctrl Pts',(0.830900527909714,0.794772684000756,
11.498364921461));
#61493=CARTESIAN_POINT('Ctrl Pts',(0.882259193644855,1.06847604194666,11.617186409127));
#61494=CARTESIAN_POINT('Ctrl Pts',(0.90450231688194,1.18514270861492,11.6782740666674));
#61495=CARTESIAN_POINT('Ctrl Pts',(0.926757299985315,1.30000000000469,11.7490159625073));
#61496=CARTESIAN_POINT('Ctrl Pts',(0.724391632493098,-1.30000000000012,
11.7943012189908));
#61497=CARTESIAN_POINT('Ctrl Pts',(0.723101127419453,-1.18514270861183,
11.7215140260944));
#61498=CARTESIAN_POINT('Ctrl Pts',(0.72144951393426,-1.06847604194509,11.6579705374978));
#61499=CARTESIAN_POINT('Ctrl Pts',(0.716799723709153,-0.79477268400076,
11.5325271731377));
#61500=CARTESIAN_POINT('Ctrl Pts',(0.70905911646003,-0.636309800095122,
11.4755695176922));
#61501=CARTESIAN_POINT('Ctrl Pts',(0.710251122888309,-0.319434907277121,
11.4014618232877));
#61502=CARTESIAN_POINT('Ctrl Pts',(0.711503517432686,-0.158333333333314,
11.3795871437005));
#61503=CARTESIAN_POINT('Ctrl Pts',(0.732900309736102,0.158333333333316,
11.3757416690285));
#61504=CARTESIAN_POINT('Ctrl Pts',(0.751632512409751,0.31943490727713,11.3940739107996));
#61505=CARTESIAN_POINT('Ctrl Pts',(0.796900770990882,0.636309800095131,
11.4597313859243));
#61506=CARTESIAN_POINT('Ctrl Pts',(0.83033283835543,0.794772684000747,11.5118499896394));
#61507=CARTESIAN_POINT('Ctrl Pts',(0.881120250462187,1.06847604194664,11.6289323109164));
#61508=CARTESIAN_POINT('Ctrl Pts',(0.903323722379641,1.18514270861491,11.6887900188793));
#61509=CARTESIAN_POINT('Ctrl Pts',(0.925746677372449,1.30000000000468,11.7578248362514));
#61510=CARTESIAN_POINT('Ctrl Pts',(0.722742798682041,-1.30000000000012,
11.8002248077556));
#61511=CARTESIAN_POINT('Ctrl Pts',(0.721419566753041,-1.18514270861183,
11.7286007197735));
#61512=CARTESIAN_POINT('Ctrl Pts',(0.719837963986194,-1.06847604194509,
11.6659004086064));
#61513=CARTESIAN_POINT('Ctrl Pts',(0.715587256873898,-0.79477268400076,
11.5416658562942));
#61514=CARTESIAN_POINT('Ctrl Pts',(0.708530478596676,-0.636309800095122,
11.4844419155667));
#61515=CARTESIAN_POINT('Ctrl Pts',(0.710307727169727,-0.319434907277121,
11.4103142310288));
#61516=CARTESIAN_POINT('Ctrl Pts',(0.711734427886754,-0.158333333333314,
11.3880287945659));
#61517=CARTESIAN_POINT('Ctrl Pts',(0.73334722574718,0.158333333333316,11.3841478302049));
#61518=CARTESIAN_POINT('Ctrl Pts',(0.752177487683406,0.319434907277129,
11.4028351922547));
#61519=CARTESIAN_POINT('Ctrl Pts',(0.797185690872596,0.636309800095131,
11.468481405373));
#61520=CARTESIAN_POINT('Ctrl Pts',(0.83004512865742,0.794772684000747,11.5208842267609));
#61521=CARTESIAN_POINT('Ctrl Pts',(0.880500610743032,1.06847604194664,11.6367846006553));
#61522=CARTESIAN_POINT('Ctrl Pts',(0.902624193344047,1.18514270861491,11.6958162840945));
#61523=CARTESIAN_POINT('Ctrl Pts',(0.925031049910914,1.30000000000467,11.7637106736459));
#61524=CARTESIAN_POINT('Ctrl Pts',(0.71994117055138,-1.30000000000009,11.8105870027124));
#61525=CARTESIAN_POINT('Ctrl Pts',(0.718688939033695,-1.18514270861181,
11.740999718903));
#61526=CARTESIAN_POINT('Ctrl Pts',(0.717294270598105,-1.06847604194506,
11.6797778294328));
#61527=CARTESIAN_POINT('Ctrl Pts',(0.71374324973466,-0.794772684000742,
11.557668751774));
#61528=CARTESIAN_POINT('Ctrl Pts',(0.707595361315513,-0.636309800095109,
11.4999959843807));
#61529=CARTESIAN_POINT('Ctrl Pts',(0.71031903400796,-0.319434907277115,
11.4258370640626));
#61530=CARTESIAN_POINT('Ctrl Pts',(0.712311439868488,-0.15833333333331,
11.4027989395063));
#61531=CARTESIAN_POINT('Ctrl Pts',(0.734014976729677,0.158333333333312,
11.3988955011669));
#61532=CARTESIAN_POINT('Ctrl Pts',(0.752221442724715,0.319434907277122,
11.4183153622965));
#61533=CARTESIAN_POINT('Ctrl Pts',(0.796771206188982,0.636309800095118,
11.4839423790098));
#61534=CARTESIAN_POINT('Ctrl Pts',(0.829569489541166,0.794772684000731,
11.5367202862584));
#61535=CARTESIAN_POINT('Ctrl Pts',(0.879553043281544,1.06847604194662,11.6505216761042));
#61536=CARTESIAN_POINT('Ctrl Pts',(0.901425593708693,1.18514270861488,11.7081115434555));
#61537=CARTESIAN_POINT('Ctrl Pts',(0.923534666221812,1.30000000000465,11.7740308732505));
#61538=CARTESIAN_POINT('Ctrl Pts',(0.715773049841682,-1.30000000000009,
11.8312567595427));
#61539=CARTESIAN_POINT('Ctrl Pts',(0.713894702046613,-1.1851427086118,11.7657401096002));
#61540=CARTESIAN_POINT('Ctrl Pts',(0.712263951197079,-1.06847604194506,
11.7074819432039));
#61541=CARTESIAN_POINT('Ctrl Pts',(0.709068588979851,-0.794772684000739,
11.5896624733687));
#61542=CARTESIAN_POINT('Ctrl Pts',(0.704527181281509,-0.636309800095106,
11.531156225655));
#61543=CARTESIAN_POINT('Ctrl Pts',(0.708833282403318,-0.319434907277113,
11.4569945983025));
#61544=CARTESIAN_POINT('Ctrl Pts',(0.711666493724411,-0.15833333333331,
11.4325322881426));
#61545=CARTESIAN_POINT('Ctrl Pts',(0.734429330765286,0.158333333333312,
11.4284919162156));
#61546=CARTESIAN_POINT('Ctrl Pts',(0.753655173885053,0.319434907277122,
11.4490887889334));
#61547=CARTESIAN_POINT('Ctrl Pts',(0.797148887319053,0.636309800095116,
11.5146641406369));
#61548=CARTESIAN_POINT('Ctrl Pts',(0.826817146073029,0.794772684000727,
11.5684948467983));
#61549=CARTESIAN_POINT('Ctrl Pts',(0.875521263709609,1.06847604194662,11.6781493133238));
#61550=CARTESIAN_POINT('Ctrl Pts',(0.897270371507951,1.18514270861487,11.7328314345891));
#61551=CARTESIAN_POINT('Ctrl Pts',(0.919686379245016,1.30000000000464,11.7947303216591));
#61552=CARTESIAN_POINT('Ctrl Pts',(0.708106339592663,-1.29999999999985,
11.8549337471632));
#61553=CARTESIAN_POINT('Ctrl Pts',(0.705716356639382,-1.18514270861158,
11.7940699885983));
#61554=CARTESIAN_POINT('Ctrl Pts',(0.704096117869523,-1.06847604194486,
11.7391945926482));
#61555=CARTESIAN_POINT('Ctrl Pts',(0.702131305233996,-0.794772684000595,
11.6262557658256));
#61556=CARTESIAN_POINT('Ctrl Pts',(0.700490171305661,-0.636309800094987,
11.5667529657947));
#61557=CARTESIAN_POINT('Ctrl Pts',(0.707123085947054,-0.319434907277052,
11.4925747952514));
#61558=CARTESIAN_POINT('Ctrl Pts',(0.710920992338189,-0.15833333333328,
11.466458146152));
#61559=CARTESIAN_POINT('Ctrl Pts',(0.734037344146519,0.158333333333282,
11.4623676047482));
#61560=CARTESIAN_POINT('Ctrl Pts',(0.752190621505164,0.319434907277065,
11.4845724982227));
#61561=CARTESIAN_POINT('Ctrl Pts',(0.795017414505158,0.636309800094999,
11.5500543566967));
#61562=CARTESIAN_POINT('Ctrl Pts',(0.824547896991247,0.794772684000577,
11.6047319280489));
#61563=CARTESIAN_POINT('Ctrl Pts',(0.872754551306088,1.06847604194641,11.7095502432165));
#61564=CARTESIAN_POINT('Ctrl Pts',(0.894271436335858,1.18514270861465,11.7609185955138));
#61565=CARTESIAN_POINT('Ctrl Pts',(0.91643833197493,1.3000000000044,11.8182833353734));
#61566=CARTESIAN_POINT('Ctrl Pts',(0.701392717589504,-1.29999999999977,
11.8785605604878));
#61567=CARTESIAN_POINT('Ctrl Pts',(0.698072695455552,-1.18514270861151,
11.8223399017));
#61568=CARTESIAN_POINT('Ctrl Pts',(0.696020255650023,-1.06847604194479,
11.7708544676842));
#61569=CARTESIAN_POINT('Ctrl Pts',(0.694207077867708,-0.794772684000542,
11.6628521319838));
#61570=CARTESIAN_POINT('Ctrl Pts',(0.694147020817013,-0.636309800094947,
11.6024830083094));
#61571=CARTESIAN_POINT('Ctrl Pts',(0.703048255663917,-0.319434907277033,
11.5283287199599));
#61572=CARTESIAN_POINT('Ctrl Pts',(0.7092636804318,-0.158333333333271,11.5005012358133));
#61573=CARTESIAN_POINT('Ctrl Pts',(0.733194250079355,0.158333333333273,
11.4963283081617));
#61574=CARTESIAN_POINT('Ctrl Pts',(0.75018486417955,0.319434907277045,11.5200944460579));
#61575=CARTESIAN_POINT('Ctrl Pts',(0.791504293676369,0.636309800094959,
11.585521497962));
#61576=CARTESIAN_POINT('Ctrl Pts',(0.819005278050289,0.794772684000529,
11.6411952916285));
#61577=CARTESIAN_POINT('Ctrl Pts',(0.866710872109081,1.06847604194635,11.7411747899911));
#61578=CARTESIAN_POINT('Ctrl Pts',(0.88844359663303,1.18514270861458,11.7891948061993));
#61579=CARTESIAN_POINT('Ctrl Pts',(0.91125906167919,1.30000000000432,11.8419574183797));
#61580=CARTESIAN_POINT('Ctrl Pts',(0.696379212651574,-1.29999999999974,
11.8962766909092));
#61581=CARTESIAN_POINT('Ctrl Pts',(0.692999191360036,-1.18514270861148,
11.8435384540665));
#61582=CARTESIAN_POINT('Ctrl Pts',(0.690970633093636,-1.06847604194477,
11.7945953930707));
#61583=CARTESIAN_POINT('Ctrl Pts',(0.689406407633882,-0.794772684000527,
11.6902947465732));
#61584=CARTESIAN_POINT('Ctrl Pts',(0.689712119805148,-0.636309800094934,
11.629249227579));
#61585=CARTESIAN_POINT('Ctrl Pts',(0.699298112195223,-0.319434907277026,
11.5551617154664));
#61586=CARTESIAN_POINT('Ctrl Pts',(0.706099181263705,-0.158333333333267,
11.5261610928535));
#61587=CARTESIAN_POINT('Ctrl Pts',(0.730556960302764,0.158333333333269,
11.5219451899244));
#61588=CARTESIAN_POINT('Ctrl Pts',(0.747648646203372,0.319434907277038,
11.5468243597819));
#61589=CARTESIAN_POINT('Ctrl Pts',(0.789032302044774,0.636309800094946,
11.61213199298));
#61590=CARTESIAN_POINT('Ctrl Pts',(0.816252297706209,0.794772684000512,
11.668461565255));
#61591=CARTESIAN_POINT('Ctrl Pts',(0.863996819850258,1.06847604194633,11.7647786583432));
#61592=CARTESIAN_POINT('Ctrl Pts',(0.885803182416638,1.18514270861455,11.8102911655351));
#61593=CARTESIAN_POINT('Ctrl Pts',(0.908749073021981,1.30000000000429,11.8596240792207));
#61594=CARTESIAN_POINT('Ctrl Pts',(0.690660095299648,-1.29999999999966,
11.9139835115398));
#61595=CARTESIAN_POINT('Ctrl Pts',(0.685682722076107,-1.18514270861141,
11.8647239191065));
#61596=CARTESIAN_POINT('Ctrl Pts',(0.682768533441947,-1.0684760419447,11.8183239634083));
#61597=CARTESIAN_POINT('Ctrl Pts',(0.680802543855727,-0.794772684000474,
11.7177371163932));
#61598=CARTESIAN_POINT('Ctrl Pts',(0.683350742237752,-0.636309800094896,
11.6560556065026));
#61599=CARTESIAN_POINT('Ctrl Pts',(0.694836451094066,-0.319434907277008,
11.5820281070802));
#61600=CARTESIAN_POINT('Ctrl Pts',(0.703081913914877,-0.158333333333258,
11.5517991314348));
#61601=CARTESIAN_POINT('Ctrl Pts',(0.728231769052573,0.15833333333326,11.5475366605752));
#61602=CARTESIAN_POINT('Ctrl Pts',(0.744790141058607,0.31943490727702,11.5735538840847));
#61603=CARTESIAN_POINT('Ctrl Pts',(0.785237694727035,0.636309800094909,
11.6387957268862));
#61604=CARTESIAN_POINT('Ctrl Pts',(0.810856804125816,0.794772684000465,
11.6958543568564));
#61605=CARTESIAN_POINT('Ctrl Pts',(0.858356073086245,1.06847604194626,11.7885319067558));
#61606=CARTESIAN_POINT('Ctrl Pts',(0.880405649972082,1.18514270861449,11.8315323060639));
#61607=CARTESIAN_POINT('Ctrl Pts',(0.903944130232002,1.30000000000422,11.87741642737));
#61608=CARTESIAN_POINT('Ctrl Pts',(0.684774161766043,-1.29999999999961,
11.9316792283627));
#61609=CARTESIAN_POINT('Ctrl Pts',(0.679670728815399,-1.18514270861137,
11.8858988962828));
#61610=CARTESIAN_POINT('Ctrl Pts',(0.676779668951229,-1.06847604194467,
11.8420404620596));
#61611=CARTESIAN_POINT('Ctrl Pts',(0.675211766723929,-0.794772684000448,
11.7451586736775));
#61612=CARTESIAN_POINT('Ctrl Pts',(0.678635652890764,-0.636309800094872,
11.682807341107));
#61613=CARTESIAN_POINT('Ctrl Pts',(0.690797413702307,-0.319434907276995,
11.6088645835443));
#61614=CARTESIAN_POINT('Ctrl Pts',(0.699162179082554,-0.158333333333252,
11.5774811768116));
#61615=CARTESIAN_POINT('Ctrl Pts',(0.724632526989099,0.158333333333254,
11.5731918390187));
#61616=CARTESIAN_POINT('Ctrl Pts',(0.741230482084265,0.319434907277007,
11.6003317903806));
#61617=CARTESIAN_POINT('Ctrl Pts',(0.781983986559276,0.636309800094885,
11.6654440165117));
#61618=CARTESIAN_POINT('Ctrl Pts',(0.807937356793683,0.794772684000434,
11.7231212970555));
#61619=CARTESIAN_POINT('Ctrl Pts',(0.855587165199985,1.06847604194622,11.812130964535));
#61620=CARTESIAN_POINT('Ctrl Pts',(0.877639911931404,1.18514270861444,11.8526284951903));
#61621=CARTESIAN_POINT('Ctrl Pts',(0.901119568934406,1.30000000000417,11.895094569582));
#61622=CARTESIAN_POINT('Ctrl Pts',(0.678549186698821,-1.29999999999946,
11.9493585018483));
#61623=CARTESIAN_POINT('Ctrl Pts',(0.672432041213187,-1.18514270861122,
11.9070486740622));
#61624=CARTESIAN_POINT('Ctrl Pts',(0.668959648382607,-1.06847604194454,
11.865729892223));
#61625=CARTESIAN_POINT('Ctrl Pts',(0.667047634008289,-0.79477268400035,
11.7725647547759));
#61626=CARTESIAN_POINT('Ctrl Pts',(0.671674453970411,-0.636309800094796,
11.7095875503082));
#61627=CARTESIAN_POINT('Ctrl Pts',(0.685080552577213,-0.319434907276958,
11.6357386986211));
#61628=CARTESIAN_POINT('Ctrl Pts',(0.694640062897662,-0.158333333333233,
11.6031714292693));
#61629=CARTESIAN_POINT('Ctrl Pts',(0.720646467007646,0.158333333333235,
11.5988554570619));
#61630=CARTESIAN_POINT('Ctrl Pts',(0.736905994278727,0.319434907276967,
11.6271197806948));
#61631=CARTESIAN_POINT('Ctrl Pts',(0.776854720427988,0.636309800094807,
11.6921507737362));
#61632=CARTESIAN_POINT('Ctrl Pts',(0.801120572561274,0.79477268400034,11.7505397288079));
#61633=CARTESIAN_POINT('Ctrl Pts',(0.84893651173128,1.0684760419461,11.8358910768284));
#61634=CARTESIAN_POINT('Ctrl Pts',(0.871504994914518,1.1851427086143,11.8738691384865));
#61635=CARTESIAN_POINT('Ctrl Pts',(0.895944212969302,1.30000000000401,11.9128798258235));
#61636=CARTESIAN_POINT('Ctrl Pts',(0.674222718308865,-1.29999999999937,
11.9640876094412));
#61637=CARTESIAN_POINT('Ctrl Pts',(0.666986355018664,-1.18514270861114,
11.9246619613613));
#61638=CARTESIAN_POINT('Ctrl Pts',(0.662836854551111,-1.06847604194446,
11.8854538539057));
#61639=CARTESIAN_POINT('Ctrl Pts',(0.660381949011449,-0.794772684000296,
11.7953778444889));
#61640=CARTESIAN_POINT('Ctrl Pts',(0.66609150822191,-0.636309800094752,
11.7318822817835));
#61641=CARTESIAN_POINT('Ctrl Pts',(0.68063358116873,-0.319434907276936,
11.6581096922817));
#61642=CARTESIAN_POINT('Ctrl Pts',(0.691415225026868,-0.158333333333222,
11.624551409228));
#61643=CARTESIAN_POINT('Ctrl Pts',(0.717918159526262,0.158333333333224,
11.6202170472644));
#61644=CARTESIAN_POINT('Ctrl Pts',(0.733451120016153,0.319434907276946,
11.6494425495418));
#61645=CARTESIAN_POINT('Ctrl Pts',(0.773277231328102,0.636309800094764,
11.7143831350432));
#61646=CARTESIAN_POINT('Ctrl Pts',(0.797580730757561,0.794772684000285,
11.7733006957295));
#61647=CARTESIAN_POINT('Ctrl Pts',(0.845788720600292,1.06847604194602,11.8555845497542));
#61648=CARTESIAN_POINT('Ctrl Pts',(0.868618068406382,1.18514270861422,11.8914654749949));
#61649=CARTESIAN_POINT('Ctrl Pts',(0.893409311497553,1.30000000000392,11.9276096939862));
#61650=CARTESIAN_POINT('Ctrl Pts',(0.667369721617846,-1.2999999999993,11.9817468175657));
#61651=CARTESIAN_POINT('Ctrl Pts',(0.659742133214706,-1.18514270861108,
11.9457950770222));
#61652=CARTESIAN_POINT('Ctrl Pts',(0.655434396033206,-1.06847604194441,
11.9091279977393));
#61653=CARTESIAN_POINT('Ctrl Pts',(0.653152181840017,-0.794772684000256,
11.8227671337809));
#61654=CARTESIAN_POINT('Ctrl Pts',(0.659921427366295,-0.636309800094721,
11.7586271846953));
#61655=CARTESIAN_POINT('Ctrl Pts',(0.675123639591609,-0.319434907276921,
11.684961005829));
#61656=CARTESIAN_POINT('Ctrl Pts',(0.686172569068147,-0.158333333333214,
11.6502500215863));
#61657=CARTESIAN_POINT('Ctrl Pts',(0.712534168854585,0.158333333333216,
11.6459109667399));
#61658=CARTESIAN_POINT('Ctrl Pts',(0.727362482686232,0.319434907276929,
11.6762765482347));
#61659=CARTESIAN_POINT('Ctrl Pts',(0.766843550399096,0.636309800094731,
11.7411173150198));
#61660=CARTESIAN_POINT('Ctrl Pts',(0.790971787147075,0.794772684000247,
11.8006841259155));
#61661=CARTESIAN_POINT('Ctrl Pts',(0.839696979707915,1.06847604194597,11.8793011898733));
#61662=CARTESIAN_POINT('Ctrl Pts',(0.862932260753159,1.18514270861416,11.9126710725441));
#61663=CARTESIAN_POINT('Ctrl Pts',(0.888311492430216,1.30000000000386,11.9453804239475));
#61664=CARTESIAN_POINT('Ctrl Pts',(0.662335531550092,-1.29999999999911,
11.99643968074));
#61665=CARTESIAN_POINT('Ctrl Pts',(0.652920552658503,-1.18514270861091,
11.9633444972165));
#61666=CARTESIAN_POINT('Ctrl Pts',(0.647516901475013,-1.06847604194426,
11.9287737920991));
#61667=CARTESIAN_POINT('Ctrl Pts',(0.644300355713498,-0.794772684000144,
11.8454997973729));
#61668=CARTESIAN_POINT('Ctrl Pts',(0.652833902539925,-0.63630980009463,
11.7808905622974));
#61669=CARTESIAN_POINT('Ctrl Pts',(0.66948372337528,-0.319434907276874,
11.7073339904357));
#61670=CARTESIAN_POINT('Ctrl Pts',(0.681622795171332,-0.158333333333192,
11.6716547229497));
#61671=CARTESIAN_POINT('Ctrl Pts',(0.709092228259606,0.158333333333194,
11.6672915509916));
#61672=CARTESIAN_POINT('Ctrl Pts',(0.724480061053731,0.319434907276885,
11.6985662875476));
#61673=CARTESIAN_POINT('Ctrl Pts',(0.76366643224308,0.636309800094642,11.7633196375378));
#61674=CARTESIAN_POINT('Ctrl Pts',(0.785832472357193,0.794772684000132,
11.823476606662));
#61675=CARTESIAN_POINT('Ctrl Pts',(0.834828940803699,1.06847604194582,11.8990326400059));
#61676=CARTESIAN_POINT('Ctrl Pts',(0.858651545639185,1.18514270861399,11.9302973597015));
#61677=CARTESIAN_POINT('Ctrl Pts',(0.885087999617585,1.30000000000367,11.9601213918847));
#61678=CARTESIAN_POINT('Ctrl Pts',(0.654500613520237,-1.29999999999899,
12.0170141288364));
#61679=CARTESIAN_POINT('Ctrl Pts',(0.644565540455188,-1.1851427086108,11.9879631922512));
#61680=CARTESIAN_POINT('Ctrl Pts',(0.63877654301765,-1.06847604194416,11.9563506643837));
#61681=CARTESIAN_POINT('Ctrl Pts',(0.634981064971107,-0.794772684000068,
11.8774016126389));
#61682=CARTESIAN_POINT('Ctrl Pts',(0.643084042498312,-0.636309800094567,
11.8120386328918));
#61683=CARTESIAN_POINT('Ctrl Pts',(0.660652874351986,-0.319434907276841,
11.7386122902342));
#61684=CARTESIAN_POINT('Ctrl Pts',(0.675025400252646,-0.158333333333176,
11.7016017791411));
#61685=CARTESIAN_POINT('Ctrl Pts',(0.702984679232211,0.158333333333178,
11.6972430066232));
#61686=CARTESIAN_POINT('Ctrl Pts',(0.716772423379789,0.319434907276852,
11.7298538736244));
#61687=CARTESIAN_POINT('Ctrl Pts',(0.755745225337548,0.636309800094577,
11.7944849629586));
#61688=CARTESIAN_POINT('Ctrl Pts',(0.778484066973515,0.794772684000052,
11.8553751368386));
#61689=CARTESIAN_POINT('Ctrl Pts',(0.828258808440125,1.06847604194571,11.9266539771194));
#61690=CARTESIAN_POINT('Ctrl Pts',(0.852499600637966,1.18514270861387,11.9549949065323));
#61691=CARTESIAN_POINT('Ctrl Pts',(0.879435543788526,1.30000000000354,11.9808227965415));
#61692=CARTESIAN_POINT('Ctrl Pts',(0.648585099106898,-1.29999999999886,
12.0346262810387));
#61693=CARTESIAN_POINT('Ctrl Pts',(0.63671231292895,-1.18514270861068,12.0089949224276));
#61694=CARTESIAN_POINT('Ctrl Pts',(0.629749814138102,-1.06847604194405,
11.9798926459143));
#61695=CARTESIAN_POINT('Ctrl Pts',(0.625008795251963,-0.794772683999986,
11.9046420505691));
#61696=CARTESIAN_POINT('Ctrl Pts',(0.635421531598707,-0.636309800094504,
11.8387169067579));
#61697=CARTESIAN_POINT('Ctrl Pts',(0.654077321348798,-0.319434907276811,
11.7654365401314));
#61698=CARTESIAN_POINT('Ctrl Pts',(0.668786882007543,-0.15833333333316,
11.7272830225411));
#61699=CARTESIAN_POINT('Ctrl Pts',(0.696966209368503,0.158333333333162,
11.722917458364));
#61700=CARTESIAN_POINT('Ctrl Pts',(0.710403034558743,0.319434907276821,
11.7566401387454));
#61701=CARTESIAN_POINT('Ctrl Pts',(0.749213605152048,0.636309800094515,
11.8211611219402));
#61702=CARTESIAN_POINT('Ctrl Pts',(0.771463328588758,0.794772683999976,
11.8827097085051));
#61703=CARTESIAN_POINT('Ctrl Pts',(0.821963976608028,1.0684760419456,11.9503235628632));
#61704=CARTESIAN_POINT('Ctrl Pts',(0.846789883164354,1.18514270861375,11.976153865767));
#61705=CARTESIAN_POINT('Ctrl Pts',(0.874581836982727,1.30000000000341,11.9985469393629));
#61706=CARTESIAN_POINT('Ctrl Pts',(0.639457684724997,-1.29999999999865,
12.055133698939));
#61707=CARTESIAN_POINT('Ctrl Pts',(0.62674097457832,-1.18514270861049,12.0335190159486));
#61708=CARTESIAN_POINT('Ctrl Pts',(0.619210639483942,-1.06847604194388,
12.0073589062376));
#61709=CARTESIAN_POINT('Ctrl Pts',(0.613795622879141,-0.794772683999862,
11.9364229744589));
#61710=CARTESIAN_POINT('Ctrl Pts',(0.624369194200539,-0.636309800094403,
11.8697763172489));
#61711=CARTESIAN_POINT('Ctrl Pts',(0.644000269036368,-0.31943490727676,
11.7966569147437));
#61712=CARTESIAN_POINT('Ctrl Pts',(0.660203030149533,-0.158333333333135,
11.7572028730154));
#61713=CARTESIAN_POINT('Ctrl Pts',(0.689570015141949,0.158333333333137,
11.7528497218579));
#61714=CARTESIAN_POINT('Ctrl Pts',(0.703522155079055,0.319434907276769,
11.7878781852481));
#61715=CARTESIAN_POINT('Ctrl Pts',(0.742104585901675,0.636309800094413,
11.8522780612349));
#61716=CARTESIAN_POINT('Ctrl Pts',(0.762340533905654,0.794772683999849,
11.914587337957));
#61717=CARTESIAN_POINT('Ctrl Pts',(0.813454919682806,1.06847604194544,11.9779296921709));
#61718=CARTESIAN_POINT('Ctrl Pts',(0.839095253705589,1.18514270861357,12.0008344718056));
#61719=CARTESIAN_POINT('Ctrl Pts',(0.86825039812271,1.30000000000321,12.0192254730012));
#61720=CARTESIAN_POINT('Ctrl Pts',(0.634180702243894,-1.29999999999847,
12.0697751580724));
#61721=CARTESIAN_POINT('Ctrl Pts',(0.619712411140887,-1.18514270861032,
12.05099069487));
#61722=CARTESIAN_POINT('Ctrl Pts',(0.611114313461518,-1.06847604194372,
12.0269109747433));
#61723=CARTESIAN_POINT('Ctrl Pts',(0.604812308915402,-0.794772683999744,
11.9590489013119));
#61724=CARTESIAN_POINT('Ctrl Pts',(0.617553440481668,-0.636309800094312,
11.8919593671572));
#61725=CARTESIAN_POINT('Ctrl Pts',(0.637867983997188,-0.319434907276715,
11.8189734347907));
#61726=CARTESIAN_POINT('Ctrl Pts',(0.654017685311995,-0.158333333333112,
11.77856682571));
#61727=CARTESIAN_POINT('Ctrl Pts',(0.683031161223074,0.158333333333114,
11.7742147812699));
#61728=CARTESIAN_POINT('Ctrl Pts',(0.695951979822126,0.319434907276722,
11.8101765875292));
#61729=CARTESIAN_POINT('Ctrl Pts',(0.734619603171526,0.636309800094321,
11.8744866608729));
#61730=CARTESIAN_POINT('Ctrl Pts',(0.755655244379573,0.794772683999735,
11.9373347308432));
#61731=CARTESIAN_POINT('Ctrl Pts',(0.807961459846468,1.06847604194528,11.9976281313998));
#61732=CARTESIAN_POINT('Ctrl Pts',(0.834216491313751,1.1851427086134,12.0184458455809));
#61733=CARTESIAN_POINT('Ctrl Pts',(0.864085131708817,1.30000000000302,12.0339824949326));
#61734=CARTESIAN_POINT('Ctrl Pts',(0.63020141310794,-1.2999999999984,12.0800255317113));
#61735=CARTESIAN_POINT('Ctrl Pts',(0.615033907744602,-1.18514270861026,
12.0632398912468));
#61736=CARTESIAN_POINT('Ctrl Pts',(0.605937831805631,-1.06847604194367,
12.0406238643243));
#61737=CARTESIAN_POINT('Ctrl Pts',(0.598950293278431,-0.794772683999704,
11.9749069587294));
#61738=CARTESIAN_POINT('Ctrl Pts',(0.611717138522065,-0.636309800094279,
11.9074519874911));
#61739=CARTESIAN_POINT('Ctrl Pts',(0.632489467969168,-0.319434907276699,
11.8345501240997));
#61740=CARTESIAN_POINT('Ctrl Pts',(0.649593654306062,-0.158333333333104,
11.7935078738823));
#61741=CARTESIAN_POINT('Ctrl Pts',(0.679139447618656,0.158333333333106,
11.7891681687253));
#61742=CARTESIAN_POINT('Ctrl Pts',(0.691964698903671,0.319434907276706,
11.8257791539708));
#61743=CARTESIAN_POINT('Ctrl Pts',(0.73059356723184,0.636309800094288,11.8900278511768));
#61744=CARTESIAN_POINT('Ctrl Pts',(0.751111017380349,0.794772683999695,
11.9532534353523));
#61745=CARTESIAN_POINT('Ctrl Pts',(0.80386579375481,1.06847604194523,12.0114142945674));
#61746=CARTESIAN_POINT('Ctrl Pts',(0.830518240483384,1.18514270861334,12.0307719737918));
#61747=CARTESIAN_POINT('Ctrl Pts',(0.860987546004967,1.30000000000295,12.0443116513584));
#61748=CARTESIAN_POINT('Ctrl Pts',(0.627856112644543,-1.29999999999838,
12.0858800499617));
#61749=CARTESIAN_POINT('Ctrl Pts',(0.612387208051074,-1.18514270861024,
12.0702385265224));
#61750=CARTESIAN_POINT('Ctrl Pts',(0.603066085512306,-1.06847604194365,
12.0484598929655));
#61751=CARTESIAN_POINT('Ctrl Pts',(0.595735034169528,-0.794772683999692,
11.9839689405519));
#61752=CARTESIAN_POINT('Ctrl Pts',(0.60841018552264,-0.63630980009427,11.9163008622495));
#61753=CARTESIAN_POINT('Ctrl Pts',(0.629369647417197,-0.319434907276694,
11.8434463136223));
#61754=CARTESIAN_POINT('Ctrl Pts',(0.64696106719286,-0.158333333333102,
11.8020427839178));
#61755=CARTESIAN_POINT('Ctrl Pts',(0.676787204160346,0.158333333333104,
11.7977112676138));
#61756=CARTESIAN_POINT('Ctrl Pts',(0.689594301071588,0.319434907276702,
11.8346940175172));
#61757=CARTESIAN_POINT('Ctrl Pts',(0.728222636350922,0.63630980009428,11.8989074026291));
#61758=CARTESIAN_POINT('Ctrl Pts',(0.748448052983879,0.794772683999683,
11.9623467578494));
#61759=CARTESIAN_POINT('Ctrl Pts',(0.801484476416064,1.06847604194521,12.0192889798408));
#61760=CARTESIAN_POINT('Ctrl Pts',(0.828377630920278,1.18514270861332,12.0378127284722));
#61761=CARTESIAN_POINT('Ctrl Pts',(0.859206437417904,1.30000000000294,12.050212047752));
#61762=CARTESIAN_POINT('Ctrl Pts',(0.624161576291421,-1.29999999999834,
12.0946516707519));
#61763=CARTESIAN_POINT('Ctrl Pts',(0.608111877397449,-1.18514270861021,
12.0807179966861));
#61764=CARTESIAN_POINT('Ctrl Pts',(0.598390121382353,-1.06847604194362,
12.0601912051343));
#61765=CARTESIAN_POINT('Ctrl Pts',(0.59054973410769,-0.794772683999669,
11.9975387899378));
#61766=CARTESIAN_POINT('Ctrl Pts',(0.603378336192844,-0.636309800094251,
11.9295685320289));
#61767=CARTESIAN_POINT('Ctrl Pts',(0.624724051565348,-0.319434907276684,
11.8567909971145));
#61768=CARTESIAN_POINT('Ctrl Pts',(0.64299874908432,-0.158333333333097,
11.814841382019));
#61769=CARTESIAN_POINT('Ctrl Pts',(0.673200200924868,0.158333333333099,
11.8105216849394));
#61770=CARTESIAN_POINT('Ctrl Pts',(0.685901221470102,0.319434907276692,
11.8480620242187));
#61771=CARTESIAN_POINT('Ctrl Pts',(0.724496564371522,0.63630980009426,11.9122231126468));
#61772=CARTESIAN_POINT('Ctrl Pts',(0.744303193228928,0.794772683999659,
11.9759842154236));
#61773=CARTESIAN_POINT('Ctrl Pts',(0.797802730050058,1.06847604194518,12.0310995623443));
#61774=CARTESIAN_POINT('Ctrl Pts',(0.825082932547686,1.18514270861328,12.0483728427296));
#61775=CARTESIAN_POINT('Ctrl Pts',(0.856485370406105,1.30000000000289,12.0590620120429));
#61776=CARTESIAN_POINT('Ctrl Pts',(0.619749336779534,-1.29999999999813,
12.104870548424));
#61777=CARTESIAN_POINT('Ctrl Pts',(0.602682915760704,-1.18514270861001,
12.0929135692186));
#61778=CARTESIAN_POINT('Ctrl Pts',(0.592312141089411,-1.06847604194344,
12.0738387098464));
#61779=CARTESIAN_POINT('Ctrl Pts',(0.583821859454634,-0.794772683999537,
12.0133282416719));
#61780=CARTESIAN_POINT('Ctrl Pts',(0.597458428936834,-0.636309800094145,
11.9450334137923));
#61781=CARTESIAN_POINT('Ctrl Pts',(0.619488733694328,-0.319434907276631,
11.8723573671982));
#61782=CARTESIAN_POINT('Ctrl Pts',(0.638601914260369,-0.158333333333071,
11.8297699041693));
#61783=CARTESIAN_POINT('Ctrl Pts',(0.668949937282336,0.158333333333073,
11.8254615373418));
#61784=CARTESIAN_POINT('Ctrl Pts',(0.68092804808564,0.319434907276639,11.8636444166396));
#61785=CARTESIAN_POINT('Ctrl Pts',(0.719200496987211,0.636309800094155,
11.9277406171235));
#61786=CARTESIAN_POINT('Ctrl Pts',(0.738593692950098,0.794772683999528,
11.9918766932466));
#61787=CARTESIAN_POINT('Ctrl Pts',(0.792873086952508,1.068476041945,12.0448646804517));
#61788=CARTESIAN_POINT('Ctrl Pts',(0.820774824770173,1.18514270861309,12.0606821506067));
#61789=CARTESIAN_POINT('Ctrl Pts',(0.853082761991445,1.30000000000268,12.069380554654));
#61790=CARTESIAN_POINT('Ctrl Pts',(0.615467141218366,-1.29999999999805,
12.1150930403923));
#61791=CARTESIAN_POINT('Ctrl Pts',(0.597625820552847,-1.18514270860994,
12.1051224765165));
#61792=CARTESIAN_POINT('Ctrl Pts',(0.586724619994118,-1.06847604194338,
12.0875038092771));
#61793=CARTESIAN_POINT('Ctrl Pts',(0.577573731738714,-0.794772683999492,
12.0291325145843));
#61794=CARTESIAN_POINT('Ctrl Pts',(0.591441124832637,-0.636309800094109,
11.9604851530946));
#61795=CARTESIAN_POINT('Ctrl Pts',(0.614019250197833,-0.319434907276613,
11.8879041059066));
#61796=CARTESIAN_POINT('Ctrl Pts',(0.634168133697368,-0.158333333333062,
11.8446920128823));
#61797=CARTESIAN_POINT('Ctrl Pts',(0.664825533059683,0.158333333333064,
11.8403984497482));
#61798=CARTESIAN_POINT('Ctrl Pts',(0.676259290560238,0.319434907276621,
11.8792215022969));
#61799=CARTESIAN_POINT('Ctrl Pts',(0.714243429693531,0.636309800094118,
11.9432513509972));
#61800=CARTESIAN_POINT('Ctrl Pts',(0.73306672545194,0.794772683999482,12.007759507101));
#61801=CARTESIAN_POINT('Ctrl Pts',(0.78803548171108,1.06847604194494,12.058621077946));
#61802=CARTESIAN_POINT('Ctrl Pts',(0.816526615288474,1.18514270861302,12.0729840605242));
#61803=CARTESIAN_POINT('Ctrl Pts',(0.849714944651654,1.30000000000261,12.0796939362685));
#61804=CARTESIAN_POINT('Ctrl Pts',(0.612875854852303,-1.29999999999804,
12.120923162107));
#61805=CARTESIAN_POINT('Ctrl Pts',(0.594468444044198,-1.18514270860993,
12.1120779219025));
#61806=CARTESIAN_POINT('Ctrl Pts',(0.583206793009732,-1.06847604194337,
12.0952865642195));
#61807=CARTESIAN_POINT('Ctrl Pts',(0.573698260816,-0.794772683999482,12.0381380478815));
#61808=CARTESIAN_POINT('Ctrl Pts',(0.588052060272601,-0.636309800094101,
11.9693126236165));
#61809=CARTESIAN_POINT('Ctrl Pts',(0.61095813111931,-0.319434907276609,
11.8967910853841));
#61810=CARTESIAN_POINT('Ctrl Pts',(0.631389225007648,-0.15833333333306,
11.853210394178));
#61811=CARTESIAN_POINT('Ctrl Pts',(0.662219798857672,0.158333333333062,
11.8489248608128));
#61812=CARTESIAN_POINT('Ctrl Pts',(0.673542143115433,0.319434907276617,
11.8881199204326));
#61813=CARTESIAN_POINT('Ctrl Pts',(0.71155592320357,0.63630980009411,11.952116028638));
#61814=CARTESIAN_POINT('Ctrl Pts',(0.730260496834435,0.794772683999472,
12.0168389022997));
#61815=CARTESIAN_POINT('Ctrl Pts',(0.78559404428569,1.06847604194493,12.0664856050893));
#61816=CARTESIAN_POINT('Ctrl Pts',(0.814343552157919,1.185142708613,12.080016779632));
#61817=CARTESIAN_POINT('Ctrl Pts',(0.847890725520545,1.30000000000259,12.0855889106711));
#61818=CARTESIAN_POINT('Ctrl Pts',(0.610887521890204,-1.29999999999802,
12.1252916341884));
#61819=CARTESIAN_POINT('Ctrl Pts',(0.592006378682212,-1.18514270860991,
12.1172867448402));
#61820=CARTESIAN_POINT('Ctrl Pts',(0.580449617324699,-1.06847604194335,
12.1011139887057));
#61821=CARTESIAN_POINT('Ctrl Pts',(0.57067197397883,-0.794772683999469,
12.0448822804338));
#61822=CARTESIAN_POINT('Ctrl Pts',(0.585512953505324,-0.636309800094091,
11.9759310928786));
#61823=CARTESIAN_POINT('Ctrl Pts',(0.608669395392358,-0.319434907276604,
11.9034560993797));
#61824=CARTESIAN_POINT('Ctrl Pts',(0.62920984988828,-0.158333333333057,
11.8595955660245));
#61825=CARTESIAN_POINT('Ctrl Pts',(0.660165216176782,0.158333333333059,
11.8553160338946));
#61826=CARTESIAN_POINT('Ctrl Pts',(0.671462899317354,0.319434907276612,
11.8947918593629));
#61827=CARTESIAN_POINT('Ctrl Pts',(0.709562168025446,0.6363098000941,11.9587639894938));
#61828=CARTESIAN_POINT('Ctrl Pts',(0.728249453803018,0.794772683999459,
12.023648584504));
#61829=CARTESIAN_POINT('Ctrl Pts',(0.783854550106997,1.06847604194491,12.0723844674039));
#61830=CARTESIAN_POINT('Ctrl Pts',(0.812776317227144,1.18514270861299,12.0852917383376));
#61831=CARTESIAN_POINT('Ctrl Pts',(0.846550465649136,1.30000000000257,12.0900103223398));
#61832=CARTESIAN_POINT('Ctrl Pts',(0.608881776228894,-1.29999999999798,
12.1296579890848));
#61833=CARTESIAN_POINT('Ctrl Pts',(0.589506189731673,-1.18514270860988,
12.12249184714));
#61834=CARTESIAN_POINT('Ctrl Pts',(0.577641880738069,-1.06847604194333,
12.1069367182218));
#61835=CARTESIAN_POINT('Ctrl Pts',(0.567585507175229,-0.794772683999451,
12.0516210205087));
#61836=CARTESIAN_POINT('Ctrl Pts',(0.582946263395987,-0.636309800094076,
11.982545953206));
#61837=CARTESIAN_POINT('Ctrl Pts',(0.606351309519338,-0.319434907276596,
11.9101183918654));
#61838=CARTESIAN_POINT('Ctrl Pts',(0.626975530392277,-0.158333333333053,
11.8659782356395));
#61839=CARTESIAN_POINT('Ctrl Pts',(0.658049576929821,0.158333333333055,
11.8617050272318));
#61840=CARTESIAN_POINT('Ctrl Pts',(0.66932884207984,0.319434907276604,11.9014615037808));
#61841=CARTESIAN_POINT('Ctrl Pts',(0.707529882837701,0.636309800094085,
11.9654098692974));
#61842=CARTESIAN_POINT('Ctrl Pts',(0.726221780561683,0.794772683999441,
12.0304562908449));
#61843=CARTESIAN_POINT('Ctrl Pts',(0.782113312648036,1.06847604194489,12.0782818608322));
#61844=CARTESIAN_POINT('Ctrl Pts',(0.811211199795286,1.18514270861296,12.0905655177454));
#61845=CARTESIAN_POINT('Ctrl Pts',(0.845213600834787,1.30000000000254,12.0944309144363));
#61846=CARTESIAN_POINT('Ctrl Pts',(0.606906390042853,-1.29999999999795,
12.1340256154503));
#61847=CARTESIAN_POINT('Ctrl Pts',(0.58706541570433,-1.18514270860985,12.1277000610048));
#61848=CARTESIAN_POINT('Ctrl Pts',(0.574903502850208,-1.0684760419433,12.1127631645127));
#61849=CARTESIAN_POINT('Ctrl Pts',(0.564547219394806,-0.794772683999432,
12.0583620226792));
#61850=CARTESIAN_POINT('Ctrl Pts',(0.580312530161547,-0.636309800094061,
11.9891555586623));
#61851=CARTESIAN_POINT('Ctrl Pts',(0.603951989620995,-0.319434907276589,
11.9167744619309));
#61852=CARTESIAN_POINT('Ctrl Pts',(0.624751753109886,-0.158333333333049,
11.8723601588131));
#61853=CARTESIAN_POINT('Ctrl Pts',(0.655942851254485,0.158333333333052,
11.8680941065743));
#61854=CARTESIAN_POINT('Ctrl Pts',(0.667141013668526,0.319434907276596,
11.9081285729616));
#61855=CARTESIAN_POINT('Ctrl Pts',(0.705392125245831,0.63630980009407,11.9720517992652));
#61856=CARTESIAN_POINT('Ctrl Pts',(0.724031221176676,0.794772683999421,
12.0372592228598));
#61857=CARTESIAN_POINT('Ctrl Pts',(0.780241753093799,1.06847604194486,12.0841751634707));
#61858=CARTESIAN_POINT('Ctrl Pts',(0.809553287601487,1.18514270861293,12.0958359487701));
#61859=CARTESIAN_POINT('Ctrl Pts',(0.843844900155231,1.30000000000251,12.0988493470852));
#61860=CARTESIAN_POINT('Ctrl Pts',(0.605306250790031,-1.29999999999793,
12.1376678988936));
#61861=CARTESIAN_POINT('Ctrl Pts',(0.58512674498234,-1.18514270860983,12.1320459852867));
#61862=CARTESIAN_POINT('Ctrl Pts',(0.572736658115396,-1.06847604194328,
12.1176255286028));
#61863=CARTESIAN_POINT('Ctrl Pts',(0.562108194845417,-0.794772683999416,
12.0639849942102));
#61864=CARTESIAN_POINT('Ctrl Pts',(0.578043239721755,-0.636309800094048,
11.9946583851704));
#61865=CARTESIAN_POINT('Ctrl Pts',(0.601859231195697,-0.319434907276582,
11.9223142599912));
#61866=CARTESIAN_POINT('Ctrl Pts',(0.622935554994119,-0.158333333333046,
11.8776783729586));
#61867=CARTESIAN_POINT('Ctrl Pts',(0.654225922229719,0.158333333333048,
11.8734192056745));
#61868=CARTESIAN_POINT('Ctrl Pts',(0.665275576234766,0.31943490727659,11.9136820531298));
#61869=CARTESIAN_POINT('Ctrl Pts',(0.703493731277744,0.636309800094057,
11.9775825108839));
#61870=CARTESIAN_POINT('Ctrl Pts',(0.722000803806554,0.794772683999405,
12.0429229622622));
#61871=CARTESIAN_POINT('Ctrl Pts',(0.778511064718178,1.06847604194484,12.0890815767378));
#61872=CARTESIAN_POINT('Ctrl Pts',(0.808047250965803,1.1851427086129,12.1002241597667));
#61873=CARTESIAN_POINT('Ctrl Pts',(0.842658425423753,1.30000000000248,12.102528971963));
#61874=CARTESIAN_POINT('Ctrl Pts',(0.604285083056295,-1.29999999999792,
12.1400363911309));
#61875=CARTESIAN_POINT('Ctrl Pts',(0.583906288881377,-1.18514270860982,
12.1348731089851));
#61876=CARTESIAN_POINT('Ctrl Pts',(0.571376200341018,-1.06847604194327,
12.1207888249669));
#61877=CARTESIAN_POINT('Ctrl Pts',(0.560561269321183,-0.794772683999411,
12.0676420123679));
#61878=CARTESIAN_POINT('Ctrl Pts',(0.576537005022671,-0.636309800094044,
11.9982329662929));
#61879=CARTESIAN_POINT('Ctrl Pts',(0.600457349747139,-0.31943490727658,
11.9259120320742));
#61880=CARTESIAN_POINT('Ctrl Pts',(0.621762735057343,-0.158333333333045,
11.8811346916932));
#61881=CARTESIAN_POINT('Ctrl Pts',(0.653118547739335,0.158333333333047,
11.8768803927112));
#61882=CARTESIAN_POINT('Ctrl Pts',(0.664043720438682,0.319434907276588,
11.9172906141691));
#61883=CARTESIAN_POINT('Ctrl Pts',(0.70221111520551,0.636309800094053,11.9811756537776));
#61884=CARTESIAN_POINT('Ctrl Pts',(0.720594222382496,0.794772683999401,
12.0466020212848));
#61885=CARTESIAN_POINT('Ctrl Pts',(0.777311411198164,1.06847604194483,12.092268747927));
#61886=CARTESIAN_POINT('Ctrl Pts',(0.807011834517717,1.1851427086129,12.1030749121673));
#61887=CARTESIAN_POINT('Ctrl Pts',(0.841861911697297,1.30000000000247,12.1049198068032));
#61888=CARTESIAN_POINT('Ctrl Pts',(0.603815899220733,-1.29999999999792,
12.1411296230263));
#61889=CARTESIAN_POINT('Ctrl Pts',(0.583347471311102,-1.18514270860982,
12.1361781416372));
#61890=CARTESIAN_POINT('Ctrl Pts',(0.570753626107481,-1.06847604194327,
12.1222490532589));
#61891=CARTESIAN_POINT('Ctrl Pts',(0.559851185652774,-0.794772683999409,
12.0693300044916));
#61892=CARTESIAN_POINT('Ctrl Pts',(0.575837369233593,-0.636309800094043,
11.9998824067175));
#61893=CARTESIAN_POINT('Ctrl Pts',(0.599803987165821,-0.31943490727658,
11.9275720589377));
#61894=CARTESIAN_POINT('Ctrl Pts',(0.621219922477897,-0.158333333333045,
11.8827297039398));
#61895=CARTESIAN_POINT('Ctrl Pts',(0.652606018081053,0.158333333333047,
11.8784777079958));
#61896=CARTESIAN_POINT('Ctrl Pts',(0.663471519768857,0.319434907276587,
11.9189558690088));
#61897=CARTESIAN_POINT('Ctrl Pts',(0.701612372747973,0.636309800094052,
11.9828337465353));
#61898=CARTESIAN_POINT('Ctrl Pts',(0.719933452155873,0.794772683999399,
12.0482996836085));
#61899=CARTESIAN_POINT('Ctrl Pts',(0.77674737768157,1.06847604194483,12.093739461978));
#61900=CARTESIAN_POINT('Ctrl Pts',(0.806525649454242,1.1851427086129,12.1043904270862));
#61901=CARTESIAN_POINT('Ctrl Pts',(0.841489549802737,1.30000000000247,12.1060231609561));
#61902=CARTESIAN_POINT('Ctrl Pts',(0.603581710836913,-1.29999999999792,
12.1416762537866));
#61903=CARTESIAN_POINT('Ctrl Pts',(0.583068922644597,-1.18514270860982,
12.1368306966218));
#61904=CARTESIAN_POINT('Ctrl Pts',(0.570443366248212,-1.06847604194327,
12.1229792133864));
#61905=CARTESIAN_POINT('Ctrl Pts',(0.559496888522581,-0.79477268399941,
12.0701740252806));
#61906=CARTESIAN_POINT('Ctrl Pts',(0.575486671213716,-0.636309800094043,
12.0007070539529));
#61907=CARTESIAN_POINT('Ctrl Pts',(0.599476059838051,-0.31943490727658,
11.9284019768101));
#61908=CARTESIAN_POINT('Ctrl Pts',(0.620948214103655,-0.158333333333045,
11.8835271674347));
#61909=CARTESIAN_POINT('Ctrl Pts',(0.652349472132746,0.158333333333047,
11.8792763341935));
#61910=CARTESIAN_POINT('Ctrl Pts',(0.663184708296504,0.319434907276587,
11.9197884496198));
#61911=CARTESIAN_POINT('Ctrl Pts',(0.701311694856169,0.636309800094052,
11.9836627377277));
#61912=CARTESIAN_POINT('Ctrl Pts',(0.719600847373781,0.794772683999399,
12.049148444006));
#61913=CARTESIAN_POINT('Ctrl Pts',(0.776463368826196,1.06847604194483,12.0944747635993));
#61914=CARTESIAN_POINT('Ctrl Pts',(0.806280949610835,1.1851427086129,12.1050481430266));
#61915=CARTESIAN_POINT('Ctrl Pts',(0.841302432607243,1.30000000000247,12.1065748176348));
#61916=CARTESIAN_POINT('Ctrl Pts',(0.603386782454753,-1.29999999999792,
12.1421317832905));
#61917=CARTESIAN_POINT('Ctrl Pts',(0.582837263443985,-1.18514270860982,
12.1373745060256));
#61918=CARTESIAN_POINT('Ctrl Pts',(0.570185353761598,-1.06847604194327,
12.1235876951198));
#61919=CARTESIAN_POINT('Ctrl Pts',(0.559201968849319,-0.794772683999408,
12.0708773748228));
#61920=CARTESIAN_POINT('Ctrl Pts',(0.575193834867384,-0.636309800094042,
12.0013942059284));
#61921=CARTESIAN_POINT('Ctrl Pts',(0.599201878836009,-0.319434907276579,
11.9290935048279));
#61922=CARTESIAN_POINT('Ctrl Pts',(0.620721225877243,-0.158333333333045,
11.8841916730529));
#61923=CARTESIAN_POINT('Ctrl Pts',(0.652135121329545,0.158333333333047,
11.8799418160112));
#61924=CARTESIAN_POINT('Ctrl Pts',(0.662945093381664,0.319434907276587,
11.9204822267212));
#61925=CARTESIAN_POINT('Ctrl Pts',(0.701060240529716,0.636309800094051,
11.9843535229102));
#61926=CARTESIAN_POINT('Ctrl Pts',(0.719322187748478,0.794772683999398,
12.0498556904397));
#61927=CARTESIAN_POINT('Ctrl Pts',(0.776225303499505,1.06847604194483,12.0950874746472));
#61928=CARTESIAN_POINT('Ctrl Pts',(0.806075850100194,1.18514270861289,12.105596210833));
#61929=CARTESIAN_POINT('Ctrl Pts',(0.841145692960999,1.30000000000247,12.1070345198236));
#61930=CARTESIAN_POINT('Ctrl Pts',(0.603250458156735,-1.29999999999792,
12.1424506569694));
#61931=CARTESIAN_POINT('Ctrl Pts',(0.582675401104163,-1.18514270860982,
12.1377551837426));
#61932=CARTESIAN_POINT('Ctrl Pts',(0.570005106414889,-1.06847604194327,
12.1240136455603));
#61933=CARTESIAN_POINT('Ctrl Pts',(0.558995773400406,-0.794772683999409,
12.0713697236677));
#61934=CARTESIAN_POINT('Ctrl Pts',(0.574988458255701,-0.636309800094042,
12.0018751789434));
#61935=CARTESIAN_POINT('Ctrl Pts',(0.599009439913919,-0.319434907276579,
11.929577533758));
#61936=CARTESIAN_POINT('Ctrl Pts',(0.620562232944649,-0.158333333333045,
11.8846568094334));
#61937=CARTESIAN_POINT('Ctrl Pts',(0.651984994328979,0.158333333333047,
11.8804076406294));
#61938=CARTESIAN_POINT('Ctrl Pts',(0.662777078632811,0.319434907276587,
11.9209678497561));
#61939=CARTESIAN_POINT('Ctrl Pts',(0.700883715604501,0.636309800094051,
11.9848370486251));
#61940=CARTESIAN_POINT('Ctrl Pts',(0.719126316881295,0.794772683999399,
12.0503507353582));
#61941=CARTESIAN_POINT('Ctrl Pts',(0.776057933517928,1.06847604194483,12.095516351444));
#61942=CARTESIAN_POINT('Ctrl Pts',(0.805931692314347,1.18514270861289,12.1059798427101));
#61943=CARTESIAN_POINT('Ctrl Pts',(0.841035622589297,1.30000000000247,12.1073563035896));
#61944=CARTESIAN_POINT('Ctrl Pts',(0.603172548320683,-1.29999999999791,
12.1426328672716));
#61945=CARTESIAN_POINT('Ctrl Pts',(0.582582836069079,-1.18514270860982,
12.1379727059308));
#61946=CARTESIAN_POINT('Ctrl Pts',(0.569902001416967,-1.06847604194327,
12.1242570353342));
#61947=CARTESIAN_POINT('Ctrl Pts',(0.558877825998678,-0.794772683999409,
12.0716510545165));
#61948=CARTESIAN_POINT('Ctrl Pts',(0.574871154895082,-0.636309800094042,
12.0021500208177));
#61949=CARTESIAN_POINT('Ctrl Pts',(0.598899431395806,-0.319434907276579,
11.9298541192445));
#61950=CARTESIAN_POINT('Ctrl Pts',(0.620471004332286,-0.158333333333045,
11.8849225841299));
#61951=CARTESIAN_POINT('Ctrl Pts',(0.651898805737524,0.158333333333047,
11.8806738081012));
#61952=CARTESIAN_POINT('Ctrl Pts',(0.662680942569796,0.319434907276587,
11.9212453435713));
#61953=CARTESIAN_POINT('Ctrl Pts',(0.700782825985886,0.636309800094051,
11.985113348793));
#61954=CARTESIAN_POINT('Ctrl Pts',(0.719014349215731,0.794772683999398,
12.0506336128885));
#61955=CARTESIAN_POINT('Ctrl Pts',(0.775962198276967,1.06847604194483,12.0957614210369));
#61956=CARTESIAN_POINT('Ctrl Pts',(0.805849179745395,1.18514270861289,12.1061990601445));
#61957=CARTESIAN_POINT('Ctrl Pts',(0.840972528949222,1.30000000000247,12.107540182362));
#61958=CARTESIAN_POINT('Ctrl Pts',(0.600643530861967,-1.29999999999796,
12.1485549289069));
#61959=CARTESIAN_POINT('Ctrl Pts',(0.579584823952958,-1.18514270860986,
12.1450428386672));
#61960=CARTESIAN_POINT('Ctrl Pts',(0.56656473266857,-1.06847604194331,12.1321680482343));
#61961=CARTESIAN_POINT('Ctrl Pts',(0.55505652735372,-0.794772683999437,
12.0807949962933));
#61962=CARTESIAN_POINT('Ctrl Pts',(0.571046633027255,-0.636309800094064,
12.0110815971801));
#61963=CARTESIAN_POINT('Ctrl Pts',(0.595315222693786,-0.31943490727659,
11.938842369259));
#61964=CARTESIAN_POINT('Ctrl Pts',(0.61752567296301,-0.15833333333305,11.8935608790396));
#61965=CARTESIAN_POINT('Ctrl Pts',(0.649119349189772,0.158333333333052,
11.8893250071093));
#61966=CARTESIAN_POINT('Ctrl Pts',(0.659557679761414,0.319434907276598,
11.9302636958771));
#61967=CARTESIAN_POINT('Ctrl Pts',(0.697493961619743,0.636309800094073,
11.9940925654044));
#61968=CARTESIAN_POINT('Ctrl Pts',(0.715360551785109,0.794772683999426,
12.0598268264269));
#61969=CARTESIAN_POINT('Ctrl Pts',(0.772840883424242,1.06847604194487,12.1037258900667));
#61970=CARTESIAN_POINT('Ctrl Pts',(0.803162869925518,1.18514270861294,12.1133233314549));
#61971=CARTESIAN_POINT('Ctrl Pts',(0.838925737217494,1.30000000000251,12.1135159362019));
#61972=CARTESIAN_POINT('Ctrl Pts',(0.595485031953642,-1.29999999999867,
12.1602434858869));
#61973=CARTESIAN_POINT('Ctrl Pts',(0.573241290581446,-1.18514270861051,
12.1589798784746));
#61974=CARTESIAN_POINT('Ctrl Pts',(0.559414705256469,-1.06847604194389,
12.1477561964616));
#61975=CARTESIAN_POINT('Ctrl Pts',(0.546917841472229,-0.794772683999873,
12.0988174808883));
#61976=CARTESIAN_POINT('Ctrl Pts',(0.56360172731629,-0.636309800094413,
12.0287328666738));
#61977=CARTESIAN_POINT('Ctrl Pts',(0.588134026213673,-0.319434907276765,
11.9566036793466));
#61978=CARTESIAN_POINT('Ctrl Pts',(0.610582825305128,-0.158333333333137,
11.9105839829202));
#61979=CARTESIAN_POINT('Ctrl Pts',(0.642469543617756,0.158333333333139,
11.9063714642218));
#61980=CARTESIAN_POINT('Ctrl Pts',(0.653078416052506,0.319434907276774,
11.9480710018856));
#61981=CARTESIAN_POINT('Ctrl Pts',(0.691111919053413,0.636309800094423,
12.0118388469959));
#61982=CARTESIAN_POINT('Ctrl Pts',(0.708360915710318,0.794772683999862,
12.0779886723153));
#61983=CARTESIAN_POINT('Ctrl Pts',(0.766684612953707,1.06847604194545,12.119467236768));
#61984=CARTESIAN_POINT('Ctrl Pts',(0.797667728588445,1.18514270861359,12.1274091500634));
#61985=CARTESIAN_POINT('Ctrl Pts',(0.834387792427035,1.30000000000323,12.1253384430347));
#61986=CARTESIAN_POINT('Ctrl Pts',(0.587185078806851,-1.29999999999891,
12.1776573032884));
#61987=CARTESIAN_POINT('Ctrl Pts',(0.562993490899537,-1.18514270861072,
12.1797310055913));
#61988=CARTESIAN_POINT('Ctrl Pts',(0.547883421785488,-1.06847604194409,
12.1709617431183));
#61989=CARTESIAN_POINT('Ctrl Pts',(0.533956264537119,-0.794772684000015,
12.1256535747606));
#61990=CARTESIAN_POINT('Ctrl Pts',(0.551875880532105,-0.636309800094528,
12.0550347186061));
#61991=CARTESIAN_POINT('Ctrl Pts',(0.577514735286172,-0.319434907276823,
11.9831127855141));
#61992=CARTESIAN_POINT('Ctrl Pts',(0.601418710125038,-0.158333333333166,
11.9360515158364));
#61993=CARTESIAN_POINT('Ctrl Pts',(0.633873956312172,0.158333333333168,
11.9318854240732));
#61994=CARTESIAN_POINT('Ctrl Pts',(0.643459387532714,0.31943490727683,11.9746628061304));
#61995=CARTESIAN_POINT('Ctrl Pts',(0.681823023208725,0.636309800094536,
12.038338651949));
#61996=CARTESIAN_POINT('Ctrl Pts',(0.699858850607088,0.794772684000005,
12.105164341511));
#61997=CARTESIAN_POINT('Ctrl Pts',(0.759403760308767,1.06847604194565,12.1430273132517));
#61998=CARTESIAN_POINT('Ctrl Pts',(0.790999049044779,1.1851427086138,12.1484856809274));
#61999=CARTESIAN_POINT('Ctrl Pts',(0.8284148414631,1.30000000000346,12.1430129387736));
#62000=CARTESIAN_POINT('Ctrl Pts',(0.579506951612649,-1.2999999999997,12.1950893665228));
#62001=CARTESIAN_POINT('Ctrl Pts',(0.553345502078091,-1.18514270861144,
12.2004957811793));
#62002=CARTESIAN_POINT('Ctrl Pts',(0.536920448834634,-1.06847604194474,
12.1941774992085));
#62003=CARTESIAN_POINT('Ctrl Pts',(0.521468313213451,-0.794772684000499,
12.1524946091617));
#62004=CARTESIAN_POINT('Ctrl Pts',(0.540639835639615,-0.636309800094918,
12.0813512164322));
#62005=CARTESIAN_POINT('Ctrl Pts',(0.567046541242541,-0.319434907277021,
12.009617450558));
#62006=CARTESIAN_POINT('Ctrl Pts',(0.591913503988528,-0.158333333333263,
11.9614795037667));
#62007=CARTESIAN_POINT('Ctrl Pts',(0.624684878793728,0.158333333333265,
11.9573439230541));
#62008=CARTESIAN_POINT('Ctrl Pts',(0.633791842433493,0.319434907277025,
12.0012228555678));
#62009=CARTESIAN_POINT('Ctrl Pts',(0.671688556708476,0.636309800094926,
12.0647841665863));
#62010=CARTESIAN_POINT('Ctrl Pts',(0.688016865714616,0.794772684000495,
12.1322217064504));
#62011=CARTESIAN_POINT('Ctrl Pts',(0.749472591398532,1.0684760419463,12.1664696953007));
#62012=CARTESIAN_POINT('Ctrl Pts',(0.782693584574102,1.18514270861453,12.1694595734739));
#62013=CARTESIAN_POINT('Ctrl Pts',(0.822533664435534,1.30000000000426,12.1606146444599));
#62014=CARTESIAN_POINT('Ctrl Pts',(0.573578201915757,-1.30000000000028,
12.2066602306644));
#62015=CARTESIAN_POINT('Ctrl Pts',(0.546373190975778,-1.18514270861197,
12.2142950671844));
#62016=CARTESIAN_POINT('Ctrl Pts',(0.529208707811323,-1.06847604194521,
12.2096111059055));
#62017=CARTESIAN_POINT('Ctrl Pts',(0.512750945720502,-0.794772684000851,
12.1703313310453));
#62018=CARTESIAN_POINT('Ctrl Pts',(0.532138549719906,-0.636309800095197,
12.0987891640359));
#62019=CARTESIAN_POINT('Ctrl Pts',(0.558956795859338,-0.319434907277159,
12.0271831232441));
#62020=CARTESIAN_POINT('Ctrl Pts',(0.584631254886148,-0.158333333333332,
11.9783681315311));
#62021=CARTESIAN_POINT('Ctrl Pts',(0.618034103223892,0.158333333333334,
11.9742859986132));
#62022=CARTESIAN_POINT('Ctrl Pts',(0.627223601649686,0.319434907277167,
12.0189115172152));
#62023=CARTESIAN_POINT('Ctrl Pts',(0.665468378425724,0.636309800095206,
12.0824211914211));
#62024=CARTESIAN_POINT('Ctrl Pts',(0.681689914147691,0.79477268400084,12.1502814912943));
#62025=CARTESIAN_POINT('Ctrl Pts',(0.743851598608587,1.06847604194677,12.1821291336617));
#62026=CARTESIAN_POINT('Ctrl Pts',(0.777519991844039,1.18514270861505,12.1834743205671));
#62027=CARTESIAN_POINT('Ctrl Pts',(0.817949288429029,1.30000000000483,12.1723790300684));
#62028=CARTESIAN_POINT('Ctrl Pts',(0.57067025537727,-1.30000000000028,12.2124460829627));
#62029=CARTESIAN_POINT('Ctrl Pts',(0.542940786613358,-1.18514270861197,
12.2211942845405));
#62030=CARTESIAN_POINT('Ctrl Pts',(0.525404772703435,-1.06847604194521,
12.2173269808077));
#62031=CARTESIAN_POINT('Ctrl Pts',(0.508441992410329,-0.794772684000851,
12.1792483945427));
#62032=CARTESIAN_POINT('Ctrl Pts',(0.52791511722475,-0.636309800095197,
12.107507287942));
#62033=CARTESIAN_POINT('Ctrl Pts',(0.554987172141785,-0.319434907277159,
12.0359668790037));
#62034=CARTESIAN_POINT('Ctrl Pts',(0.581221077759065,-0.158333333333332,
11.9868187308123));
#62035=CARTESIAN_POINT('Ctrl Pts',(0.614857791973618,0.158333333333334,
11.9827589718209));
#62036=CARTESIAN_POINT('Ctrl Pts',(0.623796233999667,0.319434907277167,
12.0277447643876));
#62037=CARTESIAN_POINT('Ctrl Pts',(0.662111769288738,0.636309800095206,
12.0912247185273));
#62038=CARTESIAN_POINT('Ctrl Pts',(0.678359592024736,0.79477268400084,12.1593033180431));
#62039=CARTESIAN_POINT('Ctrl Pts',(0.74098795051949,1.06847604194677,12.1899531249437));
#62040=CARTESIAN_POINT('Ctrl Pts',(0.774949037062868,1.18514270861505,12.1904765350795));
#62041=CARTESIAN_POINT('Ctrl Pts',(0.81576171436643,1.30000000000483,12.178256189631));
#62042=CARTESIAN_POINT('',(0.819125420164991,1.2,12.0817551706368));
#62043=CARTESIAN_POINT('Ctrl Pts',(0.819125420164991,1.2,12.0817551706368));
#62044=CARTESIAN_POINT('Ctrl Pts',(0.830644422591068,1.2183776817245,12.061187766347));
#62045=CARTESIAN_POINT('Ctrl Pts',(0.843273624387522,1.23628901120912,12.0408328984551));
#62046=CARTESIAN_POINT('Ctrl Pts',(0.866362035602099,1.27375689806004,11.9986871795306));
#62047=CARTESIAN_POINT('Ctrl Pts',(0.875510184622732,1.2880705970965,11.9824605692077));
#62048=CARTESIAN_POINT('Ctrl Pts',(0.882649956912143,1.30000000000362,11.969007134984));
#62049=CARTESIAN_POINT('',(0.664237960863694,0.65383484145594,12.1052306705389));
#62050=CARTESIAN_POINT('Ctrl Pts',(0.664237960894242,0.653834841448649,
12.1052306705503));
#62051=CARTESIAN_POINT('Ctrl Pts',(0.678771402050763,0.711663049082454,
12.1032626360241));
#62052=CARTESIAN_POINT('Ctrl Pts',(0.694178908180175,0.767421706161028,
12.1011084974005));
#62053=CARTESIAN_POINT('Ctrl Pts',(0.744496374024038,0.949876651320734,
12.0938180273354));
#62054=CARTESIAN_POINT('Ctrl Pts',(0.780817741461556,1.07527000774591,12.0881829394037));
#62055=CARTESIAN_POINT('Ctrl Pts',(0.81912542016499,1.2,12.0817551706368));
#62056=CARTESIAN_POINT('',(0.525742999963518,-0.653834841531101,12.1220010461183));
#62057=CARTESIAN_POINT('Ctrl Pts',(0.525742999963527,-0.653834841531115,
12.1220010461183));
#62058=CARTESIAN_POINT('Ctrl Pts',(0.539190022298025,-0.575736048549707,
12.0825245635937));
#62059=CARTESIAN_POINT('Ctrl Pts',(0.55145350222942,-0.493707176825078,
12.0495991382559));
#62060=CARTESIAN_POINT('Ctrl Pts',(0.571106258772745,-0.338050175537241,
12.0029165481558));
#62061=CARTESIAN_POINT('Ctrl Pts',(0.579194577471218,-0.265591481216425,
11.9869422768981));
#62062=CARTESIAN_POINT('Ctrl Pts',(0.593836166316479,-0.129668288621025,
11.9674504522924));
#62063=CARTESIAN_POINT('Ctrl Pts',(0.600389101024186,-0.0666199245840123,
11.9624587608477));
#62064=CARTESIAN_POINT('Ctrl Pts',(0.613515992006829,0.0594914647288782,
11.9604922996646));
#62065=CARTESIAN_POINT('Ctrl Pts',(0.62016841052224,0.122683940931368,11.9634887161708));
#62066=CARTESIAN_POINT('Ctrl Pts',(0.633865216238478,0.26005354284401,11.9789549475266));
#62067=CARTESIAN_POINT('Ctrl Pts',(0.640796190912842,0.333934236185787,
11.9930603476798));
#62068=CARTESIAN_POINT('Ctrl Pts',(0.653731520036761,0.491651609165574,
12.0361172105966));
#62069=CARTESIAN_POINT('Ctrl Pts',(0.659778232475277,0.575076596064635,
12.0673420839221));
#62070=CARTESIAN_POINT('Ctrl Pts',(0.664237960911195,0.653834841464539,
12.1052306705154));
#62071=CARTESIAN_POINT('',(0.597524573714823,-1.2,12.1138034539252));
#62072=CARTESIAN_POINT('Ctrl Pts',(0.597524573714823,-1.2,12.1138034539252));
#62073=CARTESIAN_POINT('Ctrl Pts',(0.58514630377234,-1.1341651966939,12.1153086668504));
#62074=CARTESIAN_POINT('Ctrl Pts',(0.569018766055164,-1.03862960183204,
12.1172216138762));
#62075=CARTESIAN_POINT('Ctrl Pts',(0.533638828669213,-0.766812999705298,
12.1211801707249));
#62076=CARTESIAN_POINT('Ctrl Pts',(0.530556512233154,-0.718567421671387,
12.121486891335));
#62077=CARTESIAN_POINT('Ctrl Pts',(0.525742999963529,-0.6538348415311,12.1220010461183));
#62078=CARTESIAN_POINT('Ctrl Pts',(0.65906282859866,-1.29999999999906,12.005011570014));
#62079=CARTESIAN_POINT('Ctrl Pts',(0.648887062337683,-1.28291444576899,
12.0236528169717));
#62080=CARTESIAN_POINT('Ctrl Pts',(0.638372322676667,-1.26592287187928,
12.0421942540332));
#62081=CARTESIAN_POINT('Ctrl Pts',(0.623146285770558,-1.24020469105829,
12.0700941915526));
#62082=CARTESIAN_POINT('Ctrl Pts',(0.610885738061428,-1.21949365620403,
12.0925414675189));
#62083=CARTESIAN_POINT('Ctrl Pts',(0.597524573714824,-1.2,12.1138034539252));
#62084=CARTESIAN_POINT('Origin',(0.,1.25,7.2));
#62085=CARTESIAN_POINT('',(0.437314692285883,1.2,12.1306445684019));
#62086=CARTESIAN_POINT('Ctrl Pts',(0.354270609538459,1.3,12.0370437599031));
#62087=CARTESIAN_POINT('Ctrl Pts',(0.367581476408574,1.28316120465979,12.0529527556245));
#62088=CARTESIAN_POINT('Ctrl Pts',(0.381406074582236,1.26649040416743,12.0686092762383));
#62089=CARTESIAN_POINT('Ctrl Pts',(0.413005097135395,1.22892242797915,12.1037420910764));
#62090=CARTESIAN_POINT('Ctrl Pts',(0.422615951166165,1.21634758534866,12.1155364885164));
#62091=CARTESIAN_POINT('Ctrl Pts',(0.437314692285883,1.2,12.1306445684019));
#62092=CARTESIAN_POINT('Origin',(0.,1.2,7.2));
#62093=CARTESIAN_POINT('Origin',(0.,0.92691742076555,7.2));
#62094=CARTESIAN_POINT('Origin',(0.,0.653834841531101,7.2));
#62095=CARTESIAN_POINT('Origin',(0.,0.92691742076555,7.2));
#62096=CARTESIAN_POINT('',(0.509087305687289,0.653834841531101,12.123751630128));
#62097=CARTESIAN_POINT('Ctrl Pts',(0.437314692285884,1.2,12.1306445684019));
#62098=CARTESIAN_POINT('Ctrl Pts',(0.447918386563704,1.14399458640636,12.1297040927225));
#62099=CARTESIAN_POINT('Ctrl Pts',(0.463097499149716,1.06151801688422,12.1283363573917));
#62100=CARTESIAN_POINT('Ctrl Pts',(0.497285011036078,0.797206845778639,
12.124974622511));
#62101=CARTESIAN_POINT('Ctrl Pts',(0.502682930763357,0.739930875460911,
12.1244138052781));
#62102=CARTESIAN_POINT('Ctrl Pts',(0.509087305687304,0.653834841531103,
12.123751630128));
#62103=CARTESIAN_POINT('Origin',(0.,0.653834841531101,7.2));
#62104=CARTESIAN_POINT('Origin',(0.,-1.25,7.2));
#62105=CARTESIAN_POINT('Origin',(0.,-1.2,7.2));
#62106=CARTESIAN_POINT('Origin',(0.,0.,7.2));
#62107=CARTESIAN_POINT('Origin',(0.,-0.653834841531101,7.2));
#62108=CARTESIAN_POINT('Origin',(0.,-0.926917420765551,7.2));
#62109=CARTESIAN_POINT('Ctrl Pts',(0.237102298033322,-1.30000000000024,
12.2390757450685));
#62110=CARTESIAN_POINT('Ctrl Pts',(0.279563873101034,-1.18514270861194,
12.2425436139055));
#62111=CARTESIAN_POINT('Ctrl Pts',(0.31267400533481,-1.0684760419452,12.2349707346125));
#62112=CARTESIAN_POINT('Ctrl Pts',(0.367561330757959,-0.794772684000851,
12.1919695316219));
#62113=CARTESIAN_POINT('Ctrl Pts',(0.369299762850422,-0.636309800095197,
12.1220005005432));
#62114=CARTESIAN_POINT('Ctrl Pts',(0.393579787165998,-0.319434907277159,
12.0519414879789));
#62115=CARTESIAN_POINT('Ctrl Pts',(0.392969830592779,-0.158333333333332,
12.0060803363189));
#62116=CARTESIAN_POINT('Ctrl Pts',(0.426715573254505,0.158333333333334,
12.0030579137102));
#62117=CARTESIAN_POINT('Ctrl Pts',(0.462594679682929,0.319434907277167,
12.0456777212709));
#62118=CARTESIAN_POINT('Ctrl Pts',(0.503949232631026,0.636309800095206,
12.1100262039159));
#62119=CARTESIAN_POINT('Ctrl Pts',(0.537912637721293,0.794772684000841,
12.1761509049009));
#62120=CARTESIAN_POINT('Ctrl Pts',(0.52923751813028,1.0684760419452,12.2169241430278));
#62121=CARTESIAN_POINT('Ctrl Pts',(0.512888765856004,1.18514270861195,12.224352879199));
#62122=CARTESIAN_POINT('Ctrl Pts',(0.483946399133541,1.30000000000025,12.2215611275538));
#62123=CARTESIAN_POINT('Ctrl Pts',(0.230378897029079,-1.30000000000024,
12.2284879305123));
#62124=CARTESIAN_POINT('Ctrl Pts',(0.271622642083581,-1.18514270861194,
12.2299142784407));
#62125=CARTESIAN_POINT('Ctrl Pts',(0.303818465808643,-1.0684760419452,12.2208554699308));
#62126=CARTESIAN_POINT('Ctrl Pts',(0.357294751064532,-0.794772684000851,
12.1757050011437));
#62127=CARTESIAN_POINT('Ctrl Pts',(0.359072532092265,-0.636309800095197,
12.1061739593177));
#62128=CARTESIAN_POINT('Ctrl Pts',(0.383201773569423,-0.319434907277159,
12.0360862285591));
#62129=CARTESIAN_POINT('Ctrl Pts',(0.383232767764448,-0.158333333333332,
11.9908254840166));
#62130=CARTESIAN_POINT('Ctrl Pts',(0.416530303335429,0.158333333333334,
11.9879440783124));
#62131=CARTESIAN_POINT('Ctrl Pts',(0.451176432830853,0.319434907277167,
12.0301447644328));
#62132=CARTESIAN_POINT('Ctrl Pts',(0.492061752143941,0.636309800095206,
12.0947271819628));
#62133=CARTESIAN_POINT('Ctrl Pts',(0.525775129538419,0.794772684000841,
12.1604982598871));
#62134=CARTESIAN_POINT('Ctrl Pts',(0.518587456936806,1.0684760419452,12.2034113791225));
#62135=CARTESIAN_POINT('Ctrl Pts',(0.503305113780037,1.18514270861195,12.2122832473731));
#62136=CARTESIAN_POINT('Ctrl Pts',(0.475851704606219,1.30000000000025,12.211451484645));
#62137=CARTESIAN_POINT('Ctrl Pts',(0.217480409460025,-1.30000000000027,
12.2072321589895));
#62138=CARTESIAN_POINT('Ctrl Pts',(0.255006220628721,-1.18514270861197,
12.2048581625234));
#62139=CARTESIAN_POINT('Ctrl Pts',(0.284649067387247,-1.06847604194522,
12.1929812542131));
#62140=CARTESIAN_POINT('Ctrl Pts',(0.334918748661489,-0.794772684000867,
12.1435895926376));
#62141=CARTESIAN_POINT('Ctrl Pts',(0.338932835191999,-0.63630980009521,
12.0744056487988));
#62142=CARTESIAN_POINT('Ctrl Pts',(0.363309405263975,-0.319434907277166,
12.0041227783375));
#62143=CARTESIAN_POINT('Ctrl Pts',(0.363778637604756,-0.158333333333336,
11.9602912653471));
#62144=CARTESIAN_POINT('Ctrl Pts',(0.396376781294448,0.158333333333338,
11.9576271363067));
#62145=CARTESIAN_POINT('Ctrl Pts',(0.429467212561655,0.319434907277176,
11.9987176860391));
#62146=CARTESIAN_POINT('Ctrl Pts',(0.469532167199508,0.636309800095223,
12.0637304232381));
#62147=CARTESIAN_POINT('Ctrl Pts',(0.501908584033921,0.794772684000859,
12.1290339635959));
#62148=CARTESIAN_POINT('Ctrl Pts',(0.497690845494853,1.06847604194522,12.1762437320941));
#62149=CARTESIAN_POINT('Ctrl Pts',(0.484688916619089,1.18514270861197,12.1879700590222));
#62150=CARTESIAN_POINT('Ctrl Pts',(0.460510761598508,1.30000000000028,12.1909873533899));
#62151=CARTESIAN_POINT('Ctrl Pts',(0.204221446243486,-1.3000000000003,12.1855696400446));
#62152=CARTESIAN_POINT('Ctrl Pts',(0.239925501229051,-1.185142708612,12.1788788856711));
#62153=CARTESIAN_POINT('Ctrl Pts',(0.268098011735459,-1.06847604194524,
12.163880376218));
#62154=CARTESIAN_POINT('Ctrl Pts',(0.31578277246951,-0.794772684000884,
12.1100382427449));
#62155=CARTESIAN_POINT('Ctrl Pts',(0.318975050902126,-0.636309800095224,
12.0419589490921));
#62156=CARTESIAN_POINT('Ctrl Pts',(0.342761455244345,-0.319434907277172,
11.9716803997706));
#62157=CARTESIAN_POINT('Ctrl Pts',(0.344489810553044,-0.158333333333339,
11.9290947507789));
#62158=CARTESIAN_POINT('Ctrl Pts',(0.376548640812749,0.158333333333341,
11.9265957252551));
#62159=CARTESIAN_POINT('Ctrl Pts',(0.408153655753568,0.319434907277179,
11.9665148817081));
#62160=CARTESIAN_POINT('Ctrl Pts',(0.447072634148667,0.636309800095232,
12.0320442142247));
#62161=CARTESIAN_POINT('Ctrl Pts',(0.477304696940038,0.794772684000872,
12.0970886036103));
#62162=CARTESIAN_POINT('Ctrl Pts',(0.476004865794366,1.06847604194524,12.1487086624893));
#62163=CARTESIAN_POINT('Ctrl Pts',(0.465438337761383,1.185142708612,12.1633146761431));
#62164=CARTESIAN_POINT('Ctrl Pts',(0.444867930434888,1.30000000000031,12.1701822926736));
#62165=CARTESIAN_POINT('Ctrl Pts',(0.197352232389149,-1.3000000000003,12.174247236372));
#62166=CARTESIAN_POINT('Ctrl Pts',(0.231242228234118,-1.185142708612,12.1654874086266));
#62167=CARTESIAN_POINT('Ctrl Pts',(0.258160357660685,-1.06847604194525,
12.1489595156624));
#62168=CARTESIAN_POINT('Ctrl Pts',(0.30424021544578,-0.794772684000887,
12.09283099187));
#62169=CARTESIAN_POINT('Ctrl Pts',(0.308345084562613,-0.636309800095226,
12.0250112049144));
#62170=CARTESIAN_POINT('Ctrl Pts',(0.332424732837815,-0.319434907277173,
11.9545881433762));
#62171=CARTESIAN_POINT('Ctrl Pts',(0.334882470599985,-0.158333333333339,
11.9126391673332));
#62172=CARTESIAN_POINT('Ctrl Pts',(0.366609291628401,0.158333333333342,
11.9102385945571));
#62173=CARTESIAN_POINT('Ctrl Pts',(0.39687726031105,0.319434907277181,11.9496881813109));
#62174=CARTESIAN_POINT('Ctrl Pts',(0.435388204392732,0.636309800095236,
12.0154227310738));
#62175=CARTESIAN_POINT('Ctrl Pts',(0.465524583282553,0.794772684000877,
12.0800332353211));
#62176=CARTESIAN_POINT('Ctrl Pts',(0.465750995849449,1.06847604194524,12.1339656762935));
#62177=CARTESIAN_POINT('Ctrl Pts',(0.45624019572631,1.185142708612,12.1501459091373));
#62178=CARTESIAN_POINT('Ctrl Pts',(0.437120589869235,1.30000000000031,12.1591610195218));
#62179=CARTESIAN_POINT('Ctrl Pts',(0.196563250283277,-1.3000000000003,12.1729109480967));
#62180=CARTESIAN_POINT('Ctrl Pts',(0.230245887700426,-1.185142708612,12.1639059355002));
#62181=CARTESIAN_POINT('Ctrl Pts',(0.25701921103806,-1.06847604194525,12.1471972339629));
#62182=CARTESIAN_POINT('Ctrl Pts',(0.302909046205741,-0.794772684000887,
12.0907997282765));
#62183=CARTESIAN_POINT('Ctrl Pts',(0.307103184371951,-0.636309800095226,
12.023015057334));
#62184=CARTESIAN_POINT('Ctrl Pts',(0.33121687505589,-0.319434907277173,
11.9525749339417));
#62185=CARTESIAN_POINT('Ctrl Pts',(0.333776829383913,-0.158333333333339,
11.9106965890592));
#62186=CARTESIAN_POINT('Ctrl Pts',(0.365464948756233,0.158333333333342,
11.9083073734864));
#62187=CARTESIAN_POINT('Ctrl Pts',(0.395565754534697,0.319434907277181,
11.9477040904735));
#62188=CARTESIAN_POINT('Ctrl Pts',(0.434017282248823,0.636309800095235,
12.0134657910199));
#62189=CARTESIAN_POINT('Ctrl Pts',(0.464130379642697,0.794772684000877,
12.0780286470565));
#62190=CARTESIAN_POINT('Ctrl Pts',(0.464534180971738,1.06847604194524,12.1322338543628));
#62191=CARTESIAN_POINT('Ctrl Pts',(0.455149630347196,1.185142708612,12.1485988036637));
#62192=CARTESIAN_POINT('Ctrl Pts',(0.436205738465085,1.30000000000031,12.1578652765235));
#62193=CARTESIAN_POINT('Ctrl Pts',(0.195186075930414,-1.3000000000003,12.1705714112126));
#62194=CARTESIAN_POINT('Ctrl Pts',(0.228514698020356,-1.185142708612,12.1611353971354));
#62195=CARTESIAN_POINT('Ctrl Pts',(0.255040140543214,-1.06847604194525,
12.144109066136));
#62196=CARTESIAN_POINT('Ctrl Pts',(0.300602513396229,-0.794772684000888,
12.087239684894));
#62197=CARTESIAN_POINT('Ctrl Pts',(0.304947137552805,-0.636309800095226,
12.0195174794346));
#62198=CARTESIAN_POINT('Ctrl Pts',(0.329109272365874,-0.319434907277173,
11.9490501487589));
#62199=CARTESIAN_POINT('Ctrl Pts',(0.331829184804893,-0.158333333333339,
11.9073002608922));
#62200=CARTESIAN_POINT('Ctrl Pts',(0.363449794366847,0.158333333333342,
11.9049307792051));
#62201=CARTESIAN_POINT('Ctrl Pts',(0.393281919043544,0.319434907277181,
11.9442287386361));
#62202=CARTESIAN_POINT('Ctrl Pts',(0.431631438286729,0.636309800095235,
12.0100375438143));
#62203=CARTESIAN_POINT('Ctrl Pts',(0.461684190827631,0.794772684000876,
12.0745224001291));
#62204=CARTESIAN_POINT('Ctrl Pts',(0.462394759484056,1.06847604194524,12.1292059131272));
#62205=CARTESIAN_POINT('Ctrl Pts',(0.453232364716767,1.185142708612,12.1458937410935));
#62206=CARTESIAN_POINT('Ctrl Pts',(0.434599996339987,1.30000000000031,12.155598930473));
#62207=CARTESIAN_POINT('Ctrl Pts',(0.192488897548456,-1.3000000000003,12.1658782086319));
#62208=CARTESIAN_POINT('Ctrl Pts',(0.225171863855822,-1.185142708612,12.1555653405062));
#62209=CARTESIAN_POINT('Ctrl Pts',(0.251237527370526,-1.06847604194524,
12.1378951147785));
#62210=CARTESIAN_POINT('Ctrl Pts',(0.296167131269672,-0.794772684000886,
12.080076390536));
#62211=CARTESIAN_POINT('Ctrl Pts',(0.300730177358066,-0.636309800095225,
12.0124981823844));
#62212=CARTESIAN_POINT('Ctrl Pts',(0.324933733863143,-0.319434907277173,
11.9419893998123));
#62213=CARTESIAN_POINT('Ctrl Pts',(0.327930015438478,-0.158333333333339,
11.9005074513403));
#62214=CARTESIAN_POINT('Ctrl Pts',(0.35941891215817,0.158333333333342,11.8981758248249));
#62215=CARTESIAN_POINT('Ctrl Pts',(0.388804632316006,0.319434907277181,
11.9372517493087));
#62216=CARTESIAN_POINT('Ctrl Pts',(0.42692250054638,0.636309800095235,12.0031627188469));
#62217=CARTESIAN_POINT('Ctrl Pts',(0.456708971916004,0.794772684000877,
12.0675320420977));
#62218=CARTESIAN_POINT('Ctrl Pts',(0.458013159641032,1.06847604194524,12.1231779190637));
#62219=CARTESIAN_POINT('Ctrl Pts',(0.449313071918081,1.185142708612,12.1405066173595));
#62220=CARTESIAN_POINT('Ctrl Pts',(0.431348361930932,1.30000000000031,12.1510769756955));
#62221=CARTESIAN_POINT('Ctrl Pts',(0.189515797580747,-1.30000000000029,
12.160485154833));
#62222=CARTESIAN_POINT('Ctrl Pts',(0.221664788052325,-1.18514270861199,
12.1491237299431));
#62223=CARTESIAN_POINT('Ctrl Pts',(0.247325613607149,-1.06847604194524,
12.1306901654602));
#62224=CARTESIAN_POINT('Ctrl Pts',(0.29161829515871,-0.794772684000884,
12.0717668866466));
#62225=CARTESIAN_POINT('Ctrl Pts',(0.296199973908871,-0.636309800095224,
12.0044049429406));
#62226=CARTESIAN_POINT('Ctrl Pts',(0.320254171005224,-0.319434907277172,
11.9338955794758));
#62227=CARTESIAN_POINT('Ctrl Pts',(0.323354127894758,-0.158333333333339,
11.8927739101461));
#62228=CARTESIAN_POINT('Ctrl Pts',(0.354696758613631,0.158333333333341,
11.8904824344401));
#62229=CARTESIAN_POINT('Ctrl Pts',(0.383904433670636,0.31943490727718,11.9292162073965));
#62230=CARTESIAN_POINT('Ctrl Pts',(0.421727280585961,0.636309800095234,
11.9952544017964));
#62231=CARTESIAN_POINT('Ctrl Pts',(0.450818647748768,0.794772684000874,
12.0596015040265));
#62232=CARTESIAN_POINT('Ctrl Pts',(0.452745866745147,1.06847604194524,12.1163624018534));
#62233=CARTESIAN_POINT('Ctrl Pts',(0.444616828462124,1.185142708612,12.1344110765862));
#62234=CARTESIAN_POINT('Ctrl Pts',(0.427524530203049,1.30000000000031,12.1459387365809));
#62235=CARTESIAN_POINT('Ctrl Pts',(0.186537501569236,-1.30000000000029,
12.1550913385809));
#62236=CARTESIAN_POINT('Ctrl Pts',(0.218151414965836,-1.18514270861199,
12.1426802740476));
#62237=CARTESIAN_POINT('Ctrl Pts',(0.24341279621573,-1.06847604194524,12.1234812599331));
#62238=CARTESIAN_POINT('Ctrl Pts',(0.28709602034639,-0.794772684000885,
12.0634461751218));
#62239=CARTESIAN_POINT('Ctrl Pts',(0.291744047657623,-0.636309800095224,
11.9962907032332));
#62240=CARTESIAN_POINT('Ctrl Pts',(0.315682053496503,-0.319434907277172,
11.9257734385231));
#62241=CARTESIAN_POINT('Ctrl Pts',(0.318895369098061,-0.158333333333339,
11.8850103867684));
#62242=CARTESIAN_POINT('Ctrl Pts',(0.350082585755415,0.158333333333341,
11.8827600112108));
#62243=CARTESIAN_POINT('Ctrl Pts',(0.379079998488632,0.31943490727718,11.9211565710733));
#62244=CARTESIAN_POINT('Ctrl Pts',(0.416583287835046,0.636309800095234,
11.987326503418));
#62245=CARTESIAN_POINT('Ctrl Pts',(0.444979632628529,0.794772684000875,
12.0516512681616));
#62246=CARTESIAN_POINT('Ctrl Pts',(0.447509768154567,1.06847604194524,12.1095336326909));
#62247=CARTESIAN_POINT('Ctrl Pts',(0.439941051572146,1.185142708612,12.1283060702387));
#62248=CARTESIAN_POINT('Ctrl Pts',(0.423708416488844,1.30000000000031,12.1407958144826));
#62249=CARTESIAN_POINT('Ctrl Pts',(0.183538689402441,-1.30000000000029,
12.1497018523168));
#62250=CARTESIAN_POINT('Ctrl Pts',(0.214582539874455,-1.18514270861199,
12.1362489176074));
#62251=CARTESIAN_POINT('Ctrl Pts',(0.23942873327211,-1.06847604194524,12.1162878162494));
#62252=CARTESIAN_POINT('Ctrl Pts',(0.282510582805826,-0.794772684000885,
12.0551385119952));
#62253=CARTESIAN_POINT('Ctrl Pts',(0.287300547318078,-0.636309800095224,
11.9881719462936));
#62254=CARTESIAN_POINT('Ctrl Pts',(0.311186548055135,-0.319434907277173,
11.9176313249842));
#62255=CARTESIAN_POINT('Ctrl Pts',(0.314572598923691,-0.158333333333339,
11.8772123082057));
#62256=CARTESIAN_POINT('Ctrl Pts',(0.345584121560986,0.158333333333341,
11.8750077977819));
#62257=CARTESIAN_POINT('Ctrl Pts',(0.374223456744635,0.31943490727718,11.9131042924092));
#62258=CARTESIAN_POINT('Ctrl Pts',(0.411440527940432,0.636309800095233,
11.9793948661069));
#62259=CARTESIAN_POINT('Ctrl Pts',(0.439379615769516,0.794772684000875,
12.0436318337386));
#62260=CARTESIAN_POINT('Ctrl Pts',(0.442514805388562,1.06847604194524,12.1026355646076));
#62261=CARTESIAN_POINT('Ctrl Pts',(0.435458341800622,1.185142708612,12.122145507241));
#62262=CARTESIAN_POINT('Ctrl Pts',(0.419988307208882,1.30000000000031,12.1356248637183));
#62263=CARTESIAN_POINT('Ctrl Pts',(0.174871610951366,-1.30000000000029,
12.1349776486484));
#62264=CARTESIAN_POINT('Ctrl Pts',(0.203767783462163,-1.18514270861199,
12.11878748013));
#62265=CARTESIAN_POINT('Ctrl Pts',(0.227142824975559,-1.06847604194524,
12.0968033580528));
#62266=CARTESIAN_POINT('Ctrl Pts',(0.268388929930062,-0.794772684000881,
12.0326304463486));
#62267=CARTESIAN_POINT('Ctrl Pts',(0.274297728470185,-0.636309800095219,
11.9660269653453));
#62268=CARTESIAN_POINT('Ctrl Pts',(0.298739555434465,-0.319434907277169,
11.8952612685211));
#62269=CARTESIAN_POINT('Ctrl Pts',(0.303310176945395,-0.158333333333338,
11.8556154250831));
#62270=CARTESIAN_POINT('Ctrl Pts',(0.333952127921591,0.15833333333334,11.8535106333163));
#62271=CARTESIAN_POINT('Ctrl Pts',(0.360878601011834,0.31943490727718,11.8909619677454));
#62272=CARTESIAN_POINT('Ctrl Pts',(0.397110355900687,0.636309800095231,
11.9576231028531));
#62273=CARTESIAN_POINT('Ctrl Pts',(0.424086307390311,0.794772684000868,
12.0215240402449));
#62274=CARTESIAN_POINT('Ctrl Pts',(0.428914422170458,1.06847604194523,12.0836039242876));
#62275=CARTESIAN_POINT('Ctrl Pts',(0.423248054611277,1.18514270861199,12.1051515713865));
#62276=CARTESIAN_POINT('Ctrl Pts',(0.409825407503875,1.3000000000003,12.1213747840685));
#62277=CARTESIAN_POINT('Ctrl Pts',(0.15989854583247,-1.30000000000028,12.1079962375592));
#62278=CARTESIAN_POINT('Ctrl Pts',(0.186097547729273,-1.18514270861198,
12.0865642185193));
#62279=CARTESIAN_POINT('Ctrl Pts',(0.207480269930789,-1.06847604194523,
12.0607499545607));
#62280=CARTESIAN_POINT('Ctrl Pts',(0.245752066225641,-0.794772684000871,
11.9909899782638));
#62281=CARTESIAN_POINT('Ctrl Pts',(0.251980650996533,-0.636309800095216,
11.9253969188526));
#62282=CARTESIAN_POINT('Ctrl Pts',(0.276297595609869,-0.319434907277169,
11.854478854774));
#62283=CARTESIAN_POINT('Ctrl Pts',(0.282316170182864,-0.158333333333337,
11.8164342936643));
#62284=CARTESIAN_POINT('Ctrl Pts',(0.312123312753905,0.15833333333334,11.8145536268061));
#62285=CARTESIAN_POINT('Ctrl Pts',(0.336365846919138,0.31943490727718,11.8507265227037));
#62286=CARTESIAN_POINT('Ctrl Pts',(0.371839209141617,0.636309800095229,
11.9177954680997));
#62287=CARTESIAN_POINT('Ctrl Pts',(0.398845696192265,0.794772684000865,
11.9806162688803));
#62288=CARTESIAN_POINT('Ctrl Pts',(0.406726498838685,1.06847604194523,12.0483032401435));
#62289=CARTESIAN_POINT('Ctrl Pts',(0.403122927646196,1.18514270861198,12.0736823929196));
#62290=CARTESIAN_POINT('Ctrl Pts',(0.392504477808099,1.30000000000029,12.0951415166614));
#62291=CARTESIAN_POINT('Ctrl Pts',(0.142368228275982,-1.30000000000025,
12.0755162243303));
#62292=CARTESIAN_POINT('Ctrl Pts',(0.164577244832849,-1.18514270861196,
12.0479100423271));
#62293=CARTESIAN_POINT('Ctrl Pts',(0.183321623936367,-1.06847604194521,
12.0175268289581));
#62294=CARTESIAN_POINT('Ctrl Pts',(0.218620883850096,-0.794772684000863,
11.9409200299361));
#62295=CARTESIAN_POINT('Ctrl Pts',(0.228261751117289,-0.636309800095203,
11.8759733523308));
#62296=CARTESIAN_POINT('Ctrl Pts',(0.25292606159555,-0.31943490727716,11.8047686637498));
#62297=CARTESIAN_POINT('Ctrl Pts',(0.258749364371646,-0.158333333333334,
11.7690234910886));
#62298=CARTESIAN_POINT('Ctrl Pts',(0.28707569305352,0.158333333333336,11.7674589260075));
#62299=CARTESIAN_POINT('Ctrl Pts',(0.309534439982334,0.319434907277173,
11.8017008235096));
#62300=CARTESIAN_POINT('Ctrl Pts',(0.34265901455359,0.636309800095215,11.8695937625149));
#62301=CARTESIAN_POINT('Ctrl Pts',(0.365625602803515,0.794772684000848,
11.9321516222108));
#62302=CARTESIAN_POINT('Ctrl Pts',(0.37682644013388,1.0684760419452,12.0066766111699));
#62303=CARTESIAN_POINT('Ctrl Pts',(0.376407879371129,1.18514270861196,12.0364913873925));
#62304=CARTESIAN_POINT('Ctrl Pts',(0.370722330397239,1.30000000000026,12.0638618335402));
#62305=CARTESIAN_POINT('Ctrl Pts',(0.127980957799861,-1.30000000000026,
12.0483368524573));
#62306=CARTESIAN_POINT('Ctrl Pts',(0.148161195722953,-1.18514270861197,
12.0153280736421));
#62307=CARTESIAN_POINT('Ctrl Pts',(0.165386717646749,-1.06847604194522,
11.9810000168413));
#62308=CARTESIAN_POINT('Ctrl Pts',(0.198355134197284,-0.794772684000868,
11.89864754226));
#62309=CARTESIAN_POINT('Ctrl Pts',(0.20788127579913,-0.636309800095204,
11.8348054186726));
#62310=CARTESIAN_POINT('Ctrl Pts',(0.232736015668612,-0.31943490727716,
11.7633758451342));
#62311=CARTESIAN_POINT('Ctrl Pts',(0.240404384429822,-0.158333333333334,
11.729168768354));
#62312=CARTESIAN_POINT('Ctrl Pts',(0.268447431824777,0.158333333333337,
11.7276671885862));
#62313=CARTESIAN_POINT('Ctrl Pts',(0.288975462966633,0.319434907277174,
11.760380825881));
#62314=CARTESIAN_POINT('Ctrl Pts',(0.320930023456981,0.636309800095217,
11.8287352083804));
#62315=CARTESIAN_POINT('Ctrl Pts',(0.342399008811111,0.794772684000848,
11.8905569992644));
#62316=CARTESIAN_POINT('Ctrl Pts',(0.355891004113073,1.06847604194521,11.9709049018606));
#62317=CARTESIAN_POINT('Ctrl Pts',(0.357375294527153,1.18514270861196,12.0046200308278));
#62318=CARTESIAN_POINT('Ctrl Pts',(0.354503690516788,1.30000000000027,12.0372706589114));
#62319=CARTESIAN_POINT('Ctrl Pts',(0.120462273527673,-1.30000000000026,
12.0318473446919));
#62320=CARTESIAN_POINT('Ctrl Pts',(0.138892560461965,-1.18514270861196,
11.9956795717989));
#62321=CARTESIAN_POINT('Ctrl Pts',(0.154959724777024,-1.06847604194521,
11.9590188344525));
#62322=CARTESIAN_POINT('Ctrl Pts',(0.186618802578527,-0.794772684000862,
11.8731863507222));
#62323=CARTESIAN_POINT('Ctrl Pts',(0.197532813745976,-0.636309800095202,
11.8097426426205));
#62324=CARTESIAN_POINT('Ctrl Pts',(0.222728594550386,-0.31943490727716,
11.7381357037543));
#62325=CARTESIAN_POINT('Ctrl Pts',(0.231038606336704,-0.158333333333334,
11.7049345709295));
#62326=CARTESIAN_POINT('Ctrl Pts',(0.25791364597085,0.158333333333336,11.7036669633902));
#62327=CARTESIAN_POINT('Ctrl Pts',(0.276036279865896,0.319434907277173,
11.735710844867));
#62328=CARTESIAN_POINT('Ctrl Pts',(0.306484144357572,0.636309800095215,
11.8045109708308));
#62329=CARTESIAN_POINT('Ctrl Pts',(0.327090231868471,0.794772684000847,
11.8659070582392));
#62330=CARTESIAN_POINT('Ctrl Pts',(0.342261698133297,1.0684760419452,11.9496835149717));
#62331=CARTESIAN_POINT('Ctrl Pts',(0.34515937151465,1.18514270861195,11.9856764880079));
#62332=CARTESIAN_POINT('Ctrl Pts',(0.344387552689541,1.30000000000026,12.0213987101844));
#62333=CARTESIAN_POINT('Ctrl Pts',(0.114879864456069,-1.30000000000026,
12.0209362197056));
#62334=CARTESIAN_POINT('Ctrl Pts',(0.132339498666072,-1.18514270861196,
11.9826291753253));
#62335=CARTESIAN_POINT('Ctrl Pts',(0.147764458409392,-1.06847604194521,
11.9443917057748));
#62336=CARTESIAN_POINT('Ctrl Pts',(0.17869869611581,-0.794772684000861,
11.8562162335089));
#62337=CARTESIAN_POINT('Ctrl Pts',(0.190404690486681,-0.636309800095203,
11.793063869767));
#62338=CARTESIAN_POINT('Ctrl Pts',(0.215752348972689,-0.31943490727716,
11.7213549202783));
#62339=CARTESIAN_POINT('Ctrl Pts',(0.224125089103901,-0.158333333333334,
11.6889015783789));
#62340=CARTESIAN_POINT('Ctrl Pts',(0.250752042061645,0.158333333333336,
11.6876746256021));
#62341=CARTESIAN_POINT('Ctrl Pts',(0.26854110742805,0.319434907277173,11.7190001728044));
#62342=CARTESIAN_POINT('Ctrl Pts',(0.298378106797284,0.636309800095215,
11.7880079299611));
#62343=CARTESIAN_POINT('Ctrl Pts',(0.317784368782244,0.794772684000847,
11.8492406110604));
#62344=CARTESIAN_POINT('Ctrl Pts',(0.333705235052286,1.0684760419452,11.9353877720829));
#62345=CARTESIAN_POINT('Ctrl Pts',(0.337385718999905,1.18514270861196,11.9729402953774));
#62346=CARTESIAN_POINT('Ctrl Pts',(0.337855133813078,1.30000000000026,12.0107554280267));
#62347=CARTESIAN_POINT('Ctrl Pts',(0.10918826148896,-1.30000000000026,12.010040768441));
#62348=CARTESIAN_POINT('Ctrl Pts',(0.125741996817306,-1.18514270861196,
11.9695834866496));
#62349=CARTESIAN_POINT('Ctrl Pts',(0.140526383380073,-1.06847604194521,
11.9297694514619));
#62350=CARTESIAN_POINT('Ctrl Pts',(0.17059372434096,-0.794772684000861,
11.8392770937437));
#62351=CARTESIAN_POINT('Ctrl Pts',(0.182555816696012,-0.636309800095203,
11.7765124961274));
#62352=CARTESIAN_POINT('Ctrl Pts',(0.20815294648653,-0.319434907277161,
11.704682908112));
#62353=CARTESIAN_POINT('Ctrl Pts',(0.217220431067991,-0.158333333333334,
11.6728605536538));
#62354=CARTESIAN_POINT('Ctrl Pts',(0.243858388181379,0.158333333333336,
11.6716291151367));
#62355=CARTESIAN_POINT('Ctrl Pts',(0.261104508940357,0.319434907277172,
11.7022838198051));
#62356=CARTESIAN_POINT('Ctrl Pts',(0.290427661000645,0.636309800095215,
11.7714751231832));
#62357=CARTESIAN_POINT('Ctrl Pts',(0.309093235239651,0.794772684000848,
11.8324306450287));
#62358=CARTESIAN_POINT('Ctrl Pts',(0.325460045223944,1.06847604194521,11.9210137645983));
#62359=CARTESIAN_POINT('Ctrl Pts',(0.329626402260167,1.18514270861196,11.9601929260328));
#62360=CARTESIAN_POINT('Ctrl Pts',(0.330874530740492,1.30000000000026,12.0002068987681));
#62361=CARTESIAN_POINT('Ctrl Pts',(0.103562192797037,-1.30000000000025,
11.9961742881129));
#62362=CARTESIAN_POINT('Ctrl Pts',(0.119158940804234,-1.18514270861196,
11.9529910346458));
#62363=CARTESIAN_POINT('Ctrl Pts',(0.133244708046977,-1.06847604194521,
11.9111830414882));
#62364=CARTESIAN_POINT('Ctrl Pts',(0.162294980389235,-0.794772684000857,
11.8177753400688));
#62365=CARTESIAN_POINT('Ctrl Pts',(0.174380721365818,-0.636309800095201,
11.7555311234643));
#62366=CARTESIAN_POINT('Ctrl Pts',(0.200082511825562,-0.31943490727716,
11.6835887744683));
#62367=CARTESIAN_POINT('Ctrl Pts',(0.209999887910456,-0.158333333333334,
11.65256476212));
#62368=CARTESIAN_POINT('Ctrl Pts',(0.236184727887872,0.158333333333336,
11.6514091690308));
#62369=CARTESIAN_POINT('Ctrl Pts',(0.252155158378876,0.319434907277171,
11.681322438965));
#62370=CARTESIAN_POINT('Ctrl Pts',(0.28039503723386,0.636309800095213,11.7508195704479));
#62371=CARTESIAN_POINT('Ctrl Pts',(0.29776887209576,0.794772684000846,11.8115163260757));
#62372=CARTESIAN_POINT('Ctrl Pts',(0.315300187630474,1.0684760419452,11.9030078072475));
#62373=CARTESIAN_POINT('Ctrl Pts',(0.320585012528572,1.18514270861195,11.9441064816108));
#62374=CARTESIAN_POINT('Ctrl Pts',(0.323566005429051,1.30000000000026,11.9867005582316));
#62375=CARTESIAN_POINT('Ctrl Pts',(0.094794633655618,-1.30000000000025,
11.9798529787367));
#62376=CARTESIAN_POINT('Ctrl Pts',(0.108885876876833,-1.18514270861196,
11.9334650249093));
#62377=CARTESIAN_POINT('Ctrl Pts',(0.122024990313988,-1.06847604194521,
11.8892865355057));
#62378=CARTESIAN_POINT('Ctrl Pts',(0.150179360550364,-0.79477268400086,
11.7923296919279));
#62379=CARTESIAN_POINT('Ctrl Pts',(0.163754820774804,-0.636309800095203,
11.7304776935039));
#62380=CARTESIAN_POINT('Ctrl Pts',(0.190187546892998,-0.319434907277161,
11.6582959379707));
#62381=CARTESIAN_POINT('Ctrl Pts',(0.200831056815098,-0.158333333333334,
11.6282797031472));
#62382=CARTESIAN_POINT('Ctrl Pts',(0.226557352250275,0.158333333333336,
11.627199545701));
#62383=CARTESIAN_POINT('Ctrl Pts',(0.241067094049417,0.319434907277171,
11.6562114221743));
#62384=CARTESIAN_POINT('Ctrl Pts',(0.268204228162709,0.636309800095214,
11.7260385774622));
#62385=CARTESIAN_POINT('Ctrl Pts',(0.284499538638445,0.794772684000848,
11.7863238456839));
#62386=CARTESIAN_POINT('Ctrl Pts',(0.303104086580015,1.06847604194521,11.8813850994134));
#62387=CARTESIAN_POINT('Ctrl Pts',(0.309408290174266,1.18514270861196,11.92486252824));
#62388=CARTESIAN_POINT('Ctrl Pts',(0.313963477925306,1.30000000000026,11.9706688915202));
#62389=CARTESIAN_POINT('Ctrl Pts',(0.0830130309313852,-1.30000000000024,
11.9521871509239));
#62390=CARTESIAN_POINT('Ctrl Pts',(0.0957161656842548,-1.18514270861195,
11.9002711856679));
#62391=CARTESIAN_POINT('Ctrl Pts',(0.107860818724359,-1.06847604194521,
11.8520460684592));
#62392=CARTESIAN_POINT('Ctrl Pts',(0.13462719229614,-0.794772684000858,
11.7491629976463));
#62393=CARTESIAN_POINT('Ctrl Pts',(0.148671537687174,-0.636309800095198,
11.6883128523622));
#62394=CARTESIAN_POINT('Ctrl Pts',(0.175072801269439,-0.319434907277158,
11.6159447109649));
#62395=CARTESIAN_POINT('Ctrl Pts',(0.186253878137799,-0.158333333333333,
11.5877234799558));
#62396=CARTESIAN_POINT('Ctrl Pts',(0.211375734943978,0.158333333333335,
11.5867225045778));
#62397=CARTESIAN_POINT('Ctrl Pts',(0.225013277830667,0.319434907277169,
11.6139407036506));
#62398=CARTESIAN_POINT('Ctrl Pts',(0.250401099768228,0.636309800095208,
11.6842741193368));
#62399=CARTESIAN_POINT('Ctrl Pts',(0.263796170364388,0.79477268400084,11.7440370831602));
#62400=CARTESIAN_POINT('Ctrl Pts',(0.283344363081088,1.0684760419452,11.8451960582538));
#62401=CARTESIAN_POINT('Ctrl Pts',(0.291000962720118,1.18514270861195,11.8927073822637));
#62402=CARTESIAN_POINT('Ctrl Pts',(0.297852473703045,1.30000000000026,11.9439420582748));
#62403=CARTESIAN_POINT('Ctrl Pts',(0.0682437123209798,-1.30000000000025,
11.9190458604761));
#62404=CARTESIAN_POINT('Ctrl Pts',(0.078446405555705,-1.18514270861195,
11.8605989204779));
#62405=CARTESIAN_POINT('Ctrl Pts',(0.0890788816669909,-1.06847604194521,
11.8075487239736));
#62406=CARTESIAN_POINT('Ctrl Pts',(0.114634912926241,-0.794772684000859,
11.6974597144792));
#62407=CARTESIAN_POINT('Ctrl Pts',(0.131740333363184,-0.636309800095201,
11.6374429325233));
#62408=CARTESIAN_POINT('Ctrl Pts',(0.1594292559344,-0.31943490727716,11.5646392296698));
#62409=CARTESIAN_POINT('Ctrl Pts',(0.171645869628339,-0.158333333333333,
11.5385002879484));
#62410=CARTESIAN_POINT('Ctrl Pts',(0.195246818017136,0.158333333333336,
11.5377061193558));
#62411=CARTESIAN_POINT('Ctrl Pts',(0.205343216370943,0.319434907277171,
11.563161128943));
#62412=CARTESIAN_POINT('Ctrl Pts',(0.228351159935257,0.636309800095212,
11.6341226238268));
#62413=CARTESIAN_POINT('Ctrl Pts',(0.240273808775317,0.794772684000846,
11.6929087520959));
#62414=CARTESIAN_POINT('Ctrl Pts',(0.261870995302839,1.0684760419452,11.8012335718407));
#62415=CARTESIAN_POINT('Ctrl Pts',(0.271386990239266,1.18514270861195,11.8535526181072));
#62416=CARTESIAN_POINT('Ctrl Pts',(0.281070358318985,1.30000000000026,11.9113009100027));
#62417=CARTESIAN_POINT('Ctrl Pts',(0.0556483962276951,-1.30000000000024,
11.8855803936001));
#62418=CARTESIAN_POINT('Ctrl Pts',(0.0644266534852743,-1.18514270861195,
11.8204697935768));
#62419=CARTESIAN_POINT('Ctrl Pts',(0.0742122621370922,-1.0684760419452,
11.7625226330136));
#62420=CARTESIAN_POINT('Ctrl Pts',(0.0991461589677387,-0.794772684000853,
11.6452020780171));
#62421=CARTESIAN_POINT('Ctrl Pts',(0.117818837276392,-0.636309800095197,
11.5862860789068));
#62422=CARTESIAN_POINT('Ctrl Pts',(0.146885729055631,-0.319434907277159,
11.5130795221398));
#62423=CARTESIAN_POINT('Ctrl Pts',(0.161014727437592,-0.158333333333332,
11.4889316353716));
#62424=CARTESIAN_POINT('Ctrl Pts',(0.183847560566396,0.158333333333335,
11.4881825033546));
#62425=CARTESIAN_POINT('Ctrl Pts',(0.191540343583512,0.319434907277169,
11.5115859798794));
#62426=CARTESIAN_POINT('Ctrl Pts',(0.211041728444421,0.636309800095208,
11.5832569907542));
#62427=CARTESIAN_POINT('Ctrl Pts',(0.218742224588253,0.794772684000841,
11.6414480623763));
#62428=CARTESIAN_POINT('Ctrl Pts',(0.240246692293113,1.0684760419452,11.7572633594441));
#62429=CARTESIAN_POINT('Ctrl Pts',(0.250868610018655,1.18514270861195,11.814519967009));
#62430=CARTESIAN_POINT('Ctrl Pts',(0.262803958219365,1.30000000000025,11.8789010314179));
#62431=CARTESIAN_POINT('Ctrl Pts',(0.0464357783185983,-1.30000000000024,
11.86333871748));
#62432=CARTESIAN_POINT('Ctrl Pts',(0.0542499946932897,-1.18514270861195,
11.793739927263));
#62433=CARTESIAN_POINT('Ctrl Pts',(0.0636295362538139,-1.0684760419452,
11.7324730561432));
#62434=CARTESIAN_POINT('Ctrl Pts',(0.0889143679509853,-0.794772684000858,
11.6101827273706));
#62435=CARTESIAN_POINT('Ctrl Pts',(0.110340899142229,-0.636309800095199,
11.5517926056029));
#62436=CARTESIAN_POINT('Ctrl Pts',(0.140424748904,-0.319434907277159,11.4783003446474));
#62437=CARTESIAN_POINT('Ctrl Pts',(0.154212363334051,-0.158333333333333,
11.4556985708264));
#62438=CARTESIAN_POINT('Ctrl Pts',(0.17615831927619,0.158333333333335,11.455019647929));
#62439=CARTESIAN_POINT('Ctrl Pts',(0.182754644700643,0.319434907277169,
11.4769817094759));
#62440=CARTESIAN_POINT('Ctrl Pts',(0.200554841333362,0.636309800095209,
11.549011184157));
#62441=CARTESIAN_POINT('Ctrl Pts',(0.206119407133801,0.794772684000844,
11.606659084153));
#62442=CARTESIAN_POINT('Ctrl Pts',(0.228088731804076,1.0684760419452,11.7274091082837));
#62443=CARTESIAN_POINT('Ctrl Pts',(0.23959717134933,1.18514270861195,11.7879587027551));
#62444=CARTESIAN_POINT('Ctrl Pts',(0.253104343833782,1.30000000000025,11.8567896804811));
#62445=CARTESIAN_POINT('Ctrl Pts',(0.0406518797623858,-1.30000000000024,
11.8465564726809));
#62446=CARTESIAN_POINT('Ctrl Pts',(0.0478819400995714,-1.18514270861195,
11.773657943409));
#62447=CARTESIAN_POINT('Ctrl Pts',(0.0569887955685448,-1.0684760419452,
11.7099645477952));
#62448=CARTESIAN_POINT('Ctrl Pts',(0.0823632257280734,-0.794772684000853,
11.5840857623383));
#62449=CARTESIAN_POINT('Ctrl Pts',(0.104982086020124,-0.636309800095198,
11.5262348933961));
#62450=CARTESIAN_POINT('Ctrl Pts',(0.136074315850756,-0.319434907277159,
11.4525214372116));
#62451=CARTESIAN_POINT('Ctrl Pts',(0.150878273702948,-0.158333333333333,
11.4308793229505));
#62452=CARTESIAN_POINT('Ctrl Pts',(0.172369064798244,0.158333333333335,
11.4302102994935));
#62453=CARTESIAN_POINT('Ctrl Pts',(0.177494189085355,0.319434907277169,
11.4511811093708));
#62454=CARTESIAN_POINT('Ctrl Pts',(0.193358242024117,0.636309800095208,
11.5235364590285));
#62455=CARTESIAN_POINT('Ctrl Pts',(0.197067540665844,0.794772684000842,
11.580789800071));
#62456=CARTESIAN_POINT('Ctrl Pts',(0.218448911255057,1.0684760419452,11.7052970606092));
#62457=CARTESIAN_POINT('Ctrl Pts',(0.230124991373547,1.18514270861195,11.7683449680977));
#62458=CARTESIAN_POINT('Ctrl Pts',(0.244221948540316,1.30000000000025,11.8405462034364));
#62459=CARTESIAN_POINT('Ctrl Pts',(0.034830413167812,-1.30000000000025,
11.829676335823));
#62460=CARTESIAN_POINT('Ctrl Pts',(0.0413983638315718,-1.18514270861195,
11.7533037192462));
#62461=CARTESIAN_POINT('Ctrl Pts',(0.050314467195016,-1.06847604194521,
11.6870370189958));
#62462=CARTESIAN_POINT('Ctrl Pts',(0.0763371521075432,-0.794772684000857,
11.5572943732051));
#62463=CARTESIAN_POINT('Ctrl Pts',(0.102225806674094,-0.6363098000952,11.4997609588548));
#62464=CARTESIAN_POINT('Ctrl Pts',(0.13310772074771,-0.31943490727716,11.4259272518795));
#62465=CARTESIAN_POINT('Ctrl Pts',(0.144692433467357,-0.158333333333333,
11.4057563231153));
#62466=CARTESIAN_POINT('Ctrl Pts',(0.165044457335305,0.158333333333335,
11.4051666385386));
#62467=CARTESIAN_POINT('Ctrl Pts',(0.171551107388644,0.319434907277168,
11.4247803349145));
#62468=CARTESIAN_POINT('Ctrl Pts',(0.186729604417125,0.636309800095209,
11.4973467940944));
#62469=CARTESIAN_POINT('Ctrl Pts',(0.188181266030554,0.794772684000846,
11.5542555919596));
#62470=CARTESIAN_POINT('Ctrl Pts',(0.209496799931565,1.0684760419452,11.6826400382386));
#62471=CARTESIAN_POINT('Ctrl Pts',(0.221636035209642,1.18514270861195,11.7482662320662));
#62472=CARTESIAN_POINT('Ctrl Pts',(0.236687800958419,1.30000000000025,11.82394575004));
#62473=CARTESIAN_POINT('Ctrl Pts',(0.0300137202382451,-1.30000000000024,
11.815727424252));
#62474=CARTESIAN_POINT('Ctrl Pts',(0.0369536379353412,-1.18514270861195,
11.7366024621951));
#62475=CARTESIAN_POINT('Ctrl Pts',(0.0459456534800434,-1.0684760419452,
11.6683507799072));
#62476=CARTESIAN_POINT('Ctrl Pts',(0.0714597647835856,-0.794772684000853,
11.5357951915782));
#62477=CARTESIAN_POINT('Ctrl Pts',(0.0956780461528079,-0.636309800095197,
11.4789939209136));
#62478=CARTESIAN_POINT('Ctrl Pts',(0.12571304728649,-0.319434907277159,
11.4052172446615));
#62479=CARTESIAN_POINT('Ctrl Pts',(0.137179957999219,-0.158333333333332,
11.3860007057705));
#62480=CARTESIAN_POINT('Ctrl Pts',(0.158144120393544,0.158333333333335,
11.385327828888));
#62481=CARTESIAN_POINT('Ctrl Pts',(0.166297992339798,0.319434907277168,
11.4037986346615));
#62482=CARTESIAN_POINT('Ctrl Pts',(0.181701848327912,0.636309800095208,
11.4763531120574));
#62483=CARTESIAN_POINT('Ctrl Pts',(0.181519653365159,0.794772684000841,
11.5328622516889));
#62484=CARTESIAN_POINT('Ctrl Pts',(0.202836953204498,1.0684760419452,11.6641532144601));
#62485=CARTESIAN_POINT('Ctrl Pts',(0.215272326681509,1.18514270861195,11.7317564899875));
#62486=CARTESIAN_POINT('Ctrl Pts',(0.230915604418885,1.30000000000025,11.8101320480683));
#62487=CARTESIAN_POINT('Ctrl Pts',(0.0249486472265458,-1.30000000000024,
11.7987654117141));
#62488=CARTESIAN_POINT('Ctrl Pts',(0.0322960695121722,-1.18514270861195,
11.7159494251139));
#62489=CARTESIAN_POINT('Ctrl Pts',(0.0411713710709376,-1.0684760419452,
11.6450237733314));
#62490=CARTESIAN_POINT('Ctrl Pts',(0.0652047999418275,-0.794772684000854,
11.5086403811676));
#62491=CARTESIAN_POINT('Ctrl Pts',(0.0861507442337192,-0.636309800095198,
11.4527126715445));
#62492=CARTESIAN_POINT('Ctrl Pts',(0.11401151949034,-0.319434907277159,
11.378979926875));
#62493=CARTESIAN_POINT('Ctrl Pts',(0.12516253329486,-0.158333333333333,
11.3610604540291));
#62494=CARTESIAN_POINT('Ctrl Pts',(0.146020139137245,0.158333333333335,
11.3603760542832));
#62495=CARTESIAN_POINT('Ctrl Pts',(0.154705006362177,0.319434907277168,
11.3774873687404));
#62496=CARTESIAN_POINT('Ctrl Pts',(0.171410852286353,0.636309800095208,
11.4500781278508));
#62497=CARTESIAN_POINT('Ctrl Pts',(0.1726664600724,0.794772684000841,11.505919375511));
#62498=CARTESIAN_POINT('Ctrl Pts',(0.195303874973743,1.0684760419452,11.6411090107818));
#62499=CARTESIAN_POINT('Ctrl Pts',(0.208193542904413,1.18514270861195,11.7113846754377));
#62500=CARTESIAN_POINT('Ctrl Pts',(0.224173980653852,1.30000000000026,11.7934174209105));
#62501=CARTESIAN_POINT('Ctrl Pts',(0.0213943747864571,-1.30000000000024,
11.7872275498583));
#62502=CARTESIAN_POINT('Ctrl Pts',(0.0303808199748146,-1.18514270861194,
11.7017443481177));
#62503=CARTESIAN_POINT('Ctrl Pts',(0.0397026858022263,-1.0684760419452,
11.6290281458668));
#62504=CARTESIAN_POINT('Ctrl Pts',(0.0620129494732972,-0.794772684000851,
11.4905334946914));
#62505=CARTESIAN_POINT('Ctrl Pts',(0.0765909966193375,-0.636309800095197,
11.4363224854433));
#62506=CARTESIAN_POINT('Ctrl Pts',(0.101057989717432,-0.319434907277159,
11.3633819083365));
#62507=CARTESIAN_POINT('Ctrl Pts',(0.112567852729614,-0.158333333333332,
11.3464812380319));
#62508=CARTESIAN_POINT('Ctrl Pts',(0.133278717910193,0.158333333333334,
11.3458490652972));
#62509=CARTESIAN_POINT('Ctrl Pts',(0.141607349608986,0.319434907277167,
11.3620417363435));
#62510=CARTESIAN_POINT('Ctrl Pts',(0.161103853485779,0.636309800095206,
11.4338490762767));
#62511=CARTESIAN_POINT('Ctrl Pts',(0.167600922680342,0.79477268400084,11.4878246451703));
#62512=CARTESIAN_POINT('Ctrl Pts',(0.192015477656447,1.0684760419452,11.6251313100261));
#62513=CARTESIAN_POINT('Ctrl Pts',(0.204772182759206,1.18514270861195,11.6972293577846));
#62514=CARTESIAN_POINT('Ctrl Pts',(0.219717436763987,1.30000000000025,11.781990485799));
#62515=CARTESIAN_POINT('Ctrl Pts',(0.0165023515695648,-1.30000000000024,
11.780151978414));
#62516=CARTESIAN_POINT('Ctrl Pts',(0.0256069538907778,-1.18514270861194,
11.6948905764801));
#62517=CARTESIAN_POINT('Ctrl Pts',(0.0347010954711953,-1.0684760419452,
11.6224333483287));
#62518=CARTESIAN_POINT('Ctrl Pts',(0.0556862153948441,-0.794772684000851,
11.4846228591836));
#62519=CARTESIAN_POINT('Ctrl Pts',(0.0677962068234778,-0.636309800095197,
11.4311131089277));
#62520=CARTESIAN_POINT('Ctrl Pts',(0.0906597384266766,-0.319434907277159,
11.3586954735785));
#62521=CARTESIAN_POINT('Ctrl Pts',(0.102179986998412,-0.158333333333332,
11.3417434974973));
#62522=CARTESIAN_POINT('Ctrl Pts',(0.12267336889205,0.158333333333334,11.341205069791));
#62523=CARTESIAN_POINT('Ctrl Pts',(0.130506918224618,0.319434907277167,
11.357626654509));
#62524=CARTESIAN_POINT('Ctrl Pts',(0.151708180499798,0.636309800095206,
11.4289311819364));
#62525=CARTESIAN_POINT('Ctrl Pts',(0.161724215836605,0.79477268400084,11.4819406028846));
#62526=CARTESIAN_POINT('Ctrl Pts',(0.187312562460002,1.0684760419452,11.618589325336));
#62527=CARTESIAN_POINT('Ctrl Pts',(0.199984062839927,1.18514270861195,11.690494969693));
#62528=CARTESIAN_POINT('Ctrl Pts',(0.214250816488192,1.30000000000025,11.7751560897922));
#62529=CARTESIAN_POINT('Ctrl Pts',(0.0165023515695838,-1.3,11.7801519784138));
#62530=CARTESIAN_POINT('Ctrl Pts',(0.0256069538907905,-1.18514270861178,
11.69489057648));
#62531=CARTESIAN_POINT('Ctrl Pts',(0.0347010954712016,-1.06847604194512,
11.6224333483286));
#62532=CARTESIAN_POINT('Ctrl Pts',(0.0556862153948441,-0.794772684000851,
11.4846228591836));
#62533=CARTESIAN_POINT('Ctrl Pts',(0.0677962068234778,-0.636309800095197,
11.4311131089277));
#62534=CARTESIAN_POINT('Ctrl Pts',(0.0906597384266766,-0.319434907277159,
11.3586954735785));
#62535=CARTESIAN_POINT('Ctrl Pts',(0.102179986998412,-0.158333333333332,
11.3417434974973));
#62536=CARTESIAN_POINT('Ctrl Pts',(0.12267336889205,0.158333333333334,11.341205069791));
#62537=CARTESIAN_POINT('Ctrl Pts',(0.130506918224618,0.319434907277167,
11.357626654509));
#62538=CARTESIAN_POINT('Ctrl Pts',(0.151708180499798,0.636309800095206,
11.4289311819364));
#62539=CARTESIAN_POINT('Ctrl Pts',(0.161724215836605,0.79477268400084,11.4819406028846));
#62540=CARTESIAN_POINT('Ctrl Pts',(0.187312562459994,1.06847604194511,11.6185893253359));
#62541=CARTESIAN_POINT('Ctrl Pts',(0.199984062839908,1.18514270861178,11.6904949696929));
#62542=CARTESIAN_POINT('Ctrl Pts',(0.214250816488161,1.3,11.775156089792));
#62543=CARTESIAN_POINT('',(0.213846491495602,-1.2,12.1453786182733));
#62544=CARTESIAN_POINT('Ctrl Pts',(0.213846491495599,-1.2,12.1453786182733));
#62545=CARTESIAN_POINT('Ctrl Pts',(0.195932239642712,-1.22117287959761,
12.1249605953279));
#62546=CARTESIAN_POINT('Ctrl Pts',(0.17709346156536,-1.24191631337165,12.1049180269287));
#62547=CARTESIAN_POINT('Ctrl Pts',(0.149359662911878,-1.27453035159476,
12.0731904402628));
#62548=CARTESIAN_POINT('Ctrl Pts',(0.135822023537843,-1.29050619980739,
12.0576008960751));
#62549=CARTESIAN_POINT('Ctrl Pts',(0.12821877836405,-1.30000000000026,12.0483048527163));
#62550=CARTESIAN_POINT('',(0.370132012244428,-0.653834841366415,12.1361424506532));
#62551=CARTESIAN_POINT('Ctrl Pts',(0.370132012242185,-0.653834841365131,
12.136142450691));
#62552=CARTESIAN_POINT('Ctrl Pts',(0.354420225940763,-0.715934737885519,
12.1373205842513));
#62553=CARTESIAN_POINT('Ctrl Pts',(0.332824972003976,-0.793120943268795,
12.1388328601562));
#62554=CARTESIAN_POINT('Ctrl Pts',(0.306961911531932,-0.886126995183554,
12.1404786488211));
#62555=CARTESIAN_POINT('Ctrl Pts',(0.300477517120967,-0.909338780067549,
12.1408773304724));
#62556=CARTESIAN_POINT('Ctrl Pts',(0.267922703219645,-1.02407623900668,
12.1428079516095));
#62557=CARTESIAN_POINT('Ctrl Pts',(0.241155291200104,-1.11212798593213,
12.1441977398301));
#62558=CARTESIAN_POINT('Ctrl Pts',(0.2138464914956,-1.2,12.1453786182733));
#62559=CARTESIAN_POINT('Ctrl Pts',(0.509087305687303,0.653834841531096,
12.123751630128));
#62560=CARTESIAN_POINT('Ctrl Pts',(0.487797291982429,0.575994836847891,
12.0880522833113));
#62561=CARTESIAN_POINT('Ctrl Pts',(0.469153198145619,0.493638162905769,
12.0582419843226));
#62562=CARTESIAN_POINT('Ctrl Pts',(0.440252074501338,0.338128653655767,
12.0166877772658));
#62563=CARTESIAN_POINT('Ctrl Pts',(0.429043836054997,0.265646903379949,
12.0027380309224));
#62564=CARTESIAN_POINT('Ctrl Pts',(0.41067468427847,0.129700315862073,11.9867102146548));
#62565=CARTESIAN_POINT('Ctrl Pts',(0.40318577277248,0.0666145002772442,
11.9831901735331));
#62566=CARTESIAN_POINT('Ctrl Pts',(0.389879396129507,-0.0595448625857636,
11.9840041603447));
#62567=CARTESIAN_POINT('Ctrl Pts',(0.383960588584499,-0.122774529296895,
11.9883274493114));
#62568=CARTESIAN_POINT('Ctrl Pts',(0.373635521614742,-0.260111751750111,
12.0063195248107));
#62569=CARTESIAN_POINT('Ctrl Pts',(0.369700559967849,-0.333922237377205,
12.0215526341913));
#62570=CARTESIAN_POINT('Ctrl Pts',(0.365867536509685,-0.491193347292214,
12.0662344420976));
#62571=CARTESIAN_POINT('Ctrl Pts',(0.366579815351903,-0.57435183090168,
12.0978053593006));
#62572=CARTESIAN_POINT('Ctrl Pts',(0.370132012193589,-0.653834841383324,
12.1361424506229));
#62573=CARTESIAN_POINT('Ctrl Pts',(0.0165023515695837,-1.3,11.7801519784138));
#62574=CARTESIAN_POINT('Ctrl Pts',(0.0256069538907904,-1.18514270861178,
11.69489057648));
#62575=CARTESIAN_POINT('Ctrl Pts',(0.0347010954712016,-1.06847604194512,
11.6224333483286));
#62576=CARTESIAN_POINT('Ctrl Pts',(0.0556862153948441,-0.794772684000851,
11.4846228591836));
#62577=CARTESIAN_POINT('Ctrl Pts',(0.0677962068234778,-0.636309800095196,
11.4311131089277));
#62578=CARTESIAN_POINT('Ctrl Pts',(0.0906597384266765,-0.319434907277159,
11.3586954735785));
#62579=CARTESIAN_POINT('Ctrl Pts',(0.102179986998412,-0.158333333333332,
11.3417434974973));
#62580=CARTESIAN_POINT('Ctrl Pts',(0.12267336889205,0.158333333333334,11.341205069791));
#62581=CARTESIAN_POINT('Ctrl Pts',(0.130506918224618,0.319434907277167,
11.357626654509));
#62582=CARTESIAN_POINT('Ctrl Pts',(0.151708180499798,0.636309800095206,
11.4289311819363));
#62583=CARTESIAN_POINT('Ctrl Pts',(0.161724215836605,0.79477268400084,11.4819406028846));
#62584=CARTESIAN_POINT('Ctrl Pts',(0.187312562459994,1.06847604194511,11.6185893253359));
#62585=CARTESIAN_POINT('Ctrl Pts',(0.199984062839908,1.18514270861178,11.6904949696929));
#62586=CARTESIAN_POINT('Ctrl Pts',(0.214250816488161,1.3,11.775156089792));
#62587=CARTESIAN_POINT('Ctrl Pts',(-0.0604153711163311,-1.3,11.7784866822066));
#62588=CARTESIAN_POINT('Ctrl Pts',(-0.0495900516861092,-1.18514270861178,
11.6934253742177));
#62589=CARTESIAN_POINT('Ctrl Pts',(-0.0393034571725303,-1.06847604194512,
11.6211520073311));
#62590=CARTESIAN_POINT('Ctrl Pts',(-0.0167839283489728,-0.794772684000851,
11.4837287737506));
#62591=CARTESIAN_POINT('Ctrl Pts',(-0.00537192228428078,-0.636309800095196,
11.4303857999306));
#62592=CARTESIAN_POINT('Ctrl Pts',(0.0169375195429119,-0.319434907277159,
11.3583392005554));
#62593=CARTESIAN_POINT('Ctrl Pts',(0.0272288683682581,-0.158333333333332,
11.3415640215952));
#62594=CARTESIAN_POINT('Ctrl Pts',(0.0477222502618957,0.158333333333334,
11.3413845456931));
#62595=CARTESIAN_POINT('Ctrl Pts',(0.0567846993408533,0.319434907277167,
11.3579829275322));
#62596=CARTESIAN_POINT('Ctrl Pts',(0.0785400513920397,0.636309800095206,
11.4296584909335));
#62597=CARTESIAN_POINT('Ctrl Pts',(0.0892540720927883,0.79477268400084,
11.4828346883176));
#62598=CARTESIAN_POINT('Ctrl Pts',(0.113308009816262,1.06847604194511,11.6198706663335));
#62599=CARTESIAN_POINT('Ctrl Pts',(0.124787057263008,1.18514270861178,11.6919601719553));
#62600=CARTESIAN_POINT('Ctrl Pts',(0.137333093802246,1.3,11.7768213859993));
#62601=CARTESIAN_POINT('Ctrl Pts',(-0.137333093802246,-1.3,11.7768213859993));
#62602=CARTESIAN_POINT('Ctrl Pts',(-0.124787057263009,-1.18514270861178,
11.6919601719553));
#62603=CARTESIAN_POINT('Ctrl Pts',(-0.113308009816262,-1.06847604194512,
11.6198706663335));
#62604=CARTESIAN_POINT('Ctrl Pts',(-0.0892540720927895,-0.794772684000851,
11.4828346883176));
#62605=CARTESIAN_POINT('Ctrl Pts',(-0.0785400513920391,-0.636309800095196,
11.4296584909335));
#62606=CARTESIAN_POINT('Ctrl Pts',(-0.0567846993408526,-0.319434907277159,
11.3579829275322));
#62607=CARTESIAN_POINT('Ctrl Pts',(-0.0477222502618955,-0.158333333333332,
11.3413845456931));
#62608=CARTESIAN_POINT('Ctrl Pts',(-0.027228868368258,0.158333333333334,
11.3415640215952));
#62609=CARTESIAN_POINT('Ctrl Pts',(-0.0169375195429113,0.319434907277167,
11.3583392005554));
#62610=CARTESIAN_POINT('Ctrl Pts',(0.00537192228428136,0.636309800095206,
11.4303857999306));
#62611=CARTESIAN_POINT('Ctrl Pts',(0.0167839283489716,0.79477268400084,
11.4837287737506));
#62612=CARTESIAN_POINT('Ctrl Pts',(0.03930345717253,1.06847604194511,11.6211520073311));
#62613=CARTESIAN_POINT('Ctrl Pts',(0.0495900516861087,1.18514270861178,
11.6934253742177));
#62614=CARTESIAN_POINT('Ctrl Pts',(0.0604153711163312,1.3,11.7784866822066));
#62615=CARTESIAN_POINT('Ctrl Pts',(-0.214250816488161,-1.3,11.775156089792));
#62616=CARTESIAN_POINT('Ctrl Pts',(-0.199984062839908,-1.18514270861178,
11.6904949696929));
#62617=CARTESIAN_POINT('Ctrl Pts',(-0.187312562459994,-1.06847604194512,
11.6185893253359));
#62618=CARTESIAN_POINT('Ctrl Pts',(-0.161724215836606,-0.794772684000851,
11.4819406028846));
#62619=CARTESIAN_POINT('Ctrl Pts',(-0.151708180499798,-0.636309800095196,
11.4289311819363));
#62620=CARTESIAN_POINT('Ctrl Pts',(-0.130506918224617,-0.319434907277159,
11.357626654509));
#62621=CARTESIAN_POINT('Ctrl Pts',(-0.122673368892049,-0.158333333333332,
11.341205069791));
#62622=CARTESIAN_POINT('Ctrl Pts',(-0.102179986998412,0.158333333333334,
11.3417434974973));
#62623=CARTESIAN_POINT('Ctrl Pts',(-0.0906597384266759,0.319434907277167,
11.3586954735785));
#62624=CARTESIAN_POINT('Ctrl Pts',(-0.0677962068234772,0.636309800095206,
11.4311131089277));
#62625=CARTESIAN_POINT('Ctrl Pts',(-0.055686215394845,0.79477268400084,
11.4846228591836));
#62626=CARTESIAN_POINT('Ctrl Pts',(-0.0347010954712021,1.06847604194511,
11.6224333483286));
#62627=CARTESIAN_POINT('Ctrl Pts',(-0.0256069538907909,1.18514270861178,
11.69489057648));
#62628=CARTESIAN_POINT('Ctrl Pts',(-0.0165023515695837,1.3,11.7801519784138));
#62629=CARTESIAN_POINT('Ctrl Pts',(-0.214250816488161,-1.3,11.775156089792));
#62630=CARTESIAN_POINT('Ctrl Pts',(-0.199984062839908,-1.18514270861178,
11.6904949696929));
#62631=CARTESIAN_POINT('Ctrl Pts',(-0.187312562459994,-1.06847604194512,
11.6185893253359));
#62632=CARTESIAN_POINT('Ctrl Pts',(-0.161724215836606,-0.794772684000851,
11.4819406028846));
#62633=CARTESIAN_POINT('Ctrl Pts',(-0.151708180499798,-0.636309800095197,
11.4289311819364));
#62634=CARTESIAN_POINT('Ctrl Pts',(-0.130506918224617,-0.319434907277159,
11.357626654509));
#62635=CARTESIAN_POINT('Ctrl Pts',(-0.122673368892049,-0.158333333333332,
11.341205069791));
#62636=CARTESIAN_POINT('Ctrl Pts',(-0.102179986998412,0.158333333333334,
11.3417434974973));
#62637=CARTESIAN_POINT('Ctrl Pts',(-0.0906597384266759,0.319434907277167,
11.3586954735785));
#62638=CARTESIAN_POINT('Ctrl Pts',(-0.0677962068234772,0.636309800095206,
11.4311131089277));
#62639=CARTESIAN_POINT('Ctrl Pts',(-0.055686215394845,0.79477268400084,
11.4846228591836));
#62640=CARTESIAN_POINT('Ctrl Pts',(-0.0347010954712021,1.06847604194511,
11.6224333483286));
#62641=CARTESIAN_POINT('Ctrl Pts',(-0.025606953890791,1.18514270861178,
11.69489057648));
#62642=CARTESIAN_POINT('Ctrl Pts',(-0.0165023515695838,1.3,11.7801519784138));
#62643=CARTESIAN_POINT('Ctrl Pts',(-0.214250816488491,-1.30000000000266,
11.775156089794));
#62644=CARTESIAN_POINT('Ctrl Pts',(-0.199984062840104,-1.18514270861358,
11.690494969694));
#62645=CARTESIAN_POINT('Ctrl Pts',(-0.18731256246008,-1.06847604194603,
11.6185893253364));
#62646=CARTESIAN_POINT('Ctrl Pts',(-0.161724215836606,-0.794772684000851,
11.4819406028846));
#62647=CARTESIAN_POINT('Ctrl Pts',(-0.151708180499798,-0.636309800095197,
11.4289311819364));
#62648=CARTESIAN_POINT('Ctrl Pts',(-0.130506918224617,-0.319434907277159,
11.357626654509));
#62649=CARTESIAN_POINT('Ctrl Pts',(-0.122673368892049,-0.158333333333332,
11.341205069791));
#62650=CARTESIAN_POINT('Ctrl Pts',(-0.102179986998412,0.158333333333334,
11.3417434974973));
#62651=CARTESIAN_POINT('Ctrl Pts',(-0.0906597384266759,0.319434907277167,
11.3586954735785));
#62652=CARTESIAN_POINT('Ctrl Pts',(-0.0677962068234772,0.636309800095206,
11.4311131089277));
#62653=CARTESIAN_POINT('Ctrl Pts',(-0.055686215394845,0.79477268400084,
11.4846228591836));
#62654=CARTESIAN_POINT('Ctrl Pts',(-0.0347010954709978,1.06847604194777,
11.62243334833));
#62655=CARTESIAN_POINT('Ctrl Pts',(-0.0256069538903818,1.18514270861702,
11.6948905764833));
#62656=CARTESIAN_POINT('Ctrl Pts',(-0.0165023515689693,1.30000000000775,
11.7801519784196));
#62657=CARTESIAN_POINT('Ctrl Pts',(-0.219717436762998,-1.30000000000266,
11.7819904857412));
#62658=CARTESIAN_POINT('Ctrl Pts',(-0.204772182758638,-1.18514270861358,
11.6972293577337));
#62659=CARTESIAN_POINT('Ctrl Pts',(-0.192015477656179,-1.06847604194603,
11.6251313099799));
#62660=CARTESIAN_POINT('Ctrl Pts',(-0.167600922680588,-0.794772684000851,
11.4878246451312));
#62661=CARTESIAN_POINT('Ctrl Pts',(-0.161103853486099,-0.636309800095197,
11.4338490762469));
#62662=CARTESIAN_POINT('Ctrl Pts',(-0.141607349608946,-0.319434907277159,
11.3620417362896));
#62663=CARTESIAN_POINT('Ctrl Pts',(-0.133278717909188,-0.158333333333332,
11.3458490651824));
#62664=CARTESIAN_POINT('Ctrl Pts',(-0.112567852728384,0.158333333333334,
11.3464812379208));
#62665=CARTESIAN_POINT('Ctrl Pts',(-0.10105798971678,0.319434907277167,
11.363381908291));
#62666=CARTESIAN_POINT('Ctrl Pts',(-0.0765909966189224,0.636309800095206,
11.4363224854275));
#62667=CARTESIAN_POINT('Ctrl Pts',(-0.0620129494727472,0.79477268400084,
11.4905334946661));
#62668=CARTESIAN_POINT('Ctrl Pts',(-0.0397026858016881,1.06847604194777,
11.6290281458399));
#62669=CARTESIAN_POINT('Ctrl Pts',(-0.030380819974229,1.18514270861702,
11.7017443480897));
#62670=CARTESIAN_POINT('Ctrl Pts',(-0.0213943747858902,1.30000000000775,
11.7872275498281));
#62671=CARTESIAN_POINT('Ctrl Pts',(-0.224217870079186,-1.30000000000266,
11.793407741607));
#62672=CARTESIAN_POINT('Ctrl Pts',(-0.208244333473234,-1.18514270861359,
11.7113717526455));
#62673=CARTESIAN_POINT('Ctrl Pts',(-0.195355471940572,-1.06847604194604,
11.6410945205255));
#62674=CARTESIAN_POINT('Ctrl Pts',(-0.172705839898739,-0.794772684000856,
11.5059051360521));
#62675=CARTESIAN_POINT('Ctrl Pts',(-0.17141959502437,-0.636309800095198,
11.4500701232598));
#62676=CARTESIAN_POINT('Ctrl Pts',(-0.154685054000868,-0.319434907277159,
11.3774846305103));
#62677=CARTESIAN_POINT('Ctrl Pts',(-0.145979289299972,-0.158333333333332,
11.3603771369061));
#62678=CARTESIAN_POINT('Ctrl Pts',(-0.125122661406262,0.158333333333334,
11.3610623482316));
#62679=CARTESIAN_POINT('Ctrl Pts',(-0.114003801242036,0.319434907277166,
11.3789777248218));
#62680=CARTESIAN_POINT('Ctrl Pts',(-0.0861527771105432,0.636309800095206,
11.4527090703651));
#62681=CARTESIAN_POINT('Ctrl Pts',(-0.0651925831004888,0.794772684000841,
11.5086371330806));
#62682=CARTESIAN_POINT('Ctrl Pts',(-0.0411580507325554,1.06847604194777,
11.6450217831126));
#62683=CARTESIAN_POINT('Ctrl Pts',(-0.0322838315682777,1.18514270861703,
11.71594832617));
#62684=CARTESIAN_POINT('Ctrl Pts',(-0.0249390517347361,1.30000000000775,
11.7987655508345));
#62685=CARTESIAN_POINT('Ctrl Pts',(-0.230940212073702,-1.30000000000266,
11.8101274281025));
#62686=CARTESIAN_POINT('Ctrl Pts',(-0.215296597918111,-1.18514270861359,
11.7317529065375));
#62687=CARTESIAN_POINT('Ctrl Pts',(-0.202859343717702,-1.06847604194603,
11.6641508310356));
#62688=CARTESIAN_POINT('Ctrl Pts',(-0.181534131377252,-0.794772684000852,
11.5328630183039));
#62689=CARTESIAN_POINT('Ctrl Pts',(-0.181705445881087,-0.636309800095196,
11.4763566179852));
#62690=CARTESIAN_POINT('Ctrl Pts',(-0.166289710338157,-0.319434907277158,
11.4038054324094));
#62691=CARTESIAN_POINT('Ctrl Pts',(-0.158119436476584,-0.158333333333332,
11.3853366219702));
#62692=CARTESIAN_POINT('Ctrl Pts',(-0.137170837613514,0.158333333333334,
11.3860097881351));
#62693=CARTESIAN_POINT('Ctrl Pts',(-0.125758787670006,0.319434907277168,
11.4052233409097));
#62694=CARTESIAN_POINT('Ctrl Pts',(-0.0957207317599793,0.636309800095206,
11.4789999219884));
#62695=CARTESIAN_POINT('Ctrl Pts',(-0.0714304791785025,0.794772684000838,
11.5358058689093));
#62696=CARTESIAN_POINT('Ctrl Pts',(-0.0459133378491548,1.06847604194777,
11.6683582509209));
#62697=CARTESIAN_POINT('Ctrl Pts',(-0.0369336206498608,1.18514270861702,
11.7366069404878));
#62698=CARTESIAN_POINT('Ctrl Pts',(-0.0300196112296146,1.30000000000775,
11.8157273049977));
#62699=CARTESIAN_POINT('Ctrl Pts',(-0.236830809019557,-1.30000000000266,
11.823913013989));
#62700=CARTESIAN_POINT('Ctrl Pts',(-0.221807828841873,-1.18514270861359,
11.7482186534331));
#62701=CARTESIAN_POINT('Ctrl Pts',(-0.209674709327399,-1.06847604194603,
11.6825842381735));
#62702=CARTESIAN_POINT('Ctrl Pts',(-0.188320932273469,-0.794772684000854,
11.5541960949243));
#62703=CARTESIAN_POINT('Ctrl Pts',(-0.186759959728292,-0.636309800095198,
11.4973087358865));
#62704=CARTESIAN_POINT('Ctrl Pts',(-0.17148164451981,-0.31943490727716,
11.4247589069605));
#62705=CARTESIAN_POINT('Ctrl Pts',(-0.164914018978241,-0.158333333333333,
11.4051578558322));
#62706=CARTESIAN_POINT('Ctrl Pts',(-0.144542563833041,0.158333333333335,
11.4057504239017));
#62707=CARTESIAN_POINT('Ctrl Pts',(-0.133007072754958,0.319434907277168,
11.4259090530163));
#62708=CARTESIAN_POINT('Ctrl Pts',(-0.102169758375363,0.636309800095207,
11.4997371727135));
#62709=CARTESIAN_POINT('Ctrl Pts',(-0.0763311114729764,0.794772684000843,
11.5572650096014));
#62710=CARTESIAN_POINT('Ctrl Pts',(-0.0503084407492601,1.06847604194778,
11.6870176439549));
#62711=CARTESIAN_POINT('Ctrl Pts',(-0.0413782275088885,1.18514270861702,
11.7532925032257));
#62712=CARTESIAN_POINT('Ctrl Pts',(-0.0347820509496016,1.30000000000775,
11.8296771141638));
#62713=CARTESIAN_POINT('Ctrl Pts',(-0.242947140261799,-1.30000000000266,
11.8377863890196));
#62714=CARTESIAN_POINT('Ctrl Pts',(-0.228673177411667,-1.18514270861359,
11.7650169188838));
#62715=CARTESIAN_POINT('Ctrl Pts',(-0.216911379186633,-1.06847604194603,
11.701547333098));
#62716=CARTESIAN_POINT('Ctrl Pts',(-0.19554287518801,-0.794772684000852,
11.5764044861699));
#62717=CARTESIAN_POINT('Ctrl Pts',(-0.192246096408202,-0.636309800095196,
11.519203297661));
#62718=CARTESIAN_POINT('Ctrl Pts',(-0.176523859962701,-0.319434907277158,
11.4468119320853));
#62719=CARTESIAN_POINT('Ctrl Pts',(-0.171159810408635,-0.158333333333333,
11.4260654238642));
#62720=CARTESIAN_POINT('Ctrl Pts',(-0.149913038564751,0.158333333333334,
11.4267203975001));
#62721=CARTESIAN_POINT('Ctrl Pts',(-0.135766465861496,0.319434907277169,
11.4481164809824));
#62722=CARTESIAN_POINT('Ctrl Pts',(-0.104674146178431,0.636309800095208,
11.5218529767954));
#62723=CARTESIAN_POINT('Ctrl Pts',(-0.0812829026006441,0.79477268400084,
11.579666864191));
#62724=CARTESIAN_POINT('Ctrl Pts',(-0.0557924094028948,1.06847604194777,
11.7061748677036));
#62725=CARTESIAN_POINT('Ctrl Pts',(-0.0467597412619023,1.18514270861702,
11.7702841191655));
#62726=CARTESIAN_POINT('Ctrl Pts',(-0.0397282949695003,1.30000000000775,
11.8437419949516));
#62727=CARTESIAN_POINT('Ctrl Pts',(-0.250450467575642,-1.30000000000266,
11.8513121660939));
#62728=CARTESIAN_POINT('Ctrl Pts',(-0.236823957280526,-1.18514270861359,
11.7813326284548));
#62729=CARTESIAN_POINT('Ctrl Pts',(-0.22527978638569,-1.06847604194603,
11.7199380521404));
#62730=CARTESIAN_POINT('Ctrl Pts',(-0.20342106280045,-0.794772684000851,
11.5979372769874));
#62731=CARTESIAN_POINT('Ctrl Pts',(-0.198182879193841,-0.636309800095198,
11.5404728242816));
#62732=CARTESIAN_POINT('Ctrl Pts',(-0.180833769426929,-0.31943490727716,
11.4683672228574));
#62733=CARTESIAN_POINT('Ctrl Pts',(-0.174706384337292,-0.158333333333333,
11.4467454432747));
#62734=CARTESIAN_POINT('Ctrl Pts',(-0.152838862898622,0.158333333333335,
11.4474283582768));
#62735=CARTESIAN_POINT('Ctrl Pts',(-0.138654662265025,0.319434907277169,
11.4697025037864));
#62736=CARTESIAN_POINT('Ctrl Pts',(-0.108291876353905,0.636309800095209,
11.5432613801654));
#62737=CARTESIAN_POINT('Ctrl Pts',(-0.0866786973629504,0.794772684000843,
11.6014545180862));
#62738=CARTESIAN_POINT('Ctrl Pts',(-0.0613805082616765,1.06847604194778,
11.7249531277311));
#62739=CARTESIAN_POINT('Ctrl Pts',(-0.0520560587818162,1.18514270861703,
11.7870408114846));
#62740=CARTESIAN_POINT('Ctrl Pts',(-0.0443578084938825,1.30000000000775,
11.8577582069501));
#62741=CARTESIAN_POINT('Ctrl Pts',(-0.260323420711465,-1.30000000000266,
11.873400837634));
#62742=CARTESIAN_POINT('Ctrl Pts',(-0.247802116813471,-1.18514270861359,
11.8079670508444));
#62743=CARTESIAN_POINT('Ctrl Pts',(-0.236836054686001,-1.06847604194603,
11.7499259468651));
#62744=CARTESIAN_POINT('Ctrl Pts',(-0.215095177033385,-0.794772684000849,
11.6329179617837));
#62745=CARTESIAN_POINT('Ctrl Pts',(-0.208135190489906,-0.636309800095196,
11.5748097817095));
#62746=CARTESIAN_POINT('Ctrl Pts',(-0.189098646525768,-0.319434907277158,
11.5030319137751));
#62747=CARTESIAN_POINT('Ctrl Pts',(-0.181564680695925,-0.158333333333333,
11.4799869089716));
#62748=CARTESIAN_POINT('Ctrl Pts',(-0.159079342990061,0.158333333333334,
11.4807109001114));
#62749=CARTESIAN_POINT('Ctrl Pts',(-0.145397680171436,0.319434907277169,
11.5044627691746));
#62750=CARTESIAN_POINT('Ctrl Pts',(-0.11604690429894,0.636309800095208,
11.5777502411529));
#62751=CARTESIAN_POINT('Ctrl Pts',(-0.0961679003060289,0.794772684000839,
11.6365852973473));
#62752=CARTESIAN_POINT('Ctrl Pts',(-0.0711454710836636,1.06847604194777,
11.7551190889297));
#62753=CARTESIAN_POINT('Ctrl Pts',(-0.0615643462518385,1.18514270861702,
11.8138663524707));
#62754=CARTESIAN_POINT('Ctrl Pts',(-0.0532333790263047,1.30000000000775,
11.8800519932859));
#62755=CARTESIAN_POINT('Ctrl Pts',(-0.276239090050472,-1.30000000000266,
11.9032333655254));
#62756=CARTESIAN_POINT('Ctrl Pts',(-0.266429290422055,-1.18514270861359,
11.8437129298302));
#62757=CARTESIAN_POINT('Ctrl Pts',(-0.256910355903995,-1.06847604194603,
11.7900873376451));
#62758=CARTESIAN_POINT('Ctrl Pts',(-0.235591669503331,-0.794772684000857,
11.6798197597031));
#62759=CARTESIAN_POINT('Ctrl Pts',(-0.224279524630662,-0.636309800095201,
11.621290618903));
#62760=CARTESIAN_POINT('Ctrl Pts',(-0.201942143076302,-0.319434907277161,
11.5502056857409));
#62761=CARTESIAN_POINT('Ctrl Pts',(-0.192515727923751,-0.158333333333333,
11.5252832663945));
#62762=CARTESIAN_POINT('Ctrl Pts',(-0.168732153072857,0.158333333333335,
11.5261075273927));
#62763=CARTESIAN_POINT('Ctrl Pts',(-0.15525846429931,0.319434907277169,
11.5517979296741));
#62764=CARTESIAN_POINT('Ctrl Pts',(-0.127350849694823,0.63630980009521,
11.6246764575031));
#62765=CARTESIAN_POINT('Ctrl Pts',(-0.110979158576652,0.794772684000847,
11.6842968419898));
#62766=CARTESIAN_POINT('Ctrl Pts',(-0.0858860639788656,1.06847604194778,
11.7961802575163));
#62767=CARTESIAN_POINT('Ctrl Pts',(-0.0754350815714248,1.18514270861703,
11.8504719847924));
#62768=CARTESIAN_POINT('Ctrl Pts',(-0.0653949876172695,1.30000000000775,
11.9106252544515));
#62769=CARTESIAN_POINT('Ctrl Pts',(-0.29517793742003,-1.30000000000266,
11.9384674305417));
#62770=CARTESIAN_POINT('Ctrl Pts',(-0.287639116641684,-1.18514270861359,
11.8861840873237));
#62771=CARTESIAN_POINT('Ctrl Pts',(-0.279540159415899,-1.06847604194604,
11.8378938566315));
#62772=CARTESIAN_POINT('Ctrl Pts',(-0.259535920785081,-0.794772684000854,
11.7355586520591));
#62773=CARTESIAN_POINT('Ctrl Pts',(-0.246694283457694,-0.636309800095197,
11.6759025600909));
#62774=CARTESIAN_POINT('Ctrl Pts',(-0.221681184675174,-0.319434907277158,
11.6054673769956));
#62775=CARTESIAN_POINT('Ctrl Pts',(-0.208422081944555,-0.158333333333332,
11.5785818413453));
#62776=CARTESIAN_POINT('Ctrl Pts',(-0.183440518011101,0.158333333333334,
11.5795669581184));
#62777=CARTESIAN_POINT('Ctrl Pts',(-0.17205280598463,0.319434907277167,
11.607442706844));
#62778=CARTESIAN_POINT('Ctrl Pts',(-0.145498397797482,0.636309800095206,
11.6798741210746));
#62779=CARTESIAN_POINT('Ctrl Pts',(-0.131176827593208,0.794772684000839,
11.7405507697081));
#62780=CARTESIAN_POINT('Ctrl Pts',(-0.104598028284302,1.06847604194777,
11.8446411509602));
#62781=CARTESIAN_POINT('Ctrl Pts',(-0.0926448526882476,1.18514270861703,
11.8936822166786));
#62782=CARTESIAN_POINT('Ctrl Pts',(-0.0802434788755316,1.30000000000775,
11.9467074789994));
#62783=CARTESIAN_POINT('Ctrl Pts',(-0.309070134152884,-1.30000000000266,
11.9626521575258));
#62784=CARTESIAN_POINT('Ctrl Pts',(-0.304257903017002,-1.18514270861359,
11.9151094210709));
#62785=CARTESIAN_POINT('Ctrl Pts',(-0.297805472165891,-1.06847604194604,
11.870356610646));
#62786=CARTESIAN_POINT('Ctrl Pts',(-0.279109876632523,-0.794772684000858,
11.7734139530484));
#62787=CARTESIAN_POINT('Ctrl Pts',(-0.263186794327446,-0.636309800095199,
11.7134052465165));
#62788=CARTESIAN_POINT('Ctrl Pts',(-0.236216413283395,-0.319434907277159,
11.6435063095043));
#62789=CARTESIAN_POINT('Ctrl Pts',(-0.221758045974766,-0.158333333333333,
11.6150838982541));
#62790=CARTESIAN_POINT('Ctrl Pts',(-0.19597593177251,0.158333333333335,
11.6161785319858));
#62791=CARTESIAN_POINT('Ctrl Pts',(-0.185020774202201,0.319434907277168,
11.6456538669924));
#62792=CARTESIAN_POINT('Ctrl Pts',(-0.158724055077794,0.636309800095208,
11.7178674543161));
#62793=CARTESIAN_POINT('Ctrl Pts',(-0.145416493623235,0.794772684000842,
11.7793663528091));
#62794=CARTESIAN_POINT('Ctrl Pts',(-0.117930848075837,1.06847604194778,
11.8780739513503));
#62795=CARTESIAN_POINT('Ctrl Pts',(-0.105163024546976,1.18514270861703,
11.9234613046999));
#62796=CARTESIAN_POINT('Ctrl Pts',(-0.09152489500333,1.30000000000776,11.971509149467));
#62797=CARTESIAN_POINT('Ctrl Pts',(-0.318947568796887,-1.30000000000267,
11.9786313169475));
#62798=CARTESIAN_POINT('Ctrl Pts',(-0.315273910384892,-1.18514270861359,
11.9343985878693));
#62799=CARTESIAN_POINT('Ctrl Pts',(-0.309537129818828,-1.06847604194604,
11.89209096527));
#62800=CARTESIAN_POINT('Ctrl Pts',(-0.2915177941702,-0.794772684000857,
11.7987992745377));
#62801=CARTESIAN_POINT('Ctrl Pts',(-0.274625041771405,-0.6363098000952,
11.7383363870941));
#62802=CARTESIAN_POINT('Ctrl Pts',(-0.246787850417295,-0.31943490727716,
11.6687157402135));
#62803=CARTESIAN_POINT('Ctrl Pts',(-0.231396951287163,-0.158333333333333,
11.6392967488708));
#62804=CARTESIAN_POINT('Ctrl Pts',(-0.205226404564591,0.158333333333335,
11.6404513861524));
#62805=CARTESIAN_POINT('Ctrl Pts',(-0.19470126514578,0.319434907277169,
11.670989837913));
#62806=CARTESIAN_POINT('Ctrl Pts',(-0.16871252234342,0.636309800095209,
11.7430340505382));
#62807=CARTESIAN_POINT('Ctrl Pts',(-0.156409891339114,0.794772684000843,
11.8050042227834));
#62808=CARTESIAN_POINT('Ctrl Pts',(-0.127831439852261,1.06847604194778,
11.9001890837079));
#62809=CARTESIAN_POINT('Ctrl Pts',(-0.114124307099296,1.18514270861703,
11.9432009124148));
#62810=CARTESIAN_POINT('Ctrl Pts',(-0.0990805943061879,1.30000000000776,
11.9880225704805));
#62811=CARTESIAN_POINT('Ctrl Pts',(-0.325037630289391,-1.30000000000267,
11.9893873191805));
#62812=CARTESIAN_POINT('Ctrl Pts',(-0.322785150534061,-1.18514270861359,
11.9472150763738));
#62813=CARTESIAN_POINT('Ctrl Pts',(-0.317960794414666,-1.06847604194604,
11.9064425391265));
#62814=CARTESIAN_POINT('Ctrl Pts',(-0.300874017766708,-0.794772684000856,
11.8154834214201));
#62815=CARTESIAN_POINT('Ctrl Pts',(-0.28289635081279,-0.636309800095199,
11.7548283828312));
#62816=CARTESIAN_POINT('Ctrl Pts',(-0.254121503986549,-0.31943490727716,
11.6854673897822));
#62817=CARTESIAN_POINT('Ctrl Pts',(-0.237602570414715,-0.158333333333333,
11.6554698969414));
#62818=CARTESIAN_POINT('Ctrl Pts',(-0.211105296395253,0.158333333333335,
11.6566798966747));
#62819=CARTESIAN_POINT('Ctrl Pts',(-0.20125636216096,0.319434907277169,
11.6878608173297));
#62820=CARTESIAN_POINT('Ctrl Pts',(-0.175794578537588,0.636309800095209,
11.7597406177987));
#62821=CARTESIAN_POINT('Ctrl Pts',(-0.164323991831707,0.794772684000842,
11.82199900382));
#62822=CARTESIAN_POINT('Ctrl Pts',(-0.135233099564808,1.06847604194778,
11.9148039470579));
#62823=CARTESIAN_POINT('Ctrl Pts',(-0.120977627755776,1.18514270861703,
11.9562217008324));
#62824=CARTESIAN_POINT('Ctrl Pts',(-0.105059053476416,1.30000000000776,
11.9988853872153));
#62825=CARTESIAN_POINT('Ctrl Pts',(-0.3326990773971,-1.30000000000267,12.0028153799187));
#62826=CARTESIAN_POINT('Ctrl Pts',(-0.33185156874756,-1.18514270861359,
11.9632961021561));
#62827=CARTESIAN_POINT('Ctrl Pts',(-0.327940416842498,-1.06847604194604,
11.9244888658819));
#62828=CARTESIAN_POINT('Ctrl Pts',(-0.311827244718624,-0.794772684000857,
11.8364813450097));
#62829=CARTESIAN_POINT('Ctrl Pts',(-0.292912661410954,-0.6363098000952,
11.7754878653476));
#62830=CARTESIAN_POINT('Ctrl Pts',(-0.263172738621346,-0.31943490727716,
11.7064116664776));
#62831=CARTESIAN_POINT('Ctrl Pts',(-0.245372626632432,-0.158333333333333,
11.6756830038836));
#62832=CARTESIAN_POINT('Ctrl Pts',(-0.21843054828428,0.158333333333335,
11.6769697718535));
#62833=CARTESIAN_POINT('Ctrl Pts',(-0.209429046196659,0.319434907277169,
11.7089467663506));
#62834=CARTESIAN_POINT('Ctrl Pts',(-0.184003779677574,0.63630980009521,
11.7807223104256));
#62835=CARTESIAN_POINT('Ctrl Pts',(-0.172594457528252,0.794772684000843,
11.843509730546));
#62836=CARTESIAN_POINT('Ctrl Pts',(-0.14234409618874,1.06847604194778,11.9334185969874));
#62837=CARTESIAN_POINT('Ctrl Pts',(-0.127315850771895,1.18514270861703,
11.972852455381));
#62838=CARTESIAN_POINT('Ctrl Pts',(-0.110353620475885,1.30000000000776,
12.0128019553371));
#62839=CARTESIAN_POINT('Ctrl Pts',(-0.342890406495062,-1.30000000000267,
12.0187005673102));
#62840=CARTESIAN_POINT('Ctrl Pts',(-0.343404801620718,-1.18514270861359,
11.9824364379119));
#62841=CARTESIAN_POINT('Ctrl Pts',(-0.340328286663603,-1.06847604194604,
11.9460455915638));
#62842=CARTESIAN_POINT('Ctrl Pts',(-0.324925201007721,-0.794772684000854,
11.8616827150327));
#62843=CARTESIAN_POINT('Ctrl Pts',(-0.30440917001716,-0.636309800095197,
11.8003810198176));
#62844=CARTESIAN_POINT('Ctrl Pts',(-0.27406327984717,-0.319434907277158,
11.7315459342188));
#62845=CARTESIAN_POINT('Ctrl Pts',(-0.256131817511993,-0.158333333333333,
11.6996667708295));
#62846=CARTESIAN_POINT('Ctrl Pts',(-0.229344633515742,0.158333333333334,
11.7009131340153));
#62847=CARTESIAN_POINT('Ctrl Pts',(-0.220929192197765,0.319434907277169,
11.7339227857933));
#62848=CARTESIAN_POINT('Ctrl Pts',(-0.195814697950992,0.636309800095208,
11.8055326520784));
#62849=CARTESIAN_POINT('Ctrl Pts',(-0.185004960135747,0.794772684000838,
11.86886708947));
#62850=CARTESIAN_POINT('Ctrl Pts',(-0.153575863981641,1.06847604194777,
11.9552861106441));
#62851=CARTESIAN_POINT('Ctrl Pts',(-0.137630621387517,1.18514270861703,
11.9923508536253));
#62852=CARTESIAN_POINT('Ctrl Pts',(-0.119344627361765,1.30000000000776,
12.0290727474613));
#62853=CARTESIAN_POINT('Ctrl Pts',(-0.35278967854841,-1.30000000000267,
12.03461531483));
#62854=CARTESIAN_POINT('Ctrl Pts',(-0.355844257705039,-1.18514270861359,
12.0013185840351));
#62855=CARTESIAN_POINT('Ctrl Pts',(-0.354443939977227,-1.06847604194604,
11.967144126374));
#62856=CARTESIAN_POINT('Ctrl Pts',(-0.340917222891307,-0.794772684000859,
11.8861665679506));
#62857=CARTESIAN_POINT('Ctrl Pts',(-0.318967482009493,-0.636309800095201,
11.8245812730303));
#62858=CARTESIAN_POINT('Ctrl Pts',(-0.286878403158749,-0.319434907277161,
11.7562488211688));
#62859=CARTESIAN_POINT('Ctrl Pts',(-0.266663621926033,-0.158333333333333,
11.7236716820602));
#62860=CARTESIAN_POINT('Ctrl Pts',(-0.238406038584845,0.158333333333335,
11.7252091998553));
#62861=CARTESIAN_POINT('Ctrl Pts',(-0.23001997737375,0.319434907277169,
11.7593411259456));
#62862=CARTESIAN_POINT('Ctrl Pts',(-0.205249587648581,0.63630980009521,
11.8307702147613));
#62863=CARTESIAN_POINT('Ctrl Pts',(-0.196579192702014,0.794772684000844,
11.8943575162252));
#62864=CARTESIAN_POINT('Ctrl Pts',(-0.163974351536508,1.06847604194778,
11.9772659406248));
#62865=CARTESIAN_POINT('Ctrl Pts',(-0.146811779920227,1.18514270861703,
12.0120066261991));
#62866=CARTESIAN_POINT('Ctrl Pts',(-0.126600064299955,1.30000000000777,
12.0456000124843));
#62867=CARTESIAN_POINT('Ctrl Pts',(-0.362458227405669,-1.30000000000267,
12.0505988729736));
#62868=CARTESIAN_POINT('Ctrl Pts',(-0.366646738676606,-1.18514270861359,
12.0206060978921));
#62869=CARTESIAN_POINT('Ctrl Pts',(-0.36606713314898,-1.06847604194604,
11.9888494879981));
#62870=CARTESIAN_POINT('Ctrl Pts',(-0.353712824767352,-0.794772684000856,
11.9114105549845));
#62871=CARTESIAN_POINT('Ctrl Pts',(-0.331642810172518,-0.636309800095202,
11.8491847076909));
#62872=CARTESIAN_POINT('Ctrl Pts',(-0.2992336617953,-0.319434907277162,
11.7810309769482));
#62873=CARTESIAN_POINT('Ctrl Pts',(-0.277779816053976,-0.158333333333334,
11.7475495932847));
#62874=CARTESIAN_POINT('Ctrl Pts',(-0.249752596286747,0.158333333333336,
11.7490435296266));
#62875=CARTESIAN_POINT('Ctrl Pts',(-0.243245132670091,0.319434907277169,
11.7839537572776));
#62876=CARTESIAN_POINT('Ctrl Pts',(-0.21843059765032,0.636309800095211,
11.8552831172205));
#62877=CARTESIAN_POINT('Ctrl Pts',(-0.20843821376195,0.794772684000847,
11.9197789423395));
#62878=CARTESIAN_POINT('Ctrl Pts',(-0.174222980806344,1.06847604194778,
11.999286491599));
#62879=CARTESIAN_POINT('Ctrl Pts',(-0.156269703867267,1.18514270861703,
12.0316394533571));
#62880=CARTESIAN_POINT('Ctrl Pts',(-0.135173656536452,1.30000000000776,
12.0619295048437));
#62881=CARTESIAN_POINT('Ctrl Pts',(-0.375985236281673,-1.30000000000266,
12.0717119172313));
#62882=CARTESIAN_POINT('Ctrl Pts',(-0.383369052387185,-1.18514270861359,
12.0457045367987));
#62883=CARTESIAN_POINT('Ctrl Pts',(-0.384870749705919,-1.06847604194604,
12.0169282275241));
#62884=CARTESIAN_POINT('Ctrl Pts',(-0.374751099814466,-0.794772684000857,
11.9440524168714));
#62885=CARTESIAN_POINT('Ctrl Pts',(-0.350303398133014,-0.636309800095203,
11.881548963167));
#62886=CARTESIAN_POINT('Ctrl Pts',(-0.316274483201399,-0.319434907277163,
11.8139400195225));
#62887=CARTESIAN_POINT('Ctrl Pts',(-0.293277812625114,-0.158333333333334,
11.7792453136778));
#62888=CARTESIAN_POINT('Ctrl Pts',(-0.26415322173086,0.158333333333336,
11.7809700651923));
#62889=CARTESIAN_POINT('Ctrl Pts',(-0.257612583060493,0.319434907277169,
11.8173973229585));
#62890=CARTESIAN_POINT('Ctrl Pts',(-0.233157480947777,0.636309800095211,
11.8885035723848));
#62891=CARTESIAN_POINT('Ctrl Pts',(-0.22547365179888,0.794772684000849,
11.9534155283702));
#62892=CARTESIAN_POINT('Ctrl Pts',(-0.189605353394397,1.06847604194778,
12.0282785934395));
#62893=CARTESIAN_POINT('Ctrl Pts',(-0.170088629217099,1.18514270861703,
12.0575394195504));
#62894=CARTESIAN_POINT('Ctrl Pts',(-0.146581238190558,1.30000000000776,
12.0836556248532));
#62895=CARTESIAN_POINT('Ctrl Pts',(-0.388002912938967,-1.30000000000267,
12.0886184370541));
#62896=CARTESIAN_POINT('Ctrl Pts',(-0.397056775472148,-1.18514270861359,
12.0660581729704));
#62897=CARTESIAN_POINT('Ctrl Pts',(-0.399691866065676,-1.06847604194604,
12.0398281403293));
#62898=CARTESIAN_POINT('Ctrl Pts',(-0.390950805233306,-0.794772684000856,
11.9707536181264));
#62899=CARTESIAN_POINT('Ctrl Pts',(-0.365574569069799,-0.6363098000952,
11.9077858528155));
#62900=CARTESIAN_POINT('Ctrl Pts',(-0.331012395793997,-0.319434907277161,
11.8404456471227));
#62901=CARTESIAN_POINT('Ctrl Pts',(-0.307244324656631,-0.158333333333333,
11.8046648039295));
#62902=CARTESIAN_POINT('Ctrl Pts',(-0.277878312564256,0.158333333333335,
11.8064520917464));
#62903=CARTESIAN_POINT('Ctrl Pts',(-0.271921220308894,0.31943490727717,
11.8440078854625));
#62904=CARTESIAN_POINT('Ctrl Pts',(-0.247398506714636,0.636309800095211,
11.9150137979284));
#62905=CARTESIAN_POINT('Ctrl Pts',(-0.240133095739699,0.794772684000846,
11.980543623939));
#62906=CARTESIAN_POINT('Ctrl Pts',(-0.202402311331478,1.06847604194778,
12.0517514903152));
#62907=CARTESIAN_POINT('Ctrl Pts',(-0.181594603253596,1.18514270861703,
12.0785149889845));
#62908=CARTESIAN_POINT('Ctrl Pts',(-0.156311445605007,1.30000000000775,
12.1012187394798));
#62909=CARTESIAN_POINT('Ctrl Pts',(-0.398046289221613,-1.30000000000267,
12.1044479065164));
#62910=CARTESIAN_POINT('Ctrl Pts',(-0.409380371236153,-1.18514270861359,
12.0848926609609));
#62911=CARTESIAN_POINT('Ctrl Pts',(-0.413583277518684,-1.06847604194604,
12.0608879172386));
#62912=CARTESIAN_POINT('Ctrl Pts',(-0.406818389292128,-0.794772684000856,
11.9951529262238));
#62913=CARTESIAN_POINT('Ctrl Pts',(-0.380431605342912,-0.636309800095201,
11.9317906969053));
#62914=CARTESIAN_POINT('Ctrl Pts',(-0.345050833649757,-0.319434907277161,
11.8647783468055));
#62915=CARTESIAN_POINT('Ctrl Pts',(-0.31985344599858,-0.158333333333334,
11.8281735574692));
#62916=CARTESIAN_POINT('Ctrl Pts',(-0.28998327846249,0.158333333333336,
11.8300842442891));
#62917=CARTESIAN_POINT('Ctrl Pts',(-0.28483235918426,0.319434907277171,
11.8686067719113));
#62918=CARTESIAN_POINT('Ctrl Pts',(-0.26034368584684,0.636309800095212,
11.9394966901605));
#62919=CARTESIAN_POINT('Ctrl Pts',(-0.253528051313759,0.794772684000847,
12.0055925283148));
#62920=CARTESIAN_POINT('Ctrl Pts',(-0.214078183372511,1.06847604194778,
12.0734284420653));
#62921=CARTESIAN_POINT('Ctrl Pts',(-0.192057012409329,1.18514270861703,
12.0978912232342));
#62922=CARTESIAN_POINT('Ctrl Pts',(-0.165091056553272,1.30000000000776,
12.1174531320774));
#62923=CARTESIAN_POINT('Ctrl Pts',(-0.405212661371279,-1.30000000000267,
12.1148940485206));
#62924=CARTESIAN_POINT('Ctrl Pts',(-0.417447748107665,-1.18514270861359,
12.0974907272638));
#62925=CARTESIAN_POINT('Ctrl Pts',(-0.422345660903717,-1.06847604194604,
12.0750525418653));
#62926=CARTESIAN_POINT('Ctrl Pts',(-0.416710479687932,-0.794772684000857,
12.011584301463));
#62927=CARTESIAN_POINT('Ctrl Pts',(-0.390689544578296,-0.6363098000952,
11.9476998442955));
#62928=CARTESIAN_POINT('Ctrl Pts',(-0.355023316128746,-0.319434907277161,
11.8808422569316));
#62929=CARTESIAN_POINT('Ctrl Pts',(-0.328684331227664,-0.158333333333334,
11.8437431505064));
#62930=CARTESIAN_POINT('Ctrl Pts',(-0.298123930914947,0.158333333333335,
11.8458196167914));
#62931=CARTESIAN_POINT('Ctrl Pts',(-0.292918278048133,0.31943490727717,
11.88511715802));
#62932=CARTESIAN_POINT('Ctrl Pts',(-0.268339992311274,0.636309800095211,
11.9559559166057));
#62933=CARTESIAN_POINT('Ctrl Pts',(-0.262312628808647,0.794772684000846,
12.0223207693886));
#62934=CARTESIAN_POINT('Ctrl Pts',(-0.221903226169962,1.06847604194778,
12.0878687935682));
#62935=CARTESIAN_POINT('Ctrl Pts',(-0.199111159992541,1.18514270861703,
12.1107901379001));
#62936=CARTESIAN_POINT('Ctrl Pts',(-0.171018760724269,1.30000000000775,
12.12825951569));
#62937=CARTESIAN_POINT('Ctrl Pts',(-0.41534867580558,-1.30000000000267,
12.129153621754));
#62938=CARTESIAN_POINT('Ctrl Pts',(-0.429894776557093,-1.1851427086136,
12.1144297574352));
#62939=CARTESIAN_POINT('Ctrl Pts',(-0.436318583411802,-1.06847604194604,
12.0939970326791));
#62940=CARTESIAN_POINT('Ctrl Pts',(-0.432394738563412,-0.79477268400086,
12.0336047412763));
#62941=CARTESIAN_POINT('Ctrl Pts',(-0.404819836431124,-0.636309800095204,
11.9695374830877));
#62942=CARTESIAN_POINT('Ctrl Pts',(-0.368076777863108,-0.319434907277163,
11.903074296202));
#62943=CARTESIAN_POINT('Ctrl Pts',(-0.340280761436702,-0.158333333333334,
11.8652579327567));
#62944=CARTESIAN_POINT('Ctrl Pts',(-0.309565682256709,0.158333333333336,
11.8673854677189));
#62945=CARTESIAN_POINT('Ctrl Pts',(-0.305791634384979,0.31943490727717,
11.9074118717088));
#62946=CARTESIAN_POINT('Ctrl Pts',(-0.281711831347124,0.636309800095213,
11.9780406361937));
#62947=CARTESIAN_POINT('Ctrl Pts',(-0.276359383968067,0.79477268400085,
12.0448633886902));
#62948=CARTESIAN_POINT('Ctrl Pts',(-0.234015232478537,1.06847604194778,
12.1074058962497));
#62949=CARTESIAN_POINT('Ctrl Pts',(-0.20977922135297,1.18514270861703,12.1282961333338));
#62950=CARTESIAN_POINT('Ctrl Pts',(-0.179636413276436,1.30000000000776,
12.1430042734075));
#62951=CARTESIAN_POINT('Ctrl Pts',(-0.424476296754516,-1.30000000000268,
12.1421342910495));
#62952=CARTESIAN_POINT('Ctrl Pts',(-0.440665495397502,-1.1851427086136,
12.1299569524641));
#62953=CARTESIAN_POINT('Ctrl Pts',(-0.448240048525547,-1.06847604194604,
12.111403173544));
#62954=CARTESIAN_POINT('Ctrl Pts',(-0.445837227042061,-0.794772684000862,
12.0538093797921));
#62955=CARTESIAN_POINT('Ctrl Pts',(-0.417803733610112,-0.636309800095205,
11.9893325638084));
#62956=CARTESIAN_POINT('Ctrl Pts',(-0.380369801383896,-0.319434907277163,
11.9231559217953));
#62957=CARTESIAN_POINT('Ctrl Pts',(-0.351121243067043,-0.158333333333334,
11.8847308731295));
#62958=CARTESIAN_POINT('Ctrl Pts',(-0.319894625120041,0.158333333333336,
11.8869907516665));
#62959=CARTESIAN_POINT('Ctrl Pts',(-0.316797578034367,0.319434907277171,
11.9278148839816));
#62960=CARTESIAN_POINT('Ctrl Pts',(-0.292904434770781,0.636309800095215,
11.9983111850674));
#62961=CARTESIAN_POINT('Ctrl Pts',(-0.288335254952031,0.794772684000851,
12.0655099666861));
#62962=CARTESIAN_POINT('Ctrl Pts',(-0.24449397264818,1.06847604194779,12.1252672188602));
#62963=CARTESIAN_POINT('Ctrl Pts',(-0.219109615872915,1.18514270861704,
12.1442784384785));
#62964=CARTESIAN_POINT('Ctrl Pts',(-0.187318168952349,1.30000000000776,
12.1564341774732));
#62965=CARTESIAN_POINT('Ctrl Pts',(-0.431265933106911,-1.30000000000268,
12.151098725605));
#62966=CARTESIAN_POINT('Ctrl Pts',(-0.449096337968213,-1.1851427086136,
12.1405654754374));
#62967=CARTESIAN_POINT('Ctrl Pts',(-0.457725079498785,-1.06847604194604,
12.1232568494019));
#62968=CARTESIAN_POINT('Ctrl Pts',(-0.456401515527817,-0.794772684000862,
12.0676179870174));
#62969=CARTESIAN_POINT('Ctrl Pts',(-0.426858480497729,-0.636309800095204,
12.0031829395948));
#62970=CARTESIAN_POINT('Ctrl Pts',(-0.38885614998925,-0.319434907277163,
11.9372443662456));
#62971=CARTESIAN_POINT('Ctrl Pts',(-0.359466334516699,-0.158333333333334,
11.8981754071227));
#62972=CARTESIAN_POINT('Ctrl Pts',(-0.327998948950437,0.158333333333336,
11.9005014725806));
#62973=CARTESIAN_POINT('Ctrl Pts',(-0.325009471962342,0.319434907277171,
11.9419757366776));
#62974=CARTESIAN_POINT('Ctrl Pts',(-0.30077249248368,0.636309800095215,
12.0124909326934));
#62975=CARTESIAN_POINT('Ctrl Pts',(-0.29612913799147,0.794772684000851,
12.0800924747781));
#62976=CARTESIAN_POINT('Ctrl Pts',(-0.251185627287519,1.06847604194779,
12.1379133478779));
#62977=CARTESIAN_POINT('Ctrl Pts',(-0.225129779128529,1.18514270861704,
12.1555798121165));
#62978=CARTESIAN_POINT('Ctrl Pts',(-0.192472463273335,1.30000000000776,
12.165884227103));
#62979=CARTESIAN_POINT('Ctrl Pts',(-0.434502644741001,-1.30000000000268,
12.1556249880944));
#62980=CARTESIAN_POINT('Ctrl Pts',(-0.452983313731051,-1.1851427086136,
12.1459617586608));
#62981=CARTESIAN_POINT('Ctrl Pts',(-0.462066356594455,-1.06847604194604,
12.1292962264643));
#62982=CARTESIAN_POINT('Ctrl Pts',(-0.461339606324205,-0.794772684000861,
12.0746187929737));
#62983=CARTESIAN_POINT('Ctrl Pts',(-0.431579525689312,-0.636309800095204,
12.010054557842));
#62984=CARTESIAN_POINT('Ctrl Pts',(-0.393350922373833,-0.319434907277162,
11.9442162999102));
#62985=CARTESIAN_POINT('Ctrl Pts',(-0.363480148592282,-0.158333333333334,
11.9049342616725));
#62986=CARTESIAN_POINT('Ctrl Pts',(-0.331875952022848,0.158333333333336,
11.9072995234825));
#62987=CARTESIAN_POINT('Ctrl Pts',(-0.329176263507277,0.319434907277171,
11.9490383339075));
#62988=CARTESIAN_POINT('Ctrl Pts',(-0.304997607702349,0.636309800095214,
12.0195080597917));
#62989=CARTESIAN_POINT('Ctrl Pts',(-0.30059676410946,0.79477268400085,12.0872480075864));
#62990=CARTESIAN_POINT('Ctrl Pts',(-0.255019206798925,1.06847604194779,
12.1441198649727));
#62991=CARTESIAN_POINT('Ctrl Pts',(-0.228496396831367,1.18514270861704,
12.1611441312157));
#62992=CARTESIAN_POINT('Ctrl Pts',(-0.195179612641289,1.30000000000776,
12.1705749439487));
#62993=CARTESIAN_POINT('Ctrl Pts',(-0.436112354604507,-1.30000000000268,
12.1578902342253));
#62994=CARTESIAN_POINT('Ctrl Pts',(-0.45490880513389,-1.1851427086136,12.1486645668709));
#62995=CARTESIAN_POINT('Ctrl Pts',(-0.46421605190099,-1.06847604194604,
12.132321362437));
#62996=CARTESIAN_POINT('Ctrl Pts',(-0.463795694841754,-0.794772684000861,
12.0781223562358));
#62997=CARTESIAN_POINT('Ctrl Pts',(-0.433965073693174,-0.636309800095204,
12.0134829209234));
#62998=CARTESIAN_POINT('Ctrl Pts',(-0.395631299550042,-0.319434907277163,
11.9476926447746));
#62999=CARTESIAN_POINT('Ctrl Pts',(-0.36549533649341,-0.158333333333334,
11.9083108979011));
#63000=CARTESIAN_POINT('Ctrl Pts',(-0.333823806975698,0.158333333333336,
11.9106958437498));
#63001=CARTESIAN_POINT('Ctrl Pts',(-0.331283738001294,0.319434907277172,
11.9525632339281));
#63002=CARTESIAN_POINT('Ctrl Pts',(-0.30715098623571,0.636309800095215,
12.0230063595812));
#63003=CARTESIAN_POINT('Ctrl Pts',(-0.302895353172418,0.794772684000851,
12.0908100086447));
#63004=CARTESIAN_POINT('Ctrl Pts',(-0.256990821320803,1.06847604194779,
12.1472098458578));
#63005=CARTESIAN_POINT('Ctrl Pts',(-0.230221724585517,1.18514270861704,
12.1639160882153));
#63006=CARTESIAN_POINT('Ctrl Pts',(-0.196553902023217,1.30000000000776,
12.1729151732204));
#63007=CARTESIAN_POINT('Ctrl Pts',(-0.437025956946848,-1.30000000000268,
12.1591863243717));
#63008=CARTESIAN_POINT('Ctrl Pts',(-0.455997165561016,-1.1851427086136,
12.1502122862774));
#63009=CARTESIAN_POINT('Ctrl Pts',(-0.465430235748078,-1.06847604194604,
12.1340539182948));
#63010=CARTESIAN_POINT('Ctrl Pts',(-0.465187507094752,-0.794772684000861,
12.0801276165228));
#63011=CARTESIAN_POINT('Ctrl Pts',(-0.435335675416772,-0.636309800095204,
12.0154399566702));
#63012=CARTESIAN_POINT('Ctrl Pts',(-0.396944310444561,-0.319434907277162,
11.9496763405232));
#63013=CARTESIAN_POINT('Ctrl Pts',(-0.36664263106812,-0.158333333333334,
11.9102413513394));
#63014=CARTESIAN_POINT('Ctrl Pts',(-0.334932443849119,0.158333333333336,
11.9126376435904));
#63015=CARTESIAN_POINT('Ctrl Pts',(-0.332492095751833,0.319434907277172,
11.954576306481));
#63016=CARTESIAN_POINT('Ctrl Pts',(-0.308393876872099,0.636309800095215,
12.0250022691105));
#63017=CARTESIAN_POINT('Ctrl Pts',(-0.304231219116808,0.79477268400085,
12.092840125262));
#63018=CARTESIAN_POINT('Ctrl Pts',(-0.25813661299071,1.06847604194779,12.1489710072257));
#63019=CARTESIAN_POINT('Ctrl Pts',(-0.231221908265117,1.18514270861704,
12.1654966449073));
#63020=CARTESIAN_POINT('Ctrl Pts',(-0.19734514583268,1.30000000000776,12.1742509413223));
#63021=CARTESIAN_POINT('Ctrl Pts',(-0.444794417751137,-1.30000000000268,
12.1702019182047));
#63022=CARTESIAN_POINT('Ctrl Pts',(-0.46522928698987,-1.1851427086136,12.1633718897678));
#63023=CARTESIAN_POINT('Ctrl Pts',(-0.475723958401096,-1.06847604194604,
12.1487861342615));
#63024=CARTESIAN_POINT('Ctrl Pts',(-0.477004903301544,-0.794772684000861,
12.0971728401138));
#63025=CARTESIAN_POINT('Ctrl Pts',(-0.447039629478921,-0.636309800095204,
12.0320561788573));
#63026=CARTESIAN_POINT('Ctrl Pts',(-0.40819871638579,-0.319434907277163,
11.9665085734518));
#63027=CARTESIAN_POINT('Ctrl Pts',(-0.376500881569381,-0.158333333333334,
11.9266191611378));
#63028=CARTESIAN_POINT('Ctrl Pts',(-0.344452505120339,0.158333333333336,
11.9291155053812));
#63029=CARTESIAN_POINT('Ctrl Pts',(-0.342808124805955,0.319434907277171,
11.9716738798763));
#63030=CARTESIAN_POINT('Ctrl Pts',(-0.319004258867317,0.636309800095214,
12.041954748453));
#63031=CARTESIAN_POINT('Ctrl Pts',(-0.315687596474742,0.79477268400085,
12.1100686400152));
#63032=CARTESIAN_POINT('Ctrl Pts',(-0.267989187339546,1.06847604194779,
12.1639125004961));
#63033=CARTESIAN_POINT('Ctrl Pts',(-0.239833641747303,1.18514270861704,
12.1789051904198));
#63034=CARTESIAN_POINT('Ctrl Pts',(-0.204169424477457,1.30000000000776,
12.1855835581765));
#63035=CARTESIAN_POINT('Ctrl Pts',(-0.460499827063455,-1.30000000000266,
12.1909882378324));
#63036=CARTESIAN_POINT('Ctrl Pts',(-0.484682298294522,-1.18514270861358,
12.1879667082804));
#63037=CARTESIAN_POINT('Ctrl Pts',(-0.497681648841877,-1.06847604194603,
12.1762391098647));
#63038=CARTESIAN_POINT('Ctrl Pts',(-0.501877503162414,-0.794772684000854,
12.1290332507087));
#63039=CARTESIAN_POINT('Ctrl Pts',(-0.46943057625706,-0.636309800095199,
12.0637512065799));
#63040=CARTESIAN_POINT('Ctrl Pts',(-0.429385621777131,-0.319434907277161,
11.9987349348556));
#63041=CARTESIAN_POINT('Ctrl Pts',(-0.396387340540971,-0.158333333333332,
11.9576216144592));
#63042=CARTESIAN_POINT('Ctrl Pts',(-0.363836289262359,0.158333333333334,
11.9602735413555));
#63043=CARTESIAN_POINT('Ctrl Pts',(-0.363378403513772,0.319434907277162,
12.0041009411279));
#63044=CARTESIAN_POINT('Ctrl Pts',(-0.338962865815543,0.636309800095203,
12.0743923968692));
#63045=CARTESIAN_POINT('Ctrl Pts',(-0.334838814901272,0.794772684000845,
12.1436020444614));
#63046=CARTESIAN_POINT('Ctrl Pts',(-0.284554381841157,1.06847604194778,
12.1929991429715));
#63047=CARTESIAN_POINT('Ctrl Pts',(-0.254927105241685,1.18514270861703,
12.2048737624313));
#63048=CARTESIAN_POINT('Ctrl Pts',(-0.217438819892861,1.30000000000775,
12.2072408277485));
#63049=CARTESIAN_POINT('Ctrl Pts',(-0.475851704605936,-1.30000000000266,
12.211451484628));
#63050=CARTESIAN_POINT('Ctrl Pts',(-0.503305113781325,-1.18514270861358,
12.2122832473818));
#63051=CARTESIAN_POINT('Ctrl Pts',(-0.518587456938927,-1.06847604194603,
12.2034113791443));
#63052=CARTESIAN_POINT('Ctrl Pts',(-0.525775129540728,-0.794772684000851,
12.1604982599099));
#63053=CARTESIAN_POINT('Ctrl Pts',(-0.492061752143856,-0.636309800095197,
12.0947271819335));
#63054=CARTESIAN_POINT('Ctrl Pts',(-0.451176432830116,-0.319434907277159,
12.0301447643824));
#63055=CARTESIAN_POINT('Ctrl Pts',(-0.41653030333555,-0.158333333333332,
11.9879440782691));
#63056=CARTESIAN_POINT('Ctrl Pts',(-0.38323276776461,0.158333333333334,
11.9908254839733));
#63057=CARTESIAN_POINT('Ctrl Pts',(-0.383201773569385,0.319434907277167,
12.0360862285271));
#63058=CARTESIAN_POINT('Ctrl Pts',(-0.359072532091704,0.636309800095206,
12.1061739592688));
#63059=CARTESIAN_POINT('Ctrl Pts',(-0.357294751063013,0.79477268400084,
12.1757050010453));
#63060=CARTESIAN_POINT('Ctrl Pts',(-0.303818465806733,1.06847604194777,
12.2208554698369));
#63061=CARTESIAN_POINT('Ctrl Pts',(-0.271622642081085,1.18514270861702,
12.2299142783607));
#63062=CARTESIAN_POINT('Ctrl Pts',(-0.230378897025869,1.30000000000775,
12.2284879304579));
#63063=CARTESIAN_POINT('Ctrl Pts',(-0.483946399133603,-1.30000000000266,
12.2215611275524));
#63064=CARTESIAN_POINT('Ctrl Pts',(-0.512888765856687,-1.18514270861358,
12.2243528792004));
#63065=CARTESIAN_POINT('Ctrl Pts',(-0.529237518131319,-1.06847604194603,
12.2169241430307));
#63066=CARTESIAN_POINT('Ctrl Pts',(-0.537912637722502,-0.794772684000851,
12.1761509049044));
#63067=CARTESIAN_POINT('Ctrl Pts',(-0.503949232631998,-0.636309800095197,
12.1100262039146));
#63068=CARTESIAN_POINT('Ctrl Pts',(-0.462594679683807,-0.319434907277159,
12.0456777212677));
#63069=CARTESIAN_POINT('Ctrl Pts',(-0.426715573255357,-0.158333333333332,
12.0030579137075));
#63070=CARTESIAN_POINT('Ctrl Pts',(-0.392969830593602,0.158333333333334,
12.0060803363164));
#63071=CARTESIAN_POINT('Ctrl Pts',(-0.393579787166861,0.319434907277167,
12.0519414879776));
#63072=CARTESIAN_POINT('Ctrl Pts',(-0.369299762851234,0.636309800095206,
12.1220005005405));
#63073=CARTESIAN_POINT('Ctrl Pts',(-0.367561330758702,0.79477268400084,
12.1919695316153));
#63074=CARTESIAN_POINT('Ctrl Pts',(-0.312674005334915,1.06847604194777,
12.2349707346061));
#63075=CARTESIAN_POINT('Ctrl Pts',(-0.279563873100157,1.18514270861702,
12.2425436138999));
#63076=CARTESIAN_POINT('Ctrl Pts',(-0.237102298031049,1.30000000000775,
12.239075745064));
#63077=CARTESIAN_POINT('Origin',(0.,-0.926917420765551,7.2));
#63078=CARTESIAN_POINT('Origin',(0.,-0.653834841531101,7.2));
#63079=CARTESIAN_POINT('Origin',(0.,-1.2,7.2));
#63080=CARTESIAN_POINT('Origin',(0.,0.,7.2));
#63081=CARTESIAN_POINT('Origin',(0.,-1.25,7.2));
#86395=UNCERTAINTY_MEASURE_WITH_UNIT(LENGTH_MEASURE(0.001),#86430,
'DISTANCE_ACCURACY_VALUE',
'Maximum model space distance between geometric entities at asserted c
onnectivities');
#86409=UNCERTAINTY_MEASURE_WITH_UNIT(LENGTH_MEASURE(0.001),#86430,
'DISTANCE_ACCURACY_VALUE',
'Maximum model space distance between geometric entities at asserted c
onnectivities');
#86415=(
GEOMETRIC_REPRESENTATION_CONTEXT(3)
GLOBAL_UNCERTAINTY_ASSIGNED_CONTEXT((#86395))
GLOBAL_UNIT_ASSIGNED_CONTEXT((#86430,#86432,#86433))
REPRESENTATION_CONTEXT('','3D')
);
#86429=(
GEOMETRIC_REPRESENTATION_CONTEXT(3)
GLOBAL_UNCERTAINTY_ASSIGNED_CONTEXT((#86409))
GLOBAL_UNIT_ASSIGNED_CONTEXT((#86430,#86432,#86433))
REPRESENTATION_CONTEXT('','3D')
);
#86430=(
LENGTH_UNIT()
NAMED_UNIT(*)
SI_UNIT(.CENTI.,.METRE.)
);
#86432=(
NAMED_UNIT(*)
PLANE_ANGLE_UNIT()
SI_UNIT($,.RADIAN.)
);
#86433=(
NAMED_UNIT(*)
SI_UNIT($,.STERADIAN.)
SOLID_ANGLE_UNIT()
);
#86439=SHAPE_DEFINITION_REPRESENTATION(#86458,#86506);
#86458=PRODUCT_DEFINITION_SHAPE('',$,#86526);
#86506=SHAPE_REPRESENTATION('',(#16477),#86415);
#86520=PRODUCT_DEFINITION_CONTEXT('part definition',#86579,'design');
#86526=PRODUCT_DEFINITION('Bronze Worm Wheel Ring z30',
'Bronze Worm Wheel Ring z30',#86545,#86520);
#86545=PRODUCT_DEFINITION_FORMATION('',$,#86586);
#86579=APPLICATION_CONTEXT(
'Core Data for Automotive Mechanical Design Process');
#86580=PRODUCT_CONTEXT('part definition',#86579,'mechanical');
#86586=PRODUCT('Bronze Worm Wheel Ring z30',
'Bronze Worm Wheel Ring z30',$,(#86580));
#86605=PRESENTATION_STYLE_ASSIGNMENT((#86623));
#86623=SURFACE_STYLE_USAGE(.BOTH.,#86641);
#86641=SURFACE_SIDE_STYLE('',(#86659));
#86659=SURFACE_STYLE_FILL_AREA(#86677);
#86677=FILL_AREA_STYLE('Opaque(214,178,102)',(#86695));
#86695=FILL_AREA_STYLE_COLOUR('Opaque(214,178,102)',#86713);
#86713=COLOUR_RGB('Opaque(214,178,102)', 0.72549020, 0.75294118, 0.79215686);
ENDSEC;
END-ISO-10303-21;
